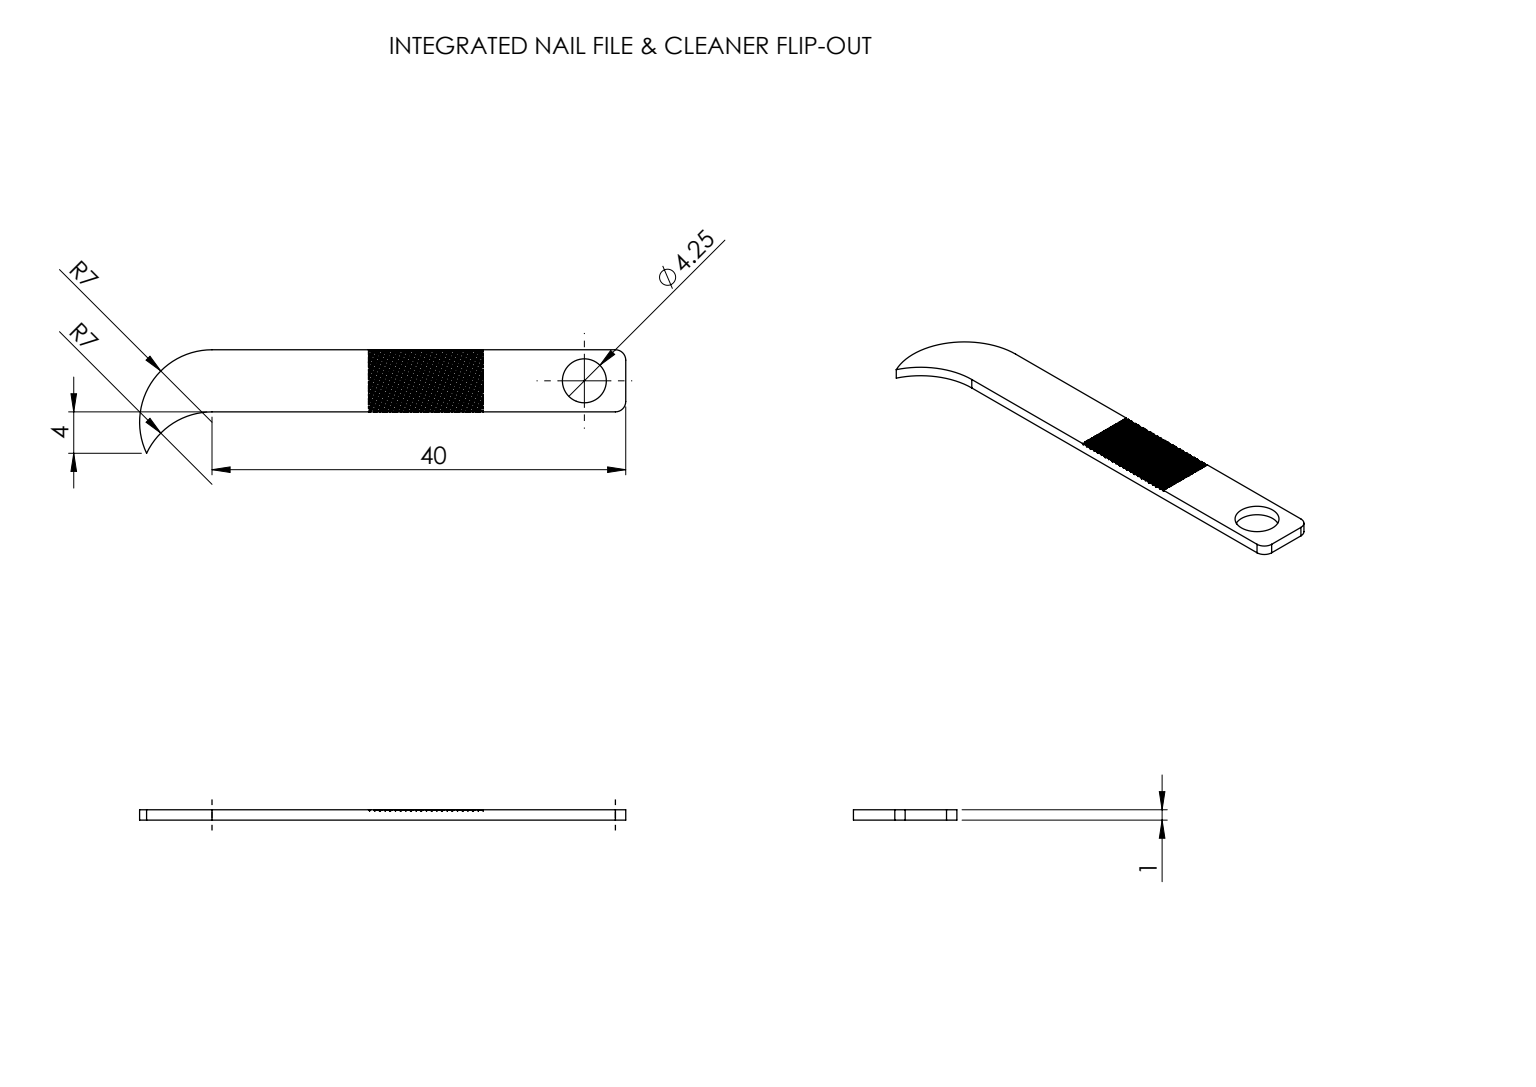
ISO-10303-21;
HEADER;
FILE_DESCRIPTION (('STEP AP214'),
    '1' );
FILE_NAME ('Integrated Nail File & Cleaner Flip-Out.step',
    '2026-09-30T04:43:20',
    ( '' ),
    ( '' ),
    'SwSTEP 2.0',
    'SolidWorks 2026',
    '' );
FILE_SCHEMA (( 'AUTOMOTIVE_DESIGN' ));
ENDSEC;

DATA;
#1=LINE ( 'NONE', #25573, #52192 ) ;
#2=VERTEX_POINT ( 'NONE', #10749 ) ;
#5=EDGE_CURVE ( 'NONE', #33225, #52332, #37701, .T. ) ;
#6=ORIENTED_EDGE ( 'NONE', *, *, #640, .F. ) ;
#7=FACE_OUTER_BOUND ( 'NONE', #50203, .T. ) ;
#8=ORIENTED_EDGE ( 'NONE', *, *, #49782, .T. ) ;
#9=DIRECTION ( 'NONE',  ( 0.7660212471507180654, -0.6427876096865404731, 0.005961354470445141482 ) ) ;
#10=EDGE_CURVE ( 'NONE', #34917, #49361, #53883, .T. ) ;
#11=ORIENTED_EDGE ( 'NONE', *, *, #22264, .F. ) ;
#12=ORIENTED_EDGE ( 'NONE', *, *, #56053, .T. ) ;
#13=ORIENTED_EDGE ( 'NONE', *, *, #9607, .F. ) ;
#14=DIRECTION ( 'NONE',  ( -0.6427681459581293666, -0.7660444431189770143, -0.005002170337467561935 ) ) ;
#15=CARTESIAN_POINT ( 'NONE',  ( -14.94838282604900748, -0.1191753592594197858, 2.588085963191248506 ) ) ;
#16=FACE_OUTER_BOUND ( 'NONE', #22473, .T. ) ;
#17=CARTESIAN_POINT ( 'NONE',  ( -15.43471928309396013, -0.1191753592594189115, 4.430961529461709070 ) ) ;
#19=ORIENTED_EDGE ( 'NONE', *, *, #1841, .F. ) ;
#20=ORIENTED_EDGE ( 'NONE', *, *, #40291, .F. ) ;
#21=CARTESIAN_POINT ( 'NONE',  ( -27.06630483948590893, -0.1191753592594197858, 7.295098399573937797 ) ) ;
#22=EDGE_LOOP ( 'NONE', ( #47630, #41472, #34640 ) ) ;
#23=PLANE ( 'NONE',  #10320 ) ;
#24=ORIENTED_EDGE ( 'NONE', *, *, #10341, .T. ) ;
#25=LINE ( 'NONE', #55156, #19677 ) ;
#26=FACE_OUTER_BOUND ( 'NONE', #52687, .T. ) ;
#28=EDGE_LOOP ( 'NONE', ( #23520, #5098, #48877, #45921 ) ) ;
#29=DIRECTION ( 'NONE',  ( -0.005961354470445682716, -0.6427876096865404731, 0.7660212471507180654 ) ) ;
#30=EDGE_CURVE ( 'NONE', #53080, #21477, #45939, .T. ) ;
#31=VERTEX_POINT ( 'NONE', #49893 ) ;
#32=AXIS2_PLACEMENT_3D ( 'NONE', #18822, #46039, #24446 ) ;
#33=CARTESIAN_POINT ( 'NONE',  ( -8.975993561185934055, -0.1191753592594197858, 10.41700724906143982 ) ) ;
#34=EDGE_LOOP ( 'NONE', ( #54000, #22369, #27701, #44259 ) ) ;
#35=CARTESIAN_POINT ( 'NONE',  ( -12.70458494993575194, -0.1191753592594197858, 11.86531876794841978 ) ) ;
#36=FACE_OUTER_BOUND ( 'NONE', #31619, .T. ) ;
#37=CARTESIAN_POINT ( 'NONE',  ( -13.73672976910459909, 0.000000000000000000, 12.22661844811216270 ) ) ;
#38=ORIENTED_EDGE ( 'NONE', *, *, #21938, .F. ) ;
#39=CARTESIAN_POINT ( 'NONE',  ( -16.82003048110239973, -0.1191753592594181482, 3.315097473835892039 ) ) ;
#40=CARTESIAN_POINT ( 'NONE',  ( -17.38829393498713571, 0.000000000000000000, 3.777097248297537124 ) ) ;
#41=DIRECTION ( 'NONE',  ( 0.007781995580012663651, -3.146120232559066537E-19, -0.9999697198139514409 ) ) ;
#42=CARTESIAN_POINT ( 'NONE',  ( -4.289188282875421088, -6.206962462949310755, 4.884439966179827231 ) ) ;
#43=CARTESIAN_POINT ( 'NONE',  ( -6.343177736738851102, -8.196582280829671774, 5.682279223835847937 ) ) ;
#44=LINE ( 'NONE', #33333, #46041 ) ;
#45=EDGE_CURVE ( 'NONE', #30649, #39352, #46465, .T. ) ;
#46=CARTESIAN_POINT ( 'NONE',  ( -17.46532115785441519, 0.000000000000000000, 13.67492996699914265 ) ) ;
#47=ORIENTED_EDGE ( 'NONE', *, *, #3666, .T. ) ;
#48=CARTESIAN_POINT ( 'NONE',  ( -10.21144203228149117, 0.000000000000000000, 2.894278973455366444 ) ) ;
#49=FACE_OUTER_BOUND ( 'NONE', #34512, .T. ) ;
#50=DIRECTION ( 'NONE',  ( -0.5449076811759708816, 0.6444004775717707689, 0.5364919789714475140 ) ) ;
#51=ORIENTED_EDGE ( 'NONE', *, *, #37599, .T. ) ;
#52=CARTESIAN_POINT ( 'NONE',  ( -19.46232870854519703, -3.756034771668159689, 10.40605410012864773 ) ) ;
#53=CARTESIAN_POINT ( 'NONE',  ( -14.22677752833734566, -0.3560938001956537868, 2.792505858709713795 ) ) ;
#54=ORIENTED_EDGE ( 'NONE', *, *, #55093, .T. ) ;
#55=DIRECTION ( 'NONE',  ( -0.005002170337468016433, -0.7660444431189770143, 0.6427681459581293666 ) ) ;
#56=AXIS2_PLACEMENT_3D ( 'NONE', #16443, #12198, #42577 ) ;
#57=EDGE_CURVE ( 'NONE', #19141, #38385, #32336, .T. ) ;
#58=LINE ( 'NONE', #52599, #10348 ) ;
#59=DIRECTION ( 'NONE',  ( 0.7660212471507180654, -0.6427876096865404731, 0.005961354470445141482 ) ) ;
#60=ADVANCED_FACE ( 'NONE', ( #15818 ), #6753, .F. ) ;
#62=ORIENTED_EDGE ( 'NONE', *, *, #8095, .T. ) ;
#64=PLANE ( 'NONE',  #40295 ) ;
#65=CARTESIAN_POINT ( 'NONE',  ( 2.072287782118878319, 0.000000000000000000, -2.950529333540147015 ) ) ;
#66=CARTESIAN_POINT ( 'NONE',  ( -10.20856797877621069, 0.000000000000000000, 2.524969270197602089 ) ) ;
#67=LINE ( 'NONE', #34732, #24784 ) ;
#68=EDGE_CURVE ( 'NONE', #2840, #34483, #50479, .T. ) ;
#69=LINE ( 'NONE', #17405, #45540 ) ;
#70=VECTOR ( 'NONE', #21292, 999.9999999999998863 ) ;
#71=FACE_OUTER_BOUND ( 'NONE', #956, .T. ) ;
#72=ORIENTED_EDGE ( 'NONE', *, *, #35043, .F. ) ;
#73=DIRECTION ( 'NONE',  ( -0.6427681459581293666, -0.7660444431189770143, -0.005002170337467561935 ) ) ;
#74=VECTOR ( 'NONE', #36543, 999.9999999999998863 ) ;
#75=ADVANCED_FACE ( 'NONE', ( #45360 ), #6472, .F. ) ;
#76=PLANE ( 'NONE',  #14275 ) ;
#77=EDGE_LOOP ( 'NONE', ( #29388, #6905, #15789, #43672 ) ) ;
#78=LINE ( 'NONE', #17411, #16572 ) ;
#79=LINE ( 'NONE', #52063, #49503 ) ;
#80=DIRECTION ( 'NONE',  ( 0.005002170337468016433, -0.7660444431189770143, -0.6427681459581293666 ) ) ;
#81=ORIENTED_EDGE ( 'NONE', *, *, #39049, .F. ) ;
#82=FACE_OUTER_BOUND ( 'NONE', #1972, .T. ) ;
#83=VERTEX_POINT ( 'NONE', #15002 ) ;
#84=ORIENTED_EDGE ( 'NONE', *, *, #47098, .T. ) ;
#85=ORIENTED_EDGE ( 'NONE', *, *, #23256, .T. ) ;
#86=ORIENTED_EDGE ( 'NONE', *, *, #47911, .T. ) ;
#87=DIRECTION ( 'NONE',  ( 0.005002170337468016433, -0.7660444431189770143, -0.6427681459581293666 ) ) ;
#88=ORIENTED_EDGE ( 'NONE', *, *, #42803, .T. ) ;
#90=DIRECTION ( 'NONE',  ( -0.5364919789714478471, 0.6444004775717705469, -0.5449076811759709926 ) ) ;
#91=AXIS2_PLACEMENT_3D ( 'NONE', #49933, #23822, #53928 ) ;
#92=VECTOR ( 'NONE', #28630, 1000.000000000000227 ) ;
#93=VERTEX_POINT ( 'NONE', #7584 ) ;
#94=CARTESIAN_POINT ( 'NONE',  ( -17.93139508144814442, 0.000000000000000000, 13.85596890686001537 ) ) ;
#95=ORIENTED_EDGE ( 'NONE', *, *, #27439, .T. ) ;
#96=CARTESIAN_POINT ( 'NONE',  ( -15.04104892662381054, -1.327505506330656670, 2.681420940547515563 ) ) ;
#97=EDGE_CURVE ( 'NONE', #51394, #16631, #45637, .T. ) ;
#98=VERTEX_POINT ( 'NONE', #19810 ) ;
#99=DIRECTION ( 'NONE',  ( -0.5449076811759708816, 0.6444004775717707689, 0.5364919789714475140 ) ) ;
#100=DIRECTION ( 'NONE',  ( 0.5449076811759707706, 0.6444004775717708799, -0.5364919789714476250 ) ) ;
#101=EDGE_CURVE ( 'NONE', #33893, #38385, #37132, .T. ) ;
#102=DIRECTION ( 'NONE',  ( 0.6427681459581294776, -0.7660444431189769032, 0.005002170337467562802 ) ) ;
#103=PLANE ( 'NONE',  #32324 ) ;
#104=DIRECTION ( 'NONE',  ( 0.9999697198139515519, 0.000000000000000000, 0.007781995580013368816 ) ) ;
#105=ORIENTED_EDGE ( 'NONE', *, *, #27186, .T. ) ;
#107=EDGE_CURVE ( 'NONE', #29873, #51521, #8427, .T. ) ;
#108=ADVANCED_FACE ( 'NONE', ( #21512 ), #30012, .F. ) ;
#109=ORIENTED_EDGE ( 'NONE', *, *, #25096, .F. ) ;
#110=DIRECTION ( 'NONE',  ( 0.005961354470445682716, -0.6427876096865404731, -0.7660212471507180654 ) ) ;
#111=PLANE ( 'NONE',  #41200 ) ;
#112=AXIS2_PLACEMENT_3D ( 'NONE', #46198, #6762, #45366 ) ;
#113=DIRECTION ( 'NONE',  ( 0.007781995580012663651, -3.146120232559066537E-19, -0.9999697198139514409 ) ) ;
#114=DIRECTION ( 'NONE',  ( -0.7660212471507179544, -0.6427876096865405842, -0.005961354470445141482 ) ) ;
#115=CARTESIAN_POINT ( 'NONE',  ( -12.13851405436063047, 0.000000000000000000, 11.68505802764555135 ) ) ;
#116=CARTESIAN_POINT ( 'NONE',  ( -18.13769215924349965, 0.000000000000000000, 6.356589746681873265 ) ) ;
#117=ORIENTED_EDGE ( 'NONE', *, *, #25709, .T. ) ;
#118=LINE ( 'NONE', #12391, #16607 ) ;
#119=CARTESIAN_POINT ( 'NONE',  ( -17.52554100038571860, -1.489407457353157049, 5.933818405385602013 ) ) ;
#120=ORIENTED_EDGE ( 'NONE', *, *, #23665, .T. ) ;
#121=DIRECTION ( 'NONE',  ( 0.5449076811759707706, 0.6444004775717708799, -0.5364919789714476250 ) ) ;
#122=LINE ( 'NONE', #21472, #18778 ) ;
#123=ADVANCED_FACE ( 'NONE', ( #38236 ), #25209, .F. ) ;
#124=DIRECTION ( 'NONE',  ( -0.7660212471507179544, -0.6427876096865405842, -0.005961354470445141482 ) ) ;
#125=FACE_OUTER_BOUND ( 'NONE', #27340, .T. ) ;
#126=EDGE_CURVE ( 'NONE', #16128, #35650, #30301, .T. ) ;
#127=LINE ( 'NONE', #17465, #18341 ) ;
#129=EDGE_LOOP ( 'NONE', ( #42984, #52877, #43620, #27077 ) ) ;
#130=EDGE_CURVE ( 'NONE', #30420, #39913, #56138, .T. ) ;
#131=DIRECTION ( 'NONE',  ( 0.007781995580012663651, 0.000000000000000000, -0.9999697198139515519 ) ) ;
#133=DIRECTION ( 'NONE',  ( -0.5449076811759708816, 0.6444004775717707689, 0.5364919789714475140 ) ) ;
#134=AXIS2_PLACEMENT_3D ( 'NONE', #24885, #20335, #55533 ) ;
#135=EDGE_CURVE ( 'NONE', #41809, #20314, #43076, .T. ) ;
#136=AXIS2_PLACEMENT_3D ( 'NONE', #8040, #24490, #3201 ) ;
#137=DIRECTION ( 'NONE',  ( 0.9999697198139515519, 0.000000000000000000, 0.007781995580013368816 ) ) ;
#138=DIRECTION ( 'NONE',  ( 0.007781995580012663651, 0.000000000000000000, -0.9999697198139515519 ) ) ;
#139=CARTESIAN_POINT ( 'NONE',  ( -18.03530320978490664, 0.7721120973665048792, 3.662821561289850703 ) ) ;
#140=DIRECTION ( 'NONE',  ( 0.5364919789714477361, 0.6444004775717706579, 0.5449076811759711036 ) ) ;
#141=EDGE_CURVE ( 'NONE', #45048, #20126, #4465, .T. ) ;
#142=EDGE_LOOP ( 'NONE', ( #43408, #23853, #54595 ) ) ;
#143=DIRECTION ( 'NONE',  ( 0.5449076811759707706, 0.6444004775717708799, -0.5364919789714476250 ) ) ;
#144=CARTESIAN_POINT ( 'NONE',  ( -12.60458797795435615, 0.000000000000000000, 11.86609696750642229 ) ) ;
#146=ORIENTED_EDGE ( 'NONE', *, *, #35409, .F. ) ;
#147=LINE ( 'NONE', #43889, #14715 ) ;
#148=ORIENTED_EDGE ( 'NONE', *, *, #30639, .T. ) ;
#149=DIRECTION ( 'NONE',  ( 0.007781995580012663651, 0.000000000000000000, -0.9999697198139515519 ) ) ;
#150=DIRECTION ( 'NONE',  ( 0.005961354470445682716, -0.6427876096865404731, -0.7660212471507180654 ) ) ;
#151=ORIENTED_EDGE ( 'NONE', *, *, #26951, .F. ) ;
#152=AXIS2_PLACEMENT_3D ( 'NONE', #22680, #53358, #9066 ) ;
#153=ORIENTED_EDGE ( 'NONE', *, *, #46826, .T. ) ;
#154=VECTOR ( 'NONE', #54316, 999.9999999999998863 ) ;
#155=ORIENTED_EDGE ( 'NONE', *, *, #18719, .T. ) ;
#156=VERTEX_POINT ( 'NONE', #55864 ) ;
#157=ORIENTED_EDGE ( 'NONE', *, *, #3395, .T. ) ;
#158=EDGE_LOOP ( 'NONE', ( #12558, #55338, #5576, #52336 ) ) ;
#159=LINE ( 'NONE', #30004, #37792 ) ;
#160=DIRECTION ( 'NONE',  ( -0.5364919789714478471, 0.6444004775717705469, -0.5449076811759709926 ) ) ;
#161=LINE ( 'NONE', #43615, #10427 ) ;
#162=ORIENTED_EDGE ( 'NONE', *, *, #35168, .T. ) ;
#163=DIRECTION ( 'NONE',  ( 0.9999697198139515519, 0.000000000000000000, 0.007781995580013368816 ) ) ;
#164=ORIENTED_EDGE ( 'NONE', *, *, #30145, .F. ) ;
#165=VERTEX_POINT ( 'NONE', #25754 ) ;
#166=CARTESIAN_POINT ( 'NONE',  ( -28.92982233430281980, 0.000000000000000000, 7.919257187036034651 ) ) ;
#167=DIRECTION ( 'NONE',  ( 0.000000000000000000, -0.000000000000000000, -1.000000000000000000 ) ) ;
#168=PLANE ( 'NONE',  #1458 ) ;
#169=ORIENTED_EDGE ( 'NONE', *, *, #7771, .F. ) ;
#170=LINE ( 'NONE', #34552, #2862 ) ;
#171=VERTEX_POINT ( 'NONE', #17226 ) ;
#172=EDGE_CURVE ( 'NONE', #2345, #30417, #47903, .T. ) ;
#173=EDGE_CURVE ( 'NONE', #12870, #165, #47619, .T. ) ;
#174=VECTOR ( 'NONE', #52609, 999.9999999999998863 ) ;
#175=AXIS2_PLACEMENT_3D ( 'NONE', #29245, #50566, #11082 ) ;
#176=DIRECTION ( 'NONE',  ( -0.6246952433987893460, -0.7422098413412802076, 0.2426528472758542054 ) ) ;
#177=FACE_OUTER_BOUND ( 'NONE', #19384, .T. ) ;
#178=ADVANCED_FACE ( 'NONE', ( #38828 ), #34544, .F. ) ;
#179=PLANE ( 'NONE',  #54119 ) ;
#180=VECTOR ( 'NONE', #20646, 999.9999999999998863 ) ;
#181=VECTOR ( 'NONE', #8523, 999.9999999999998863 ) ;
#182=CARTESIAN_POINT ( 'NONE',  ( -13.92566315350489958, 0.000000000000000000, 2.496041976053526401 ) ) ;
#183=DIRECTION ( 'NONE',  ( 0.9999697198139515519, 0.000000000000000000, 0.007781995580013368816 ) ) ;
#184=PLANE ( 'NONE',  #4946 ) ;
#185=DIRECTION ( 'NONE',  ( 0.9999697198139515519, 0.000000000000000000, 0.007781995580013368816 ) ) ;
#187=VERTEX_POINT ( 'NONE', #9005 ) ;
#188=LINE ( 'NONE', #21229, #46462 ) ;
#189=LINE ( 'NONE', #16995, #9319 ) ;
#190=FACE_OUTER_BOUND ( 'NONE', #52164, .T. ) ;
#191=CARTESIAN_POINT ( 'NONE',  ( -10.67549210721878694, 8.288742281967422798, 0.9283501000179719131 ) ) ;
#194=DIRECTION ( 'NONE',  ( 0.000000000000000000, -0.000000000000000000, -1.000000000000000000 ) ) ;
#195=ADVANCED_FACE ( 'NONE', ( #42236 ), #20662, .F. ) ;
#196=DIRECTION ( 'NONE',  ( 0.005961354470445682716, -0.6427876096865404731, -0.7660212471507180654 ) ) ;
#197=DIRECTION ( 'NONE',  ( 0.5449076811759707706, 0.6444004775717708799, -0.5364919789714476250 ) ) ;
#199=ORIENTED_EDGE ( 'NONE', *, *, #4188, .F. ) ;
#200=ADVANCED_FACE ( 'NONE', ( #33997 ), #16371, .F. ) ;
#201=FACE_OUTER_BOUND ( 'NONE', #9129, .T. ) ;
#202=FACE_OUTER_BOUND ( 'NONE', #53678, .T. ) ;
#203=DIRECTION ( 'NONE',  ( 0.6427681459581294776, -0.7660444431189769032, 0.005002170337467562802 ) ) ;
#204=EDGE_CURVE ( 'NONE', #54577, #15326, #19532, .T. ) ;
#205=DIRECTION ( 'NONE',  ( 0.9999697198139515519, 0.000000000000000000, 0.007781995580013368816 ) ) ;
#206=CARTESIAN_POINT ( 'NONE',  ( -13.48976679171663484, 0.000000000000000000, 6.192754920399180740 ) ) ;
#207=VECTOR ( 'NONE', #19976, 1000.000000000000227 ) ;
#208=EDGE_CURVE ( 'NONE', #16268, #38932, #12121, .T. ) ;
#209=CARTESIAN_POINT ( 'NONE',  ( -15.52531589500150666, 0.000000000000000000, 3.222257248149021258 ) ) ;
#211=CARTESIAN_POINT ( 'NONE',  ( -19.32961685222932147, 0.000000000000000000, 14.39908572644263351 ) ) ;
#212=CARTESIAN_POINT ( 'NONE',  ( -17.36187534420177769, 4.333955019861509328, 10.73802165171122347 ) ) ;
#213=EDGE_CURVE ( 'NONE', #291, #19762, #47053, .T. ) ;
#214=AXIS2_PLACEMENT_3D ( 'NONE', #5223, #35051, #73 ) ;
#215=EDGE_LOOP ( 'NONE', ( #36869, #50678, #13094, #16447 ) ) ;
#216=DIRECTION ( 'NONE',  ( 0.5364919789714477361, 0.6444004775717706579, 0.5449076811759711036 ) ) ;
#217=EDGE_CURVE ( 'NONE', #7467, #3951, #3878, .T. ) ;
#218=VECTOR ( 'NONE', #12479, 1000.000000000000227 ) ;
#219=AXIS2_PLACEMENT_3D ( 'NONE', #34025, #46802, #8180 ) ;
#220=EDGE_LOOP ( 'NONE', ( #56199, #45802, #49366, #38955 ) ) ;
#221=ADVANCED_FACE ( 'NONE', ( #13537 ), #1011, .F. ) ;
#222=VECTOR ( 'NONE', #40260, 1000.000000000000227 ) ;
#223=VERTEX_POINT ( 'NONE', #1301 ) ;
#224=EDGE_LOOP ( 'NONE', ( #49282, #54509, #50774, #34578 ) ) ;
#225=AXIS2_PLACEMENT_3D ( 'NONE', #48781, #44235, #9876 ) ;
#226=ORIENTED_EDGE ( 'NONE', *, *, #56206, .F. ) ;
#227=ORIENTED_EDGE ( 'NONE', *, *, #29291, .F. ) ;
#228=CARTESIAN_POINT ( 'NONE',  ( -14.01701317841955508, 0.000000000000000000, 2.326005055450897085 ) ) ;
#229=DIRECTION ( 'NONE',  ( -0.005961354470445682716, -0.6427876096865404731, 0.7660212471507180654 ) ) ;
#230=ORIENTED_EDGE ( 'NONE', *, *, #6847, .F. ) ;
#231=ORIENTED_EDGE ( 'NONE', *, *, #14544, .F. ) ;
#232=VECTOR ( 'NONE', #3897, 1000.000000000000227 ) ;
#233=AXIS2_PLACEMENT_3D ( 'NONE', #39851, #932, #52902 ) ;
#234=LINE ( 'NONE', #25830, #10239 ) ;
#235=VERTEX_POINT ( 'NONE', #4730 ) ;
#236=CARTESIAN_POINT ( 'NONE',  ( -18.67619601524082285, 0.000000000000000000, 3.936400510096834893 ) ) ;
#238=ORIENTED_EDGE ( 'NONE', *, *, #26646, .F. ) ;
#239=FACE_OUTER_BOUND ( 'NONE', #22439, .T. ) ;
#240=AXIS2_PLACEMENT_3D ( 'NONE', #41868, #37631, #6419 ) ;
#241=EDGE_CURVE ( 'NONE', #29572, #36873, #1603, .T. ) ;
#242=ORIENTED_EDGE ( 'NONE', *, *, #47787, .F. ) ;
#243=DIRECTION ( 'NONE',  ( 0.000000000000000000, -1.000000000000000000, 0.000000000000000000 ) ) ;
#244=VECTOR ( 'NONE', #39775, 1000.000000000000114 ) ;
#245=EDGE_CURVE ( 'NONE', #18842, #26839, #48755, .T. ) ;
#246=EDGE_CURVE ( 'NONE', #931, #21351, #36247, .T. ) ;
#247=CARTESIAN_POINT ( 'NONE',  ( -13.46034487804917390, 5.305366725996514710, 1.741117822157838724 ) ) ;
#248=EDGE_LOOP ( 'NONE', ( #22673, #25406, #16303, #10944 ) ) ;
#249=PLANE ( 'NONE',  #50315 ) ;
#250=CARTESIAN_POINT ( 'NONE',  ( -14.17032429916292813, 0.000000000000000000, 8.234125069766777827 ) ) ;
#251=CARTESIAN_POINT ( 'NONE',  ( -11.20636620717317378, 0.000000000000000000, 11.32298014792380414 ) ) ;
#252=VECTOR ( 'NONE', #13641, 999.9999999999998863 ) ;
#254=CARTESIAN_POINT ( 'NONE',  ( -23.33849165029409889, 0.000000000000000000, 5.946783852668351855 ) ) ;
#255=ORIENTED_EDGE ( 'NONE', *, *, #35065, .T. ) ;
#256=VECTOR ( 'NONE', #15844, 1000.000000000000227 ) ;
#257=AXIS2_PLACEMENT_3D ( 'NONE', #26686, #13372, #44005 ) ;
#258=DIRECTION ( 'NONE',  ( -0.6427681459581293666, -0.7660444431189770143, -0.005002170337467561935 ) ) ;
#259=LINE ( 'NONE', #22700, #51384 ) ;
#260=DIRECTION ( 'NONE',  ( -0.9999697198139514409, -0.000000000000000000, -0.007781995580013368816 ) ) ;
#261=DIRECTION ( 'NONE',  ( -0.6427681459581293666, -0.7660444431189770143, -0.005002170337467561935 ) ) ;
#262=PLANE ( 'NONE',  #7783 ) ;
#263=CARTESIAN_POINT ( 'NONE',  ( -18.19747506107908563, 0.000000000000000000, 14.03856424583689311 ) ) ;
#264=DIRECTION ( 'NONE',  ( -0.7660212471507179544, -0.6427876096865405842, -0.005961354470445141482 ) ) ;
#265=AXIS2_PLACEMENT_3D ( 'NONE', #36413, #10611, #26789 ) ;
#266=DIRECTION ( 'NONE',  ( 0.000000000000000000, -0.000000000000000000, -1.000000000000000000 ) ) ;
#267=VECTOR ( 'NONE', #8315, 999.9999999999998863 ) ;
#268=CARTESIAN_POINT ( 'NONE',  ( -23.33771345073609638, -0.1191753592594197858, 5.846786880686956955 ) ) ;
#269=ORIENTED_EDGE ( 'NONE', *, *, #16189, .T. ) ;
#270=DIRECTION ( 'NONE',  ( -0.005002170337468016433, -0.7660444431189770143, 0.6427681459581293666 ) ) ;
#271=LINE ( 'NONE', #1112, #10920 ) ;
#272=CARTESIAN_POINT ( 'NONE',  ( 2.072287782118878319, 0.000000000000000000, -2.950529333540147015 ) ) ;
#273=CARTESIAN_POINT ( 'NONE',  ( -11.87243407472968926, 0.000000000000000000, 11.50246268866867361 ) ) ;
#274=AXIS2_PLACEMENT_3D ( 'NONE', #26963, #39157, #26121 ) ;
#275=AXIS2_PLACEMENT_3D ( 'NONE', #49131, #52299, #27016 ) ;
#276=EDGE_CURVE ( 'NONE', #2654, #52427, #22050, .T. ) ;
#277=FACE_OUTER_BOUND ( 'NONE', #5267, .T. ) ;
#278=CARTESIAN_POINT ( 'NONE',  ( -16.79925329029790149, 0.000000000000000000, 13.49544742625427496 ) ) ;
#279=ORIENTED_EDGE ( 'NONE', *, *, #9058, .T. ) ;
#281=EDGE_CURVE ( 'NONE', #14069, #52686, #39928, .T. ) ;
#282=DIRECTION ( 'NONE',  ( 0.005002170337468016433, -0.7660444431189770143, -0.6427681459581293666 ) ) ;
#283=CARTESIAN_POINT ( 'NONE',  ( -17.73140113748535285, 0.000000000000000000, 13.85752530597602039 ) ) ;
#284=ORIENTED_EDGE ( 'NONE', *, *, #29998, .F. ) ;
#285=VECTOR ( 'NONE', #53236, 1000.000000000000227 ) ;
#286=FACE_OUTER_BOUND ( 'NONE', #8165, .T. ) ;
#287=EDGE_LOOP ( 'NONE', ( #31043, #13115, #52818, #45322 ) ) ;
#288=CARTESIAN_POINT ( 'NONE',  ( -19.79569077582305070, 0.000000000000000000, 14.58012466630350445 ) ) ;
#289=EDGE_CURVE ( 'NONE', #36837, #44524, #470, .T. ) ;
#290=VECTOR ( 'NONE', #6881, 999.9999999999998863 ) ;
#291=VERTEX_POINT ( 'NONE', #9262 ) ;
#292=CARTESIAN_POINT ( 'NONE',  ( -18.44716714978218164, 2.876837460659007473, 8.768207690109344199 ) ) ;
#293=ORIENTED_EDGE ( 'NONE', *, *, #18760, .T. ) ;
#294=VERTEX_POINT ( 'NONE', #53546 ) ;
#295=ORIENTED_EDGE ( 'NONE', *, *, #8160, .T. ) ;
#296=CARTESIAN_POINT ( 'NONE',  ( -15.86710544311044302, 0.000000000000000000, 13.13336954653252953 ) ) ;
#297=VECTOR ( 'NONE', #13524, 1000.000000000000000 ) ;
#298=FACE_OUTER_BOUND ( 'NONE', #53215, .T. ) ;
#300=EDGE_CURVE ( 'NONE', #33548, #11209, #18927, .T. ) ;
#301=AXIS2_PLACEMENT_3D ( 'NONE', #8298, #21377, #55722 ) ;
#302=VECTOR ( 'NONE', #4764, 999.9999999999998863 ) ;
#303=DIRECTION ( 'NONE',  ( 0.007781995580012663651, 0.000000000000000000, -0.9999697198139515519 ) ) ;
#304=EDGE_LOOP ( 'NONE', ( #25150, #34611, #28054, #8360, #39695 ) ) ;
#305=ORIENTED_EDGE ( 'NONE', *, *, #38261, .F. ) ;
#306=EDGE_CURVE ( 'NONE', #53467, #42919, #52440, .T. ) ;
#307=VECTOR ( 'NONE', #12261, 1000.000000000000114 ) ;
#308=VERTEX_POINT ( 'NONE', #35146 ) ;
#309=VECTOR ( 'NONE', #14747, 999.9999999999998863 ) ;
#311=DIRECTION ( 'NONE',  ( 0.9999697198139515519, 0.000000000000000000, 0.007781995580013368816 ) ) ;
#312=ORIENTED_EDGE ( 'NONE', *, *, #31310, .T. ) ;
#313=DIRECTION ( 'NONE',  ( 0.000000000000000000, -0.000000000000000000, -1.000000000000000000 ) ) ;
#314=EDGE_CURVE ( 'NONE', #9163, #26799, #27158, .T. ) ;
#315=ORIENTED_EDGE ( 'NONE', *, *, #40972, .T. ) ;
#316=PLANE ( 'NONE',  #44171 ) ;
#317=LINE ( 'NONE', #31273, #54806 ) ;
#318=ORIENTED_EDGE ( 'NONE', *, *, #12951, .T. ) ;
#319=EDGE_CURVE ( 'NONE', #50963, #26160, #44464, .T. ) ;
#320=CARTESIAN_POINT ( 'NONE',  ( -27.99767448711536133, 0.000000000000000000, 7.557179307314289218 ) ) ;
#321=ORIENTED_EDGE ( 'NONE', *, *, #1045, .T. ) ;
#322=EDGE_CURVE ( 'NONE', #38023, #19674, #26588, .T. ) ;
#323=LINE ( 'NONE', #12572, #26385 ) ;
#324=VECTOR ( 'NONE', #8090, 1000.000000000000227 ) ;
#325=ORIENTED_EDGE ( 'NONE', *, *, #12524, .F. ) ;
#326=CARTESIAN_POINT ( 'NONE',  ( -20.54049170961573267, 0.000000000000000000, 4.660556269540326646 ) ) ;
#327=CARTESIAN_POINT ( 'NONE',  ( -17.33634854152196780, -0.1191753592594171213, 9.952400094065581015 ) ) ;
#328=DIRECTION ( 'NONE',  ( 0.6427681459581294776, -0.7660444431189769032, 0.005002170337467562802 ) ) ;
#329=VERTEX_POINT ( 'NONE', #5025 ) ;
#330=VECTOR ( 'NONE', #29769, 999.9999999999998863 ) ;
#331=EDGE_CURVE ( 'NONE', #20000, #39753, #13803, .T. ) ;
#332=LINE ( 'NONE', #21661, #54656 ) ;
#333=CARTESIAN_POINT ( 'NONE',  ( -17.75117697256323268, -2.298917212465658277, 7.350006499361532164 ) ) ;
#334=CARTESIAN_POINT ( 'NONE',  ( -17.36532418587302473, -0.1191753592594177458, 13.67570816655714516 ) ) ;
#335=VECTOR ( 'NONE', #1032, 999.9999999999998863 ) ;
#336=LINE ( 'NONE', #47792, #17706 ) ;
#337=LINE ( 'NONE', #39552, #37612 ) ;
#338=DIRECTION ( 'NONE',  ( 0.9999697198139515519, 0.000000000000000000, 0.007781995580013368816 ) ) ;
#340=DIRECTION ( 'NONE',  ( -0.7660212471507179544, -0.6427876096865405842, -0.005961354470445141482 ) ) ;
#341=ORIENTED_EDGE ( 'NONE', *, *, #38336, .T. ) ;
#342=CARTESIAN_POINT ( 'NONE',  ( 2.072287782118878319, 0.000000000000000000, -2.950529333540147015 ) ) ;
#343=LINE ( 'NONE', #21391, #3196 ) ;
#344=DIRECTION ( 'NONE',  ( 0.007781995580012662783, 0.000000000000000000, -0.9999697198139514409 ) ) ;
#345=VERTEX_POINT ( 'NONE', #31128 ) ;
#346=VECTOR ( 'NONE', #15392, 999.9999999999998863 ) ;
#347=DIRECTION ( 'NONE',  ( 0.7660212471507180654, -0.6427876096865404731, 0.005961354470445141482 ) ) ;
#348=FACE_OUTER_BOUND ( 'NONE', #54993, .T. ) ;
#349=VERTEX_POINT ( 'NONE', #31706 ) ;
#350=VECTOR ( 'NONE', #2759, 999.9999999999998863 ) ;
#352=DIRECTION ( 'NONE',  ( 0.5449076811759707706, 0.6444004775717708799, -0.5364919789714476250 ) ) ;
#353=DIRECTION ( 'NONE',  ( 0.7660212471507180654, -0.6427876096865404731, 0.005961354470445141482 ) ) ;
#355=ORIENTED_EDGE ( 'NONE', *, *, #29279, .T. ) ;
#356=VECTOR ( 'NONE', #10520, 1000.000000000000114 ) ;
#357=VECTOR ( 'NONE', #13768, 1000.000000000000000 ) ;
#358=ORIENTED_EDGE ( 'NONE', *, *, #4456, .T. ) ;
#359=CARTESIAN_POINT ( 'NONE',  ( -19.33878870862964305, -1.975113310420658852, 7.435271445270302593 ) ) ;
#360=DIRECTION ( 'NONE',  ( 0.007781995580012662783, 0.000000000000000000, -0.9999697198139514409 ) ) ;
#361=DIRECTION ( 'NONE',  ( -0.9999697198139514409, -0.000000000000000000, -0.007781995580013368816 ) ) ;
#362=PLANE ( 'NONE',  #37468 ) ;
#363=DIRECTION ( 'NONE',  ( 0.5449076811759707706, 0.6444004775717708799, -0.5364919789714476250 ) ) ;
#364=FACE_OUTER_BOUND ( 'NONE', #14108, .T. ) ;
#365=EDGE_CURVE ( 'NONE', #15522, #6083, #49011, .T. ) ;
#367=LINE ( 'NONE', #4924, #1109 ) ;
#368=VECTOR ( 'NONE', #37920, 1000.000000000000227 ) ;
#370=VERTEX_POINT ( 'NONE', #48452 ) ;
#371=AXIS2_PLACEMENT_3D ( 'NONE', #6600, #33303, #28757 ) ;
#372=DIRECTION ( 'NONE',  ( 0.005961354470445682716, -0.6427876096865404731, -0.7660212471507180654 ) ) ;
#374=AXIS2_PLACEMENT_3D ( 'NONE', #30248, #4416, #8373 ) ;
#375=LINE ( 'NONE', #930, #8550 ) ;
#376=EDGE_CURVE ( 'NONE', #36173, #27809, #10111, .T. ) ;
#377=ORIENTED_EDGE ( 'NONE', *, *, #20121, .F. ) ;
#378=PLANE ( 'NONE',  #3086 ) ;
#379=VECTOR ( 'NONE', #26653, 1000.000000000000114 ) ;
#380=ORIENTED_EDGE ( 'NONE', *, *, #23171, .F. ) ;
#381=EDGE_CURVE ( 'NONE', #34243, #38141, #26893, .T. ) ;
#382=ADVANCED_FACE ( 'NONE', ( #5312 ), #20295, .F. ) ;
#383=ORIENTED_EDGE ( 'NONE', *, *, #43761, .F. ) ;
#384=EDGE_LOOP ( 'NONE', ( #49839, #18862, #38770, #29467 ) ) ;
#385=ORIENTED_EDGE ( 'NONE', *, *, #20357, .F. ) ;
#386=VECTOR ( 'NONE', #38602, 999.9999999999998863 ) ;
#387=PLANE ( 'NONE',  #36628 ) ;
#388=ORIENTED_EDGE ( 'NONE', *, *, #50925, .F. ) ;
#389=CARTESIAN_POINT ( 'NONE',  ( -18.35912213213254773, 0.000000000000000000, 9.109517029665196830 ) ) ;
#390=VECTOR ( 'NONE', #55175, 999.9999999999998863 ) ;
#391=ORIENTED_EDGE ( 'NONE', *, *, #38213, .F. ) ;
#392=LINE ( 'NONE', #30530, #43118 ) ;
#393=EDGE_CURVE ( 'NONE', #50596, #19103, #2684, .T. ) ;
#394=VERTEX_POINT ( 'NONE', #27729 ) ;
#395=DIRECTION ( 'NONE',  ( 0.8531650599175527594, 0.4028455766673922356, -0.3313982828793700652 ) ) ;
#397=EDGE_CURVE ( 'NONE', #27291, #53062, #24006, .T. ) ;
#398=VECTOR ( 'NONE', #12673, 999.9999999999998863 ) ;
#399=VECTOR ( 'NONE', #24658, 1000.000000000000227 ) ;
#400=LINE ( 'NONE', #29953, #50150 ) ;
#401=LINE ( 'NONE', #38179, #16866 ) ;
#402=DIRECTION ( 'NONE',  ( -0.5449076811759708816, 0.6444004775717707689, 0.5364919789714475140 ) ) ;
#403=CARTESIAN_POINT ( 'NONE',  ( -26.13337879274045505, 0.000000000000000000, 6.833023547870798353 ) ) ;
#404=DIRECTION ( 'NONE',  ( 0.5449076811759707706, 0.6444004775717708799, -0.5364919789714476250 ) ) ;
#405=ORIENTED_EDGE ( 'NONE', *, *, #31844, .T. ) ;
#406=EDGE_CURVE ( 'NONE', #17338, #35631, #37331, .T. ) ;
#407=ORIENTED_EDGE ( 'NONE', *, *, #12412, .F. ) ;
#408=PLANE ( 'NONE',  #43098 ) ;
#409=LINE ( 'NONE', #47855, #23972 ) ;
#410=FACE_OUTER_BOUND ( 'NONE', #52245, .T. ) ;
#411=VECTOR ( 'NONE', #55065, 1000.000000000000227 ) ;
#412=ADVANCED_FACE ( 'NONE', ( #32269 ), #15751, .F. ) ;
#413=CARTESIAN_POINT ( 'NONE',  ( -11.79828090536769203, 0.000000000000000000, 1.973939673224830660 ) ) ;
#414=AXIS2_PLACEMENT_3D ( 'NONE', #46926, #25913, #21902 ) ;
#415=DIRECTION ( 'NONE',  ( 0.007781995580012662783, 0.000000000000000000, -0.9999697198139514409 ) ) ;
#416=DIRECTION ( 'NONE',  ( 0.005002170337468016433, -0.7660444431189770143, -0.6427681459581293666 ) ) ;
#417=ORIENTED_EDGE ( 'NONE', *, *, #24919, .T. ) ;
#419=DIRECTION ( 'NONE',  ( 0.007781995580012663651, -3.146120232559066537E-19, -0.9999697198139514409 ) ) ;
#420=AXIS2_PLACEMENT_3D ( 'NONE', #54266, #23873, #24706 ) ;
#421=ORIENTED_EDGE ( 'NONE', *, *, #9837, .T. ) ;
#422=DIRECTION ( 'NONE',  ( -0.7660212471507179544, -0.6427876096865405842, -0.005961354470445141482 ) ) ;
#423=CARTESIAN_POINT ( 'NONE',  ( -27.99845268667336384, -0.1191753592594197858, 7.657176279295684118 ) ) ;
#424=VECTOR ( 'NONE', #53367, 1000.000000000000227 ) ;
#425=LINE ( 'NONE', #973, #5079 ) ;
#426=FACE_OUTER_BOUND ( 'NONE', #14338, .T. ) ;
#427=CARTESIAN_POINT ( 'NONE',  ( -14.15727168602579766, 0.000000000000000000, 6.556892312772929721 ) ) ;
#428=VERTEX_POINT ( 'NONE', #28541 ) ;
#429=VECTOR ( 'NONE', #53252, 999.9999999999998863 ) ;
#430=ORIENTED_EDGE ( 'NONE', *, *, #18527, .F. ) ;
#431=AXIS2_PLACEMENT_3D ( 'NONE', #56006, #3733, #42926 ) ;
#432=CARTESIAN_POINT ( 'NONE',  ( -11.26448342554532012, -0.1191753592594185784, 5.940743548404852525 ) ) ;
#434=LINE ( 'NONE', #30827, #44226 ) ;
#435=AXIS2_PLACEMENT_3D ( 'NONE', #40606, #36325, #43706 ) ;
#436=CARTESIAN_POINT ( 'NONE',  ( -13.73672976910459909, 0.000000000000000000, 12.22661844811216270 ) ) ;
#437=DIRECTION ( 'NONE',  ( 0.6427681459581294776, -0.7660444431189769032, 0.005002170337467562802 ) ) ;
#438=EDGE_CURVE ( 'NONE', #41253, #2345, #2131, .T. ) ;
#439=DIRECTION ( 'NONE',  ( -0.5449076811759708816, 0.6444004775717707689, 0.5364919789714475140 ) ) ;
#440=CARTESIAN_POINT ( 'NONE',  ( -27.06552663992790997, 0.000000000000000000, 7.195101427592543786 ) ) ;
#441=VERTEX_POINT ( 'NONE', #46137 ) ;
#442=VECTOR ( 'NONE', #33608, 999.9999999999998863 ) ;
#443=FACE_OUTER_BOUND ( 'NONE', #30904, .T. ) ;
#444=VECTOR ( 'NONE', #34245, 1000.000000000000000 ) ;
#445=LINE ( 'NONE', #48427, #46891 ) ;
#447=EDGE_CURVE ( 'NONE', #485, #27823, #40779, .T. ) ;
#448=ORIENTED_EDGE ( 'NONE', *, *, #34618, .F. ) ;
#449=CARTESIAN_POINT ( 'NONE',  ( -16.04172443374966761, 4.495856970884011261, 2.769640905047572321 ) ) ;
#450=EDGE_LOOP ( 'NONE', ( #19965, #9347, #24938, #27730 ) ) ;
#451=DIRECTION ( 'NONE',  ( 0.9321478471874541372, 0.000000000000000000, -0.3620778797217453771 ) ) ;
#452=ADVANCED_FACE ( 'NONE', ( #1852 ), #50104, .F. ) ;
#453=ADVANCED_FACE ( 'NONE', ( #7244 ), #2428, .F. ) ;
#454=LINE ( 'NONE', #35131, #43843 ) ;
#456=ORIENTED_EDGE ( 'NONE', *, *, #13239, .F. ) ;
#457=ORIENTED_EDGE ( 'NONE', *, *, #32580, .T. ) ;
#458=EDGE_CURVE ( 'NONE', #51710, #23249, #53825, .T. ) ;
#459=VECTOR ( 'NONE', #16090, 1000.000000000000114 ) ;
#461=ORIENTED_EDGE ( 'NONE', *, *, #35316, .F. ) ;
#462=ORIENTED_EDGE ( 'NONE', *, *, #15003, .T. ) ;
#463=AXIS2_PLACEMENT_3D ( 'NONE', #24547, #54121, #23720 ) ;
#464=ORIENTED_EDGE ( 'NONE', *, *, #30689, .T. ) ;
#465=DIRECTION ( 'NONE',  ( -0.005002170337468016433, -0.7660444431189770143, 0.6427681459581293666 ) ) ;
#466=CARTESIAN_POINT ( 'NONE',  ( 2.072287782118878319, 0.000000000000000000, -2.950529333540147015 ) ) ;
#467=DIRECTION ( 'NONE',  ( 0.007781995580012663651, -3.146120232559066537E-19, -0.9999697198139514409 ) ) ;
#468=AXIS2_PLACEMENT_3D ( 'NONE', #39473, #17904, #31219 ) ;
#469=EDGE_LOOP ( 'NONE', ( #53568, #47753, #23192, #24265 ) ) ;
#470=LINE ( 'NONE', #52994, #35822 ) ;
#471=EDGE_CURVE ( 'NONE', #12574, #40953, #33382, .T. ) ;
#472=ORIENTED_EDGE ( 'NONE', *, *, #19438, .F. ) ;
#473=AXIS2_PLACEMENT_3D ( 'NONE', #21788, #43922, #34860 ) ;
#474=EDGE_LOOP ( 'NONE', ( #13344, #7979, #54982, #50764 ) ) ;
#475=EDGE_CURVE ( 'NONE', #5277, #30292, #6413, .T. ) ;
#476=AXIS2_PLACEMENT_3D ( 'NONE', #44666, #26511, #49210 ) ;
#477=AXIS2_PLACEMENT_3D ( 'NONE', #5497, #53744, #35905 ) ;
#478=CARTESIAN_POINT ( 'NONE',  ( -16.79925329029790149, 0.000000000000000000, 13.49544742625427496 ) ) ;
#479=DIRECTION ( 'NONE',  ( -0.6427681459581293666, -0.7660444431189770143, -0.005002170337467561935 ) ) ;
#480=EDGE_CURVE ( 'NONE', #29959, #40913, #28257, .T. ) ;
#481=AXIS2_PLACEMENT_3D ( 'NONE', #37816, #3148, #21324 ) ;
#482=CARTESIAN_POINT ( 'NONE',  ( -17.46532115785441519, 0.000000000000000000, 13.67492996699914265 ) ) ;
#483=ORIENTED_EDGE ( 'NONE', *, *, #47027, .F. ) ;
#485=VERTEX_POINT ( 'NONE', #6690 ) ;
#486=VECTOR ( 'NONE', #22922, 1000.000000000000000 ) ;
#487=ADVANCED_FACE ( 'NONE', ( #41340 ), #54375, .F. ) ;
#488=VECTOR ( 'NONE', #16446, 1000.000000000000227 ) ;
#489=CARTESIAN_POINT ( 'NONE',  ( -9.274408763410345813, 2.384096728371167817, 3.117008339208958034 ) ) ;
#490=FACE_OUTER_BOUND ( 'NONE', #41737, .T. ) ;
#491=AXIS2_PLACEMENT_3D ( 'NONE', #51141, #37826, #24737 ) ;
#493=AXIS2_PLACEMENT_3D ( 'NONE', #21084, #8312, #42665 ) ;
#494=DIRECTION ( 'NONE',  ( 0.007781995580012663651, -3.146120232559066537E-19, -0.9999697198139514409 ) ) ;
#497=LINE ( 'NONE', #34563, #49322 ) ;
#498=CARTESIAN_POINT ( 'NONE',  ( -16.43317633868556626, -0.1191753592594197858, 13.31363028683540151 ) ) ;
#499=ORIENTED_EDGE ( 'NONE', *, *, #29532, .F. ) ;
#500=CARTESIAN_POINT ( 'NONE',  ( -16.81190032086591302, 0.000000000000000000, 3.212244750653343583 ) ) ;
#501=LINE ( 'NONE', #50440, #2942 ) ;
#502=CARTESIAN_POINT ( 'NONE',  ( -8.129252104341238905, 0.000000000000000000, 6.065145671608219935 ) ) ;
#503=DIRECTION ( 'NONE',  ( -0.7660212471507179544, -0.6427876096865405842, -0.005961354470445141482 ) ) ;
#504=DIRECTION ( 'NONE',  ( 0.000000000000000000, -0.000000000000000000, -1.000000000000000000 ) ) ;
#505=LINE ( 'NONE', #40549, #49453 ) ;
#506=LINE ( 'NONE', #14144, #19589 ) ;
#507=AXIS2_PLACEMENT_3D ( 'NONE', #4307, #52278, #48266 ) ;
#508=LINE ( 'NONE', #12467, #14837 ) ;
#509=VECTOR ( 'NONE', #35497, 999.9999999999998863 ) ;
#510=ORIENTED_EDGE ( 'NONE', *, *, #7779, .T. ) ;
#511=DIRECTION ( 'NONE',  ( 0.005002170337468016433, -0.7660444431189770143, -0.6427681459581293666 ) ) ;
#512=DIRECTION ( 'NONE',  ( -0.7660212471507179544, -0.6427876096865405842, -0.005961354470445141482 ) ) ;
#513=CARTESIAN_POINT ( 'NONE',  ( -11.87243407472968926, 0.000000000000000000, 11.50246268866867361 ) ) ;
#514=AXIS2_PLACEMENT_3D ( 'NONE', #20814, #20245, #54594 ) ;
#515=DIRECTION ( 'NONE',  ( 0.6427681459581294776, -0.7660444431189769032, 0.005002170337467562802 ) ) ;
#516=AXIS2_PLACEMENT_3D ( 'NONE', #41205, #19635, #11091 ) ;
#517=DIRECTION ( 'NONE',  ( 0.5449076811759707706, 0.6444004775717708799, -0.5364919789714476250 ) ) ;
#519=DIRECTION ( 'NONE',  ( 0.007781995580012662783, 0.000000000000000000, -0.9999697198139514409 ) ) ;
#520=DIRECTION ( 'NONE',  ( -0.5449076811759708816, 0.6444004775717707689, 0.5364919789714475140 ) ) ;
#521=AXIS2_PLACEMENT_3D ( 'NONE', #2355, #53746, #14865 ) ;
#522=EDGE_CURVE ( 'NONE', #20635, #3861, #4114, .T. ) ;
#523=FACE_OUTER_BOUND ( 'NONE', #1524, .T. ) ;
#524=VECTOR ( 'NONE', #3188, 999.9999999999998863 ) ;
#525=DIRECTION ( 'NONE',  ( 0.007781995580012663651, 0.000000000000000000, -0.9999697198139515519 ) ) ;
#526=EDGE_CURVE ( 'NONE', #25674, #51083, #56082, .T. ) ;
#527=VECTOR ( 'NONE', #10360, 1000.000000000000227 ) ;
#528=EDGE_CURVE ( 'NONE', #1446, #21707, #38460, .T. ) ;
#529=EDGE_CURVE ( 'NONE', #49849, #20973, #21442, .T. ) ;
#530=VERTEX_POINT ( 'NONE', #7826 ) ;
#532=VECTOR ( 'NONE', #47092, 1000.000000000000227 ) ;
#535=ORIENTED_EDGE ( 'NONE', *, *, #54295, .T. ) ;
#536=VECTOR ( 'NONE', #8972, 999.9999999999998863 ) ;
#537=ORIENTED_EDGE ( 'NONE', *, *, #7657, .T. ) ;
#538=ORIENTED_EDGE ( 'NONE', *, *, #30952, .T. ) ;
#539=ORIENTED_EDGE ( 'NONE', *, *, #36020, .F. ) ;
#540=DIRECTION ( 'NONE',  ( 0.000000000000000000, -1.000000000000000000, 0.000000000000000000 ) ) ;
#541=CARTESIAN_POINT ( 'NONE',  ( -29.86352658060627618, 0.000000000000000000, 8.481329010720569883 ) ) ;
#542=ORIENTED_EDGE ( 'NONE', *, *, #52767, .T. ) ;
#543=ORIENTED_EDGE ( 'NONE', *, *, #26233, .T. ) ;
#544=EDGE_CURVE ( 'NONE', #8877, #51526, #29948, .T. ) ;
#545=VECTOR ( 'NONE', #143, 1000.000000000000114 ) ;
#546=DIRECTION ( 'NONE',  ( 0.007781995580012663651, 0.000000000000000000, -0.9999697198139515519 ) ) ;
#547=VERTEX_POINT ( 'NONE', #50943 ) ;
#548=EDGE_CURVE ( 'NONE', #41034, #45002, #12631, .T. ) ;
#549=PLANE ( 'NONE',  #48198 ) ;
#550=CARTESIAN_POINT ( 'NONE',  ( -18.76354595665420177, -0.1191753592594177458, 14.21882498613976331 ) ) ;
#551=ORIENTED_EDGE ( 'NONE', *, *, #39784, .T. ) ;
#552=VECTOR ( 'NONE', #28211, 1000.000000000000227 ) ;
#553=CARTESIAN_POINT ( 'NONE',  ( 2.072287782118878319, 0.000000000000000000, -2.950529333540147015 ) ) ;
#554=EDGE_LOOP ( 'NONE', ( #27214, #4765, #35761, #21660 ) ) ;
#555=EDGE_CURVE ( 'NONE', #23263, #55993, #51792, .T. ) ;
#556=DIRECTION ( 'NONE',  ( 0.007781995580012662783, 0.000000000000000000, -0.9999697198139514409 ) ) ;
#557=VECTOR ( 'NONE', #29488, 999.9999999999998863 ) ;
#558=EDGE_CURVE ( 'NONE', #9839, #31046, #34234, .T. ) ;
#559=CARTESIAN_POINT ( 'NONE',  ( -16.72498074857254124, 0.000000000000000000, 3.951585318476526165 ) ) ;
#560=CARTESIAN_POINT ( 'NONE',  ( -12.14776819164751309, 3.686347215771509145, 7.649850626033056322 ) ) ;
#561=AXIS2_PLACEMENT_3D ( 'NONE', #36902, #10769, #32613 ) ;
#562=VECTOR ( 'NONE', #9493, 1000.000000000000000 ) ;
#564=DIRECTION ( 'NONE',  ( -0.005961354470445682716, -0.6427876096865404731, 0.7660212471507180654 ) ) ;
#565=LINE ( 'NONE', #9928, #26557 ) ;
#566=FACE_OUTER_BOUND ( 'NONE', #49151, .T. ) ;
#567=ORIENTED_EDGE ( 'NONE', *, *, #4643, .T. ) ;
#568=CARTESIAN_POINT ( 'NONE',  ( -24.26908309836554878, 0.000000000000000000, 6.108867788427308376 ) ) ;
#569=ORIENTED_EDGE ( 'NONE', *, *, #49303, .F. ) ;
#570=VECTOR ( 'NONE', #19577, 1000.000000000000227 ) ;
#572=CARTESIAN_POINT ( 'NONE',  ( -14.31835180280831032, 0.7721120973665051013, 3.710222702829293784 ) ) ;
#573=LINE ( 'NONE', #48546, #32385 ) ;
#574=CARTESIAN_POINT ( 'NONE',  ( -14.56888064431065821, -0.1191753592594197858, 12.58947452739191064 ) ) ;
#575=CARTESIAN_POINT ( 'NONE',  ( -18.67775241435682432, 0.000000000000000000, 4.136394454059623804 ) ) ;
#576=DIRECTION ( 'NONE',  ( -0.7660212471507179544, -0.6427876096865405842, -0.005961354470445141482 ) ) ;
#577=DIRECTION ( 'NONE',  ( -0.005961354470445682716, -0.6427876096865404731, 0.7660212471507180654 ) ) ;
#578=FACE_OUTER_BOUND ( 'NONE', #34988, .T. ) ;
#579=AXIS2_PLACEMENT_3D ( 'NONE', #39286, #43295, #22800 ) ;
#580=VECTOR ( 'NONE', #27612, 1000.000000000000227 ) ;
#581=DIRECTION ( 'NONE',  ( -0.6427681459581293666, -0.7660444431189770143, -0.005002170337467561935 ) ) ;
#583=DIRECTION ( 'NONE',  ( 0.007781995580012662783, 0.000000000000000000, -0.9999697198139514409 ) ) ;
#584=ORIENTED_EDGE ( 'NONE', *, *, #25515, .T. ) ;
#585=CARTESIAN_POINT ( 'NONE',  ( -29.86352658060627618, 0.000000000000000000, 8.481329010720569883 ) ) ;
#586=DIRECTION ( 'NONE',  ( 0.005961354470445682716, -0.6427876096865404731, -0.7660212471507180654 ) ) ;
#587=DIRECTION ( 'NONE',  ( 0.5364919789714477361, 0.6444004775717706579, 0.5449076811759711036 ) ) ;
#588=FACE_OUTER_BOUND ( 'NONE', #19042, .T. ) ;
#589=DIRECTION ( 'NONE',  ( 0.7660212471507180654, -0.6427876096865404731, 0.005961354470445141482 ) ) ;
#590=CARTESIAN_POINT ( 'NONE',  ( -16.06709938707323460, 0.000000000000000000, 13.13181314741652628 ) ) ;
#591=VECTOR ( 'NONE', #18457, 1000.000000000000227 ) ;
#592=EDGE_LOOP ( 'NONE', ( #35703, #16663, #21212, #3946 ) ) ;
#593=VERTEX_POINT ( 'NONE', #47249 ) ;
#594=DIRECTION ( 'NONE',  ( 0.005002170337468016433, -0.7660444431189770143, -0.6427681459581293666 ) ) ;
#595=CARTESIAN_POINT ( 'NONE',  ( -30.79411802867772607, 0.000000000000000000, 8.643412946479525516 ) ) ;
#596=AXIS2_PLACEMENT_3D ( 'NONE', #22993, #40312, #41442 ) ;
#597=ADVANCED_FACE ( 'NONE', ( #12900 ), #30231, .F. ) ;
#598=ORIENTED_EDGE ( 'NONE', *, *, #54063, .F. ) ;
#599=LINE ( 'NONE', #43470, #29524 ) ;
#600=AXIS2_PLACEMENT_3D ( 'NONE', #53044, #795, #17864 ) ;
#601=ORIENTED_EDGE ( 'NONE', *, *, #47560, .F. ) ;
#602=DIRECTION ( 'NONE',  ( 0.5364919789714477361, 0.6444004775717706579, 0.5449076811759711036 ) ) ;
#603=ADVANCED_FACE ( 'NONE', ( #16312 ), #46704, .F. ) ;
#604=ADVANCED_FACE ( 'NONE', ( #8660 ), #46992, .F. ) ;
#605=VECTOR ( 'NONE', #30042, 1000.000000000000227 ) ;
#606=VERTEX_POINT ( 'NONE', #33927 ) ;
#608=VERTEX_POINT ( 'NONE', #43310 ) ;
#609=CARTESIAN_POINT ( 'NONE',  ( -19.53004645065075096, 0.000000000000000000, 6.145748067415055971 ) ) ;
#610=PLANE ( 'NONE',  #25062 ) ;
#611=DIRECTION ( 'NONE',  ( -0.6246952433987894571, 0.7422098413412802076, 0.2426528472758539834 ) ) ;
#612=VECTOR ( 'NONE', #28011, 1000.000000000000227 ) ;
#613=LINE ( 'NONE', #17941, #43776 ) ;
#615=ORIENTED_EDGE ( 'NONE', *, *, #49932, .F. ) ;
#617=VECTOR ( 'NONE', #49691, 1000.000000000000000 ) ;
#618=CARTESIAN_POINT ( 'NONE',  ( -24.26986129792355129, -0.1191753592594197858, 6.208864760408702388 ) ) ;
#619=EDGE_LOOP ( 'NONE', ( #16851, #28850, #45454, #750 ) ) ;
#620=DIRECTION ( 'NONE',  ( -0.6427681459581293666, -0.7660444431189770143, -0.005002170337467561935 ) ) ;
#621=VERTEX_POINT ( 'NONE', #21132 ) ;
#622=DIRECTION ( 'NONE',  ( 0.007781995580012663651, -3.146120232559066537E-19, -0.9999697198139514409 ) ) ;
#623=LINE ( 'NONE', #13414, #8577 ) ;
#624=ORIENTED_EDGE ( 'NONE', *, *, #35606, .T. ) ;
#625=LINE ( 'NONE', #17951, #37691 ) ;
#626=ORIENTED_EDGE ( 'NONE', *, *, #33083, .F. ) ;
#627=EDGE_CURVE ( 'NONE', #9201, #34530, #21715, .T. ) ;
#628=VECTOR ( 'NONE', #26135, 1000.000000000000000 ) ;
#629=DIRECTION ( 'NONE',  ( 0.7660212471507180654, -0.6427876096865404731, 0.005961354470445141482 ) ) ;
#630=ORIENTED_EDGE ( 'NONE', *, *, #51305, .F. ) ;
#631=ADVANCED_FACE ( 'NONE', ( #8097 ), #25681, .F. ) ;
#632=PLANE ( 'NONE',  #51220 ) ;
#633=DIRECTION ( 'NONE',  ( 0.7660212471507180654, -0.6427876096865404731, 0.005961354470445141482 ) ) ;
#634=PLANE ( 'NONE',  #54566 ) ;
#635=EDGE_CURVE ( 'NONE', #12509, #54234, #44135, .T. ) ;
#636=VERTEX_POINT ( 'NONE', #26809 ) ;
#637=FACE_OUTER_BOUND ( 'NONE', #19734, .T. ) ;
#638=CARTESIAN_POINT ( 'NONE',  ( -12.13851405436063047, 0.000000000000000000, 11.68505802764555135 ) ) ;
#639=VECTOR ( 'NONE', #8987, 1000.000000000000227 ) ;
#640=EDGE_CURVE ( 'NONE', #7467, #15470, #13194, .T. ) ;
#642=PLANE ( 'NONE',  #54018 ) ;
#643=FACE_OUTER_BOUND ( 'NONE', #43485, .T. ) ;
#644=CARTESIAN_POINT ( 'NONE',  ( -6.856675100204708606, -8.693987235299761807, 5.881739038249853557 ) ) ;
#645=VECTOR ( 'NONE', #14355, 999.9999999999998863 ) ;
#647=ORIENTED_EDGE ( 'NONE', *, *, #17303, .F. ) ;
#648=LINE ( 'NONE', #35292, #46115 ) ;
#649=LINE ( 'NONE', #10277, #15006 ) ;
#650=DIRECTION ( 'NONE',  ( 0.5449076811759707706, 0.6444004775717708799, -0.5364919789714476250 ) ) ;
#651=ORIENTED_EDGE ( 'NONE', *, *, #50347, .T. ) ;
#652=DIRECTION ( 'NONE',  ( 0.000000000000000000, -0.000000000000000000, -1.000000000000000000 ) ) ;
#654=EDGE_LOOP ( 'NONE', ( #18887, #14699, #6276, #17282 ) ) ;
#655=DIRECTION ( 'NONE',  ( 0.6427681459581294776, -0.7660444431189769032, 0.005002170337467562802 ) ) ;
#656=AXIS2_PLACEMENT_3D ( 'NONE', #49372, #27815, #45127 ) ;
#657=CARTESIAN_POINT ( 'NONE',  ( -32.65841372305263235, 0.000000000000000000, 9.367568705923016381 ) ) ;
#658=LINE ( 'NONE', #8914, #45018 ) ;
#659=FACE_OUTER_BOUND ( 'NONE', #24133, .T. ) ;
#660=EDGE_LOOP ( 'NONE', ( #9631, #12538, #45330, #12184 ) ) ;
#661=VERTEX_POINT ( 'NONE', #44397 ) ;
#662=PLANE ( 'NONE',  #17637 ) ;
#663=CARTESIAN_POINT ( 'NONE',  ( -13.07066190154808361, 0.000000000000000000, 12.04713590736729678 ) ) ;
#664=DIRECTION ( 'NONE',  ( -0.6427681459581293666, -0.7660444431189770143, -0.005002170337467561935 ) ) ;
#665=ADVANCED_FACE ( 'NONE', ( #14026 ), #9200, .F. ) ;
#666=CARTESIAN_POINT ( 'NONE',  ( -17.73140113748535285, 0.000000000000000000, 13.85752530597602039 ) ) ;
#667=EDGE_CURVE ( 'NONE', #48589, #43836, #26245, .T. ) ;
#668=CARTESIAN_POINT ( 'NONE',  ( -14.15179153153711944, -3.594132820645663084, 2.263685890564126613 ) ) ;
#669=DIRECTION ( 'NONE',  ( -0.5364919789714478471, 0.6444004775717705469, -0.5449076811759709926 ) ) ;
#670=ORIENTED_EDGE ( 'NONE', *, *, #55307, .F. ) ;
#671=LINE ( 'NONE', #17991, #33788 ) ;
#672=EDGE_CURVE ( 'NONE', #23998, #48095, #5247, .T. ) ;
#673=DIRECTION ( 'NONE',  ( 0.007781995580012663651, 0.000000000000000000, -0.9999697198139515519 ) ) ;
#676=LINE ( 'NONE', #5229, #15931 ) ;
#677=DIRECTION ( 'NONE',  ( 0.9999697198139515519, 0.000000000000000000, 0.007781995580013368816 ) ) ;
#678=VERTEX_POINT ( 'NONE', #1225 ) ;
#679=CARTESIAN_POINT ( 'NONE',  ( -14.93495759592298988, 0.000000000000000000, 12.77129166681078409 ) ) ;
#680=ORIENTED_EDGE ( 'NONE', *, *, #9478, .T. ) ;
#681=EDGE_CURVE ( 'NONE', #23840, #12179, #22555, .T. ) ;
#683=AXIS2_PLACEMENT_3D ( 'NONE', #13512, #43590, #4698 ) ;
#684=ORIENTED_EDGE ( 'NONE', *, *, #35245, .F. ) ;
#686=ORIENTED_EDGE ( 'NONE', *, *, #20248, .T. ) ;
#687=DIRECTION ( 'NONE',  ( 0.5364919789714477361, 0.6444004775717706579, 0.5449076811759711036 ) ) ;
#690=VECTOR ( 'NONE', #32497, 999.9999999999998863 ) ;
#691=ORIENTED_EDGE ( 'NONE', *, *, #53911, .F. ) ;
#693=VERTEX_POINT ( 'NONE', #18268 ) ;
#694=CARTESIAN_POINT ( 'NONE',  ( -30.79489622823572859, -0.1191753592594197858, 8.743409918460921304 ) ) ;
#695=VERTEX_POINT ( 'NONE', #5499 ) ;
#696=CARTESIAN_POINT ( 'NONE',  ( -11.33208760941060333, 0.000000000000000000, 1.777561641030050543 ) ) ;
#698=DIRECTION ( 'NONE',  ( 0.5449076811759707706, 0.6444004775717708799, -0.5364919789714476250 ) ) ;
#699=DIRECTION ( 'NONE',  ( 0.5364919789714477361, 0.6444004775717706579, 0.5449076811759711036 ) ) ;
#700=FACE_OUTER_BOUND ( 'NONE', #10945, .T. ) ;
#701=ORIENTED_EDGE ( 'NONE', *, *, #46881, .T. ) ;
#702=ORIENTED_EDGE ( 'NONE', *, *, #51890, .F. ) ;
#703=DIRECTION ( 'NONE',  ( 0.5449076811759707706, 0.6444004775717708799, -0.5364919789714476250 ) ) ;
#704=EDGE_CURVE ( 'NONE', #51394, #48900, #35074, .T. ) ;
#705=PLANE ( 'NONE',  #42988 ) ;
#706=CARTESIAN_POINT ( 'NONE',  ( -17.92576495860976493, -3.594132820645661308, 9.543491873778670254 ) ) ;
#707=LINE ( 'NONE', #5517, #23983 ) ;
#708=LINE ( 'NONE', #56098, #4999 ) ;
#710=ORIENTED_EDGE ( 'NONE', *, *, #19298, .F. ) ;
#711=CARTESIAN_POINT ( 'NONE',  ( -11.16526465312192506, 0.000000000000000000, 6.041518719944250826 ) ) ;
#712=CARTESIAN_POINT ( 'NONE',  ( -18.61514292449499663, 0.000000000000000000, 7.999528407239896666 ) ) ;
#713=VERTEX_POINT ( 'NONE', #30793 ) ;
#714=EDGE_CURVE ( 'NONE', #18910, #36080, #39864, .T. ) ;
#715=LINE ( 'NONE', #35102, #2539 ) ;
#716=DIRECTION ( 'NONE',  ( -0.5364919789714478471, 0.6444004775717705469, -0.5449076811759709926 ) ) ;
#718=EDGE_CURVE ( 'NONE', #14438, #53765, #392, .T. ) ;
#719=EDGE_CURVE ( 'NONE', #45990, #23916, #47841, .T. ) ;
#720=CARTESIAN_POINT ( 'NONE',  ( -28.93137873341882127, 0.000000000000000000, 8.119251130998824451 ) ) ;
#721=CARTESIAN_POINT ( 'NONE',  ( -11.19767518203325807, -2.298917212465660054, 1.157530937302438057 ) ) ;
#722=VERTEX_POINT ( 'NONE', #35907 ) ;
#723=ORIENTED_EDGE ( 'NONE', *, *, #7385, .F. ) ;
#724=LINE ( 'NONE', #22590, #4018 ) ;
#725=PLANE ( 'NONE',  #5945 ) ;
#726=CARTESIAN_POINT ( 'NONE',  ( -8.409922665610809034, 0.000000000000000000, 10.23674650875856962 ) ) ;
#728=VECTOR ( 'NONE', #25296, 999.9999999999998863 ) ;
#729=CARTESIAN_POINT ( 'NONE',  ( -13.20656186341736316, 0.000000000000000000, 3.809640454209623606 ) ) ;
#730=EDGE_CURVE ( 'NONE', #36112, #44493, #22276, .T. ) ;
#731=LINE ( 'NONE', #17782, #17679 ) ;
#733=DIRECTION ( 'NONE',  ( -0.7660212471507179544, -0.6427876096865405842, -0.005961354470445141482 ) ) ;
#734=EDGE_CURVE ( 'NONE', #931, #20189, #34762, .T. ) ;
#735=LINE ( 'NONE', #27135, #14181 ) ;
#736=CARTESIAN_POINT ( 'NONE',  ( -10.47421230394850866, 0.000000000000000000, 10.95934586908605723 ) ) ;
#737=EDGE_LOOP ( 'NONE', ( #27448, #47886, #41645, #33349 ) ) ;
#738=FACE_OUTER_BOUND ( 'NONE', #7670, .T. ) ;
#739=EDGE_LOOP ( 'NONE', ( #34761, #3095, #2567, #15272 ) ) ;
#740=LINE ( 'NONE', #40192, #35004 ) ;
#741=CARTESIAN_POINT ( 'NONE',  ( -13.11188176427955021, -5.051250379848162275, 10.06499431649357135 ) ) ;
#742=ADVANCED_FACE ( 'NONE', ( #43558 ), #48679, .F. ) ;
#743=EDGE_LOOP ( 'NONE', ( #16734, #26904, #34478, #37376 ) ) ;
#744=CARTESIAN_POINT ( 'NONE',  ( -19.53447690327204000, 0.000000000000000000, 6.715051714635608349 ) ) ;
#745=ORIENTED_EDGE ( 'NONE', *, *, #46697, .F. ) ;
#747=EDGE_LOOP ( 'NONE', ( #1784, #12752, #14548, #47746 ) ) ;
#748=EDGE_LOOP ( 'NONE', ( #4796, #32251, #45492, #46225 ) ) ;
#749=CARTESIAN_POINT ( 'NONE',  ( -22.40556560354864146, -0.1191753592594197858, 5.484709000965211523 ) ) ;
#750=ORIENTED_EDGE ( 'NONE', *, *, #21517, .T. ) ;
#751=ORIENTED_EDGE ( 'NONE', *, *, #19934, .F. ) ;
#752=DIRECTION ( 'NONE',  ( -0.9999697198139514409, -0.000000000000000000, -0.007781995580013368816 ) ) ;
#753=CARTESIAN_POINT ( 'NONE',  ( -15.06223539727642446, 0.000000000000000000, 3.425867103879820519 ) ) ;
#754=EDGE_LOOP ( 'NONE', ( #38885, #6213, #1229, #11222 ) ) ;
#755=EDGE_LOOP ( 'NONE', ( #56123, #8490, #39156, #20788 ) ) ;
#757=ORIENTED_EDGE ( 'NONE', *, *, #46611, .F. ) ;
#758=ORIENTED_EDGE ( 'NONE', *, *, #26540, .F. ) ;
#759=DIRECTION ( 'NONE',  ( 0.5449076811759707706, 0.6444004775717708799, -0.5364919789714476250 ) ) ;
#760=CARTESIAN_POINT ( 'NONE',  ( -19.69569380384165669, -0.1191753592594177458, 14.58090286586150697 ) ) ;
#762=ORIENTED_EDGE ( 'NONE', *, *, #37791, .F. ) ;
#763=FACE_OUTER_BOUND ( 'NONE', #43535, .T. ) ;
#764=EDGE_LOOP ( 'NONE', ( #4573, #19800, #42115, #4177 ) ) ;
#765=CIRCLE ( 'NONE', #52451, 6.999999999999988454 ) ;
#766=EDGE_CURVE ( 'NONE', #40769, #6080, #17627, .T. ) ;
#767=DIRECTION ( 'NONE',  ( 0.7660212471507180654, -0.6427876096865404731, 0.005961354470445141482 ) ) ;
#768=CARTESIAN_POINT ( 'NONE',  ( -17.73140113748535285, 0.000000000000000000, 13.85752530597602039 ) ) ;
#769=CARTESIAN_POINT ( 'NONE',  ( -18.33768610320628767, 0.000000000000000000, 6.355033347565870017 ) ) ;
#770=CARTESIAN_POINT ( 'NONE',  ( -18.13038765311693368, 0.000000000000000000, 5.417976396203555645 ) ) ;
#772=DIRECTION ( 'NONE',  ( 0.6427681459581294776, -0.7660444431189769032, 0.005002170337467562802 ) ) ;
#773=LINE ( 'NONE', #5051, #27725 ) ;
#774=ORIENTED_EDGE ( 'NONE', *, *, #17283, .T. ) ;
#775=LINE ( 'NONE', #14417, #8425 ) ;
#776=ADVANCED_FACE ( 'NONE', ( #4006 ), #51696, .F. ) ;
#777=CARTESIAN_POINT ( 'NONE',  ( -15.78376999578702211, 1.419719901456505617, 2.767587519033712695 ) ) ;
#778=DIRECTION ( 'NONE',  ( -0.9999697198139514409, -0.000000000000000000, -0.007781995580013368816 ) ) ;
#779=DIRECTION ( 'NONE',  ( -0.5449076811759708816, 0.6444004775717707689, 0.5364919789714475140 ) ) ;
#781=FACE_OUTER_BOUND ( 'NONE', #23886, .T. ) ;
#782=EDGE_CURVE ( 'NONE', #48488, #51983, #46900, .T. ) ;
#783=CARTESIAN_POINT ( 'NONE',  ( -20.26176469941677993, 0.000000000000000000, 14.76116360616437895 ) ) ;
#784=DIRECTION ( 'NONE',  ( 0.5449076811759707706, 0.6444004775717708799, -0.5364919789714476250 ) ) ;
#785=EDGE_LOOP ( 'NONE', ( #49145, #47097, #14506, #35154 ) ) ;
#786=LINE ( 'NONE', #27189, #22992 ) ;
#787=DIRECTION ( 'NONE',  ( 0.6427681459581294776, -0.7660444431189769032, 0.005002170337467562802 ) ) ;
#788=CARTESIAN_POINT ( 'NONE',  ( -20.21451535923326048, 0.000000000000000000, 5.601763288707669375 ) ) ;
#789=CARTESIAN_POINT ( 'NONE',  ( -25.20123094555300369, 0.000000000000000000, 6.470945668149052032 ) ) ;
#790=ADVANCED_FACE ( 'NONE', ( #42897 ), #30124, .F. ) ;
#791=DIRECTION ( 'NONE',  ( 0.5364919789714477361, 0.6444004775717706579, 0.5449076811759711036 ) ) ;
#792=CARTESIAN_POINT ( 'NONE',  ( -17.36532418587302473, -0.1191753592594177458, 13.67570816655714516 ) ) ;
#793=LINE ( 'NONE', #34887, #12928 ) ;
#794=ADVANCED_FACE ( 'NONE', ( #30422 ), #47438, .F. ) ;
#795=DIRECTION ( 'NONE',  ( 0.005961354470445682716, -0.6427876096865404731, -0.7660212471507180654 ) ) ;
#796=DIRECTION ( 'NONE',  ( 0.000000000000000000, -0.000000000000000000, -1.000000000000000000 ) ) ;
#797=EDGE_CURVE ( 'NONE', #8862, #33893, #21029, .T. ) ;
#798=AXIS2_PLACEMENT_3D ( 'NONE', #26207, #47495, #43510 ) ;
#799=ORIENTED_EDGE ( 'NONE', *, *, #34159, .F. ) ;
#800=EDGE_LOOP ( 'NONE', ( #34379, #40262, #53179, #16521 ) ) ;
#801=EDGE_LOOP ( 'NONE', ( #50622, #1176, #31607, #10321 ) ) ;
#802=ORIENTED_EDGE ( 'NONE', *, *, #22600, .F. ) ;
#803=EDGE_LOOP ( 'NONE', ( #41732, #40202, #30983, #54274 ) ) ;
#804=CARTESIAN_POINT ( 'NONE',  ( -20.92640044469605698, -1.651309408375657428, 7.520536391179072133 ) ) ;
#805=DIRECTION ( 'NONE',  ( 0.005002170337468016433, -0.7660444431189770143, -0.6427681459581293666 ) ) ;
#806=ORIENTED_EDGE ( 'NONE', *, *, #27941, .T. ) ;
#807=ORIENTED_EDGE ( 'NONE', *, *, #43920, .T. ) ;
#808=CARTESIAN_POINT ( 'NONE',  ( -14.87373766733476543, 0.000000000000000000, 4.904662316026882074 ) ) ;
#809=ORIENTED_EDGE ( 'NONE', *, *, #21309, .T. ) ;
#810=DIRECTION ( 'NONE',  ( 0.007781995580012662783, 0.000000000000000000, -0.9999697198139514409 ) ) ;
#811=CARTESIAN_POINT ( 'NONE',  ( -13.97686547933248313, 0.9340140483890051470, 2.081221001769270718 ) ) ;
#812=EDGE_LOOP ( 'NONE', ( #7481, #934, #10633, #30423 ) ) ;
#813=PLANE ( 'NONE',  #17394 ) ;
#814=ADVANCED_FACE ( 'NONE', ( #34965 ), #21621, .F. ) ;
#815=ORIENTED_EDGE ( 'NONE', *, *, #55028, .T. ) ;
#816=LINE ( 'NONE', #31202, #6482 ) ;
#817=EDGE_CURVE ( 'NONE', #29054, #35683, #8551, .T. ) ;
#819=CARTESIAN_POINT ( 'NONE',  ( -16.43317633868556626, -0.1191753592594197858, 13.31363028683540151 ) ) ;
#820=DIRECTION ( 'NONE',  ( 0.9999697198139515519, 0.000000000000000000, 0.007781995580013368816 ) ) ;
#821=ORIENTED_EDGE ( 'NONE', *, *, #1158, .F. ) ;
#822=CARTESIAN_POINT ( 'NONE',  ( 2.072287782118878319, 0.000000000000000000, -2.950529333540147015 ) ) ;
#823=LINE ( 'NONE', #4809, #12037 ) ;
#824=DIRECTION ( 'NONE',  ( -0.9999697198139514409, -0.000000000000000000, -0.007781995580013368816 ) ) ;
#825=EDGE_CURVE ( 'NONE', #18340, #40757, #55982, .T. ) ;
#826=ORIENTED_EDGE ( 'NONE', *, *, #31707, .T. ) ;
#827=CARTESIAN_POINT ( 'NONE',  ( -15.03495456790438389, -0.1191753592594197858, 12.77051346725278158 ) ) ;
#828=ORIENTED_EDGE ( 'NONE', *, *, #6980, .T. ) ;
#829=ADVANCED_FACE ( 'NONE', ( #7709 ), #51441, .F. ) ;
#830=ADVANCED_FACE ( 'NONE', ( #43211 ), #17330, .F. ) ;
#831=EDGE_CURVE ( 'NONE', #12964, #15779, #47153, .T. ) ;
#832=AXIS2_PLACEMENT_3D ( 'NONE', #32437, #46287, #42036 ) ;
#833=LINE ( 'NONE', #9080, #34650 ) ;
#834=CARTESIAN_POINT ( 'NONE',  ( -22.40478740399063895, 0.000000000000000000, 5.384712028983816623 ) ) ;
#835=CARTESIAN_POINT ( 'NONE',  ( -17.91524326081876950, 4.981562823951510843, 12.01580327878066790 ) ) ;
#836=CARTESIAN_POINT ( 'NONE',  ( -19.52010663574562344, 0.000000000000000000, 4.868503198346786576 ) ) ;
#837=LINE ( 'NONE', #17906, #4175 ) ;
#838=DIRECTION ( 'NONE',  ( -0.6246952433987894571, 0.7422098413412802076, 0.2426528472758539834 ) ) ;
#839=CARTESIAN_POINT ( 'NONE',  ( -15.10378980073966204, 0.000000000000000000, 8.765518708783501367 ) ) ;
#840=CARTESIAN_POINT ( 'NONE',  ( -19.58700580672034519, -2.298917212465660054, 4.416231854798146728 ) ) ;
#842=FACE_OUTER_BOUND ( 'NONE', #30586, .T. ) ;
#843=ORIENTED_EDGE ( 'NONE', *, *, #24261, .T. ) ;
#844=LINE ( 'NONE', #18163, #21196 ) ;
#845=DIRECTION ( 'NONE',  ( 0.7660212471507180654, -0.6427876096865404731, 0.005961354470445141482 ) ) ;
#846=DIRECTION ( 'NONE',  ( 0.7660212471507180654, -0.6427876096865404731, 0.005961354470445141482 ) ) ;
#847=CARTESIAN_POINT ( 'NONE',  ( -15.87975247367846166, 0.000000000000000000, 2.850166870931599927 ) ) ;
#848=FACE_OUTER_BOUND ( 'NONE', #36100, .T. ) ;
#849=EDGE_CURVE ( 'NONE', #38597, #41331, #1, .T. ) ;
#850=DIRECTION ( 'NONE',  ( 0.9999697198139515519, 0.000000000000000000, 0.007781995580013368816 ) ) ;
#851=EDGE_CURVE ( 'NONE', #6183, #53549, #4564, .T. ) ;
#852=DIRECTION ( 'NONE',  ( -0.9999697198139514409, -0.000000000000000000, -0.007781995580013368816 ) ) ;
#853=ORIENTED_EDGE ( 'NONE', *, *, #11175, .F. ) ;
#854=ADVANCED_FACE ( 'NONE', ( #3448 ), #20765, .F. ) ;
#855=ORIENTED_EDGE ( 'NONE', *, *, #28585, .T. ) ;
#856=ADVANCED_FACE ( 'NONE', ( #33820 ), #23304, .F. ) ;
#857=DIRECTION ( 'NONE',  ( 0.9999697198139515519, 0.000000000000000000, 0.007781995580013368816 ) ) ;
#858=DIRECTION ( 'NONE',  ( -0.005002170337468016433, -0.7660444431189770143, 0.6427681459581293666 ) ) ;
#859=ADVANCED_FACE ( 'NONE', ( #52543 ), #1124, .F. ) ;
#860=ORIENTED_EDGE ( 'NONE', *, *, #9914, .T. ) ;
#861=DIRECTION ( 'NONE',  ( 0.5364919789714477361, 0.6444004775717706579, 0.5449076811759711036 ) ) ;
#862=ORIENTED_EDGE ( 'NONE', *, *, #20952, .F. ) ;
#863=CARTESIAN_POINT ( 'NONE',  ( -9.772671616987951282, 0.000000000000000000, 6.221682214543255540 ) ) ;
#864=EDGE_CURVE ( 'NONE', #18999, #53740, #1426, .T. ) ;
#865=ORIENTED_EDGE ( 'NONE', *, *, #18651, .T. ) ;
#866=VERTEX_POINT ( 'NONE', #18458 ) ;
#867=ORIENTED_EDGE ( 'NONE', *, *, #30697, .F. ) ;
#868=CARTESIAN_POINT ( 'NONE',  ( -13.53673582514181106, 0.000000000000000000, 12.22817484722816772 ) ) ;
#869=DIRECTION ( 'NONE',  ( 0.007781995580012662783, 0.000000000000000000, -0.9999697198139514409 ) ) ;
#870=CARTESIAN_POINT ( 'NONE',  ( -25.20123094555300369, 0.000000000000000000, 6.470945668149052032 ) ) ;
#871=ORIENTED_EDGE ( 'NONE', *, *, #22259, .F. ) ;
#872=CARTESIAN_POINT ( 'NONE',  ( -15.86710544311044302, 0.000000000000000000, 13.13336954653252953 ) ) ;
#873=VERTEX_POINT ( 'NONE', #14235 ) ;
#874=ORIENTED_EDGE ( 'NONE', *, *, #20758, .T. ) ;
#875=CARTESIAN_POINT ( 'NONE',  ( -14.13140520447825388, 0.000000000000000000, 3.233104983453049641 ) ) ;
#876=ORIENTED_EDGE ( 'NONE', *, *, #34204, .F. ) ;
#877=DIRECTION ( 'NONE',  ( -0.005961354470445682716, -0.6427876096865404731, 0.7660212471507180654 ) ) ;
#878=ORIENTED_EDGE ( 'NONE', *, *, #14782, .T. ) ;
#879=CARTESIAN_POINT ( 'NONE',  ( 2.072287782118878319, 0.000000000000000000, -2.950529333540147015 ) ) ;
#880=DIRECTION ( 'NONE',  ( 0.007781995580012663651, 0.000000000000000000, -0.9999697198139515519 ) ) ;
#881=ORIENTED_EDGE ( 'NONE', *, *, #130, .F. ) ;
#882=DIRECTION ( 'NONE',  ( 0.000000000000000000, -1.000000000000000000, 0.000000000000000000 ) ) ;
#883=VERTEX_POINT ( 'NONE', #40037 ) ;
#884=LINE ( 'NONE', #45187, #36368 ) ;
#885=ORIENTED_EDGE ( 'NONE', *, *, #21590, .F. ) ;
#886=CARTESIAN_POINT ( 'NONE',  ( -18.39746900504187010, 0.000000000000000000, 14.03700784672088808 ) ) ;
#887=CARTESIAN_POINT ( 'NONE',  ( -13.16225250642930078, -4.079838673713163111, 1.863818768663334069 ) ) ;
#888=DIRECTION ( 'NONE',  ( -0.5449076811759708816, 0.6444004775717707689, 0.5364919789714475140 ) ) ;
#889=ORIENTED_EDGE ( 'NONE', *, *, #10422, .T. ) ;
#890=EDGE_CURVE ( 'NONE', #5503, #38452, #22724, .T. ) ;
#891=EDGE_CURVE ( 'NONE', #14388, #9720, #9381, .T. ) ;
#892=LINE ( 'NONE', #47788, #42868 ) ;
#893=LINE ( 'NONE', #48893, #11053 ) ;
#894=DIRECTION ( 'NONE',  ( 0.9999697198139515519, 0.000000000000000000, 0.007781995580013368816 ) ) ;
#895=CARTESIAN_POINT ( 'NONE',  ( -17.55224900710100044, -2.653845599528779520, 12.45560879478165184 ) ) ;
#896=ADVANCED_FACE ( 'NONE', ( #27003 ), #35798, .F. ) ;
#897=FACE_OUTER_BOUND ( 'NONE', #29201, .T. ) ;
#898=CARTESIAN_POINT ( 'NONE',  ( -14.19192946519435417, 1.743523803501506375, 2.138931558044772085 ) ) ;
#899=AXIS2_PLACEMENT_3D ( 'NONE', #35422, #22386, #47649 ) ;
#900=ORIENTED_EDGE ( 'NONE', *, *, #52309, .T. ) ;
#901=LINE ( 'NONE', #53997, #50661 ) ;
#902=CARTESIAN_POINT ( 'NONE',  ( -16.52924358339377164, 5.629170628041515023, 2.922851259777623500 ) ) ;
#903=CARTESIAN_POINT ( 'NONE',  ( -13.14027533394136071, -0.1191753592594181482, 8.142138120879399921 ) ) ;
#904=VERTEX_POINT ( 'NONE', #40625 ) ;
#905=DIRECTION ( 'NONE',  ( -0.6427681459581293666, -0.7660444431189770143, -0.005002170337467561935 ) ) ;
#906=DIRECTION ( 'NONE',  ( -0.7660212471507179544, -0.6427876096865405842, -0.005961354470445141482 ) ) ;
#907=ORIENTED_EDGE ( 'NONE', *, *, #38915, .F. ) ;
#908=PLANE ( 'NONE',  #55197 ) ;
#909=CARTESIAN_POINT ( 'NONE',  ( -17.73140113748535285, 0.000000000000000000, 13.85752530597602039 ) ) ;
#910=DIRECTION ( 'NONE',  ( -0.5364919789714478471, 0.6444004775717705469, -0.5449076811759709926 ) ) ;
#911=EDGE_CURVE ( 'NONE', #21477, #24227, #26703, .T. ) ;
#912=CARTESIAN_POINT ( 'NONE',  ( -16.95658928109344288, 0.000000000000000000, 8.012435655195931261 ) ) ;
#913=ORIENTED_EDGE ( 'NONE', *, *, #52568, .F. ) ;
#915=CARTESIAN_POINT ( 'NONE',  ( -18.32044178217458708, 0.000000000000000000, 4.139175128019283001 ) ) ;
#916=DIRECTION ( 'NONE',  ( 0.007781995580012662783, 0.000000000000000000, -0.9999697198139514409 ) ) ;
#917=CARTESIAN_POINT ( 'NONE',  ( -21.47419595591918906, 0.000000000000000000, 5.222628093224860102 ) ) ;
#918=DIRECTION ( 'NONE',  ( 0.5364919789714477361, 0.6444004775717706579, 0.5449076811759711036 ) ) ;
#920=CARTESIAN_POINT ( 'NONE',  ( -12.08304223278296874, 0.000000000000000000, 4.557048083377176262 ) ) ;
#921=ORIENTED_EDGE ( 'NONE', *, *, #19041, .F. ) ;
#922=CARTESIAN_POINT ( 'NONE',  ( -19.59569683186026268, 0.000000000000000000, 14.58168106541950948 ) ) ;
#923=EDGE_CURVE ( 'NONE', #2679, #53048, #44027, .T. ) ;
#924=FACE_OUTER_BOUND ( 'NONE', #49835, .T. ) ;
#925=ORIENTED_EDGE ( 'NONE', *, *, #9121, .F. ) ;
#926=ADVANCED_FACE ( 'NONE', ( #44865 ), #23006, .F. ) ;
#928=DIRECTION ( 'NONE',  ( -0.3620778797217457101, 0.000000000000000000, -0.9321478471874540261 ) ) ;
#929=EDGE_CURVE ( 'NONE', #51848, #27227, #40328, .T. ) ;
#930=CARTESIAN_POINT ( 'NONE',  ( -16.83345271725875136, -4.565544526780663581, 3.274341045371267800 ) ) ;
#931=VERTEX_POINT ( 'NONE', #9101 ) ;
#932=DIRECTION ( 'NONE',  ( 0.7660212471507180654, -0.6427876096865404731, 0.005961354470445141482 ) ) ;
#934=ORIENTED_EDGE ( 'NONE', *, *, #4863, .T. ) ;
#935=VECTOR ( 'NONE', #8845, 1000.000000000000000 ) ;
#936=EDGE_LOOP ( 'NONE', ( #37602, #6068, #49001, #22421 ) ) ;
#937=ORIENTED_EDGE ( 'NONE', *, *, #53272, .F. ) ;
#938=ORIENTED_EDGE ( 'NONE', *, *, #25465, .T. ) ;
#939=CARTESIAN_POINT ( 'NONE',  ( -12.33850799832341849, 0.000000000000000000, 11.68350162852954632 ) ) ;
#940=VERTEX_POINT ( 'NONE', #22167 ) ;
#941=PLANE ( 'NONE',  #37648 ) ;
#942=LINE ( 'NONE', #19105, #39482 ) ;
#943=ORIENTED_EDGE ( 'NONE', *, *, #31942, .T. ) ;
#944=CARTESIAN_POINT ( 'NONE',  ( -10.27421835998572064, 0.000000000000000000, 10.96090226820206048 ) ) ;
#946=DIRECTION ( 'NONE',  ( 0.5449076811759707706, 0.6444004775717708799, -0.5364919789714476250 ) ) ;
#947=VERTEX_POINT ( 'NONE', #48859 ) ;
#948=PLANE ( 'NONE',  #54545 ) ;
#949=CARTESIAN_POINT ( 'NONE',  ( -14.02258558381341658, -2.298917212465657833, 5.901694980474549546 ) ) ;
#950=CARTESIAN_POINT ( 'NONE',  ( -26.13337879274045505, 0.000000000000000000, 6.833023547870798353 ) ) ;
#952=CARTESIAN_POINT ( 'NONE',  ( -11.60822677631003152, 0.000000000000000000, 3.252740941409099751 ) ) ;
#953=DIRECTION ( 'NONE',  ( -0.7660212471507179544, -0.6427876096865405842, -0.005961354470445141482 ) ) ;
#954=EDGE_LOOP ( 'NONE', ( #10869, #39100, #31754, #41856 ) ) ;
#955=ADVANCED_FACE ( 'NONE', ( #36093 ), #49115, .F. ) ;
#956=EDGE_LOOP ( 'NONE', ( #1313, #15938, #4938, #5565 ) ) ;
#957=CARTESIAN_POINT ( 'NONE',  ( -2.730566055856384011, -5.007877867457373178, -2.157728989155597077 ) ) ;
#959=EDGE_CURVE ( 'NONE', #15160, #32655, #19024, .T. ) ;
#960=EDGE_CURVE ( 'NONE', #29871, #32511, #43730, .T. ) ;
#961=LINE ( 'NONE', #48109, #12461 ) ;
#962=CARTESIAN_POINT ( 'NONE',  ( -15.43942292826481477, 4.333955019861512881, 2.540852065959424255 ) ) ;
#964=DIRECTION ( 'NONE',  ( 0.6427681459581294776, -0.7660444431189769032, 0.005002170337467562802 ) ) ;
#965=DIRECTION ( 'NONE',  ( -0.9999697198139514409, -0.000000000000000000, -0.007781995580013368816 ) ) ;
#966=ORIENTED_EDGE ( 'NONE', *, *, #16669, .T. ) ;
#967=PLANE ( 'NONE',  #37478 ) ;
#969=EDGE_LOOP ( 'NONE', ( #47151, #36627, #20030, #10583 ) ) ;
#971=LINE ( 'NONE', #18595, #52330 ) ;
#972=VECTOR ( 'NONE', #8034, 1000.000000000000000 ) ;
#973=CARTESIAN_POINT ( 'NONE',  ( -11.30636317915456779, -0.1191753592594197858, 11.32220194836580340 ) ) ;
#975=VECTOR ( 'NONE', #31233, 1000.000000000000227 ) ;
#977=ORIENTED_EDGE ( 'NONE', *, *, #21951, .F. ) ;
#978=ORIENTED_EDGE ( 'NONE', *, *, #32584, .T. ) ;
#979=PLANE ( 'NONE',  #20299 ) ;
#980=DIRECTION ( 'NONE',  ( 0.000000000000000000, -0.000000000000000000, -1.000000000000000000 ) ) ;
#981=DIRECTION ( 'NONE',  ( 0.007781995580012663651, -3.146120232559066537E-19, -0.9999697198139514409 ) ) ;
#982=DIRECTION ( 'NONE',  ( -0.005961354470445682716, -0.6427876096865404731, 0.7660212471507180654 ) ) ;
#983=DIRECTION ( 'NONE',  ( 0.007781995580012663651, -3.146120232559066537E-19, -0.9999697198139514409 ) ) ;
#984=ORIENTED_EDGE ( 'NONE', *, *, #52966, .F. ) ;
#986=LINE ( 'NONE', #1824, #42914 ) ;
#987=CARTESIAN_POINT ( 'NONE',  ( -7.416723841188632704, 7.236484701362529748, 6.099280988583309693 ) ) ;
#988=FACE_OUTER_BOUND ( 'NONE', #30286, .T. ) ;
#990=LINE ( 'NONE', #27405, #40172 ) ;
#991=ORIENTED_EDGE ( 'NONE', *, *, #20362, .F. ) ;
#992=CARTESIAN_POINT ( 'NONE',  ( -9.542064456761055524, 0.000000000000000000, 10.59726798936431180 ) ) ;
#993=DIRECTION ( 'NONE',  ( 0.000000000000000000, -1.000000000000000000, 0.000000000000000000 ) ) ;
#995=VECTOR ( 'NONE', #13081, 999.9999999999998863 ) ;
#996=VECTOR ( 'NONE', #24156, 1000.000000000000000 ) ;
#997=LINE ( 'NONE', #53534, #29938 ) ;
#998=EDGE_CURVE ( 'NONE', #8255, #46454, #9688, .T. ) ;
#999=ORIENTED_EDGE ( 'NONE', *, *, #22365, .T. ) ;
#1000=ORIENTED_EDGE ( 'NONE', *, *, #40100, .F. ) ;
#1001=ORIENTED_EDGE ( 'NONE', *, *, #101, .T. ) ;
#1002=CARTESIAN_POINT ( 'NONE',  ( -16.53317331066696383, 0.000000000000000000, 13.31285208727739899 ) ) ;
#1003=VERTEX_POINT ( 'NONE', #37450 ) ;
#1004=VERTEX_POINT ( 'NONE', #19594 ) ;
#1005=CARTESIAN_POINT ( 'NONE',  ( -13.70700505671111991, 0.000000000000000000, 8.407056740829760955 ) ) ;
#1006=CARTESIAN_POINT ( 'NONE',  ( -11.74258550959773473, -2.946525016555661125, 1.348530534211536569 ) ) ;
#1007=EDGE_LOOP ( 'NONE', ( #32540, #50590, #12185 ) ) ;
#1010=ORIENTED_EDGE ( 'NONE', *, *, #51804, .T. ) ;
#1011=PLANE ( 'NONE',  #21343 ) ;
#1012=ORIENTED_EDGE ( 'NONE', *, *, #34768, .T. ) ;
#1013=EDGE_CURVE ( 'NONE', #52907, #40102, #40881, .T. ) ;
#1014=ORIENTED_EDGE ( 'NONE', *, *, #44687, .F. ) ;
#1015=EDGE_CURVE ( 'NONE', #6174, #4939, #19857, .T. ) ;
#1016=AXIS2_PLACEMENT_3D ( 'NONE', #11002, #28060, #6476 ) ;
#1017=CARTESIAN_POINT ( 'NONE',  ( -14.01545677930355183, 0.000000000000000000, 2.126011111488108174 ) ) ;
#1018=DIRECTION ( 'NONE',  ( 0.007781995580012662783, 0.000000000000000000, -0.9999697198139514409 ) ) ;
#1019=DIRECTION ( 'NONE',  ( 0.9999697198139515519, 0.000000000000000000, 0.007781995580013368816 ) ) ;
#1020=DIRECTION ( 'NONE',  ( 0.5449076811759707706, 0.6444004775717708799, -0.5364919789714476250 ) ) ;
#1021=ADVANCED_FACE ( 'NONE', ( #54225 ), #6262, .F. ) ;
#1022=EDGE_LOOP ( 'NONE', ( #31924, #11783, #54419, #4672 ) ) ;
#1023=DIRECTION ( 'NONE',  ( -0.7660212471507179544, -0.6427876096865405842, -0.005961354470445141482 ) ) ;
#1025=EDGE_CURVE ( 'NONE', #25299, #40139, #41984, .T. ) ;
#1026=CARTESIAN_POINT ( 'NONE',  ( -24.26908309836554878, 0.000000000000000000, 6.108867788427308376 ) ) ;
#1027=ADVANCED_FACE ( 'NONE', ( #28102 ), #46241, .F. ) ;
#1028=CARTESIAN_POINT ( 'NONE',  ( -21.47263955680318404, 0.000000000000000000, 5.022634149262071190 ) ) ;
#1029=CARTESIAN_POINT ( 'NONE',  ( -27.99923088623136636, 0.000000000000000000, 7.757173251277078130 ) ) ;
#1030=CARTESIAN_POINT ( 'NONE',  ( -16.99924723426068951, 0.000000000000000000, 13.49389102713827171 ) ) ;
#1032=DIRECTION ( 'NONE',  ( 0.9999697198139515519, 0.000000000000000000, 0.007781995580013368816 ) ) ;
#1033=DIRECTION ( 'NONE',  ( 0.8531650599175529814, -0.4028455766673920135, -0.3313982828793697877 ) ) ;
#1034=ORIENTED_EDGE ( 'NONE', *, *, #29741, .T. ) ;
#1035=DIRECTION ( 'NONE',  ( -0.7660212471507179544, -0.6427876096865405842, -0.005961354470445141482 ) ) ;
#1036=EDGE_CURVE ( 'NONE', #40968, #15460, #7347, .T. ) ;
#1037=VECTOR ( 'NONE', #30828, 1000.000000000000227 ) ;
#1038=VECTOR ( 'NONE', #2284, 1000.000000000000227 ) ;
#1040=PLANE ( 'NONE',  #55004 ) ;
#1041=PLANE ( 'NONE',  #6322 ) ;
#1043=PLANE ( 'NONE',  #11381 ) ;
#1044=PLANE ( 'NONE',  #25022 ) ;
#1045=EDGE_CURVE ( 'NONE', #53756, #29871, #2790, .T. ) ;
#1046=DIRECTION ( 'NONE',  ( 0.007781995580012663651, 0.000000000000000000, -0.9999697198139515519 ) ) ;
#1047=VECTOR ( 'NONE', #21180, 1000.000000000000114 ) ;
#1048=ORIENTED_EDGE ( 'NONE', *, *, #6882, .T. ) ;
#1049=CARTESIAN_POINT ( 'NONE',  ( 2.072287782118878319, 0.000000000000000000, -2.950529333540147015 ) ) ;
#1051=DIRECTION ( 'NONE',  ( 0.9999697198139515519, 0.000000000000000000, 0.007781995580013368816 ) ) ;
#1052=CARTESIAN_POINT ( 'NONE',  ( -15.45392365408441826, 1.581621852479004664, 2.634298478400116661 ) ) ;
#1053=LINE ( 'NONE', #49050, #32156 ) ;
#1054=DIRECTION ( 'NONE',  ( -0.6427681459581293666, -0.7660444431189770143, -0.005002170337467561935 ) ) ;
#1055=DIRECTION ( 'NONE',  ( 0.9999697198139515519, 0.000000000000000000, 0.007781995580013368816 ) ) ;
#1056=AXIS2_PLACEMENT_3D ( 'NONE', #46333, #7749, #45795 ) ;
#1057=CARTESIAN_POINT ( 'NONE',  ( -10.42448858938141321, 0.000000000000000000, 4.569955331333209969 ) ) ;
#1058=LINE ( 'NONE', #4508, #34692 ) ;
#1059=ORIENTED_EDGE ( 'NONE', *, *, #9491, .T. ) ;
#1060=EDGE_CURVE ( 'NONE', #52765, #2187, #54478, .T. ) ;
#1061=ORIENTED_EDGE ( 'NONE', *, *, #28759, .T. ) ;
#1062=ORIENTED_EDGE ( 'NONE', *, *, #16103, .T. ) ;
#1063=ORIENTED_EDGE ( 'NONE', *, *, #52829, .T. ) ;
#1064=ORIENTED_EDGE ( 'NONE', *, *, #44421, .T. ) ;
#1066=CARTESIAN_POINT ( 'NONE',  ( -22.40556560354864146, -0.1191753592594197858, 5.484709000965211523 ) ) ;
#1067=EDGE_CURVE ( 'NONE', #38273, #21098, #53942, .T. ) ;
#1068=AXIS2_PLACEMENT_3D ( 'NONE', #38433, #16875, #51514 ) ;
#1069=VECTOR ( 'NONE', #18804, 999.9999999999998863 ) ;
#1070=ORIENTED_EDGE ( 'NONE', *, *, #44192, .T. ) ;
#1071=ORIENTED_EDGE ( 'NONE', *, *, #14890, .T. ) ;
#1072=EDGE_CURVE ( 'NONE', #30915, #18980, #14765, .T. ) ;
#1073=VECTOR ( 'NONE', #39471, 1000.000000000000227 ) ;
#1075=ORIENTED_EDGE ( 'NONE', *, *, #36477, .T. ) ;
#1076=PLANE ( 'NONE',  #9214 ) ;
#1077=DIRECTION ( 'NONE',  ( 0.007781995580012663651, -3.146120232559066537E-19, -0.9999697198139514409 ) ) ;
#1078=ORIENTED_EDGE ( 'NONE', *, *, #56058, .F. ) ;
#1079=FACE_OUTER_BOUND ( 'NONE', #48733, .T. ) ;
#1080=VERTEX_POINT ( 'NONE', #32094 ) ;
#1081=CARTESIAN_POINT ( 'NONE',  ( -18.66354898467281132, 0.000000000000000000, 14.21960318569776582 ) ) ;
#1082=ADVANCED_FACE ( 'NONE', ( #28673 ), #23565, .F. ) ;
#1084=DIRECTION ( 'NONE',  ( -0.9999697198139514409, -0.000000000000000000, -0.007781995580013368816 ) ) ;
#1085=EDGE_CURVE ( 'NONE', #36106, #20635, #41457, .T. ) ;
#1086=CARTESIAN_POINT ( 'NONE',  ( -10.66613911421745264, 0.000000000000000000, 1.613418192619087588 ) ) ;
#1087=PLANE ( 'NONE',  #45093 ) ;
#1088=ORIENTED_EDGE ( 'NONE', *, *, #55992, .F. ) ;
#1089=CARTESIAN_POINT ( 'NONE',  ( -14.65381140700083229, -1.975113310420658852, 2.510342657734869753 ) ) ;
#1090=CARTESIAN_POINT ( 'NONE',  ( -19.45503627000849889, -1.000000000000000000, 7.556996783084074742 ) ) ;
#1091=CARTESIAN_POINT ( 'NONE',  ( -27.06708303904391144, 0.000000000000000000, 7.395095371555332697 ) ) ;
#1092=EDGE_LOOP ( 'NONE', ( #33982, #22318, #12217, #35445 ) ) ;
#1093=LINE ( 'NONE', #23536, #39186 ) ;
#1094=ORIENTED_EDGE ( 'NONE', *, *, #34768, .F. ) ;
#1095=EDGE_CURVE ( 'NONE', #28751, #18842, #32389, .T. ) ;
#1096=LINE ( 'NONE', #39754, #2894 ) ;
#1097=CARTESIAN_POINT ( 'NONE',  ( -19.60990026154428278, 0.000000000000000000, 4.498472333781370125 ) ) ;
#1098=PLANE ( 'NONE',  #40317 ) ;
#1099=DIRECTION ( 'NONE',  ( 0.6427681459581294776, -0.7660444431189769032, 0.005002170337467562802 ) ) ;
#1100=AXIS2_PLACEMENT_3D ( 'NONE', #1492, #4626, #4911 ) ;
#1101=DIRECTION ( 'NONE',  ( -0.005002170337468016433, -0.7660444431189770143, 0.6427681459581293666 ) ) ;
#1102=FACE_OUTER_BOUND ( 'NONE', #19728, .T. ) ;
#1103=CARTESIAN_POINT ( 'NONE',  ( -9.847580306979804021, -0.1191753592594190225, 2.997113657646766516 ) ) ;
#1104=EDGE_CURVE ( 'NONE', #32862, #27005, #10793, .T. ) ;
#1105=PLANE ( 'NONE',  #11081 ) ;
#1106=SURFACE_STYLE_FILL_AREA ( #18752 ) ;
#1108=ORIENTED_EDGE ( 'NONE', *, *, #24121, .F. ) ;
#1109=VECTOR ( 'NONE', #22249, 1000.000000000000227 ) ;
#1110=CARTESIAN_POINT ( 'NONE',  ( -17.18961764541363024, 0.000000000000000000, 3.947969406708516704 ) ) ;
#1111=PLANE ( 'NONE',  #28547 ) ;
#1112=CARTESIAN_POINT ( 'NONE',  ( -19.97424332634331989, -1.651309408375658760, 4.587310137610792538 ) ) ;
#1113=CARTESIAN_POINT ( 'NONE',  ( -22.40556560354864146, -0.1191753592594197858, 5.484709000965211523 ) ) ;
#1114=VECTOR ( 'NONE', #14489, 1000.000000000000227 ) ;
#1115=VECTOR ( 'NONE', #5387, 999.9999999999998863 ) ;
#1116=LINE ( 'NONE', #25872, #47246 ) ;
#1117=PLANE ( 'NONE',  #16062 ) ;
#1118=DIRECTION ( 'NONE',  ( 0.6427681459581294776, -0.7660444431189769032, 0.005002170337467562802 ) ) ;
#1119=VERTEX_POINT ( 'NONE', #15325 ) ;
#1120=VECTOR ( 'NONE', #5356, 999.9999999999998863 ) ;
#1121=VECTOR ( 'NONE', #32886, 1000.000000000000227 ) ;
#1122=ORIENTED_EDGE ( 'NONE', *, *, #48950, .T. ) ;
#1124=PLANE ( 'NONE',  #9605 ) ;
#1125=EDGE_LOOP ( 'NONE', ( #11524, #5118, #3400, #21702 ) ) ;
#1126=PLANE ( 'NONE',  #50338 ) ;
#1127=ADVANCED_FACE ( 'NONE', ( #41701 ), #45409, .F. ) ;
#1128=VERTEX_POINT ( 'NONE', #11045 ) ;
#1129=LINE ( 'NONE', #31252, #252 ) ;
#1130=EDGE_LOOP ( 'NONE', ( #36116, #1815, #51661, #8244 ) ) ;
#1131=VERTEX_POINT ( 'NONE', #28370 ) ;
#1132=EDGE_CURVE ( 'NONE', #3861, #40733, #6809, .T. ) ;
#1133=ORIENTED_EDGE ( 'NONE', *, *, #12182, .F. ) ;
#1134=EDGE_CURVE ( 'NONE', #21716, #44513, #51470, .T. ) ;
#1135=LINE ( 'NONE', #22480, #12068 ) ;
#1136=DIRECTION ( 'NONE',  ( 0.7660212471507180654, -0.6427876096865404731, 0.005961354470445141482 ) ) ;
#1137=PLANE ( 'NONE',  #47499 ) ;
#1138=ADVANCED_FACE ( 'NONE', ( #33850 ), #50875, .F. ) ;
#1139=ADVANCED_FACE ( 'NONE', ( #33566 ), #7742, .F. ) ;
#1140=EDGE_CURVE ( 'NONE', #29285, #27679, #8026, .T. ) ;
#1141=DIRECTION ( 'NONE',  ( -0.7660212471507179544, -0.6427876096865405842, -0.005961354470445141482 ) ) ;
#1142=ORIENTED_EDGE ( 'NONE', *, *, #25881, .F. ) ;
#1144=VECTOR ( 'NONE', #22161, 999.9999999999998863 ) ;
#1145=CARTESIAN_POINT ( 'NONE',  ( -17.80222495869421451, -1.813211359398156919, 6.572709218920322449 ) ) ;
#1146=ORIENTED_EDGE ( 'NONE', *, *, #41593, .F. ) ;
#1147=VECTOR ( 'NONE', #55689, 1000.000000000000114 ) ;
#1148=CARTESIAN_POINT ( 'NONE',  ( -17.74404816805336793, 0.000000000000000000, 3.574322630375089460 ) ) ;
#1149=EDGE_LOOP ( 'NONE', ( #52643, #9477, #12356, #26488 ) ) ;
#1150=DIRECTION ( 'NONE',  ( 0.9999697198139515519, 0.000000000000000000, 0.007781995580013368816 ) ) ;
#1151=FACE_OUTER_BOUND ( 'NONE', #44393, .T. ) ;
#1152=VECTOR ( 'NONE', #35541, 1000.000000000000227 ) ;
#1153=AXIS2_PLACEMENT_3D ( 'NONE', #22380, #1035, #40542 ) ;
#1154=VERTEX_POINT ( 'NONE', #25339 ) ;
#1155=CARTESIAN_POINT ( 'NONE',  ( -14.93495759592298988, 0.000000000000000000, 12.77129166681078409 ) ) ;
#1156=EDGE_CURVE ( 'NONE', #29456, #32397, #8288, .T. ) ;
#1157=ORIENTED_EDGE ( 'NONE', *, *, #53864, .F. ) ;
#1158=EDGE_CURVE ( 'NONE', #34260, #18621, #47181, .T. ) ;
#1159=VECTOR ( 'NONE', #7810, 1000.000000000000114 ) ;
#1160=DIRECTION ( 'NONE',  ( 0.5364919789714477361, 0.6444004775717706579, 0.5449076811759711036 ) ) ;
#1161=AXIS2_PLACEMENT_3D ( 'NONE', #8248, #51124, #25562 ) ;
#1162=ORIENTED_EDGE ( 'NONE', *, *, #48359, .F. ) ;
#1163=PLANE ( 'NONE',  #31379 ) ;
#1164=DIRECTION ( 'NONE',  ( 0.9999697198139515519, 0.000000000000000000, 0.007781995580013368816 ) ) ;
#1165=EDGE_CURVE ( 'NONE', #13096, #1131, #46626, .T. ) ;
#1166=DIRECTION ( 'NONE',  ( 0.007781995580012662783, 0.000000000000000000, -0.9999697198139514409 ) ) ;
#1167=VERTEX_POINT ( 'NONE', #38105 ) ;
#1168=ADVANCED_FACE ( 'NONE', ( #51169 ), #12282, .F. ) ;
#1169=CARTESIAN_POINT ( 'NONE',  ( -14.67804947269237203, -1.975113310420657520, 5.624882046661574542 ) ) ;
#1170=DIRECTION ( 'NONE',  ( 0.000000000000000000, -0.000000000000000000, -1.000000000000000000 ) ) ;
#1171=AXIS2_PLACEMENT_3D ( 'NONE', #24094, #11305, #41422 ) ;
#1172=FACE_OUTER_BOUND ( 'NONE', #56171, .T. ) ;
#1173=VECTOR ( 'NONE', #47615, 1000.000000000000227 ) ;
#1174=DIRECTION ( 'NONE',  ( -0.6427681459581293666, -0.7660444431189770143, -0.005002170337467561935 ) ) ;
#1175=CARTESIAN_POINT ( 'NONE',  ( -9.394439624159845792, -0.1191753592594179401, 4.477968382445831175 ) ) ;
#1176=ORIENTED_EDGE ( 'NONE', *, *, #5629, .F. ) ;
#1177=DIRECTION ( 'NONE',  ( 0.007781995580012662783, 0.000000000000000000, -0.9999697198139514409 ) ) ;
#1178=FACE_OUTER_BOUND ( 'NONE', #8509, .T. ) ;
#1179=CARTESIAN_POINT ( 'NONE',  ( -18.67619601524082285, 0.000000000000000000, 3.936400510096834893 ) ) ;
#1181=PLANE ( 'NONE',  #2092 ) ;
#1182=FACE_OUTER_BOUND ( 'NONE', #21499, .T. ) ;
#1183=ORIENTED_EDGE ( 'NONE', *, *, #22124, .F. ) ;
#1184=AXIS2_PLACEMENT_3D ( 'NONE', #26250, #51542, #51252 ) ;
#1185=DIRECTION ( 'NONE',  ( -0.7660212471507179544, -0.6427876096865405842, -0.005961354470445141482 ) ) ;
#1186=CARTESIAN_POINT ( 'NONE',  ( -15.60102546347950536, 0.000000000000000000, 12.95077420755565356 ) ) ;
#1187=AXIS2_PLACEMENT_3D ( 'NONE', #30707, #43214, #21625 ) ;
#1188=LINE ( 'NONE', #18521, #5171 ) ;
#1189=DIRECTION ( 'NONE',  ( 0.5364919789714477361, 0.6444004775717706579, 0.5449076811759711036 ) ) ;
#1190=EDGE_LOOP ( 'NONE', ( #52515, #25889, #24218, #32180 ) ) ;
#1192=DIRECTION ( 'NONE',  ( -0.6427681459581293666, -0.7660444431189770143, -0.005002170337467561935 ) ) ;
#1193=PLANE ( 'NONE',  #17787 ) ;
#1194=VECTOR ( 'NONE', #24398, 1000.000000000000227 ) ;
#1195=CARTESIAN_POINT ( 'NONE',  ( -13.58191980274018462, -0.1191753592594188005, 5.184044583049274735 ) ) ;
#1197=FACE_OUTER_BOUND ( 'NONE', #37198, .T. ) ;
#1198=AXIS2_PLACEMENT_3D ( 'NONE', #51681, #25861, #30690 ) ;
#1199=CARTESIAN_POINT ( 'NONE',  ( -14.94760462649100496, 0.000000000000000000, 2.488088991209854051 ) ) ;
#1200=CARTESIAN_POINT ( 'NONE',  ( -20.26688789326949092, -0.6003329984493698257, 5.466933331983609534 ) ) ;
#1201=VERTEX_POINT ( 'NONE', #43241 ) ;
#1202=CARTESIAN_POINT ( 'NONE',  ( -15.03495456790438389, -0.1191753592594197858, 12.77051346725278158 ) ) ;
#1203=VECTOR ( 'NONE', #49764, 1000.000000000000227 ) ;
#1204=DIRECTION ( 'NONE',  ( 0.005961354470445682716, -0.6427876096865404731, -0.7660212471507180654 ) ) ;
#1205=AXIS2_PLACEMENT_3D ( 'NONE', #21549, #51628, #34880 ) ;
#1206=ORIENTED_EDGE ( 'NONE', *, *, #7060, .F. ) ;
#1207=DIRECTION ( 'NONE',  ( -0.7660212471507179544, -0.6427876096865405842, -0.005961354470445141482 ) ) ;
#1208=FACE_OUTER_BOUND ( 'NONE', #45868, .T. ) ;
#1209=DIRECTION ( 'NONE',  ( 0.6427681459581294776, -0.7660444431189769032, 0.005002170337467562802 ) ) ;
#1210=EDGE_CURVE ( 'NONE', #11984, #43814, #42642, .T. ) ;
#1211=ADVANCED_FACE ( 'NONE', ( #21362 ), #55420, .F. ) ;
#1212=ORIENTED_EDGE ( 'NONE', *, *, #28692, .F. ) ;
#1213=CARTESIAN_POINT ( 'NONE',  ( -10.42580624377069398, 0.000000000000000000, 4.739271090628184524 ) ) ;
#1214=ORIENTED_EDGE ( 'NONE', *, *, #17604, .T. ) ;
#1215=ADVANCED_FACE ( 'NONE', ( #55710 ), #42932, .F. ) ;
#1216=ORIENTED_EDGE ( 'NONE', *, *, #54700, .F. ) ;
#1217=ORIENTED_EDGE ( 'NONE', *, *, #5235, .F. ) ;
#1219=DIRECTION ( 'NONE',  ( 0.000000000000000000, -1.000000000000000000, 0.000000000000000000 ) ) ;
#1220=VERTEX_POINT ( 'NONE', #4337 ) ;
#1221=VECTOR ( 'NONE', #37144, 1000.000000000000114 ) ;
#1222=CARTESIAN_POINT ( 'NONE',  ( -20.26176469941677993, 0.000000000000000000, 14.76116360616437895 ) ) ;
#1223=LINE ( 'NONE', #56140, #49492 ) ;
#1224=VERTEX_POINT ( 'NONE', #34158 ) ;
#1225=CARTESIAN_POINT ( 'NONE',  ( -11.15796014699535910, 0.000000000000000000, 5.102905369465933205 ) ) ;
#1227=CARTESIAN_POINT ( 'NONE',  ( -31.72782227498118601, 0.000000000000000000, 9.205484770164058972 ) ) ;
#1228=VECTOR ( 'NONE', #3408, 999.9999999999998863 ) ;
#1229=ORIENTED_EDGE ( 'NONE', *, *, #9897, .F. ) ;
#1230=EDGE_CURVE ( 'NONE', #31801, #20518, #12566, .T. ) ;
#1231=CARTESIAN_POINT ( 'NONE',  ( -17.93139508144814442, 0.000000000000000000, 13.85596890686001537 ) ) ;
#1232=PLANE ( 'NONE',  #41080 ) ;
#1233=DIRECTION ( 'NONE',  ( 0.6427681459581294776, -0.7660444431189769032, 0.005002170337467562802 ) ) ;
#1235=EDGE_CURVE ( 'NONE', #37629, #10857, #21649, .T. ) ;
#1236=FACE_OUTER_BOUND ( 'NONE', #19862, .T. ) ;
#1237=AXIS2_PLACEMENT_3D ( 'NONE', #54105, #41025, #45852 ) ;
#1238=LINE ( 'NONE', #10643, #55534 ) ;
#1239=ORIENTED_EDGE ( 'NONE', *, *, #43794, .T. ) ;
#1240=VECTOR ( 'NONE', #9345, 1000.000000000000000 ) ;
#1241=EDGE_CURVE ( 'NONE', #8596, #49849, #12831, .T. ) ;
#1242=EDGE_LOOP ( 'NONE', ( #33007, #29909, #54777, #5167 ) ) ;
#1243=CARTESIAN_POINT ( 'NONE',  ( -17.75217832828985820, -0.1191753592594190225, 3.677175353557638360 ) ) ;
#1244=CARTESIAN_POINT ( 'NONE',  ( -13.27065584551087163, 0.000000000000000000, 12.04557950825129176 ) ) ;
#1245=ADVANCED_FACE ( 'NONE', ( #26 ), #17357, .F. ) ;
#1246=DIRECTION ( 'NONE',  ( 0.005002170337468016433, -0.7660444431189770143, -0.6427681459581293666 ) ) ;
#1247=AXIS2_PLACEMENT_3D ( 'NONE', #53931, #1951, #32382 ) ;
#1248=VECTOR ( 'NONE', #31091, 999.9999999999998863 ) ;
#1249=CARTESIAN_POINT ( 'NONE',  ( -24.26908309836554878, 0.000000000000000000, 6.108867788427308376 ) ) ;
#1250=EDGE_LOOP ( 'NONE', ( #46634, #5454, #20723, #15875 ) ) ;
#1251=CARTESIAN_POINT ( 'NONE',  ( -11.20636620717317378, 0.000000000000000000, 11.32298014792380414 ) ) ;
#1252=CARTESIAN_POINT ( 'NONE',  ( -14.49107522188537800, -0.1191753592594191197, 2.591644836708906663 ) ) ;
#1253=ORIENTED_EDGE ( 'NONE', *, *, #34974, .T. ) ;
#1255=CARTESIAN_POINT ( 'NONE',  ( -8.975993561185934055, -0.1191753592594197858, 10.41700724906143982 ) ) ;
#1256=VERTEX_POINT ( 'NONE', #4590 ) ;
#1257=DIRECTION ( 'NONE',  ( 0.9999697198139515519, 0.000000000000000000, 0.007781995580013368816 ) ) ;
#1258=CARTESIAN_POINT ( 'NONE',  ( -19.60990026154428278, 0.000000000000000000, 4.498472333781370125 ) ) ;
#1259=PLANE ( 'NONE',  #49497 ) ;
#1260=DIRECTION ( 'NONE',  ( -0.6427681459581293666, -0.7660444431189770143, -0.005002170337467561935 ) ) ;
#1261=CARTESIAN_POINT ( 'NONE',  ( -9.867698681516781534, -0.1191753592594181482, 5.582281580451115666 ) ) ;
#1262=EDGE_LOOP ( 'NONE', ( #22416, #28896, #47549, #43417 ) ) ;
#1263=VECTOR ( 'NONE', #44655, 1000.000000000000227 ) ;
#1264=ORIENTED_EDGE ( 'NONE', *, *, #30729, .T. ) ;
#1265=CARTESIAN_POINT ( 'NONE',  ( -15.13495153988577968, 0.000000000000000000, 12.76973526769478084 ) ) ;
#1266=FACE_OUTER_BOUND ( 'NONE', #11393, .T. ) ;
#1267=LINE ( 'NONE', #22855, #52369 ) ;
#1268=AXIS2_PLACEMENT_3D ( 'NONE', #28854, #37644, #54973 ) ;
#1269=DIRECTION ( 'NONE',  ( 0.7660212471507180654, -0.6427876096865404731, 0.005961354470445141482 ) ) ;
#1270=CARTESIAN_POINT ( 'NONE',  ( -16.79925329029790149, 0.000000000000000000, 13.49544742625427496 ) ) ;
#1271=VECTOR ( 'NONE', #54648, 999.9999999999998863 ) ;
#1272=ORIENTED_EDGE ( 'NONE', *, *, #50044, .F. ) ;
#1273=FACE_OUTER_BOUND ( 'NONE', #23658, .T. ) ;
#1274=CARTESIAN_POINT ( 'NONE',  ( -14.59739752808399693, -5.698858183938163791, 11.70485382328475765 ) ) ;
#1275=DIRECTION ( 'NONE',  ( 0.9999697198139515519, 0.000000000000000000, 0.007781995580013368816 ) ) ;
#1276=CARTESIAN_POINT ( 'NONE',  ( -18.48268442577178661, -3.756034771668162797, 3.940786248539256853 ) ) ;
#1277=ORIENTED_EDGE ( 'NONE', *, *, #6006, .F. ) ;
#1278=AXIS2_PLACEMENT_3D ( 'NONE', #55144, #50605, #11698 ) ;
#1279=DIRECTION ( 'NONE',  ( 0.6427681459581294776, -0.7660444431189769032, 0.005002170337467562802 ) ) ;
#1280=EDGE_LOOP ( 'NONE', ( #46976, #26824, #5714, #7174 ) ) ;
#1281=DIRECTION ( 'NONE',  ( 0.007781995580012662783, 0.000000000000000000, -0.9999697198139514409 ) ) ;
#1282=FACE_OUTER_BOUND ( 'NONE', #16307, .T. ) ;
#1283=VECTOR ( 'NONE', #40595, 999.9999999999998863 ) ;
#1284=ADVANCED_FACE ( 'NONE', ( #1151 ), #13661, .F. ) ;
#1285=ORIENTED_EDGE ( 'NONE', *, *, #18893, .T. ) ;
#1286=CARTESIAN_POINT ( 'NONE',  ( -10.21431608578677519, 0.000000000000000000, 3.263588676713128578 ) ) ;
#1287=VERTEX_POINT ( 'NONE', #44333 ) ;
#1288=EDGE_CURVE ( 'NONE', #9606, #17353, #317, .T. ) ;
#1289=EDGE_CURVE ( 'NONE', #42137, #2279, #22746, .T. ) ;
#1290=VECTOR ( 'NONE', #5907, 1000.000000000000114 ) ;
#1291=EDGE_LOOP ( 'NONE', ( #10494, #29693, #27691, #54552 ) ) ;
#1292=VERTEX_POINT ( 'NONE', #35527 ) ;
#1293=CARTESIAN_POINT ( 'NONE',  ( -18.02080248396530848, 3.524445264749011208, 3.569375148849157853 ) ) ;
#1294=VECTOR ( 'NONE', #21814, 1000.000000000000227 ) ;
#1295=ORIENTED_EDGE ( 'NONE', *, *, #24887, .F. ) ;
#1296=ORIENTED_EDGE ( 'NONE', *, *, #16534, .F. ) ;
#1297=CARTESIAN_POINT ( 'NONE',  ( -5.829680373272994487, -7.699177326359582629, 5.482819409421843204 ) ) ;
#1298=LINE ( 'NONE', #9849, #30364 ) ;
#1299=ORIENTED_EDGE ( 'NONE', *, *, #8340, .T. ) ;
#1300=VERTEX_POINT ( 'NONE', #31572 ) ;
#1301=CARTESIAN_POINT ( 'NONE',  ( -15.36136699221811064, 0.000000000000000000, 7.855524030320988338 ) ) ;
#1302=ORIENTED_EDGE ( 'NONE', *, *, #43624, .T. ) ;
#1303=ORIENTED_EDGE ( 'NONE', *, *, #54137, .T. ) ;
#1304=AXIS2_PLACEMENT_3D ( 'NONE', #45579, #12056, #50690 ) ;
#1305=DIRECTION ( 'NONE',  ( -0.5364919789714478471, 0.6444004775717705469, -0.5449076811759709926 ) ) ;
#1306=VECTOR ( 'NONE', #56012, 1000.000000000000227 ) ;
#1308=CARTESIAN_POINT ( 'NONE',  ( -16.77606153933838229, -5.051250379848164052, 3.236551803192220245 ) ) ;
#1309=DIRECTION ( 'NONE',  ( -0.5449076811759708816, 0.6444004775717707689, 0.5364919789714475140 ) ) ;
#1310=ORIENTED_EDGE ( 'NONE', *, *, #55422, .T. ) ;
#1311=LINE ( 'NONE', #54384, #47388 ) ;
#1312=AXIS2_PLACEMENT_3D ( 'NONE', #4287, #55657, #30394 ) ;
#1313=ORIENTED_EDGE ( 'NONE', *, *, #45290, .F. ) ;
#1314=PLANE ( 'NONE',  #36669 ) ;
#1315=ADVANCED_FACE ( 'NONE', ( #14515 ), #5437, .F. ) ;
#1316=DIRECTION ( 'NONE',  ( 0.9999697198139515519, 0.000000000000000000, 0.007781995580013368816 ) ) ;
#1317=VECTOR ( 'NONE', #25702, 999.9999999999998863 ) ;
#1318=CARTESIAN_POINT ( 'NONE',  ( -12.00514593104556305, -3.756034771668160577, 7.509431062354686937 ) ) ;
#1319=LINE ( 'NONE', #30867, #45881 ) ;
#1320=EDGE_CURVE ( 'NONE', #15806, #5087, #40357, .T. ) ;
#1322=AXIS2_PLACEMENT_3D ( 'NONE', #44807, #9906, #32032 ) ;
#1323=CARTESIAN_POINT ( 'NONE',  ( -15.03495456790438389, -0.1191753592594197858, 12.77051346725278158 ) ) ;
#1324=ORIENTED_EDGE ( 'NONE', *, *, #35734, .T. ) ;
#1325=CARTESIAN_POINT ( 'NONE',  ( -13.86208312349174854, 1.905425754524006532, 2.005642517411173831 ) ) ;
#1326=EDGE_CURVE ( 'NONE', #22884, #34361, #1455, .T. ) ;
#1327=VERTEX_POINT ( 'NONE', #6014 ) ;
#1328=AXIS2_PLACEMENT_3D ( 'NONE', #55885, #8446, #34562 ) ;
#1329=FACE_OUTER_BOUND ( 'NONE', #32283, .T. ) ;
#1331=PLANE ( 'NONE',  #55336 ) ;
#1332=ADVANCED_FACE ( 'NONE', ( #52836 ), #48293, .F. ) ;
#1333=PLANE ( 'NONE',  #14999 ) ;
#1334=CARTESIAN_POINT ( 'NONE',  ( -25.20278734466900517, 0.000000000000000000, 6.670939612111840944 ) ) ;
#1335=VECTOR ( 'NONE', #36218, 1000.000000000000114 ) ;
#1337=VECTOR ( 'NONE', #51375, 999.9999999999998863 ) ;
#1338=ORIENTED_EDGE ( 'NONE', *, *, #28103, .T. ) ;
#1339=CARTESIAN_POINT ( 'NONE',  ( -2.056461029976381472, 6.659969651376628441, 4.017172877417169552 ) ) ;
#1340=LINE ( 'NONE', #54159, #41235 ) ;
#1341=CARTESIAN_POINT ( 'NONE',  ( -18.67775241435682432, 0.000000000000000000, 4.136394454059623804 ) ) ;
#1342=DIRECTION ( 'NONE',  ( 0.005002170337468016433, -0.7660444431189770143, -0.6427681459581293666 ) ) ;
#1343=DIRECTION ( 'NONE',  ( 0.007781995580012663651, 0.000000000000000000, -0.9999697198139515519 ) ) ;
#1344=CARTESIAN_POINT ( 'NONE',  ( -21.88142947281899708, -3.917936722690662066, 5.255808726792642105 ) ) ;
#1345=EDGE_CURVE ( 'NONE', #55101, #40102, #9409, .T. ) ;
#1346=DIRECTION ( 'NONE',  ( 0.005961354470445682716, -0.6427876096865404731, -0.7660212471507180654 ) ) ;
#1347=VECTOR ( 'NONE', #7334, 1000.000000000000227 ) ;
#1348=DIRECTION ( 'NONE',  ( -0.005961354470445682716, -0.6427876096865404731, 0.7660212471507180654 ) ) ;
#1349=VECTOR ( 'NONE', #22887, 1000.000000000000227 ) ;
#1350=CARTESIAN_POINT ( 'NONE',  ( -14.60466426183518607, 0.000000000000000000, 4.337418181458335020 ) ) ;
#1351=ADVANCED_FACE ( 'NONE', ( #9975 ), #36114, .F. ) ;
#1353=VERTEX_POINT ( 'NONE', #53417 ) ;
#1354=ADVANCED_FACE ( 'NONE', ( #9716 ), #13947, .F. ) ;
#1355=VECTOR ( 'NONE', #9417, 1000.000000000000114 ) ;
#1356=EDGE_CURVE ( 'NONE', #43988, #8731, #22491, .T. ) ;
#1357=ADVANCED_FACE ( 'NONE', ( #52312 ), #31828, .F. ) ;
#1358=VERTEX_POINT ( 'NONE', #48600 ) ;
#1359=EDGE_LOOP ( 'NONE', ( #10415, #15887, #48999, #40635 ) ) ;
#1360=VECTOR ( 'NONE', #27646, 1000.000000000000000 ) ;
#1361=VECTOR ( 'NONE', #49736, 999.9999999999998863 ) ;
#1362=ORIENTED_EDGE ( 'NONE', *, *, #53870, .F. ) ;
#1363=AXIS2_PLACEMENT_3D ( 'NONE', #48257, #22158, #39494 ) ;
#1365=PLANE ( 'NONE',  #48657 ) ;
#1366=CARTESIAN_POINT ( 'NONE',  ( -14.60622066095118576, 0.000000000000000000, 4.537412125421123932 ) ) ;
#1367=VECTOR ( 'NONE', #37803, 1000.000000000000227 ) ;
#1368=ORIENTED_EDGE ( 'NONE', *, *, #8155, .F. ) ;
#1369=VERTEX_POINT ( 'NONE', #34996 ) ;
#1371=EDGE_CURVE ( 'NONE', #27421, #2828, #623, .T. ) ;
#1372=VECTOR ( 'NONE', #49413, 1000.000000000000227 ) ;
#1373=VECTOR ( 'NONE', #51812, 999.9999999999998863 ) ;
#1374=CARTESIAN_POINT ( 'NONE',  ( -9.033451952363439119, 0.000000000000000000, 4.950112769895002707 ) ) ;
#1375=CARTESIAN_POINT ( 'NONE',  ( -18.31855849401743086, 0.000000000000000000, 3.897176644277617896 ) ) ;
#1376=DIRECTION ( 'NONE',  ( 0.005961354470445682716, -0.6427876096865404731, -0.7660212471507180654 ) ) ;
#1377=ORIENTED_EDGE ( 'NONE', *, *, #26173, .T. ) ;
#1378=LINE ( 'NONE', #4800, #8362 ) ;
#1380=DIRECTION ( 'NONE',  ( 0.7660212471507180654, -0.6427876096865404731, 0.005961354470445141482 ) ) ;
#1381=DIRECTION ( 'NONE',  ( 0.9321478471874540261, 0.000000000000000000, -0.3620778797217456546 ) ) ;
#1382=AXIS2_PLACEMENT_3D ( 'NONE', #22527, #31018, #9452 ) ;
#1383=CARTESIAN_POINT ( 'NONE',  ( -12.33850799832341849, 0.000000000000000000, 11.68350162852954632 ) ) ;
#1384=LINE ( 'NONE', #9925, #1544 ) ;
#1385=LINE ( 'NONE', #14460, #45774 ) ;
#1386=DIRECTION ( 'NONE',  ( 0.9999697198139515519, 0.000000000000000000, 0.007781995580013368816 ) ) ;
#1387=CARTESIAN_POINT ( 'NONE',  ( -13.07066190154808361, 0.000000000000000000, 12.04713590736729678 ) ) ;
#1388=VECTOR ( 'NONE', #53123, 999.9999999999998863 ) ;
#1389=ORIENTED_EDGE ( 'NONE', *, *, #17850, .T. ) ;
#1390=DIRECTION ( 'NONE',  ( 0.9999697198139515519, 0.000000000000000000, 0.007781995580013368816 ) ) ;
#1391=ORIENTED_EDGE ( 'NONE', *, *, #47578, .T. ) ;
#1392=VECTOR ( 'NONE', #54145, 999.9999999999998863 ) ;
#1393=PLANE ( 'NONE',  #27403 ) ;
#1394=LINE ( 'NONE', #31785, #45045 ) ;
#1395=LINE ( 'NONE', #27519, #14987 ) ;
#1396=DIRECTION ( 'NONE',  ( -0.005002170337468016433, -0.7660444431189770143, 0.6427681459581293666 ) ) ;
#1397=ADVANCED_FACE ( 'NONE', ( #10249 ), #27572, .F. ) ;
#1398=VECTOR ( 'NONE', #29174, 999.9999999999998863 ) ;
#1399=CARTESIAN_POINT ( 'NONE',  ( -17.46532115785441519, 0.000000000000000000, 13.67492996699914265 ) ) ;
#1400=PLANE ( 'NONE',  #3189 ) ;
#1401=FACE_OUTER_BOUND ( 'NONE', #53127, .T. ) ;
#1402=CARTESIAN_POINT ( 'NONE',  ( -14.20280369269832832, 0.000000000000000000, 12.40765738797303719 ) ) ;
#1403=AXIS2_PLACEMENT_3D ( 'NONE', #38051, #46555, #50813 ) ;
#1404=AXIS2_PLACEMENT_3D ( 'NONE', #55284, #38238, #29759 ) ;
#1406=DIRECTION ( 'NONE',  ( 0.007781995580012662783, 0.000000000000000000, -0.9999697198139514409 ) ) ;
#1407=ORIENTED_EDGE ( 'NONE', *, *, #43869, .T. ) ;
#1408=CARTESIAN_POINT ( 'NONE',  ( -14.46888367232926420, 0.000000000000000000, 12.59025272694991315 ) ) ;
#1410=CARTESIAN_POINT ( 'NONE',  ( 2.072287782118878319, 0.000000000000000000, -2.950529333540147015 ) ) ;
#1411=DIRECTION ( 'NONE',  ( -0.9999697198139514409, -0.000000000000000000, -0.007781995580013368816 ) ) ;
#1412=VECTOR ( 'NONE', #29489, 999.9999999999998863 ) ;
#1414=VECTOR ( 'NONE', #33309, 1000.000000000000227 ) ;
#1415=CARTESIAN_POINT ( 'NONE',  ( -16.44346267919223692, 1.095915999411505526, 3.034165600300908316 ) ) ;
#1416=AXIS2_PLACEMENT_3D ( 'NONE', #28813, #46114, #2932 ) ;
#1417=EDGE_CURVE ( 'NONE', #18340, #51526, #19618, .T. ) ;
#1418=PLANE ( 'NONE',  #2434 ) ;
#1419=ADVANCED_FACE ( 'NONE', ( #45430 ), #46018, .F. ) ;
#1420=DIRECTION ( 'NONE',  ( -0.005961354470445682716, -0.6427876096865404731, 0.7660212471507180654 ) ) ;
#1421=VERTEX_POINT ( 'NONE', #36366 ) ;
#1422=VECTOR ( 'NONE', #47528, 999.9999999999998863 ) ;
#1423=AXIS2_PLACEMENT_3D ( 'NONE', #1553, #32215, #31919 ) ;
#1424=ORIENTED_EDGE ( 'NONE', *, *, #42445, .T. ) ;
#1425=DIRECTION ( 'NONE',  ( -0.3620778797217455991, 0.000000000000000000, -0.9321478471874540261 ) ) ;
#1426=LINE ( 'NONE', #22468, #34979 ) ;
#1427=EDGE_CURVE ( 'NONE', #54304, #8877, #15346, .T. ) ;
#1428=VERTEX_POINT ( 'NONE', #53969 ) ;
#1429=EDGE_CURVE ( 'NONE', #4025, #83, #14793, .T. ) ;
#1430=CARTESIAN_POINT ( 'NONE',  ( -16.06709938707323460, 0.000000000000000000, 13.13181314741652628 ) ) ;
#1431=EDGE_LOOP ( 'NONE', ( #16342, #44010, #36700, #33808 ) ) ;
#1432=DIRECTION ( 'NONE',  ( 0.005961354470445682716, -0.6427876096865404731, -0.7660212471507180654 ) ) ;
#1433=ADVANCED_FACE ( 'NONE', ( #11069 ), #23584, .F. ) ;
#1434=VECTOR ( 'NONE', #38934, 1000.000000000000227 ) ;
#1435=VERTEX_POINT ( 'NONE', #54250 ) ;
#1436=ORIENTED_EDGE ( 'NONE', *, *, #48216, .T. ) ;
#1437=VERTEX_POINT ( 'NONE', #50556 ) ;
#1438=AXIS2_PLACEMENT_3D ( 'NONE', #9953, #1699, #27259 ) ;
#1439=PLANE ( 'NONE',  #39281 ) ;
#1440=LINE ( 'NONE', #54237, #2392 ) ;
#1441=AXIS2_PLACEMENT_3D ( 'NONE', #56035, #34438, #47497 ) ;
#1442=CARTESIAN_POINT ( 'NONE',  ( -15.53393805551735518, 0.000000000000000000, 4.330186357922316986 ) ) ;
#1443=EDGE_CURVE ( 'NONE', #5744, #52834, #50257, .T. ) ;
#1444=DIRECTION ( 'NONE',  ( 0.005002170337468016433, -0.7660444431189770143, -0.6427681459581293666 ) ) ;
#1445=ORIENTED_EDGE ( 'NONE', *, *, #245, .T. ) ;
#1446=VERTEX_POINT ( 'NONE', #24416 ) ;
#1447=EDGE_CURVE ( 'NONE', #35209, #22415, #6545, .T. ) ;
#1448=VECTOR ( 'NONE', #51351, 1000.000000000000227 ) ;
#1449=VECTOR ( 'NONE', #30800, 999.9999999999998863 ) ;
#1451=VERTEX_POINT ( 'NONE', #20143 ) ;
#1452=CARTESIAN_POINT ( 'NONE',  ( -18.66354898467281132, 0.000000000000000000, 14.21960318569776582 ) ) ;
#1453=ORIENTED_EDGE ( 'NONE', *, *, #9204, .F. ) ;
#1454=CARTESIAN_POINT ( 'NONE',  ( -10.27421835998572064, 0.000000000000000000, 10.96090226820206048 ) ) ;
#1455=LINE ( 'NONE', #26729, #38520 ) ;
#1457=ORIENTED_EDGE ( 'NONE', *, *, #49593, .F. ) ;
#1458=AXIS2_PLACEMENT_3D ( 'NONE', #12983, #17516, #34849 ) ;
#1460=EDGE_LOOP ( 'NONE', ( #55447, #31584, #11570, #21958 ) ) ;
#1461=VECTOR ( 'NONE', #27925, 1000.000000000000227 ) ;
#1462=CARTESIAN_POINT ( 'NONE',  ( -19.45503627000849889, 0.000000000000000000, 7.556996783084074742 ) ) ;
#1463=VECTOR ( 'NONE', #33129, 1000.000000000000000 ) ;
#1464=EDGE_LOOP ( 'NONE', ( #52364, #1521, #20842, #38091 ) ) ;
#1465=LINE ( 'NONE', #326, #4980 ) ;
#1466=DIRECTION ( 'NONE',  ( 0.5449076811759707706, 0.6444004775717708799, -0.5364919789714476250 ) ) ;
#1467=CARTESIAN_POINT ( 'NONE',  ( -12.60458797795435615, 0.000000000000000000, 11.86609696750642229 ) ) ;
#1468=EDGE_LOOP ( 'NONE', ( #876, #46291, #23991, #39804 ) ) ;
#1469=CARTESIAN_POINT ( 'NONE',  ( -17.62242848232430248, -0.5179957512181546653, 3.709944023437250937 ) ) ;
#1470=CARTESIAN_POINT ( 'NONE',  ( -17.68167742291825917, 0.000000000000000000, 7.468134768223175790 ) ) ;
#1471=EDGE_CURVE ( 'NONE', #33376, #28974, #15086, .T. ) ;
#1472=CARTESIAN_POINT ( 'NONE',  ( -11.40636015113596180, 0.000000000000000000, 11.32142374880780089 ) ) ;
#1473=DIRECTION ( 'NONE',  ( -0.7660212471507179544, -0.6427876096865405842, -0.005961354470445141482 ) ) ;
#1474=DIRECTION ( 'NONE',  ( 0.7660212471507180654, -0.6427876096865404731, 0.005961354470445141482 ) ) ;
#1475=VECTOR ( 'NONE', #48134, 1000.000000000000227 ) ;
#1476=DIRECTION ( 'NONE',  ( 0.005002170337468016433, -0.7660444431189770143, -0.6427681459581293666 ) ) ;
#1477=VERTEX_POINT ( 'NONE', #37476 ) ;
#1478=DIRECTION ( 'NONE',  ( 0.7660212471507180654, -0.6427876096865404731, 0.005961354470445141482 ) ) ;
#1479=DIRECTION ( 'NONE',  ( 0.005002170337468016433, -0.7660444431189770143, -0.6427681459581293666 ) ) ;
#1481=ORIENTED_EDGE ( 'NONE', *, *, #25153, .F. ) ;
#1482=CARTESIAN_POINT ( 'NONE',  ( -13.53673582514181106, 0.000000000000000000, 12.22817484722816772 ) ) ;
#1483=DIRECTION ( 'NONE',  ( 0.9999697198139515519, 0.000000000000000000, 0.007781995580013368816 ) ) ;
#1484=VECTOR ( 'NONE', #18223, 999.9999999999998863 ) ;
#1485=ORIENTED_EDGE ( 'NONE', *, *, #19321, .F. ) ;
#1486=EDGE_CURVE ( 'NONE', #3168, #13096, #49718, .T. ) ;
#1487=EDGE_CURVE ( 'NONE', #51971, #54306, #32119, .T. ) ;
#1488=VECTOR ( 'NONE', #8921, 1000.000000000000227 ) ;
#1489=LINE ( 'NONE', #5748, #12278 ) ;
#1490=CARTESIAN_POINT ( 'NONE',  ( -12.28303617674575676, 0.000000000000000000, 4.555491684261172125 ) ) ;
#1491=EDGE_CURVE ( 'NONE', #22884, #49289, #1983, .T. ) ;
#1492=CARTESIAN_POINT ( 'NONE',  ( 2.072287782118878319, 0.000000000000000000, -2.950529333540147015 ) ) ;
#1493=ORIENTED_EDGE ( 'NONE', *, *, #46265, .F. ) ;
#1494=VECTOR ( 'NONE', #9598, 1000.000000000000227 ) ;
#1495=VERTEX_POINT ( 'NONE', #32662 ) ;
#1496=FACE_OUTER_BOUND ( 'NONE', #15908, .T. ) ;
#1497=DIRECTION ( 'NONE',  ( 0.6427681459581294776, -0.7660444431189769032, 0.005002170337467562802 ) ) ;
#1499=DIRECTION ( 'NONE',  ( 0.007781995580012663651, 0.000000000000000000, -0.9999697198139515519 ) ) ;
#1500=AXIS2_PLACEMENT_3D ( 'NONE', #43014, #38774, #50692 ) ;
#1501=DIRECTION ( 'NONE',  ( 0.007781995580012663651, -3.146120232559066537E-19, -0.9999697198139514409 ) ) ;
#1502=ORIENTED_EDGE ( 'NONE', *, *, #53584, .F. ) ;
#1503=EDGE_CURVE ( 'NONE', #30960, #29943, #6837, .T. ) ;
#1504=LINE ( 'NONE', #1200, #53029 ) ;
#1505=ORIENTED_EDGE ( 'NONE', *, *, #3606, .T. ) ;
#1506=DIRECTION ( 'NONE',  ( 0.000000000000000000, 1.000000000000000000, 0.000000000000000000 ) ) ;
#1507=AXIS2_PLACEMENT_3D ( 'NONE', #20130, #46845, #16175 ) ;
#1508=ADVANCED_FACE ( 'NONE', ( #2560 ), #19881, .F. ) ;
#1510=CARTESIAN_POINT ( 'NONE',  ( -20.03477888584858846, 2.553033558614007603, 8.853472636018112851 ) ) ;
#1511=ORIENTED_EDGE ( 'NONE', *, *, #27999, .T. ) ;
#1512=EDGE_CURVE ( 'NONE', #29979, #50929, #15906, .T. ) ;
#1513=FACE_OUTER_BOUND ( 'NONE', #55549, .T. ) ;
#1514=DIRECTION ( 'NONE',  ( 0.6427681459581294776, -0.7660444431189769032, 0.005002170337467562802 ) ) ;
#1515=LINE ( 'NONE', #26231, #7564 ) ;
#1516=EDGE_LOOP ( 'NONE', ( #28306, #44050, #3769, #25827 ) ) ;
#1517=EDGE_CURVE ( 'NONE', #28225, #21479, #11655, .T. ) ;
#1518=DIRECTION ( 'NONE',  ( -0.6427681459581293666, -0.7660444431189770143, -0.005002170337467561935 ) ) ;
#1519=ORIENTED_EDGE ( 'NONE', *, *, #39376, .F. ) ;
#1520=VECTOR ( 'NONE', #41202, 1000.000000000000227 ) ;
#1521=ORIENTED_EDGE ( 'NONE', *, *, #45656, .F. ) ;
#1522=ORIENTED_EDGE ( 'NONE', *, *, #10895, .F. ) ;
#1523=CARTESIAN_POINT ( 'NONE',  ( -13.43725194175183901, 0.2864062442990034651, 2.570847542666338192 ) ) ;
#1524=EDGE_LOOP ( 'NONE', ( #27416, #46123, #51377, #53382 ) ) ;
#1525=CARTESIAN_POINT ( 'NONE',  ( -19.84496024468298003, -5.375054281893166142, 4.418285240812005910 ) ) ;
#1526=ORIENTED_EDGE ( 'NONE', *, *, #11212, .T. ) ;
#1527=DIRECTION ( 'NONE',  ( 0.007781995580012663651, -3.146120232559066537E-19, -0.9999697198139514409 ) ) ;
#1528=CARTESIAN_POINT ( 'NONE',  ( -21.47341775636118655, -0.1191753592594197858, 5.122631121243466090 ) ) ;
#1530=AXIS2_PLACEMENT_3D ( 'NONE', #51224, #50923, #33906 ) ;
#1531=CARTESIAN_POINT ( 'NONE',  ( -9.777102069609235002, 0.000000000000000000, 6.790985861763807030 ) ) ;
#1532=ORIENTED_EDGE ( 'NONE', *, *, #1719, .F. ) ;
#1534=LINE ( 'NONE', #39869, #13793 ) ;
#1535=FACE_OUTER_BOUND ( 'NONE', #7711, .T. ) ;
#1536=CARTESIAN_POINT ( 'NONE',  ( -22.40634380310664397, 0.000000000000000000, 5.584705972946605534 ) ) ;
#1537=FACE_OUTER_BOUND ( 'NONE', #25561, .T. ) ;
#1538=CARTESIAN_POINT ( 'NONE',  ( -17.74560456716937296, 0.000000000000000000, 3.774316574337878372 ) ) ;
#1539=PLANE ( 'NONE',  #18308 ) ;
#1541=ORIENTED_EDGE ( 'NONE', *, *, #2850, .F. ) ;
#1542=ADVANCED_FACE ( 'NONE', ( #25538 ), #55356, .F. ) ;
#1543=ORIENTED_EDGE ( 'NONE', *, *, #7873, .F. ) ;
#1544=VECTOR ( 'NONE', #27226, 1000.000000000000114 ) ;
#1545=LINE ( 'NONE', #15176, #16486 ) ;
#1546=CARTESIAN_POINT ( 'NONE',  ( -6.389729114256917697, 6.241674792422348794, 5.700361359755299340 ) ) ;
#1547=EDGE_CURVE ( 'NONE', #35486, #53425, #42856, .T. ) ;
#1548=CARTESIAN_POINT ( 'NONE',  ( -20.31146284415708791, 2.876837460659007473, 9.492363449552833288 ) ) ;
#1549=VECTOR ( 'NONE', #27844, 999.9999999999998863 ) ;
#1550=CARTESIAN_POINT ( 'NONE',  ( -19.85946097050258174, -2.622721114510660367, 4.511731653252694763 ) ) ;
#1553=CARTESIAN_POINT ( 'NONE',  ( -15.88130887279446490, 0.000000000000000000, 3.050160814894388839 ) ) ;
#1555=ORIENTED_EDGE ( 'NONE', *, *, #5021, .T. ) ;
#1556=LINE ( 'NONE', #14052, #54697 ) ;
#1557=DIRECTION ( 'NONE',  ( -0.5364919789714478471, 0.6444004775717705469, -0.5449076811759709926 ) ) ;
#1558=VERTEX_POINT ( 'NONE', #16745 ) ;
#1559=EDGE_CURVE ( 'NONE', #32592, #16959, #50811, .T. ) ;
#1560=ADVANCED_FACE ( 'NONE', ( #7372 ), #3960, .F. ) ;
#1561=EDGE_CURVE ( 'NONE', #35486, #15388, #38900, .T. ) ;
#1563=CARTESIAN_POINT ( 'NONE',  ( -12.15271748404464880, 0.000000000000000000, 1.601849296007406664 ) ) ;
#1564=CARTESIAN_POINT ( 'NONE',  ( -26.13337879274045505, 0.000000000000000000, 6.833023547870798353 ) ) ;
#1565=ADVANCED_FACE ( 'NONE', ( #21285 ), #16449, .F. ) ;
#1566=PLANE ( 'NONE',  #2395 ) ;
#1567=DIRECTION ( 'NONE',  ( -0.9999697198139514409, -0.000000000000000000, -0.007781995580013368816 ) ) ;
#1568=EDGE_LOOP ( 'NONE', ( #10952, #49342, #29271, #51314 ) ) ;
#1570=DIRECTION ( 'NONE',  ( 0.6427681459581294776, -0.7660444431189769032, 0.005002170337467562802 ) ) ;
#1571=DIRECTION ( 'NONE',  ( 0.000000000000000000, -0.000000000000000000, -1.000000000000000000 ) ) ;
#1572=DIRECTION ( 'NONE',  ( 0.6427681459581294776, -0.7660444431189769032, 0.005002170337467562802 ) ) ;
#1573=CARTESIAN_POINT ( 'NONE',  ( -26.13493519185646008, 0.000000000000000000, 7.033017491833586377 ) ) ;
#1575=VERTEX_POINT ( 'NONE', #34083 ) ;
#1576=CARTESIAN_POINT ( 'NONE',  ( -15.70074161002902180, -1.003701604285657911, 2.947999021814709852 ) ) ;
#1577=CARTESIAN_POINT ( 'NONE',  ( -29.86197018149027116, 0.000000000000000000, 8.281335066757780083 ) ) ;
#1578=EDGE_CURVE ( 'NONE', #13246, #30223, #12504, .T. ) ;
#1579=DIRECTION ( 'NONE',  ( 0.5364919789714477361, 0.6444004775717706579, 0.5449076811759711036 ) ) ;
#1580=VECTOR ( 'NONE', #33352, 1000.000000000000000 ) ;
#1581=DIRECTION ( 'NONE',  ( -0.9999697198139514409, -0.000000000000000000, -0.007781995580013368816 ) ) ;
#1582=ORIENTED_EDGE ( 'NONE', *, *, #44254, .F. ) ;
#1583=EDGE_CURVE ( 'NONE', #28250, #41541, #34356, .T. ) ;
#1584=CARTESIAN_POINT ( 'NONE',  ( -24.26908309836554878, 0.000000000000000000, 6.108867788427308376 ) ) ;
#1585=EDGE_LOOP ( 'NONE', ( #23253, #50007, #8190, #13525 ) ) ;
#1586=LINE ( 'NONE', #52975, #43142 ) ;
#1587=LINE ( 'NONE', #18914, #3012 ) ;
#1588=VERTEX_POINT ( 'NONE', #29546 ) ;
#1589=ADVANCED_FACE ( 'NONE', ( #55100 ), #12204, .F. ) ;
#1590=VECTOR ( 'NONE', #12067, 1000.000000000000227 ) ;
#1591=CARTESIAN_POINT ( 'NONE',  ( -21.64383464956858560, 4.981562823951511731, 13.46411479766764785 ) ) ;
#1592=ORIENTED_EDGE ( 'NONE', *, *, #6327, .F. ) ;
#1593=EDGE_CURVE ( 'NONE', #30130, #34473, #3113, .T. ) ;
#1594=ORIENTED_EDGE ( 'NONE', *, *, #32462, .T. ) ;
#1595=ORIENTED_EDGE ( 'NONE', *, *, #40065, .F. ) ;
#1596=DIRECTION ( 'NONE',  ( 0.005002170337468016433, -0.7660444431189770143, -0.6427681459581293666 ) ) ;
#1597=ORIENTED_EDGE ( 'NONE', *, *, #51155, .F. ) ;
#1598=EDGE_LOOP ( 'NONE', ( #12539, #23880, #1828, #12173 ) ) ;
#1600=FACE_OUTER_BOUND ( 'NONE', #30295, .T. ) ;
#1601=ORIENTED_EDGE ( 'NONE', *, *, #54889, .T. ) ;
#1602=EDGE_LOOP ( 'NONE', ( #43725, #53528, #14096, #9125 ) ) ;
#1603=LINE ( 'NONE', #18643, #29493 ) ;
#1604=VERTEX_POINT ( 'NONE', #46550 ) ;
#1605=ORIENTED_EDGE ( 'NONE', *, *, #16748, .T. ) ;
#1606=CARTESIAN_POINT ( 'NONE',  ( 2.072287782118878319, 0.000000000000000000, -2.950529333540147015 ) ) ;
#1607=CARTESIAN_POINT ( 'NONE',  ( -17.65868499487599763, 0.000000000000000000, 4.513657142161060065 ) ) ;
#1608=CARTESIAN_POINT ( 'NONE',  ( 2.072287782118878319, 0.000000000000000000, -2.950529333540147015 ) ) ;
#1609=DIRECTION ( 'NONE',  ( 0.005961354470445682716, -0.6427876096865404731, -0.7660212471507180654 ) ) ;
#1610=EDGE_LOOP ( 'NONE', ( #22629, #50899, #33846, #1644 ) ) ;
#1611=CARTESIAN_POINT ( 'NONE',  ( -20.04277098628171672, 4.819660872929012463, 4.313452222389104307 ) ) ;
#1612=ORIENTED_EDGE ( 'NONE', *, *, #40578, .F. ) ;
#1613=DIRECTION ( 'NONE',  ( 0.5364919789714477361, 0.6444004775717706579, 0.5449076811759711036 ) ) ;
#1614=FACE_OUTER_BOUND ( 'NONE', #10339, .T. ) ;
#1615=VECTOR ( 'NONE', #55757, 999.9999999999998863 ) ;
#1616=CARTESIAN_POINT ( 'NONE',  ( -19.60912206198628027, -0.1191753592594197858, 4.398475361799976113 ) ) ;
#1617=DIRECTION ( 'NONE',  ( -0.005961354470445682716, -0.6427876096865404731, 0.7660212471507180654 ) ) ;
#1618=CARTESIAN_POINT ( 'NONE',  ( -13.09143909235258363, -0.1191753592594181482, 1.866785954948907866 ) ) ;
#1619=LINE ( 'NONE', #17833, #9611 ) ;
#1620=EDGE_LOOP ( 'NONE', ( #6107, #50680, #51894, #38119 ) ) ;
#1621=CARTESIAN_POINT ( 'NONE',  ( -10.47421230394850866, 0.000000000000000000, 10.95934586908605723 ) ) ;
#1622=EDGE_LOOP ( 'NONE', ( #44451, #53456, #18787, #13593 ) ) ;
#1623=EDGE_CURVE ( 'NONE', #29206, #2049, #17289, .T. ) ;
#1624=EDGE_CURVE ( 'NONE', #10121, #53596, #17042, .T. ) ;
#1625=VECTOR ( 'NONE', #36384, 1000.000000000000227 ) ;
#1626=DIRECTION ( 'NONE',  ( -0.5449076811759708816, 0.6444004775717707689, 0.5364919789714475140 ) ) ;
#1627=CARTESIAN_POINT ( 'NONE',  ( -12.19950532623806083, -0.1191753592594194527, 6.672131131384362313 ) ) ;
#1628=DIRECTION ( 'NONE',  ( 0.007781995580012663651, -3.146120232559066537E-19, -0.9999697198139514409 ) ) ;
#1629=DIRECTION ( 'NONE',  ( 0.5364919789714477361, 0.6444004775717706579, 0.5449076811759711036 ) ) ;
#1630=EDGE_CURVE ( 'NONE', #15384, #51326, #24995, .T. ) ;
#1631=FACE_OUTER_BOUND ( 'NONE', #54256, .T. ) ;
#1633=EDGE_LOOP ( 'NONE', ( #50284, #3568, #21928 ) ) ;
#1635=CARTESIAN_POINT ( 'NONE',  ( -9.601946002769009780, -9.248839861434568377, 0.5113483352705097129 ) ) ;
#1637=LINE ( 'NONE', #36281, #49116 ) ;
#1638=DIRECTION ( 'NONE',  ( 0.9999697198139515519, 0.000000000000000000, 0.007781995580013368816 ) ) ;
#1639=FACE_OUTER_BOUND ( 'NONE', #12689, .T. ) ;
#1640=LINE ( 'NONE', #18969, #39650 ) ;
#1641=CARTESIAN_POINT ( 'NONE',  ( -20.54204810873173415, 0.000000000000000000, 4.860550213503115558 ) ) ;
#1642=ORIENTED_EDGE ( 'NONE', *, *, #33678, .F. ) ;
#1643=EDGE_CURVE ( 'NONE', #21963, #1847, #29822, .T. ) ;
#1644=ORIENTED_EDGE ( 'NONE', *, *, #32334, .T. ) ;
#1645=VERTEX_POINT ( 'NONE', #42583 ) ;
#1646=ORIENTED_EDGE ( 'NONE', *, *, #2853, .T. ) ;
#1647=EDGE_CURVE ( 'NONE', #9132, #31598, #12762, .T. ) ;
#1648=ORIENTED_EDGE ( 'NONE', *, *, #21805, .T. ) ;
#1649=CARTESIAN_POINT ( 'NONE',  ( -16.53317331066696383, 0.000000000000000000, 13.31285208727739899 ) ) ;
#1650=FACE_OUTER_BOUND ( 'NONE', #10084, .T. ) ;
#1651=VECTOR ( 'NONE', #21471, 999.9999999999998863 ) ;
#1652=ORIENTED_EDGE ( 'NONE', *, *, #31807, .T. ) ;
#1653=ORIENTED_EDGE ( 'NONE', *, *, #47917, .F. ) ;
#1654=EDGE_CURVE ( 'NONE', #18340, #41698, #56203, .T. ) ;
#1655=ORIENTED_EDGE ( 'NONE', *, *, #42198, .T. ) ;
#1657=LINE ( 'NONE', #15534, #41867 ) ;
#1658=CARTESIAN_POINT ( 'NONE',  ( -19.60990026154428278, 0.000000000000000000, 4.498472333781370125 ) ) ;
#1659=ORIENTED_EDGE ( 'NONE', *, *, #8572, .F. ) ;
#1660=CARTESIAN_POINT ( 'NONE',  ( -14.01701317841955508, 0.000000000000000000, 2.326005055450897085 ) ) ;
#1661=VERTEX_POINT ( 'NONE', #52502 ) ;
#1662=CARTESIAN_POINT ( 'NONE',  ( -16.81190032086591302, 0.000000000000000000, 3.212244750653343583 ) ) ;
#1663=FACE_OUTER_BOUND ( 'NONE', #52430, .T. ) ;
#1664=LINE ( 'NONE', #819, #18243 ) ;
#1665=CARTESIAN_POINT ( 'NONE',  ( -21.47263955680318404, 0.000000000000000000, 5.022634149262071190 ) ) ;
#1666=CARTESIAN_POINT ( 'NONE',  ( -18.15206242676991266, 0.000000000000000000, 8.203138262970696815 ) ) ;
#1667=CARTESIAN_POINT ( 'NONE',  ( -12.15193928448664629, -0.1191753592594197858, 1.501852324026012209 ) ) ;
#1669=FACE_OUTER_BOUND ( 'NONE', #21654, .T. ) ;
#1670=ORIENTED_EDGE ( 'NONE', *, *, #52960, .T. ) ;
#1671=CARTESIAN_POINT ( 'NONE',  ( -13.11440885239381693, -0.1191753592594183703, 4.818350791559519841 ) ) ;
#1672=ADVANCED_FACE ( 'NONE', ( #1079 ), #17888, .F. ) ;
#1673=ORIENTED_EDGE ( 'NONE', *, *, #54482, .F. ) ;
#1674=EDGE_CURVE ( 'NONE', #6876, #28453, #39741, .T. ) ;
#1675=CARTESIAN_POINT ( 'NONE',  ( -13.31607370880347929, -3.108426967578159061, 6.955805194728735152 ) ) ;
#1676=DIRECTION ( 'NONE',  ( -0.5364919789714478471, 0.6444004775717705469, -0.5449076811759709926 ) ) ;
#1677=FACE_OUTER_BOUND ( 'NONE', #42898, .T. ) ;
#1678=DIRECTION ( 'NONE',  ( 0.007781995580012663651, 0.000000000000000000, -0.9999697198139515519 ) ) ;
#1679=CARTESIAN_POINT ( 'NONE',  ( -13.48270103031678957, 0.000000000000000000, 5.284819754588673923 ) ) ;
#1680=CARTESIAN_POINT ( 'NONE',  ( -23.33693525117809386, 0.000000000000000000, 5.746789908705562944 ) ) ;
#1681=ADVANCED_FACE ( 'NONE', ( #18414 ), #9333, .F. ) ;
#1682=EDGE_CURVE ( 'NONE', #1080, #35417, #22122, .T. ) ;
#1683=DIRECTION ( 'NONE',  ( 0.7660212471507180654, -0.6427876096865404731, 0.005961354470445141482 ) ) ;
#1684=DIRECTION ( 'NONE',  ( 0.7660212471507180654, -0.6427876096865404731, 0.005961354470445141482 ) ) ;
#1685=FACE_OUTER_BOUND ( 'NONE', #47461, .T. ) ;
#1686=ORIENTED_EDGE ( 'NONE', *, *, #18158, .F. ) ;
#1687=LINE ( 'NONE', #31535, #13941 ) ;
#1688=DIRECTION ( 'NONE',  ( -0.005002170337468016433, -0.7660444431189770143, 0.6427681459581293666 ) ) ;
#1690=FACE_OUTER_BOUND ( 'NONE', #55480, .T. ) ;
#1692=DIRECTION ( 'NONE',  ( 0.007781995580012662783, 0.000000000000000000, -0.9999697198139514409 ) ) ;
#1693=LINE ( 'NONE', #31541, #10608 ) ;
#1694=CARTESIAN_POINT ( 'NONE',  ( -28.93137873341882127, 0.000000000000000000, 8.119251130998824451 ) ) ;
#1695=ADVANCED_FACE ( 'NONE', ( #9918 ), #31506, .F. ) ;
#1696=ORIENTED_EDGE ( 'NONE', *, *, #17502, .T. ) ;
#1697=ORIENTED_EDGE ( 'NONE', *, *, #15275, .T. ) ;
#1698=FACE_OUTER_BOUND ( 'NONE', #9318, .T. ) ;
#1699=DIRECTION ( 'NONE',  ( -0.005961354470445682716, -0.6427876096865404731, 0.7660212471507180654 ) ) ;
#1700=ORIENTED_EDGE ( 'NONE', *, *, #48020, .F. ) ;
#1701=CARTESIAN_POINT ( 'NONE',  ( -19.60990026154428278, 0.000000000000000000, 4.498472333781370125 ) ) ;
#1702=VERTEX_POINT ( 'NONE', #44276 ) ;
#1704=ORIENTED_EDGE ( 'NONE', *, *, #38915, .T. ) ;
#1705=ORIENTED_EDGE ( 'NONE', *, *, #38327, .F. ) ;
#1706=ORIENTED_EDGE ( 'NONE', *, *, #33420, .F. ) ;
#1707=DIRECTION ( 'NONE',  ( 0.9999697198139515519, 0.000000000000000000, 0.007781995580013368816 ) ) ;
#1708=LINE ( 'NONE', #19605, #26848 ) ;
#1709=DIRECTION ( 'NONE',  ( 0.6427681459581294776, -0.7660444431189769032, 0.005002170337467562802 ) ) ;
#1710=EDGE_LOOP ( 'NONE', ( #9317, #630, #4247, #49002 ) ) ;
#1711=EDGE_CURVE ( 'NONE', #14416, #38344, #35207, .T. ) ;
#1712=ORIENTED_EDGE ( 'NONE', *, *, #14966, .F. ) ;
#1713=DIRECTION ( 'NONE',  ( -0.5364919789714478471, 0.6444004775717705469, -0.5449076811759709926 ) ) ;
#1714=EDGE_LOOP ( 'NONE', ( #14645, #47327, #53878, #47076 ) ) ;
#1715=FACE_OUTER_BOUND ( 'NONE', #7240, .T. ) ;
#1716=VERTEX_POINT ( 'NONE', #35753 ) ;
#1717=PLANE ( 'NONE',  #40309 ) ;
#1718=DIRECTION ( 'NONE',  ( 0.7660212471507180654, -0.6427876096865404731, 0.005961354470445141482 ) ) ;
#1719=EDGE_CURVE ( 'NONE', #2367, #13439, #22962, .T. ) ;
#1720=EDGE_LOOP ( 'NONE', ( #41677, #45771, #5248, #31726 ) ) ;
#1721=DIRECTION ( 'NONE',  ( 0.5449076811759707706, 0.6444004775717708799, -0.5364919789714476250 ) ) ;
#1722=ORIENTED_EDGE ( 'NONE', *, *, #3150, .T. ) ;
#1723=EDGE_CURVE ( 'NONE', #25204, #23927, #44525, .T. ) ;
#1724=ADVANCED_FACE ( 'NONE', ( #4528 ), #39456, .F. ) ;
#1725=CARTESIAN_POINT ( 'NONE',  ( -26.13415699229845757, -0.1191753592594197858, 6.933020519852192365 ) ) ;
#1726=ORIENTED_EDGE ( 'NONE', *, *, #18025, .T. ) ;
#1727=FACE_OUTER_BOUND ( 'NONE', #754, .T. ) ;
#1728=DIRECTION ( 'NONE',  ( -0.2426528472758542054, 0.7422098413412800966, -0.6246952433987894571 ) ) ;
#1729=DIRECTION ( 'NONE',  ( 0.7660212471507180654, -0.6427876096865404731, 0.005961354470445141482 ) ) ;
#1730=ADVANCED_FACE ( 'NONE', ( #34922 ), #22430, .F. ) ;
#1731=ORIENTED_EDGE ( 'NONE', *, *, #49822, .F. ) ;
#1732=EDGE_CURVE ( 'NONE', #55625, #45339, #1378, .T. ) ;
#1733=DIRECTION ( 'NONE',  ( -0.8531650599175529814, -0.4028455766673920135, 0.3313982828793697877 ) ) ;
#1734=LINE ( 'NONE', #6296, #1520 ) ;
#1735=CARTESIAN_POINT ( 'NONE',  ( -14.55352977697969585, -0.1941918491731554897, 2.528210585817464384 ) ) ;
#1737=PLANE ( 'NONE',  #40329 ) ;
#1738=ADVANCED_FACE ( 'NONE', ( #13345 ), #813, .F. ) ;
#1739=CARTESIAN_POINT ( 'NONE',  ( -12.09166439329881726, 0.000000000000000000, 5.664977193150467549 ) ) ;
#1740=CARTESIAN_POINT ( 'NONE',  ( 3.004435629306332345, 0.000000000000000000, -3.312607213261892003 ) ) ;
#1742=ORIENTED_EDGE ( 'NONE', *, *, #52628, .F. ) ;
#1744=PLANE ( 'NONE',  #25922 ) ;
#1746=EDGE_LOOP ( 'NONE', ( #15239, #15077, #53540, #43309 ) ) ;
#1747=DIRECTION ( 'NONE',  ( -0.5364919789714478471, 0.6444004775717705469, -0.5449076811759709926 ) ) ;
#1748=CARTESIAN_POINT ( 'NONE',  ( -14.03218643205485883, -0.1191753592594197164, 3.333880154992445277 ) ) ;
#1750=ADVANCED_FACE ( 'NONE', ( #47698 ), #36054, .F. ) ;
#1751=DIRECTION ( 'NONE',  ( -0.2426528472758542054, 0.7422098413412800966, -0.6246952433987894571 ) ) ;
#1752=CARTESIAN_POINT ( 'NONE',  ( -15.86710544311044302, 0.000000000000000000, 13.13336954653252953 ) ) ;
#1753=CARTESIAN_POINT ( 'NONE',  ( -27.99923088623136636, 0.000000000000000000, 7.757173251277078130 ) ) ;
#1754=ADVANCED_FACE ( 'NONE', ( #239 ), #30667, .F. ) ;
#1755=ORIENTED_EDGE ( 'NONE', *, *, #44018, .T. ) ;
#1756=ORIENTED_EDGE ( 'NONE', *, *, #38402, .T. ) ;
#1757=CARTESIAN_POINT ( 'NONE',  ( -17.69161723782338669, 0.000000000000000000, 8.745379637291446073 ) ) ;
#1758=CARTESIAN_POINT ( 'NONE',  ( -28.93060053386082231, -0.1191753592594197858, 8.019254159017428663 ) ) ;
#1759=DIRECTION ( 'NONE',  ( 0.007781995580012663651, -3.146120232559066537E-19, -0.9999697198139514409 ) ) ;
#1761=ORIENTED_EDGE ( 'NONE', *, *, #21176, .F. ) ;
#1762=CARTESIAN_POINT ( 'NONE',  ( -19.60834386242827776, 0.000000000000000000, 4.298478389818581213 ) ) ;
#1763=EDGE_LOOP ( 'NONE', ( #33530, #9431, #3298, #1481 ) ) ;
#1764=CARTESIAN_POINT ( 'NONE',  ( -18.68917496928920485, -0.1134144341941974582, 4.041136669461655728 ) ) ;
#1766=ORIENTED_EDGE ( 'NONE', *, *, #22536, .T. ) ;
#1767=CARTESIAN_POINT ( 'NONE',  ( -7.241878385602738888, 3.035725714417215393, 8.349636240898133721 ) ) ;
#1768=CARTESIAN_POINT ( 'NONE',  ( -12.13851405436063047, 0.000000000000000000, 11.68505802764555135 ) ) ;
#1769=FACE_OUTER_BOUND ( 'NONE', #8875, .T. ) ;
#1770=ORIENTED_EDGE ( 'NONE', *, *, #31393, .T. ) ;
#1771=FACE_OUTER_BOUND ( 'NONE', #10275, .T. ) ;
#1772=EDGE_CURVE ( 'NONE', #19751, #25320, #26659, .T. ) ;
#1773=ORIENTED_EDGE ( 'NONE', *, *, #35731, .T. ) ;
#1774=ORIENTED_EDGE ( 'NONE', *, *, #48004, .F. ) ;
#1775=ORIENTED_EDGE ( 'NONE', *, *, #40793, .T. ) ;
#1776=CARTESIAN_POINT ( 'NONE',  ( -16.81345671998191449, 0.000000000000000000, 3.412238694616132495 ) ) ;
#1777=ORIENTED_EDGE ( 'NONE', *, *, #37045, .T. ) ;
#1778=LINE ( 'NONE', #1525, #29366 ) ;
#1779=ORIENTED_EDGE ( 'NONE', *, *, #52572, .F. ) ;
#1780=DIRECTION ( 'NONE',  ( -0.9999697198139514409, -0.000000000000000000, -0.007781995580013368816 ) ) ;
#1781=LINE ( 'NONE', #1528, #50375 ) ;
#1782=EDGE_LOOP ( 'NONE', ( #5617, #52032, #32023, #12756 ) ) ;
#1783=PLANE ( 'NONE',  #41250 ) ;
#1784=ORIENTED_EDGE ( 'NONE', *, *, #40845, .F. ) ;
#1785=EDGE_CURVE ( 'NONE', #28760, #24516, #10176, .T. ) ;
#1786=LINE ( 'NONE', #35607, #52772 ) ;
#1787=DIRECTION ( 'NONE',  ( 0.000000000000000000, -1.000000000000000000, 0.000000000000000000 ) ) ;
#1788=CARTESIAN_POINT ( 'NONE',  ( -9.110551994824897193, 0.000000000000000000, 3.538847790438064411 ) ) ;
#1789=LINE ( 'NONE', #5797, #9397 ) ;
#1790=PLANE ( 'NONE',  #53200 ) ;
#1791=LINE ( 'NONE', #32730, #8345 ) ;
#1792=DIRECTION ( 'NONE',  ( -0.7660212471507179544, -0.6427876096865405842, -0.005961354470445141482 ) ) ;
#1793=ORIENTED_EDGE ( 'NONE', *, *, #49135, .F. ) ;
#1794=EDGE_LOOP ( 'NONE', ( #7989, #15707, #6396, #6214 ) ) ;
#1796=CARTESIAN_POINT ( 'NONE',  ( -19.06409189942038651, 0.000000000000000000, 5.980048219888089989 ) ) ;
#1797=CARTESIAN_POINT ( 'NONE',  ( 2.072287782118878319, 0.000000000000000000, -2.950529333540147015 ) ) ;
#1798=EDGE_CURVE ( 'NONE', #10838, #20767, #53890, .T. ) ;
#1799=PLANE ( 'NONE',  #29697 ) ;
#1800=FACE_OUTER_BOUND ( 'NONE', #16212, .T. ) ;
#1801=ORIENTED_EDGE ( 'NONE', *, *, #21933, .F. ) ;
#1802=DIRECTION ( 'NONE',  ( 0.005961354470445682716, -0.6427876096865404731, -0.7660212471507180654 ) ) ;
#1803=DIRECTION ( 'NONE',  ( 0.9999697198139515519, 0.000000000000000000, 0.007781995580013368816 ) ) ;
#1804=EDGE_LOOP ( 'NONE', ( #46986, #41214, #8796, #21069 ) ) ;
#1805=CARTESIAN_POINT ( 'NONE',  ( -17.36532418587302473, -0.1191753592594177458, 13.67570816655714516 ) ) ;
#1806=FACE_OUTER_BOUND ( 'NONE', #12422, .T. ) ;
#1807=ORIENTED_EDGE ( 'NONE', *, *, #39907, .F. ) ;
#1808=EDGE_CURVE ( 'NONE', #9203, #5331, #5940, .T. ) ;
#1810=DIRECTION ( 'NONE',  ( -0.5364919789714478471, 0.6444004775717705469, -0.5449076811759709926 ) ) ;
#1811=CARTESIAN_POINT ( 'NONE',  ( -15.57130075108602618, 0.000000000000000000, 9.131212500273253596 ) ) ;
#1812=LINE ( 'NONE', #22848, #12386 ) ;
#1813=CARTESIAN_POINT ( 'NONE',  ( -15.87975247367846166, 0.000000000000000000, 2.850166870931599927 ) ) ;
#1814=EDGE_CURVE ( 'NONE', #40640, #13341, #41412, .T. ) ;
#1815=ORIENTED_EDGE ( 'NONE', *, *, #7028, .T. ) ;
#1816=ORIENTED_EDGE ( 'NONE', *, *, #27941, .F. ) ;
#1817=LINE ( 'NONE', #45282, #36653 ) ;
#1818=FACE_OUTER_BOUND ( 'NONE', #11541, .T. ) ;
#1819=CARTESIAN_POINT ( 'NONE',  ( -13.93672754567525018, -2.784623065533161856, 2.205975334288626133 ) ) ;
#1820=DIRECTION ( 'NONE',  ( 0.000000000000000000, -0.000000000000000000, -1.000000000000000000 ) ) ;
#1821=DIRECTION ( 'NONE',  ( 0.6246952433987893460, 0.7422098413412802076, -0.2426528472758539279 ) ) ;
#1822=ORIENTED_EDGE ( 'NONE', *, *, #18531, .F. ) ;
#1823=CARTESIAN_POINT ( 'NONE',  ( -19.22961988024793101, -0.1191753592594177458, 14.39986392600063603 ) ) ;
#1824=CARTESIAN_POINT ( 'NONE',  ( -11.20636620717317378, 0.000000000000000000, 11.32298014792380414 ) ) ;
#1825=AXIS2_PLACEMENT_3D ( 'NONE', #11547, #16336, #50711 ) ;
#1826=CARTESIAN_POINT ( 'NONE',  ( -14.59316804781405352, 0.000000000000000000, 2.860179368427277602 ) ) ;
#1828=ORIENTED_EDGE ( 'NONE', *, *, #26813, .T. ) ;
#1829=FACE_OUTER_BOUND ( 'NONE', #1763, .T. ) ;
#1830=ORIENTED_EDGE ( 'NONE', *, *, #42815, .T. ) ;
#1831=PLANE ( 'NONE',  #19535 ) ;
#1832=ADVANCED_FACE ( 'NONE', ( #49075 ), #7056, .F. ) ;
#1833=DIRECTION ( 'NONE',  ( -0.3620778797217457101, 0.000000000000000000, -0.9321478471874540261 ) ) ;
#1834=ORIENTED_EDGE ( 'NONE', *, *, #7038, .F. ) ;
#1835=CARTESIAN_POINT ( 'NONE',  ( -11.87243407472968926, 0.000000000000000000, 11.50246268866867361 ) ) ;
#1836=ADVANCED_FACE ( 'NONE', ( #32600 ), #19820, .F. ) ;
#1837=EDGE_LOOP ( 'NONE', ( #12268, #29340, #18634, #34154 ) ) ;
#1838=EDGE_LOOP ( 'NONE', ( #6597, #46127, #54432, #23639 ) ) ;
#1839=ORIENTED_EDGE ( 'NONE', *, *, #23407, .T. ) ;
#1841=EDGE_CURVE ( 'NONE', #39352, #17429, #23262, .T. ) ;
#1842=ORIENTED_EDGE ( 'NONE', *, *, #12734, .T. ) ;
#1843=EDGE_CURVE ( 'NONE', #48446, #42740, #49362, .T. ) ;
#1844=ORIENTED_EDGE ( 'NONE', *, *, #33961, .T. ) ;
#1845=PLANE ( 'NONE',  #52857 ) ;
#1846=CARTESIAN_POINT ( 'NONE',  ( -7.296103114018933411, -3.208161209119383628, 8.210037920513791221 ) ) ;
#1847=VERTEX_POINT ( 'NONE', #6765 ) ;
#1848=ADVANCED_FACE ( 'NONE', ( #23525 ), #54723, .F. ) ;
#1849=EDGE_CURVE ( 'NONE', #50804, #17276, #37402, .T. ) ;
#1850=EDGE_CURVE ( 'NONE', #29513, #38157, #10481, .T. ) ;
#1851=ORIENTED_EDGE ( 'NONE', *, *, #8213, .F. ) ;
#1852=FACE_OUTER_BOUND ( 'NONE', #55211, .T. ) ;
#1853=VERTEX_POINT ( 'NONE', #6223 ) ;
#1854=VERTEX_POINT ( 'NONE', #49659 ) ;
#1855=DIRECTION ( 'NONE',  ( 0.5364919789714477361, 0.6444004775717706579, 0.5449076811759711036 ) ) ;
#1856=LINE ( 'NONE', #14400, #15807 ) ;
#1858=CARTESIAN_POINT ( 'NONE',  ( -16.76102578975193680, 0.000000000000000000, 8.583295701532488664 ) ) ;
#1859=ORIENTED_EDGE ( 'NONE', *, *, #27376, .T. ) ;
#1860=DIRECTION ( 'NONE',  ( 0.9999697198139515519, 0.000000000000000000, 0.007781995580013368816 ) ) ;
#1861=ORIENTED_EDGE ( 'NONE', *, *, #23294, .F. ) ;
#1862=AXIS2_PLACEMENT_3D ( 'NONE', #32665, #37204, #36662 ) ;
#1863=EDGE_CURVE ( 'NONE', #7513, #21986, #2499, .T. ) ;
#1864=LINE ( 'NONE', #31143, #6672 ) ;
#1865=AXIS2_PLACEMENT_3D ( 'NONE', #9153, #13691, #35858 ) ;
#1866=EDGE_CURVE ( 'NONE', #42382, #46574, #32870, .T. ) ;
#1867=DIRECTION ( 'NONE',  ( 0.000000000000000000, -0.000000000000000000, -1.000000000000000000 ) ) ;
#1868=CARTESIAN_POINT ( 'NONE',  ( -14.95858617223174569, -0.1191753592594189115, 2.957338628198661556 ) ) ;
#1869=PLANE ( 'NONE',  #6895 ) ;
#1870=EDGE_CURVE ( 'NONE', #47896, #25894, #45645, .T. ) ;
#1871=LINE ( 'NONE', #18668, #29375 ) ;
#1872=FACE_OUTER_BOUND ( 'NONE', #39528, .T. ) ;
#1873=ORIENTED_EDGE ( 'NONE', *, *, #3756, .F. ) ;
#1874=CARTESIAN_POINT ( 'NONE',  ( -11.34645787693701635, 0.000000000000000000, 3.624110157318871206 ) ) ;
#1876=EDGE_CURVE ( 'NONE', #26373, #28453, #50184, .T. ) ;
#1877=CARTESIAN_POINT ( 'NONE',  ( -19.15468851132792949, -0.1191753592594168992, 4.771343938575395072 ) ) ;
#1878=LINE ( 'NONE', #28028, #3322 ) ;
#1879=DIRECTION ( 'NONE',  ( 0.9999697198139515519, 0.000000000000000000, 0.007781995580013368816 ) ) ;
#1880=CARTESIAN_POINT ( 'NONE',  ( -11.21901323774118708, 0.000000000000000000, 1.039777472322872098 ) ) ;
#1881=DIRECTION ( 'NONE',  ( 0.5364919789714477361, 0.6444004775717706579, 0.5449076811759711036 ) ) ;
#1882=LINE ( 'NONE', #53030, #51097 ) ;
#1883=ORIENTED_EDGE ( 'NONE', *, *, #48403, .T. ) ;
#1884=CARTESIAN_POINT ( 'NONE',  ( -10.37421533196711465, -0.1191753592594197858, 10.96012406864405975 ) ) ;
#1885=CARTESIAN_POINT ( 'NONE',  ( -21.10695443357304768, -5.213152330870665097, 4.913652161167348709 ) ) ;
#1886=LINE ( 'NONE', #45092, #74 ) ;
#1887=VECTOR ( 'NONE', #32657, 999.9999999999998863 ) ;
#1888=DIRECTION ( 'NONE',  ( -0.5449076811759708816, 0.6444004775717707689, 0.5364919789714475140 ) ) ;
#1889=DIRECTION ( 'NONE',  ( -0.5449076811759708816, 0.6444004775717707689, 0.5364919789714475140 ) ) ;
#1890=CARTESIAN_POINT ( 'NONE',  ( -18.86354292863559579, 0.000000000000000000, 14.21804678658176080 ) ) ;
#1891=PLANE ( 'NONE',  #16563 ) ;
#1892=DIRECTION ( 'NONE',  ( -0.005961354470445682716, -0.6427876096865404731, 0.7660212471507180654 ) ) ;
#1893=DIRECTION ( 'NONE',  ( -0.5364919789714478471, 0.6444004775717705469, -0.5449076811759709926 ) ) ;
#1895=EDGE_LOOP ( 'NONE', ( #2877, #24204, #52473, #51482 ) ) ;
#1896=VECTOR ( 'NONE', #13418, 1000.000000000000227 ) ;
#1897=VECTOR ( 'NONE', #27769, 1000.000000000000000 ) ;
#1898=ORIENTED_EDGE ( 'NONE', *, *, #3465, .T. ) ;
#1899=EDGE_LOOP ( 'NONE', ( #54836, #24136, #39930, #22886 ) ) ;
#1900=EDGE_LOOP ( 'NONE', ( #22867, #22739, #46322, #54821 ) ) ;
#1901=VERTEX_POINT ( 'NONE', #2205 ) ;
#1902=FACE_OUTER_BOUND ( 'NONE', #4725, .T. ) ;
#1903=LINE ( 'NONE', #36571, #15791 ) ;
#1905=EDGE_CURVE ( 'NONE', #33489, #34665, #55035, .T. ) ;
#1907=EDGE_LOOP ( 'NONE', ( #23537, #20296, #38827, #53020 ) ) ;
#1908=ORIENTED_EDGE ( 'NONE', *, *, #1427, .F. ) ;
#1909=VERTEX_POINT ( 'NONE', #51604 ) ;
#1910=ADVANCED_FACE ( 'NONE', ( #42247 ), #16380, .F. ) ;
#1911=LINE ( 'NONE', #18409, #14781 ) ;
#1912=CARTESIAN_POINT ( 'NONE',  ( -10.67607892912258194, 0.000000000000000000, 2.890663061687355651 ) ) ;
#1913=LINE ( 'NONE', #19247, #34098 ) ;
#1914=VERTEX_POINT ( 'NONE', #28905 ) ;
#1915=DIRECTION ( 'NONE',  ( -0.6427681459581293666, -0.7660444431189770143, -0.005002170337467561935 ) ) ;
#1916=ORIENTED_EDGE ( 'NONE', *, *, #43531, .T. ) ;
#1917=VECTOR ( 'NONE', #13379, 1000.000000000000000 ) ;
#1918=VECTOR ( 'NONE', #52240, 1000.000000000000227 ) ;
#1919=DIRECTION ( 'NONE',  ( -0.6427681459581293666, -0.7660444431189770143, -0.005002170337467561935 ) ) ;
#1920=LINE ( 'NONE', #14725, #40237 ) ;
#1921=DIRECTION ( 'NONE',  ( 0.9999697198139515519, 0.000000000000000000, 0.007781995580013368816 ) ) ;
#1922=DIRECTION ( 'NONE',  ( 0.005002170337468016433, -0.7660444431189770143, -0.6427681459581293666 ) ) ;
#1924=CARTESIAN_POINT ( 'NONE',  ( -18.34343421021684861, 0.000000000000000000, 7.093652754081396949 ) ) ;
#1925=FACE_OUTER_BOUND ( 'NONE', #48388, .T. ) ;
#1926=LINE ( 'NONE', #7067, #350 ) ;
#1927=EDGE_CURVE ( 'NONE', #43311, #9641, #11589, .T. ) ;
#1928=CARTESIAN_POINT ( 'NONE',  ( -9.470713295052064495, 9.226104519242889879, 6.897120246239332175 ) ) ;
#1929=ORIENTED_EDGE ( 'NONE', *, *, #37571, .T. ) ;
#1930=CARTESIAN_POINT ( 'NONE',  ( 2.072287782118878319, 0.000000000000000000, -2.950529333540147015 ) ) ;
#1931=ORIENTED_EDGE ( 'NONE', *, *, #36461, .F. ) ;
#1932=EDGE_CURVE ( 'NONE', #7363, #44540, #47328, .T. ) ;
#1933=CARTESIAN_POINT ( 'NONE',  ( -20.48605083020362017, 4.172053068839010059, 11.68584882396997493 ) ) ;
#1934=DIRECTION ( 'NONE',  ( 0.5449076811759707706, 0.6444004775717708799, -0.5364919789714476250 ) ) ;
#1935=LINE ( 'NONE', #12075, #34937 ) ;
#1936=CARTESIAN_POINT ( 'NONE',  ( -9.319383251525813705, -0.1191753592594193140, 3.001224209265955345 ) ) ;
#1937=FACE_OUTER_BOUND ( 'NONE', #6335, .T. ) ;
#1938=DIRECTION ( 'NONE',  ( -0.6427681459581293666, -0.7660444431189770143, -0.005002170337467561935 ) ) ;
#1939=CARTESIAN_POINT ( 'NONE',  ( -17.93139508144814442, 0.000000000000000000, 13.85596890686001537 ) ) ;
#1940=VECTOR ( 'NONE', #11066, 1000.000000000000227 ) ;
#1941=CARTESIAN_POINT ( 'NONE',  ( -16.79925329029790149, 0.000000000000000000, 13.49544742625427496 ) ) ;
#1944=ORIENTED_EDGE ( 'NONE', *, *, #33891, .T. ) ;
#1945=CARTESIAN_POINT ( 'NONE',  ( -13.63673279712320507, -0.1191753592594197858, 12.22739664767016521 ) ) ;
#1946=LINE ( 'NONE', #36615, #45762 ) ;
#1947=DIRECTION ( 'NONE',  ( 0.005002170337468016433, -0.7660444431189770143, -0.6427681459581293666 ) ) ;
#1948=EDGE_CURVE ( 'NONE', #13435, #15529, #41937, .T. ) ;
#1949=DIRECTION ( 'NONE',  ( 0.007781995580012663651, -3.146120232559066537E-19, -0.9999697198139514409 ) ) ;
#1950=LINE ( 'NONE', #10784, #4659 ) ;
#1951=DIRECTION ( 'NONE',  ( -0.7660212471507179544, -0.6427876096865405842, -0.005961354470445141482 ) ) ;
#1952=CARTESIAN_POINT ( 'NONE',  ( -12.45966937092331861, -2.137015261443157677, 1.652897857657781522 ) ) ;
#1953=DIRECTION ( 'NONE',  ( 0.005961354470445682716, -0.6427876096865404731, -0.7660212471507180654 ) ) ;
#1954=EDGE_LOOP ( 'NONE', ( #7900, #50069, #40658, #38237 ) ) ;
#1955=ORIENTED_EDGE ( 'NONE', *, *, #2128, .F. ) ;
#1956=LINE ( 'NONE', #27849, #51338 ) ;
#1957=CARTESIAN_POINT ( 'NONE',  ( -19.79569077582305070, 0.000000000000000000, 14.58012466630350445 ) ) ;
#1958=AXIS2_PLACEMENT_3D ( 'NONE', #2173, #18379, #49628 ) ;
#1959=VECTOR ( 'NONE', #888, 1000.000000000000227 ) ;
#1960=ORIENTED_EDGE ( 'NONE', *, *, #23851, .F. ) ;
#1961=CARTESIAN_POINT ( 'NONE',  ( -25.20278734466900517, 0.000000000000000000, 6.670939612111840944 ) ) ;
#1962=ORIENTED_EDGE ( 'NONE', *, *, #49369, .T. ) ;
#1963=LINE ( 'NONE', #10230, #31121 ) ;
#1964=EDGE_LOOP ( 'NONE', ( #32203, #28848, #1655, #21035 ) ) ;
#1966=VECTOR ( 'NONE', #50986, 1000.000000000000114 ) ;
#1967=ORIENTED_EDGE ( 'NONE', *, *, #41514, .F. ) ;
#1968=CARTESIAN_POINT ( 'NONE',  ( -15.93812677074078721, -0.1191753592594209099, 9.409283274482961090 ) ) ;
#1969=LINE ( 'NONE', #2268, #2342 ) ;
#1970=FACE_OUTER_BOUND ( 'NONE', #7950, .T. ) ;
#1971=ADVANCED_FACE ( 'NONE', ( #24924 ), #8438, .F. ) ;
#1972=EDGE_LOOP ( 'NONE', ( #41603, #54047, #31424, #43067 ) ) ;
#1973=AXIS2_PLACEMENT_3D ( 'NONE', #13811, #48164, #17233 ) ;
#1974=ORIENTED_EDGE ( 'NONE', *, *, #10264, .T. ) ;
#1975=ADVANCED_FACE ( 'NONE', ( #34010 ), #25763, .F. ) ;
#1976=ADVANCED_FACE ( 'NONE', ( #3348 ), #37712, .F. ) ;
#1977=VECTOR ( 'NONE', #25078, 1000.000000000000227 ) ;
#1978=LINE ( 'NONE', #14787, #34533 ) ;
#1980=CARTESIAN_POINT ( 'NONE',  ( -27.06708303904391144, 0.000000000000000000, 7.395095371555332697 ) ) ;
#1981=ORIENTED_EDGE ( 'NONE', *, *, #46750, .F. ) ;
#1982=DIRECTION ( 'NONE',  ( -0.5449076811759708816, 0.6444004775717707689, 0.5364919789714475140 ) ) ;
#1983=LINE ( 'NONE', #54796, #14941 ) ;
#1984=ORIENTED_EDGE ( 'NONE', *, *, #34145, .F. ) ;
#1985=LINE ( 'NONE', #22493, #38584 ) ;
#1986=DIRECTION ( 'NONE',  ( 0.7660212471507180654, -0.6427876096865404731, 0.005961354470445141482 ) ) ;
#1987=VERTEX_POINT ( 'NONE', #46789 ) ;
#1989=LINE ( 'NONE', #6291, #26660 ) ;
#1990=VECTOR ( 'NONE', #53920, 999.9999999999998863 ) ;
#1991=CARTESIAN_POINT ( 'NONE',  ( -13.63673279712320507, -0.1191753592594197858, 12.22739664767016521 ) ) ;
#1992=ORIENTED_EDGE ( 'NONE', *, *, #45850, .T. ) ;
#1993=AXIS2_PLACEMENT_3D ( 'NONE', #42978, #47518, #29671 ) ;
#1994=VECTOR ( 'NONE', #1166, 1000.000000000000227 ) ;
#1995=DIRECTION ( 'NONE',  ( 0.000000000000000000, -1.000000000000000000, 0.000000000000000000 ) ) ;
#1996=PLANE ( 'NONE',  #5144 ) ;
#1997=CARTESIAN_POINT ( 'NONE',  ( -17.64587796725810165, 3.409179049219567048, 12.21456663636006468 ) ) ;
#1998=LINE ( 'NONE', #38063, #24999 ) ;
#1999=ADVANCED_FACE ( 'NONE', ( #38837 ), #42782, .F. ) ;
#2000=LINE ( 'NONE', #22509, #23109 ) ;
#2001=DIRECTION ( 'NONE',  ( -0.5364919789714478471, 0.6444004775717705469, -0.5449076811759709926 ) ) ;
#2002=AXIS2_PLACEMENT_3D ( 'NONE', #16355, #46758, #25447 ) ;
#2004=VECTOR ( 'NONE', #49455, 1000.000000000000227 ) ;
#2005=ORIENTED_EDGE ( 'NONE', *, *, #22159, .T. ) ;
#2006=CARTESIAN_POINT ( 'NONE',  ( -16.17100751540999681, 0.7721120973665049902, 2.938665801846358505 ) ) ;
#2007=EDGE_CURVE ( 'NONE', #47104, #36655, #15828, .T. ) ;
#2008=FACE_OUTER_BOUND ( 'NONE', #4329, .T. ) ;
#2010=VERTEX_POINT ( 'NONE', #20372 ) ;
#2011=LINE ( 'NONE', #19346, #23865 ) ;
#2012=CARTESIAN_POINT ( 'NONE',  ( 2.072287782118878319, 0.000000000000000000, -2.950529333540147015 ) ) ;
#2013=EDGE_CURVE ( 'NONE', #9641, #50706, #51334, .T. ) ;
#2014=DIRECTION ( 'NONE',  ( -0.9999697198139514409, -0.000000000000000000, -0.007781995580013368816 ) ) ;
#2015=VECTOR ( 'NONE', #2440, 999.9999999999998863 ) ;
#2016=LINE ( 'NONE', #49175, #30593 ) ;
#2017=CARTESIAN_POINT ( 'NONE',  ( 2.072287782118878319, 0.000000000000000000, -2.950529333540147015 ) ) ;
#2019=ORIENTED_EDGE ( 'NONE', *, *, #43484, .F. ) ;
#2020=CARTESIAN_POINT ( 'NONE',  ( -11.72912032238640556, -0.1191753592594190225, 5.937127636636843953 ) ) ;
#2021=CARTESIAN_POINT ( 'NONE',  ( -14.93495759592298988, 0.000000000000000000, 12.77129166681078409 ) ) ;
#2022=ORIENTED_EDGE ( 'NONE', *, *, #51670, .F. ) ;
#2024=AXIS2_PLACEMENT_3D ( 'NONE', #25241, #11614, #24379 ) ;
#2025=ORIENTED_EDGE ( 'NONE', *, *, #30562, .T. ) ;
#2026=DIRECTION ( 'NONE',  ( 0.000000000000000000, 1.000000000000000000, 0.000000000000000000 ) ) ;
#2027=EDGE_CURVE ( 'NONE', #28956, #29054, #50749, .T. ) ;
#2028=VERTEX_POINT ( 'NONE', #46476 ) ;
#2029=EDGE_LOOP ( 'NONE', ( #22916, #37565, #35525, #17878 ) ) ;
#2030=CARTESIAN_POINT ( 'NONE',  ( -20.54049170961573267, 0.000000000000000000, 4.660556269540326646 ) ) ;
#2031=CIRCLE ( 'NONE', #34679, 6.999999999999988454 ) ;
#2032=EDGE_CURVE ( 'NONE', #36770, #46531, #37987, .T. ) ;
#2033=CARTESIAN_POINT ( 'NONE',  ( -20.19095613468760320, 0.000000000000000000, 5.662415103335279198 ) ) ;
#2034=CARTESIAN_POINT ( 'NONE',  ( -25.20123094555300369, 0.000000000000000000, 6.470945668149052032 ) ) ;
#2035=ORIENTED_EDGE ( 'NONE', *, *, #5359, .T. ) ;
#2036=VECTOR ( 'NONE', #18693, 1000.000000000000227 ) ;
#2037=VECTOR ( 'NONE', #47569, 1000.000000000000227 ) ;
#2038=LINE ( 'NONE', #2872, #4928 ) ;
#2039=EDGE_CURVE ( 'NONE', #37913, #17469, #33705, .T. ) ;
#2040=ORIENTED_EDGE ( 'NONE', *, *, #5282, .T. ) ;
#2041=ADVANCED_FACE ( 'NONE', ( #7905 ), #29765, .F. ) ;
#2042=VERTEX_POINT ( 'NONE', #25476 ) ;
#2043=AXIS2_PLACEMENT_3D ( 'NONE', #54026, #36162, #6074 ) ;
#2044=ORIENTED_EDGE ( 'NONE', *, *, #13964, .F. ) ;
#2045=LINE ( 'NONE', #45489, #38592 ) ;
#2046=VECTOR ( 'NONE', #9933, 1000.000000000000227 ) ;
#2047=ORIENTED_EDGE ( 'NONE', *, *, #7137, .F. ) ;
#2048=CARTESIAN_POINT ( 'NONE',  ( -24.27063949748155380, 0.000000000000000000, 6.308861732390097288 ) ) ;
#2049=VERTEX_POINT ( 'NONE', #47061 ) ;
#2050=LINE ( 'NONE', #10328, #54862 ) ;
#2051=DIRECTION ( 'NONE',  ( -0.005961354470445682716, -0.6427876096865404731, 0.7660212471507180654 ) ) ;
#2052=EDGE_CURVE ( 'NONE', #44744, #47896, #52708, .T. ) ;
#2053=ORIENTED_EDGE ( 'NONE', *, *, #52670, .F. ) ;
#2054=DIRECTION ( 'NONE',  ( -0.7660212471507179544, -0.6427876096865405842, -0.005961354470445141482 ) ) ;
#2055=VECTOR ( 'NONE', #51107, 1000.000000000000227 ) ;
#2056=ORIENTED_EDGE ( 'NONE', *, *, #49126, .T. ) ;
#2057=VECTOR ( 'NONE', #31968, 1000.000000000000227 ) ;
#2058=ADVANCED_FACE ( 'NONE', ( #763 ), #22630, .F. ) ;
#2059=DIRECTION ( 'NONE',  ( -0.7660212471507179544, -0.6427876096865405842, -0.005961354470445141482 ) ) ;
#2060=LINE ( 'NONE', #19393, #53805 ) ;
#2061=DIRECTION ( 'NONE',  ( 0.005961354470445682716, -0.6427876096865404731, -0.7660212471507180654 ) ) ;
#2062=PLANE ( 'NONE',  #51096 ) ;
#2063=DIRECTION ( 'NONE',  ( 0.007781995580012662783, 0.000000000000000000, -0.9999697198139514409 ) ) ;
#2064=LINE ( 'NONE', #40722, #15582 ) ;
#2065=EDGE_LOOP ( 'NONE', ( #43818, #17178, #9439, #28162 ) ) ;
#2066=AXIS2_PLACEMENT_3D ( 'NONE', #5631, #49655, #13868 ) ;
#2069=LINE ( 'NONE', #29330, #9466 ) ;
#2070=VECTOR ( 'NONE', #39496, 1000.000000000000227 ) ;
#2071=CARTESIAN_POINT ( 'NONE',  ( -13.17065887352947762, -0.1191753592594197858, 12.04635770780929427 ) ) ;
#2072=LINE ( 'NONE', #33035, #26965 ) ;
#2073=DIRECTION ( 'NONE',  ( -0.005961354470445682716, -0.6427876096865404731, 0.7660212471507180654 ) ) ;
#2074=ORIENTED_EDGE ( 'NONE', *, *, #27339, .T. ) ;
#2075=FACE_OUTER_BOUND ( 'NONE', #2430, .T. ) ;
#2076=PLANE ( 'NONE',  #26868 ) ;
#2077=ORIENTED_EDGE ( 'NONE', *, *, #16674, .T. ) ;
#2079=DIRECTION ( 'NONE',  ( 0.007781995580012663651, -3.146120232559066537E-19, -0.9999697198139514409 ) ) ;
#2080=DIRECTION ( 'NONE',  ( 0.000000000000000000, -0.000000000000000000, -1.000000000000000000 ) ) ;
#2081=EDGE_LOOP ( 'NONE', ( #41452, #25307, #16223, #11978 ) ) ;
#2082=AXIS2_PLACEMENT_3D ( 'NONE', #20184, #45027, #27133 ) ;
#2083=VECTOR ( 'NONE', #15039, 1000.000000000000227 ) ;
#2084=CARTESIAN_POINT ( 'NONE',  ( -13.52026565332740482, -1.165603555308156736, 3.846616072963900290 ) ) ;
#2085=LINE ( 'NONE', #48971, #39656 ) ;
#2086=EDGE_CURVE ( 'NONE', #51694, #9097, #27167, .T. ) ;
#2087=CARTESIAN_POINT ( 'NONE',  ( -18.67775241435682432, 0.000000000000000000, 4.136394454059623804 ) ) ;
#2088=FACE_OUTER_BOUND ( 'NONE', #24345, .T. ) ;
#2089=DIRECTION ( 'NONE',  ( 0.007781995580012662783, 0.000000000000000000, -0.9999697198139514409 ) ) ;
#2090=ORIENTED_EDGE ( 'NONE', *, *, #30344, .F. ) ;
#2091=VECTOR ( 'NONE', #34344, 1000.000000000000000 ) ;
#2092=AXIS2_PLACEMENT_3D ( 'NONE', #14288, #27307, #5459 ) ;
#2093=ORIENTED_EDGE ( 'NONE', *, *, #49879, .T. ) ;
#2094=FACE_OUTER_BOUND ( 'NONE', #7215, .T. ) ;
#2095=PLANE ( 'NONE',  #55793 ) ;
#2096=LINE ( 'NONE', #1819, #46032 ) ;
#2097=ADVANCED_FACE ( 'NONE', ( #39937 ), #56149, .F. ) ;
#2098=LINE ( 'NONE', #5833, #41850 ) ;
#2099=DIRECTION ( 'NONE',  ( -0.005961354470445682716, -0.6427876096865404731, 0.7660212471507180654 ) ) ;
#2100=EDGE_LOOP ( 'NONE', ( #22012, #1505, #24804, #48534 ) ) ;
#2101=EDGE_CURVE ( 'NONE', #3819, #47757, #26066, .T. ) ;
#2102=DIRECTION ( 'NONE',  ( 0.000000000000000000, -0.000000000000000000, -1.000000000000000000 ) ) ;
#2103=AXIS2_PLACEMENT_3D ( 'NONE', #41336, #54640, #24002 ) ;
#2104=EDGE_CURVE ( 'NONE', #31339, #2694, #170, .T. ) ;
#2105=DIRECTION ( 'NONE',  ( -0.005002170337468016433, -0.7660444431189770143, 0.6427681459581293666 ) ) ;
#2106=DIRECTION ( 'NONE',  ( 0.9999697198139515519, 0.000000000000000000, 0.007781995580013368816 ) ) ;
#2107=EDGE_LOOP ( 'NONE', ( #47687, #15501, #17139, #35280 ) ) ;
#2108=DIRECTION ( 'NONE',  ( 0.7660212471507180654, -0.6427876096865404731, 0.005961354470445141482 ) ) ;
#2109=EDGE_LOOP ( 'NONE', ( #6, #16158, #21082, #50793 ) ) ;
#2110=DIRECTION ( 'NONE',  ( 0.7660212471507180654, -0.6427876096865404731, 0.005961354470445141482 ) ) ;
#2111=VECTOR ( 'NONE', #48952, 1000.000000000000000 ) ;
#2112=DIRECTION ( 'NONE',  ( -0.6427681459581293666, -0.7660444431189770143, -0.005002170337467561935 ) ) ;
#2113=ORIENTED_EDGE ( 'NONE', *, *, #38991, .T. ) ;
#2114=PLANE ( 'NONE',  #54024 ) ;
#2115=EDGE_CURVE ( 'NONE', #42375, #18224, #18351, .T. ) ;
#2116=VECTOR ( 'NONE', #43468, 999.9999999999998863 ) ;
#2117=EDGE_LOOP ( 'NONE', ( #22976, #10330, #5618, #19865 ) ) ;
#2118=ADVANCED_FACE ( 'NONE', ( #9273 ), #43914, .F. ) ;
#2119=ORIENTED_EDGE ( 'NONE', *, *, #8292, .T. ) ;
#2120=EDGE_LOOP ( 'NONE', ( #29756, #40103, #54588, #22343 ) ) ;
#2122=ORIENTED_EDGE ( 'NONE', *, *, #28360, .F. ) ;
#2123=ORIENTED_EDGE ( 'NONE', *, *, #25714, .T. ) ;
#2124=VECTOR ( 'NONE', #55210, 999.9999999999998863 ) ;
#2125=LINE ( 'NONE', #18923, #2057 ) ;
#2126=VERTEX_POINT ( 'NONE', #53007 ) ;
#2127=VECTOR ( 'NONE', #54884, 1000.000000000000114 ) ;
#2128=EDGE_CURVE ( 'NONE', #29102, #17107, #31140, .T. ) ;
#2129=VECTOR ( 'NONE', #43312, 1000.000000000000227 ) ;
#2130=ORIENTED_EDGE ( 'NONE', *, *, #10800, .T. ) ;
#2131=LINE ( 'NONE', #19175, #54850 ) ;
#2132=VERTEX_POINT ( 'NONE', #9013 ) ;
#2133=ORIENTED_EDGE ( 'NONE', *, *, #18160, .T. ) ;
#2134=ORIENTED_EDGE ( 'NONE', *, *, #35473, .T. ) ;
#2135=EDGE_CURVE ( 'NONE', #54647, #50938, #44472, .T. ) ;
#2136=AXIS2_PLACEMENT_3D ( 'NONE', #23823, #10785, #54760 ) ;
#2137=VECTOR ( 'NONE', #13624, 1000.000000000000227 ) ;
#2138=DIRECTION ( 'NONE',  ( 0.5449076811759707706, 0.6444004775717708799, -0.5364919789714476250 ) ) ;
#2139=PLANE ( 'NONE',  #29403 ) ;
#2140=LINE ( 'NONE', #53003, #45922 ) ;
#2141=CARTESIAN_POINT ( 'NONE',  ( -24.26908309836554878, 0.000000000000000000, 6.108867788427308376 ) ) ;
#2143=DIRECTION ( 'NONE',  ( 0.007781995580012663651, 0.000000000000000000, -0.9999697198139515519 ) ) ;
#2144=ORIENTED_EDGE ( 'NONE', *, *, #3036, .F. ) ;
#2145=EDGE_LOOP ( 'NONE', ( #7055, #3714, #30518, #47275 ) ) ;
#2146=DIRECTION ( 'NONE',  ( 0.6427681459581294776, -0.7660444431189769032, 0.005002170337467562802 ) ) ;
#2147=PLANE ( 'NONE',  #40587 ) ;
#2148=LINE ( 'NONE', #19485, #38495 ) ;
#2149=VECTOR ( 'NONE', #50327, 999.9999999999998863 ) ;
#2150=LINE ( 'NONE', #6437, #21219 ) ;
#2151=DIRECTION ( 'NONE',  ( -0.3620778797217455991, 0.000000000000000000, -0.9321478471874540261 ) ) ;
#2152=ORIENTED_EDGE ( 'NONE', *, *, #43562, .F. ) ;
#2153=DIRECTION ( 'NONE',  ( -0.005961354470445682716, -0.6427876096865404731, 0.7660212471507180654 ) ) ;
#2154=AXIS2_PLACEMENT_3D ( 'NONE', #49605, #44224, #2146 ) ;
#2155=EDGE_LOOP ( 'NONE', ( #4127, #53544, #41314, #16182 ) ) ;
#2156=DIRECTION ( 'NONE',  ( 0.9999697198139515519, 0.000000000000000000, 0.007781995580013368816 ) ) ;
#2157=LINE ( 'NONE', #10435, #45918 ) ;
#2158=DIRECTION ( 'NONE',  ( 0.7660212471507180654, -0.6427876096865404731, 0.005961354470445141482 ) ) ;
#2159=ADVANCED_FACE ( 'NONE', ( #4738 ), #47629, .F. ) ;
#2160=VECTOR ( 'NONE', #24632, 999.9999999999998863 ) ;
#2161=CARTESIAN_POINT ( 'NONE',  ( -16.99924723426068951, 0.000000000000000000, 13.49389102713827171 ) ) ;
#2162=CARTESIAN_POINT ( 'NONE',  ( -12.27285761711391032, 0.000000000000000000, 3.247568630525088818 ) ) ;
#2163=EDGE_CURVE ( 'NONE', #40212, #12044, #48461, .T. ) ;
#2164=ORIENTED_EDGE ( 'NONE', *, *, #19730, .T. ) ;
#2165=AXIS2_PLACEMENT_3D ( 'NONE', #34407, #30138, #47456 ) ;
#2166=CARTESIAN_POINT ( 'NONE',  ( -19.16420072258311436, -0.6798977022406551551, 5.241786070853162727 ) ) ;
#2167=CARTESIAN_POINT ( 'NONE',  ( -13.73672976910459909, 0.000000000000000000, 12.22661844811216270 ) ) ;
#2168=DIRECTION ( 'NONE',  ( -0.5449076811759708816, 0.6444004775717707689, 0.5364919789714475140 ) ) ;
#2170=ADVANCED_FACE ( 'NONE', ( #13282 ), #9863, .F. ) ;
#2171=EDGE_CURVE ( 'NONE', #33602, #55501, #5321, .T. ) ;
#2172=VECTOR ( 'NONE', #7976, 1000.000000000000114 ) ;
#2173=CARTESIAN_POINT ( 'NONE',  ( -22.40478740399063895, 0.000000000000000000, 5.384712028983816623 ) ) ;
#2174=PLANE ( 'NONE',  #43896 ) ;
#2175=CARTESIAN_POINT ( 'NONE',  ( -18.67697421479882181, -0.1191753592594197858, 4.036397482078229793 ) ) ;
#2176=LINE ( 'NONE', #15263, #34685 ) ;
#2177=ADVANCED_FACE ( 'NONE', ( #47913 ), #22059, .F. ) ;
#2178=VECTOR ( 'NONE', #1638, 999.9999999999998863 ) ;
#2179=VECTOR ( 'NONE', #10973, 999.9999999999998863 ) ;
#2180=DIRECTION ( 'NONE',  ( -0.9321478471874540261, 0.000000000000000000, 0.3620778797217457656 ) ) ;
#2181=DIRECTION ( 'NONE',  ( 0.5449076811759707706, 0.6444004775717708799, -0.5364919789714476250 ) ) ;
#2182=EDGE_LOOP ( 'NONE', ( #18550, #14027, #27487, #4916, #1801 ) ) ;
#2183=EDGE_CURVE ( 'NONE', #11699, #42663, #13547, .T. ) ;
#2184=EDGE_CURVE ( 'NONE', #38162, #8156, #45882, .T. ) ;
#2185=AXIS2_PLACEMENT_3D ( 'NONE', #45061, #6168, #53305 ) ;
#2187=VERTEX_POINT ( 'NONE', #15481 ) ;
#2188=ORIENTED_EDGE ( 'NONE', *, *, #4643, .F. ) ;
#2189=EDGE_CURVE ( 'NONE', #44901, #31339, #6173, .T. ) ;
#2190=ORIENTED_EDGE ( 'NONE', *, *, #32674, .T. ) ;
#2191=LINE ( 'NONE', #31758, #34148 ) ;
#2192=DIRECTION ( 'NONE',  ( -0.6427681459581293666, -0.7660444431189770143, -0.005002170337467561935 ) ) ;
#2194=EDGE_CURVE ( 'NONE', #33225, #40269, #49301, .T. ) ;
#2195=ORIENTED_EDGE ( 'NONE', *, *, #43381, .T. ) ;
#2196=DIRECTION ( 'NONE',  ( 0.5364919789714477361, 0.6444004775717706579, 0.5449076811759711036 ) ) ;
#2197=ORIENTED_EDGE ( 'NONE', *, *, #42916, .F. ) ;
#2199=AXIS2_PLACEMENT_3D ( 'NONE', #5585, #30619, #14130 ) ;
#2201=VECTOR ( 'NONE', #17876, 1000.000000000000227 ) ;
#2202=DIRECTION ( 'NONE',  ( 0.9999697198139515519, 0.000000000000000000, 0.007781995580013368816 ) ) ;
#2203=CARTESIAN_POINT ( 'NONE',  ( -19.25103323024604052, 0.000000000000000000, 4.301259063778239522 ) ) ;
#2204=ORIENTED_EDGE ( 'NONE', *, *, #17300, .T. ) ;
#2205=CARTESIAN_POINT ( 'NONE',  ( -13.00213746683328964, 0.000000000000000000, 3.241893206105073144 ) ) ;
#2206=VECTOR ( 'NONE', #38846, 999.9999999999998863 ) ;
#2207=DIRECTION ( 'NONE',  ( 0.5449076811759707706, 0.6444004775717708799, -0.5364919789714476250 ) ) ;
#2208=FACE_OUTER_BOUND ( 'NONE', #20967, .T. ) ;
#2209=VECTOR ( 'NONE', #45024, 1000.000000000000114 ) ;
#2210=DIRECTION ( 'NONE',  ( -0.5449076811759708816, 0.6444004775717707689, 0.5364919789714475140 ) ) ;
#2211=PLANE ( 'NONE',  #3368 ) ;
#2212=AXIS2_PLACEMENT_3D ( 'NONE', #3387, #41454, #36924 ) ;
#2214=DIRECTION ( 'NONE',  ( -0.7660212471507179544, -0.6427876096865405842, -0.005961354470445141482 ) ) ;
#2215=CARTESIAN_POINT ( 'NONE',  ( -0.9971735401232131313, -6.078073896745635807, 3.605709642803621939 ) ) ;
#2216=CARTESIAN_POINT ( 'NONE',  ( -16.32763152475235913, 5.305366725996512045, 11.93053833287189747 ) ) ;
#2218=CARTESIAN_POINT ( 'NONE',  ( -10.37421533196711465, -0.1191753592594197858, 10.96012406864405975 ) ) ;
#2219=ORIENTED_EDGE ( 'NONE', *, *, #45835, .F. ) ;
#2220=ADVANCED_FACE ( 'NONE', ( #14946 ), #5877, .F. ) ;
#2221=LINE ( 'NONE', #19563, #29258 ) ;
#2222=FACE_OUTER_BOUND ( 'NONE', #39220, .T. ) ;
#2223=FACE_OUTER_BOUND ( 'NONE', #4457, .T. ) ;
#2224=DIRECTION ( 'NONE',  ( -0.5449076811759708816, 0.6444004775717707689, 0.5364919789714475140 ) ) ;
#2225=ADVANCED_FACE ( 'NONE', ( #41351 ), #11231, .F. ) ;
#2226=CARTESIAN_POINT ( 'NONE',  ( -8.061453912371437269, -7.756624998024296502, -0.08703110797150630240 ) ) ;
#2227=CARTESIAN_POINT ( 'NONE',  ( -19.60990026154428278, 0.000000000000000000, 4.498472333781370125 ) ) ;
#2228=VECTOR ( 'NONE', #20101, 999.9999999999998863 ) ;
#2229=DIRECTION ( 'NONE',  ( 0.9999697198139515519, 0.000000000000000000, 0.007781995580013368816 ) ) ;
#2231=VECTOR ( 'NONE', #47775, 1000.000000000000114 ) ;
#2232=DIRECTION ( 'NONE',  ( 0.005961354470445682716, -0.6427876096865404731, -0.7660212471507180654 ) ) ;
#2233=DIRECTION ( 'NONE',  ( 0.000000000000000000, -1.000000000000000000, 0.000000000000000000 ) ) ;
#2234=DIRECTION ( 'NONE',  ( -0.5449076811759708816, 0.6444004775717707689, 0.5364919789714475140 ) ) ;
#2236=VECTOR ( 'NONE', #48621, 999.9999999999998863 ) ;
#2237=EDGE_CURVE ( 'NONE', #29513, #1224, #14661, .T. ) ;
#2238=DIRECTION ( 'NONE',  ( 0.9999697198139515519, 0.000000000000000000, 0.007781995580013368816 ) ) ;
#2239=EDGE_CURVE ( 'NONE', #19378, #19054, #36516, .T. ) ;
#2240=EDGE_CURVE ( 'NONE', #3565, #2953, #31981, .T. ) ;
#2241=DIRECTION ( 'NONE',  ( 0.9999697198139515519, 0.000000000000000000, 0.007781995580013368816 ) ) ;
#2243=DIRECTION ( 'NONE',  ( 0.007781995580012663651, 0.000000000000000000, -0.9999697198139515519 ) ) ;
#2244=EDGE_CURVE ( 'NONE', #32088, #34543, #40225, .T. ) ;
#2245=FACE_OUTER_BOUND ( 'NONE', #33427, .T. ) ;
#2246=DIRECTION ( 'NONE',  ( 0.005002170337468016433, -0.7660444431189770143, -0.6427681459581293666 ) ) ;
#2247=ORIENTED_EDGE ( 'NONE', *, *, #39992, .T. ) ;
#2248=FACE_OUTER_BOUND ( 'NONE', #43148, .T. ) ;
#2249=VECTOR ( 'NONE', #33727, 1000.000000000000227 ) ;
#2250=VECTOR ( 'NONE', #24711, 999.9999999999998863 ) ;
#2251=ORIENTED_EDGE ( 'NONE', *, *, #8873, .T. ) ;
#2252=PLANE ( 'NONE',  #47739 ) ;
#2254=DIRECTION ( 'NONE',  ( 0.6427681459581294776, -0.7660444431189769032, 0.005002170337467562802 ) ) ;
#2255=AXIS2_PLACEMENT_3D ( 'NONE', #15107, #33523, #11926 ) ;
#2256=ORIENTED_EDGE ( 'NONE', *, *, #53680, .F. ) ;
#2257=CARTESIAN_POINT ( 'NONE',  ( -12.92993527630429185, 1.905425754524006532, 1.643564637689428620 ) ) ;
#2258=ORIENTED_EDGE ( 'NONE', *, *, #4489, .T. ) ;
#2260=EDGE_CURVE ( 'NONE', #16010, #10235, #23730, .T. ) ;
#2261=VECTOR ( 'NONE', #14306, 1000.000000000000114 ) ;
#2262=VERTEX_POINT ( 'NONE', #19763 ) ;
#2263=VECTOR ( 'NONE', #21465, 1000.000000000000227 ) ;
#2264=ORIENTED_EDGE ( 'NONE', *, *, #8457, .F. ) ;
#2265=ORIENTED_EDGE ( 'NONE', *, *, #22264, .T. ) ;
#2266=EDGE_CURVE ( 'NONE', #42909, #30703, #14404, .T. ) ;
#2267=DIRECTION ( 'NONE',  ( -0.005002170337468016433, -0.7660444431189770143, 0.6427681459581293666 ) ) ;
#2268=CARTESIAN_POINT ( 'NONE',  ( -10.15248364251277913, -0.02656858173836865178, 0.8564570764427139604 ) ) ;
#2269=FACE_OUTER_BOUND ( 'NONE', #13609, .T. ) ;
#2270=EDGE_CURVE ( 'NONE', #25263, #29020, #1311, .T. ) ;
#2271=ORIENTED_EDGE ( 'NONE', *, *, #27435, .T. ) ;
#2272=ORIENTED_EDGE ( 'NONE', *, *, #5337, .F. ) ;
#2273=ADVANCED_FACE ( 'NONE', ( #19186 ), #53834, .F. ) ;
#2274=VECTOR ( 'NONE', #50073, 1000.000000000000227 ) ;
#2275=LINE ( 'NONE', #45710, #1887 ) ;
#2276=VECTOR ( 'NONE', #2196, 999.9999999999998863 ) ;
#2277=ORIENTED_EDGE ( 'NONE', *, *, #28600, .T. ) ;
#2278=FACE_OUTER_BOUND ( 'NONE', #17971, .T. ) ;
#2279=VERTEX_POINT ( 'NONE', #45320 ) ;
#2282=DIRECTION ( 'NONE',  ( -0.5449076811759708816, 0.6444004775717707689, 0.5364919789714475140 ) ) ;
#2283=ORIENTED_EDGE ( 'NONE', *, *, #11508, .F. ) ;
#2284=DIRECTION ( 'NONE',  ( -0.5449076811759708816, 0.6444004775717707689, 0.5364919789714475140 ) ) ;
#2285=VECTOR ( 'NONE', #16986, 1000.000000000000227 ) ;
#2286=PLANE ( 'NONE',  #5528 ) ;
#2287=VECTOR ( 'NONE', #6286, 1000.000000000000227 ) ;
#2288=VECTOR ( 'NONE', #24226, 999.9999999999998863 ) ;
#2289=VERTEX_POINT ( 'NONE', #41052 ) ;
#2290=FACE_OUTER_BOUND ( 'NONE', #31705, .T. ) ;
#2291=DIRECTION ( 'NONE',  ( -0.8531650599175529814, -0.4028455766673920135, 0.3313982828793697877 ) ) ;
#2292=CARTESIAN_POINT ( 'NONE',  ( -29.86197018149027116, 0.000000000000000000, 8.281335066757780083 ) ) ;
#2293=EDGE_LOOP ( 'NONE', ( #35221, #36493, #16059, #46308 ) ) ;
#2294=VECTOR ( 'NONE', #54153, 999.9999999999998863 ) ;
#2295=VECTOR ( 'NONE', #34920, 999.9999999999998863 ) ;
#2297=CARTESIAN_POINT ( 'NONE',  ( -12.60458797795435615, 0.000000000000000000, 11.86609696750642229 ) ) ;
#2298=CARTESIAN_POINT ( 'NONE',  ( -21.04994044461160740, -3.432230869623158487, 10.49131904603741816 ) ) ;
#2299=CARTESIAN_POINT ( 'NONE',  ( 2.072287782118878319, 0.000000000000000000, -2.950529333540147015 ) ) ;
#2300=CARTESIAN_POINT ( 'NONE',  ( -12.71165780605550211, -2.946525016555658905, 6.455320848100502218 ) ) ;
#2301=DIRECTION ( 'NONE',  ( 0.9999697198139515519, 0.000000000000000000, 0.007781995580013368816 ) ) ;
#2302=VECTOR ( 'NONE', #13178, 999.9999999999998863 ) ;
#2303=VECTOR ( 'NONE', #26760, 1000.000000000000114 ) ;
#2305=VERTEX_POINT ( 'NONE', #18936 ) ;
#2306=DIRECTION ( 'NONE',  ( 0.007781995580012663651, -3.146120232559066537E-19, -0.9999697198139514409 ) ) ;
#2307=DIRECTION ( 'NONE',  ( 0.000000000000000000, -0.000000000000000000, -1.000000000000000000 ) ) ;
#2309=VERTEX_POINT ( 'NONE', #40531 ) ;
#2310=CARTESIAN_POINT ( 'NONE',  ( 2.072287782118878319, 0.000000000000000000, -2.950529333540147015 ) ) ;
#2311=PLANE ( 'NONE',  #19096 ) ;
#2312=EDGE_CURVE ( 'NONE', #32666, #3230, #31717, .T. ) ;
#2313=DIRECTION ( 'NONE',  ( 0.007781995580012663651, -3.146120232559066537E-19, -0.9999697198139514409 ) ) ;
#2314=EDGE_CURVE ( 'NONE', #9006, #32397, #19475, .T. ) ;
#2316=CARTESIAN_POINT ( 'NONE',  ( -14.01623497886155256, -0.1191753592594197858, 2.226008083469502630 ) ) ;
#2317=LINE ( 'NONE', #27614, #44686 ) ;
#2318=VECTOR ( 'NONE', #9380, 999.9999999999998863 ) ;
#2319=ORIENTED_EDGE ( 'NONE', *, *, #30602, .T. ) ;
#2320=VERTEX_POINT ( 'NONE', #32550 ) ;
#2321=VECTOR ( 'NONE', #48092, 1000.000000000000114 ) ;
#2322=CARTESIAN_POINT ( 'NONE',  ( -24.26908309836554878, 0.000000000000000000, 6.108867788427308376 ) ) ;
#2323=VECTOR ( 'NONE', #41289, 999.9999999999998863 ) ;
#2324=CARTESIAN_POINT ( 'NONE',  ( -18.24265903867745919, -0.1191753592594168992, 6.994433981658000121 ) ) ;
#2325=ORIENTED_EDGE ( 'NONE', *, *, #1723, .T. ) ;
#2326=CARTESIAN_POINT ( 'NONE',  ( -28.93060053386082231, -0.1191753592594197858, 8.019254159017428663 ) ) ;
#2327=VECTOR ( 'NONE', #19336, 1000.000000000000114 ) ;
#2328=VERTEX_POINT ( 'NONE', #10951 ) ;
#2329=DIRECTION ( 'NONE',  ( 0.007781995580012663651, -3.146120232559066537E-19, -0.9999697198139514409 ) ) ;
#2330=VECTOR ( 'NONE', #30164, 999.9999999999998863 ) ;
#2331=ORIENTED_EDGE ( 'NONE', *, *, #41111, .F. ) ;
#2332=ORIENTED_EDGE ( 'NONE', *, *, #33090, .F. ) ;
#2333=CARTESIAN_POINT ( 'NONE',  ( -10.77972815416725894, -0.1191753592594185784, 3.359191537368509728 ) ) ;
#2334=LINE ( 'NONE', #44955, #15973 ) ;
#2335=CARTESIAN_POINT ( 'NONE',  ( -14.94838282604900748, -0.1191753592594197858, 2.588085963191248506 ) ) ;
#2336=VECTOR ( 'NONE', #43038, 999.9999999999998863 ) ;
#2337=EDGE_LOOP ( 'NONE', ( #55218, #651, #33952, #27378 ) ) ;
#2338=VECTOR ( 'NONE', #44819, 999.9999999999998863 ) ;
#2339=DIRECTION ( 'NONE',  ( 0.007781995580012663651, -3.146120232559066537E-19, -0.9999697198139514409 ) ) ;
#2340=ORIENTED_EDGE ( 'NONE', *, *, #7096, .F. ) ;
#2341=ADVANCED_FACE ( 'NONE', ( #41611 ), #7836, .F. ) ;
#2342=VECTOR ( 'NONE', #53666, 1000.000000000000114 ) ;
#2343=EDGE_LOOP ( 'NONE', ( #38952, #30792, #45064, #46395 ) ) ;
#2344=VECTOR ( 'NONE', #45609, 1000.000000000000000 ) ;
#2345=VERTEX_POINT ( 'NONE', #12060 ) ;
#2346=DIRECTION ( 'NONE',  ( 0.5449076811759707706, 0.6444004775717708799, -0.5364919789714476250 ) ) ;
#2347=ADVANCED_FACE ( 'NONE', ( #50693 ), #2693, .F. ) ;
#2348=ORIENTED_EDGE ( 'NONE', *, *, #44025, .T. ) ;
#2349=PLANE ( 'NONE',  #13952 ) ;
#2350=ORIENTED_EDGE ( 'NONE', *, *, #40253, .F. ) ;
#2351=LINE ( 'NONE', #45241, #7733 ) ;
#2352=DIRECTION ( 'NONE',  ( -0.5364919789714478471, 0.6444004775717705469, -0.5449076811759709926 ) ) ;
#2353=ORIENTED_EDGE ( 'NONE', *, *, #52080, .T. ) ;
#2354=ADVANCED_FACE ( 'NONE', ( #33638 ), #11782, .F. ) ;
#2355=CARTESIAN_POINT ( 'NONE',  ( -15.60102546347950536, 0.000000000000000000, 12.95077420755565356 ) ) ;
#2356=EDGE_LOOP ( 'NONE', ( #53429, #41604, #29760, #51916 ) ) ;
#2357=VECTOR ( 'NONE', #19289, 1000.000000000000227 ) ;
#2358=LINE ( 'NONE', #15412, #4721 ) ;
#2359=CARTESIAN_POINT ( 'NONE',  ( -20.54049170961573267, 0.000000000000000000, 4.660556269540326646 ) ) ;
#2360=DIRECTION ( 'NONE',  ( -0.6427681459581293666, -0.7660444431189770143, -0.005002170337467561935 ) ) ;
#2361=FACE_OUTER_BOUND ( 'NONE', #24008, .T. ) ;
#2362=DIRECTION ( 'NONE',  ( -0.7660212471507179544, -0.6427876096865405842, -0.005961354470445141482 ) ) ;
#2363=LINE ( 'NONE', #17826, #17373 ) ;
#2364=CARTESIAN_POINT ( 'NONE',  ( -19.25546368286732601, 0.000000000000000000, 4.870562710998793676 ) ) ;
#2365=AXIS2_PLACEMENT_3D ( 'NONE', #3828, #16925, #51554 ) ;
#2366=ORIENTED_EDGE ( 'NONE', *, *, #16292, .T. ) ;
#2367=VERTEX_POINT ( 'NONE', #47001 ) ;
#2368=DIRECTION ( 'NONE',  ( 0.6427681459581294776, -0.7660444431189769032, 0.005002170337467562802 ) ) ;
#2370=VECTOR ( 'NONE', #45386, 999.9999999999998863 ) ;
#2371=DIRECTION ( 'NONE',  ( -0.5364919789714478471, 0.6444004775717705469, -0.5449076811759709926 ) ) ;
#2372=CARTESIAN_POINT ( 'NONE',  ( -17.93139508144814442, 0.000000000000000000, 13.85596890686001537 ) ) ;
#2373=VECTOR ( 'NONE', #13068, 999.9999999999998863 ) ;
#2374=VECTOR ( 'NONE', #13671, 1000.000000000000000 ) ;
#2375=DIRECTION ( 'NONE',  ( 0.005002170337468016433, -0.7660444431189770143, -0.6427681459581293666 ) ) ;
#2376=VERTEX_POINT ( 'NONE', #16604 ) ;
#2377=CARTESIAN_POINT ( 'NONE',  ( -19.06773268699349799, 2.553033558614008047, 4.007031512929001948 ) ) ;
#2378=DIRECTION ( 'NONE',  ( -0.7660212471507179544, -0.6427876096865405842, -0.005961354470445141482 ) ) ;
#2379=ORIENTED_EDGE ( 'NONE', *, *, #46707, .F. ) ;
#2380=DIRECTION ( 'NONE',  ( -0.9999697198139514409, -0.000000000000000000, -0.007781995580013368816 ) ) ;
#2381=EDGE_CURVE ( 'NONE', #33688, #5490, #37341, .T. ) ;
#2382=CARTESIAN_POINT ( 'NONE',  ( -13.27065584551087163, 0.000000000000000000, 12.04557950825129176 ) ) ;
#2383=EDGE_LOOP ( 'NONE', ( #27741, #52301, #35795, #41586, #3485 ) ) ;
#2384=VECTOR ( 'NONE', #45879, 999.9999999999998863 ) ;
#2385=EDGE_CURVE ( 'NONE', #30192, #45499, #7253, .T. ) ;
#2387=DIRECTION ( 'NONE',  ( 0.7660212471507180654, -0.6427876096865404731, 0.005961354470445141482 ) ) ;
#2388=AXIS2_PLACEMENT_3D ( 'NONE', #29323, #46637, #20534 ) ;
#2389=LINE ( 'NONE', #19717, #5975 ) ;
#2390=ADVANCED_FACE ( 'NONE', ( #16910 ), #55498, .F. ) ;
#2391=CARTESIAN_POINT ( 'NONE',  ( -24.27063949748155380, 0.000000000000000000, 6.308861732390097288 ) ) ;
#2392=VECTOR ( 'NONE', #40341, 1000.000000000000227 ) ;
#2394=VERTEX_POINT ( 'NONE', #24854 ) ;
#2395=AXIS2_PLACEMENT_3D ( 'NONE', #36209, #18892, #27385 ) ;
#2396=EDGE_LOOP ( 'NONE', ( #12277, #6153, #16177, #40514 ) ) ;
#2398=LINE ( 'NONE', #36215, #42166 ) ;
#2399=DIRECTION ( 'NONE',  ( -0.5364919789714478471, 0.6444004775717705469, -0.5449076811759709926 ) ) ;
#2400=DIRECTION ( 'NONE',  ( -0.5449076811759708816, 0.6444004775717707689, 0.5364919789714475140 ) ) ;
#2402=LINE ( 'NONE', #48983, #20377 ) ;
#2403=VERTEX_POINT ( 'NONE', #20304 ) ;
#2404=CARTESIAN_POINT ( 'NONE',  ( -13.27065584551087163, 0.000000000000000000, 12.04557950825129176 ) ) ;
#2405=VECTOR ( 'NONE', #46121, 999.9999999999998863 ) ;
#2406=EDGE_CURVE ( 'NONE', #54118, #12005, #54654, .T. ) ;
#2407=CARTESIAN_POINT ( 'NONE',  ( -20.54126990917373519, -0.1191753592594197858, 4.760553241521720658 ) ) ;
#2408=LINE ( 'NONE', #14914, #53228 ) ;
#2409=ORIENTED_EDGE ( 'NONE', *, *, #10214, .T. ) ;
#2413=AXIS2_PLACEMENT_3D ( 'NONE', #3140, #55121, #12229 ) ;
#2414=FACE_OUTER_BOUND ( 'NONE', #44645, .T. ) ;
#2415=ORIENTED_EDGE ( 'NONE', *, *, #54672, .T. ) ;
#2416=FACE_OUTER_BOUND ( 'NONE', #22042, .T. ) ;
#2417=VECTOR ( 'NONE', #51836, 999.9999999999998863 ) ;
#2418=ORIENTED_EDGE ( 'NONE', *, *, #48924, .F. ) ;
#2419=ORIENTED_EDGE ( 'NONE', *, *, #18520, .F. ) ;
#2420=AXIS2_PLACEMENT_3D ( 'NONE', #19201, #40546, #40240 ) ;
#2421=ORIENTED_EDGE ( 'NONE', *, *, #14087, .F. ) ;
#2422=ORIENTED_EDGE ( 'NONE', *, *, #14638, .T. ) ;
#2423=EDGE_LOOP ( 'NONE', ( #14543, #51405, #35060, #33867 ) ) ;
#2424=DIRECTION ( 'NONE',  ( 0.7660212471507180654, -0.6427876096865404731, 0.005961354470445141482 ) ) ;
#2425=ORIENTED_EDGE ( 'NONE', *, *, #48924, .T. ) ;
#2426=VECTOR ( 'NONE', #40847, 999.9999999999998863 ) ;
#2428=PLANE ( 'NONE',  #14148 ) ;
#2429=EDGE_CURVE ( 'NONE', #40913, #40301, #8105, .T. ) ;
#2430=EDGE_LOOP ( 'NONE', ( #10941, #48817, #52631, #54645 ) ) ;
#2431=ORIENTED_EDGE ( 'NONE', *, *, #15801, .T. ) ;
#2433=ORIENTED_EDGE ( 'NONE', *, *, #21854, .F. ) ;
#2434=AXIS2_PLACEMENT_3D ( 'NONE', #10521, #45154, #6256 ) ;
#2435=LINE ( 'NONE', #11227, #7557 ) ;
#2436=DIRECTION ( 'NONE',  ( -0.005961354470445682716, -0.6427876096865404731, 0.7660212471507180654 ) ) ;
#2437=DIRECTION ( 'NONE',  ( -0.7660212471507179544, -0.6427876096865405842, -0.005961354470445141482 ) ) ;
#2438=LINE ( 'NONE', #2141, #14166 ) ;
#2439=ORIENTED_EDGE ( 'NONE', *, *, #30729, .F. ) ;
#2440=DIRECTION ( 'NONE',  ( 0.5364919789714477361, 0.6444004775717706579, 0.5449076811759711036 ) ) ;
#2441=ORIENTED_EDGE ( 'NONE', *, *, #25891, .F. ) ;
#2442=EDGE_CURVE ( 'NONE', #8484, #36489, #3818, .T. ) ;
#2443=ORIENTED_EDGE ( 'NONE', *, *, #20343, .T. ) ;
#2444=DIRECTION ( 'NONE',  ( -0.5364919789714478471, 0.6444004775717705469, -0.5449076811759709926 ) ) ;
#2445=DIRECTION ( 'NONE',  ( 0.000000000000000000, -0.000000000000000000, -1.000000000000000000 ) ) ;
#2447=EDGE_CURVE ( 'NONE', #83, #1327, #16319, .T. ) ;
#2448=EDGE_CURVE ( 'NONE', #52648, #17442, #47259, .T. ) ;
#2449=VECTOR ( 'NONE', #17949, 1000.000000000000000 ) ;
#2451=DIRECTION ( 'NONE',  ( -0.5449076811759708816, 0.6444004775717707689, 0.5364919789714475140 ) ) ;
#2453=DIRECTION ( 'NONE',  ( -0.9999697198139514409, -0.000000000000000000, -0.007781995580013368816 ) ) ;
#2454=ORIENTED_EDGE ( 'NONE', *, *, #7570, .T. ) ;
#2455=PLANE ( 'NONE',  #34686 ) ;
#2456=EDGE_CURVE ( 'NONE', #13435, #22728, #39034, .T. ) ;
#2457=EDGE_LOOP ( 'NONE', ( #12102, #15454, #25794, #32455 ) ) ;
#2459=DIRECTION ( 'NONE',  ( 0.9999697198139515519, 0.000000000000000000, 0.007781995580013368816 ) ) ;
#2460=ADVANCED_FACE ( 'NONE', ( #12911 ), #31064, .F. ) ;
#2461=VECTOR ( 'NONE', #30511, 1000.000000000000000 ) ;
#2463=LINE ( 'NONE', #24321, #2294 ) ;
#2464=EDGE_CURVE ( 'NONE', #22669, #33221, #48103, .T. ) ;
#2465=FACE_OUTER_BOUND ( 'NONE', #50742, .T. ) ;
#2466=VECTOR ( 'NONE', #3509, 999.9999999999998863 ) ;
#2467=ORIENTED_EDGE ( 'NONE', *, *, #54466, .T. ) ;
#2468=DIRECTION ( 'NONE',  ( 0.007781995580012663651, 0.000000000000000000, -0.9999697198139515519 ) ) ;
#2469=DIRECTION ( 'NONE',  ( -0.7660212471507179544, -0.6427876096865405842, -0.005961354470445141482 ) ) ;
#2470=LINE ( 'NONE', #15794, #3398 ) ;
#2471=ADVANCED_FACE ( 'NONE', ( #21724 ), #8671, .F. ) ;
#2472=AXIS2_PLACEMENT_3D ( 'NONE', #20023, #24025, #10712 ) ;
#2473=DIRECTION ( 'NONE',  ( -0.005002170337468016433, -0.7660444431189770143, 0.6427681459581293666 ) ) ;
#2474=PLANE ( 'NONE',  #3105 ) ;
#2475=DIRECTION ( 'NONE',  ( 0.000000000000000000, 1.000000000000000000, 0.000000000000000000 ) ) ;
#2476=PLANE ( 'NONE',  #53730 ) ;
#2477=EDGE_CURVE ( 'NONE', #27257, #5134, #34774, .T. ) ;
#2478=DIRECTION ( 'NONE',  ( -0.3620778797217457656, 0.000000000000000000, -0.9321478471874540261 ) ) ;
#2479=CARTESIAN_POINT ( 'NONE',  ( -25.20278734466900517, 0.000000000000000000, 6.670939612111840944 ) ) ;
#2480=ORIENTED_EDGE ( 'NONE', *, *, #19962, .F. ) ;
#2481=ORIENTED_EDGE ( 'NONE', *, *, #31753, .F. ) ;
#2482=ORIENTED_EDGE ( 'NONE', *, *, #34192, .T. ) ;
#2483=ORIENTED_EDGE ( 'NONE', *, *, #36120, .T. ) ;
#2484=ORIENTED_EDGE ( 'NONE', *, *, #53692, .T. ) ;
#2486=DIRECTION ( 'NONE',  ( 0.005002170337468016433, -0.7660444431189770143, -0.6427681459581293666 ) ) ;
#2487=LINE ( 'NONE', #19805, #38349 ) ;
#2488=CARTESIAN_POINT ( 'NONE',  ( -15.43759333659924415, -0.1191753592594194527, 4.800271232719476089 ) ) ;
#2489=ORIENTED_EDGE ( 'NONE', *, *, #45101, .T. ) ;
#2490=DIRECTION ( 'NONE',  ( -0.5364919789714478471, 0.6444004775717705469, -0.5449076811759709926 ) ) ;
#2491=EDGE_CURVE ( 'NONE', #9864, #44261, #18280, .T. ) ;
#2492=ORIENTED_EDGE ( 'NONE', *, *, #46593, .F. ) ;
#2493=VERTEX_POINT ( 'NONE', #21985 ) ;
#2494=VECTOR ( 'NONE', #36470, 999.9999999999998863 ) ;
#2496=DIRECTION ( 'NONE',  ( 0.6246952433987893460, 0.7422098413412802076, -0.2426528472758539279 ) ) ;
#2497=FACE_OUTER_BOUND ( 'NONE', #3491, .T. ) ;
#2498=ORIENTED_EDGE ( 'NONE', *, *, #32208, .T. ) ;
#2499=LINE ( 'NONE', #49903, #12904 ) ;
#2500=EDGE_CURVE ( 'NONE', #23765, #44810, #25999, .T. ) ;
#2501=VECTOR ( 'NONE', #29255, 1000.000000000000227 ) ;
#2502=DIRECTION ( 'NONE',  ( 0.9999697198139515519, 0.000000000000000000, 0.007781995580013368816 ) ) ;
#2503=PLANE ( 'NONE',  #16677 ) ;
#2504=EDGE_CURVE ( 'NONE', #18224, #23248, #5257, .T. ) ;
#2505=LINE ( 'NONE', #40846, #24484 ) ;
#2506=DIRECTION ( 'NONE',  ( -0.5449076811759708816, 0.6444004775717707689, 0.5364919789714475140 ) ) ;
#2507=LINE ( 'NONE', #10185, #14989 ) ;
#2508=DIRECTION ( 'NONE',  ( -0.5449076811759708816, 0.6444004775717707689, 0.5364919789714475140 ) ) ;
#2509=CARTESIAN_POINT ( 'NONE',  ( -9.110551994824897193, -1.000000000000000000, 3.538847790438064411 ) ) ;
#2510=CARTESIAN_POINT ( 'NONE',  ( -13.73537992771392702, 3.362543313726507499, 7.735115571941824086 ) ) ;
#2511=ORIENTED_EDGE ( 'NONE', *, *, #44312, .T. ) ;
#2513=ORIENTED_EDGE ( 'NONE', *, *, #16957, .T. ) ;
#2514=DIRECTION ( 'NONE',  ( 0.9999697198139515519, 0.000000000000000000, 0.007781995580013368816 ) ) ;
#2515=CARTESIAN_POINT ( 'NONE',  ( -11.69321732157139948, -0.1191753592594181482, 1.323669135366288829 ) ) ;
#2516=EDGE_CURVE ( 'NONE', #55726, #52569, #22564, .T. ) ;
#2517=LINE ( 'NONE', #37157, #45875 ) ;
#2518=PLANE ( 'NONE',  #19609 ) ;
#2519=CARTESIAN_POINT ( 'NONE',  ( -11.40636015113596180, 0.000000000000000000, 11.32142374880780089 ) ) ;
#2520=EDGE_CURVE ( 'NONE', #35585, #1901, #9497, .T. ) ;
#2521=LINE ( 'NONE', #41960, #31031 ) ;
#2522=ORIENTED_EDGE ( 'NONE', *, *, #37873, .F. ) ;
#2523=CARTESIAN_POINT ( 'NONE',  ( -20.54204810873173415, 0.000000000000000000, 4.860550213503115558 ) ) ;
#2524=FACE_OUTER_BOUND ( 'NONE', #13127, .T. ) ;
#2525=DIRECTION ( 'NONE',  ( 0.9999697198139515519, 0.000000000000000000, 0.007781995580013368816 ) ) ;
#2526=DIRECTION ( 'NONE',  ( 0.000000000000000000, -0.000000000000000000, -1.000000000000000000 ) ) ;
#2527=CARTESIAN_POINT ( 'NONE',  ( -24.26986129792355129, -0.1191753592594197858, 6.208864760408702388 ) ) ;
#2528=ADVANCED_FACE ( 'NONE', ( #25691 ), #26821, .F. ) ;
#2529=LINE ( 'NONE', #44857, #52683 ) ;
#2530=LINE ( 'NONE', #36622, #11225 ) ;
#2531=DIRECTION ( 'NONE',  ( 0.005002170337468016433, -0.7660444431189770143, -0.6427681459581293666 ) ) ;
#2532=LINE ( 'NONE', #45682, #29280 ) ;
#2533=ORIENTED_EDGE ( 'NONE', *, *, #522, .F. ) ;
#2534=EDGE_CURVE ( 'NONE', #41874, #50265, #39621, .T. ) ;
#2535=CARTESIAN_POINT ( 'NONE',  ( -10.28764359011176488, -0.1191753592594198830, 0.7776965645825208995 ) ) ;
#2536=EDGE_LOOP ( 'NONE', ( #8985, #21040, #11183, #53662 ) ) ;
#2537=CARTESIAN_POINT ( 'NONE',  ( -17.83139810946674686, -0.1191753592594197858, 13.85674710641801788 ) ) ;
#2538=DIRECTION ( 'NONE',  ( 0.9999697198139515519, 0.000000000000000000, 0.007781995580013368816 ) ) ;
#2539=VECTOR ( 'NONE', #9517, 1000.000000000000114 ) ;
#2540=ORIENTED_EDGE ( 'NONE', *, *, #55280, .F. ) ;
#2542=CARTESIAN_POINT ( 'NONE',  ( -12.73617685956571322, 0.000000000000000000, 3.074636959462103469 ) ) ;
#2543=ORIENTED_EDGE ( 'NONE', *, *, #53364, .T. ) ;
#2544=ORIENTED_EDGE ( 'NONE', *, *, #39856, .T. ) ;
#2545=VERTEX_POINT ( 'NONE', #34489 ) ;
#2546=DIRECTION ( 'NONE',  ( -0.9999697198139514409, -0.000000000000000000, -0.007781995580013368816 ) ) ;
#2547=LINE ( 'NONE', #32402, #38641 ) ;
#2548=DIRECTION ( 'NONE',  ( 0.000000000000000000, -1.000000000000000000, 0.000000000000000000 ) ) ;
#2549=ADVANCED_FACE ( 'NONE', ( #700 ), #35613, .F. ) ;
#2550=ORIENTED_EDGE ( 'NONE', *, *, #45445, .F. ) ;
#2551=EDGE_CURVE ( 'NONE', #49537, #2028, #30541, .T. ) ;
#2552=VERTEX_POINT ( 'NONE', #30242 ) ;
#2554=LINE ( 'NONE', #19876, #6454 ) ;
#2555=ORIENTED_EDGE ( 'NONE', *, *, #37718, .T. ) ;
#2556=EDGE_CURVE ( 'NONE', #8862, #55978, #35341, .T. ) ;
#2557=PLANE ( 'NONE',  #26432 ) ;
#2558=ORIENTED_EDGE ( 'NONE', *, *, #16904, .T. ) ;
#2559=LINE ( 'NONE', #49717, #10363 ) ;
#2560=FACE_OUTER_BOUND ( 'NONE', #8428, .T. ) ;
#2561=EDGE_CURVE ( 'NONE', #37629, #44931, #8954, .T. ) ;
#2562=ADVANCED_FACE ( 'NONE', ( #13485 ), #21454, .F. ) ;
#2563=EDGE_CURVE ( 'NONE', #52991, #17775, #32202, .T. ) ;
#2564=ORIENTED_EDGE ( 'NONE', *, *, #36836, .F. ) ;
#2565=CARTESIAN_POINT ( 'NONE',  ( -11.40636015113596180, 0.000000000000000000, 11.32142374880780089 ) ) ;
#2566=PLANE ( 'NONE',  #24559 ) ;
#2567=ORIENTED_EDGE ( 'NONE', *, *, #25164, .T. ) ;
#2569=LINE ( 'NONE', #23593, #40251 ) ;
#2570=CARTESIAN_POINT ( 'NONE',  ( -13.96236475351288497, 3.686347215771509589, 1.987774589328580532 ) ) ;
#2571=ORIENTED_EDGE ( 'NONE', *, *, #2504, .T. ) ;
#2572=VECTOR ( 'NONE', #43518, 1000.000000000000000 ) ;
#2574=CARTESIAN_POINT ( 'NONE',  ( -19.88163492745564298, 4.010151117816508126, 11.18536447734173933 ) ) ;
#2576=ADVANCED_FACE ( 'NONE', ( #10049 ), #49526, .F. ) ;
#2577=DIRECTION ( 'NONE',  ( -0.9999697198139514409, -0.000000000000000000, -0.007781995580013368816 ) ) ;
#2578=CARTESIAN_POINT ( 'NONE',  ( -17.83139810946674686, -0.1191753592594197858, 13.85674710641801788 ) ) ;
#2579=DIRECTION ( 'NONE',  ( 0.6427681459581294776, -0.7660444431189769032, 0.005002170337467562802 ) ) ;
#2580=EDGE_CURVE ( 'NONE', #35585, #12064, #10884, .T. ) ;
#2581=FACE_OUTER_BOUND ( 'NONE', #35716, .T. ) ;
#2582=ORIENTED_EDGE ( 'NONE', *, *, #6427, .T. ) ;
#2583=CARTESIAN_POINT ( 'NONE',  ( -17.74560456716937296, 0.000000000000000000, 3.774316574337878372 ) ) ;
#2584=LINE ( 'NONE', #37810, #48571 ) ;
#2585=ADVANCED_FACE ( 'NONE', ( #49792 ), #23123, .F. ) ;
#2588=CARTESIAN_POINT ( 'NONE',  ( -16.53317331066696383, 0.000000000000000000, 13.31285208727739899 ) ) ;
#2590=CARTESIAN_POINT ( 'NONE',  ( -12.67969208061091813, 1.581621852479006440, 4.402255037361733514 ) ) ;
#2591=EDGE_CURVE ( 'NONE', #7363, #17655, #15417, .T. ) ;
#2592=CARTESIAN_POINT ( 'NONE',  ( 2.072287782118878319, 0.000000000000000000, -2.950529333540147015 ) ) ;
#2593=CARTESIAN_POINT ( 'NONE',  ( -23.33693525117809386, 0.000000000000000000, 5.746789908705562944 ) ) ;
#2594=EDGE_CURVE ( 'NONE', #20663, #18937, #19696, .T. ) ;
#2595=LINE ( 'NONE', #1753, #23849 ) ;
#2596=ORIENTED_EDGE ( 'NONE', *, *, #22720, .T. ) ;
#2597=ORIENTED_EDGE ( 'NONE', *, *, #9887, .T. ) ;
#2598=DIRECTION ( 'NONE',  ( 0.007781995580012663651, -3.146120232559066537E-19, -0.9999697198139514409 ) ) ;
#2599=CARTESIAN_POINT ( 'NONE',  ( -16.75240362923608473, 0.000000000000000000, 7.475366591759194712 ) ) ;
#2600=VERTEX_POINT ( 'NONE', #2364 ) ;
#2601=CARTESIAN_POINT ( 'NONE',  ( -15.53262040112807441, 0.000000000000000000, 4.160870598627338879 ) ) ;
#2603=DIRECTION ( 'NONE',  ( 0.005002170337468016433, -0.7660444431189770143, -0.6427681459581293666 ) ) ;
#2605=ORIENTED_EDGE ( 'NONE', *, *, #26683, .T. ) ;
#2606=CARTESIAN_POINT ( 'NONE',  ( -11.65596995895249854, -1.165603555308155626, 3.122460313520408093 ) ) ;
#2607=PLANE ( 'NONE',  #50430 ) ;
#2608=DIRECTION ( 'NONE',  ( 0.5364919789714477361, 0.6444004775717706579, 0.5449076811759711036 ) ) ;
#2609=ORIENTED_EDGE ( 'NONE', *, *, #31310, .F. ) ;
#2610=AXIS2_PLACEMENT_3D ( 'NONE', #34638, #13373, #3697 ) ;
#2611=DIRECTION ( 'NONE',  ( 0.007781995580012662783, 0.000000000000000000, -0.9999697198139514409 ) ) ;
#2612=ORIENTED_EDGE ( 'NONE', *, *, #21713, .T. ) ;
#2613=ORIENTED_EDGE ( 'NONE', *, *, #24050, .F. ) ;
#2614=ORIENTED_EDGE ( 'NONE', *, *, #25582, .F. ) ;
#2615=DIRECTION ( 'NONE',  ( 0.005002170337468016433, -0.7660444431189770143, -0.6427681459581293666 ) ) ;
#2616=EDGE_LOOP ( 'NONE', ( #31636, #8403, #13235, #6325 ) ) ;
#2617=DIRECTION ( 'NONE',  ( 0.6427681459581294776, -0.7660444431189769032, 0.005002170337467562802 ) ) ;
#2619=DIRECTION ( 'NONE',  ( -0.7660212471507179544, -0.6427876096865405842, -0.005961354470445141482 ) ) ;
#2620=CARTESIAN_POINT ( 'NONE',  ( -14.01701317841955508, 0.000000000000000000, 2.326005055450897085 ) ) ;
#2621=EDGE_CURVE ( 'NONE', #25423, #34828, #1238, .T. ) ;
#2622=EDGE_CURVE ( 'NONE', #10480, #16665, #45252, .T. ) ;
#2623=ORIENTED_EDGE ( 'NONE', *, *, #45, .F. ) ;
#2624=DIRECTION ( 'NONE',  ( -0.005002170337468016433, -0.7660444431189770143, 0.6427681459581293666 ) ) ;
#2625=ORIENTED_EDGE ( 'NONE', *, *, #41798, .T. ) ;
#2626=EDGE_CURVE ( 'NONE', #4790, #18918, #44406, .T. ) ;
#2627=LINE ( 'NONE', #24485, #51846 ) ;
#2629=CARTESIAN_POINT ( 'NONE',  ( -27.06630483948590893, -0.1191753592594197858, 7.295098399573937797 ) ) ;
#2630=DIRECTION ( 'NONE',  ( 0.005961354470445682716, -0.6427876096865404731, -0.7660212471507180654 ) ) ;
#2631=CARTESIAN_POINT ( 'NONE',  ( -11.87243407472968926, 0.000000000000000000, 11.50246268866867361 ) ) ;
#2632=VERTEX_POINT ( 'NONE', #31908 ) ;
#2633=VERTEX_POINT ( 'NONE', #40723 ) ;
#2634=DIRECTION ( 'NONE',  ( -0.9999697198139514409, -0.000000000000000000, -0.007781995580013368816 ) ) ;
#2635=DIRECTION ( 'NONE',  ( 0.007781995580012663651, -3.146120232559066537E-19, -0.9999697198139514409 ) ) ;
#2636=CARTESIAN_POINT ( 'NONE',  ( -15.50102849149811135, -0.1191753592594197858, 12.95155240711365430 ) ) ;
#2638=EDGE_CURVE ( 'NONE', #33054, #36712, #49224, .T. ) ;
#2639=PLANE ( 'NONE',  #52159 ) ;
#2640=ORIENTED_EDGE ( 'NONE', *, *, #14569, .F. ) ;
#2641=CARTESIAN_POINT ( 'NONE',  ( -9.075990533167328067, 0.000000000000000000, 10.41622904950343909 ) ) ;
#2642=DIRECTION ( 'NONE',  ( 0.000000000000000000, -1.000000000000000000, 0.000000000000000000 ) ) ;
#2643=ORIENTED_EDGE ( 'NONE', *, *, #5906, .T. ) ;
#2644=CARTESIAN_POINT ( 'NONE',  ( -16.95084117408287483, 0.000000000000000000, 7.273816248680401664 ) ) ;
#2645=DIRECTION ( 'NONE',  ( 0.7660212471507180654, -0.6427876096865404731, 0.005961354470445141482 ) ) ;
#2646=ORIENTED_EDGE ( 'NONE', *, *, #34681, .T. ) ;
#2647=CARTESIAN_POINT ( 'NONE',  ( -11.80690306588353877, 0.000000000000000000, 3.081868782998124168 ) ) ;
#2648=CARTESIAN_POINT ( 'NONE',  ( -8.409922665610809034, 0.000000000000000000, 10.23674650875856962 ) ) ;
#2649=ADVANCED_FACE ( 'NONE', ( #44679 ), #10338, .F. ) ;
#2650=CARTESIAN_POINT ( 'NONE',  ( -15.87975247367846166, 0.000000000000000000, 2.850166870931599927 ) ) ;
#2651=EDGE_CURVE ( 'NONE', #48176, #17974, #6105, .T. ) ;
#2652=LINE ( 'NONE', #50370, #9671 ) ;
#2653=LINE ( 'NONE', #41571, #207 ) ;
#2654=VERTEX_POINT ( 'NONE', #56210 ) ;
#2655=ADVANCED_FACE ( 'NONE', ( #28480 ), #25286, .F. ) ;
#2656=EDGE_LOOP ( 'NONE', ( #28530, #2219, #10536, #11574 ) ) ;
#2657=FACE_OUTER_BOUND ( 'NONE', #21406, .T. ) ;
#2658=LINE ( 'NONE', #8068, #39459 ) ;
#2659=LINE ( 'NONE', #7218, #55894 ) ;
#2660=ADVANCED_FACE ( 'NONE', ( #8824 ), #55954, .F. ) ;
#2661=FACE_OUTER_BOUND ( 'NONE', #13265, .T. ) ;
#2662=LINE ( 'NONE', #37053, #38291 ) ;
#2663=ADVANCED_FACE ( 'NONE', ( #11154 ), #16458, .F. ) ;
#2664=PLANE ( 'NONE',  #47596 ) ;
#2665=ORIENTED_EDGE ( 'NONE', *, *, #16428, .T. ) ;
#2666=DIRECTION ( 'NONE',  ( -0.7660212471507179544, -0.6427876096865405842, -0.005961354470445141482 ) ) ;
#2667=LINE ( 'NONE', #33066, #23300 ) ;
#2668=LINE ( 'NONE', #46682, #49617 ) ;
#2669=ORIENTED_EDGE ( 'NONE', *, *, #33178, .T. ) ;
#2670=CARTESIAN_POINT ( 'NONE',  ( 2.072287782118878319, 0.000000000000000000, -2.950529333540147015 ) ) ;
#2671=DIRECTION ( 'NONE',  ( 0.005002170337468016433, -0.7660444431189770143, -0.6427681459581293666 ) ) ;
#2672=FACE_OUTER_BOUND ( 'NONE', #36158, .T. ) ;
#2673=VERTEX_POINT ( 'NONE', #17048 ) ;
#2674=LINE ( 'NONE', #28246, #4137 ) ;
#2675=EDGE_LOOP ( 'NONE', ( #22676, #55865, #37196, #47851 ) ) ;
#2676=ORIENTED_EDGE ( 'NONE', *, *, #13463, .F. ) ;
#2678=ORIENTED_EDGE ( 'NONE', *, *, #50651, .T. ) ;
#2679=VERTEX_POINT ( 'NONE', #34363 ) ;
#2680=CARTESIAN_POINT ( 'NONE',  ( -12.66989033008971077, -0.1191753592594181482, 7.407134626131880673 ) ) ;
#2681=ORIENTED_EDGE ( 'NONE', *, *, #18929, .T. ) ;
#2682=EDGE_CURVE ( 'NONE', #19674, #30623, #30386, .T. ) ;
#2684=LINE ( 'NONE', #10404, #50307 ) ;
#2685=ORIENTED_EDGE ( 'NONE', *, *, #33239, .F. ) ;
#2687=EDGE_CURVE ( 'NONE', #41949, #53748, #25005, .T. ) ;
#2688=ADVANCED_FACE ( 'NONE', ( #29555 ), #33786, .F. ) ;
#2689=LINE ( 'NONE', #24012, #47534 ) ;
#2690=DIRECTION ( 'NONE',  ( -0.5449076811759708816, 0.6444004775717707689, 0.5364919789714475140 ) ) ;
#2692=DIRECTION ( 'NONE',  ( 0.5449076811759707706, 0.6444004775717708799, -0.5364919789714476250 ) ) ;
#2693=PLANE ( 'NONE',  #22921 ) ;
#2694=VERTEX_POINT ( 'NONE', #3683 ) ;
#2695=VERTEX_POINT ( 'NONE', #25547 ) ;
#2696=DIRECTION ( 'NONE',  ( 0.9999697198139515519, 0.000000000000000000, 0.007781995580013368816 ) ) ;
#2697=CARTESIAN_POINT ( 'NONE',  ( -16.33317936670417225, 0.000000000000000000, 13.31440848639340224 ) ) ;
#2698=EDGE_CURVE ( 'NONE', #38787, #27265, #51667, .T. ) ;
#2699=FACE_OUTER_BOUND ( 'NONE', #6781, .T. ) ;
#2700=DIRECTION ( 'NONE',  ( -0.005961354470445682716, -0.6427876096865404731, 0.7660212471507180654 ) ) ;
#2701=DIRECTION ( 'NONE',  ( 0.9321478471874541372, 0.000000000000000000, -0.3620778797217453771 ) ) ;
#2702=DIRECTION ( 'NONE',  ( 0.7660212471507180654, -0.6427876096865404731, 0.005961354470445141482 ) ) ;
#2703=ORIENTED_EDGE ( 'NONE', *, *, #46106, .T. ) ;
#2704=LINE ( 'NONE', #54669, #7488 ) ;
#2705=ORIENTED_EDGE ( 'NONE', *, *, #17146, .F. ) ;
#2706=DIRECTION ( 'NONE',  ( 0.005961354470445682716, -0.6427876096865404731, -0.7660212471507180654 ) ) ;
#2707=DIRECTION ( 'NONE',  ( 0.7660212471507180654, -0.6427876096865404731, 0.005961354470445141482 ) ) ;
#2708=CARTESIAN_POINT ( 'NONE',  ( -12.09672020551653127, 4.172053068839010059, 8.427147906474264261 ) ) ;
#2709=CARTESIAN_POINT ( 'NONE',  ( -21.47419595591918906, 0.000000000000000000, 5.222628093224860102 ) ) ;
#2710=EDGE_CURVE ( 'NONE', #34537, #54647, #20738, .T. ) ;
#2711=LINE ( 'NONE', #55250, #33218 ) ;
#2712=VECTOR ( 'NONE', #41371, 999.9999999999998863 ) ;
#2714=CARTESIAN_POINT ( 'NONE',  ( -21.43680077527565686, -5.051250379848164052, 5.046941201800946963 ) ) ;
#2715=DIRECTION ( 'NONE',  ( 0.7660212471507180654, -0.6427876096865404731, 0.005961354470445141482 ) ) ;
#2716=DIRECTION ( 'NONE',  ( -0.9321478471874540261, 0.000000000000000000, 0.3620778797217457656 ) ) ;
#2717=CARTESIAN_POINT ( 'NONE',  ( -13.27065584551087163, 0.000000000000000000, 12.04557950825129176 ) ) ;
#2718=EDGE_CURVE ( 'NONE', #16343, #8547, #13061, .T. ) ;
#2719=DIRECTION ( 'NONE',  ( -0.9999697198139514409, -0.000000000000000000, -0.007781995580013368816 ) ) ;
#2720=PLANE ( 'NONE',  #51756 ) ;
#2721=LINE ( 'NONE', #21181, #31080 ) ;
#2723=CARTESIAN_POINT ( 'NONE',  ( -11.39548592363199120, 1.743523803501506375, 1.052697918879536676 ) ) ;
#2724=ORIENTED_EDGE ( 'NONE', *, *, #36479, .F. ) ;
#2725=ADVANCED_FACE ( 'NONE', ( #46869 ), #3423, .F. ) ;
#2726=VERTEX_POINT ( 'NONE', #250 ) ;
#2727=EDGE_CURVE ( 'NONE', #44057, #38668, #38322, .T. ) ;
#2728=EDGE_CURVE ( 'NONE', #10018, #30955, #55651, .T. ) ;
#2729=ORIENTED_EDGE ( 'NONE', *, *, #52591, .F. ) ;
#2730=EDGE_LOOP ( 'NONE', ( #27336, #48814, #5995 ) ) ;
#2731=EDGE_LOOP ( 'NONE', ( #39469, #448, #52549, #15398 ) ) ;
#2732=ORIENTED_EDGE ( 'NONE', *, *, #27498, .T. ) ;
#2733=DIRECTION ( 'NONE',  ( 0.007781995580012663651, 0.000000000000000000, -0.9999697198139515519 ) ) ;
#2734=LINE ( 'NONE', #15525, #45608 ) ;
#2735=EDGE_CURVE ( 'NONE', #52431, #43283, #16754, .T. ) ;
#2736=PLANE ( 'NONE',  #48471 ) ;
#2737=ORIENTED_EDGE ( 'NONE', *, *, #55575, .T. ) ;
#2738=EDGE_CURVE ( 'NONE', #55501, #41332, #51938, .T. ) ;
#2739=CARTESIAN_POINT ( 'NONE',  ( -15.96710241509184058, -0.1191753592594218814, 13.13259134697452879 ) ) ;
#2740=ORIENTED_EDGE ( 'NONE', *, *, #5946, .F. ) ;
#2741=LINE ( 'NONE', #54716, #19523 ) ;
#2742=ORIENTED_EDGE ( 'NONE', *, *, #8559, .T. ) ;
#2743=EDGE_CURVE ( 'NONE', #11370, #17587, #12511, .T. ) ;
#2744=VECTOR ( 'NONE', #28996, 999.9999999999998863 ) ;
#2746=CARTESIAN_POINT ( 'NONE',  ( -10.71015603238914515, -1.165603555308157846, 1.004320582572386655 ) ) ;
#2747=DIRECTION ( 'NONE',  ( 0.9999697198139515519, 0.000000000000000000, 0.007781995580013368816 ) ) ;
#2748=ORIENTED_EDGE ( 'NONE', *, *, #41111, .T. ) ;
#2749=DIRECTION ( 'NONE',  ( -0.5449076811759708816, 0.6444004775717707689, 0.5364919789714475140 ) ) ;
#2750=ORIENTED_EDGE ( 'NONE', *, *, #1486, .F. ) ;
#2751=EDGE_CURVE ( 'NONE', #25140, #49888, #47129, .T. ) ;
#2752=LINE ( 'NONE', #54726, #20044 ) ;
#2753=LINE ( 'NONE', #3620, #4887 ) ;
#2754=EDGE_CURVE ( 'NONE', #38944, #15364, #30676, .T. ) ;
#2755=LINE ( 'NONE', #32875, #40834 ) ;
#2756=DIRECTION ( 'NONE',  ( -0.7660212471507179544, -0.6427876096865405842, -0.005961354470445141482 ) ) ;
#2757=DIRECTION ( 'NONE',  ( 0.7660212471507180654, -0.6427876096865404731, 0.005961354470445141482 ) ) ;
#2758=DIRECTION ( 'NONE',  ( -0.5449076811759708816, 0.6444004775717707689, 0.5364919789714475140 ) ) ;
#2759=DIRECTION ( 'NONE',  ( 0.9999697198139515519, 0.000000000000000000, 0.007781995580013368816 ) ) ;
#2760=CARTESIAN_POINT ( 'NONE',  ( -10.74029228357944987, 0.000000000000000000, 11.14194120806293320 ) ) ;
#2761=CARTESIAN_POINT ( 'NONE',  ( -17.68012102380225414, 0.000000000000000000, 7.268140824260386879 ) ) ;
#2762=EDGE_LOOP ( 'NONE', ( #56046, #24354, #14204, #40634 ) ) ;
#2765=VECTOR ( 'NONE', #55631, 1000.000000000000227 ) ;
#2767=DIRECTION ( 'NONE',  ( 0.9999697198139515519, 0.000000000000000000, 0.007781995580013368816 ) ) ;
#2768=DIRECTION ( 'NONE',  ( 0.005002170337468016433, -0.7660444431189770143, -0.6427681459581293666 ) ) ;
#2769=LINE ( 'NONE', #36906, #22342 ) ;
#2770=FACE_OUTER_BOUND ( 'NONE', #9873, .T. ) ;
#2771=LINE ( 'NONE', #16147, #55511 ) ;
#2773=ORIENTED_EDGE ( 'NONE', *, *, #22297, .F. ) ;
#2774=LINE ( 'NONE', #51050, #21993 ) ;
#2775=DIRECTION ( 'NONE',  ( -0.6246952433987893460, -0.7422098413412802076, 0.2426528472758542054 ) ) ;
#2776=CARTESIAN_POINT ( 'NONE',  ( -11.16658230751120584, 0.000000000000000000, 6.210834479239226269 ) ) ;
#2777=DIRECTION ( 'NONE',  ( 0.005002170337468016433, -0.7660444431189770143, -0.6427681459581293666 ) ) ;
#2778=DIRECTION ( 'NONE',  ( 0.6246952433987894571, -0.7422098413412800966, -0.2426528472758541777 ) ) ;
#2779=VECTOR ( 'NONE', #30383, 1000.000000000000114 ) ;
#2780=CARTESIAN_POINT ( 'NONE',  ( -11.24522430293745501, 0.4483081953215036219, 1.985098250129335495 ) ) ;
#2781=ADVANCED_FACE ( 'NONE', ( #40004 ), #9656, .F. ) ;
#2782=DIRECTION ( 'NONE',  ( 0.6427681459581294776, -0.7660444431189769032, 0.005002170337467562802 ) ) ;
#2783=LINE ( 'NONE', #20408, #617 ) ;
#2784=DIRECTION ( 'NONE',  ( -0.2426528472758541499, 0.7422098413412800966, -0.6246952433987894571 ) ) ;
#2786=VECTOR ( 'NONE', #9300, 1000.000000000000227 ) ;
#2787=DIRECTION ( 'NONE',  ( 0.007781995580012663651, 0.000000000000000000, -0.9999697198139515519 ) ) ;
#2788=DIRECTION ( 'NONE',  ( 0.5449076811759707706, 0.6444004775717708799, -0.5364919789714476250 ) ) ;
#2789=VERTEX_POINT ( 'NONE', #26670 ) ;
#2790=LINE ( 'NONE', #15878, #12215 ) ;
#2791=CARTESIAN_POINT ( 'NONE',  ( -9.745487481051126721, 0.000000000000000000, 2.728579125928399574 ) ) ;
#2792=EDGE_CURVE ( 'NONE', #32241, #56100, #565, .T. ) ;
#2793=ORIENTED_EDGE ( 'NONE', *, *, #11703, .F. ) ;
#2794=ORIENTED_EDGE ( 'NONE', *, *, #32132, .T. ) ;
#2795=CARTESIAN_POINT ( 'NONE',  ( -15.60102546347950536, 0.000000000000000000, 12.95077420755565356 ) ) ;
#2796=ADVANCED_FACE ( 'NONE', ( #35468 ), #26380, .F. ) ;
#2797=ORIENTED_EDGE ( 'NONE', *, *, #4762, .F. ) ;
#2798=ORIENTED_EDGE ( 'NONE', *, *, #40347, .T. ) ;
#2799=VERTEX_POINT ( 'NONE', #39464 ) ;
#2801=PLANE ( 'NONE',  #50166 ) ;
#2802=FACE_OUTER_BOUND ( 'NONE', #39333, .T. ) ;
#2804=DIRECTION ( 'NONE',  ( -0.005961354470445682716, -0.6427876096865404731, 0.7660212471507180654 ) ) ;
#2805=AXIS2_PLACEMENT_3D ( 'NONE', #4769, #22095, #9613 ) ;
#2806=AXIS2_PLACEMENT_3D ( 'NONE', #29236, #24997, #28705 ) ;
#2807=ADVANCED_FACE ( 'NONE', ( #5114 ), #27229, .T. ) ;
#2808=ORIENTED_EDGE ( 'NONE', *, *, #17190, .T. ) ;
#2809=ORIENTED_EDGE ( 'NONE', *, *, #18861, .T. ) ;
#2810=EDGE_CURVE ( 'NONE', #28463, #18921, #43990, .T. ) ;
#2811=DIRECTION ( 'NONE',  ( 0.000000000000000000, -0.000000000000000000, -1.000000000000000000 ) ) ;
#2813=ORIENTED_EDGE ( 'NONE', *, *, #381, .F. ) ;
#2814=DIRECTION ( 'NONE',  ( -0.005002170337468016433, -0.7660444431189770143, 0.6427681459581293666 ) ) ;
#2815=VERTEX_POINT ( 'NONE', #18732 ) ;
#2816=PLANE ( 'NONE',  #41191 ) ;
#2817=DIRECTION ( 'NONE',  ( 0.007781995580012662783, 0.000000000000000000, -0.9999697198139514409 ) ) ;
#2818=EDGE_CURVE ( 'NONE', #40788, #43960, #13883, .T. ) ;
#2819=ORIENTED_EDGE ( 'NONE', *, *, #33090, .T. ) ;
#2821=VECTOR ( 'NONE', #46547, 1000.000000000000000 ) ;
#2822=EDGE_CURVE ( 'NONE', #42246, #17041, #52778, .T. ) ;
#2823=PLANE ( 'NONE',  #30010 ) ;
#2824=ORIENTED_EDGE ( 'NONE', *, *, #16381, .F. ) ;
#2825=PLANE ( 'NONE',  #20406 ) ;
#2826=CARTESIAN_POINT ( 'NONE',  ( -14.32396506529822666, -2.137015261443159009, 2.377053617101271499 ) ) ;
#2827=LINE ( 'NONE', #46871, #26501 ) ;
#2828=VERTEX_POINT ( 'NONE', #39749 ) ;
#2830=CARTESIAN_POINT ( 'NONE',  ( -15.08522782531868245, 0.000000000000000000, 6.380344729941936244 ) ) ;
#2831=LINE ( 'NONE', #37493, #29453 ) ;
#2832=DIRECTION ( 'NONE',  ( -0.005961354470445682716, -0.6427876096865404731, 0.7660212471507180654 ) ) ;
#2833=CARTESIAN_POINT ( 'NONE',  ( -13.02512989487554940, 0.000000000000000000, 6.196370832167189313 ) ) ;
#2834=DIRECTION ( 'NONE',  ( 0.2426528472758541499, 0.7422098413412800966, 0.6246952433987894571 ) ) ;
#2835=DIRECTION ( 'NONE',  ( 0.5364919789714477361, 0.6444004775717706579, 0.5449076811759711036 ) ) ;
#2836=ORIENTED_EDGE ( 'NONE', *, *, #20286, .T. ) ;
#2837=CARTESIAN_POINT ( 'NONE',  ( -25.20200914511100265, -0.1191753592594197858, 6.570942640130446932 ) ) ;
#2838=DIRECTION ( 'NONE',  ( 0.005002170337468016433, -0.7660444431189770143, -0.6427681459581293666 ) ) ;
#2839=FACE_OUTER_BOUND ( 'NONE', #25705, .T. ) ;
#2840=VERTEX_POINT ( 'NONE', #5384 ) ;
#2841=FACE_OUTER_BOUND ( 'NONE', #18482, .T. ) ;
#2842=LINE ( 'NONE', #29264, #19987 ) ;
#2843=VECTOR ( 'NONE', #20640, 1000.000000000000227 ) ;
#2844=AXIS2_PLACEMENT_3D ( 'NONE', #47481, #8595, #4349 ) ;
#2845=CARTESIAN_POINT ( 'NONE',  ( -18.29747203306047609, -0.1191753592594177458, 14.03778604627889059 ) ) ;
#2846=EDGE_CURVE ( 'NONE', #12718, #33290, #53368, .T. ) ;
#2847=CARTESIAN_POINT ( 'NONE',  ( -12.06711556614055425, 0.000000000000000000, 2.510505623125562913 ) ) ;
#2849=ORIENTED_EDGE ( 'NONE', *, *, #8680, .T. ) ;
#2850=EDGE_CURVE ( 'NONE', #42368, #7355, #52513, .T. ) ;
#2851=AXIS2_PLACEMENT_3D ( 'NONE', #4890, #39549, #12848 ) ;
#2852=ORIENTED_EDGE ( 'NONE', *, *, #36181, .T. ) ;
#2853=EDGE_CURVE ( 'NONE', #41757, #16888, #43694, .T. ) ;
#2854=CARTESIAN_POINT ( 'NONE',  ( -14.20280369269832832, 0.000000000000000000, 12.40765738797303719 ) ) ;
#2856=EDGE_CURVE ( 'NONE', #44514, #12005, #22441, .T. ) ;
#2857=EDGE_CURVE ( 'NONE', #33148, #14703, #823, .T. ) ;
#2858=DIRECTION ( 'NONE',  ( 0.5364919789714477361, 0.6444004775717706579, 0.5449076811759711036 ) ) ;
#2859=CARTESIAN_POINT ( 'NONE',  ( -18.62663913851612563, 0.000000000000000000, 9.476767220270952308 ) ) ;
#2860=EDGE_LOOP ( 'NONE', ( #1705, #6529, #37523, #49504 ) ) ;
#2861=CARTESIAN_POINT ( 'NONE',  ( -13.02093818698098637, 0.000000000000000000, 5.657745369614448627 ) ) ;
#2862=VECTOR ( 'NONE', #12985, 1000.000000000000227 ) ;
#2863=EDGE_LOOP ( 'NONE', ( #42435, #41654, #17547, #53947 ) ) ;
#2864=CARTESIAN_POINT ( 'NONE',  ( 1.086233639165236964, 0.000000000000000000, 2.796443541562362078 ) ) ;
#2865=AXIS2_PLACEMENT_3D ( 'NONE', #17953, #29888, #34422 ) ;
#2866=VERTEX_POINT ( 'NONE', #30924 ) ;
#2867=VERTEX_POINT ( 'NONE', #48827 ) ;
#2868=DIRECTION ( 'NONE',  ( -0.5449076811759708816, 0.6444004775717707689, 0.5364919789714475140 ) ) ;
#2869=DIRECTION ( 'NONE',  ( -0.7660212471507179544, -0.6427876096865405842, -0.005961354470445141482 ) ) ;
#2870=FACE_OUTER_BOUND ( 'NONE', #43731, .T. ) ;
#2871=ORIENTED_EDGE ( 'NONE', *, *, #8357, .T. ) ;
#2872=CARTESIAN_POINT ( 'NONE',  ( -18.09544690614880835, -4.403642575758163424, 3.769707965726611487 ) ) ;
#2873=EDGE_CURVE ( 'NONE', #5037, #51473, #23271, .T. ) ;
#2874=ORIENTED_EDGE ( 'NONE', *, *, #30411, .T. ) ;
#2875=ADVANCED_FACE ( 'NONE', ( #47974 ), #48233, .F. ) ;
#2877=ORIENTED_EDGE ( 'NONE', *, *, #44526, .F. ) ;
#2879=CARTESIAN_POINT ( 'NONE',  ( -17.88741947389161524, 0.000000000000000000, 8.205197775622702139 ) ) ;
#2880=EDGE_CURVE ( 'NONE', #24728, #43341, #28914, .T. ) ;
#2881=ORIENTED_EDGE ( 'NONE', *, *, #27054, .F. ) ;
#2882=FACE_OUTER_BOUND ( 'NONE', #23254, .T. ) ;
#2883=ORIENTED_EDGE ( 'NONE', *, *, #24520, .T. ) ;
#2884=CARTESIAN_POINT ( 'NONE',  ( -11.69463168032301326, -0.1191753592594202577, 1.505411197543670365 ) ) ;
#2885=CARTESIAN_POINT ( 'NONE',  ( -15.87975247367846166, 0.000000000000000000, 2.850166870931599927 ) ) ;
#2886=VECTOR ( 'NONE', #39581, 1000.000000000000114 ) ;
#2887=EDGE_CURVE ( 'NONE', #43329, #54540, #28637, .T. ) ;
#2888=VECTOR ( 'NONE', #13063, 999.9999999999998863 ) ;
#2889=ORIENTED_EDGE ( 'NONE', *, *, #52752, .T. ) ;
#2890=PLANE ( 'NONE',  #39525 ) ;
#2891=ORIENTED_EDGE ( 'NONE', *, *, #15645, .F. ) ;
#2892=CARTESIAN_POINT ( 'NONE',  ( -11.87243407472968926, 0.000000000000000000, 11.50246268866867361 ) ) ;
#2893=LINE ( 'NONE', #46080, #9382 ) ;
#2894=VECTOR ( 'NONE', #48238, 1000.000000000000227 ) ;
#2895=DIRECTION ( 'NONE',  ( 0.7660212471507180654, -0.6427876096865404731, 0.005961354470445141482 ) ) ;
#2896=LINE ( 'NONE', #11986, #27515 ) ;
#2897=CARTESIAN_POINT ( 'NONE',  ( -28.92982233430281980, 0.000000000000000000, 7.919257187036034651 ) ) ;
#2898=CARTESIAN_POINT ( 'NONE',  ( -20.43633616049215718, 0.000000000000000000, 5.030698901913927656 ) ) ;
#2899=ORIENTED_EDGE ( 'NONE', *, *, #21688, .T. ) ;
#2900=ORIENTED_EDGE ( 'NONE', *, *, #32772, .F. ) ;
#2902=LINE ( 'NONE', #16003, #44808 ) ;
#2903=VECTOR ( 'NONE', #33445, 999.9999999999998863 ) ;
#2905=DIRECTION ( 'NONE',  ( 0.005961354470445682716, -0.6427876096865404731, -0.7660212471507180654 ) ) ;
#2906=FACE_OUTER_BOUND ( 'NONE', #32702, .T. ) ;
#2907=PLANE ( 'NONE',  #7691 ) ;
#2908=ORIENTED_EDGE ( 'NONE', *, *, #24683, .F. ) ;
#2909=PLANE ( 'NONE',  #55826 ) ;
#2910=FACE_OUTER_BOUND ( 'NONE', #55312, .T. ) ;
#2912=DIRECTION ( 'NONE',  ( 0.9999697198139515519, 0.000000000000000000, 0.007781995580013368816 ) ) ;
#2913=PLANE ( 'NONE',  #14153 ) ;
#2914=ORIENTED_EDGE ( 'NONE', *, *, #43481, .T. ) ;
#2915=DIRECTION ( 'NONE',  ( -0.6427681459581293666, -0.7660444431189770143, -0.005002170337467561935 ) ) ;
#2916=DIRECTION ( 'NONE',  ( 0.007781995580012662783, 0.000000000000000000, -0.9999697198139514409 ) ) ;
#2917=FACE_OUTER_BOUND ( 'NONE', #18796, .T. ) ;
#2918=AXIS2_PLACEMENT_3D ( 'NONE', #41002, #46366, #32228 ) ;
#2919=PLANE ( 'NONE',  #19624 ) ;
#2920=CARTESIAN_POINT ( 'NONE',  ( -19.59569683186026268, 0.000000000000000000, 14.58168106541950948 ) ) ;
#2921=EDGE_LOOP ( 'NONE', ( #19656, #11735, #44024, #28947 ) ) ;
#2922=EDGE_CURVE ( 'NONE', #20518, #8803, #19258, .T. ) ;
#2923=EDGE_LOOP ( 'NONE', ( #52614, #13442, #55232, #24009 ) ) ;
#2924=LINE ( 'NONE', #28228, #44797 ) ;
#2925=DIRECTION ( 'NONE',  ( 0.007781995580012662783, 0.000000000000000000, -0.9999697198139514409 ) ) ;
#2926=VECTOR ( 'NONE', #5765, 1000.000000000000000 ) ;
#2927=CARTESIAN_POINT ( 'NONE',  ( -11.80822072027282132, 0.000000000000000000, 3.251184542293097390 ) ) ;
#2928=EDGE_CURVE ( 'NONE', #4850, #1558, #10491, .T. ) ;
#2929=ADVANCED_FACE ( 'NONE', ( #37411 ), #36312, .F. ) ;
#2930=ADVANCED_FACE ( 'NONE', ( #1925 ), #54732, .F. ) ;
#2931=VECTOR ( 'NONE', #10735, 1000.000000000000227 ) ;
#2932=DIRECTION ( 'NONE',  ( 0.005002170337468016433, -0.7660444431189770143, -0.6427681459581293666 ) ) ;
#2933=VECTOR ( 'NONE', #18950, 1000.000000000000227 ) ;
#2934=CARTESIAN_POINT ( 'NONE',  ( -23.33693525117809386, 0.000000000000000000, 5.746789908705562944 ) ) ;
#2935=DIRECTION ( 'NONE',  ( -0.005961354470445682716, -0.6427876096865404731, 0.7660212471507180654 ) ) ;
#2936=ORIENTED_EDGE ( 'NONE', *, *, #46529, .T. ) ;
#2937=EDGE_CURVE ( 'NONE', #32587, #49888, #53902, .T. ) ;
#2938=DIRECTION ( 'NONE',  ( 0.9999697198139515519, 0.000000000000000000, 0.007781995580013368816 ) ) ;
#2939=PLANE ( 'NONE',  #34163 ) ;
#2940=VECTOR ( 'NONE', #5078, 1000.000000000000227 ) ;
#2941=DIRECTION ( 'NONE',  ( 0.007781995580012662783, 0.000000000000000000, -0.9999697198139514409 ) ) ;
#2942=VECTOR ( 'NONE', #45333, 999.9999999999998863 ) ;
#2943=VERTEX_POINT ( 'NONE', #36590 ) ;
#2945=PLANE ( 'NONE',  #8701 ) ;
#2946=DIRECTION ( 'NONE',  ( 0.7660212471507180654, -0.6427876096865404731, 0.005961354470445141482 ) ) ;
#2947=ORIENTED_EDGE ( 'NONE', *, *, #28986, .T. ) ;
#2948=LINE ( 'NONE', #28831, #5967 ) ;
#2949=AXIS2_PLACEMENT_3D ( 'NONE', #19117, #1792, #27952 ) ;
#2950=ORIENTED_EDGE ( 'NONE', *, *, #25639, .T. ) ;
#2951=AXIS2_PLACEMENT_3D ( 'NONE', #679, #52619, #23096 ) ;
#2952=ADVANCED_FACE ( 'NONE', ( #28070 ), #53623, .F. ) ;
#2953=VERTEX_POINT ( 'NONE', #41673 ) ;
#2954=ORIENTED_EDGE ( 'NONE', *, *, #25341, .T. ) ;
#2955=ORIENTED_EDGE ( 'NONE', *, *, #45559, .F. ) ;
#2956=EDGE_CURVE ( 'NONE', #40825, #9112, #32054, .T. ) ;
#2957=ORIENTED_EDGE ( 'NONE', *, *, #28999, .F. ) ;
#2958=DIRECTION ( 'NONE',  ( -0.9999697198139514409, -0.000000000000000000, -0.007781995580013368816 ) ) ;
#2959=EDGE_LOOP ( 'NONE', ( #42217, #35903, #17895, #34758 ) ) ;
#2960=VECTOR ( 'NONE', #50948, 1000.000000000000000 ) ;
#2961=EDGE_CURVE ( 'NONE', #19083, #21088, #50196, .T. ) ;
#2962=ORIENTED_EDGE ( 'NONE', *, *, #16469, .F. ) ;
#2965=VECTOR ( 'NONE', #31800, 999.9999999999998863 ) ;
#2966=ORIENTED_EDGE ( 'NONE', *, *, #35287, .T. ) ;
#2967=ADVANCED_FACE ( 'NONE', ( #33182 ), #50501, .F. ) ;
#2968=DIRECTION ( 'NONE',  ( 0.007781995580012663651, -3.146120232559066537E-19, -0.9999697198139514409 ) ) ;
#2969=CARTESIAN_POINT ( 'NONE',  ( -18.86354292863559579, 0.000000000000000000, 14.21804678658176080 ) ) ;
#2970=LINE ( 'NONE', #50419, #13270 ) ;
#2971=CARTESIAN_POINT ( 'NONE',  ( -12.65552006256329776, -0.1191753592594181482, 5.560586109843058011 ) ) ;
#2972=VECTOR ( 'NONE', #20123, 999.9999999999998863 ) ;
#2973=CARTESIAN_POINT ( 'NONE',  ( -17.73140113748535285, 0.000000000000000000, 13.85752530597602039 ) ) ;
#2974=ORIENTED_EDGE ( 'NONE', *, *, #54492, .T. ) ;
#2975=AXIS2_PLACEMENT_3D ( 'NONE', #51575, #8402, #13516 ) ;
#2976=VECTOR ( 'NONE', #2912, 999.9999999999998863 ) ;
#2977=ORIENTED_EDGE ( 'NONE', *, *, #26956, .F. ) ;
#2978=CARTESIAN_POINT ( 'NONE',  ( -12.76491739461853925, 0.000000000000000000, 6.767733992039747015 ) ) ;
#2979=DIRECTION ( 'NONE',  ( 0.000000000000000000, -1.000000000000000000, 0.000000000000000000 ) ) ;
#2980=DIRECTION ( 'NONE',  ( 0.005961354470445682716, -0.6427876096865404731, -0.7660212471507180654 ) ) ;
#2981=AXIS2_PLACEMENT_3D ( 'NONE', #1584, #27709, #18911 ) ;
#2982=VECTOR ( 'NONE', #50286, 1000.000000000000227 ) ;
#2983=CARTESIAN_POINT ( 'NONE',  ( -16.33317936670417225, 0.000000000000000000, 13.31440848639340224 ) ) ;
#2984=DIRECTION ( 'NONE',  ( 0.007781995580012662783, 0.000000000000000000, -0.9999697198139514409 ) ) ;
#2985=LINE ( 'NONE', #20027, #25899 ) ;
#2986=ORIENTED_EDGE ( 'NONE', *, *, #28270, .F. ) ;
#2987=CARTESIAN_POINT ( 'NONE',  ( -17.73140113748535285, 0.000000000000000000, 13.85752530597602039 ) ) ;
#2988=ORIENTED_EDGE ( 'NONE', *, *, #29125, .F. ) ;
#2989=CARTESIAN_POINT ( 'NONE',  ( -10.00813838035478298, 0.000000000000000000, 10.77830692922518452 ) ) ;
#2990=CARTESIAN_POINT ( 'NONE',  ( -9.442067484779661513, -0.1191753592594197858, 10.59804618892231254 ) ) ;
#2991=CARTESIAN_POINT ( 'NONE',  ( -18.19747506107908563, 0.000000000000000000, 14.03856424583689311 ) ) ;
#2992=CARTESIAN_POINT ( 'NONE',  ( -16.03843301287463419, 0.000000000000000000, 9.448245625342075016 ) ) ;
#2993=VECTOR ( 'NONE', #22135, 1000.000000000000227 ) ;
#2994=CARTESIAN_POINT ( 'NONE',  ( -15.13495153988577968, 0.000000000000000000, 12.76973526769478084 ) ) ;
#2995=VECTOR ( 'NONE', #14646, 999.9999999999998863 ) ;
#2996=CARTESIAN_POINT ( 'NONE',  ( -20.17205406794205302, 1.095915999411505526, 4.482477119187890935 ) ) ;
#2997=EDGE_LOOP ( 'NONE', ( #8233, #40338, #18781, #7169 ) ) ;
#2998=ORIENTED_EDGE ( 'NONE', *, *, #49170, .T. ) ;
#2999=LINE ( 'NONE', #20331, #9449 ) ;
#3000=DIRECTION ( 'NONE',  ( -0.8531650599175529814, -0.4028455766673920135, 0.3313982828793697877 ) ) ;
#3001=PLANE ( 'NONE',  #24276 ) ;
#3002=VECTOR ( 'NONE', #42716, 1000.000000000000114 ) ;
#3003=ADVANCED_FACE ( 'NONE', ( #45654 ), #7315, .F. ) ;
#3004=PLANE ( 'NONE',  #134 ) ;
#3006=AXIS2_PLACEMENT_3D ( 'NONE', #31023, #4920, #47517 ) ;
#3007=EDGE_CURVE ( 'NONE', #29949, #485, #45375, .T. ) ;
#3008=PLANE ( 'NONE',  #46303 ) ;
#3009=ADVANCED_FACE ( 'NONE', ( #54446 ), #23796, .F. ) ;
#3010=DIRECTION ( 'NONE',  ( 0.5364919789714477361, 0.6444004775717706579, 0.5449076811759711036 ) ) ;
#3011=CARTESIAN_POINT ( 'NONE',  ( -19.95974260052372529, -4.403642575758163424, 4.493863725170102796 ) ) ;
#3012=VECTOR ( 'NONE', #48995, 1000.000000000000227 ) ;
#3013=CARTESIAN_POINT ( 'NONE',  ( -17.40439531852770827, -1.726076655135827531, 12.83624927358758150 ) ) ;
#3015=VECTOR ( 'NONE', #7754, 1000.000000000000227 ) ;
#3016=VECTOR ( 'NONE', #30105, 999.9999999999998863 ) ;
#3017=ORIENTED_EDGE ( 'NONE', *, *, #22656, .F. ) ;
#3018=VECTOR ( 'NONE', #21344, 1000.000000000000000 ) ;
#3019=EDGE_LOOP ( 'NONE', ( #37350, #37916, #12693, #18271 ) ) ;
#3020=VERTEX_POINT ( 'NONE', #32606 ) ;
#3021=AXIS2_PLACEMENT_3D ( 'NONE', #14685, #49329, #511 ) ;
#3022=VERTEX_POINT ( 'NONE', #36894 ) ;
#3023=ORIENTED_EDGE ( 'NONE', *, *, #25164, .F. ) ;
#3024=CARTESIAN_POINT ( 'NONE',  ( -12.57198921205559650, 0.000000000000000000, 7.677225556966255304 ) ) ;
#3025=CARTESIAN_POINT ( 'NONE',  ( -12.70458494993575194, -0.1191753592594197858, 11.86531876794841978 ) ) ;
#3026=CARTESIAN_POINT ( 'NONE',  ( -9.308034720146865837, 0.000000000000000000, 6.225298126311265889 ) ) ;
#3027=ORIENTED_EDGE ( 'NONE', *, *, #20319, .T. ) ;
#3028=ORIENTED_EDGE ( 'NONE', *, *, #21970, .T. ) ;
#3030=PLANE ( 'NONE',  #30447 ) ;
#3031=ORIENTED_EDGE ( 'NONE', *, *, #36729, .T. ) ;
#3032=EDGE_CURVE ( 'NONE', #9919, #40769, #54197, .T. ) ;
#3034=AXIS2_PLACEMENT_3D ( 'NONE', #9972, #36111, #27280 ) ;
#3036=EDGE_CURVE ( 'NONE', #46187, #16497, #51341, .T. ) ;
#3037=LINE ( 'NONE', #46473, #16500 ) ;
#3038=CARTESIAN_POINT ( 'NONE',  ( -12.66937793510369836, -0.1117717739993998177, 8.139590219543800131 ) ) ;
#3039=EDGE_CURVE ( 'NONE', #547, #45990, #8174, .T. ) ;
#3040=EDGE_LOOP ( 'NONE', ( #25753, #41866, #19410, #8096 ) ) ;
#3041=CARTESIAN_POINT ( 'NONE',  ( -17.24885704207722270, -1.165603555308156736, 5.294927591850882465 ) ) ;
#3042=VECTOR ( 'NONE', #26070, 999.9999999999998863 ) ;
#3043=EDGE_LOOP ( 'NONE', ( #5014, #21818, #42478, #22197 ) ) ;
#3044=CARTESIAN_POINT ( 'NONE',  ( -17.38673753587113424, 0.000000000000000000, 3.577103304334748213 ) ) ;
#3045=ADVANCED_FACE ( 'NONE', ( #29175 ), #55578, .F. ) ;
#3046=CARTESIAN_POINT ( 'NONE',  ( -16.89925026227929195, -0.1191753592594197858, 13.49466922669627422 ) ) ;
#3047=VECTOR ( 'NONE', #25229, 1000.000000000000227 ) ;
#3048=CARTESIAN_POINT ( 'NONE',  ( -12.83283603900386538, 0.1245042932765033361, 2.070363196038105702 ) ) ;
#3049=CARTESIAN_POINT ( 'NONE',  ( -11.87243407472968926, 0.000000000000000000, 11.50246268866867361 ) ) ;
#3051=LINE ( 'NONE', #46487, #53022 ) ;
#3053=AXIS2_PLACEMENT_3D ( 'NONE', #49954, #2548, #49129 ) ;
#3054=DIRECTION ( 'NONE',  ( 0.9999697198139515519, 0.000000000000000000, 0.007781995580013368816 ) ) ;
#3055=ORIENTED_EDGE ( 'NONE', *, *, #35926, .F. ) ;
#3056=FACE_OUTER_BOUND ( 'NONE', #42855, .T. ) ;
#3058=AXIS2_PLACEMENT_3D ( 'NONE', #13884, #18146, #35469 ) ;
#3059=LINE ( 'NONE', #10499, #1121 ) ;
#3060=CARTESIAN_POINT ( 'NONE',  ( -22.40634380310664397, 0.000000000000000000, 5.584705972946605534 ) ) ;
#3061=LINE ( 'NONE', #20941, #16905 ) ;
#3062=LINE ( 'NONE', #3634, #51225 ) ;
#3063=DIRECTION ( 'NONE',  ( 0.007781995580012663651, -3.146120232559066537E-19, -0.9999697198139514409 ) ) ;
#3064=AXIS2_PLACEMENT_3D ( 'NONE', #35299, #43277, #22232 ) ;
#3065=DIRECTION ( 'NONE',  ( -0.5364919789714478471, 0.6444004775717705469, -0.5449076811759709926 ) ) ;
#3066=VECTOR ( 'NONE', #50377, 1000.000000000000227 ) ;
#3068=EDGE_LOOP ( 'NONE', ( #47046, #46184, #18788, #22466 ) ) ;
#3069=FACE_OUTER_BOUND ( 'NONE', #44691, .T. ) ;
#3070=DIRECTION ( 'NONE',  ( 0.5449076811759707706, 0.6444004775717708799, -0.5364919789714476250 ) ) ;
#3071=DIRECTION ( 'NONE',  ( 0.007781995580012662783, 0.000000000000000000, -0.9999697198139514409 ) ) ;
#3072=EDGE_CURVE ( 'NONE', #14373, #36044, #12141, .T. ) ;
#3073=LINE ( 'NONE', #55599, #38188 ) ;
#3074=DIRECTION ( 'NONE',  ( 0.000000000000000000, -1.000000000000000000, 0.000000000000000000 ) ) ;
#3075=DIRECTION ( 'NONE',  ( -0.5449076811759708816, 0.6444004775717707689, 0.5364919789714475140 ) ) ;
#3076=FACE_OUTER_BOUND ( 'NONE', #6412, .T. ) ;
#3077=CARTESIAN_POINT ( 'NONE',  ( -27.99767448711536133, 0.000000000000000000, 7.557179307314289218 ) ) ;
#3078=EDGE_CURVE ( 'NONE', #55515, #38688, #12994, .T. ) ;
#3079=DIRECTION ( 'NONE',  ( 0.5364919789714477361, 0.6444004775717706579, 0.5449076811759711036 ) ) ;
#3080=ADVANCED_FACE ( 'NONE', ( #17240 ), #56156, .F. ) ;
#3081=EDGE_LOOP ( 'NONE', ( #39139, #29071, #8654, #36254 ) ) ;
#3082=VECTOR ( 'NONE', #11779, 1000.000000000000114 ) ;
#3083=CARTESIAN_POINT ( 'NONE',  ( -17.26532721389163072, 0.000000000000000000, 13.67648636611514590 ) ) ;
#3084=PLANE ( 'NONE',  #20541 ) ;
#3085=VERTEX_POINT ( 'NONE', #42791 ) ;
#3086=AXIS2_PLACEMENT_3D ( 'NONE', #4649, #12620, #3798 ) ;
#3087=CARTESIAN_POINT ( 'NONE',  ( -14.00280974873554030, 0.000000000000000000, 12.40921378708904044 ) ) ;
#3088=DIRECTION ( 'NONE',  ( 0.5449076811759707706, 0.6444004775717708799, -0.5364919789714476250 ) ) ;
#3089=VECTOR ( 'NONE', #48108, 1000.000000000000114 ) ;
#3090=EDGE_LOOP ( 'NONE', ( #5536, #2164, #53372, #44752, #49270 ) ) ;
#3091=VECTOR ( 'NONE', #39681, 1000.000000000000000 ) ;
#3092=ORIENTED_EDGE ( 'NONE', *, *, #22942, .F. ) ;
#3093=DIRECTION ( 'NONE',  ( 0.5364919789714477361, 0.6444004775717706579, 0.5449076811759711036 ) ) ;
#3094=ADVANCED_FACE ( 'NONE', ( #37722 ), #33715, .F. ) ;
#3095=ORIENTED_EDGE ( 'NONE', *, *, #13668, .T. ) ;
#3096=ORIENTED_EDGE ( 'NONE', *, *, #20339, .T. ) ;
#3097=ORIENTED_EDGE ( 'NONE', *, *, #53075, .T. ) ;
#3098=DIRECTION ( 'NONE',  ( 0.000000000000000000, -1.000000000000000000, 0.000000000000000000 ) ) ;
#3099=VECTOR ( 'NONE', #43967, 999.9999999999998863 ) ;
#3100=LINE ( 'NONE', #29810, #46864 ) ;
#3101=DIRECTION ( 'NONE',  ( 0.9999697198139515519, 0.000000000000000000, 0.007781995580013368816 ) ) ;
#3102=VECTOR ( 'NONE', #38409, 1000.000000000000227 ) ;
#3103=ORIENTED_EDGE ( 'NONE', *, *, #38974, .T. ) ;
#3104=ORIENTED_EDGE ( 'NONE', *, *, #20854, .F. ) ;
#3105=AXIS2_PLACEMENT_3D ( 'NONE', #32314, #36282, #32013 ) ;
#3106=AXIS2_PLACEMENT_3D ( 'NONE', #19590, #15577, #54222 ) ;
#3107=LINE ( 'NONE', #16180, #1228 ) ;
#3108=DIRECTION ( 'NONE',  ( -0.9999697198139514409, -0.000000000000000000, -0.007781995580013368816 ) ) ;
#3109=ORIENTED_EDGE ( 'NONE', *, *, #43723, .F. ) ;
#3110=LINE ( 'NONE', #15343, #18247 ) ;
#3111=ORIENTED_EDGE ( 'NONE', *, *, #14473, .F. ) ;
#3112=LINE ( 'NONE', #20991, #23085 ) ;
#3113=LINE ( 'NONE', #29234, #50267 ) ;
#3114=ORIENTED_EDGE ( 'NONE', *, *, #51577, .T. ) ;
#3116=EDGE_CURVE ( 'NONE', #39305, #54919, #7913, .T. ) ;
#3117=VECTOR ( 'NONE', #13013, 1000.000000000000000 ) ;
#3118=LINE ( 'NONE', #55103, #11872 ) ;
#3119=ORIENTED_EDGE ( 'NONE', *, *, #2464, .F. ) ;
#3120=CARTESIAN_POINT ( 'NONE',  ( -20.26176469941677993, 0.000000000000000000, 14.76116360616437895 ) ) ;
#3121=CARTESIAN_POINT ( 'NONE',  ( -15.98897725045028650, -1.327505506330656893, 5.071256179035622758 ) ) ;
#3122=VECTOR ( 'NONE', #46264, 1000.000000000000227 ) ;
#3123=DIRECTION ( 'NONE',  ( -0.5364919789714478471, 0.6444004775717705469, -0.5449076811759709926 ) ) ;
#3124=ORIENTED_EDGE ( 'NONE', *, *, #25835, .F. ) ;
#3125=VECTOR ( 'NONE', #18742, 999.9999999999998863 ) ;
#3126=ADVANCED_FACE ( 'NONE', ( #38845 ), #12712, .F. ) ;
#3127=FACE_OUTER_BOUND ( 'NONE', #39854, .T. ) ;
#3128=CARTESIAN_POINT ( 'NONE',  ( -28.92982233430281980, 0.000000000000000000, 7.919257187036034651 ) ) ;
#3129=CARTESIAN_POINT ( 'NONE',  ( -15.13495153988577968, 0.000000000000000000, 12.76973526769478084 ) ) ;
#3130=DIRECTION ( 'NONE',  ( 0.7660212471507180654, -0.6427876096865404731, 0.005961354470445141482 ) ) ;
#3131=EDGE_CURVE ( 'NONE', #28798, #27319, #46486, .T. ) ;
#3132=CARTESIAN_POINT ( 'NONE',  ( -20.54049170961573267, 0.000000000000000000, 4.660556269540326646 ) ) ;
#3133=CARTESIAN_POINT ( 'NONE',  ( -15.87975247367846166, 0.000000000000000000, 2.850166870931599927 ) ) ;
#3134=EDGE_CURVE ( 'NONE', #24424, #39217, #55884, .T. ) ;
#3136=VECTOR ( 'NONE', #37095, 1000.000000000000227 ) ;
#3137=ORIENTED_EDGE ( 'NONE', *, *, #32947, .F. ) ;
#3138=DIRECTION ( 'NONE',  ( 0.007781995580012663651, 0.000000000000000000, -0.9999697198139515519 ) ) ;
#3139=DIRECTION ( 'NONE',  ( -0.7660212471507179544, -0.6427876096865405842, -0.005961354470445141482 ) ) ;
#3140=CARTESIAN_POINT ( 'NONE',  ( -17.93139508144814442, 0.000000000000000000, 13.85596890686001537 ) ) ;
#3141=EDGE_LOOP ( 'NONE', ( #28178, #47376, #2053, #11930 ) ) ;
#3142=VECTOR ( 'NONE', #44207, 1000.000000000000000 ) ;
#3143=DIRECTION ( 'NONE',  ( 0.9999697198139515519, 0.000000000000000000, 0.007781995580013368816 ) ) ;
#3144=EDGE_CURVE ( 'NONE', #5924, #13188, #16987, .T. ) ;
#3145=LINE ( 'NONE', #50840, #34510 ) ;
#3146=AXIS2_PLACEMENT_3D ( 'NONE', #45199, #6300, #44919 ) ;
#3148=DIRECTION ( 'NONE',  ( -0.7660212471507179544, -0.6427876096865405842, -0.005961354470445141482 ) ) ;
#3149=DIRECTION ( 'NONE',  ( -0.005961354470445682716, -0.6427876096865404731, 0.7660212471507180654 ) ) ;
#3150=EDGE_CURVE ( 'NONE', #5616, #32386, #20381, .T. ) ;
#3151=PLANE ( 'NONE',  #12051 ) ;
#3152=ORIENTED_EDGE ( 'NONE', *, *, #56206, .T. ) ;
#3153=VECTOR ( 'NONE', #27066, 1000.000000000000000 ) ;
#3154=VECTOR ( 'NONE', #26834, 1000.000000000000000 ) ;
#3155=ORIENTED_EDGE ( 'NONE', *, *, #46332, .F. ) ;
#3157=DIRECTION ( 'NONE',  ( -0.005961354470445682716, -0.6427876096865404731, 0.7660212471507180654 ) ) ;
#3159=EDGE_CURVE ( 'NONE', #52910, #43897, #16135, .T. ) ;
#3160=EDGE_LOOP ( 'NONE', ( #36097, #10100, #38673, #5435 ) ) ;
#3161=CARTESIAN_POINT ( 'NONE',  ( -15.96710241509184058, -0.1191753592594218814, 13.13259134697452879 ) ) ;
#3162=ORIENTED_EDGE ( 'NONE', *, *, #44223, .F. ) ;
#3163=FACE_OUTER_BOUND ( 'NONE', #1568, .T. ) ;
#3164=AXIS2_PLACEMENT_3D ( 'NONE', #43944, #53034, #34881 ) ;
#3166=VERTEX_POINT ( 'NONE', #55296 ) ;
#3167=VERTEX_POINT ( 'NONE', #770 ) ;
#3168=VERTEX_POINT ( 'NONE', #43384 ) ;
#3169=VECTOR ( 'NONE', #18339, 999.9999999999998863 ) ;
#3170=DIRECTION ( 'NONE',  ( 0.007781995580012663651, 0.000000000000000000, -0.9999697198139515519 ) ) ;
#3171=DIRECTION ( 'NONE',  ( 0.007781995580012663651, -3.146120232559066537E-19, -0.9999697198139514409 ) ) ;
#3172=VECTOR ( 'NONE', #33044, 1000.000000000000227 ) ;
#3173=DIRECTION ( 'NONE',  ( 0.007781995580012663651, -3.146120232559066537E-19, -0.9999697198139514409 ) ) ;
#3174=LINE ( 'NONE', #49769, #14771 ) ;
#3175=VECTOR ( 'NONE', #55438, 999.9999999999998863 ) ;
#3176=ORIENTED_EDGE ( 'NONE', *, *, #1230, .T. ) ;
#3177=EDGE_LOOP ( 'NONE', ( #23035, #7420, #52955, #11886, #36290 ) ) ;
#3178=VERTEX_POINT ( 'NONE', #9591 ) ;
#3179=VECTOR ( 'NONE', #19684, 999.9999999999998863 ) ;
#3180=CARTESIAN_POINT ( 'NONE',  ( -20.54049170961573267, 0.000000000000000000, 4.660556269540326646 ) ) ;
#3181=VECTOR ( 'NONE', #26205, 1000.000000000000227 ) ;
#3182=FACE_OUTER_BOUND ( 'NONE', #22117, .T. ) ;
#3183=ORIENTED_EDGE ( 'NONE', *, *, #52450, .T. ) ;
#3184=VECTOR ( 'NONE', #23070, 1000.000000000000000 ) ;
#3185=CARTESIAN_POINT ( 'NONE',  ( -19.60834386242827776, 0.000000000000000000, 4.298478389818581213 ) ) ;
#3186=VERTEX_POINT ( 'NONE', #36008 ) ;
#3187=CARTESIAN_POINT ( 'NONE',  ( -19.27689971179358253, 0.000000000000000000, 7.625046393098118713 ) ) ;
#3188=DIRECTION ( 'NONE',  ( 0.9999697198139515519, 0.000000000000000000, 0.007781995580013368816 ) ) ;
#3189=AXIS2_PLACEMENT_3D ( 'NONE', #52789, #31223, #31529 ) ;
#3190=EDGE_LOOP ( 'NONE', ( #23473, #4661, #4874, #25203 ) ) ;
#3191=DIRECTION ( 'NONE',  ( 0.7660212471507180654, -0.6427876096865404731, 0.005961354470445141482 ) ) ;
#3192=EDGE_CURVE ( 'NONE', #54019, #5570, #53317, .T. ) ;
#3193=VERTEX_POINT ( 'NONE', #31457 ) ;
#3194=VECTOR ( 'NONE', #41765, 999.9999999999998863 ) ;
#3195=FACE_OUTER_BOUND ( 'NONE', #20613, .T. ) ;
#3196=VECTOR ( 'NONE', #12858, 1000.000000000000227 ) ;
#3197=FACE_OUTER_BOUND ( 'NONE', #32327, .T. ) ;
#3198=CARTESIAN_POINT ( 'NONE',  ( -11.80402901237825652, 0.000000000000000000, 2.712559079740358481 ) ) ;
#3199=CARTESIAN_POINT ( 'NONE',  ( -15.13495153988577968, 0.000000000000000000, 12.76973526769478084 ) ) ;
#3200=FACE_OUTER_BOUND ( 'NONE', #36237, .T. ) ;
#3201=DIRECTION ( 'NONE',  ( -0.6427681459581293666, -0.7660444431189770143, -0.005002170337467561935 ) ) ;
#3202=VERTEX_POINT ( 'NONE', #48771 ) ;
#3203=EDGE_CURVE ( 'NONE', #52569, #44385, #40231, .T. ) ;
#3204=EDGE_CURVE ( 'NONE', #39994, #11098, #1319, .T. ) ;
#3205=ORIENTED_EDGE ( 'NONE', *, *, #34669, .T. ) ;
#3206=PLANE ( 'NONE',  #8309 ) ;
#3207=CARTESIAN_POINT ( 'NONE',  ( -12.32763377081944789, 1.743523803501506375, 1.414775798601282331 ) ) ;
#3208=LINE ( 'NONE', #15695, #30442 ) ;
#3209=DIRECTION ( 'NONE',  ( 0.9999697198139515519, 0.000000000000000000, 0.007781995580013368816 ) ) ;
#3210=LINE ( 'NONE', #46947, #14326 ) ;
#3211=ADVANCED_FACE ( 'NONE', ( #49026 ), #9870, .F. ) ;
#3212=VECTOR ( 'NONE', #48720, 1000.000000000000227 ) ;
#3213=FACE_OUTER_BOUND ( 'NONE', #44582, .T. ) ;
#3214=ORIENTED_EDGE ( 'NONE', *, *, #24753, .T. ) ;
#3215=AXIS2_PLACEMENT_3D ( 'NONE', #595, #13635, #39779 ) ;
#3216=DIRECTION ( 'NONE',  ( 0.007781995580012663651, -3.146120232559066537E-19, -0.9999697198139514409 ) ) ;
#3217=CARTESIAN_POINT ( 'NONE',  ( 2.072287782118878319, 0.000000000000000000, -2.950529333540147015 ) ) ;
#3218=EDGE_LOOP ( 'NONE', ( #44652, #1493, #28736, #47844 ) ) ;
#3219=CARTESIAN_POINT ( 'NONE',  ( -21.92051860787708506, 5.305366725996512045, 14.10300561120236829 ) ) ;
#3220=VECTOR ( 'NONE', #52177, 1000.000000000000227 ) ;
#3221=EDGE_LOOP ( 'NONE', ( #24910, #12552, #9508, #26640 ) ) ;
#3222=PLANE ( 'NONE',  #31625 ) ;
#3223=CARTESIAN_POINT ( 'NONE',  ( -24.26908309836554878, 0.000000000000000000, 6.108867788427308376 ) ) ;
#3225=VECTOR ( 'NONE', #30101, 999.9999999999998863 ) ;
#3226=CARTESIAN_POINT ( 'NONE',  ( -19.59569683186026268, 0.000000000000000000, 14.58168106541950948 ) ) ;
#3227=LINE ( 'NONE', #37042, #11485 ) ;
#3228=EDGE_CURVE ( 'NONE', #33629, #48984, #22375, .T. ) ;
#3230=VERTEX_POINT ( 'NONE', #52714 ) ;
#3231=VECTOR ( 'NONE', #27577, 1000.000000000000227 ) ;
#3232=VECTOR ( 'NONE', #6092, 999.9999999999998863 ) ;
#3233=ORIENTED_EDGE ( 'NONE', *, *, #22010, .F. ) ;
#3235=FACE_OUTER_BOUND ( 'NONE', #53824, .T. ) ;
#3236=FACE_OUTER_BOUND ( 'NONE', #25218, .T. ) ;
#3237=AXIS2_PLACEMENT_3D ( 'NONE', #27969, #23963, #15190 ) ;
#3238=CARTESIAN_POINT ( 'NONE',  ( -17.74404816805336793, 0.000000000000000000, 3.574322630375089460 ) ) ;
#3239=ADVANCED_FACE ( 'NONE', ( #31723 ), #44479, .F. ) ;
#3240=AXIS2_PLACEMENT_3D ( 'NONE', #51092, #25274, #47395 ) ;
#3241=DIRECTION ( 'NONE',  ( 0.000000000000000000, -1.000000000000000000, 0.000000000000000000 ) ) ;
#3242=CARTESIAN_POINT ( 'NONE',  ( -24.27063949748155380, 0.000000000000000000, 6.308861732390097288 ) ) ;
#3243=VECTOR ( 'NONE', #8785, 1000.000000000000227 ) ;
#3244=ORIENTED_EDGE ( 'NONE', *, *, #54262, .F. ) ;
#3245=LINE ( 'NONE', #33904, #42826 ) ;
#3246=AXIS2_PLACEMENT_3D ( 'NONE', #12349, #21117, #50672 ) ;
#3247=CARTESIAN_POINT ( 'NONE',  ( -12.15193928448664629, -0.1191753592594197858, 1.501852324026012209 ) ) ;
#3248=VECTOR ( 'NONE', #32969, 999.9999999999998863 ) ;
#3249=LINE ( 'NONE', #55470, #45951 ) ;
#3250=EDGE_LOOP ( 'NONE', ( #6976, #32229, #2742, #44453 ) ) ;
#3251=PLANE ( 'NONE',  #10255 ) ;
#3252=LINE ( 'NONE', #42695, #44967 ) ;
#3254=VERTEX_POINT ( 'NONE', #9020 ) ;
#3255=DIRECTION ( 'NONE',  ( 0.007781995580012663651, 0.000000000000000000, -0.9999697198139515519 ) ) ;
#3256=ORIENTED_EDGE ( 'NONE', *, *, #41988, .F. ) ;
#3257=AXIS2_PLACEMENT_3D ( 'NONE', #65, #56049, #26482 ) ;
#3258=ORIENTED_EDGE ( 'NONE', *, *, #48896, .F. ) ;
#3259=ORIENTED_EDGE ( 'NONE', *, *, #22885, .F. ) ;
#3260=EDGE_LOOP ( 'NONE', ( #43362, #36796, #10568, #21821 ) ) ;
#3261=DIRECTION ( 'NONE',  ( 0.5449076811759707706, 0.6444004775717708799, -0.5364919789714476250 ) ) ;
#3262=AXIS2_PLACEMENT_3D ( 'NONE', #3217, #29053, #8313 ) ;
#3263=ORIENTED_EDGE ( 'NONE', *, *, #15711, .F. ) ;
#3264=EDGE_CURVE ( 'NONE', #42364, #52074, #22911, .T. ) ;
#3265=ORIENTED_EDGE ( 'NONE', *, *, #16683, .T. ) ;
#3266=CARTESIAN_POINT ( 'NONE',  ( -15.87975247367846166, 0.000000000000000000, 2.850166870931599927 ) ) ;
#3267=ORIENTED_EDGE ( 'NONE', *, *, #47021, .F. ) ;
#3268=VECTOR ( 'NONE', #33871, 1000.000000000000227 ) ;
#3269=EDGE_CURVE ( 'NONE', #6150, #1131, #31147, .T. ) ;
#3270=ORIENTED_EDGE ( 'NONE', *, *, #27910, .T. ) ;
#3271=VECTOR ( 'NONE', #11860, 1000.000000000000227 ) ;
#3272=VECTOR ( 'NONE', #12374, 1000.000000000000227 ) ;
#3273=DIRECTION ( 'NONE',  ( 0.000000000000000000, -0.000000000000000000, -1.000000000000000000 ) ) ;
#3274=LINE ( 'NONE', #41869, #26685 ) ;
#3277=CARTESIAN_POINT ( 'NONE',  ( -12.66060981992452028, -3.432230869623160263, 7.232618128541711933 ) ) ;
#3279=ORIENTED_EDGE ( 'NONE', *, *, #10440, .F. ) ;
#3280=EDGE_CURVE ( 'NONE', #20837, #35428, #4748, .T. ) ;
#3281=VECTOR ( 'NONE', #53110, 999.9999999999998863 ) ;
#3282=EDGE_CURVE ( 'NONE', #55101, #50478, #35161, .T. ) ;
#3283=EDGE_CURVE ( 'NONE', #23095, #33080, #52458, .T. ) ;
#3284=ORIENTED_EDGE ( 'NONE', *, *, #29779, .T. ) ;
#3285=AXIS2_PLACEMENT_3D ( 'NONE', #54437, #15535, #25215 ) ;
#3286=CARTESIAN_POINT ( 'NONE',  ( -24.27063949748155380, 0.000000000000000000, 6.308861732390097288 ) ) ;
#3287=CARTESIAN_POINT ( 'NONE',  ( -10.89774764673834895, 0.000000000000000000, 5.674268529338492684 ) ) ;
#3288=EDGE_CURVE ( 'NONE', #51394, #40825, #9283, .T. ) ;
#3289=VECTOR ( 'NONE', #3171, 1000.000000000000227 ) ;
#3290=CARTESIAN_POINT ( 'NONE',  ( 2.072287782118878319, 0.000000000000000000, -2.950529333540147015 ) ) ;
#3291=VECTOR ( 'NONE', #16278, 999.9999999999998863 ) ;
#3292=DIRECTION ( 'NONE',  ( 0.005961354470445682716, -0.6427876096865404731, -0.7660212471507180654 ) ) ;
#3293=CARTESIAN_POINT ( 'NONE',  ( -12.71762380888595700, -5.213152330870666873, 1.654951243671639372 ) ) ;
#3294=DIRECTION ( 'NONE',  ( 0.005002170337468016433, -0.7660444431189770143, -0.6427681459581293666 ) ) ;
#3296=DIRECTION ( 'NONE',  ( 0.7660212471507180654, -0.6427876096865404731, 0.005961354470445141482 ) ) ;
#3297=FACE_OUTER_BOUND ( 'NONE', #42415, .T. ) ;
#3298=ORIENTED_EDGE ( 'NONE', *, *, #15621, .T. ) ;
#3299=DIRECTION ( 'NONE',  ( 0.000000000000000000, -0.000000000000000000, -1.000000000000000000 ) ) ;
#3300=DIRECTION ( 'NONE',  ( -0.6427681459581293666, -0.7660444431189770143, -0.005002170337467561935 ) ) ;
#3301=DIRECTION ( 'NONE',  ( 0.2426528472758542054, 0.7422098413412800966, 0.6246952433987894571 ) ) ;
#3302=EDGE_CURVE ( 'NONE', #33305, #52665, #43923, .T. ) ;
#3303=DIRECTION ( 'NONE',  ( -0.005961354470445682716, -0.6427876096865404731, 0.7660212471507180654 ) ) ;
#3304=CARTESIAN_POINT ( 'NONE',  ( -27.06630483948590893, -0.1191753592594197858, 7.295098399573937797 ) ) ;
#3305=AXIS2_PLACEMENT_3D ( 'NONE', #10676, #41318, #14371 ) ;
#3306=EDGE_CURVE ( 'NONE', #36173, #14307, #35413, .T. ) ;
#3307=ORIENTED_EDGE ( 'NONE', *, *, #34691, .F. ) ;
#3308=VERTEX_POINT ( 'NONE', #32811 ) ;
#3309=EDGE_CURVE ( 'NONE', #4402, #17065, #10425, .T. ) ;
#3310=LINE ( 'NONE', #56111, #16705 ) ;
#3311=CARTESIAN_POINT ( 'NONE',  ( -19.03013902487656495, 0.2864062442990046309, 4.743314820996812564 ) ) ;
#3312=LINE ( 'NONE', #37109, #33320 ) ;
#3313=VECTOR ( 'NONE', #5201, 999.9999999999998863 ) ;
#3314=EDGE_CURVE ( 'NONE', #18318, #35555, #54665, .T. ) ;
#3315=DIRECTION ( 'NONE',  ( 0.005961354470445682716, -0.6427876096865404731, -0.7660212471507180654 ) ) ;
#3316=VECTOR ( 'NONE', #3388, 1000.000000000000227 ) ;
#3317=DIRECTION ( 'NONE',  ( 0.005002170337468016433, -0.7660444431189770143, -0.6427681459581293666 ) ) ;
#3319=LINE ( 'NONE', #20643, #46461 ) ;
#3320=EDGE_CURVE ( 'NONE', #3819, #39923, #41619, .T. ) ;
#3321=CARTESIAN_POINT ( 'NONE',  ( -10.44173291041310847, 0.000000000000000000, 6.785813550879795208 ) ) ;
#3322=VECTOR ( 'NONE', #6718, 1000.000000000000227 ) ;
#3324=CARTESIAN_POINT ( 'NONE',  ( -21.47341775636118655, -0.1191753592594197858, 5.122631121243466090 ) ) ;
#3325=ORIENTED_EDGE ( 'NONE', *, *, #9204, .T. ) ;
#3326=CARTESIAN_POINT ( 'NONE',  ( -14.17742873937475423, 4.495856970884013037, 2.045485145604081012 ) ) ;
#3327=ORIENTED_EDGE ( 'NONE', *, *, #36979, .T. ) ;
#3328=VECTOR ( 'NONE', #20303, 1000.000000000000000 ) ;
#3329=VECTOR ( 'NONE', #39144, 1000.000000000000000 ) ;
#3330=ORIENTED_EDGE ( 'NONE', *, *, #8084, .F. ) ;
#3331=VECTOR ( 'NONE', #37226, 1000.000000000000227 ) ;
#3332=EDGE_LOOP ( 'NONE', ( #33829, #36635, #20089, #6403 ) ) ;
#3333=ORIENTED_EDGE ( 'NONE', *, *, #7758, .T. ) ;
#3334=ORIENTED_EDGE ( 'NONE', *, *, #28833, .T. ) ;
#3335=PLANE ( 'NONE',  #53205 ) ;
#3336=LINE ( 'NONE', #46458, #12081 ) ;
#3338=ORIENTED_EDGE ( 'NONE', *, *, #31775, .T. ) ;
#3339=CARTESIAN_POINT ( 'NONE',  ( 2.072287782118878319, 0.000000000000000000, -2.950529333540147015 ) ) ;
#3340=VERTEX_POINT ( 'NONE', #14666 ) ;
#3341=DIRECTION ( 'NONE',  ( 0.000000000000000000, -0.000000000000000000, -1.000000000000000000 ) ) ;
#3342=ORIENTED_EDGE ( 'NONE', *, *, #41815, .F. ) ;
#3343=VECTOR ( 'NONE', #17600, 999.9999999999998863 ) ;
#3345=DIRECTION ( 'NONE',  ( 0.005002170337468016433, -0.7660444431189770143, -0.6427681459581293666 ) ) ;
#3347=ORIENTED_EDGE ( 'NONE', *, *, #48896, .T. ) ;
#3348=FACE_OUTER_BOUND ( 'NONE', #55072, .T. ) ;
#3350=ORIENTED_EDGE ( 'NONE', *, *, #1814, .F. ) ;
#3351=ADVANCED_FACE ( 'NONE', ( #40798 ), #1869, .F. ) ;
#3352=ADVANCED_FACE ( 'NONE', ( #10958 ), #31991, .F. ) ;
#3354=CARTESIAN_POINT ( 'NONE',  ( -17.99722147484924051, 0.000000000000000000, 3.772358433381585385 ) ) ;
#3355=VECTOR ( 'NONE', #10923, 999.9999999999998863 ) ;
#3356=DIRECTION ( 'NONE',  ( 0.7660212471507180654, -0.6427876096865404731, 0.005961354470445141482 ) ) ;
#3357=EDGE_CURVE ( 'NONE', #50871, #10700, #50130, .T. ) ;
#3358=LINE ( 'NONE', #24627, #10647 ) ;
#3359=VECTOR ( 'NONE', #47213, 1000.000000000000227 ) ;
#3360=CARTESIAN_POINT ( 'NONE',  ( -16.33317936670417225, 0.000000000000000000, 13.31440848639340224 ) ) ;
#3362=CARTESIAN_POINT ( 'NONE',  ( -14.03793453906542688, -0.1191753592594188005, 4.072499561507972210 ) ) ;
#3364=PLANE ( 'NONE',  #24748 ) ;
#3366=CARTESIAN_POINT ( 'NONE',  ( -13.73672976910459909, 0.000000000000000000, 12.22661844811216270 ) ) ;
#3367=ORIENTED_EDGE ( 'NONE', *, *, #9914, .F. ) ;
#3368=AXIS2_PLACEMENT_3D ( 'NONE', #36891, #41125, #54730 ) ;
#3369=DIRECTION ( 'NONE',  ( 0.000000000000000000, -1.000000000000000000, 0.000000000000000000 ) ) ;
#3370=CARTESIAN_POINT ( 'NONE',  ( -17.88454542038633122, 0.000000000000000000, 7.835888072364936008 ) ) ;
#3371=CARTESIAN_POINT ( 'NONE',  ( -19.59569683186026268, 0.000000000000000000, 14.58168106541950948 ) ) ;
#3372=FACE_OUTER_BOUND ( 'NONE', #26240, .T. ) ;
#3373=LINE ( 'NONE', #17542, #6853 ) ;
#3374=AXIS2_PLACEMENT_3D ( 'NONE', #20265, #51217, #6961 ) ;
#3376=ORIENTED_EDGE ( 'NONE', *, *, #44258, .T. ) ;
#3377=FACE_OUTER_BOUND ( 'NONE', #36993, .T. ) ;
#3378=CARTESIAN_POINT ( 'NONE',  ( -9.075990533167328067, 0.000000000000000000, 10.41622904950343909 ) ) ;
#3379=CARTESIAN_POINT ( 'NONE',  ( -15.52687229411750813, 0.000000000000000000, 3.422251192111810170 ) ) ;
#3380=CARTESIAN_POINT ( 'NONE',  ( -13.09628788616446116, -0.1134144341942139589, 1.868669391131170698 ) ) ;
#3381=CARTESIAN_POINT ( 'NONE',  ( -14.01545677930355183, 0.000000000000000000, 2.126011111488108174 ) ) ;
#3382=DIRECTION ( 'NONE',  ( 0.007781995580012663651, -3.146120232559066537E-19, -0.9999697198139514409 ) ) ;
#3383=ADVANCED_FACE ( 'NONE', ( #23480 ), #11239, .F. ) ;
#3384=LINE ( 'NONE', #34586, #54928 ) ;
#3385=DIRECTION ( 'NONE',  ( 0.000000000000000000, 1.000000000000000000, 0.000000000000000000 ) ) ;
#3386=ORIENTED_EDGE ( 'NONE', *, *, #19417, .F. ) ;
#3387=CARTESIAN_POINT ( 'NONE',  ( -10.47421230394850866, 0.000000000000000000, 10.95934586908605723 ) ) ;
#3388=DIRECTION ( 'NONE',  ( 0.007781995580012662783, 0.000000000000000000, -0.9999697198139514409 ) ) ;
#3389=ORIENTED_EDGE ( 'NONE', *, *, #27915, .F. ) ;
#3390=ADVANCED_FACE ( 'NONE', ( #28565 ), #44769, .F. ) ;
#3391=ORIENTED_EDGE ( 'NONE', *, *, #39249, .F. ) ;
#3392=LINE ( 'NONE', #37451, #42835 ) ;
#3393=EDGE_CURVE ( 'NONE', #3819, #12179, #10126, .T. ) ;
#3394=ORIENTED_EDGE ( 'NONE', *, *, #2477, .T. ) ;
#3395=EDGE_CURVE ( 'NONE', #44587, #48743, #24028, .T. ) ;
#3396=ORIENTED_EDGE ( 'NONE', *, *, #41729, .F. ) ;
#3397=DIRECTION ( 'NONE',  ( -0.5364919789714478471, 0.6444004775717705469, -0.5449076811759709926 ) ) ;
#3398=VECTOR ( 'NONE', #2716, 1000.000000000000000 ) ;
#3399=VERTEX_POINT ( 'NONE', #23210 ) ;
#3400=ORIENTED_EDGE ( 'NONE', *, *, #34127, .T. ) ;
#3401=ORIENTED_EDGE ( 'NONE', *, *, #40228, .F. ) ;
#3402=CARTESIAN_POINT ( 'NONE',  ( -25.20200914511100265, -0.1191753592594197858, 6.570942640130446932 ) ) ;
#3403=CARTESIAN_POINT ( 'NONE',  ( -28.92982233430281980, 0.000000000000000000, 7.919257187036034651 ) ) ;
#3404=DIRECTION ( 'NONE',  ( -0.005002170337468016433, -0.7660444431189770143, 0.6427681459581293666 ) ) ;
#3405=AXIS2_PLACEMENT_3D ( 'NONE', #26830, #13493, #44156 ) ;
#3406=ORIENTED_EDGE ( 'NONE', *, *, #8580, .F. ) ;
#3407=ORIENTED_EDGE ( 'NONE', *, *, #44777, .T. ) ;
#3408=DIRECTION ( 'NONE',  ( 0.9999697198139515519, 0.000000000000000000, 0.007781995580013368816 ) ) ;
#3409=DIRECTION ( 'NONE',  ( 0.5449076811759707706, 0.6444004775717708799, -0.5364919789714476250 ) ) ;
#3410=ORIENTED_EDGE ( 'NONE', *, *, #39397, .T. ) ;
#3411=CARTESIAN_POINT ( 'NONE',  ( -13.59629007026659941, -0.1191753592594190225, 7.030593099338098284 ) ) ;
#3412=ORIENTED_EDGE ( 'NONE', *, *, #28944, .F. ) ;
#3413=CARTESIAN_POINT ( 'NONE',  ( -21.55226037509761738, -4.565544526780660917, 12.54639795354807141 ) ) ;
#3414=CARTESIAN_POINT ( 'NONE',  ( -19.69569380384165669, -0.1191753592594177458, 14.58090286586150697 ) ) ;
#3415=EDGE_CURVE ( 'NONE', #17026, #4038, #28277, .T. ) ;
#3416=EDGE_LOOP ( 'NONE', ( #23314, #10175, #32909, #13734 ) ) ;
#3417=DIRECTION ( 'NONE',  ( -0.005002170337468016433, -0.7660444431189770143, 0.6427681459581293666 ) ) ;
#3418=EDGE_CURVE ( 'NONE', #29528, #18631, #15243, .T. ) ;
#3419=ADVANCED_FACE ( 'NONE', ( #45892 ), #7007, .F. ) ;
#3420=DIRECTION ( 'NONE',  ( 0.5449076811759707706, 0.6444004775717708799, -0.5364919789714476250 ) ) ;
#3421=ORIENTED_EDGE ( 'NONE', *, *, #10902, .T. ) ;
#3422=DIRECTION ( 'NONE',  ( 0.005961354470445682716, -0.6427876096865404731, -0.7660212471507180654 ) ) ;
#3423=PLANE ( 'NONE',  #39244 ) ;
#3424=CARTESIAN_POINT ( 'NONE',  ( -15.16984770538739014, 4.495856970884011261, 10.15227235917422455 ) ) ;
#3425=DIRECTION ( 'NONE',  ( 0.005002170337468016433, -0.7660444431189770143, -0.6427681459581293666 ) ) ;
#3427=CARTESIAN_POINT ( 'NONE',  ( -13.11936205432852987, -1.813211359398158029, 1.919475938924976255 ) ) ;
#3428=CARTESIAN_POINT ( 'NONE',  ( -13.02800394838083342, 0.000000000000000000, 6.565680535424952780 ) ) ;
#3429=CARTESIAN_POINT ( 'NONE',  ( -13.39181721811076997, -2.137015261443160341, 2.014975737379525178 ) ) ;
#3430=LINE ( 'NONE', #8834, #40458 ) ;
#3431=DIRECTION ( 'NONE',  ( 0.005961354470445682716, -0.6427876096865404731, -0.7660212471507180654 ) ) ;
#3432=CARTESIAN_POINT ( 'NONE',  ( -19.59569683186026268, 0.000000000000000000, 14.58168106541950948 ) ) ;
#3433=EDGE_CURVE ( 'NONE', #83, #29572, #24309, .T. ) ;
#3435=ORIENTED_EDGE ( 'NONE', *, *, #26539, .T. ) ;
#3436=FACE_OUTER_BOUND ( 'NONE', #35039, .T. ) ;
#3437=CARTESIAN_POINT ( 'NONE',  ( -16.33317936670417225, 0.000000000000000000, 13.31440848639340224 ) ) ;
#3438=ORIENTED_EDGE ( 'NONE', *, *, #9188, .T. ) ;
#3439=DIRECTION ( 'NONE',  ( 0.005961354470445682716, -0.6427876096865404731, -0.7660212471507180654 ) ) ;
#3440=CARTESIAN_POINT ( 'NONE',  ( -15.93097076849315386, -0.1191753592594191752, 8.489752353529109286 ) ) ;
#3441=VECTOR ( 'NONE', #40082, 999.9999999999998863 ) ;
#3442=DIRECTION ( 'NONE',  ( -0.5364919789714478471, 0.6444004775717705469, -0.5449076811759709926 ) ) ;
#3444=CARTESIAN_POINT ( 'NONE',  ( -24.27063949748155380, 0.000000000000000000, 6.308861732390097288 ) ) ;
#3445=ORIENTED_EDGE ( 'NONE', *, *, #11205, .T. ) ;
#3446=ORIENTED_EDGE ( 'NONE', *, *, #29401, .F. ) ;
#3447=LINE ( 'NONE', #2322, #16849 ) ;
#3448=FACE_OUTER_BOUND ( 'NONE', #11114, .T. ) ;
#3451=ORIENTED_EDGE ( 'NONE', *, *, #8832, .F. ) ;
#3453=EDGE_CURVE ( 'NONE', #55170, #5309, #45325, .T. ) ;
#3454=ORIENTED_EDGE ( 'NONE', *, *, #18798, .F. ) ;
#3455=CARTESIAN_POINT ( 'NONE',  ( 2.072287782118878319, 0.000000000000000000, -2.950529333540147015 ) ) ;
#3456=VERTEX_POINT ( 'NONE', #41062 ) ;
#3457=EDGE_LOOP ( 'NONE', ( #36767, #49794, #55702, #37261 ) ) ;
#3458=ORIENTED_EDGE ( 'NONE', *, *, #42269, .T. ) ;
#3459=LINE ( 'NONE', #2606, #40218 ) ;
#3460=CARTESIAN_POINT ( 'NONE',  ( -26.13337879274045505, 0.000000000000000000, 6.833023547870798353 ) ) ;
#3461=CARTESIAN_POINT ( 'NONE',  ( -10.37219204796779337, -9.994947293139700761, 0.8105380568915174777 ) ) ;
#3462=EDGE_CURVE ( 'NONE', #41178, #1421, #2148, .T. ) ;
#3463=LINE ( 'NONE', #20779, #50227 ) ;
#3465=EDGE_CURVE ( 'NONE', #40362, #49112, #54143, .T. ) ;
#3466=ADVANCED_FACE ( 'NONE', ( #50434 ), #16617, .F. ) ;
#3467=ORIENTED_EDGE ( 'NONE', *, *, #56052, .F. ) ;
#3468=VERTEX_POINT ( 'NONE', #20619 ) ;
#3469=FACE_OUTER_BOUND ( 'NONE', #45038, .T. ) ;
#3470=CARTESIAN_POINT ( 'NONE',  ( -16.86599266918588924, -0.1191753592594177180, 9.221139936508615520 ) ) ;
#3471=ORIENTED_EDGE ( 'NONE', *, *, #15401, .F. ) ;
#3472=LINE ( 'NONE', #38102, #42939 ) ;
#3474=ORIENTED_EDGE ( 'NONE', *, *, #47318, .T. ) ;
#3475=DIRECTION ( 'NONE',  ( 0.000000000000000000, -1.000000000000000000, 0.000000000000000000 ) ) ;
#3476=DIRECTION ( 'NONE',  ( 0.005961354470445682716, -0.6427876096865404731, -0.7660212471507180654 ) ) ;
#3477=VECTOR ( 'NONE', #12224, 999.9999999999998863 ) ;
#3478=VERTEX_POINT ( 'NONE', #43025 ) ;
#3479=EDGE_CURVE ( 'NONE', #27552, #55206, #25166, .T. ) ;
#3480=CARTESIAN_POINT ( 'NONE',  ( -21.47263955680318404, 0.000000000000000000, 5.022634149262071190 ) ) ;
#3481=VERTEX_POINT ( 'NONE', #24566 ) ;
#3482=EDGE_CURVE ( 'NONE', #29459, #34227, #11538, .T. ) ;
#3483=LINE ( 'NONE', #20795, #5612 ) ;
#3484=DIRECTION ( 'NONE',  ( -0.9999697198139514409, -0.000000000000000000, -0.007781995580013368816 ) ) ;
#3485=ORIENTED_EDGE ( 'NONE', *, *, #50766, .F. ) ;
#3486=DIRECTION ( 'NONE',  ( -0.005002170337468016433, -0.7660444431189770143, 0.6427681459581293666 ) ) ;
#3487=CARTESIAN_POINT ( 'NONE',  ( -14.97295643975815871, -0.1191753592594183703, 4.803887144487482885 ) ) ;
#3488=DIRECTION ( 'NONE',  ( -0.5364919789714478471, 0.6444004775717705469, -0.5449076811759709926 ) ) ;
#3489=ADVANCED_FACE ( 'NONE', ( #24861 ), #16326, .F. ) ;
#3490=DIRECTION ( 'NONE',  ( 0.000000000000000000, -0.000000000000000000, -1.000000000000000000 ) ) ;
#3491=EDGE_LOOP ( 'NONE', ( #24539, #39559, #35140, #18071 ) ) ;
#3492=EDGE_CURVE ( 'NONE', #29905, #3617, #47010, .T. ) ;
#3493=EDGE_LOOP ( 'NONE', ( #13375, #23166, #30243, #39850 ) ) ;
#3494=DIRECTION ( 'NONE',  ( 0.000000000000000000, -0.000000000000000000, -1.000000000000000000 ) ) ;
#3495=CARTESIAN_POINT ( 'NONE',  ( -9.943925025897915049, 0.000000000000000000, 2.527028782849607857 ) ) ;
#3496=LINE ( 'NONE', #30172, #4132 ) ;
#3497=LINE ( 'NONE', #11729, #50288 ) ;
#3498=CARTESIAN_POINT ( 'NONE',  ( -13.07066190154808361, 0.000000000000000000, 12.04713590736729678 ) ) ;
#3499=EDGE_CURVE ( 'NONE', #25139, #32467, #20869, .T. ) ;
#3500=CARTESIAN_POINT ( 'NONE',  ( -14.00280974873554030, 0.000000000000000000, 12.40921378708904044 ) ) ;
#3501=ORIENTED_EDGE ( 'NONE', *, *, #44751, .T. ) ;
#3504=CARTESIAN_POINT ( 'NONE',  ( -19.15040009907104235, -0.1191753592594162470, 4.220292173140257397 ) ) ;
#3505=VERTEX_POINT ( 'NONE', #56097 ) ;
#3506=CARTESIAN_POINT ( 'NONE',  ( -16.06709938707323460, 0.000000000000000000, 13.13181314741652628 ) ) ;
#3507=ORIENTED_EDGE ( 'NONE', *, *, #25874, .F. ) ;
#3509=DIRECTION ( 'NONE',  ( 0.9999697198139515519, 0.000000000000000000, 0.007781995580013368816 ) ) ;
#3510=CARTESIAN_POINT ( 'NONE',  ( -30.79411802867772607, 0.000000000000000000, 8.643412946479525516 ) ) ;
#3511=DIRECTION ( 'NONE',  ( -0.005002170337468016433, -0.7660444431189770143, 0.6427681459581293666 ) ) ;
#3514=ORIENTED_EDGE ( 'NONE', *, *, #26059, .F. ) ;
#3516=CARTESIAN_POINT ( 'NONE',  ( -13.27065584551087163, 0.000000000000000000, 12.04557950825129176 ) ) ;
#3517=DIRECTION ( 'NONE',  ( 0.005961354470445682716, -0.6427876096865404731, -0.7660212471507180654 ) ) ;
#3518=CARTESIAN_POINT ( 'NONE',  ( 2.072287782118878319, 0.000000000000000000, -2.950529333540147015 ) ) ;
#3519=VECTOR ( 'NONE', #51754, 1000.000000000000114 ) ;
#3520=PLANE ( 'NONE',  #16519 ) ;
#3521=DIRECTION ( 'NONE',  ( 0.000000000000000000, -0.000000000000000000, -1.000000000000000000 ) ) ;
#3522=ADVANCED_FACE ( 'NONE', ( #42728 ), #33650, .F. ) ;
#3523=ORIENTED_EDGE ( 'NONE', *, *, #7285, .T. ) ;
#3524=CARTESIAN_POINT ( 'NONE',  ( -16.49770049126292193, 0.000000000000000000, 8.754670973479470319 ) ) ;
#3525=DIRECTION ( 'NONE',  ( 0.5449076811759707706, 0.6444004775717708799, -0.5364919789714476250 ) ) ;
#3526=LINE ( 'NONE', #54622, #44137 ) ;
#3527=ORIENTED_EDGE ( 'NONE', *, *, #8696, .F. ) ;
#3530=DIRECTION ( 'NONE',  ( 0.7660212471507180654, -0.6427876096865404731, 0.005961354470445141482 ) ) ;
#3531=VERTEX_POINT ( 'NONE', #38480 ) ;
#3532=CARTESIAN_POINT ( 'NONE',  ( -19.53866861116660303, 0.000000000000000000, 7.253677177188349035 ) ) ;
#3533=ORIENTED_EDGE ( 'NONE', *, *, #246, .T. ) ;
#3534=ADVANCED_FACE ( 'NONE', ( #33395 ), #29712, .F. ) ;
#3536=ORIENTED_EDGE ( 'NONE', *, *, #11158, .F. ) ;
#3537=ORIENTED_EDGE ( 'NONE', *, *, #25672, .T. ) ;
#3538=LINE ( 'NONE', #42159, #49263 ) ;
#3539=ORIENTED_EDGE ( 'NONE', *, *, #51811, .F. ) ;
#3541=EDGE_LOOP ( 'NONE', ( #15578, #43860, #22731, #39612 ) ) ;
#3543=ADVANCED_FACE ( 'NONE', ( #47269 ), #37931, .F. ) ;
#3544=ORIENTED_EDGE ( 'NONE', *, *, #20901, .F. ) ;
#3545=ORIENTED_EDGE ( 'NONE', *, *, #18337, .T. ) ;
#3546=EDGE_CURVE ( 'NONE', #32426, #10918, #7846, .T. ) ;
#3547=CARTESIAN_POINT ( 'NONE',  ( -10.42736264288669723, 0.000000000000000000, 4.939265034590974324 ) ) ;
#3548=CARTESIAN_POINT ( 'NONE',  ( -20.97744843082703881, -1.165603555308156736, 6.743239110737863307 ) ) ;
#3549=LINE ( 'NONE', #37921, #33249 ) ;
#3550=FACE_OUTER_BOUND ( 'NONE', #51387, .T. ) ;
#3552=EDGE_LOOP ( 'NONE', ( #12740, #41321, #55076, #31005 ) ) ;
#3553=EDGE_CURVE ( 'NONE', #18849, #17489, #33945, .T. ) ;
#3554=VECTOR ( 'NONE', #6570, 1000.000000000000000 ) ;
#3555=ORIENTED_EDGE ( 'NONE', *, *, #245, .F. ) ;
#3556=DIRECTION ( 'NONE',  ( 0.9999697198139515519, 0.000000000000000000, 0.007781995580013368816 ) ) ;
#3557=DIRECTION ( 'NONE',  ( 0.005961354470445682716, -0.6427876096865404731, -0.7660212471507180654 ) ) ;
#3560=DIRECTION ( 'NONE',  ( 0.7660212471507180654, -0.6427876096865404731, 0.005961354470445141482 ) ) ;
#3561=EDGE_CURVE ( 'NONE', #29456, #7607, #8376, .T. ) ;
#3562=DIRECTION ( 'NONE',  ( 0.005002170337468016433, -0.7660444431189770143, -0.6427681459581293666 ) ) ;
#3563=LINE ( 'NONE', #3293, #12241 ) ;
#3564=CARTESIAN_POINT ( 'NONE',  ( -23.33849165029409889, 0.000000000000000000, 5.946783852668351855 ) ) ;
#3565=VERTEX_POINT ( 'NONE', #54978 ) ;
#3566=CARTESIAN_POINT ( 'NONE',  ( -14.54935328597183819, -0.1191753592594172878, 8.869836490052643185 ) ) ;
#3567=CARTESIAN_POINT ( 'NONE',  ( -16.06146926423485866, -3.594132820645661308, 8.819336114335181165 ) ) ;
#3568=ORIENTED_EDGE ( 'NONE', *, *, #40271, .T. ) ;
#3569=LINE ( 'NONE', #7855, #27979 ) ;
#3570=CARTESIAN_POINT ( 'NONE',  ( -14.61196876796175204, 0.000000000000000000, 5.276031531936651753 ) ) ;
#3571=FACE_OUTER_BOUND ( 'NONE', #44321, .T. ) ;
#3572=CARTESIAN_POINT ( 'NONE',  ( -18.76354595665420177, -0.1191753592594177458, 14.21882498613976331 ) ) ;
#3573=PLANE ( 'NONE',  #9628 ) ;
#3574=EDGE_LOOP ( 'NONE', ( #36640, #40801, #23513 ) ) ;
#3575=EDGE_LOOP ( 'NONE', ( #25272, #45240, #10854, #12770 ) ) ;
#3576=LINE ( 'NONE', #26027, #8516 ) ;
#3577=DIRECTION ( 'NONE',  ( 0.000000000000000000, -0.000000000000000000, -1.000000000000000000 ) ) ;
#3579=EDGE_CURVE ( 'NONE', #11430, #10812, #50701, .T. ) ;
#3580=CARTESIAN_POINT ( 'NONE',  ( -13.93957187223785077, 1.419719901456504285, 4.625926450176987892 ) ) ;
#3581=DIRECTION ( 'NONE',  ( 0.007781995580012663651, 0.000000000000000000, -0.9999697198139515519 ) ) ;
#3582=EDGE_CURVE ( 'NONE', #54123, #13455, #39041, .T. ) ;
#3583=CARTESIAN_POINT ( 'NONE',  ( -19.60990026154428278, 0.000000000000000000, 4.498472333781370125 ) ) ;
#3584=DIRECTION ( 'NONE',  ( -0.6427681459581293666, -0.7660444431189770143, -0.005002170337467561935 ) ) ;
#3585=CARTESIAN_POINT ( 'NONE',  ( -10.28842178966973897, 0.000000000000000000, 0.8776935365639153552 ) ) ;
#3587=EDGE_CURVE ( 'NONE', #21782, #10029, #14046, .T. ) ;
#3588=ADVANCED_FACE ( 'NONE', ( #30809 ), #52100, .F. ) ;
#3589=LINE ( 'NONE', #33682, #180 ) ;
#3591=DIRECTION ( 'NONE',  ( 0.9321478471874540261, 0.000000000000000000, -0.3620778797217457101 ) ) ;
#3592=EDGE_CURVE ( 'NONE', #44810, #31885, #47564, .T. ) ;
#3593=EDGE_CURVE ( 'NONE', #47105, #49493, #707, .T. ) ;
#3594=ADVANCED_FACE ( 'NONE', ( #35350 ), #4968, .F. ) ;
#3595=ORIENTED_EDGE ( 'NONE', *, *, #3264, .F. ) ;
#3598=ORIENTED_EDGE ( 'NONE', *, *, #11027, .T. ) ;
#3599=ORIENTED_EDGE ( 'NONE', *, *, #8048, .F. ) ;
#3600=ORIENTED_EDGE ( 'NONE', *, *, #52374, .F. ) ;
#3601=CARTESIAN_POINT ( 'NONE',  ( -27.06552663992790997, 0.000000000000000000, 7.195101427592543786 ) ) ;
#3602=PLANE ( 'NONE',  #41073 ) ;
#3604=ORIENTED_EDGE ( 'NONE', *, *, #45738, .T. ) ;
#3605=DIRECTION ( 'NONE',  ( 0.6427681459581294776, -0.7660444431189769032, 0.005002170337467562802 ) ) ;
#3606=EDGE_CURVE ( 'NONE', #21318, #55411, #52647, .T. ) ;
#3607=ORIENTED_EDGE ( 'NONE', *, *, #29372, .F. ) ;
#3608=DIRECTION ( 'NONE',  ( 0.9999697198139515519, 0.000000000000000000, 0.007781995580013368816 ) ) ;
#3609=ORIENTED_EDGE ( 'NONE', *, *, #22281, .T. ) ;
#3610=EDGE_CURVE ( 'NONE', #21327, #34381, #34498, .T. ) ;
#3611=DIRECTION ( 'NONE',  ( 0.7660212471507180654, -0.6427876096865404731, 0.005961354470445141482 ) ) ;
#3612=ADVANCED_FACE ( 'NONE', ( #13753 ), #17449, .F. ) ;
#3613=CARTESIAN_POINT ( 'NONE',  ( -13.68113857516357967, 0.000000000000000000, 5.083269411509881763 ) ) ;
#3614=FACE_OUTER_BOUND ( 'NONE', #12624, .T. ) ;
#3615=VERTEX_POINT ( 'NONE', #22571 ) ;
#3616=CARTESIAN_POINT ( 'NONE',  ( -3.335658863730355694, -6.482724466489810489, -1.922690393539094433 ) ) ;
#3617=VERTEX_POINT ( 'NONE', #34786 ) ;
#3618=EDGE_CURVE ( 'NONE', #8639, #20837, #4678, .T. ) ;
#3619=DIRECTION ( 'NONE',  ( 0.007781995580012663651, -3.146120232559066537E-19, -0.9999697198139514409 ) ) ;
#3620=CARTESIAN_POINT ( 'NONE',  ( -16.15650678959040221, 3.524445264749011208, 2.845219389405668320 ) ) ;
#3621=VECTOR ( 'NONE', #5850, 1000.000000000000000 ) ;
#3623=CARTESIAN_POINT ( 'NONE',  ( -16.49638283687364293, 0.000000000000000000, 8.585355214184495765 ) ) ;
#3624=CARTESIAN_POINT ( 'NONE',  ( -19.32961685222932147, 0.000000000000000000, 14.39908572644263351 ) ) ;
#3626=FACE_OUTER_BOUND ( 'NONE', #3696, .T. ) ;
#3628=VERTEX_POINT ( 'NONE', #31071 ) ;
#3630=EDGE_LOOP ( 'NONE', ( #44556, #45588, #23509, #56008 ) ) ;
#3631=CARTESIAN_POINT ( 'NONE',  ( -11.15478472993248715, -0.03228989815065527735, 1.213188107564080020 ) ) ;
#3632=LINE ( 'NONE', #16698, #16948 ) ;
#3633=LINE ( 'NONE', #7326, #10551 ) ;
#3634=CARTESIAN_POINT ( 'NONE',  ( -21.26187472307101345, 2.391131607591508335, 4.864476313006088404 ) ) ;
#3635=CARTESIAN_POINT ( 'NONE',  ( -11.52190826124595091, 0.7721120973665037690, 2.623989063664057042 ) ) ;
#3636=LINE ( 'NONE', #42547, #9270 ) ;
#3638=ORIENTED_EDGE ( 'NONE', *, *, #20025, .T. ) ;
#3639=DIRECTION ( 'NONE',  ( 0.000000000000000000, -0.000000000000000000, -1.000000000000000000 ) ) ;
#3640=PLANE ( 'NONE',  #53043 ) ;
#3641=DIRECTION ( 'NONE',  ( 0.5364919789714477361, 0.6444004775717706579, 0.5449076811759711036 ) ) ;
#3642=CARTESIAN_POINT ( 'NONE',  ( -13.17065887352947762, -0.1191753592594197858, 12.04635770780929427 ) ) ;
#3643=CARTESIAN_POINT ( 'NONE',  ( -14.89316374707889423, 4.172053068839010059, 9.513381545639502335 ) ) ;
#3644=DIRECTION ( 'NONE',  ( 0.007781995580012662783, 0.000000000000000000, -0.9999697198139514409 ) ) ;
#3645=CARTESIAN_POINT ( 'NONE',  ( -17.42122617793452477, 0.000000000000000000, 8.008819743427922688 ) ) ;
#3646=ORIENTED_EDGE ( 'NONE', *, *, #15003, .F. ) ;
#3647=CARTESIAN_POINT ( 'NONE',  ( -16.93647090655645826, 0.000000000000000000, 5.427267732391580779 ) ) ;
#3648=CARTESIAN_POINT ( 'NONE',  ( -14.34960227313585790, 3.038739411681509850, 2.158852872141225898 ) ) ;
#3649=VERTEX_POINT ( 'NONE', #413 ) ;
#3650=VERTEX_POINT ( 'NONE', #51810 ) ;
#3651=CARTESIAN_POINT ( 'NONE',  ( -12.20525343324862355, -0.1191753592594177180, 7.410750537899888357 ) ) ;
#3652=EDGE_CURVE ( 'NONE', #22884, #21327, #9507, .T. ) ;
#3653=EDGE_CURVE ( 'NONE', #40408, #13812, #12920, .T. ) ;
#3654=VERTEX_POINT ( 'NONE', #8684 ) ;
#3655=FACE_OUTER_BOUND ( 'NONE', #46060, .T. ) ;
#3656=EDGE_CURVE ( 'NONE', #39352, #20003, #13215, .T. ) ;
#3657=VECTOR ( 'NONE', #6871, 1000.000000000000227 ) ;
#3659=EDGE_LOOP ( 'NONE', ( #42625, #8808, #26182, #49251 ) ) ;
#3660=VERTEX_POINT ( 'NONE', #44159 ) ;
#3661=FACE_OUTER_BOUND ( 'NONE', #42039, .T. ) ;
#3663=CARTESIAN_POINT ( 'NONE',  ( -20.34698012014669999, -3.756034771668160577, 4.664942007982749494 ) ) ;
#3664=ORIENTED_EDGE ( 'NONE', *, *, #36806, .T. ) ;
#3665=VERTEX_POINT ( 'NONE', #35623 ) ;
#3666=EDGE_CURVE ( 'NONE', #49206, #6270, #35094, .T. ) ;
#3667=FACE_OUTER_BOUND ( 'NONE', #8087, .T. ) ;
#3668=CARTESIAN_POINT ( 'NONE',  ( -13.27065584551087163, 0.000000000000000000, 12.04557950825129176 ) ) ;
#3669=ORIENTED_EDGE ( 'NONE', *, *, #23512, .F. ) ;
#3670=EDGE_CURVE ( 'NONE', #15326, #187, #52940, .T. ) ;
#3671=FACE_OUTER_BOUND ( 'NONE', #40330, .T. ) ;
#3672=CARTESIAN_POINT ( 'NONE',  ( -24.26986129792355129, -0.1191753592594197858, 6.208864760408702388 ) ) ;
#3673=VERTEX_POINT ( 'NONE', #31380 ) ;
#3674=FACE_OUTER_BOUND ( 'NONE', #5919, .T. ) ;
#3676=ORIENTED_EDGE ( 'NONE', *, *, #53272, .T. ) ;
#3677=EDGE_CURVE ( 'NONE', #52348, #36108, #48701, .T. ) ;
#3678=CARTESIAN_POINT ( 'NONE',  ( -22.40478740399063895, 0.000000000000000000, 5.384712028983816623 ) ) ;
#3679=EDGE_CURVE ( 'NONE', #27005, #10812, #36748, .T. ) ;
#3680=LINE ( 'NONE', #7972, #35439 ) ;
#3681=VERTEX_POINT ( 'NONE', #18880 ) ;
#3682=DIRECTION ( 'NONE',  ( -0.9999697198139514409, -0.000000000000000000, -0.007781995580013368816 ) ) ;
#3683=CARTESIAN_POINT ( 'NONE',  ( -11.81552522639938907, 0.000000000000000000, 4.189797892771416343 ) ) ;
#3684=DIRECTION ( 'NONE',  ( 0.007781995580012663651, 0.000000000000000000, -0.9999697198139515519 ) ) ;
#3685=FACE_OUTER_BOUND ( 'NONE', #34439, .T. ) ;
#3686=EDGE_LOOP ( 'NONE', ( #27087, #1582, #10444, #55744, #6293 ) ) ;
#3687=VECTOR ( 'NONE', #38903, 999.9999999999998863 ) ;
#3688=CARTESIAN_POINT ( 'NONE',  ( -17.29990502820820453, -0.6798977022406551551, 4.517630311409670973 ) ) ;
#3689=FACE_OUTER_BOUND ( 'NONE', #39722, .T. ) ;
#3690=FACE_OUTER_BOUND ( 'NONE', #36286, .T. ) ;
#3691=DIRECTION ( 'NONE',  ( -0.5364919789714478471, 0.6444004775717705469, -0.5449076811759709926 ) ) ;
#3692=FACE_OUTER_BOUND ( 'NONE', #23485, .T. ) ;
#3693=CARTESIAN_POINT ( 'NONE',  ( -13.47484560386877028, 2.553033558614008047, 1.834564234598528465 ) ) ;
#3694=VECTOR ( 'NONE', #30113, 1000.000000000000227 ) ;
#3695=DIRECTION ( 'NONE',  ( 0.007781995580012662783, 0.000000000000000000, -0.9999697198139514409 ) ) ;
#3696=EDGE_LOOP ( 'NONE', ( #50013, #22668, #7321, #9847 ) ) ;
#3697=DIRECTION ( 'NONE',  ( 1.000000000000000000, 0.000000000000000000, 0.000000000000000000 ) ) ;
#3699=VERTEX_POINT ( 'NONE', #6935 ) ;
#3700=CARTESIAN_POINT ( 'NONE',  ( -18.68332481975068760, -2.298917212465658277, 7.712084379083277597 ) ) ;
#3701=CARTESIAN_POINT ( 'NONE',  ( -18.12332189171708663, 0.000000000000000000, 4.510041230393051492 ) ) ;
#3702=DIRECTION ( 'NONE',  ( -0.005002170337468016433, -0.7660444431189770143, 0.6427681459581293666 ) ) ;
#3703=LINE ( 'NONE', #34647, #41439 ) ;
#3704=CARTESIAN_POINT ( 'NONE',  ( -12.62864409447993808, 2.067327705546504912, 5.179552317802938788 ) ) ;
#3705=ORIENTED_EDGE ( 'NONE', *, *, #45656, .T. ) ;
#3706=VERTEX_POINT ( 'NONE', #45261 ) ;
#3707=FACE_OUTER_BOUND ( 'NONE', #4565, .T. ) ;
#3708=CARTESIAN_POINT ( 'NONE',  ( -26.13493519185646008, 0.000000000000000000, 7.033017491833586377 ) ) ;
#3710=CARTESIAN_POINT ( 'NONE',  ( -8.831699957570222637, -8.502732429729430663, 0.2121586136495015040 ) ) ;
#3711=EDGE_CURVE ( 'NONE', #40367, #11131, #54069, .T. ) ;
#3712=VECTOR ( 'NONE', #23295, 999.9999999999998863 ) ;
#3713=VECTOR ( 'NONE', #30723, 999.9999999999998863 ) ;
#3714=ORIENTED_EDGE ( 'NONE', *, *, #35463, .T. ) ;
#3715=LINE ( 'NONE', #55396, #3194 ) ;
#3716=ORIENTED_EDGE ( 'NONE', *, *, #25034, .F. ) ;
#3717=LINE ( 'NONE', #24460, #6642 ) ;
#3720=ORIENTED_EDGE ( 'NONE', *, *, #36641, .T. ) ;
#3721=ORIENTED_EDGE ( 'NONE', *, *, #24479, .F. ) ;
#3722=ORIENTED_EDGE ( 'NONE', *, *, #16123, .F. ) ;
#3723=CARTESIAN_POINT ( 'NONE',  ( -10.24493344548221430, 0.000000000000000000, 7.197853645293383451 ) ) ;
#3724=CARTESIAN_POINT ( 'NONE',  ( -19.19976828709737049, -2.946525016555661125, 4.245153571985499141 ) ) ;
#3725=DIRECTION ( 'NONE',  ( 0.6246952433987894571, -0.7422098413412800966, -0.2426528472758541777 ) ) ;
#3726=AXIS2_PLACEMENT_3D ( 'NONE', #10183, #26665, #18992 ) ;
#3728=VERTEX_POINT ( 'NONE', #24247 ) ;
#3729=VECTOR ( 'NONE', #31537, 1000.000000000000227 ) ;
#3730=ORIENTED_EDGE ( 'NONE', *, *, #17146, .T. ) ;
#3731=ORIENTED_EDGE ( 'NONE', *, *, #14251, .T. ) ;
#3732=CARTESIAN_POINT ( 'NONE',  ( 2.072287782118878319, 0.000000000000000000, -2.950529333540147015 ) ) ;
#3733=DIRECTION ( 'NONE',  ( 0.7660212471507180654, -0.6427876096865404731, 0.005961354470445141482 ) ) ;
#3734=ORIENTED_EDGE ( 'NONE', *, *, #14449, .F. ) ;
#3735=CARTESIAN_POINT ( 'NONE',  ( -13.96458224818957561, 0.000000000000000000, 7.497062062367251478 ) ) ;
#3736=ORIENTED_EDGE ( 'NONE', *, *, #39966, .T. ) ;
#3737=LINE ( 'NONE', #7438, #12438 ) ;
#3738=DIRECTION ( 'NONE',  ( 0.007781995580012662783, 0.000000000000000000, -0.9999697198139514409 ) ) ;
#3740=LINE ( 'NONE', #47777, #35884 ) ;
#3741=ORIENTED_EDGE ( 'NONE', *, *, #39483, .F. ) ;
#3742=EDGE_CURVE ( 'NONE', #21263, #55546, #15180, .T. ) ;
#3743=LINE ( 'NONE', #25921, #14695 ) ;
#3744=LINE ( 'NONE', #29889, #55585 ) ;
#3745=ORIENTED_EDGE ( 'NONE', *, *, #55058, .T. ) ;
#3746=ADVANCED_FACE ( 'NONE', ( #14598 ), #14345, .F. ) ;
#3747=DIRECTION ( 'NONE',  ( 0.6427681459581294776, -0.7660444431189769032, 0.005002170337467562802 ) ) ;
#3748=CARTESIAN_POINT ( 'NONE',  ( -17.73140113748535285, 0.000000000000000000, 13.85752530597602039 ) ) ;
#3750=DIRECTION ( 'NONE',  ( 0.9999697198139515519, 0.000000000000000000, 0.007781995580013368816 ) ) ;
#3751=ADVANCED_FACE ( 'NONE', ( #19126 ), #49232, .F. ) ;
#3753=AXIS2_PLACEMENT_3D ( 'NONE', #49561, #26856, #1820 ) ;
#3754=VECTOR ( 'NONE', #35210, 1000.000000000000114 ) ;
#3756=EDGE_CURVE ( 'NONE', #7643, #16969, #49536, .T. ) ;
#3757=FACE_OUTER_BOUND ( 'NONE', #26067, .T. ) ;
#3758=CARTESIAN_POINT ( 'NONE',  ( -9.751071550147864642, -0.1191753592594205075, 1.889868501687798741 ) ) ;
#3759=DIRECTION ( 'NONE',  ( 0.005002170337468016433, -0.7660444431189770143, -0.6427681459581293666 ) ) ;
#3760=DIRECTION ( 'NONE',  ( -0.9999697198139514409, -0.000000000000000000, -0.007781995580013368816 ) ) ;
#3761=DIRECTION ( 'NONE',  ( 0.007781995580012663651, 0.000000000000000000, -0.9999697198139515519 ) ) ;
#3762=VECTOR ( 'NONE', #52967, 999.9999999999998863 ) ;
#3763=ORIENTED_EDGE ( 'NONE', *, *, #25850, .T. ) ;
#3764=CARTESIAN_POINT ( 'NONE',  ( 2.072287782118878319, 0.000000000000000000, -2.950529333540147015 ) ) ;
#3765=DIRECTION ( 'NONE',  ( 0.000000000000000000, -1.000000000000000000, 0.000000000000000000 ) ) ;
#3766=CARTESIAN_POINT ( 'NONE',  ( -16.13086958175276919, -2.622721114510659479, 3.063420134365714809 ) ) ;
#3767=VERTEX_POINT ( 'NONE', #45519 ) ;
#3768=FACE_OUTER_BOUND ( 'NONE', #49837, .T. ) ;
#3769=ORIENTED_EDGE ( 'NONE', *, *, #11557, .T. ) ;
#3770=DIRECTION ( 'NONE',  ( -0.7660212471507179544, -0.6427876096865405842, -0.005961354470445141482 ) ) ;
#3771=CARTESIAN_POINT ( 'NONE',  ( -8.875996589204540044, 0.000000000000000000, 10.41778544861944233 ) ) ;
#3772=ADVANCED_FACE ( 'NONE', ( #10350 ), #23413, .F. ) ;
#3773=CARTESIAN_POINT ( 'NONE',  ( -17.73140113748535285, 0.000000000000000000, 13.85752530597602039 ) ) ;
#3774=VECTOR ( 'NONE', #31503, 1000.000000000000227 ) ;
#3776=ORIENTED_EDGE ( 'NONE', *, *, #20339, .F. ) ;
#3777=ORIENTED_EDGE ( 'NONE', *, *, #24800, .T. ) ;
#3780=DIRECTION ( 'NONE',  ( -0.5449076811759708816, 0.6444004775717707689, 0.5364919789714475140 ) ) ;
#3781=ADVANCED_FACE ( 'NONE', ( #1800 ), #19409, .F. ) ;
#3782=CARTESIAN_POINT ( 'NONE',  ( -21.66636548695712250, -3.108426967578159950, 5.198098170517139849 ) ) ;
#3783=FACE_OUTER_BOUND ( 'NONE', #50688, .T. ) ;
#3784=EDGE_CURVE ( 'NONE', #40645, #45163, #45001, .T. ) ;
#3785=DIRECTION ( 'NONE',  ( -0.2426528472758541499, 0.7422098413412800966, -0.6246952433987894571 ) ) ;
#3786=ORIENTED_EDGE ( 'NONE', *, *, #16463, .F. ) ;
#3787=LINE ( 'NONE', #29072, #21101 ) ;
#3788=EDGE_CURVE ( 'NONE', #42922, #32724, #35930, .T. ) ;
#3789=LINE ( 'NONE', #21111, #45069 ) ;
#3790=CARTESIAN_POINT ( 'NONE',  ( -17.76560056444620272, -4.565544526780662693, 3.636418925093014121 ) ) ;
#3791=VERTEX_POINT ( 'NONE', #27959 ) ;
#3792=LINE ( 'NONE', #8079, #24755 ) ;
#3793=CARTESIAN_POINT ( 'NONE',  ( -16.73072885558310929, 0.000000000000000000, 4.690204724992056207 ) ) ;
#3794=CARTESIAN_POINT ( 'NONE',  ( -12.24460538506144580, -1.327505506330657781, 1.595187301382279488 ) ) ;
#3795=ORIENTED_EDGE ( 'NONE', *, *, #30079, .F. ) ;
#3796=VECTOR ( 'NONE', #18535, 1000.000000000000114 ) ;
#3797=VECTOR ( 'NONE', #43253, 999.9999999999998863 ) ;
#3798=DIRECTION ( 'NONE',  ( -0.6427681459581293666, -0.7660444431189770143, -0.005002170337467561935 ) ) ;
#3799=VERTEX_POINT ( 'NONE', #53764 ) ;
#3800=EDGE_CURVE ( 'NONE', #40584, #33081, #23952, .T. ) ;
#3801=EDGE_LOOP ( 'NONE', ( #49292, #19039, #48026, #9314, #35593 ) ) ;
#3802=ORIENTED_EDGE ( 'NONE', *, *, #47332, .F. ) ;
#3803=VECTOR ( 'NONE', #6295, 1000.000000000000114 ) ;
#3804=VERTEX_POINT ( 'NONE', #50053 ) ;
#3805=FACE_OUTER_BOUND ( 'NONE', #21835, .T. ) ;
#3806=ORIENTED_EDGE ( 'NONE', *, *, #31549, .F. ) ;
#3807=CARTESIAN_POINT ( 'NONE',  ( -16.84012618763835434, -0.1191753592594188005, 5.897352607188737217 ) ) ;
#3808=ORIENTED_EDGE ( 'NONE', *, *, #48998, .T. ) ;
#3809=CARTESIAN_POINT ( 'NONE',  ( -11.42723989371472548, -0.3560938001956568399, 1.308687906018629166 ) ) ;
#3810=ORIENTED_EDGE ( 'NONE', *, *, #21752, .F. ) ;
#3811=VECTOR ( 'NONE', #16978, 1000.000000000000114 ) ;
#3812=ORIENTED_EDGE ( 'NONE', *, *, #56007, .T. ) ;
#3813=VECTOR ( 'NONE', #23785, 1000.000000000000227 ) ;
#3814=DIRECTION ( 'NONE',  ( -0.7660212471507179544, -0.6427876096865405842, -0.005961354470445141482 ) ) ;
#3815=DIRECTION ( 'NONE',  ( 0.5449076811759707706, 0.6444004775717708799, -0.5364919789714476250 ) ) ;
#3816=PLANE ( 'NONE',  #33117 ) ;
#3817=FACE_OUTER_BOUND ( 'NONE', #29021, .T. ) ;
#3818=LINE ( 'NONE', #15762, #5686 ) ;
#3819=VERTEX_POINT ( 'NONE', #11165 ) ;
#3820=ORIENTED_EDGE ( 'NONE', *, *, #22266, .F. ) ;
#3821=CARTESIAN_POINT ( 'NONE',  ( 2.072287782118878319, 0.000000000000000000, -2.950529333540147015 ) ) ;
#3822=EDGE_CURVE ( 'NONE', #34361, #51066, #10057, .T. ) ;
#3824=VECTOR ( 'NONE', #41146, 1000.000000000000227 ) ;
#3825=LINE ( 'NONE', #21153, #16093 ) ;
#3826=DIRECTION ( 'NONE',  ( 0.5449076811759707706, 0.6444004775717708799, -0.5364919789714476250 ) ) ;
#3827=DIRECTION ( 'NONE',  ( 0.007781995580012662783, 0.000000000000000000, -0.9999697198139514409 ) ) ;
#3828=CARTESIAN_POINT ( 'NONE',  ( -23.33849165029409889, 0.000000000000000000, 5.946783852668351855 ) ) ;
#3829=ORIENTED_EDGE ( 'NONE', *, *, #37551, .T. ) ;
#3830=VECTOR ( 'NONE', #21801, 1000.000000000000227 ) ;
#3831=CARTESIAN_POINT ( 'NONE',  ( -17.39404204199770376, 0.000000000000000000, 4.515716654813066278 ) ) ;
#3832=CARTESIAN_POINT ( 'NONE',  ( -19.99336569310255740, 0.000000000000000000, 5.972816396352070178 ) ) ;
#3833=ORIENTED_EDGE ( 'NONE', *, *, #50571, .F. ) ;
#3834=ADVANCED_FACE ( 'NONE', ( #44690 ), #25361, .F. ) ;
#3835=VECTOR ( 'NONE', #31745, 1000.000000000000227 ) ;
#3836=VECTOR ( 'NONE', #19329, 1000.000000000000227 ) ;
#3837=DIRECTION ( 'NONE',  ( 0.007781995580012662783, 0.000000000000000000, -0.9999697198139514409 ) ) ;
#3838=DIRECTION ( 'NONE',  ( 0.7660212471507180654, -0.6427876096865404731, 0.005961354470445141482 ) ) ;
#3840=EDGE_CURVE ( 'NONE', #17107, #4086, #7466, .T. ) ;
#3841=EDGE_CURVE ( 'NONE', #12750, #47914, #19964, .T. ) ;
#3842=LINE ( 'NONE', #50143, #8744 ) ;
#3843=ORIENTED_EDGE ( 'NONE', *, *, #35667, .T. ) ;
#3844=VECTOR ( 'NONE', #525, 999.9999999999998863 ) ;
#3845=VECTOR ( 'NONE', #40239, 999.9999999999998863 ) ;
#3846=ORIENTED_EDGE ( 'NONE', *, *, #10440, .T. ) ;
#3847=PLANE ( 'NONE',  #23951 ) ;
#3849=CARTESIAN_POINT ( 'NONE',  ( -10.37421533196711465, -0.1191753592594197858, 10.96012406864405975 ) ) ;
#3850=EDGE_CURVE ( 'NONE', #25320, #21782, #7768, .T. ) ;
#3852=EDGE_CURVE ( 'NONE', #42332, #5412, #42662, .T. ) ;
#3854=CARTESIAN_POINT ( 'NONE',  ( -18.39746900504187010, 0.000000000000000000, 14.03700784672088808 ) ) ;
#3855=CARTESIAN_POINT ( 'NONE',  ( 2.072287782118878319, 0.000000000000000000, -2.950529333540147015 ) ) ;
#3856=CARTESIAN_POINT ( 'NONE',  ( -19.12962290826653700, 0.000000000000000000, 14.40064212555863854 ) ) ;
#3857=ADVANCED_FACE ( 'NONE', ( #54587 ), #25098, .F. ) ;
#3859=PLANE ( 'NONE',  #26922 ) ;
#3860=FACE_OUTER_BOUND ( 'NONE', #50099, .T. ) ;
#3861=VERTEX_POINT ( 'NONE', #29050 ) ;
#3862=CARTESIAN_POINT ( 'NONE',  ( -12.66414222307914450, -0.1191753592594190225, 6.668515219616352852 ) ) ;
#3863=EDGE_CURVE ( 'NONE', #19811, #13531, #16544, .T. ) ;
#3864=ORIENTED_EDGE ( 'NONE', *, *, #48035, .F. ) ;
#3865=ORIENTED_EDGE ( 'NONE', *, *, #3822, .T. ) ;
#3866=ADVANCED_FACE ( 'NONE', ( #21081 ), #33875, .F. ) ;
#3867=ORIENTED_EDGE ( 'NONE', *, *, #714, .T. ) ;
#3868=EDGE_LOOP ( 'NONE', ( #33554, #45631, #19997 ) ) ;
#3869=ORIENTED_EDGE ( 'NONE', *, *, #29298, .F. ) ;
#3870=ORIENTED_EDGE ( 'NONE', *, *, #6691, .T. ) ;
#3871=VECTOR ( 'NONE', #24820, 1000.000000000000227 ) ;
#3872=CARTESIAN_POINT ( 'NONE',  ( -21.30476517517178436, 4.657758921906512306, 4.808819142744448882 ) ) ;
#3873=CARTESIAN_POINT ( 'NONE',  ( -12.60458797795435615, 0.000000000000000000, 11.86609696750642229 ) ) ;
#3874=LINE ( 'NONE', #46460, #20330 ) ;
#3875=AXIS2_PLACEMENT_3D ( 'NONE', #52206, #47944, #52481 ) ;
#3876=VECTOR ( 'NONE', #15494, 999.9999999999998863 ) ;
#3877=ORIENTED_EDGE ( 'NONE', *, *, #48509, .T. ) ;
#3878=LINE ( 'NONE', #21203, #53963 ) ;
#3879=ORIENTED_EDGE ( 'NONE', *, *, #41297, .F. ) ;
#3880=CARTESIAN_POINT ( 'NONE',  ( -19.22617103857668397, 4.333955019861509328, 11.46217741115471433 ) ) ;
#3881=ORIENTED_EDGE ( 'NONE', *, *, #17818, .F. ) ;
#3882=AXIS2_PLACEMENT_3D ( 'NONE', #2030, #49190, #10309 ) ;
#3883=VECTOR ( 'NONE', #18095, 1000.000000000000000 ) ;
#3884=PLANE ( 'NONE',  #30184 ) ;
#3885=LINE ( 'NONE', #34007, #47308 ) ;
#3886=DIRECTION ( 'NONE',  ( 0.005002170337468016433, -0.7660444431189770143, -0.6427681459581293666 ) ) ;
#3888=DIRECTION ( 'NONE',  ( 0.000000000000000000, -1.000000000000000000, 0.000000000000000000 ) ) ;
#3890=DIRECTION ( 'NONE',  ( 0.9999697198139515519, 0.000000000000000000, 0.007781995580013368816 ) ) ;
#3891=VECTOR ( 'NONE', #14337, 999.9999999999998863 ) ;
#3892=ADVANCED_FACE ( 'NONE', ( #54897 ), #2907, .F. ) ;
#3893=PLANE ( 'NONE',  #17572 ) ;
#3894=AXIS2_PLACEMENT_3D ( 'NONE', #12116, #46189, #29149 ) ;
#3895=DIRECTION ( 'NONE',  ( -0.7660212471507179544, -0.6427876096865405842, -0.005961354470445141482 ) ) ;
#3896=PLANE ( 'NONE',  #9569 ) ;
#3897=DIRECTION ( 'NONE',  ( 0.007781995580012662783, 0.000000000000000000, -0.9999697198139514409 ) ) ;
#3898=LINE ( 'NONE', #30031, #10387 ) ;
#3899=LINE ( 'NONE', #50760, #12137 ) ;
#3900=DIRECTION ( 'NONE',  ( 0.9999697198139515519, 0.000000000000000000, 0.007781995580013368816 ) ) ;
#3901=ORIENTED_EDGE ( 'NONE', *, *, #25657, .F. ) ;
#3902=CARTESIAN_POINT ( 'NONE',  ( -19.99468334749183995, 0.000000000000000000, 6.142132155647047398 ) ) ;
#3903=ORIENTED_EDGE ( 'NONE', *, *, #49899, .T. ) ;
#3904=ADVANCED_FACE ( 'NONE', ( #50898 ), #29646, .F. ) ;
#3905=VECTOR ( 'NONE', #43838, 999.9999999999998863 ) ;
#3906=EDGE_CURVE ( 'NONE', #17592, #39633, #51197, .T. ) ;
#3907=ADVANCED_FACE ( 'NONE', ( #3213 ), #55736, .F. ) ;
#3908=DIRECTION ( 'NONE',  ( 0.5449076811759707706, 0.6444004775717708799, -0.5364919789714476250 ) ) ;
#3909=DIRECTION ( 'NONE',  ( 0.9999697198139515519, 0.000000000000000000, 0.007781995580013368816 ) ) ;
#3910=CARTESIAN_POINT ( 'NONE',  ( -17.93139508144814442, 0.000000000000000000, 13.85596890686001537 ) ) ;
#3911=AXIS2_PLACEMENT_3D ( 'NONE', #9096, #31240, #1118 ) ;
#3912=DIRECTION ( 'NONE',  ( -0.5449076811759708816, 0.6444004775717707689, 0.5364919789714475140 ) ) ;
#3913=CARTESIAN_POINT ( 'NONE',  ( -12.56911515855031425, 0.000000000000000000, 7.307915853708490950 ) ) ;
#3914=EDGE_CURVE ( 'NONE', #49603, #49579, #33334, .T. ) ;
#3915=FACE_OUTER_BOUND ( 'NONE', #2107, .T. ) ;
#3917=VERTEX_POINT ( 'NONE', #20809 ) ;
#3918=AXIS2_PLACEMENT_3D ( 'NONE', #48578, #47754, #43219 ) ;
#3919=DIRECTION ( 'NONE',  ( -0.005002170337468016433, -0.7660444431189770143, 0.6427681459581293666 ) ) ;
#3920=FACE_OUTER_BOUND ( 'NONE', #45311, .T. ) ;
#3921=DIRECTION ( 'NONE',  ( 0.9999697198139515519, 0.000000000000000000, 0.007781995580013368816 ) ) ;
#3922=AXIS2_PLACEMENT_3D ( 'NONE', #49264, #35961, #5544 ) ;
#3923=VECTOR ( 'NONE', #34377, 1000.000000000000000 ) ;
#3925=EDGE_CURVE ( 'NONE', #428, #13272, #25627, .T. ) ;
#3926=DIRECTION ( 'NONE',  ( 0.9999697198139515519, 0.000000000000000000, 0.007781995580013368816 ) ) ;
#3927=DIRECTION ( 'NONE',  ( -0.005961354470445682716, -0.6427876096865404731, 0.7660212471507180654 ) ) ;
#3928=CARTESIAN_POINT ( 'NONE',  ( 2.072287782118878319, 0.000000000000000000, -2.950529333540147015 ) ) ;
#3929=VERTEX_POINT ( 'NONE', #46949 ) ;
#3930=ADVANCED_FACE ( 'NONE', ( #8050 ), #2639, .F. ) ;
#3931=VECTOR ( 'NONE', #41468, 1000.000000000000000 ) ;
#3932=DIRECTION ( 'NONE',  ( 0.9999697198139515519, 0.000000000000000000, 0.007781995580013368816 ) ) ;
#3933=VECTOR ( 'NONE', #48905, 999.9999999999998863 ) ;
#3934=CARTESIAN_POINT ( 'NONE',  ( -23.33849165029409889, 0.000000000000000000, 5.946783852668351855 ) ) ;
#3935=ORIENTED_EDGE ( 'NONE', *, *, #53244, .T. ) ;
#3936=ADVANCED_FACE ( 'NONE', ( #29336 ), #46092, .F. ) ;
#3937=ORIENTED_EDGE ( 'NONE', *, *, #27808, .F. ) ;
#3938=DIRECTION ( 'NONE',  ( 0.007781995580012663651, 0.000000000000000000, -0.9999697198139515519 ) ) ;
#3939=ADVANCED_FACE ( 'NONE', ( #25937 ), #30478, .F. ) ;
#3940=ORIENTED_EDGE ( 'NONE', *, *, #55010, .T. ) ;
#3941=ORIENTED_EDGE ( 'NONE', *, *, #53311, .T. ) ;
#3942=ORIENTED_EDGE ( 'NONE', *, *, #40428, .T. ) ;
#3943=ORIENTED_EDGE ( 'NONE', *, *, #51392, .F. ) ;
#3944=VECTOR ( 'NONE', #49207, 1000.000000000000114 ) ;
#3945=CARTESIAN_POINT ( 'NONE',  ( -19.60834386242827776, 0.000000000000000000, 4.298478389818581213 ) ) ;
#3946=ORIENTED_EDGE ( 'NONE', *, *, #3320, .F. ) ;
#3947=DIRECTION ( 'NONE',  ( -0.5364919789714478471, 0.6444004775717705469, -0.5449076811759709926 ) ) ;
#3948=CARTESIAN_POINT ( 'NONE',  ( -13.91947430141211584, 1.419719901456504507, 2.043431759590222718 ) ) ;
#3949=VECTOR ( 'NONE', #11593, 999.9999999999998863 ) ;
#3950=ORIENTED_EDGE ( 'NONE', *, *, #15506, .F. ) ;
#3951=VERTEX_POINT ( 'NONE', #13145 ) ;
#3953=DIRECTION ( 'NONE',  ( 0.000000000000000000, -0.000000000000000000, -1.000000000000000000 ) ) ;
#3954=CARTESIAN_POINT ( 'NONE',  ( -13.89383709357448282, -0.5179957512181557755, 2.261632504550268763 ) ) ;
#3955=ORIENTED_EDGE ( 'NONE', *, *, #20590, .T. ) ;
#3956=VECTOR ( 'NONE', #41846, 1000.000000000000227 ) ;
#3957=CARTESIAN_POINT ( 'NONE',  ( -20.28683642378279117, 0.1245042932765029059, 4.558055603545987822 ) ) ;
#3958=DIRECTION ( 'NONE',  ( 0.007781995580012663651, -3.146120232559066537E-19, -0.9999697198139514409 ) ) ;
#3959=ORIENTED_EDGE ( 'NONE', *, *, #34204, .T. ) ;
#3960=PLANE ( 'NONE',  #10410 ) ;
#3961=EDGE_CURVE ( 'NONE', #25102, #1588, #52860, .T. ) ;
#3962=VECTOR ( 'NONE', #698, 1000.000000000000114 ) ;
#3963=VERTEX_POINT ( 'NONE', #17681 ) ;
#3964=FACE_OUTER_BOUND ( 'NONE', #56057, .T. ) ;
#3965=EDGE_CURVE ( 'NONE', #23095, #41647, #43264, .T. ) ;
#3966=AXIS2_PLACEMENT_3D ( 'NONE', #39829, #9158, #22521 ) ;
#3967=PLANE ( 'NONE',  #6430 ) ;
#3968=VECTOR ( 'NONE', #55064, 999.9999999999998863 ) ;
#3969=ORIENTED_EDGE ( 'NONE', *, *, #41662, .F. ) ;
#3970=LINE ( 'NONE', #11917, #30396 ) ;
#3971=DIRECTION ( 'NONE',  ( -0.3313982828793700652, 0.4028455766673916250, -0.8531650599175529814 ) ) ;
#3972=LINE ( 'NONE', #55363, #17586 ) ;
#3973=DIRECTION ( 'NONE',  ( 0.5449076811759707706, 0.6444004775717708799, -0.5364919789714476250 ) ) ;
#3974=ORIENTED_EDGE ( 'NONE', *, *, #35887, .F. ) ;
#3975=EDGE_CURVE ( 'NONE', #37937, #52731, #21387, .T. ) ;
#3977=EDGE_CURVE ( 'NONE', #41994, #11772, #52331, .T. ) ;
#3978=PLANE ( 'NONE',  #54572 ) ;
#3979=CARTESIAN_POINT ( 'NONE',  ( -14.66887761629205222, 0.000000000000000000, 12.58869632783390990 ) ) ;
#3980=PLANE ( 'NONE',  #1312 ) ;
#3982=EDGE_CURVE ( 'NONE', #21963, #34820, #42952, .T. ) ;
#3983=CARTESIAN_POINT ( 'NONE',  ( -18.32501161783028110, -2.460819163488160655, 3.920864934442803040 ) ) ;
#3984=DIRECTION ( 'NONE',  ( -0.7660212471507179544, -0.6427876096865405842, -0.005961354470445141482 ) ) ;
#3985=LINE ( 'NONE', #18159, #3016 ) ;
#3986=LINE ( 'NONE', #4294, #41302 ) ;
#3988=VERTEX_POINT ( 'NONE', #30750 ) ;
#3989=CARTESIAN_POINT ( 'NONE',  ( 2.072287782118878319, 0.000000000000000000, -2.950529333540147015 ) ) ;
#3990=ORIENTED_EDGE ( 'NONE', *, *, #45835, .T. ) ;
#3991=PLANE ( 'NONE',  #46517 ) ;
#3992=MANIFOLD_SOLID_BREP ( 'Boss-Extrude3', #22238 ) ;
#3993=CARTESIAN_POINT ( 'NONE',  ( -27.06552663992790997, 0.000000000000000000, 7.195101427592543786 ) ) ;
#3994=AXIS2_PLACEMENT_3D ( 'NONE', #9213, #16917, #4964 ) ;
#3995=DIRECTION ( 'NONE',  ( 0.5449076811759707706, 0.6444004775717708799, -0.5364919789714476250 ) ) ;
#3996=AXIS2_PLACEMENT_3D ( 'NONE', #7317, #29177, #55298 ) ;
#3997=CARTESIAN_POINT ( 'NONE',  ( 1.086233639165236964, 0.000000000000000000, 2.796443541562362078 ) ) ;
#3998=EDGE_CURVE ( 'NONE', #13117, #49510, #35549, .T. ) ;
#3999=CARTESIAN_POINT ( 'NONE',  ( -13.60152578229115505, -0.1117717739994002479, 8.501668099265545564 ) ) ;
#4000=ORIENTED_EDGE ( 'NONE', *, *, #19227, .F. ) ;
#4001=ADVANCED_FACE ( 'NONE', ( #30175 ), #21667, .F. ) ;
#4002=ORIENTED_EDGE ( 'NONE', *, *, #5169, .T. ) ;
#4003=EDGE_CURVE ( 'NONE', #56039, #14373, #8606, .T. ) ;
#4004=LINE ( 'NONE', #42615, #50400 ) ;
#4005=VECTOR ( 'NONE', #5772, 1000.000000000000227 ) ;
#4006=FACE_OUTER_BOUND ( 'NONE', #15641, .T. ) ;
#4007=ORIENTED_EDGE ( 'NONE', *, *, #29411, .F. ) ;
#4008=VECTOR ( 'NONE', #1466, 1000.000000000000114 ) ;
#4009=FACE_OUTER_BOUND ( 'NONE', #1359, .T. ) ;
#4010=ADVANCED_FACE ( 'NONE', ( #13683 ), #30996, .F. ) ;
#4012=CARTESIAN_POINT ( 'NONE',  ( -21.47263955680318404, 0.000000000000000000, 5.022634149262071190 ) ) ;
#4014=LINE ( 'NONE', #28747, #12967 ) ;
#4015=EDGE_CURVE ( 'NONE', #21230, #9004, #40085, .T. ) ;
#4016=VECTOR ( 'NONE', #791, 999.9999999999998863 ) ;
#4017=ORIENTED_EDGE ( 'NONE', *, *, #55575, .F. ) ;
#4018=VECTOR ( 'NONE', #18303, 999.9999999999998863 ) ;
#4019=ORIENTED_EDGE ( 'NONE', *, *, #10225, .F. ) ;
#4020=ORIENTED_EDGE ( 'NONE', *, *, #21577, .T. ) ;
#4021=FACE_OUTER_BOUND ( 'NONE', #50685, .T. ) ;
#4022=CARTESIAN_POINT ( 'NONE',  ( -13.73672976910459909, 0.000000000000000000, 12.22661844811216270 ) ) ;
#4023=LINE ( 'NONE', #3461, #48429 ) ;
#4024=CARTESIAN_POINT ( 'NONE',  ( -10.47421230394850866, 0.000000000000000000, 10.95934586908605723 ) ) ;
#4025=VERTEX_POINT ( 'NONE', #28144 ) ;
#4026=ORIENTED_EDGE ( 'NONE', *, *, #35168, .F. ) ;
#4029=LINE ( 'NONE', #7433, #1414 ) ;
#4030=DIRECTION ( 'NONE',  ( 0.007781995580012663651, 0.000000000000000000, -0.9999697198139515519 ) ) ;
#4031=VECTOR ( 'NONE', #30379, 1000.000000000000227 ) ;
#4032=VERTEX_POINT ( 'NONE', #36676 ) ;
#4033=DIRECTION ( 'NONE',  ( -0.5364919789714478471, 0.6444004775717705469, -0.5449076811759709926 ) ) ;
#4034=ORIENTED_EDGE ( 'NONE', *, *, #44223, .T. ) ;
#4035=VECTOR ( 'NONE', #38334, 1000.000000000000114 ) ;
#4036=FACE_OUTER_BOUND ( 'NONE', #24428, .T. ) ;
#4037=CARTESIAN_POINT ( 'NONE',  ( -28.92982233430281980, 0.000000000000000000, 7.919257187036034651 ) ) ;
#4038=VERTEX_POINT ( 'NONE', #1740 ) ;
#4039=CARTESIAN_POINT ( 'NONE',  ( -22.43336023615409047, -5.051250379848161387, 13.68577311371102567 ) ) ;
#4040=EDGE_LOOP ( 'NONE', ( #4527, #28209, #32537, #50784 ) ) ;
#4041=DIRECTION ( 'NONE',  ( 0.007781995580012662783, 0.000000000000000000, -0.9999697198139514409 ) ) ;
#4042=DIRECTION ( 'NONE',  ( 0.9999697198139515519, 0.000000000000000000, 0.007781995580013368816 ) ) ;
#4043=VECTOR ( 'NONE', #44228, 999.9999999999998863 ) ;
#4045=LINE ( 'NONE', #17111, #19571 ) ;
#4046=LINE ( 'NONE', #38397, #47457 ) ;
#4047=AXIS2_PLACEMENT_3D ( 'NONE', #46006, #50545, #12189 ) ;
#4048=CARTESIAN_POINT ( 'NONE',  ( -10.68625748875443016, 0.000000000000000000, 4.198586115423438514 ) ) ;
#4050=VECTOR ( 'NONE', #33033, 1000.000000000000000 ) ;
#4052=LINE ( 'NONE', #9141, #17382 ) ;
#4054=LINE ( 'NONE', #38406, #52203 ) ;
#4055=EDGE_CURVE ( 'NONE', #10808, #55191, #46883, .T. ) ;
#4056=ADVANCED_FACE ( 'NONE', ( #15626 ), #41746, .F. ) ;
#4057=CARTESIAN_POINT ( 'NONE',  ( -27.99767448711536133, 0.000000000000000000, 7.557179307314289218 ) ) ;
#4058=LINE ( 'NONE', #50897, #16130 ) ;
#4060=VECTOR ( 'NONE', #29509, 1000.000000000000114 ) ;
#4061=DIRECTION ( 'NONE',  ( -0.5449076811759708816, 0.6444004775717707689, 0.5364919789714475140 ) ) ;
#4062=EDGE_LOOP ( 'NONE', ( #33383, #6408, #9272, #13183 ) ) ;
#4063=CARTESIAN_POINT ( 'NONE',  ( -18.13194405223293515, 0.000000000000000000, 5.617970340166344556 ) ) ;
#4064=DIRECTION ( 'NONE',  ( 0.005961354470445682716, -0.6427876096865404731, -0.7660212471507180654 ) ) ;
#4065=DIRECTION ( 'NONE',  ( 0.000000000000000000, 1.000000000000000000, 0.000000000000000000 ) ) ;
#4067=CARTESIAN_POINT ( 'NONE',  ( -19.24265873919813430, -5.213152330870665097, 4.189496401723858732 ) ) ;
#4068=DIRECTION ( 'NONE',  ( 0.000000000000000000, -0.000000000000000000, -1.000000000000000000 ) ) ;
#4069=ORIENTED_EDGE ( 'NONE', *, *, #13133, .T. ) ;
#4071=LINE ( 'NONE', #42671, #8621 ) ;
#4072=CARTESIAN_POINT ( 'NONE',  ( -14.10280672071693431, -0.1191753592594197858, 12.40843558753103792 ) ) ;
#4074=VECTOR ( 'NONE', #54463, 1000.000000000000227 ) ;
#4075=ORIENTED_EDGE ( 'NONE', *, *, #12242, .F. ) ;
#4076=ORIENTED_EDGE ( 'NONE', *, *, #34202, .T. ) ;
#4077=VECTOR ( 'NONE', #35395, 999.9999999999998863 ) ;
#4079=PLANE ( 'NONE',  #3257 ) ;
#4080=PLANE ( 'NONE',  #26106 ) ;
#4081=AXIS2_PLACEMENT_3D ( 'NONE', #10660, #27114, #39888 ) ;
#4082=DIRECTION ( 'NONE',  ( 0.007781995580012663651, -3.146120232559066537E-19, -0.9999697198139514409 ) ) ;
#4083=LINE ( 'NONE', #12337, #35540 ) ;
#4084=DIRECTION ( 'NONE',  ( 0.005002170337468016433, -0.7660444431189770143, -0.6427681459581293666 ) ) ;
#4085=AXIS2_PLACEMENT_3D ( 'NONE', #18495, #5443, #48038 ) ;
#4086=VERTEX_POINT ( 'NONE', #29571 ) ;
#4088=EDGE_CURVE ( 'NONE', #13096, #45339, #33802, .T. ) ;
#4089=CARTESIAN_POINT ( 'NONE',  ( -18.67775241435682432, 0.000000000000000000, 4.136394454059623804 ) ) ;
#4090=AXIS2_PLACEMENT_3D ( 'NONE', #29696, #46990, #34477 ) ;
#4093=EDGE_CURVE ( 'NONE', #47084, #291, #11929, .T. ) ;
#4094=VECTOR ( 'NONE', #46295, 1000.000000000000114 ) ;
#4095=AXIS2_PLACEMENT_3D ( 'NONE', #52990, #49007, #6159 ) ;
#4096=CARTESIAN_POINT ( 'NONE',  ( -26.13493519185646008, 0.000000000000000000, 7.033017491833586377 ) ) ;
#4097=CARTESIAN_POINT ( 'NONE',  ( -11.36945030497927789, 0.000000000000000000, 6.578587783380987375 ) ) ;
#4098=ADVANCED_FACE ( 'NONE', ( #11392 ), #7988, .F. ) ;
#4099=CARTESIAN_POINT ( 'NONE',  ( -9.542064456761055524, 0.000000000000000000, 10.59726798936431180 ) ) ;
#4100=VECTOR ( 'NONE', #30103, 999.9999999999998863 ) ;
#4101=ORIENTED_EDGE ( 'NONE', *, *, #5244, .T. ) ;
#4102=LINE ( 'NONE', #12352, #20311 ) ;
#4103=EDGE_CURVE ( 'NONE', #20460, #40803, #46285, .T. ) ;
#4104=VERTEX_POINT ( 'NONE', #55374 ) ;
#4105=VECTOR ( 'NONE', #44639, 1000.000000000000227 ) ;
#4106=EDGE_LOOP ( 'NONE', ( #43685, #39669, #51110, #44680 ) ) ;
#4107=VECTOR ( 'NONE', #26526, 1000.000000000000000 ) ;
#4108=EDGE_LOOP ( 'NONE', ( #16444, #19843, #55183, #6160, #885 ) ) ;
#4109=ORIENTED_EDGE ( 'NONE', *, *, #10021, .T. ) ;
#4110=FACE_OUTER_BOUND ( 'NONE', #46545, .T. ) ;
#4111=ORIENTED_EDGE ( 'NONE', *, *, #51080, .T. ) ;
#4112=LINE ( 'NONE', #29384, #17712 ) ;
#4113=ORIENTED_EDGE ( 'NONE', *, *, #51878, .T. ) ;
#4114=LINE ( 'NONE', #12366, #29539 ) ;
#4115=EDGE_LOOP ( 'NONE', ( #8416, #31665, #54866, #30897 ) ) ;
#4116=FACE_OUTER_BOUND ( 'NONE', #51961, .T. ) ;
#4117=ORIENTED_EDGE ( 'NONE', *, *, #16794, .T. ) ;
#4118=AXIS2_PLACEMENT_3D ( 'NONE', #38499, #12403, #55830 ) ;
#4119=CARTESIAN_POINT ( 'NONE',  ( -10.90193935463291375, 0.000000000000000000, 6.212893991891234258 ) ) ;
#4120=VECTOR ( 'NONE', #42359, 999.9999999999998863 ) ;
#4121=LINE ( 'NONE', #29954, #29598 ) ;
#4122=DIRECTION ( 'NONE',  ( 0.005961354470445682716, -0.6427876096865404731, -0.7660212471507180654 ) ) ;
#4124=EDGE_CURVE ( 'NONE', #34978, #31046, #7392, .T. ) ;
#4125=CARTESIAN_POINT ( 'NONE',  ( -12.33850799832341849, 0.000000000000000000, 11.68350162852954632 ) ) ;
#4126=VECTOR ( 'NONE', #54667, 1000.000000000000227 ) ;
#4127=ORIENTED_EDGE ( 'NONE', *, *, #24960, .F. ) ;
#4128=ADVANCED_FACE ( 'NONE', ( #19900 ), #20474, .F. ) ;
#4129=ORIENTED_EDGE ( 'NONE', *, *, #51950, .F. ) ;
#4131=CARTESIAN_POINT ( 'NONE',  ( -17.79814051637334416, -0.1191753592594177180, 9.583217816230360953 ) ) ;
#4132=VECTOR ( 'NONE', #16845, 1000.000000000000227 ) ;
#4133=EDGE_CURVE ( 'NONE', #15482, #24338, #46572, .T. ) ;
#4134=EDGE_CURVE ( 'NONE', #25745, #47834, #55116, .T. ) ;
#4135=LINE ( 'NONE', #12918, #25188 ) ;
#4136=VECTOR ( 'NONE', #16248, 1000.000000000000000 ) ;
#4137=VECTOR ( 'NONE', #33076, 1000.000000000000114 ) ;
#4138=DIRECTION ( 'NONE',  ( -0.005961354470445682716, -0.6427876096865404731, 0.7660212471507180654 ) ) ;
#4139=CARTESIAN_POINT ( 'NONE',  ( -24.27063949748155380, 0.000000000000000000, 6.308861732390097288 ) ) ;
#4140=LINE ( 'NONE', #42474, #28645 ) ;
#4141=ORIENTED_EDGE ( 'NONE', *, *, #1948, .F. ) ;
#4142=PLANE ( 'NONE',  #39276 ) ;
#4143=LINE ( 'NONE', #30814, #42173 ) ;
#4144=ORIENTED_EDGE ( 'NONE', *, *, #12828, .T. ) ;
#4145=VECTOR ( 'NONE', #34317, 1000.000000000000114 ) ;
#4146=LINE ( 'NONE', #51819, #39771 ) ;
#4147=CARTESIAN_POINT ( 'NONE',  ( -14.69394934065806346, 0.1245042932765029059, 2.385588325215514782 ) ) ;
#4148=VECTOR ( 'NONE', #45780, 1000.000000000000227 ) ;
#4150=DIRECTION ( 'NONE',  ( 0.5449076811759707706, 0.6444004775717708799, -0.5364919789714476250 ) ) ;
#4152=AXIS2_PLACEMENT_3D ( 'NONE', #25449, #3591, #55543 ) ;
#4153=ORIENTED_EDGE ( 'NONE', *, *, #41885, .T. ) ;
#4154=VECTOR ( 'NONE', #7203, 1000.000000000000227 ) ;
#4155=ORIENTED_EDGE ( 'NONE', *, *, #51174, .T. ) ;
#4156=DIRECTION ( 'NONE',  ( -0.3620778797217457656, 0.000000000000000000, -0.9321478471874539151 ) ) ;
#4157=LINE ( 'NONE', #34516, #27716 ) ;
#4158=CARTESIAN_POINT ( 'NONE',  ( -17.87149280724919720, 0.000000000000000000, 6.158655315371090566 ) ) ;
#4159=DIRECTION ( 'NONE',  ( -0.6427681459581293666, -0.7660444431189770143, -0.005002170337467561935 ) ) ;
#4160=FACE_OUTER_BOUND ( 'NONE', #9057, .T. ) ;
#4161=CARTESIAN_POINT ( 'NONE',  ( -12.27153996272462955, 0.000000000000000000, 3.078252871230112486 ) ) ;
#4162=CARTESIAN_POINT ( 'NONE',  ( -12.23851102634202448, -0.1191753592594197858, 11.68427982808754884 ) ) ;
#4163=ORIENTED_EDGE ( 'NONE', *, *, #10390, .T. ) ;
#4165=DIRECTION ( 'NONE',  ( 0.005002170337468016433, -0.7660444431189770143, -0.6427681459581293666 ) ) ;
#4166=DIRECTION ( 'NONE',  ( 0.5364919789714477361, 0.6444004775717706579, 0.5449076811759711036 ) ) ;
#4168=ORIENTED_EDGE ( 'NONE', *, *, #10986, .F. ) ;
#4169=DIRECTION ( 'NONE',  ( 0.000000000000000000, -1.000000000000000000, 0.000000000000000000 ) ) ;
#4170=EDGE_LOOP ( 'NONE', ( #12133, #46183, #26468, #26256 ) ) ;
#4171=CARTESIAN_POINT ( 'NONE',  ( -7.081010562957787080, 4.806907600676791681, -0.4678686008800659324 ) ) ;
#4172=VECTOR ( 'NONE', #31383, 1000.000000000000227 ) ;
#4173=ORIENTED_EDGE ( 'NONE', *, *, #24544, .T. ) ;
#4174=ADVANCED_FACE ( 'NONE', ( #2581 ), #37807, .F. ) ;
#4175=VECTOR ( 'NONE', #52788, 999.9999999999998863 ) ;
#4176=ORIENTED_EDGE ( 'NONE', *, *, #15511, .T. ) ;
#4177=ORIENTED_EDGE ( 'NONE', *, *, #2682, .F. ) ;
#4178=VECTOR ( 'NONE', #21601, 999.9999999999998863 ) ;
#4179=ORIENTED_EDGE ( 'NONE', *, *, #24442, .F. ) ;
#4180=VECTOR ( 'NONE', #35081, 1000.000000000000227 ) ;
#4181=EDGE_LOOP ( 'NONE', ( #52548, #34976, #4615, #32027 ) ) ;
#4182=VERTEX_POINT ( 'NONE', #55967 ) ;
#4183=CARTESIAN_POINT ( 'NONE',  ( 3.882677180727608146, 0.000000000000000000, 1.710209902397122894 ) ) ;
#4184=AXIS2_PLACEMENT_3D ( 'NONE', #34248, #3292, #51552 ) ;
#4185=CARTESIAN_POINT ( 'NONE',  ( -14.62765668987744228, 0.000000000000000000, 7.291895807520449857 ) ) ;
#4186=FACE_OUTER_BOUND ( 'NONE', #40053, .T. ) ;
#4187=VECTOR ( 'NONE', #12397, 1000.000000000000227 ) ;
#4188=EDGE_CURVE ( 'NONE', #37711, #28907, #51425, .T. ) ;
#4189=AXIS2_PLACEMENT_3D ( 'NONE', #32343, #24085, #16125 ) ;
#4190=EDGE_LOOP ( 'NONE', ( #16548, #22768, #40044, #24905 ) ) ;
#4192=ORIENTED_EDGE ( 'NONE', *, *, #17150, .F. ) ;
#4193=DIRECTION ( 'NONE',  ( -0.6427681459581293666, -0.7660444431189770143, -0.005002170337467561935 ) ) ;
#4194=EDGE_CURVE ( 'NONE', #27982, #52283, #47730, .T. ) ;
#4196=EDGE_CURVE ( 'NONE', #30483, #51416, #8839, .T. ) ;
#4197=VECTOR ( 'NONE', #31560, 1000.000000000000227 ) ;
#4198=AXIS2_PLACEMENT_3D ( 'NONE', #18957, #12083, #21169 ) ;
#4199=LINE ( 'NONE', #34005, #19306 ) ;
#4200=CARTESIAN_POINT ( 'NONE',  ( -12.23851102634202448, -0.1191753592594197858, 11.68427982808754884 ) ) ;
#4201=DIRECTION ( 'NONE',  ( -0.005002170337468016433, -0.7660444431189770143, 0.6427681459581293666 ) ) ;
#4202=EDGE_CURVE ( 'NONE', #8687, #29343, #13073, .T. ) ;
#4203=ORIENTED_EDGE ( 'NONE', *, *, #14094, .F. ) ;
#4204=CARTESIAN_POINT ( 'NONE',  ( -18.39746900504187010, 0.000000000000000000, 14.03700784672088808 ) ) ;
#4205=ORIENTED_EDGE ( 'NONE', *, *, #53531, .T. ) ;
#4206=LINE ( 'NONE', #12447, #34604 ) ;
#4207=EDGE_CURVE ( 'NONE', #35585, #45114, #34378, .T. ) ;
#4208=DIRECTION ( 'NONE',  ( 0.005961354470445682716, -0.6427876096865404731, -0.7660212471507180654 ) ) ;
#4209=EDGE_CURVE ( 'NONE', #13117, #16694, #51682, .T. ) ;
#4210=VECTOR ( 'NONE', #1275, 999.9999999999998863 ) ;
#4211=LINE ( 'NONE', #16984, #21498 ) ;
#4212=DIRECTION ( 'NONE',  ( 0.005002170337468016433, -0.7660444431189770143, -0.6427681459581293666 ) ) ;
#4213=CARTESIAN_POINT ( 'NONE',  ( 2.072287782118878319, 0.000000000000000000, -2.950529333540147015 ) ) ;
#4214=DIRECTION ( 'NONE',  ( -0.9999697198139514409, -0.000000000000000000, -0.007781995580013368816 ) ) ;
#4215=CARTESIAN_POINT ( 'NONE',  ( -19.27115160478301803, 0.000000000000000000, 6.886426986582589116 ) ) ;
#4216=DIRECTION ( 'NONE',  ( 0.000000000000000000, -1.000000000000000000, 0.000000000000000000 ) ) ;
#4218=FACE_OUTER_BOUND ( 'NONE', #10818, .T. ) ;
#4220=VECTOR ( 'NONE', #583, 1000.000000000000227 ) ;
#4221=EDGE_CURVE ( 'NONE', #16268, #24035, #38920, .T. ) ;
#4223=DIRECTION ( 'NONE',  ( 0.7660212471507180654, -0.6427876096865404731, 0.005961354470445141482 ) ) ;
#4224=AXIS2_PLACEMENT_3D ( 'NONE', #3934, #11881, #35189 ) ;
#4225=CARTESIAN_POINT ( 'NONE',  ( 2.072287782118878319, 0.000000000000000000, -2.950529333540147015 ) ) ;
#4226=CARTESIAN_POINT ( 'NONE',  ( -10.00813838035478298, 0.000000000000000000, 10.77830692922518452 ) ) ;
#4227=DIRECTION ( 'NONE',  ( -0.5449076811759708816, 0.6444004775717707689, 0.5364919789714475140 ) ) ;
#4228=CARTESIAN_POINT ( 'NONE',  ( -6.007464458508009919, -5.767005180143939036, -0.8848703656275269669 ) ) ;
#4229=ADVANCED_FACE ( 'NONE', ( #30106 ), #47422, .F. ) ;
#4230=VECTOR ( 'NONE', #42195, 1000.000000000000227 ) ;
#4231=FACE_OUTER_BOUND ( 'NONE', #13736, .T. ) ;
#4232=ORIENTED_EDGE ( 'NONE', *, *, #27277, .T. ) ;
#4234=LINE ( 'NONE', #25243, #40348 ) ;
#4235=PLANE ( 'NONE',  #11878 ) ;
#4236=VECTOR ( 'NONE', #2238, 999.9999999999998863 ) ;
#4237=VECTOR ( 'NONE', #26254, 1000.000000000000000 ) ;
#4240=LINE ( 'NONE', #46825, #15051 ) ;
#4241=PLANE ( 'NONE',  #3875 ) ;
#4242=ORIENTED_EDGE ( 'NONE', *, *, #45670, .T. ) ;
#4243=VECTOR ( 'NONE', #24341, 1000.000000000000227 ) ;
#4244=AXIS2_PLACEMENT_3D ( 'NONE', #3773, #42968, #17395 ) ;
#4245=CARTESIAN_POINT ( 'NONE',  ( -11.62547109734172501, 0.000000000000000000, 5.468599160955688987 ) ) ;
#4247=ORIENTED_EDGE ( 'NONE', *, *, #33800, .T. ) ;
#4248=ORIENTED_EDGE ( 'NONE', *, *, #8217, .F. ) ;
#4249=CARTESIAN_POINT ( 'NONE',  ( -19.22961988024793101, -0.1191753592594177458, 14.39986392600063603 ) ) ;
#4250=ORIENTED_EDGE ( 'NONE', *, *, #53798, .F. ) ;
#4251=EDGE_CURVE ( 'NONE', #38604, #17725, #8243, .T. ) ;
#4252=AXIS2_PLACEMENT_3D ( 'NONE', #32134, #53987, #23599 ) ;
#4253=VERTEX_POINT ( 'NONE', #43195 ) ;
#4254=ORIENTED_EDGE ( 'NONE', *, *, #35222, .T. ) ;
#4255=ORIENTED_EDGE ( 'NONE', *, *, #23423, .F. ) ;
#4256=LINE ( 'NONE', #3402, #9402 ) ;
#4258=CARTESIAN_POINT ( 'NONE',  ( -17.41850097848045920, 3.362543313726510164, 3.340586309761012451 ) ) ;
#4259=FACE_OUTER_BOUND ( 'NONE', #15402, .T. ) ;
#4260=VECTOR ( 'NONE', #42754, 1000.000000000000227 ) ;
#4261=EDGE_LOOP ( 'NONE', ( #25981, #22306, #30077, #5804 ) ) ;
#4262=ORIENTED_EDGE ( 'NONE', *, *, #26618, .T. ) ;
#4263=EDGE_CURVE ( 'NONE', #44057, #46834, #3986, .T. ) ;
#4264=VECTOR ( 'NONE', #7782, 1000.000000000000227 ) ;
#4265=CARTESIAN_POINT ( 'NONE',  ( -19.60990026154428278, 0.000000000000000000, 4.498472333781370125 ) ) ;
#4266=ORIENTED_EDGE ( 'NONE', *, *, #54011, .F. ) ;
#4267=PLANE ( 'NONE',  #15519 ) ;
#4268=PLANE ( 'NONE',  #3240 ) ;
#4269=VERTEX_POINT ( 'NONE', #33439 ) ;
#4270=DIRECTION ( 'NONE',  ( 0.6427681459581294776, -0.7660444431189769032, 0.005002170337467562802 ) ) ;
#4271=ORIENTED_EDGE ( 'NONE', *, *, #6842, .F. ) ;
#4272=VECTOR ( 'NONE', #820, 999.9999999999998863 ) ;
#4273=DIRECTION ( 'NONE',  ( 0.000000000000000000, -0.000000000000000000, -1.000000000000000000 ) ) ;
#4275=EDGE_CURVE ( 'NONE', #8639, #947, #46467, .T. ) ;
#4276=CARTESIAN_POINT ( 'NONE',  ( -16.17376003385353300, -4.889348428825664783, 3.007762964104071735 ) ) ;
#4277=VECTOR ( 'NONE', #36690, 999.9999999999998863 ) ;
#4278=EDGE_LOOP ( 'NONE', ( #3722, #27860, #49278, #43043 ) ) ;
#4279=LINE ( 'NONE', #51937, #10421 ) ;
#4280=DIRECTION ( 'NONE',  ( -0.005002170337468016433, -0.7660444431189770143, 0.6427681459581293666 ) ) ;
#4281=CARTESIAN_POINT ( 'NONE',  ( -17.69604769044466863, 0.000000000000000000, 9.314683284511998451 ) ) ;
#4282=LINE ( 'NONE', #52516, #43719 ) ;
#4284=EDGE_CURVE ( 'NONE', #6902, #6537, #34290, .T. ) ;
#4285=CARTESIAN_POINT ( 'NONE',  ( 2.072287782118878319, 0.000000000000000000, -2.950529333540147015 ) ) ;
#4286=DIRECTION ( 'NONE',  ( -0.7660212471507179544, -0.6427876096865405842, -0.005961354470445141482 ) ) ;
#4287=CARTESIAN_POINT ( 'NONE',  ( -29.86197018149027116, 0.000000000000000000, 8.281335066757780083 ) ) ;
#4288=DIRECTION ( 'NONE',  ( 0.000000000000000000, -1.000000000000000000, 0.000000000000000000 ) ) ;
#4289=LINE ( 'NONE', #17308, #27773 ) ;
#4290=CARTESIAN_POINT ( 'NONE',  ( -15.38203175034444747, 4.819660872929013351, 2.503062823780374924 ) ) ;
#4291=PLANE ( 'NONE',  #47915 ) ;
#4292=EDGE_CURVE ( 'NONE', #35264, #24902, #50743, .T. ) ;
#4293=CARTESIAN_POINT ( 'NONE',  ( -16.50057454476819885, 0.000000000000000000, 9.123980676737234674 ) ) ;
#4294=CARTESIAN_POINT ( 'NONE',  ( -9.808144436391993182, 0.000000000000000000, 10.77986332834118777 ) ) ;
#4295=EDGE_LOOP ( 'NONE', ( #23358, #5510, #1944, #12764 ) ) ;
#4296=CARTESIAN_POINT ( 'NONE',  ( -18.29747203306047609, -0.1191753592594177458, 14.03778604627889059 ) ) ;
#4297=ORIENTED_EDGE ( 'NONE', *, *, #7814, .F. ) ;
#4298=FACE_OUTER_BOUND ( 'NONE', #19361, .T. ) ;
#4299=LINE ( 'NONE', #14225, #3729 ) ;
#4301=FACE_OUTER_BOUND ( 'NONE', #19185, .T. ) ;
#4302=PLANE ( 'NONE',  #36910 ) ;
#4303=CARTESIAN_POINT ( 'NONE',  ( -25.20278734466900517, 0.000000000000000000, 6.670939612111840944 ) ) ;
#4304=ORIENTED_EDGE ( 'NONE', *, *, #17856, .T. ) ;
#4305=VECTOR ( 'NONE', #12404, 1000.000000000000227 ) ;
#4306=ORIENTED_EDGE ( 'NONE', *, *, #29314, .T. ) ;
#4307=CARTESIAN_POINT ( 'NONE',  ( -17.73140113748535285, 0.000000000000000000, 13.85752530597602039 ) ) ;
#4308=DIRECTION ( 'NONE',  ( -0.6427681459581293666, -0.7660444431189770143, -0.005002170337467561935 ) ) ;
#4309=VERTEX_POINT ( 'NONE', #7899 ) ;
#4310=ADVANCED_FACE ( 'NONE', ( #25211 ), #7049, .F. ) ;
#4311=PLANE ( 'NONE',  #25684 ) ;
#4312=VECTOR ( 'NONE', #39628, 1000.000000000000114 ) ;
#4313=EDGE_LOOP ( 'NONE', ( #49019, #12159, #54261, #55365, #15419 ) ) ;
#4314=PLANE ( 'NONE',  #11347 ) ;
#4315=ADVANCED_FACE ( 'NONE', ( #45941 ), #16373, .F. ) ;
#4316=ORIENTED_EDGE ( 'NONE', *, *, #45969, .F. ) ;
#4317=DIRECTION ( 'NONE',  ( -0.9999697198139514409, -0.000000000000000000, -0.007781995580013368816 ) ) ;
#4318=ORIENTED_EDGE ( 'NONE', *, *, #4451, .T. ) ;
#4319=ORIENTED_EDGE ( 'NONE', *, *, #529, .T. ) ;
#4320=ORIENTED_EDGE ( 'NONE', *, *, #31957, .F. ) ;
#4321=ADVANCED_FACE ( 'NONE', ( #29155 ), #47055, .F. ) ;
#4322=CARTESIAN_POINT ( 'NONE',  ( -15.07660566480283748, 0.000000000000000000, 5.272415620168643180 ) ) ;
#4323=DIRECTION ( 'NONE',  ( 0.005002170337468016433, -0.7660444431189770143, -0.6427681459581293666 ) ) ;
#4324=CARTESIAN_POINT ( 'NONE',  ( -12.13851405436063047, 0.000000000000000000, 11.68505802764555135 ) ) ;
#4325=EDGE_CURVE ( 'NONE', #43270, #32747, #21206, .T. ) ;
#4326=EDGE_CURVE ( 'NONE', #33148, #46628, #33699, .T. ) ;
#4327=EDGE_CURVE ( 'NONE', #21477, #9006, #28899, .T. ) ;
#4328=CARTESIAN_POINT ( 'NONE',  ( 2.072287782118878319, 0.000000000000000000, -2.950529333540147015 ) ) ;
#4329=EDGE_LOOP ( 'NONE', ( #27371, #12486, #40200, #8277 ) ) ;
#4330=ORIENTED_EDGE ( 'NONE', *, *, #42708, .T. ) ;
#4331=ORIENTED_EDGE ( 'NONE', *, *, #13855, .T. ) ;
#4332=PLANE ( 'NONE',  #46684 ) ;
#4333=ORIENTED_EDGE ( 'NONE', *, *, #12165, .T. ) ;
#4334=PLANE ( 'NONE',  #11198 ) ;
#4335=EDGE_LOOP ( 'NONE', ( #43770, #37186, #35086, #8647 ) ) ;
#4336=DIRECTION ( 'NONE',  ( -0.005961354470445682716, -0.6427876096865404731, 0.7660212471507180654 ) ) ;
#4337=CARTESIAN_POINT ( 'NONE',  ( -11.36370219796871339, 0.000000000000000000, 5.839968376865459554 ) ) ;
#4338=ORIENTED_EDGE ( 'NONE', *, *, #6358, .T. ) ;
#4339=PLANE ( 'NONE',  #51266 ) ;
#4340=ADVANCED_FACE ( 'NONE', ( #7297 ), #25467, .F. ) ;
#4341=ORIENTED_EDGE ( 'NONE', *, *, #47393, .T. ) ;
#4342=EDGE_CURVE ( 'NONE', #18162, #17751, #2741, .T. ) ;
#4343=VECTOR ( 'NONE', #9043, 1000.000000000000114 ) ;
#4344=CARTESIAN_POINT ( 'NONE',  ( -11.40636015113596180, 0.000000000000000000, 11.32142374880780089 ) ) ;
#4346=FACE_OUTER_BOUND ( 'NONE', #23649, .T. ) ;
#4347=FACE_OUTER_BOUND ( 'NONE', #48451, .T. ) ;
#4348=EDGE_CURVE ( 'NONE', #42292, #36024, #33165, .T. ) ;
#4349=DIRECTION ( 'NONE',  ( -0.005002170337468016433, -0.7660444431189770143, 0.6427681459581293666 ) ) ;
#4350=ORIENTED_EDGE ( 'NONE', *, *, #40743, .T. ) ;
#4351=LINE ( 'NONE', #25929, #40163 ) ;
#4352=ADVANCED_FACE ( 'NONE', ( #41928 ), #3030, .F. ) ;
#4353=VECTOR ( 'NONE', #8603, 1000.000000000000114 ) ;
#4355=PLANE ( 'NONE',  #54810 ) ;
#4356=DIRECTION ( 'NONE',  ( 0.5449076811759707706, 0.6444004775717708799, -0.5364919789714476250 ) ) ;
#4357=LINE ( 'NONE', #21665, #19492 ) ;
#4358=ADVANCED_FACE ( 'NONE', ( #22553 ), #48676, .F. ) ;
#4359=CARTESIAN_POINT ( 'NONE',  ( -15.82732154344847864, 0.000000000000000000, 8.021223877847955208 ) ) ;
#4361=CARTESIAN_POINT ( 'NONE',  ( -10.70350180978612542, 0.000000000000000000, 6.414444334970025530 ) ) ;
#4362=PLANE ( 'NONE',  #42202 ) ;
#4363=DIRECTION ( 'NONE',  ( 0.007781995580012663651, 0.000000000000000000, -0.9999697198139515519 ) ) ;
#4364=ORIENTED_EDGE ( 'NONE', *, *, #34202, .F. ) ;
#4365=CARTESIAN_POINT ( 'NONE',  ( -15.45771171113622167, -0.1191753592594177180, 7.385439155523823906 ) ) ;
#4366=CARTESIAN_POINT ( 'NONE',  ( -17.73140113748535285, 0.000000000000000000, 13.85752530597602039 ) ) ;
#4367=ORIENTED_EDGE ( 'NONE', *, *, #16453, .F. ) ;
#4369=DIRECTION ( 'NONE',  ( -0.6427681459581293666, -0.7660444431189770143, -0.005002170337467561935 ) ) ;
#4370=CARTESIAN_POINT ( 'NONE',  ( -14.93495759592298988, 0.000000000000000000, 12.77129166681078409 ) ) ;
#4372=ORIENTED_EDGE ( 'NONE', *, *, #55975, .T. ) ;
#4373=ORIENTED_EDGE ( 'NONE', *, *, #548, .F. ) ;
#4374=LINE ( 'NONE', #9755, #42106 ) ;
#4375=CARTESIAN_POINT ( 'NONE',  ( -10.19707176475507815, 0.000000000000000000, 1.047730457166543783 ) ) ;
#4376=CARTESIAN_POINT ( 'NONE',  ( -13.27065584551087163, 0.000000000000000000, 12.04557950825129176 ) ) ;
#4377=DIRECTION ( 'NONE',  ( 0.6427681459581294776, -0.7660444431189769032, 0.005002170337467562802 ) ) ;
#4378=DIRECTION ( 'NONE',  ( 0.5364919789714477361, 0.6444004775717706579, 0.5449076811759711036 ) ) ;
#4379=PLANE ( 'NONE',  #43056 ) ;
#4380=ORIENTED_EDGE ( 'NONE', *, *, #5523, .T. ) ;
#4381=DIRECTION ( 'NONE',  ( -0.6427681459581293666, -0.7660444431189770143, -0.005002170337467561935 ) ) ;
#4383=EDGE_LOOP ( 'NONE', ( #29653, #51259, #50694, #43168 ) ) ;
#4384=LINE ( 'NONE', #26494, #14761 ) ;
#4385=DIRECTION ( 'NONE',  ( -0.7660212471507179544, -0.6427876096865405842, -0.005961354470445141482 ) ) ;
#4386=CARTESIAN_POINT ( 'NONE',  ( -13.63673279712320507, -0.1191753592594197858, 12.22739664767016521 ) ) ;
#4387=EDGE_CURVE ( 'NONE', #36809, #37046, #1781, .T. ) ;
#4388=EDGE_CURVE ( 'NONE', #36400, #44385, #942, .T. ) ;
#4389=EDGE_LOOP ( 'NONE', ( #6909, #4179, #56103, #38966 ) ) ;
#4390=AXIS2_PLACEMENT_3D ( 'NONE', #31082, #40741, #22845 ) ;
#4391=CYLINDRICAL_SURFACE ( 'NONE', #27582, 2.125000000000000000 ) ;
#4392=ORIENTED_EDGE ( 'NONE', *, *, #44249, .T. ) ;
#4393=EDGE_CURVE ( 'NONE', #1220, #41647, #35599, .T. ) ;
#4394=ORIENTED_EDGE ( 'NONE', *, *, #28199, .T. ) ;
#4395=EDGE_LOOP ( 'NONE', ( #35165, #27222, #49716, #38811 ) ) ;
#4396=EDGE_LOOP ( 'NONE', ( #3514, #52501, #14243, #7609 ) ) ;
#4397=FACE_OUTER_BOUND ( 'NONE', #3040, .T. ) ;
#4398=ORIENTED_EDGE ( 'NONE', *, *, #1711, .T. ) ;
#4400=ORIENTED_EDGE ( 'NONE', *, *, #23595, .F. ) ;
#4401=CARTESIAN_POINT ( 'NONE',  ( -29.86274838104827367, -0.1191753592594197858, 8.381332038739175871 ) ) ;
#4402=VERTEX_POINT ( 'NONE', #44395 ) ;
#4403=DIRECTION ( 'NONE',  ( 0.7660212471507180654, -0.6427876096865404731, 0.005961354470445141482 ) ) ;
#4405=ADVANCED_FACE ( 'NONE', ( #36429 ), #18857, .F. ) ;
#4406=CARTESIAN_POINT ( 'NONE',  ( -4.592488342126416434, 4.500757451777032792, 5.002252009306281444 ) ) ;
#4408=CARTESIAN_POINT ( 'NONE',  ( -14.94916102560700821, 0.000000000000000000, 2.688082935172642962 ) ) ;
#4409=FACE_OUTER_BOUND ( 'NONE', #32469, .T. ) ;
#4410=PLANE ( 'NONE',  #29607 ) ;
#4411=DIRECTION ( 'NONE',  ( 0.7660212471507180654, -0.6427876096865404731, 0.005961354470445141482 ) ) ;
#4412=ORIENTED_EDGE ( 'NONE', *, *, #47711, .T. ) ;
#4413=ADVANCED_FACE ( 'NONE', ( #53480 ), #53225, .F. ) ;
#4414=ORIENTED_EDGE ( 'NONE', *, *, #32772, .T. ) ;
#4415=CARTESIAN_POINT ( 'NONE',  ( -13.49994535134848661, 0.000000000000000000, 7.500677974135260939 ) ) ;
#4416=DIRECTION ( 'NONE',  ( 0.7660212471507180654, -0.6427876096865404731, 0.005961354470445141482 ) ) ;
#4417=ADVANCED_FACE ( 'NONE', ( #14580 ), #34546, .F. ) ;
#4418=LINE ( 'NONE', #47009, #16994 ) ;
#4419=CARTESIAN_POINT ( 'NONE',  ( -11.40636015113596180, 0.000000000000000000, 11.32142374880780089 ) ) ;
#4420=ADVANCED_FACE ( 'NONE', ( #22813 ), #40132, .F. ) ;
#4421=CARTESIAN_POINT ( 'NONE',  ( -1.086233639165236964, 0.000000000000000000, -2.796443541562362078 ) ) ;
#4422=FACE_OUTER_BOUND ( 'NONE', #25383, .T. ) ;
#4423=ORIENTED_EDGE ( 'NONE', *, *, #319, .F. ) ;
#4424=CARTESIAN_POINT ( 'NONE',  ( -19.21524870871409618, -0.1941918491731548790, 4.464488790411954788 ) ) ;
#4425=EDGE_CURVE ( 'NONE', #48142, #48104, #31638, .T. ) ;
#4426=LINE ( 'NONE', #51557, #26778 ) ;
#4427=ORIENTED_EDGE ( 'NONE', *, *, #10218, .T. ) ;
#4428=VECTOR ( 'NONE', #18508, 1000.000000000000227 ) ;
#4429=CARTESIAN_POINT ( 'NONE',  ( -16.02156738040070394, 0.000000000000000000, 7.281048072216421474 ) ) ;
#4430=CARTESIAN_POINT ( 'NONE',  ( -13.47252247068494135, 0.000000000000000000, 3.976896700852591948 ) ) ;
#4431=ADVANCED_FACE ( 'NONE', ( #27347 ), #26806, .F. ) ;
#4432=PLANE ( 'NONE',  #34097 ) ;
#4433=CARTESIAN_POINT ( 'NONE',  ( -27.99767448711536133, 0.000000000000000000, 7.557179307314289218 ) ) ;
#4434=CARTESIAN_POINT ( 'NONE',  ( -21.47263955680318404, 0.000000000000000000, 5.022634149262071190 ) ) ;
#4435=ORIENTED_EDGE ( 'NONE', *, *, #37563, .F. ) ;
#4436=ORIENTED_EDGE ( 'NONE', *, *, #42302, .F. ) ;
#4437=DIRECTION ( 'NONE',  ( 0.000000000000000000, -1.000000000000000000, 0.000000000000000000 ) ) ;
#4438=DIRECTION ( 'NONE',  ( 0.005002170337468016433, -0.7660444431189770143, -0.6427681459581293666 ) ) ;
#4439=PLANE ( 'NONE',  #19732 ) ;
#4440=LINE ( 'NONE', #22322, #25525 ) ;
#4441=LINE ( 'NONE', #43881, #55690 ) ;
#4442=DIRECTION ( 'NONE',  ( -0.5449076811759708816, 0.6444004775717707689, 0.5364919789714475140 ) ) ;
#4443=DIRECTION ( 'NONE',  ( 0.7660212471507180654, -0.6427876096865404731, 0.005961354470445141482 ) ) ;
#4444=ORIENTED_EDGE ( 'NONE', *, *, #29952, .T. ) ;
#4445=DIRECTION ( 'NONE',  ( 0.9999697198139515519, 0.000000000000000000, 0.007781995580013368816 ) ) ;
#4446=CARTESIAN_POINT ( 'NONE',  ( 2.072287782118878319, 0.000000000000000000, -2.950529333540147015 ) ) ;
#4447=ORIENTED_EDGE ( 'NONE', *, *, #27977, .T. ) ;
#4448=DIRECTION ( 'NONE',  ( -0.005961354470445682716, -0.6427876096865404731, 0.7660212471507180654 ) ) ;
#4449=VERTEX_POINT ( 'NONE', #10326 ) ;
#4450=FACE_OUTER_BOUND ( 'NONE', #17507, .T. ) ;
#4451=EDGE_CURVE ( 'NONE', #24292, #14805, #51860, .T. ) ;
#4452=ORIENTED_EDGE ( 'NONE', *, *, #23447, .F. ) ;
#4453=ORIENTED_EDGE ( 'NONE', *, *, #38327, .T. ) ;
#4456=EDGE_CURVE ( 'NONE', #45853, #47084, #13729, .T. ) ;
#4457=EDGE_LOOP ( 'NONE', ( #9913, #22248, #14318, #18600 ) ) ;
#4458=EDGE_LOOP ( 'NONE', ( #4807, #41929, #53330, #20915 ) ) ;
#4459=ORIENTED_EDGE ( 'NONE', *, *, #37806, .T. ) ;
#4460=ORIENTED_EDGE ( 'NONE', *, *, #9376, .F. ) ;
#4461=DIRECTION ( 'NONE',  ( 0.007781995580012663651, 0.000000000000000000, -0.9999697198139515519 ) ) ;
#4462=PLANE ( 'NONE',  #27492 ) ;
#4463=FACE_OUTER_BOUND ( 'NONE', #9263, .T. ) ;
#4464=EDGE_LOOP ( 'NONE', ( #14186, #33756, #40060, #26649 ) ) ;
#4465=LINE ( 'NONE', #30601, #33098 ) ;
#4466=VERTEX_POINT ( 'NONE', #38830 ) ;
#4467=ORIENTED_EDGE ( 'NONE', *, *, #6960, .T. ) ;
#4468=EDGE_CURVE ( 'NONE', #52808, #46492, #1223, .T. ) ;
#4469=CARTESIAN_POINT ( 'NONE',  ( -21.47341775636118655, -0.1191753592594197858, 5.122631121243466090 ) ) ;
#4470=PLANE ( 'NONE',  #18701 ) ;
#4471=ORIENTED_EDGE ( 'NONE', *, *, #8942, .T. ) ;
#4472=DIRECTION ( 'NONE',  ( 0.005002170337468016433, -0.7660444431189770143, -0.6427681459581293666 ) ) ;
#4473=ORIENTED_EDGE ( 'NONE', *, *, #7377, .T. ) ;
#4474=DIRECTION ( 'NONE',  ( 0.007781995580012663651, -3.146120232559066537E-19, -0.9999697198139514409 ) ) ;
#4475=CARTESIAN_POINT ( 'NONE',  ( -24.26908309836554878, 0.000000000000000000, 6.108867788427308376 ) ) ;
#4477=CARTESIAN_POINT ( 'NONE',  ( -15.60102546347950536, 0.000000000000000000, 12.95077420755565356 ) ) ;
#4478=PLANE ( 'NONE',  #473 ) ;
#4479=CARTESIAN_POINT ( 'NONE',  ( -27.99845268667336384, -0.1191753592594197858, 7.657176279295684118 ) ) ;
#4480=EDGE_CURVE ( 'NONE', #24312, #13470, #41539, .T. ) ;
#4481=CARTESIAN_POINT ( 'NONE',  ( -19.24620501330758060, -0.1191753592594167188, 8.094620364256195799 ) ) ;
#4482=DIRECTION ( 'NONE',  ( -0.9999697198139514409, -0.000000000000000000, -0.007781995580013368816 ) ) ;
#4486=CARTESIAN_POINT ( 'NONE',  ( -11.37519841198984416, 0.000000000000000000, 7.317207189896516972 ) ) ;
#4488=FACE_OUTER_BOUND ( 'NONE', #32078, .T. ) ;
#4489=EDGE_CURVE ( 'NONE', #25204, #52744, #41793, .T. ) ;
#4491=CARTESIAN_POINT ( 'NONE',  ( -13.01231602646514141, 0.000000000000000000, 4.549816259841156452 ) ) ;
#4492=DIRECTION ( 'NONE',  ( 0.5364919789714477361, 0.6444004775717706579, 0.5449076811759711036 ) ) ;
#4493=CARTESIAN_POINT ( 'NONE',  ( -16.29064078590028330, 0.000000000000000000, 7.848292206784967640 ) ) ;
#4497=DIRECTION ( 'NONE',  ( 0.007781995580012663651, -3.146120232559066537E-19, -0.9999697198139514409 ) ) ;
#4498=CARTESIAN_POINT ( 'NONE',  ( -16.81190032086591302, 0.000000000000000000, 3.212244750653343583 ) ) ;
#4500=LINE ( 'NONE', #39716, #29131 ) ;
#4501=LINE ( 'NONE', #17008, #4865 ) ;
#4502=CARTESIAN_POINT ( 'NONE',  ( -13.73672976910459909, 0.000000000000000000, 12.22661844811216270 ) ) ;
#4503=ADVANCED_FACE ( 'NONE', ( #46326 ), #24477, .F. ) ;
#4504=DIRECTION ( 'NONE',  ( 0.9999697198139515519, 0.000000000000000000, 0.007781995580013368816 ) ) ;
#4505=CARTESIAN_POINT ( 'NONE',  ( 2.072287782118878319, 0.000000000000000000, -2.950529333540147015 ) ) ;
#4507=VERTEX_POINT ( 'NONE', #32476 ) ;
#4508=CARTESIAN_POINT ( 'NONE',  ( -13.33515596948987714, 1.257817950434005461, 4.125442103548757622 ) ) ;
#4509=ADVANCED_FACE ( 'NONE', ( #45788 ), #37263, .F. ) ;
#4510=ORIENTED_EDGE ( 'NONE', *, *, #12597, .F. ) ;
#4512=EDGE_CURVE ( 'NONE', #10554, #46790, #50618, .T. ) ;
#4513=ORIENTED_EDGE ( 'NONE', *, *, #1785, .F. ) ;
#4514=ORIENTED_EDGE ( 'NONE', *, *, #2638, .T. ) ;
#4515=ORIENTED_EDGE ( 'NONE', *, *, #24498, .T. ) ;
#4516=ORIENTED_EDGE ( 'NONE', *, *, #46167, .F. ) ;
#4517=FACE_OUTER_BOUND ( 'NONE', #37004, .T. ) ;
#4518=CARTESIAN_POINT ( 'NONE',  ( -16.81345671998191449, 0.000000000000000000, 3.412238694616132495 ) ) ;
#4519=EDGE_CURVE ( 'NONE', #8314, #46588, #37548, .T. ) ;
#4520=EDGE_CURVE ( 'NONE', #5827, #38038, #10873, .T. ) ;
#4521=ORIENTED_EDGE ( 'NONE', *, *, #53652, .F. ) ;
#4522=EDGE_CURVE ( 'NONE', #53284, #31756, #7439, .T. ) ;
#4523=DIRECTION ( 'NONE',  ( -0.6427681459581293666, -0.7660444431189770143, -0.005002170337467561935 ) ) ;
#4524=EDGE_LOOP ( 'NONE', ( #35276, #1445, #55737, #37988 ) ) ;
#4525=DIRECTION ( 'NONE',  ( 0.000000000000000000, -0.000000000000000000, -1.000000000000000000 ) ) ;
#4526=DIRECTION ( 'NONE',  ( -0.9999697198139514409, -0.000000000000000000, -0.007781995580013368816 ) ) ;
#4527=ORIENTED_EDGE ( 'NONE', *, *, #22969, .F. ) ;
#4528=FACE_OUTER_BOUND ( 'NONE', #15448, .T. ) ;
#4530=DIRECTION ( 'NONE',  ( -0.6427681459581293666, -0.7660444431189770143, -0.005002170337467561935 ) ) ;
#4531=DIRECTION ( 'NONE',  ( 0.007781995580012662783, 0.000000000000000000, -0.9999697198139514409 ) ) ;
#4532=EDGE_LOOP ( 'NONE', ( #16575, #23388, #20917, #37832 ) ) ;
#4533=DIRECTION ( 'NONE',  ( 0.007781995580012663651, -3.146120232559066537E-19, -0.9999697198139514409 ) ) ;
#4534=CARTESIAN_POINT ( 'NONE',  ( -27.06708303904391144, 0.000000000000000000, 7.395095371555332697 ) ) ;
#4535=DIRECTION ( 'NONE',  ( -0.9321478471874540261, 0.000000000000000000, 0.3620778797217457656 ) ) ;
#4536=EDGE_LOOP ( 'NONE', ( #47272, #38177, #28158, #5649 ) ) ;
#4539=LINE ( 'NONE', #47413, #52807 ) ;
#4540=DIRECTION ( 'NONE',  ( -0.005961354470445682716, -0.6427876096865404731, 0.7660212471507180654 ) ) ;
#4541=CARTESIAN_POINT ( 'NONE',  ( -27.99767448711536133, 0.000000000000000000, 7.557179307314289218 ) ) ;
#4542=PLANE ( 'NONE',  #12371 ) ;
#4544=LINE ( 'NONE', #29839, #39521 ) ;
#4545=DIRECTION ( 'NONE',  ( 0.8531650599175527594, 0.4028455766673922356, -0.3313982828793700652 ) ) ;
#4546=PLANE ( 'NONE',  #25258 ) ;
#4547=CARTESIAN_POINT ( 'NONE',  ( -13.25978161800689747, 1.743523803501506375, 1.776853678323026431 ) ) ;
#4548=CARTESIAN_POINT ( 'NONE',  ( -10.74029228357944987, 0.000000000000000000, 11.14194120806293320 ) ) ;
#4549=DIRECTION ( 'NONE',  ( 0.9999697198139515519, 0.000000000000000000, 0.007781995580013368816 ) ) ;
#4550=EDGE_LOOP ( 'NONE', ( #55627, #25518, #33804, #3183 ) ) ;
#4551=CARTESIAN_POINT ( 'NONE',  ( -20.54204810873173415, 0.000000000000000000, 4.860550213503115558 ) ) ;
#4552=FACE_OUTER_BOUND ( 'NONE', #4108, .T. ) ;
#4553=DIRECTION ( 'NONE',  ( -0.005002170337468016433, -0.7660444431189770143, 0.6427681459581293666 ) ) ;
#4554=ADVANCED_FACE ( 'NONE', ( #20522 ), #32721, .F. ) ;
#4556=EDGE_CURVE ( 'NONE', #55970, #15628, #40965, .T. ) ;
#4557=DIRECTION ( 'NONE',  ( 0.005002170337468016433, -0.7660444431189770143, -0.6427681459581293666 ) ) ;
#4558=ADVANCED_FACE ( 'NONE', ( #28768 ), #41260, .F. ) ;
#4559=DIRECTION ( 'NONE',  ( -0.5364919789714478471, 0.6444004775717705469, -0.5449076811759709926 ) ) ;
#4560=ORIENTED_EDGE ( 'NONE', *, *, #55040, .F. ) ;
#4561=VECTOR ( 'NONE', #52467, 999.9999999999998863 ) ;
#4562=ORIENTED_EDGE ( 'NONE', *, *, #21166, .F. ) ;
#4563=LINE ( 'NONE', #39195, #29535 ) ;
#4564=LINE ( 'NONE', #25040, #4120 ) ;
#4565=EDGE_LOOP ( 'NONE', ( #19931, #23706, #10728, #20773 ) ) ;
#4566=CARTESIAN_POINT ( 'NONE',  ( -10.27421835998572064, 0.000000000000000000, 10.96090226820206048 ) ) ;
#4567=ORIENTED_EDGE ( 'NONE', *, *, #37915, .F. ) ;
#4568=EDGE_CURVE ( 'NONE', #40584, #5725, #19387, .T. ) ;
#4569=DIRECTION ( 'NONE',  ( 0.007781995580012662783, 0.000000000000000000, -0.9999697198139514409 ) ) ;
#4570=VERTEX_POINT ( 'NONE', #50028 ) ;
#4571=CARTESIAN_POINT ( 'NONE',  ( -12.97282572840506276, 4.172053068839010947, 1.587907467427786878 ) ) ;
#4572=EDGE_CURVE ( 'NONE', #45990, #32478, #33012, .T. ) ;
#4573=ORIENTED_EDGE ( 'NONE', *, *, #4877, .T. ) ;
#4574=ORIENTED_EDGE ( 'NONE', *, *, #9358, .F. ) ;
#4575=VERTEX_POINT ( 'NONE', #11140 ) ;
#4576=CARTESIAN_POINT ( 'NONE',  ( -17.26532721389163072, 0.000000000000000000, 13.67648636611514590 ) ) ;
#4577=DIRECTION ( 'NONE',  ( 0.000000000000000000, -1.000000000000000000, 0.000000000000000000 ) ) ;
#4578=FACE_OUTER_BOUND ( 'NONE', #47962, .T. ) ;
#4579=EDGE_CURVE ( 'NONE', #35206, #4870, #46073, .T. ) ;
#4580=DIRECTION ( 'NONE',  ( 0.6427681459581294776, -0.7660444431189769032, 0.005002170337467562802 ) ) ;
#4581=ORIENTED_EDGE ( 'NONE', *, *, #27597, .T. ) ;
#4582=ORIENTED_EDGE ( 'NONE', *, *, #53363, .T. ) ;
#4583=ADVANCED_FACE ( 'NONE', ( #37614 ), #28529, .F. ) ;
#4584=ORIENTED_EDGE ( 'NONE', *, *, #9060, .T. ) ;
#4585=DIRECTION ( 'NONE',  ( -0.6427681459581293666, -0.7660444431189770143, -0.005002170337467561935 ) ) ;
#4586=VERTEX_POINT ( 'NONE', #42152 ) ;
#4587=LINE ( 'NONE', #16515, #28420 ) ;
#4588=ORIENTED_EDGE ( 'NONE', *, *, #12266, .F. ) ;
#4589=DIRECTION ( 'NONE',  ( 0.6427681459581294776, -0.7660444431189769032, 0.005002170337467562802 ) ) ;
#4590=CARTESIAN_POINT ( 'NONE',  ( -10.80559463571480450, -0.1191753592594190225, 6.682978866688390696 ) ) ;
#4591=VERTEX_POINT ( 'NONE', #32784 ) ;
#4592=CARTESIAN_POINT ( 'NONE',  ( -13.20787951780664393, 0.000000000000000000, 3.978956213504597272 ) ) ;
#4593=VERTEX_POINT ( 'NONE', #50093 ) ;
#4594=VECTOR ( 'NONE', #31004, 999.9999999999998863 ) ;
#4596=VERTEX_POINT ( 'NONE', #54940 ) ;
#4597=CARTESIAN_POINT ( 'NONE',  ( 2.072287782118878319, 0.000000000000000000, -2.950529333540147015 ) ) ;
#4598=CARTESIAN_POINT ( 'NONE',  ( -11.36813265058999889, 0.000000000000000000, 6.409272024086013708 ) ) ;
#4599=DIRECTION ( 'NONE',  ( -0.005002170337468016433, -0.7660444431189770143, 0.6427681459581293666 ) ) ;
#4600=EDGE_LOOP ( 'NONE', ( #20810, #41303, #5689, #28557 ) ) ;
#4601=DIRECTION ( 'NONE',  ( 0.5449076811759707706, 0.6444004775717708799, -0.5364919789714476250 ) ) ;
#4602=DIRECTION ( 'NONE',  ( 0.000000000000000000, -1.000000000000000000, 0.000000000000000000 ) ) ;
#4603=CARTESIAN_POINT ( 'NONE',  ( -10.36412444188097837, -0.03739765774599676518, 0.8457230899663811252 ) ) ;
#4604=EDGE_CURVE ( 'NONE', #40212, #48365, #46128, .T. ) ;
#4605=LINE ( 'NONE', #48047, #35925 ) ;
#4606=CARTESIAN_POINT ( 'NONE',  ( 2.072287782118878319, 0.000000000000000000, -2.950529333540147015 ) ) ;
#4607=DIRECTION ( 'NONE',  ( 0.007781995580012662783, 0.000000000000000000, -0.9999697198139514409 ) ) ;
#4608=EDGE_CURVE ( 'NONE', #49012, #1661, #2674, .T. ) ;
#4609=FILL_AREA_STYLE ('',( #48050 ) ) ;
#4610=EDGE_LOOP ( 'NONE', ( #6702, #32543, #4812, #11437 ) ) ;
#4611=CARTESIAN_POINT ( 'NONE',  ( -9.342070512798265725, 0.000000000000000000, 10.59882438848031505 ) ) ;
#4612=ADVANCED_FACE ( 'NONE', ( #45854 ), #11204, .F. ) ;
#4613=CARTESIAN_POINT ( 'NONE',  ( -21.47419595591918906, 0.000000000000000000, 5.222628093224860102 ) ) ;
#4614=CARTESIAN_POINT ( 'NONE',  ( -10.68913154225971418, 0.000000000000000000, 4.567895818681203757 ) ) ;
#4615=ORIENTED_EDGE ( 'NONE', *, *, #44256, .T. ) ;
#4616=DIRECTION ( 'NONE',  ( 0.007781995580012663651, -3.146120232559066537E-19, -0.9999697198139514409 ) ) ;
#4618=EDGE_LOOP ( 'NONE', ( #48224, #4467, #25533, #11808, #50889 ) ) ;
#4619=EDGE_CURVE ( 'NONE', #27886, #21134, #6977, .T. ) ;
#4620=EDGE_CURVE ( 'NONE', #34091, #12500, #2948, .T. ) ;
#4621=ADVANCED_FACE ( 'NONE', ( #2416 ), #7504, .F. ) ;
#4622=CARTESIAN_POINT ( 'NONE',  ( -16.47183400971537282, 0.000000000000000000, 5.430883644159590240 ) ) ;
#4623=VECTOR ( 'NONE', #33418, 1000.000000000000227 ) ;
#4624=DIRECTION ( 'NONE',  ( 0.000000000000000000, -0.000000000000000000, -1.000000000000000000 ) ) ;
#4625=FACE_OUTER_BOUND ( 'NONE', #36330, .T. ) ;
#4626=DIRECTION ( 'NONE',  ( 0.000000000000000000, -1.000000000000000000, 0.000000000000000000 ) ) ;
#4627=ORIENTED_EDGE ( 'NONE', *, *, #19660, .T. ) ;
#4631=DIRECTION ( 'NONE',  ( 0.5364919789714477361, 0.6444004775717706579, 0.5449076811759711036 ) ) ;
#4632=CARTESIAN_POINT ( 'NONE',  ( -16.53317331066696383, 0.000000000000000000, 13.31285208727739899 ) ) ;
#4633=LINE ( 'NONE', #17704, #42784 ) ;
#4634=VECTOR ( 'NONE', #27506, 1000.000000000000000 ) ;
#4635=EDGE_CURVE ( 'NONE', #3505, #30167, #37904, .T. ) ;
#4636=PLANE ( 'NONE',  #36693 ) ;
#4637=ORIENTED_EDGE ( 'NONE', *, *, #26651, .T. ) ;
#4639=AXIS2_PLACEMENT_3D ( 'NONE', #44559, #49396, #36333 ) ;
#4640=ADVANCED_FACE ( 'NONE', ( #6676 ), #2114, .F. ) ;
#4641=CARTESIAN_POINT ( 'NONE',  ( -18.66354898467281132, 0.000000000000000000, 14.21960318569776582 ) ) ;
#4642=ORIENTED_EDGE ( 'NONE', *, *, #21273, .F. ) ;
#4643=EDGE_CURVE ( 'NONE', #47620, #19207, #7234, .T. ) ;
#4644=CARTESIAN_POINT ( 'NONE',  ( -22.71004419446258993, -5.375054281893161701, 14.32466392724574256 ) ) ;
#4645=DIRECTION ( 'NONE',  ( 0.9999697198139515519, 0.000000000000000000, 0.007781995580013368816 ) ) ;
#4646=CARTESIAN_POINT ( 'NONE',  ( -16.87027461792824212, -0.1191753592594190225, 9.771361154204708299 ) ) ;
#4647=ORIENTED_EDGE ( 'NONE', *, *, #10087, .F. ) ;
#4648=EDGE_CURVE ( 'NONE', #3650, #47902, #19742, .T. ) ;
#4649=CARTESIAN_POINT ( 'NONE',  ( -15.86710544311044302, 0.000000000000000000, 13.13336954653252953 ) ) ;
#4650=EDGE_LOOP ( 'NONE', ( #27067, #1842, #2188, #36358 ) ) ;
#4652=EDGE_LOOP ( 'NONE', ( #16229, #4076, #49345, #27637 ) ) ;
#4654=VERTEX_POINT ( 'NONE', #54364 ) ;
#4655=DIRECTION ( 'NONE',  ( 0.005002170337468016433, -0.7660444431189770143, -0.6427681459581293666 ) ) ;
#4657=ORIENTED_EDGE ( 'NONE', *, *, #54244, .F. ) ;
#4658=LINE ( 'NONE', #43829, #31280 ) ;
#4659=VECTOR ( 'NONE', #15050, 999.9999999999998863 ) ;
#4660=AXIS2_PLACEMENT_3D ( 'NONE', #21217, #55571, #56151 ) ;
#4661=ORIENTED_EDGE ( 'NONE', *, *, #29292, .F. ) ;
#4662=CARTESIAN_POINT ( 'NONE',  ( -16.01042127810387683, -4.079838673713161334, 9.596633394776388215 ) ) ;
#4663=ORIENTED_EDGE ( 'NONE', *, *, #53798, .T. ) ;
#4664=CARTESIAN_POINT ( 'NONE',  ( -10.94028622754223967, 0.000000000000000000, 11.14038480894692995 ) ) ;
#4665=ORIENTED_EDGE ( 'NONE', *, *, #6546, .T. ) ;
#4666=PLANE ( 'NONE',  #18415 ) ;
#4667=CARTESIAN_POINT ( 'NONE',  ( -18.67697421479882181, -0.1191753592594197858, 4.036397482078229793 ) ) ;
#4668=LINE ( 'NONE', #38773, #52162 ) ;
#4669=LINE ( 'NONE', #35612, #16915 ) ;
#4670=DIRECTION ( 'NONE',  ( -0.005961354470445682716, -0.6427876096865404731, 0.7660212471507180654 ) ) ;
#4671=ORIENTED_EDGE ( 'NONE', *, *, #17504, .T. ) ;
#4672=ORIENTED_EDGE ( 'NONE', *, *, #31453, .F. ) ;
#4673=LINE ( 'NONE', #51549, #55780 ) ;
#4674=PLANE ( 'NONE',  #374 ) ;
#4675=EDGE_CURVE ( 'NONE', #15181, #18631, #20584, .T. ) ;
#4676=AXIS2_PLACEMENT_3D ( 'NONE', #36363, #18483, #52833 ) ;
#4677=PLANE ( 'NONE',  #37867 ) ;
#4678=LINE ( 'NONE', #40154, #55719 ) ;
#4679=LINE ( 'NONE', #17451, #39450 ) ;
#4680=CARTESIAN_POINT ( 'NONE',  ( -15.03495456790438389, -0.1191753592594197858, 12.77051346725278158 ) ) ;
#4681=ORIENTED_EDGE ( 'NONE', *, *, #19211, .F. ) ;
#4682=DIRECTION ( 'NONE',  ( 0.9999697198139515519, 0.000000000000000000, 0.007781995580013368816 ) ) ;
#4683=CARTESIAN_POINT ( 'NONE',  ( -10.86613305818024244, 0.000000000000000000, 1.611861793503084783 ) ) ;
#4684=EDGE_LOOP ( 'NONE', ( #28834, #20802, #50716, #30370 ) ) ;
#4685=EDGE_CURVE ( 'NONE', #29674, #19075, #29083, .T. ) ;
#4686=ADVANCED_FACE ( 'NONE', ( #55212 ), #20283, .F. ) ;
#4687=EDGE_CURVE ( 'NONE', #41210, #44810, #23704, .T. ) ;
#4688=PLANE ( 'NONE',  #54263 ) ;
#4689=CARTESIAN_POINT ( 'NONE',  ( -18.81513686845778111, 0.000000000000000000, 7.997972008123892529 ) ) ;
#4690=DIRECTION ( 'NONE',  ( -0.6427681459581293666, -0.7660444431189770143, -0.005002170337467561935 ) ) ;
#4691=EDGE_CURVE ( 'NONE', #51537, #46161, #15215, .T. ) ;
#4692=DIRECTION ( 'NONE',  ( -0.6427681459581293666, -0.7660444431189770143, -0.005002170337467561935 ) ) ;
#4693=DIRECTION ( 'NONE',  ( 0.000000000000000000, -0.000000000000000000, -1.000000000000000000 ) ) ;
#4695=ORIENTED_EDGE ( 'NONE', *, *, #8334, .T. ) ;
#4696=DIRECTION ( 'NONE',  ( 0.9999697198139515519, 0.000000000000000000, 0.007781995580013368816 ) ) ;
#4697=CARTESIAN_POINT ( 'NONE',  ( -26.13493519185646008, 0.000000000000000000, 7.033017491833586377 ) ) ;
#4698=DIRECTION ( 'NONE',  ( 0.005002170337468016433, -0.7660444431189770143, -0.6427681459581293666 ) ) ;
#4699=VECTOR ( 'NONE', #6389, 1000.000000000000000 ) ;
#4700=VECTOR ( 'NONE', #6355, 1000.000000000000114 ) ;
#4702=DIRECTION ( 'NONE',  ( -0.7660212471507179544, -0.6427876096865405842, -0.005961354470445141482 ) ) ;
#4703=PLANE ( 'NONE',  #4709 ) ;
#4704=LINE ( 'NONE', #440, #23859 ) ;
#4705=ORIENTED_EDGE ( 'NONE', *, *, #25445, .F. ) ;
#4706=EDGE_CURVE ( 'NONE', #32268, #14910, #51236, .T. ) ;
#4707=DIRECTION ( 'NONE',  ( 0.6246952433987893460, 0.7422098413412802076, -0.2426528472758539279 ) ) ;
#4709=AXIS2_PLACEMENT_3D ( 'NONE', #22024, #17783, #26559 ) ;
#4710=ADVANCED_FACE ( 'NONE', ( #82 ), #13467, .F. ) ;
#4711=EDGE_LOOP ( 'NONE', ( #20363, #4716, #10512, #3937 ) ) ;
#4712=LINE ( 'NONE', #449, #11980 ) ;
#4713=ORIENTED_EDGE ( 'NONE', *, *, #21220, .T. ) ;
#4714=DIRECTION ( 'NONE',  ( -0.7660212471507179544, -0.6427876096865405842, -0.005961354470445141482 ) ) ;
#4715=FACE_OUTER_BOUND ( 'NONE', #54681, .T. ) ;
#4716=ORIENTED_EDGE ( 'NONE', *, *, #35208, .F. ) ;
#4717=EDGE_CURVE ( 'NONE', #30652, #9548, #38448, .T. ) ;
#4718=AXIS2_PLACEMENT_3D ( 'NONE', #553, #17585, #30913 ) ;
#4719=ORIENTED_EDGE ( 'NONE', *, *, #20424, .T. ) ;
#4720=ADVANCED_FACE ( 'NONE', ( #55776 ), #4391, .F. ) ;
#4721=VECTOR ( 'NONE', #41544, 1000.000000000000227 ) ;
#4722=ORIENTED_EDGE ( 'NONE', *, *, #1156, .T. ) ;
#4723=VERTEX_POINT ( 'NONE', #42991 ) ;
#4724=EDGE_LOOP ( 'NONE', ( #46716, #23607, #27045, #41861 ) ) ;
#4725=EDGE_LOOP ( 'NONE', ( #21949, #25511, #26549, #4961 ) ) ;
#4726=CARTESIAN_POINT ( 'NONE',  ( -11.16945636101648809, 0.000000000000000000, 6.580144182496990624 ) ) ;
#4727=LINE ( 'NONE', #25751, #19299 ) ;
#4728=CARTESIAN_POINT ( 'NONE',  ( -16.99924723426068951, 0.000000000000000000, 13.49389102713827171 ) ) ;
#4729=ORIENTED_EDGE ( 'NONE', *, *, #45073, .F. ) ;
#4730=CARTESIAN_POINT ( 'NONE',  ( -17.39116798849241974, 0.000000000000000000, 4.146406951555302811 ) ) ;
#4731=VERTEX_POINT ( 'NONE', #34748 ) ;
#4732=EDGE_LOOP ( 'NONE', ( #36213, #20385, #16789, #18805 ) ) ;
#4733=CARTESIAN_POINT ( 'NONE',  ( -16.98309541363131814, 4.981562823951510843, 11.65372539905892069 ) ) ;
#4734=FACE_OUTER_BOUND ( 'NONE', #19166, .T. ) ;
#4736=AXIS2_PLACEMENT_3D ( 'NONE', #39028, #4403, #17739 ) ;
#4737=ORIENTED_EDGE ( 'NONE', *, *, #55921, .F. ) ;
#4738=FACE_OUTER_BOUND ( 'NONE', #20647, .T. ) ;
#4739=VERTEX_POINT ( 'NONE', #8646 ) ;
#4740=VECTOR ( 'NONE', #4378, 999.9999999999998863 ) ;
#4741=VECTOR ( 'NONE', #54260, 1000.000000000000227 ) ;
#4742=DIRECTION ( 'NONE',  ( 0.005002170337468016433, -0.7660444431189770143, -0.6427681459581293666 ) ) ;
#4743=DIRECTION ( 'NONE',  ( 0.9999697198139515519, 0.000000000000000000, 0.007781995580013368816 ) ) ;
#4744=CARTESIAN_POINT ( 'NONE',  ( -14.94760462649100496, 0.000000000000000000, 2.488088991209854051 ) ) ;
#4745=AXIS2_PLACEMENT_3D ( 'NONE', #29991, #26040, #16950 ) ;
#4746=VECTOR ( 'NONE', #52021, 1000.000000000000227 ) ;
#4747=DIRECTION ( 'NONE',  ( 0.9999697198139515519, 0.000000000000000000, 0.007781995580013368816 ) ) ;
#4748=LINE ( 'NONE', #52174, #24116 ) ;
#4749=DIRECTION ( 'NONE',  ( -0.005961354470445682716, -0.6427876096865404731, 0.7660212471507180654 ) ) ;
#4750=DIRECTION ( 'NONE',  ( 0.000000000000000000, -1.000000000000000000, 0.000000000000000000 ) ) ;
#4752=ORIENTED_EDGE ( 'NONE', *, *, #55010, .F. ) ;
#4753=CARTESIAN_POINT ( 'NONE',  ( -11.09208034454450775, 1.905425754524005200, 4.316990091452962197 ) ) ;
#4754=ADVANCED_FACE ( 'NONE', ( #16889 ), #8346, .F. ) ;
#4755=CARTESIAN_POINT ( 'NONE',  ( -30.79411802867772607, 0.000000000000000000, 8.643412946479525516 ) ) ;
#4756=CARTESIAN_POINT ( 'NONE',  ( -14.01701317841955508, 0.000000000000000000, 2.326005055450897085 ) ) ;
#4757=LINE ( 'NONE', #38565, #22675 ) ;
#4758=VECTOR ( 'NONE', #32489, 1000.000000000000227 ) ;
#4760=FACE_OUTER_BOUND ( 'NONE', #19363, .T. ) ;
#4761=EDGE_CURVE ( 'NONE', #6528, #16795, #51529, .T. ) ;
#4762=EDGE_CURVE ( 'NONE', #17219, #12564, #4102, .T. ) ;
#4763=CARTESIAN_POINT ( 'NONE',  ( -21.47419595591918906, 0.000000000000000000, 5.222628093224860102 ) ) ;
#4764=DIRECTION ( 'NONE',  ( 0.9999697198139515519, 0.000000000000000000, 0.007781995580013368816 ) ) ;
#4765=ORIENTED_EDGE ( 'NONE', *, *, #13222, .F. ) ;
#4766=PLANE ( 'NONE',  #34785 ) ;
#4767=FACE_OUTER_BOUND ( 'NONE', #9387, .T. ) ;
#4768=DIRECTION ( 'NONE',  ( -0.7660212471507179544, -0.6427876096865405842, -0.005961354470445141482 ) ) ;
#4769=CARTESIAN_POINT ( 'NONE',  ( -12.13851405436063047, 0.000000000000000000, 11.68505802764555135 ) ) ;
#4770=CARTESIAN_POINT ( 'NONE',  ( -17.77262100021681945, -5.051250379848161387, 11.87538371510229673 ) ) ;
#4771=VECTOR ( 'NONE', #1406, 1000.000000000000227 ) ;
#4772=CARTESIAN_POINT ( 'NONE',  ( -1.086233639165236964, 0.000000000000000000, -2.796443541562362078 ) ) ;
#4773=DIRECTION ( 'NONE',  ( 0.007781995580012663651, -3.146120232559066537E-19, -0.9999697198139514409 ) ) ;
#4774=LINE ( 'NONE', #39429, #11461 ) ;
#4775=AXIS2_PLACEMENT_3D ( 'NONE', #34481, #35334, #18270 ) ;
#4776=CARTESIAN_POINT ( 'NONE',  ( -16.79925329029790149, 0.000000000000000000, 13.49544742625427496 ) ) ;
#4777=VECTOR ( 'NONE', #3079, 999.9999999999998863 ) ;
#4778=AXIS2_PLACEMENT_3D ( 'NONE', #11542, #24866, #50705 ) ;
#4779=EDGE_LOOP ( 'NONE', ( #37352, #48207, #16588, #21709 ) ) ;
#4780=ADVANCED_FACE ( 'NONE', ( #25976 ), #378, .F. ) ;
#4781=VECTOR ( 'NONE', #14007, 999.9999999999998863 ) ;
#4782=EDGE_LOOP ( 'NONE', ( #24536, #15010, #279, #31129 ) ) ;
#4783=EDGE_LOOP ( 'NONE', ( #24569, #29689, #34119, #52291 ) ) ;
#4784=VECTOR ( 'NONE', #45135, 1000.000000000000227 ) ;
#4785=ORIENTED_EDGE ( 'NONE', *, *, #44025, .F. ) ;
#4786=EDGE_CURVE ( 'NONE', #48904, #36106, #7815, .T. ) ;
#4787=ORIENTED_EDGE ( 'NONE', *, *, #11387, .T. ) ;
#4788=PLANE ( 'NONE',  #52303 ) ;
#4789=DIRECTION ( 'NONE',  ( -0.9999697198139514409, -0.000000000000000000, -0.007781995580013368816 ) ) ;
#4790=VERTEX_POINT ( 'NONE', #3532 ) ;
#4792=EDGE_CURVE ( 'NONE', #25448, #49293, #43544, .T. ) ;
#4793=AXIS2_PLACEMENT_3D ( 'NONE', #46562, #7676, #4280 ) ;
#4794=AXIS2_PLACEMENT_3D ( 'NONE', #51459, #17346, #4580 ) ;
#4795=PLANE ( 'NONE',  #49356 ) ;
#4796=ORIENTED_EDGE ( 'NONE', *, *, #48274, .F. ) ;
#4797=FACE_OUTER_BOUND ( 'NONE', #4115, .T. ) ;
#4798=CARTESIAN_POINT ( 'NONE',  ( -9.290790399115168796, 0.000000000000000000, 4.009439906764677097 ) ) ;
#4799=ORIENTED_EDGE ( 'NONE', *, *, #39261, .F. ) ;
#4800=CARTESIAN_POINT ( 'NONE',  ( -18.66354898467281132, 0.000000000000000000, 14.21960318569776582 ) ) ;
#4801=VECTOR ( 'NONE', #759, 1000.000000000000114 ) ;
#4802=ORIENTED_EDGE ( 'NONE', *, *, #26406, .F. ) ;
#4803=CARTESIAN_POINT ( 'NONE',  ( -5.619483069058131441, 5.495567360717212857, 5.401171638134291797 ) ) ;
#4804=VECTOR ( 'NONE', #26216, 1000.000000000000227 ) ;
#4805=PLANE ( 'NONE',  #55405 ) ;
#4806=CARTESIAN_POINT ( 'NONE',  ( -15.88130887279446490, 0.000000000000000000, 3.050160814894388839 ) ) ;
#4807=ORIENTED_EDGE ( 'NONE', *, *, #35426, .F. ) ;
#4808=DIRECTION ( 'NONE',  ( 0.005961354470445682716, -0.6427876096865404731, -0.7660212471507180654 ) ) ;
#4809=CARTESIAN_POINT ( 'NONE',  ( -19.08354877797473037, -4.403642575758160760, 11.32175784747634673 ) ) ;
#4810=DIRECTION ( 'NONE',  ( -0.7660212471507179544, -0.6427876096865405842, -0.005961354470445141482 ) ) ;
#4811=VECTOR ( 'NONE', #9109, 1000.000000000000114 ) ;
#4812=ORIENTED_EDGE ( 'NONE', *, *, #35245, .T. ) ;
#4813=DIRECTION ( 'NONE',  ( 0.007781995580012663651, 0.000000000000000000, -0.9999697198139515519 ) ) ;
#4814=ADVANCED_FACE ( 'NONE', ( #47533 ), #42698, .F. ) ;
#4815=ORIENTED_EDGE ( 'NONE', *, *, #5590, .F. ) ;
#4816=VECTOR ( 'NONE', #45377, 1000.000000000000227 ) ;
#4817=AXIS2_PLACEMENT_3D ( 'NONE', #6504, #40310, #6244 ) ;
#4818=LINE ( 'NONE', #36319, #30121 ) ;
#4819=DIRECTION ( 'NONE',  ( 0.005961354470445682716, -0.6427876096865404731, -0.7660212471507180654 ) ) ;
#4820=CARTESIAN_POINT ( 'NONE',  ( 2.072287782118878319, 0.000000000000000000, -2.950529333540147015 ) ) ;
#4821=DIRECTION ( 'NONE',  ( 0.007781995580012662783, 0.000000000000000000, -0.9999697198139514409 ) ) ;
#4822=CARTESIAN_POINT ( 'NONE',  ( -15.50102849149811135, -0.1191753592594197858, 12.95155240711365430 ) ) ;
#4823=CARTESIAN_POINT ( 'NONE',  ( -12.53330886209764117, 0.000000000000000000, 2.706883655320341919 ) ) ;
#4824=ADVANCED_FACE ( 'NONE', ( #46982 ), #38163, .F. ) ;
#4825=CARTESIAN_POINT ( 'NONE',  ( -21.47263955680318404, 0.000000000000000000, 5.022634149262071190 ) ) ;
#4826=VECTOR ( 'NONE', #12553, 999.9999999999998863 ) ;
#4827=LINE ( 'NONE', #13621, #53775 ) ;
#4828=VECTOR ( 'NONE', #47803, 999.9999999999998863 ) ;
#4829=DIRECTION ( 'NONE',  ( 0.000000000000000000, -0.000000000000000000, -1.000000000000000000 ) ) ;
#4830=VERTEX_POINT ( 'NONE', #8083 ) ;
#4831=DIRECTION ( 'NONE',  ( 0.5449076811759707706, 0.6444004775717708799, -0.5364919789714476250 ) ) ;
#4832=CARTESIAN_POINT ( 'NONE',  ( -17.68586913081282219, 0.000000000000000000, 8.006760230775915588 ) ) ;
#4833=LINE ( 'NONE', #46959, #31389 ) ;
#4834=CARTESIAN_POINT ( 'NONE',  ( -20.08902568218405449, -0.6798977022406558213, 4.662888621968888536 ) ) ;
#4835=VECTOR ( 'NONE', #33509, 1000.000000000000227 ) ;
#4837=CARTESIAN_POINT ( 'NONE',  ( -1.086233639165236964, 0.000000000000000000, -2.796443541562362078 ) ) ;
#4838=PLANE ( 'NONE',  #35619 ) ;
#4840=ORIENTED_EDGE ( 'NONE', *, *, #46193, .F. ) ;
#4841=EDGE_LOOP ( 'NONE', ( #27717, #13397, #38909, #40421 ) ) ;
#4842=LINE ( 'NONE', #34121, #1434 ) ;
#4843=CARTESIAN_POINT ( 'NONE',  ( -26.13337879274045505, 0.000000000000000000, 6.833023547870798353 ) ) ;
#4844=ORIENTED_EDGE ( 'NONE', *, *, #52200, .T. ) ;
#4845=VECTOR ( 'NONE', #12573, 1000.000000000000227 ) ;
#4846=LINE ( 'NONE', #4566, #45649 ) ;
#4847=ORIENTED_EDGE ( 'NONE', *, *, #54362, .F. ) ;
#4848=FACE_OUTER_BOUND ( 'NONE', #48453, .T. ) ;
#4849=AXIS2_PLACEMENT_3D ( 'NONE', #55133, #24455, #11688 ) ;
#4850=VERTEX_POINT ( 'NONE', #52365 ) ;
#4851=DIRECTION ( 'NONE',  ( -0.6427681459581293666, -0.7660444431189770143, -0.005002170337467561935 ) ) ;
#4853=ORIENTED_EDGE ( 'NONE', *, *, #14983, .F. ) ;
#4854=ORIENTED_EDGE ( 'NONE', *, *, #11241, .F. ) ;
#4855=DIRECTION ( 'NONE',  ( 0.9999697198139515519, 0.000000000000000000, 0.007781995580013368816 ) ) ;
#4856=AXIS2_PLACEMENT_3D ( 'NONE', #39915, #5296, #13785 ) ;
#4857=DIRECTION ( 'NONE',  ( 0.000000000000000000, -0.000000000000000000, -1.000000000000000000 ) ) ;
#4858=LINE ( 'NONE', #26716, #13975 ) ;
#4859=VECTOR ( 'NONE', #32127, 999.9999999999998863 ) ;
#4860=AXIS2_PLACEMENT_3D ( 'NONE', #26091, #55899, #34318 ) ;
#4861=DIRECTION ( 'NONE',  ( -0.005961354470445682716, -0.6427876096865404731, 0.7660212471507180654 ) ) ;
#4862=ORIENTED_EDGE ( 'NONE', *, *, #891, .T. ) ;
#4863=EDGE_CURVE ( 'NONE', #39017, #19141, #55478, .T. ) ;
#4864=ORIENTED_EDGE ( 'NONE', *, *, #12599, .T. ) ;
#4865=VECTOR ( 'NONE', #34584, 1000.000000000000227 ) ;
#4866=VECTOR ( 'NONE', #22457, 1000.000000000000114 ) ;
#4868=ORIENTED_EDGE ( 'NONE', *, *, #12708, .F. ) ;
#4869=FACE_OUTER_BOUND ( 'NONE', #20593, .T. ) ;
#4870=VERTEX_POINT ( 'NONE', #16581 ) ;
#4871=DIRECTION ( 'NONE',  ( 0.007781995580012663651, 0.000000000000000000, -0.9999697198139515519 ) ) ;
#4872=DIRECTION ( 'NONE',  ( 0.005002170337468016433, -0.7660444431189770143, -0.6427681459581293666 ) ) ;
#4873=EDGE_CURVE ( 'NONE', #16497, #34987, #12889, .T. ) ;
#4874=ORIENTED_EDGE ( 'NONE', *, *, #10852, .T. ) ;
#4875=CARTESIAN_POINT ( 'NONE',  ( -14.94916102560700821, 0.000000000000000000, 2.688082935172642962 ) ) ;
#4876=ORIENTED_EDGE ( 'NONE', *, *, #37121, .F. ) ;
#4877=EDGE_CURVE ( 'NONE', #19674, #12574, #27079, .T. ) ;
#4878=EDGE_CURVE ( 'NONE', #33225, #39974, #9185, .T. ) ;
#4879=FACE_OUTER_BOUND ( 'NONE', #54378, .T. ) ;
#4880=VECTOR ( 'NONE', #25983, 999.9999999999998863 ) ;
#4881=ORIENTED_EDGE ( 'NONE', *, *, #28199, .F. ) ;
#4882=FACE_OUTER_BOUND ( 'NONE', #32398, .T. ) ;
#4883=LINE ( 'NONE', #35837, #18432 ) ;
#4884=LINE ( 'NONE', #9419, #3797 ) ;
#4885=EDGE_CURVE ( 'NONE', #26046, #12964, #18548, .T. ) ;
#4886=EDGE_LOOP ( 'NONE', ( #14796, #43143, #51428, #32221 ) ) ;
#4887=VECTOR ( 'NONE', #16681, 1000.000000000000000 ) ;
#4888=PLANE ( 'NONE',  #44699 ) ;
#4889=ADVANCED_FACE ( 'NONE', ( #31884 ), #5774, .F. ) ;
#4890=CARTESIAN_POINT ( 'NONE',  ( 2.072287782118878319, 0.000000000000000000, -2.950529333540147015 ) ) ;
#4891=CARTESIAN_POINT ( 'NONE',  ( -17.06507362766180691, 0.000000000000000000, 3.410280553659843505 ) ) ;
#4892=AXIS2_PLACEMENT_3D ( 'NONE', #46012, #11649, #37469 ) ;
#4893=CARTESIAN_POINT ( 'NONE',  ( -13.60491223078244616, -0.1191753592594181482, 8.138522209111389571 ) ) ;
#4894=DIRECTION ( 'NONE',  ( 0.7660212471507180654, -0.6427876096865404731, 0.005961354470445141482 ) ) ;
#4895=ADVANCED_FACE ( 'NONE', ( #48934 ), #14568, .F. ) ;
#4896=DIRECTION ( 'NONE',  ( 0.9999697198139515519, 0.000000000000000000, 0.007781995580013368816 ) ) ;
#4897=ORIENTED_EDGE ( 'NONE', *, *, #39111, .T. ) ;
#4898=DIRECTION ( 'NONE',  ( -0.7660212471507179544, -0.6427876096865405842, -0.005961354470445141482 ) ) ;
#4899=PLANE ( 'NONE',  #19536 ) ;
#4901=EDGE_LOOP ( 'NONE', ( #10034, #23064, #8167, #23110, #42832 ) ) ;
#4902=VECTOR ( 'NONE', #36997, 999.9999999999998863 ) ;
#4903=PLANE ( 'NONE',  #32028 ) ;
#4904=PLANE ( 'NONE',  #1865 ) ;
#4905=ORIENTED_EDGE ( 'NONE', *, *, #48509, .F. ) ;
#4906=VECTOR ( 'NONE', #23868, 1000.000000000000114 ) ;
#4907=EDGE_CURVE ( 'NONE', #29013, #27017, #13720, .T. ) ;
#4908=PLANE ( 'NONE',  #7132 ) ;
#4909=PLANE ( 'NONE',  #3064 ) ;
#4910=LINE ( 'NONE', #39568, #42288 ) ;
#4911=DIRECTION ( 'NONE',  ( 0.000000000000000000, -0.000000000000000000, -1.000000000000000000 ) ) ;
#4912=ADVANCED_FACE ( 'NONE', ( #36418 ), #36167, .F. ) ;
#4913=ORIENTED_EDGE ( 'NONE', *, *, #4480, .F. ) ;
#4914=VECTOR ( 'NONE', #21751, 1000.000000000000227 ) ;
#4915=AXIS2_PLACEMENT_3D ( 'NONE', #48127, #18898, #31674 ) ;
#4916=ORIENTED_EDGE ( 'NONE', *, *, #5344, .T. ) ;
#4918=DIRECTION ( 'NONE',  ( -0.7660212471507179544, -0.6427876096865405842, -0.005961354470445141482 ) ) ;
#4919=DIRECTION ( 'NONE',  ( -0.7660212471507179544, -0.6427876096865405842, -0.005961354470445141482 ) ) ;
#4920=DIRECTION ( 'NONE',  ( 0.005961354470445682716, -0.6427876096865404731, -0.7660212471507180654 ) ) ;
#4921=LINE ( 'NONE', #22244, #2886 ) ;
#4922=CARTESIAN_POINT ( 'NONE',  ( -10.66458271510145117, 0.000000000000000000, 1.413424248656298676 ) ) ;
#4923=ORIENTED_EDGE ( 'NONE', *, *, #5709, .T. ) ;
#4924=CARTESIAN_POINT ( 'NONE',  ( -12.92677208044202253, 5.143464774974012776, 10.34382034707842912 ) ) ;
#4925=VECTOR ( 'NONE', #52090, 999.9999999999998863 ) ;
#4926=LINE ( 'NONE', #12614, #26954 ) ;
#4928=VECTOR ( 'NONE', #41244, 999.9999999999998863 ) ;
#4929=DIRECTION ( 'NONE',  ( -0.005002170337468016433, -0.7660444431189770143, 0.6427681459581293666 ) ) ;
#4930=LINE ( 'NONE', #14008, #21371 ) ;
#4931=VECTOR ( 'NONE', #34246, 999.9999999999998863 ) ;
#4932=DIRECTION ( 'NONE',  ( -0.7660212471507179544, -0.6427876096865405842, -0.005961354470445141482 ) ) ;
#4933=ORIENTED_EDGE ( 'NONE', *, *, #33996, .T. ) ;
#4934=CARTESIAN_POINT ( 'NONE',  ( -32.65919192261063841, -0.1191753592594197858, 9.467565677904410393 ) ) ;
#4935=EDGE_CURVE ( 'NONE', #27147, #19740, #22803, .T. ) ;
#4936=ORIENTED_EDGE ( 'NONE', *, *, #15714, .T. ) ;
#4937=ORIENTED_EDGE ( 'NONE', *, *, #11703, .T. ) ;
#4938=ORIENTED_EDGE ( 'NONE', *, *, #33034, .T. ) ;
#4939=VERTEX_POINT ( 'NONE', #1213 ) ;
#4940=VECTOR ( 'NONE', #55020, 1000.000000000000227 ) ;
#4941=DIRECTION ( 'NONE',  ( 0.005002170337468016433, -0.7660444431189770143, -0.6427681459581293666 ) ) ;
#4943=ADVANCED_FACE ( 'NONE', ( #1771 ), #40423, .F. ) ;
#4944=CARTESIAN_POINT ( 'NONE',  ( -20.15831888576414244, 4.333955019861509328, 11.82425529087645977 ) ) ;
#4946=AXIS2_PLACEMENT_3D ( 'NONE', #39401, #31458, #18090 ) ;
#4947=ORIENTED_EDGE ( 'NONE', *, *, #3587, .T. ) ;
#4948=CARTESIAN_POINT ( 'NONE',  ( -13.05847201118137768, 0.9340140483890039258, 3.486551290014034965 ) ) ;
#4949=ORIENTED_EDGE ( 'NONE', *, *, #47919, .T. ) ;
#4950=FACE_OUTER_BOUND ( 'NONE', #48058, .T. ) ;
#4951=ORIENTED_EDGE ( 'NONE', *, *, #38855, .T. ) ;
#4952=EDGE_CURVE ( 'NONE', #6678, #15287, #53214, .T. ) ;
#4953=AXIS2_PLACEMENT_3D ( 'NONE', #13454, #30506, #35310 ) ;
#4954=VECTOR ( 'NONE', #38998, 1000.000000000000114 ) ;
#4955=DIRECTION ( 'NONE',  ( -0.7660212471507179544, -0.6427876096865405842, -0.005961354470445141482 ) ) ;
#4956=CARTESIAN_POINT ( 'NONE',  ( -19.72010057970841146, 0.000000000000000000, 4.866946799230784215 ) ) ;
#4957=PLANE ( 'NONE',  #27692 ) ;
#4958=CARTESIAN_POINT ( 'NONE',  ( -9.493658396583240844, 0.000000000000000000, 4.377193210906439980 ) ) ;
#4959=CARTESIAN_POINT ( 'NONE',  ( -10.94028622754223967, 0.000000000000000000, 11.14038480894692995 ) ) ;
#4960=ORIENTED_EDGE ( 'NONE', *, *, #9307, .F. ) ;
#4961=ORIENTED_EDGE ( 'NONE', *, *, #51856, .F. ) ;
#4962=EDGE_CURVE ( 'NONE', #1446, #37525, #53732, .T. ) ;
#4963=CARTESIAN_POINT ( 'NONE',  ( -12.33850799832341849, 0.000000000000000000, 11.68350162852954632 ) ) ;
#4964=DIRECTION ( 'NONE',  ( 0.6427681459581294776, -0.7660444431189769032, 0.005002170337467562802 ) ) ;
#4965=ADVANCED_FACE ( 'NONE', ( #31626 ), #31037, .F. ) ;
#4966=FACE_OUTER_BOUND ( 'NONE', #30441, .T. ) ;
#4967=VECTOR ( 'NONE', #52196, 999.9999999999998863 ) ;
#4968=PLANE ( 'NONE',  #51177 ) ;
#4969=VECTOR ( 'NONE', #16187, 1000.000000000000000 ) ;
#4970=DIRECTION ( 'NONE',  ( 0.007781995580012663651, 0.000000000000000000, -0.9999697198139515519 ) ) ;
#4971=LINE ( 'NONE', #48704, #15071 ) ;
#4972=ORIENTED_EDGE ( 'NONE', *, *, #44268, .T. ) ;
#4974=CARTESIAN_POINT ( 'NONE',  ( -16.53317331066696383, 0.000000000000000000, 13.31285208727739899 ) ) ;
#4975=VECTOR ( 'NONE', #14528, 1000.000000000000227 ) ;
#4976=ORIENTED_EDGE ( 'NONE', *, *, #6151, .T. ) ;
#4977=EDGE_CURVE ( 'NONE', #8089, #36178, #9469, .T. ) ;
#4978=CARTESIAN_POINT ( 'NONE',  ( -13.63673279712320507, -0.1191753592594197858, 12.22739664767016521 ) ) ;
#4979=DIRECTION ( 'NONE',  ( 0.5449076811759707706, 0.6444004775717708799, -0.5364919789714476250 ) ) ;
#4980=VECTOR ( 'NONE', #22755, 999.9999999999998863 ) ;
#4981=LINE ( 'NONE', #48712, #23240 ) ;
#4982=FACE_OUTER_BOUND ( 'NONE', #24546, .T. ) ;
#4983=DIRECTION ( 'NONE',  ( -0.005961354470445682716, -0.6427876096865404731, 0.7660212471507180654 ) ) ;
#4984=ORIENTED_EDGE ( 'NONE', *, *, #12178, .F. ) ;
#4985=VECTOR ( 'NONE', #10632, 1000.000000000000114 ) ;
#4986=VECTOR ( 'NONE', #48627, 1000.000000000000227 ) ;
#4987=EDGE_LOOP ( 'NONE', ( #430, #2685, #2467, #17533 ) ) ;
#4988=AXIS2_PLACEMENT_3D ( 'NONE', #30147, #42077, #17352 ) ;
#4989=LINE ( 'NONE', #39646, #1248 ) ;
#4990=LINE ( 'NONE', #35366, #52188 ) ;
#4991=DIRECTION ( 'NONE',  ( 0.000000000000000000, -0.000000000000000000, -1.000000000000000000 ) ) ;
#4992=AXIS2_PLACEMENT_3D ( 'NONE', #49734, #24178, #45733 ) ;
#4993=DIRECTION ( 'NONE',  ( 0.5449076811759707706, 0.6444004775717708799, -0.5364919789714476250 ) ) ;
#4994=CARTESIAN_POINT ( 'NONE',  ( -12.75054712709212623, 0.000000000000000000, 4.921185475750926130 ) ) ;
#4995=LINE ( 'NONE', #22325, #3762 ) ;
#4996=CARTESIAN_POINT ( 'NONE',  ( -13.27065584551087163, 0.000000000000000000, 12.04557950825129176 ) ) ;
#4997=VECTOR ( 'NONE', #23690, 1000.000000000000000 ) ;
#4998=DIRECTION ( 'NONE',  ( -0.7660212471507179544, -0.6427876096865405842, -0.005961354470445141482 ) ) ;
#4999=VECTOR ( 'NONE', #34499, 1000.000000000000000 ) ;
#5000=FACE_OUTER_BOUND ( 'NONE', #32329, .T. ) ;
#5002=ORIENTED_EDGE ( 'NONE', *, *, #5251, .T. ) ;
#5003=CARTESIAN_POINT ( 'NONE',  ( -15.87975247367846166, 0.000000000000000000, 2.850166870931599927 ) ) ;
#5004=ORIENTED_EDGE ( 'NONE', *, *, #10381, .T. ) ;
#5005=PLANE ( 'NONE',  #20472 ) ;
#5006=ADVANCED_FACE ( 'NONE', ( #35588 ), #5232, .F. ) ;
#5007=CARTESIAN_POINT ( 'NONE',  ( -19.60834386242827776, 0.000000000000000000, 4.298478389818581213 ) ) ;
#5008=ORIENTED_EDGE ( 'NONE', *, *, #53310, .F. ) ;
#5009=ADVANCED_FACE ( 'NONE', ( #14013 ), #31341, .F. ) ;
#5010=VERTEX_POINT ( 'NONE', #15394 ) ;
#5011=VECTOR ( 'NONE', #37889, 1000.000000000000227 ) ;
#5012=ORIENTED_EDGE ( 'NONE', *, *, #46994, .T. ) ;
#5013=VERTEX_POINT ( 'NONE', #23635 ) ;
#5014=ORIENTED_EDGE ( 'NONE', *, *, #38271, .F. ) ;
#5015=VECTOR ( 'NONE', #27422, 999.9999999999998863 ) ;
#5016=EDGE_CURVE ( 'NONE', #2953, #18999, #19375, .T. ) ;
#5018=LINE ( 'NONE', #22351, #37457 ) ;
#5019=CARTESIAN_POINT ( 'NONE',  ( -14.85437466704310516, -5.536956232915666298, 2.474606801569680492 ) ) ;
#5020=VECTOR ( 'NONE', #52256, 1000.000000000000000 ) ;
#5021=EDGE_CURVE ( 'NONE', #7467, #10997, #46315, .T. ) ;
#5022=EDGE_CURVE ( 'NONE', #33373, #44514, #45484, .T. ) ;
#5023=EDGE_CURVE ( 'NONE', #547, #23151, #3174, .T. ) ;
#5024=ORIENTED_EDGE ( 'NONE', *, *, #29108, .T. ) ;
#5025=CARTESIAN_POINT ( 'NONE',  ( -13.14168322917842069, -0.1191753592594198830, 8.323049635317726569 ) ) ;
#5026=VERTEX_POINT ( 'NONE', #36711 ) ;
#5027=AXIS2_PLACEMENT_3D ( 'NONE', #34431, #12303, #51740 ) ;
#5028=EDGE_LOOP ( 'NONE', ( #49887, #43223, #54034, #13700 ) ) ;
#5029=AXIS2_PLACEMENT_3D ( 'NONE', #48032, #22199, #8587 ) ;
#5030=AXIS2_PLACEMENT_3D ( 'NONE', #14325, #36177, #40438 ) ;
#5031=DIRECTION ( 'NONE',  ( -0.9999697198139514409, -0.000000000000000000, -0.007781995580013368816 ) ) ;
#5032=DIRECTION ( 'NONE',  ( 0.007781995580012662783, 0.000000000000000000, -0.9999697198139514409 ) ) ;
#5033=VECTOR ( 'NONE', #30539, 1000.000000000000227 ) ;
#5035=ORIENTED_EDGE ( 'NONE', *, *, #19421, .T. ) ;
#5036=CARTESIAN_POINT ( 'NONE',  ( -9.110551994824897193, -1.000000000000000000, 3.538847790438064411 ) ) ;
#5037=VERTEX_POINT ( 'NONE', #32177 ) ;
#5039=VECTOR ( 'NONE', #3958, 1000.000000000000227 ) ;
#5040=ADVANCED_FACE ( 'NONE', ( #24467 ), #54554, .F. ) ;
#5041=DIRECTION ( 'NONE',  ( -0.6427681459581293666, -0.7660444431189770143, -0.005002170337467561935 ) ) ;
#5042=VECTOR ( 'NONE', #29861, 1000.000000000000227 ) ;
#5043=ADVANCED_FACE ( 'NONE', ( #36999 ), #20509, .F. ) ;
#5044=PLANE ( 'NONE',  #55089 ) ;
#5046=DIRECTION ( 'NONE',  ( -0.5449076811759708816, 0.6444004775717707689, 0.5364919789714475140 ) ) ;
#5047=CARTESIAN_POINT ( 'NONE',  ( -18.39746900504187010, 0.000000000000000000, 14.03700784672088808 ) ) ;
#5048=DIRECTION ( 'NONE',  ( 0.9999697198139515519, 0.000000000000000000, 0.007781995580013368816 ) ) ;
#5050=CARTESIAN_POINT ( 'NONE',  ( -21.47419595591918906, 0.000000000000000000, 5.222628093224860102 ) ) ;
#5051=CARTESIAN_POINT ( 'NONE',  ( -14.01623497886155256, -0.1191753592594197858, 2.226008083469502630 ) ) ;
#5052=VERTEX_POINT ( 'NONE', #11432 ) ;
#5053=LINE ( 'NONE', #14670, #13852 ) ;
#5054=ADVANCED_FACE ( 'NONE', ( #7428 ), #42069, .F. ) ;
#5055=LINE ( 'NONE', #5594, #3845 ) ;
#5056=LINE ( 'NONE', #30627, #23269 ) ;
#5057=DIRECTION ( 'NONE',  ( 0.7660212471507180654, -0.6427876096865404731, 0.005961354470445141482 ) ) ;
#5059=DIRECTION ( 'NONE',  ( -0.005002170337468016433, -0.7660444431189770143, 0.6427681459581293666 ) ) ;
#5060=EDGE_CURVE ( 'NONE', #873, #34138, #46061, .T. ) ;
#5061=DIRECTION ( 'NONE',  ( 0.9999697198139515519, 0.000000000000000000, 0.007781995580013368816 ) ) ;
#5062=AXIS2_PLACEMENT_3D ( 'NONE', #33287, #29004, #17328 ) ;
#5063=DIRECTION ( 'NONE',  ( -0.9999697198139514409, -0.000000000000000000, -0.007781995580013368816 ) ) ;
#5064=VECTOR ( 'NONE', #12049, 999.9999999999998863 ) ;
#5065=ORIENTED_EDGE ( 'NONE', *, *, #26541, .T. ) ;
#5066=CARTESIAN_POINT ( 'NONE',  ( -14.04080859257070912, -0.1191753592594186895, 4.441809264765737453 ) ) ;
#5067=FACE_OUTER_BOUND ( 'NONE', #9366, .T. ) ;
#5068=LINE ( 'NONE', #51897, #35441 ) ;
#5069=VECTOR ( 'NONE', #55446, 1000.000000000000114 ) ;
#5070=LINE ( 'NONE', #13315, #53614 ) ;
#5071=AXIS2_PLACEMENT_3D ( 'NONE', #37494, #32431, #49459 ) ;
#5072=LINE ( 'NONE', #48493, #50248 ) ;
#5073=LINE ( 'NONE', #23974, #30461 ) ;
#5074=CARTESIAN_POINT ( 'NONE',  ( -17.74404816805336793, 0.000000000000000000, 3.574322630375089460 ) ) ;
#5075=AXIS2_PLACEMENT_3D ( 'NONE', #26732, #21904, #34689 ) ;
#5076=CARTESIAN_POINT ( 'NONE',  ( -14.60179020832990204, 0.000000000000000000, 3.968108478200570666 ) ) ;
#5077=VECTOR ( 'NONE', #49831, 999.9999999999998863 ) ;
#5078=DIRECTION ( 'NONE',  ( -0.9999697198139514409, -0.000000000000000000, -0.007781995580013368816 ) ) ;
#5079=VECTOR ( 'NONE', #35946, 1000.000000000000227 ) ;
#5080=ORIENTED_EDGE ( 'NONE', *, *, #14001, .F. ) ;
#5081=VECTOR ( 'NONE', #41348, 1000.000000000000227 ) ;
#5082=AXIS2_PLACEMENT_3D ( 'NONE', #20958, #21249, #30056 ) ;
#5083=VECTOR ( 'NONE', #39661, 1000.000000000000227 ) ;
#5084=VERTEX_POINT ( 'NONE', #20202 ) ;
#5087=VERTEX_POINT ( 'NONE', #23917 ) ;
#5089=DIRECTION ( 'NONE',  ( -0.5364919789714478471, 0.6444004775717705469, -0.5449076811759709926 ) ) ;
#5090=DIRECTION ( 'NONE',  ( 0.000000000000000000, 1.000000000000000000, 0.000000000000000000 ) ) ;
#5091=EDGE_CURVE ( 'NONE', #50886, #29241, #54300, .T. ) ;
#5092=EDGE_CURVE ( 'NONE', #40865, #15204, #2038, .T. ) ;
#5093=ORIENTED_EDGE ( 'NONE', *, *, #2810, .T. ) ;
#5095=ADVANCED_FACE ( 'NONE', ( #50019 ), #11701, .F. ) ;
#5096=AXIS2_PLACEMENT_3D ( 'NONE', #6807, #29739, #46755 ) ;
#5097=DIRECTION ( 'NONE',  ( 0.7660212471507180654, -0.6427876096865404731, 0.005961354470445141482 ) ) ;
#5098=ORIENTED_EDGE ( 'NONE', *, *, #35815, .T. ) ;
#5099=DIRECTION ( 'NONE',  ( -0.7660212471507179544, -0.6427876096865405842, -0.005961354470445141482 ) ) ;
#5100=DIRECTION ( 'NONE',  ( 0.9999697198139515519, 0.000000000000000000, 0.007781995580013368816 ) ) ;
#5101=ORIENTED_EDGE ( 'NONE', *, *, #22730, .F. ) ;
#5102=AXIS2_PLACEMENT_3D ( 'NONE', #16328, #7848, #55509 ) ;
#5103=CARTESIAN_POINT ( 'NONE',  ( -11.67244013076689946, 0.000000000000000000, 11.50401908778467863 ) ) ;
#5104=EDGE_LOOP ( 'NONE', ( #29800, #7473, #29320, #10867 ) ) ;
#5105=LINE ( 'NONE', #39743, #25526 ) ;
#5106=VECTOR ( 'NONE', #41436, 1000.000000000000000 ) ;
#5107=LINE ( 'NONE', #38112, #30270 ) ;
#5108=CARTESIAN_POINT ( 'NONE',  ( -17.20267025855076426, 0.000000000000000000, 5.625202163702363478 ) ) ;
#5109=LINE ( 'NONE', #35465, #53247 ) ;
#5110=VECTOR ( 'NONE', #30685, 999.9999999999998863 ) ;
#5111=AXIS2_PLACEMENT_3D ( 'NONE', #52015, #12575, #8297 ) ;
#5112=ORIENTED_EDGE ( 'NONE', *, *, #49843, .T. ) ;
#5113=CARTESIAN_POINT ( 'NONE',  ( -11.87243407472968926, 0.000000000000000000, 11.50246268866867361 ) ) ;
#5114=FACE_OUTER_BOUND ( 'NONE', #8974, .T. ) ;
#5116=ORIENTED_EDGE ( 'NONE', *, *, #40879, .F. ) ;
#5117=CARTESIAN_POINT ( 'NONE',  ( -15.34412267118641715, 0.000000000000000000, 5.639665810774401322 ) ) ;
#5118=ORIENTED_EDGE ( 'NONE', *, *, #42816, .F. ) ;
#5119=AXIS2_PLACEMENT_3D ( 'NONE', #11619, #15569, #45980 ) ;
#5120=AXIS2_PLACEMENT_3D ( 'NONE', #42653, #22131, #42397 ) ;
#5121=LINE ( 'NONE', #572, #2046 ) ;
#5122=PLANE ( 'NONE',  #41407 ) ;
#5123=CARTESIAN_POINT ( 'NONE',  ( -14.01623497886155256, -0.1191753592594197858, 2.226008083469502630 ) ) ;
#5124=CARTESIAN_POINT ( 'NONE',  ( -15.08367142620268098, 0.000000000000000000, 6.180350785979147332 ) ) ;
#5125=CARTESIAN_POINT ( 'NONE',  ( -11.83564360093636658, 0.000000000000000000, 6.774965815575766825 ) ) ;
#5126=ADVANCED_FACE ( 'NONE', ( #6334 ), #27928, .F. ) ;
#5127=DIRECTION ( 'NONE',  ( 0.005961354470445682716, -0.6427876096865404731, -0.7660212471507180654 ) ) ;
#5129=VECTOR ( 'NONE', #24464, 999.9999999999998863 ) ;
#5130=VECTOR ( 'NONE', #9816, 1000.000000000000227 ) ;
#5131=LINE ( 'NONE', #43709, #51056 ) ;
#5132=EDGE_CURVE ( 'NONE', #39753, #44131, #45233, .T. ) ;
#5133=CARTESIAN_POINT ( 'NONE',  ( -14.20280369269832832, 0.000000000000000000, 12.40765738797303719 ) ) ;
#5134=VERTEX_POINT ( 'NONE', #6901 ) ;
#5135=DIRECTION ( 'NONE',  ( 0.007781995580012663651, 0.000000000000000000, -0.9999697198139515519 ) ) ;
#5136=LINE ( 'NONE', #39766, #33285 ) ;
#5137=FACE_OUTER_BOUND ( 'NONE', #19379, .T. ) ;
#5138=ADVANCED_FACE ( 'NONE', ( #42917 ), #43229, .F. ) ;
#5140=ADVANCED_FACE ( 'NONE', ( #8868 ), #42631, .F. ) ;
#5141=CARTESIAN_POINT ( 'NONE',  ( -11.77243710274829525, -0.1191753592594197858, 11.50324088822667612 ) ) ;
#5142=PLANE ( 'NONE',  #34197 ) ;
#5143=LINE ( 'NONE', #43724, #1144 ) ;
#5144=AXIS2_PLACEMENT_3D ( 'NONE', #24175, #45447, #53691 ) ;
#5145=EDGE_LOOP ( 'NONE', ( #14642, #22516, #34299, #53745 ) ) ;
#5146=ORIENTED_EDGE ( 'NONE', *, *, #20846, .T. ) ;
#5147=DIRECTION ( 'NONE',  ( 0.5449076811759707706, 0.6444004775717708799, -0.5364919789714476250 ) ) ;
#5149=CARTESIAN_POINT ( 'NONE',  ( -12.60458797795435615, 0.000000000000000000, 11.86609696750642229 ) ) ;
#5150=VECTOR ( 'NONE', #18510, 1000.000000000000227 ) ;
#5151=EDGE_LOOP ( 'NONE', ( #53537, #52965, #38342, #36972 ) ) ;
#5152=LINE ( 'NONE', #48007, #10475 ) ;
#5153=VECTOR ( 'NONE', #32017, 999.9999999999998863 ) ;
#5154=ORIENTED_EDGE ( 'NONE', *, *, #47091, .T. ) ;
#5156=VECTOR ( 'NONE', #47930, 999.9999999999998863 ) ;
#5157=ORIENTED_EDGE ( 'NONE', *, *, #45855, .T. ) ;
#5158=VERTEX_POINT ( 'NONE', #51994 ) ;
#5159=ORIENTED_EDGE ( 'NONE', *, *, #20970, .T. ) ;
#5160=CARTESIAN_POINT ( 'NONE',  ( -8.940786546353891140, -0.1117717739994061044, 6.691278700656821066 ) ) ;
#5161=DIRECTION ( 'NONE',  ( 0.6246952433987894571, -0.7422098413412800966, -0.2426528472758541777 ) ) ;
#5162=DIRECTION ( 'NONE',  ( 0.6427681459581294776, -0.7660444431189769032, 0.005002170337467562802 ) ) ;
#5163=ADVANCED_FACE ( 'NONE', ( #43480 ), #12265, .F. ) ;
#5164=AXIS2_PLACEMENT_3D ( 'NONE', #46484, #20378, #37720 ) ;
#5165=CARTESIAN_POINT ( 'NONE',  ( -32.65841372305263235, 0.000000000000000000, 9.367568705923016381 ) ) ;
#5166=ORIENTED_EDGE ( 'NONE', *, *, #34783, .F. ) ;
#5167=ORIENTED_EDGE ( 'NONE', *, *, #34885, .F. ) ;
#5168=EDGE_CURVE ( 'NONE', #55683, #51210, #21637, .T. ) ;
#5169=EDGE_CURVE ( 'NONE', #39497, #29979, #21044, .T. ) ;
#5170=VECTOR ( 'NONE', #16436, 1000.000000000000227 ) ;
#5171=VECTOR ( 'NONE', #35864, 1000.000000000000227 ) ;
#5172=LINE ( 'NONE', #13409, #8261 ) ;
#5173=EDGE_LOOP ( 'NONE', ( #45810, #49233, #40598, #47149 ) ) ;
#5174=DIRECTION ( 'NONE',  ( -0.6427681459581293666, -0.7660444431189770143, -0.005002170337467561935 ) ) ;
#5175=ORIENTED_EDGE ( 'NONE', *, *, #23296, .F. ) ;
#5176=LINE ( 'NONE', #30727, #26944 ) ;
#5177=DIRECTION ( 'NONE',  ( 0.000000000000000000, -0.000000000000000000, -1.000000000000000000 ) ) ;
#5178=EDGE_LOOP ( 'NONE', ( #35111, #37001, #4562, #13465 ) ) ;
#5179=FACE_OUTER_BOUND ( 'NONE', #52698, .T. ) ;
#5180=EDGE_LOOP ( 'NONE', ( #26217, #26167, #30151, #24634 ) ) ;
#5181=AXIS2_PLACEMENT_3D ( 'NONE', #40356, #22490, #13119 ) ;
#5182=EDGE_CURVE ( 'NONE', #29996, #49857, #51709, .T. ) ;
#5183=CARTESIAN_POINT ( 'NONE',  ( -17.74560456716937296, 0.000000000000000000, 3.774316574337878372 ) ) ;
#5184=ORIENTED_EDGE ( 'NONE', *, *, #45461, .F. ) ;
#5185=DIRECTION ( 'NONE',  ( 0.6427681459581294776, -0.7660444431189769032, 0.005002170337467562802 ) ) ;
#5186=CARTESIAN_POINT ( 'NONE',  ( -15.55693048355961672, 0.000000000000000000, 7.284663983984430935 ) ) ;
#5187=DIRECTION ( 'NONE',  ( 0.005961354470445682716, -0.6427876096865404731, -0.7660212471507180654 ) ) ;
#5189=CARTESIAN_POINT ( 'NONE',  ( -13.72166355981337738, -1.975113310420658852, 2.148264778013123877 ) ) ;
#5190=LINE ( 'NONE', #22505, #13819 ) ;
#5191=AXIS2_PLACEMENT_3D ( 'NONE', #25128, #42434, #37310 ) ;
#5192=LINE ( 'NONE', #1735, #2236 ) ;
#5194=PLANE ( 'NONE',  #31289 ) ;
#5195=CARTESIAN_POINT ( 'NONE',  ( -24.26908309836554878, 0.000000000000000000, 6.108867788427308376 ) ) ;
#5196=VECTOR ( 'NONE', #716, 1000.000000000000000 ) ;
#5197=DIRECTION ( 'NONE',  ( 0.6427681459581294776, -0.7660444431189769032, 0.005002170337467562802 ) ) ;
#5198=EDGE_LOOP ( 'NONE', ( #37033, #31982, #40882, #49241 ) ) ;
#5199=DIRECTION ( 'NONE',  ( 0.7660212471507180654, -0.6427876096865404731, 0.005961354470445141482 ) ) ;
#5200=DIRECTION ( 'NONE',  ( -0.5449076811759708816, 0.6444004775717707689, 0.5364919789714475140 ) ) ;
#5201=DIRECTION ( 'NONE',  ( 0.9999697198139515519, 0.000000000000000000, 0.007781995580013368816 ) ) ;
#5202=EDGE_LOOP ( 'NONE', ( #2056, #40033, #32232, #42776, #31641 ) ) ;
#5203=FACE_OUTER_BOUND ( 'NONE', #55401, .T. ) ;
#5204=CARTESIAN_POINT ( 'NONE',  ( -23.33693525117809386, 0.000000000000000000, 5.746789908705562944 ) ) ;
#5205=ORIENTED_EDGE ( 'NONE', *, *, #9048, .F. ) ;
#5206=DIRECTION ( 'NONE',  ( -0.5364919789714478471, 0.6444004775717705469, -0.5449076811759709926 ) ) ;
#5207=VECTOR ( 'NONE', #11790, 999.9999999999998863 ) ;
#5208=EDGE_CURVE ( 'NONE', #10857, #25116, #29870, .T. ) ;
#5209=PLANE ( 'NONE',  #3966 ) ;
#5210=DIRECTION ( 'NONE',  ( 0.6427681459581294776, -0.7660444431189769032, 0.005002170337467562802 ) ) ;
#5211=DIRECTION ( 'NONE',  ( 0.007781995580012663651, 0.000000000000000000, -0.9999697198139515519 ) ) ;
#5212=ORIENTED_EDGE ( 'NONE', *, *, #42571, .T. ) ;
#5213=ORIENTED_EDGE ( 'NONE', *, *, #54497, .T. ) ;
#5214=CARTESIAN_POINT ( 'NONE',  ( -14.00280974873554030, 0.000000000000000000, 12.40921378708904044 ) ) ;
#5215=DIRECTION ( 'NONE',  ( 0.005002170337468016433, -0.7660444431189770143, -0.6427681459581293666 ) ) ;
#5217=ADVANCED_FACE ( 'NONE', ( #55145 ), #16507, .F. ) ;
#5218=LINE ( 'NONE', #48068, #53810 ) ;
#5219=DIRECTION ( 'NONE',  ( -0.5449076811759708816, 0.6444004775717707689, 0.5364919789714475140 ) ) ;
#5220=PLANE ( 'NONE',  #4953 ) ;
#5221=ORIENTED_EDGE ( 'NONE', *, *, #11737, .F. ) ;
#5222=ADVANCED_FACE ( 'NONE', ( #38377 ), #8015, .F. ) ;
#5223=CARTESIAN_POINT ( 'NONE',  ( -11.67244013076689946, 0.000000000000000000, 11.50401908778467863 ) ) ;
#5224=EDGE_CURVE ( 'NONE', #3767, #7042, #11960, .T. ) ;
#5226=EDGE_LOOP ( 'NONE', ( #52178, #26962, #6543, #15584 ) ) ;
#5227=PLANE ( 'NONE',  #265 ) ;
#5228=EDGE_CURVE ( 'NONE', #30507, #31662, #25901, .T. ) ;
#5229=CARTESIAN_POINT ( 'NONE',  ( -14.93495759592298988, 0.000000000000000000, 12.77129166681078409 ) ) ;
#5230=DIRECTION ( 'NONE',  ( 0.007781995580012663651, 0.000000000000000000, -0.9999697198139515519 ) ) ;
#5231=ORIENTED_EDGE ( 'NONE', *, *, #20545, .T. ) ;
#5232=PLANE ( 'NONE',  #233 ) ;
#5234=ORIENTED_EDGE ( 'NONE', *, *, #27983, .T. ) ;
#5235=EDGE_CURVE ( 'NONE', #33148, #13801, #42373, .T. ) ;
#5236=ORIENTED_EDGE ( 'NONE', *, *, #18610, .T. ) ;
#5237=VECTOR ( 'NONE', #26029, 999.9999999999998863 ) ;
#5238=ORIENTED_EDGE ( 'NONE', *, *, #730, .F. ) ;
#5239=ORIENTED_EDGE ( 'NONE', *, *, #32639, .T. ) ;
#5240=FACE_OUTER_BOUND ( 'NONE', #8591, .T. ) ;
#5241=EDGE_LOOP ( 'NONE', ( #47600, #15520, #23028, #38428 ) ) ;
#5243=DIRECTION ( 'NONE',  ( 0.007781995580012663651, -3.146120232559066537E-19, -0.9999697198139514409 ) ) ;
#5244=EDGE_CURVE ( 'NONE', #38808, #44862, #47168, .T. ) ;
#5245=AXIS2_PLACEMENT_3D ( 'NONE', #32677, #32965, #24179 ) ;
#5246=ORIENTED_EDGE ( 'NONE', *, *, #5360, .T. ) ;
#5247=LINE ( 'NONE', #39304, #54899 ) ;
#5248=ORIENTED_EDGE ( 'NONE', *, *, #44490, .T. ) ;
#5249=PLANE ( 'NONE',  #35628 ) ;
#5250=ORIENTED_EDGE ( 'NONE', *, *, #21287, .F. ) ;
#5251=EDGE_CURVE ( 'NONE', #33592, #45853, #3463, .T. ) ;
#5252=LINE ( 'NONE', #22559, #38270 ) ;
#5253=DIRECTION ( 'NONE',  ( -0.9999697198139514409, -0.000000000000000000, -0.007781995580013368816 ) ) ;
#5254=FACE_OUTER_BOUND ( 'NONE', #45192, .T. ) ;
#5255=CARTESIAN_POINT ( 'NONE',  ( -23.33849165029409889, 0.000000000000000000, 5.946783852668351855 ) ) ;
#5256=DIRECTION ( 'NONE',  ( 0.7660212471507180654, -0.6427876096865404731, 0.005961354470445141482 ) ) ;
#5257=LINE ( 'NONE', #31367, #18370 ) ;
#5258=ORIENTED_EDGE ( 'NONE', *, *, #53760, .T. ) ;
#5259=ORIENTED_EDGE ( 'NONE', *, *, #14393, .T. ) ;
#5260=CARTESIAN_POINT ( 'NONE',  ( -12.30734625917730085, 0.000000000000000000, 7.679285069618262405 ) ) ;
#5261=DIRECTION ( 'NONE',  ( 0.005961354470445682716, -0.6427876096865404731, -0.7660212471507180654 ) ) ;
#5262=CARTESIAN_POINT ( 'NONE',  ( -11.87243407472968926, 0.000000000000000000, 11.50246268866867361 ) ) ;
#5263=DIRECTION ( 'NONE',  ( 0.007781995580012662783, 0.000000000000000000, -0.9999697198139514409 ) ) ;
#5264=EDGE_LOOP ( 'NONE', ( #3833, #43863, #8611, #53821 ) ) ;
#5266=CARTESIAN_POINT ( 'NONE',  ( -28.93060053386082231, -0.1191753592594197858, 8.019254159017428663 ) ) ;
#5267=EDGE_LOOP ( 'NONE', ( #11711, #23640, #37389, #37561 ) ) ;
#5268=CARTESIAN_POINT ( 'NONE',  ( -9.442067484779661513, -0.1191753592594197858, 10.59804618892231254 ) ) ;
#5269=CARTESIAN_POINT ( 'NONE',  ( -14.63783524950929404, 0.000000000000000000, 8.599818861256533609 ) ) ;
#5270=ORIENTED_EDGE ( 'NONE', *, *, #51039, .T. ) ;
#5272=CARTESIAN_POINT ( 'NONE',  ( -17.44488905577733817, -5.213152330870661544, 12.01379018200878512 ) ) ;
#5273=ADVANCED_FACE ( 'NONE', ( #25326 ), #25590, .F. ) ;
#5274=CARTESIAN_POINT ( 'NONE',  ( -10.41431002974956321, 0.000000000000000000, 3.262032277597125773 ) ) ;
#5276=LINE ( 'NONE', #22587, #40110 ) ;
#5277=VERTEX_POINT ( 'NONE', #17 ) ;
#5278=ORIENTED_EDGE ( 'NONE', *, *, #44157, .F. ) ;
#5279=CARTESIAN_POINT ( 'NONE',  ( -10.47421230394850866, 0.000000000000000000, 10.95934586908605723 ) ) ;
#5280=CARTESIAN_POINT ( 'NONE',  ( -15.88130887279446490, 0.000000000000000000, 3.050160814894388839 ) ) ;
#5281=CARTESIAN_POINT ( 'NONE',  ( -19.32961685222932147, 0.000000000000000000, 14.39908572644263351 ) ) ;
#5282=EDGE_CURVE ( 'NONE', #34792, #24768, #39210, .T. ) ;
#5283=VECTOR ( 'NONE', #25710, 999.9999999999998863 ) ;
#5284=FACE_OUTER_BOUND ( 'NONE', #10109, .T. ) ;
#5285=DIRECTION ( 'NONE',  ( 0.5364919789714477361, 0.6444004775717706579, 0.5449076811759711036 ) ) ;
#5286=ORIENTED_EDGE ( 'NONE', *, *, #44268, .F. ) ;
#5287=LINE ( 'NONE', #40490, #9244 ) ;
#5288=LINE ( 'NONE', #43350, #12062 ) ;
#5289=EDGE_CURVE ( 'NONE', #25391, #40382, #30966, .T. ) ;
#5290=PLANE ( 'NONE',  #18715 ) ;
#5291=DIRECTION ( 'NONE',  ( -0.005961354470445682716, -0.6427876096865404731, 0.7660212471507180654 ) ) ;
#5293=FACE_OUTER_BOUND ( 'NONE', #53876, .T. ) ;
#5294=EDGE_LOOP ( 'NONE', ( #32492, #21844, #14852, #50467 ) ) ;
#5295=DIRECTION ( 'NONE',  ( 0.5449076811759707706, 0.6444004775717708799, -0.5364919789714476250 ) ) ;
#5296=DIRECTION ( 'NONE',  ( -0.005961354470445682716, -0.6427876096865404731, 0.7660212471507180654 ) ) ;
#5297=ORIENTED_EDGE ( 'NONE', *, *, #29418, .F. ) ;
#5298=LINE ( 'NONE', #22610, #52621 ) ;
#5299=EDGE_CURVE ( 'NONE', #36106, #1914, #31562, .T. ) ;
#5300=ORIENTED_EDGE ( 'NONE', *, *, #21017, .T. ) ;
#5301=ADVANCED_FACE ( 'NONE', ( #40343 ), #44586, .F. ) ;
#5302=ORIENTED_EDGE ( 'NONE', *, *, #44378, .T. ) ;
#5303=ORIENTED_EDGE ( 'NONE', *, *, #17504, .F. ) ;
#5304=CARTESIAN_POINT ( 'NONE',  ( -27.99845268667336384, -0.1191753592594197858, 7.657176279295684118 ) ) ;
#5305=VERTEX_POINT ( 'NONE', #14505 ) ;
#5306=ORIENTED_EDGE ( 'NONE', *, *, #46940, .T. ) ;
#5308=DIRECTION ( 'NONE',  ( 0.5364919789714477361, 0.6444004775717706579, 0.5449076811759711036 ) ) ;
#5309=VERTEX_POINT ( 'NONE', #10240 ) ;
#5310=ADVANCED_FACE ( 'NONE', ( #35518 ), #34984, .F. ) ;
#5311=ORIENTED_EDGE ( 'NONE', *, *, #38030, .F. ) ;
#5312=FACE_OUTER_BOUND ( 'NONE', #23302, .T. ) ;
#5313=ORIENTED_EDGE ( 'NONE', *, *, #47830, .F. ) ;
#5314=EDGE_LOOP ( 'NONE', ( #28668, #49703, #13798, #28861 ) ) ;
#5315=ADVANCED_FACE ( 'NONE', ( #9399 ), #48588, .F. ) ;
#5316=DIRECTION ( 'NONE',  ( 0.5364919789714477361, 0.6444004775717706579, 0.5449076811759711036 ) ) ;
#5317=DIRECTION ( 'NONE',  ( 0.000000000000000000, -0.000000000000000000, -1.000000000000000000 ) ) ;
#5318=FACE_OUTER_BOUND ( 'NONE', #10834, .T. ) ;
#5319=CARTESIAN_POINT ( 'NONE',  ( -21.29465867747552110, 2.391131607591507446, 9.077144048833369894 ) ) ;
#5320=ORIENTED_EDGE ( 'NONE', *, *, #13526, .F. ) ;
#5321=LINE ( 'NONE', #44221, #11950 ) ;
#5322=ORIENTED_EDGE ( 'NONE', *, *, #40791, .F. ) ;
#5323=VECTOR ( 'NONE', #24870, 999.9999999999998863 ) ;
#5324=PLANE ( 'NONE',  #38401 ) ;
#5325=DIRECTION ( 'NONE',  ( 0.000000000000000000, -1.000000000000000000, 0.000000000000000000 ) ) ;
#5326=CARTESIAN_POINT ( 'NONE',  ( -14.10280672071693431, -0.1191753592594197858, 12.40843558753103792 ) ) ;
#5327=DIRECTION ( 'NONE',  ( -0.9999697198139514409, -0.000000000000000000, -0.007781995580013368816 ) ) ;
#5328=LINE ( 'NONE', #43637, #33968 ) ;
#5329=CARTESIAN_POINT ( 'NONE',  ( -6.132980432523989833, 5.992972315187304666, 5.600631452548297418 ) ) ;
#5330=CARTESIAN_POINT ( 'NONE',  ( -13.11153479888853468, -0.1191753592594190225, 4.449041088301757263 ) ) ;
#5331=VERTEX_POINT ( 'NONE', #35816 ) ;
#5332=LINE ( 'NONE', #27757, #22004 ) ;
#5333=EDGE_CURVE ( 'NONE', #50963, #24424, #26717, .T. ) ;
#5334=DIRECTION ( 'NONE',  ( 0.9999697198139515519, 0.000000000000000000, 0.007781995580013368816 ) ) ;
#5335=PLANE ( 'NONE',  #52289 ) ;
#5336=LINE ( 'NONE', #14967, #19062 ) ;
#5337=EDGE_CURVE ( 'NONE', #21088, #41034, #613, .T. ) ;
#5339=DIRECTION ( 'NONE',  ( -0.5364919789714478471, 0.6444004775717705469, -0.5449076811759709926 ) ) ;
#5340=LINE ( 'NONE', #22084, #45891 ) ;
#5341=CARTESIAN_POINT ( 'NONE',  ( -17.54698502803930893, -4.241740624735659715, 10.45919562112636747 ) ) ;
#5342=ADVANCED_FACE ( 'NONE', ( #14249 ), #23027, .F. ) ;
#5343=VERTEX_POINT ( 'NONE', #35262 ) ;
#5344=EDGE_CURVE ( 'NONE', #20170, #13159, #52556, .T. ) ;
#5345=DIRECTION ( 'NONE',  ( -0.5364919789714478471, 0.6444004775717705469, -0.5449076811759709926 ) ) ;
#5346=DIRECTION ( 'NONE',  ( 0.000000000000000000, -1.000000000000000000, 0.000000000000000000 ) ) ;
#5347=DIRECTION ( 'NONE',  ( -0.7660212471507179544, -0.6427876096865405842, -0.005961354470445141482 ) ) ;
#5348=EDGE_CURVE ( 'NONE', #41657, #34394, #30719, .T. ) ;
#5349=EDGE_CURVE ( 'NONE', #55849, #12500, #48022, .T. ) ;
#5350=EDGE_CURVE ( 'NONE', #16795, #25477, #26429, .T. ) ;
#5352=CARTESIAN_POINT ( 'NONE',  ( -9.300968958747018789, 0.000000000000000000, 5.317362960500759961 ) ) ;
#5353=DIRECTION ( 'NONE',  ( 0.007781995580012663651, 0.000000000000000000, -0.9999697198139515519 ) ) ;
#5354=CARTESIAN_POINT ( 'NONE',  ( -16.81267852042391198, -0.1191753592594197858, 3.312241722634738039 ) ) ;
#5355=FACE_OUTER_BOUND ( 'NONE', #8662, .T. ) ;
#5356=DIRECTION ( 'NONE',  ( 0.5364919789714477361, 0.6444004775717706579, 0.5449076811759711036 ) ) ;
#5357=VECTOR ( 'NONE', #6039, 1000.000000000000227 ) ;
#5358=ORIENTED_EDGE ( 'NONE', *, *, #46368, .F. ) ;
#5359=EDGE_CURVE ( 'NONE', #22392, #11173, #52824, .T. ) ;
#5360=EDGE_CURVE ( 'NONE', #32296, #33683, #13936, .T. ) ;
#5361=ORIENTED_EDGE ( 'NONE', *, *, #31135, .F. ) ;
#5362=ORIENTED_EDGE ( 'NONE', *, *, #34330, .T. ) ;
#5363=ORIENTED_EDGE ( 'NONE', *, *, #38203, .F. ) ;
#5364=ADVANCED_FACE ( 'NONE', ( #18786 ), #31262, .F. ) ;
#5365=ORIENTED_EDGE ( 'NONE', *, *, #12607, .T. ) ;
#5366=CARTESIAN_POINT ( 'NONE',  ( -16.76234344414121580, 0.000000000000000000, 8.752611460827463219 ) ) ;
#5367=DIRECTION ( 'NONE',  ( 0.7660212471507180654, -0.6427876096865404731, 0.005961354470445141482 ) ) ;
#5368=EDGE_CURVE ( 'NONE', #50886, #40382, #18474, .T. ) ;
#5369=ORIENTED_EDGE ( 'NONE', *, *, #31371, .F. ) ;
#5370=VERTEX_POINT ( 'NONE', #7581 ) ;
#5371=FACE_OUTER_BOUND ( 'NONE', #49986, .T. ) ;
#5372=ORIENTED_EDGE ( 'NONE', *, *, #44379, .F. ) ;
#5374=CARTESIAN_POINT ( 'NONE',  ( -15.35639454250681801, -3.917936722690662954, 2.721263568740423189 ) ) ;
#5375=VERTEX_POINT ( 'NONE', #55553 ) ;
#5376=DIRECTION ( 'NONE',  ( 0.005002170337468016433, -0.7660444431189770143, -0.6427681459581293666 ) ) ;
#5377=ORIENTED_EDGE ( 'NONE', *, *, #35224, .F. ) ;
#5378=CARTESIAN_POINT ( 'NONE',  ( 2.072287782118878319, 0.000000000000000000, -2.950529333540147015 ) ) ;
#5379=DIRECTION ( 'NONE',  ( -0.3620778797217456546, 0.000000000000000000, -0.9321478471874540261 ) ) ;
#5380=CARTESIAN_POINT ( 'NONE',  ( -20.75985484760730060, 4.010151117816511679, 4.617819545835347483 ) ) ;
#5381=CARTESIAN_POINT ( 'NONE',  ( -17.74560456716937296, 0.000000000000000000, 3.774316574337878372 ) ) ;
#5383=CARTESIAN_POINT ( 'NONE',  ( -11.97215022127920392, -1.003701604285657911, 1.499687502927729010 ) ) ;
#5384=CARTESIAN_POINT ( 'NONE',  ( -9.298094905241734764, 0.000000000000000000, 4.948053257242996494 ) ) ;
#5385=DIRECTION ( 'NONE',  ( 0.7660212471507180654, -0.6427876096865404731, 0.005961354470445141482 ) ) ;
#5386=ORIENTED_EDGE ( 'NONE', *, *, #6314, .F. ) ;
#5387=DIRECTION ( 'NONE',  ( 0.5364919789714477361, 0.6444004775717706579, 0.5449076811759711036 ) ) ;
#5390=DIRECTION ( 'NONE',  ( -0.5364919789714478471, 0.6444004775717705469, -0.5449076811759709926 ) ) ;
#5391=FACE_OUTER_BOUND ( 'NONE', #5553, .T. ) ;
#5392=CARTESIAN_POINT ( 'NONE',  ( -23.33771345073609638, -0.1191753592594197858, 5.846786880686956955 ) ) ;
#5393=CARTESIAN_POINT ( 'NONE',  ( -16.33317936670417225, 0.000000000000000000, 13.31440848639340224 ) ) ;
#5394=PLANE ( 'NONE',  #55846 ) ;
#5395=DIRECTION ( 'NONE',  ( -0.005002170337468016433, -0.7660444431189770143, 0.6427681459581293666 ) ) ;
#5396=DIRECTION ( 'NONE',  ( 0.6427681459581294776, -0.7660444431189769032, 0.005002170337467562802 ) ) ;
#5397=DIRECTION ( 'NONE',  ( -0.005002170337468016433, -0.7660444431189770143, 0.6427681459581293666 ) ) ;
#5399=LINE ( 'NONE', #22708, #27806 ) ;
#5400=EDGE_LOOP ( 'NONE', ( #6954, #33903, #48942, #54106 ) ) ;
#5401=DIRECTION ( 'NONE',  ( 0.007781995580012663651, 0.000000000000000000, -0.9999697198139515519 ) ) ;
#5402=DIRECTION ( 'NONE',  ( 0.007781995580012663651, 0.000000000000000000, -0.9999697198139515519 ) ) ;
#5403=PLANE ( 'NONE',  #35410 ) ;
#5404=DIRECTION ( 'NONE',  ( -0.5364919789714478471, 0.6444004775717705469, -0.5449076811759709926 ) ) ;
#5405=EDGE_CURVE ( 'NONE', #47531, #51306, #16660, .T. ) ;
#5406=EDGE_CURVE ( 'NONE', #6150, #27710, #3336, .T. ) ;
#5407=DIRECTION ( 'NONE',  ( 0.9999697198139515519, 0.000000000000000000, 0.007781995580013368816 ) ) ;
#5408=EDGE_CURVE ( 'NONE', #18340, #54304, #11829, .T. ) ;
#5409=FACE_OUTER_BOUND ( 'NONE', #3659, .T. ) ;
#5410=DIRECTION ( 'NONE',  ( 0.6427681459581294776, -0.7660444431189769032, 0.005002170337467562802 ) ) ;
#5411=ORIENTED_EDGE ( 'NONE', *, *, #47305, .T. ) ;
#5412=VERTEX_POINT ( 'NONE', #32854 ) ;
#5414=CARTESIAN_POINT ( 'NONE',  ( -15.13495153988577968, 0.000000000000000000, 12.76973526769478084 ) ) ;
#5415=ORIENTED_EDGE ( 'NONE', *, *, #19914, .F. ) ;
#5416=DIRECTION ( 'NONE',  ( -0.005961354470445682716, -0.6427876096865404731, 0.7660212471507180654 ) ) ;
#5417=ORIENTED_EDGE ( 'NONE', *, *, #22124, .T. ) ;
#5418=DIRECTION ( 'NONE',  ( 0.3313982828793700097, 0.4028455766673916805, 0.8531650599175528704 ) ) ;
#5419=EDGE_CURVE ( 'NONE', #26758, #9638, #20656, .T. ) ;
#5420=ORIENTED_EDGE ( 'NONE', *, *, #22951, .T. ) ;
#5421=ORIENTED_EDGE ( 'NONE', *, *, #52601, .F. ) ;
#5422=ORIENTED_EDGE ( 'NONE', *, *, #3492, .T. ) ;
#5424=CARTESIAN_POINT ( 'NONE',  ( -10.74029228357944987, 0.000000000000000000, 11.14194120806293320 ) ) ;
#5425=CARTESIAN_POINT ( 'NONE',  ( -13.53673582514181106, 0.000000000000000000, 12.22817484722816772 ) ) ;
#5426=DIRECTION ( 'NONE',  ( -0.7660212471507179544, -0.6427876096865405842, -0.005961354470445141482 ) ) ;
#5427=EDGE_CURVE ( 'NONE', #33190, #36986, #24907, .T. ) ;
#5428=CARTESIAN_POINT ( 'NONE',  ( -26.13493519185646008, 0.000000000000000000, 7.033017491833586377 ) ) ;
#5429=ORIENTED_EDGE ( 'NONE', *, *, #4088, .F. ) ;
#5430=ORIENTED_EDGE ( 'NONE', *, *, #54776, .F. ) ;
#5431=ADVANCED_FACE ( 'NONE', ( #55278 ), #16112, .F. ) ;
#5433=ORIENTED_EDGE ( 'NONE', *, *, #55489, .T. ) ;
#5434=CARTESIAN_POINT ( 'NONE',  ( -18.67775241435682432, 0.000000000000000000, 4.136394454059623804 ) ) ;
#5435=ORIENTED_EDGE ( 'NONE', *, *, #29401, .T. ) ;
#5436=CARTESIAN_POINT ( 'NONE',  ( -15.20077793328688820, 0.000000000000000000, 2.686124794216351308 ) ) ;
#5437=PLANE ( 'NONE',  #20353 ) ;
#5438=ORIENTED_EDGE ( 'NONE', *, *, #53652, .T. ) ;
#5439=LINE ( 'NONE', #27286, #3231 ) ;
#5440=EDGE_LOOP ( 'NONE', ( #39725, #46621, #23708, #19308 ) ) ;
#5441=CARTESIAN_POINT ( 'NONE',  ( -17.18728735815524544, 3.038739411681508518, 8.544536277294087157 ) ) ;
#5442=ORIENTED_EDGE ( 'NONE', *, *, #18135, .F. ) ;
#5443=DIRECTION ( 'NONE',  ( -0.7660212471507179544, -0.6427876096865405842, -0.005961354470445141482 ) ) ;
#5444=CARTESIAN_POINT ( 'NONE',  ( -15.88130887279446490, 0.000000000000000000, 3.050160814894388839 ) ) ;
#5445=CARTESIAN_POINT ( 'NONE',  ( -16.79925329029790149, 0.000000000000000000, 13.49544742625427496 ) ) ;
#5446=EDGE_LOOP ( 'NONE', ( #45412, #6756, #35669, #45940 ) ) ;
#5447=LINE ( 'NONE', #40661, #3803 ) ;
#5448=LINE ( 'NONE', #23054, #31271 ) ;
#5449=CARTESIAN_POINT ( 'NONE',  ( -15.52399824061222589, 0.000000000000000000, 3.052941488854047591 ) ) ;
#5450=CARTESIAN_POINT ( 'NONE',  ( -21.47419595591918906, 0.000000000000000000, 5.222628093224860102 ) ) ;
#5451=LINE ( 'NONE', #898, #36094 ) ;
#5454=ORIENTED_EDGE ( 'NONE', *, *, #49173, .F. ) ;
#5455=LINE ( 'NONE', #27600, #9866 ) ;
#5456=DIRECTION ( 'NONE',  ( -0.5449076811759708816, 0.6444004775717707689, 0.5364919789714475140 ) ) ;
#5457=CARTESIAN_POINT ( 'NONE',  ( -9.485036236067394100, 0.000000000000000000, 3.269264101133144695 ) ) ;
#5458=ORIENTED_EDGE ( 'NONE', *, *, #44379, .T. ) ;
#5459=DIRECTION ( 'NONE',  ( 0.6427681459581294776, -0.7660444431189769032, 0.005002170337467562802 ) ) ;
#5460=CARTESIAN_POINT ( 'NONE',  ( -16.06709938707323460, 0.000000000000000000, 13.13181314741652628 ) ) ;
#5461=EDGE_LOOP ( 'NONE', ( #977, #16102, #10393, #24899 ) ) ;
#5462=ADVANCED_FACE ( 'NONE', ( #28893 ), #12430, .F. ) ;
#5463=FACE_OUTER_BOUND ( 'NONE', #27212, .T. ) ;
#5464=CARTESIAN_POINT ( 'NONE',  ( -11.12303075984975109, 1.419719901456505617, 0.9571981204249864206 ) ) ;
#5466=EDGE_CURVE ( 'NONE', #39497, #1446, #47049, .T. ) ;
#5467=CARTESIAN_POINT ( 'NONE',  ( -14.46888367232926420, 0.000000000000000000, 12.59025272694991315 ) ) ;
#5468=DIRECTION ( 'NONE',  ( 0.005961354470445682716, -0.6427876096865404731, -0.7660212471507180654 ) ) ;
#5469=ORIENTED_EDGE ( 'NONE', *, *, #8754, .F. ) ;
#5470=ORIENTED_EDGE ( 'NONE', *, *, #35942, .T. ) ;
#5471=CARTESIAN_POINT ( 'NONE',  ( -20.44450923172429668, 1.419719901456506728, 4.577976917642439858 ) ) ;
#5472=CARTESIAN_POINT ( 'NONE',  ( -20.54126990917373874, -0.1191753592594138877, 4.760553241521714440 ) ) ;
#5473=DIRECTION ( 'NONE',  ( 0.007781995580012663651, -3.146120232559066537E-19, -0.9999697198139514409 ) ) ;
#5474=DIRECTION ( 'NONE',  ( 0.005002170337468016433, -0.7660444431189770143, -0.6427681459581293666 ) ) ;
#5475=PLANE ( 'NONE',  #28315 ) ;
#5476=PLANE ( 'NONE',  #51195 ) ;
#5478=DIRECTION ( 'NONE',  ( 0.7660212471507180654, -0.6427876096865404731, 0.005961354470445141482 ) ) ;
#5479=DIRECTION ( 'NONE',  ( 0.005961354470445682716, -0.6427876096865404731, -0.7660212471507180654 ) ) ;
#5480=ORIENTED_EDGE ( 'NONE', *, *, #21309, .F. ) ;
#5481=DIRECTION ( 'NONE',  ( 0.005002170337468016433, -0.7660444431189770143, -0.6427681459581293666 ) ) ;
#5482=LINE ( 'NONE', #47826, #24081 ) ;
#5483=LINE ( 'NONE', #40118, #49284 ) ;
#5484=ORIENTED_EDGE ( 'NONE', *, *, #29952, .F. ) ;
#5485=DIRECTION ( 'NONE',  ( -0.6427681459581293666, -0.7660444431189770143, -0.005002170337467561935 ) ) ;
#5487=EDGE_CURVE ( 'NONE', #46187, #40733, #46772, .T. ) ;
#5488=AXIS2_PLACEMENT_3D ( 'NONE', #48906, #33955, #22229 ) ;
#5490=VERTEX_POINT ( 'NONE', #50476 ) ;
#5491=ADVANCED_FACE ( 'NONE', ( #55019 ), #3602, .F. ) ;
#5492=EDGE_LOOP ( 'NONE', ( #11348, #53541, #24500, #55607 ) ) ;
#5493=PLANE ( 'NONE',  #32091 ) ;
#5494=EDGE_CURVE ( 'NONE', #52808, #44596, #2487, .T. ) ;
#5495=ORIENTED_EDGE ( 'NONE', *, *, #35313, .F. ) ;
#5496=DIRECTION ( 'NONE',  ( -0.7660212471507179544, -0.6427876096865405842, -0.005961354470445141482 ) ) ;
#5497=CARTESIAN_POINT ( 'NONE',  ( -23.33849165029409889, 0.000000000000000000, 5.946783852668351855 ) ) ;
#5498=EDGE_LOOP ( 'NONE', ( #34651, #3347, #4109, #3386 ) ) ;
#5499=CARTESIAN_POINT ( 'NONE',  ( -15.73389624039720580, 0.000000000000000000, 9.329953200799501190 ) ) ;
#5500=EDGE_CURVE ( 'NONE', #21894, #4790, #2734, .T. ) ;
#5501=VERTEX_POINT ( 'NONE', #11278 ) ;
#5502=DIRECTION ( 'NONE',  ( 0.9999697198139515519, 0.000000000000000000, 0.007781995580013368816 ) ) ;
#5503=VERTEX_POINT ( 'NONE', #28610 ) ;
#5504=DIRECTION ( 'NONE',  ( 0.005961354470445682716, -0.6427876096865404731, -0.7660212471507180654 ) ) ;
#5505=PLANE ( 'NONE',  #25678 ) ;
#5506=LINE ( 'NONE', #44145, #23236 ) ;
#5507=DIRECTION ( 'NONE',  ( 0.9999697198139515519, 0.000000000000000000, 0.007781995580013368816 ) ) ;
#5508=DIRECTION ( 'NONE',  ( 0.005961354470445682716, -0.6427876096865404731, -0.7660212471507180654 ) ) ;
#5510=ORIENTED_EDGE ( 'NONE', *, *, #1356, .F. ) ;
#5511=ORIENTED_EDGE ( 'NONE', *, *, #51380, .T. ) ;
#5512=AXIS2_PLACEMENT_3D ( 'NONE', #10734, #41384, #11562 ) ;
#5513=PLANE ( 'NONE',  #20984 ) ;
#5514=LINE ( 'NONE', #40730, #34852 ) ;
#5515=EDGE_CURVE ( 'NONE', #6270, #24207, #45935, .T. ) ;
#5516=DIRECTION ( 'NONE',  ( 0.5449076811759707706, 0.6444004775717708799, -0.5364919789714476250 ) ) ;
#5517=CARTESIAN_POINT ( 'NONE',  ( -18.67619601524082285, 0.000000000000000000, 3.936400510096834893 ) ) ;
#5518=ORIENTED_EDGE ( 'NONE', *, *, #28799, .F. ) ;
#5519=DIRECTION ( 'NONE',  ( -0.6427681459581293666, -0.7660444431189770143, -0.005002170337467561935 ) ) ;
#5520=CARTESIAN_POINT ( 'NONE',  ( -15.88130887279446490, 0.000000000000000000, 3.050160814894388839 ) ) ;
#5521=ORIENTED_EDGE ( 'NONE', *, *, #30632, .T. ) ;
#5522=FACE_OUTER_BOUND ( 'NONE', #43462, .T. ) ;
#5523=EDGE_CURVE ( 'NONE', #26368, #6316, #41649, .T. ) ;
#5524=LINE ( 'NONE', #31387, #11328 ) ;
#5525=ORIENTED_EDGE ( 'NONE', *, *, #46707, .T. ) ;
#5526=DIRECTION ( 'NONE',  ( 0.007781995580012663651, -3.146120232559066537E-19, -0.9999697198139514409 ) ) ;
#5527=DIRECTION ( 'NONE',  ( 0.5449076811759707706, 0.6444004775717708799, -0.5364919789714476250 ) ) ;
#5528=AXIS2_PLACEMENT_3D ( 'NONE', #19623, #54255, #28405 ) ;
#5529=EDGE_CURVE ( 'NONE', #5490, #52907, #7291, .T. ) ;
#5530=CARTESIAN_POINT ( 'NONE',  ( -13.07066190154808361, 0.000000000000000000, 12.04713590736729678 ) ) ;
#5531=EDGE_CURVE ( 'NONE', #42246, #41830, #38523, .T. ) ;
#5532=CARTESIAN_POINT ( 'NONE',  ( 2.072287782118878319, 0.000000000000000000, -2.950529333540147015 ) ) ;
#5533=VECTOR ( 'NONE', #3641, 999.9999999999998863 ) ;
#5534=LINE ( 'NONE', #31671, #6587 ) ;
#5535=VERTEX_POINT ( 'NONE', #21769 ) ;
#5536=ORIENTED_EDGE ( 'NONE', *, *, #51283, .F. ) ;
#5537=DIRECTION ( 'NONE',  ( -0.005961354470445682716, -0.6427876096865404731, 0.7660212471507180654 ) ) ;
#5538=PLANE ( 'NONE',  #9554 ) ;
#5539=DIRECTION ( 'NONE',  ( -0.6427681459581293666, -0.7660444431189770143, -0.005002170337467561935 ) ) ;
#5540=CARTESIAN_POINT ( 'NONE',  ( -15.89935617993504913, -0.1191753592594213540, 4.427345617693702273 ) ) ;
#5541=CARTESIAN_POINT ( 'NONE',  ( -12.13851405436063047, 0.000000000000000000, 11.68505802764555135 ) ) ;
#5542=ORIENTED_EDGE ( 'NONE', *, *, #47970, .T. ) ;
#5544=DIRECTION ( 'NONE',  ( 0.005002170337468016433, -0.7660444431189770143, -0.6427681459581293666 ) ) ;
#5545=EDGE_CURVE ( 'NONE', #7363, #29459, #30847, .T. ) ;
#5546=PLANE ( 'NONE',  #23255 ) ;
#5548=EDGE_LOOP ( 'NONE', ( #13659, #55595, #11651, #54303 ) ) ;
#5549=DIRECTION ( 'NONE',  ( 0.3313982828793700097, 0.4028455766673915694, 0.8531650599175529814 ) ) ;
#5550=ORIENTED_EDGE ( 'NONE', *, *, #2270, .F. ) ;
#5551=DIRECTION ( 'NONE',  ( -0.6427681459581293666, -0.7660444431189770143, -0.005002170337467561935 ) ) ;
#5552=CARTESIAN_POINT ( 'NONE',  ( -19.60834386242827776, 0.000000000000000000, 4.298478389818581213 ) ) ;
#5553=EDGE_LOOP ( 'NONE', ( #27049, #14418, #43549, #2197 ) ) ;
#5554=AXIS2_PLACEMENT_3D ( 'NONE', #20105, #46823, #16154 ) ;
#5555=AXIS2_PLACEMENT_3D ( 'NONE', #7309, #55037, #45647 ) ;
#5556=CARTESIAN_POINT ( 'NONE',  ( -10.37421533196711465, -0.1191753592594197858, 10.96012406864405975 ) ) ;
#5557=ORIENTED_EDGE ( 'NONE', *, *, #22662, .T. ) ;
#5558=ORIENTED_EDGE ( 'NONE', *, *, #23447, .T. ) ;
#5559=ORIENTED_EDGE ( 'NONE', *, *, #27794, .T. ) ;
#5562=ORIENTED_EDGE ( 'NONE', *, *, #20447, .F. ) ;
#5563=DIRECTION ( 'NONE',  ( 0.000000000000000000, -0.000000000000000000, -1.000000000000000000 ) ) ;
#5564=DIRECTION ( 'NONE',  ( 0.5364919789714477361, 0.6444004775717706579, 0.5449076811759711036 ) ) ;
#5565=ORIENTED_EDGE ( 'NONE', *, *, #23424, .T. ) ;
#5566=ORIENTED_EDGE ( 'NONE', *, *, #46147, .T. ) ;
#5567=DIRECTION ( 'NONE',  ( -0.5449076811759708816, 0.6444004775717707689, 0.5364919789714475140 ) ) ;
#5568=ADVANCED_FACE ( 'NONE', ( #56134 ), #38825, .F. ) ;
#5570=VERTEX_POINT ( 'NONE', #4185 ) ;
#5571=VECTOR ( 'NONE', #16742, 999.9999999999998863 ) ;
#5572=DIRECTION ( 'NONE',  ( 0.7660212471507180654, -0.6427876096865404731, 0.005961354470445141482 ) ) ;
#5573=DIRECTION ( 'NONE',  ( 0.7660212471507180654, -0.6427876096865404731, 0.005961354470445141482 ) ) ;
#5574=CARTESIAN_POINT ( 'NONE',  ( -11.73486842939697006, -0.1191753592594185784, 6.675747043152371774 ) ) ;
#5575=PLANE ( 'NONE',  #23242 ) ;
#5576=ORIENTED_EDGE ( 'NONE', *, *, #36228, .F. ) ;
#5577=DIRECTION ( 'NONE',  ( -0.9999697198139514409, -0.000000000000000000, -0.007781995580013368816 ) ) ;
#5578=ORIENTED_EDGE ( 'NONE', *, *, #31690, .T. ) ;
#5579=EDGE_CURVE ( 'NONE', #12964, #18005, #51852, .T. ) ;
#5580=DIRECTION ( 'NONE',  ( 0.5364919789714477361, 0.6444004775717706579, 0.5449076811759711036 ) ) ;
#5581=EDGE_CURVE ( 'NONE', #19391, #51083, #12691, .T. ) ;
#5582=ADVANCED_FACE ( 'NONE', ( #34540 ), #4462, .F. ) ;
#5583=DIRECTION ( 'NONE',  ( -0.6427681459581293666, -0.7660444431189770143, -0.005002170337467561935 ) ) ;
#5584=DIRECTION ( 'NONE',  ( 0.007781995580012663651, 0.000000000000000000, -0.9999697198139515519 ) ) ;
#5585=CARTESIAN_POINT ( 'NONE',  ( -14.66887761629205222, 0.000000000000000000, 12.58869632783390990 ) ) ;
#5586=DIRECTION ( 'NONE',  ( 0.5364919789714477361, 0.6444004775717706579, 0.5449076811759711036 ) ) ;
#5587=LINE ( 'NONE', #36266, #48586 ) ;
#5588=ORIENTED_EDGE ( 'NONE', *, *, #53311, .F. ) ;
#5589=PLANE ( 'NONE',  #40164 ) ;
#5590=EDGE_CURVE ( 'NONE', #13391, #30427, #47314, .T. ) ;
#5592=VECTOR ( 'NONE', #35722, 1000.000000000000000 ) ;
#5593=AXIS2_PLACEMENT_3D ( 'NONE', #23122, #53755, #37021 ) ;
#5594=CARTESIAN_POINT ( 'NONE',  ( -9.110551994824897193, 0.000000000000000000, 3.538847790438064411 ) ) ;
#5595=LINE ( 'NONE', #22919, #39616 ) ;
#5596=EDGE_CURVE ( 'NONE', #30427, #10301, #18069, .T. ) ;
#5597=LINE ( 'NONE', #40548, #49871 ) ;
#5598=LINE ( 'NONE', #48481, #486 ) ;
#5599=ADVANCED_FACE ( 'NONE', ( #13533 ), #31122, .F. ) ;
#5600=CARTESIAN_POINT ( 'NONE',  ( -16.89084389517911688, -4.079838673713163111, 3.312130287550314911 ) ) ;
#5602=VECTOR ( 'NONE', #33868, 1000.000000000000227 ) ;
#5603=ORIENTED_EDGE ( 'NONE', *, *, #22061, .T. ) ;
#5605=DIRECTION ( 'NONE',  ( 0.005002170337468016433, -0.7660444431189770143, -0.6427681459581293666 ) ) ;
#5606=CARTESIAN_POINT ( 'NONE',  ( -13.08330893211609869, 0.000000000000000000, 1.763933231766363630 ) ) ;
#5607=EDGE_CURVE ( 'NONE', #17276, #904, #43902, .T. ) ;
#5609=LINE ( 'NONE', #28299, #11265 ) ;
#5610=PLANE ( 'NONE',  #26845 ) ;
#5611=DIRECTION ( 'NONE',  ( 0.7660212471507180654, -0.6427876096865404731, 0.005961354470445141482 ) ) ;
#5612=VECTOR ( 'NONE', #38111, 1000.000000000000227 ) ;
#5613=EDGE_CURVE ( 'NONE', #36877, #12432, #4727, .T. ) ;
#5614=CARTESIAN_POINT ( 'NONE',  ( -17.67592931590769112, 0.000000000000000000, 6.729515361707646193 ) ) ;
#5615=DIRECTION ( 'NONE',  ( 0.5449076811759707706, 0.6444004775717708799, -0.5364919789714476250 ) ) ;
#5616=VERTEX_POINT ( 'NONE', #34836 ) ;
#5617=ORIENTED_EDGE ( 'NONE', *, *, #28588, .T. ) ;
#5618=ORIENTED_EDGE ( 'NONE', *, *, #30492, .T. ) ;
#5619=ORIENTED_EDGE ( 'NONE', *, *, #8471, .T. ) ;
#5620=ORIENTED_EDGE ( 'NONE', *, *, #39320, .F. ) ;
#5621=CARTESIAN_POINT ( 'NONE',  ( -12.33850799832341849, 0.000000000000000000, 11.68350162852954632 ) ) ;
#5622=DIRECTION ( 'NONE',  ( -0.005961354470445682716, -0.6427876096865404731, 0.7660212471507180654 ) ) ;
#5623=AXIS2_PLACEMENT_3D ( 'NONE', #16163, #37761, #42828 ) ;
#5624=VECTOR ( 'NONE', #36125, 999.9999999999998863 ) ;
#5625=ORIENTED_EDGE ( 'NONE', *, *, #44018, .F. ) ;
#5626=EDGE_LOOP ( 'NONE', ( #12270, #18429, #24845, #18973 ) ) ;
#5627=EDGE_CURVE ( 'NONE', #31317, #43546, #12969, .T. ) ;
#5628=ORIENTED_EDGE ( 'NONE', *, *, #11680, .T. ) ;
#5629=EDGE_CURVE ( 'NONE', #33244, #48860, #30297, .T. ) ;
#5630=VECTOR ( 'NONE', #33261, 1000.000000000000227 ) ;
#5631=CARTESIAN_POINT ( 'NONE',  ( -15.40103151951671734, 0.000000000000000000, 12.95233060667165681 ) ) ;
#5632=DIRECTION ( 'NONE',  ( 0.007781995580012662783, 0.000000000000000000, -0.9999697198139514409 ) ) ;
#5633=PLANE ( 'NONE',  #41355 ) ;
#5634=ORIENTED_EDGE ( 'NONE', *, *, #26433, .T. ) ;
#5635=CARTESIAN_POINT ( 'NONE',  ( -26.13337879274045505, 0.000000000000000000, 6.833023547870798353 ) ) ;
#5636=ADVANCED_FACE ( 'NONE', ( #8734 ), #26053, .F. ) ;
#5637=EDGE_CURVE ( 'NONE', #54774, #53284, #5018, .T. ) ;
#5638=ORIENTED_EDGE ( 'NONE', *, *, #39578, .T. ) ;
#5639=LINE ( 'NONE', #36057, #43643 ) ;
#5640=VECTOR ( 'NONE', #55290, 1000.000000000000114 ) ;
#5641=CARTESIAN_POINT ( 'NONE',  ( -20.73421763976967114, -3.108426967578159950, 4.836020290795394416 ) ) ;
#5642=ADVANCED_FACE ( 'NONE', ( #42769 ), #8421, .F. ) ;
#5643=PLANE ( 'NONE',  #3726 ) ;
#5644=PLANE ( 'NONE',  #13348 ) ;
#5645=VERTEX_POINT ( 'NONE', #34285 ) ;
#5646=LINE ( 'NONE', #35467, #17661 ) ;
#5647=CARTESIAN_POINT ( 'NONE',  ( -32.65841372305263235, 0.000000000000000000, 9.367568705923016381 ) ) ;
#5648=CARTESIAN_POINT ( 'NONE',  ( -17.83139810946674686, -0.1191753592594197858, 13.85674710641801788 ) ) ;
#5649=ORIENTED_EDGE ( 'NONE', *, *, #3679, .F. ) ;
#5650=DIRECTION ( 'NONE',  ( -0.7660212471507179544, -0.6427876096865405842, -0.005961354470445141482 ) ) ;
#5651=VERTEX_POINT ( 'NONE', #51593 ) ;
#5652=DIRECTION ( 'NONE',  ( -0.5364919789714478471, 0.6444004775717705469, -0.5449076811759709926 ) ) ;
#5653=PLANE ( 'NONE',  #50415 ) ;
#5654=CARTESIAN_POINT ( 'NONE',  ( -13.27065584551087163, 0.000000000000000000, 12.04557950825129176 ) ) ;
#5655=EDGE_CURVE ( 'NONE', #27148, #20460, #49006, .T. ) ;
#5656=LINE ( 'NONE', #40858, #9653 ) ;
#5658=CARTESIAN_POINT ( 'NONE',  ( -15.40103151951671734, 0.000000000000000000, 12.95233060667165681 ) ) ;
#5659=FACE_OUTER_BOUND ( 'NONE', #3493, .T. ) ;
#5660=DIRECTION ( 'NONE',  ( -0.7660212471507179544, -0.6427876096865405842, -0.005961354470445141482 ) ) ;
#5661=EDGE_CURVE ( 'NONE', #45510, #52307, #53819, .T. ) ;
#5662=PLANE ( 'NONE',  #38420 ) ;
#5664=ADVANCED_FACE ( 'NONE', ( #32265 ), #1845, .F. ) ;
#5665=FACE_OUTER_BOUND ( 'NONE', #7153, .T. ) ;
#5666=VERTEX_POINT ( 'NONE', #48448 ) ;
#5667=AXIS2_PLACEMENT_3D ( 'NONE', #33359, #30205, #12879 ) ;
#5668=LINE ( 'NONE', #40612, #36611 ) ;
#5669=CARTESIAN_POINT ( 'NONE',  ( -10.69332325015427543, 0.000000000000000000, 5.106521281233943554 ) ) ;
#5670=CARTESIAN_POINT ( 'NONE',  ( -23.33849165029409889, 0.000000000000000000, 5.946783852668351855 ) ) ;
#5672=VECTOR ( 'NONE', #52739, 1000.000000000000227 ) ;
#5673=EDGE_CURVE ( 'NONE', #28952, #36269, #41036, .T. ) ;
#5674=VECTOR ( 'NONE', #51415, 999.9999999999998863 ) ;
#5675=LINE ( 'NONE', #54217, #33672 ) ;
#5676=DIRECTION ( 'NONE',  ( 0.005002170337468016433, -0.7660444431189770143, -0.6427681459581293666 ) ) ;
#5677=DIRECTION ( 'NONE',  ( 0.9999697198139515519, 0.000000000000000000, 0.007781995580013368816 ) ) ;
#5678=ORIENTED_EDGE ( 'NONE', *, *, #32768, .T. ) ;
#5679=VECTOR ( 'NONE', #6739, 999.9999999999998863 ) ;
#5680=VECTOR ( 'NONE', #24317, 1000.000000000000227 ) ;
#5681=ORIENTED_EDGE ( 'NONE', *, *, #46260, .T. ) ;
#5682=LINE ( 'NONE', #36629, #26861 ) ;
#5683=DIRECTION ( 'NONE',  ( 0.007781995580012662783, 0.000000000000000000, -0.9999697198139514409 ) ) ;
#5685=DIRECTION ( 'NONE',  ( -0.005961354470445682716, -0.6427876096865404731, 0.7660212471507180654 ) ) ;
#5686=VECTOR ( 'NONE', #20611, 1000.000000000000227 ) ;
#5687=ORIENTED_EDGE ( 'NONE', *, *, #3415, .F. ) ;
#5688=LINE ( 'NONE', #36932, #35674 ) ;
#5689=ORIENTED_EDGE ( 'NONE', *, *, #50119, .T. ) ;
#5690=VERTEX_POINT ( 'NONE', #49585 ) ;
#5691=ORIENTED_EDGE ( 'NONE', *, *, #6022, .T. ) ;
#5692=DIRECTION ( 'NONE',  ( 0.007781995580012663651, 0.000000000000000000, -0.9999697198139515519 ) ) ;
#5693=LINE ( 'NONE', #53136, #4197 ) ;
#5694=CARTESIAN_POINT ( 'NONE',  ( -17.74404816805336793, 0.000000000000000000, 3.574322630375089460 ) ) ;
#5697=DIRECTION ( 'NONE',  ( 0.9999697198139515519, 0.000000000000000000, 0.007781995580013368816 ) ) ;
#5698=ORIENTED_EDGE ( 'NONE', *, *, #29171, .F. ) ;
#5699=ADVANCED_FACE ( 'NONE', ( #14389 ), #31431, .F. ) ;
#5700=ORIENTED_EDGE ( 'NONE', *, *, #18864, .F. ) ;
#5701=VECTOR ( 'NONE', #28362, 1000.000000000000227 ) ;
#5702=LINE ( 'NONE', #52830, #25491 ) ;
#5703=VERTEX_POINT ( 'NONE', #44206 ) ;
#5704=VECTOR ( 'NONE', #41707, 999.9999999999998863 ) ;
#5705=DIRECTION ( 'NONE',  ( 0.005002170337468016433, -0.7660444431189770143, -0.6427681459581293666 ) ) ;
#5706=VERTEX_POINT ( 'NONE', #39924 ) ;
#5707=LINE ( 'NONE', #21901, #51424 ) ;
#5708=DIRECTION ( 'NONE',  ( -0.5364919789714478471, 0.6444004775717705469, -0.5449076811759709926 ) ) ;
#5709=EDGE_CURVE ( 'NONE', #21014, #24397, #2125, .T. ) ;
#5712=VECTOR ( 'NONE', #18052, 999.9999999999998863 ) ;
#5713=AXIS2_PLACEMENT_3D ( 'NONE', #19490, #37655, #37935 ) ;
#5714=ORIENTED_EDGE ( 'NONE', *, *, #19360, .T. ) ;
#5715=LINE ( 'NONE', #44597, #2287 ) ;
#5716=EDGE_LOOP ( 'NONE', ( #35266, #10739, #43199, #14261 ) ) ;
#5717=EDGE_CURVE ( 'NONE', #50946, #45163, #28001, .T. ) ;
#5718=VECTOR ( 'NONE', #31620, 1000.000000000000227 ) ;
#5719=CARTESIAN_POINT ( 'NONE',  ( -17.67018120889713018, 0.000000000000000000, 5.990895955192118372 ) ) ;
#5720=AXIS2_PLACEMENT_3D ( 'NONE', #34953, #8537, #21863 ) ;
#5721=EDGE_LOOP ( 'NONE', ( #34108, #16188, #51, #38760 ) ) ;
#5722=DIRECTION ( 'NONE',  ( 0.007781995580012662783, 0.000000000000000000, -0.9999697198139514409 ) ) ;
#5723=LINE ( 'NONE', #9984, #54696 ) ;
#5724=LINE ( 'NONE', #13956, #1069 ) ;
#5725=VERTEX_POINT ( 'NONE', #1005 ) ;
#5726=DIRECTION ( 'NONE',  ( 0.007781995580012662783, 0.000000000000000000, -0.9999697198139514409 ) ) ;
#5727=DIRECTION ( 'NONE',  ( 0.000000000000000000, -1.000000000000000000, 0.000000000000000000 ) ) ;
#5728=AXIS2_PLACEMENT_3D ( 'NONE', #12213, #21594, #50042 ) ;
#5729=FACE_OUTER_BOUND ( 'NONE', #46000, .T. ) ;
#5731=CARTESIAN_POINT ( 'NONE',  ( -10.41874048237084693, 0.000000000000000000, 3.831335924817679484 ) ) ;
#5733=EDGE_CURVE ( 'NONE', #27927, #31034, #19461, .T. ) ;
#5735=EDGE_LOOP ( 'NONE', ( #35507, #862, #29776, #12547 ) ) ;
#5736=DIRECTION ( 'NONE',  ( -0.6427681459581293666, -0.7660444431189770143, -0.005002170337467561935 ) ) ;
#5737=LINE ( 'NONE', #13972, #23164 ) ;
#5738=ADVANCED_FACE ( 'NONE', ( #31701 ), #6409, .F. ) ;
#5740=ORIENTED_EDGE ( 'NONE', *, *, #13032, .F. ) ;
#5741=CARTESIAN_POINT ( 'NONE',  ( -8.599902753822396662, -0.1191753592594186617, 4.853483721896219016 ) ) ;
#5742=LINE ( 'NONE', #17688, #28176 ) ;
#5744=VERTEX_POINT ( 'NONE', #54117 ) ;
#5745=AXIS2_PLACEMENT_3D ( 'NONE', #46996, #12636, #38465 ) ;
#5746=FACE_OUTER_BOUND ( 'NONE', #55715, .T. ) ;
#5747=EDGE_CURVE ( 'NONE', #12432, #53402, #27152, .T. ) ;
#5748=CARTESIAN_POINT ( 'NONE',  ( -9.750021733713985839, 1.198032013860655054, 1.892571191312284906 ) ) ;
#5749=VECTOR ( 'NONE', #47155, 999.9999999999998863 ) ;
#5750=CARTESIAN_POINT ( 'NONE',  ( -19.26408584338317098, 0.000000000000000000, 5.978491820772086740 ) ) ;
#5751=EDGE_CURVE ( 'NONE', #34091, #23582, #44742, .T. ) ;
#5752=PLANE ( 'NONE',  #1100 ) ;
#5753=VERTEX_POINT ( 'NONE', #9848 ) ;
#5754=ORIENTED_EDGE ( 'NONE', *, *, #35787, .T. ) ;
#5755=CARTESIAN_POINT ( 'NONE',  ( -20.54126990917373519, -0.1191753592594197858, 4.760553241521720658 ) ) ;
#5756=VECTOR ( 'NONE', #13716, 1000.000000000000227 ) ;
#5757=DIRECTION ( 'NONE',  ( -0.005961354470445682716, -0.6427876096865404731, 0.7660212471507180654 ) ) ;
#5759=CARTESIAN_POINT ( 'NONE',  ( -11.87243407472968926, 0.000000000000000000, 11.50246268866867361 ) ) ;
#5760=AXIS2_PLACEMENT_3D ( 'NONE', #35935, #14350, #49238 ) ;
#5761=DIRECTION ( 'NONE',  ( -0.005002170337468016433, -0.7660444431189770143, 0.6427681459581293666 ) ) ;
#5762=ORIENTED_EDGE ( 'NONE', *, *, #17362, .T. ) ;
#5763=CARTESIAN_POINT ( 'NONE',  ( -9.039200059374007168, 0.000000000000000000, 5.688732176410531416 ) ) ;
#5764=EDGE_LOOP ( 'NONE', ( #29127, #53218, #8128, #13175 ) ) ;
#5765=DIRECTION ( 'NONE',  ( -0.5364919789714478471, 0.6444004775717705469, -0.5449076811759709926 ) ) ;
#5766=VECTOR ( 'NONE', #32105, 999.9999999999998863 ) ;
#5767=DIRECTION ( 'NONE',  ( -0.5449076811759708816, 0.6444004775717707689, 0.5364919789714475140 ) ) ;
#5768=VECTOR ( 'NONE', #29789, 1000.000000000000114 ) ;
#5769=VERTEX_POINT ( 'NONE', #45309 ) ;
#5770=PLANE ( 'NONE',  #36522 ) ;
#5771=FACE_OUTER_BOUND ( 'NONE', #18979, .T. ) ;
#5772=DIRECTION ( 'NONE',  ( 0.007781995580012663651, -3.146120232559066537E-19, -0.9999697198139514409 ) ) ;
#5773=EDGE_LOOP ( 'NONE', ( #1122, #2809, #26018, #17365 ) ) ;
#5774=PLANE ( 'NONE',  #46618 ) ;
#5775=ORIENTED_EDGE ( 'NONE', *, *, #21982, .T. ) ;
#5776=ORIENTED_EDGE ( 'NONE', *, *, #33851, .F. ) ;
#5777=ORIENTED_EDGE ( 'NONE', *, *, #36764, .T. ) ;
#5778=FACE_OUTER_BOUND ( 'NONE', #16646, .T. ) ;
#5779=VECTOR ( 'NONE', #25335, 999.9999999999998863 ) ;
#5780=ORIENTED_EDGE ( 'NONE', *, *, #40899, .T. ) ;
#5782=VERTEX_POINT ( 'NONE', #22882 ) ;
#5783=VECTOR ( 'NONE', #49906, 999.9999999999998863 ) ;
#5784=DIRECTION ( 'NONE',  ( 0.007781995580012663651, -3.146120232559066537E-19, -0.9999697198139514409 ) ) ;
#5785=DIRECTION ( 'NONE',  ( -0.6427681459581293666, -0.7660444431189770143, -0.005002170337467561935 ) ) ;
#5786=ADVANCED_FACE ( 'NONE', ( #44460 ), #53542, .F. ) ;
#5787=EDGE_CURVE ( 'NONE', #16268, #48488, #6158, .T. ) ;
#5788=ORIENTED_EDGE ( 'NONE', *, *, #51919, .F. ) ;
#5789=ORIENTED_EDGE ( 'NONE', *, *, #8043, .T. ) ;
#5790=DIRECTION ( 'NONE',  ( -0.7660212471507179544, -0.6427876096865405842, -0.005961354470445141482 ) ) ;
#5791=AXIS2_PLACEMENT_3D ( 'NONE', #38307, #28694, #45709 ) ;
#5792=ORIENTED_EDGE ( 'NONE', *, *, #36954, .F. ) ;
#5793=EDGE_CURVE ( 'NONE', #44937, #28121, #3538, .T. ) ;
#5794=DIRECTION ( 'NONE',  ( 0.007781995580012663651, -3.146120232559066537E-19, -0.9999697198139514409 ) ) ;
#5795=LINE ( 'NONE', #18573, #11156 ) ;
#5796=FACE_OUTER_BOUND ( 'NONE', #1460, .T. ) ;
#5797=CARTESIAN_POINT ( 'NONE',  ( -14.94760462649100496, 0.000000000000000000, 2.488088991209854051 ) ) ;
#5798=LINE ( 'NONE', #53240, #4237 ) ;
#5799=AXIS2_PLACEMENT_3D ( 'NONE', #37189, #32928, #27864 ) ;
#5800=PLANE ( 'NONE',  #5593 ) ;
#5801=DIRECTION ( 'NONE',  ( -0.6427681459581293666, -0.7660444431189770143, -0.005002170337467561935 ) ) ;
#5802=VERTEX_POINT ( 'NONE', #11517 ) ;
#5803=VECTOR ( 'NONE', #47710, 1000.000000000000227 ) ;
#5804=ORIENTED_EDGE ( 'NONE', *, *, #9478, .F. ) ;
#5805=LINE ( 'NONE', #18283, #6530 ) ;
#5806=DIRECTION ( 'NONE',  ( 0.5449076811759707706, 0.6444004775717708799, -0.5364919789714476250 ) ) ;
#5808=AXIS2_PLACEMENT_3D ( 'NONE', #26768, #9750, #4369 ) ;
#5810=CARTESIAN_POINT ( 'NONE',  ( -14.59642022908046499, -2.460819163488160655, 2.472553415555822198 ) ) ;
#5811=ORIENTED_EDGE ( 'NONE', *, *, #54283, .T. ) ;
#5812=DIRECTION ( 'NONE',  ( 0.7660212471507180654, -0.6427876096865404731, 0.005961354470445141482 ) ) ;
#5814=ORIENTED_EDGE ( 'NONE', *, *, #30730, .F. ) ;
#5815=CARTESIAN_POINT ( 'NONE',  ( 2.072287782118878319, 0.000000000000000000, -2.950529333540147015 ) ) ;
#5817=VERTEX_POINT ( 'NONE', #11771 ) ;
#5818=DIRECTION ( 'NONE',  ( 0.005002170337468016433, -0.7660444431189770143, -0.6427681459581293666 ) ) ;
#5819=DIRECTION ( 'NONE',  ( 0.000000000000000000, 0.000000000000000000, 1.000000000000000000 ) ) ;
#5820=LINE ( 'NONE', #3226, #32284 ) ;
#5821=EDGE_CURVE ( 'NONE', #11647, #2600, #16308, .T. ) ;
#5822=CARTESIAN_POINT ( 'NONE',  ( -15.60102546347950536, 0.000000000000000000, 12.95077420755565356 ) ) ;
#5823=DIRECTION ( 'NONE',  ( 0.6427681459581294776, -0.7660444431189769032, 0.005002170337467562802 ) ) ;
#5824=EDGE_LOOP ( 'NONE', ( #8863, #29999, #13723, #22333 ) ) ;
#5825=VECTOR ( 'NONE', #44119, 999.9999999999998863 ) ;
#5826=ADVANCED_FACE ( 'NONE', ( #19749 ), #45567, .F. ) ;
#5827=VERTEX_POINT ( 'NONE', #2680 ) ;
#5828=DIRECTION ( 'NONE',  ( -0.7660212471507179544, -0.6427876096865405842, -0.005961354470445141482 ) ) ;
#5829=CARTESIAN_POINT ( 'NONE',  ( -18.66354898467281132, 0.000000000000000000, 14.21960318569776582 ) ) ;
#5830=CARTESIAN_POINT ( 'NONE',  ( -22.40634380310664397, 0.000000000000000000, 5.584705972946605534 ) ) ;
#5831=ADVANCED_FACE ( 'NONE', ( #24290 ), #55219, .F. ) ;
#5832=AXIS2_PLACEMENT_3D ( 'NONE', #10889, #32494, #20542 ) ;
#5833=CARTESIAN_POINT ( 'NONE',  ( -15.51406735044831997, -5.213152330870665097, 2.741184882836876113 ) ) ;
#5834=ADVANCED_FACE ( 'NONE', ( #54949 ), #16053, .F. ) ;
#5835=DIRECTION ( 'NONE',  ( 0.007781995580012663651, 0.000000000000000000, -0.9999697198139515519 ) ) ;
#5836=AXIS2_PLACEMENT_3D ( 'NONE', #26311, #26062, #51330 ) ;
#5837=ORIENTED_EDGE ( 'NONE', *, *, #26390, .F. ) ;
#5839=FACE_OUTER_BOUND ( 'NONE', #31708, .T. ) ;
#5840=DIRECTION ( 'NONE',  ( 0.007781995580012662783, 0.000000000000000000, -0.9999697198139514409 ) ) ;
#5841=CARTESIAN_POINT ( 'NONE',  ( -16.89925026227929195, -0.1191753592594197858, 13.49466922669627422 ) ) ;
#5842=ORIENTED_EDGE ( 'NONE', *, *, #42512, .T. ) ;
#5843=VECTOR ( 'NONE', #33761, 1000.000000000000227 ) ;
#5844=DIRECTION ( 'NONE',  ( 0.7660212471507180654, -0.6427876096865404731, 0.005961354470445141482 ) ) ;
#5845=ORIENTED_EDGE ( 'NONE', *, *, #17009, .T. ) ;
#5846=FACE_OUTER_BOUND ( 'NONE', #25240, .T. ) ;
#5847=FACE_OUTER_BOUND ( 'NONE', #24098, .T. ) ;
#5848=VECTOR ( 'NONE', #33716, 1000.000000000000227 ) ;
#5849=VERTEX_POINT ( 'NONE', #20291 ) ;
#5850=DIRECTION ( 'NONE',  ( -0.5364919789714478471, 0.6444004775717705469, -0.5449076811759709926 ) ) ;
#5851=EDGE_LOOP ( 'NONE', ( #10953, #52318, #1061, #49540 ) ) ;
#5853=ORIENTED_EDGE ( 'NONE', *, *, #39892, .F. ) ;
#5854=ORIENTED_EDGE ( 'NONE', *, *, #26539, .F. ) ;
#5855=CARTESIAN_POINT ( 'NONE',  ( -27.06708303904391144, 0.000000000000000000, 7.395095371555332697 ) ) ;
#5857=VERTEX_POINT ( 'NONE', #12043 ) ;
#5858=ORIENTED_EDGE ( 'NONE', *, *, #31690, .F. ) ;
#5859=CARTESIAN_POINT ( 'NONE',  ( -12.70458494993575194, -0.1191753592594197858, 11.86531876794841978 ) ) ;
#5860=EDGE_CURVE ( 'NONE', #2010, #8607, #33378, .T. ) ;
#5861=DIRECTION ( 'NONE',  ( 0.6427681459581294776, -0.7660444431189769032, 0.005002170337467562802 ) ) ;
#5863=EDGE_CURVE ( 'NONE', #23769, #30544, #42448, .T. ) ;
#5865=DIRECTION ( 'NONE',  ( -0.5364919789714478471, 0.6444004775717705469, -0.5449076811759709926 ) ) ;
#5866=ORIENTED_EDGE ( 'NONE', *, *, #34558, .T. ) ;
#5867=EDGE_LOOP ( 'NONE', ( #55251, #10809, #23707, #39370 ) ) ;
#5868=ADVANCED_FACE ( 'NONE', ( #7241 ), #20594, .F. ) ;
#5869=EDGE_CURVE ( 'NONE', #2187, #17736, #50939, .T. ) ;
#5870=VECTOR ( 'NONE', #14657, 1000.000000000000227 ) ;
#5871=DIRECTION ( 'NONE',  ( -0.6427681459581293666, -0.7660444431189770143, -0.005002170337467561935 ) ) ;
#5872=VECTOR ( 'NONE', #26184, 999.9999999999998863 ) ;
#5874=DIRECTION ( 'NONE',  ( -0.9999697198139514409, -0.000000000000000000, -0.007781995580013368816 ) ) ;
#5875=DIRECTION ( 'NONE',  ( 0.6427681459581294776, -0.7660444431189769032, 0.005002170337467562802 ) ) ;
#5876=ORIENTED_EDGE ( 'NONE', *, *, #31751, .F. ) ;
#5877=PLANE ( 'NONE',  #55491 ) ;
#5878=VECTOR ( 'NONE', #50572, 999.9999999999998863 ) ;
#5879=ORIENTED_EDGE ( 'NONE', *, *, #33488, .F. ) ;
#5880=DIRECTION ( 'NONE',  ( 0.007781995580012663651, 0.000000000000000000, -0.9999697198139515519 ) ) ;
#5881=EDGE_CURVE ( 'NONE', #50938, #6281, #29382, .T. ) ;
#5882=CARTESIAN_POINT ( 'NONE',  ( -25.20200914511100265, -0.1191753592594197858, 6.570942640130446932 ) ) ;
#5883=AXIS2_PLACEMENT_3D ( 'NONE', #22070, #13290, #48468 ) ;
#5885=DIRECTION ( 'NONE',  ( 0.005961354470445682716, -0.6427876096865404731, -0.7660212471507180654 ) ) ;
#5886=CARTESIAN_POINT ( 'NONE',  ( -17.74560456716937296, 0.000000000000000000, 3.774316574337878372 ) ) ;
#5887=VECTOR ( 'NONE', #47175, 1000.000000000000114 ) ;
#5888=CARTESIAN_POINT ( 'NONE',  ( -11.10260204233550496, -0.5179957512181551094, 1.844678686450966332 ) ) ;
#5889=ORIENTED_EDGE ( 'NONE', *, *, #97, .F. ) ;
#5890=CARTESIAN_POINT ( 'NONE',  ( 2.072287782118878319, 0.000000000000000000, -2.950529333540147015 ) ) ;
#5891=EDGE_LOOP ( 'NONE', ( #11041, #52070, #11588, #11052 ) ) ;
#5892=VECTOR ( 'NONE', #39817, 1000.000000000000227 ) ;
#5893=CARTESIAN_POINT ( 'NONE',  ( -21.46924666352205335, 3.686347215771509145, 11.27062942325050976 ) ) ;
#5894=DIRECTION ( 'NONE',  ( 0.5449076811759707706, 0.6444004775717708799, -0.5364919789714476250 ) ) ;
#5895=PLANE ( 'NONE',  #20882 ) ;
#5896=CARTESIAN_POINT ( 'NONE',  ( -20.10958161055168247, -0.1191753592594196887, 5.871908949099878150 ) ) ;
#5897=DIRECTION ( 'NONE',  ( 0.9321478471874540261, 0.000000000000000000, -0.3620778797217457101 ) ) ;
#5898=VECTOR ( 'NONE', #41313, 999.9999999999998863 ) ;
#5900=VECTOR ( 'NONE', #21996, 1000.000000000000000 ) ;
#5901=ORIENTED_EDGE ( 'NONE', *, *, #7231, .T. ) ;
#5902=DIRECTION ( 'NONE',  ( -0.9999697198139514409, -0.000000000000000000, -0.007781995580013368816 ) ) ;
#5903=CARTESIAN_POINT ( 'NONE',  ( -22.40478740399063895, 0.000000000000000000, 5.384712028983816623 ) ) ;
#5904=CARTESIAN_POINT ( 'NONE',  ( -19.35113876198915861, 0.000000000000000000, 7.824474703863986136 ) ) ;
#5906=EDGE_CURVE ( 'NONE', #37913, #9089, #41860, .T. ) ;
#5907=DIRECTION ( 'NONE',  ( 0.5449076811759707706, 0.6444004775717708799, -0.5364919789714476250 ) ) ;
#5908=DIRECTION ( 'NONE',  ( 0.6427681459581294776, -0.7660444431189769032, 0.005002170337467562802 ) ) ;
#5909=AXIS2_PLACEMENT_3D ( 'NONE', #8779, #13572, #5605 ) ;
#5910=FACE_OUTER_BOUND ( 'NONE', #5492, .T. ) ;
#5911=CARTESIAN_POINT ( 'NONE',  ( -14.93495759592298988, 0.000000000000000000, 12.77129166681078409 ) ) ;
#5912=VECTOR ( 'NONE', #47570, 1000.000000000000000 ) ;
#5913=EDGE_CURVE ( 'NONE', #24516, #48984, #32792, .T. ) ;
#5914=VERTEX_POINT ( 'NONE', #28253 ) ;
#5915=AXIS2_PLACEMENT_3D ( 'NONE', #22440, #9927, #30675 ) ;
#5916=EDGE_CURVE ( 'NONE', #5706, #50902, #49840, .T. ) ;
#5917=EDGE_CURVE ( 'NONE', #19489, #6417, #50100, .T. ) ;
#5919=EDGE_LOOP ( 'NONE', ( #34905, #12353, #43617, #11943 ) ) ;
#5920=AXIS2_PLACEMENT_3D ( 'NONE', #27353, #31899, #10875 ) ;
#5921=VECTOR ( 'NONE', #37574, 1000.000000000000227 ) ;
#5922=ORIENTED_EDGE ( 'NONE', *, *, #35503, .T. ) ;
#5923=VECTOR ( 'NONE', #27905, 999.9999999999998863 ) ;
#5924=VERTEX_POINT ( 'NONE', #24542 ) ;
#5925=DIRECTION ( 'NONE',  ( 0.007781995580012663651, 0.000000000000000000, -0.9999697198139515519 ) ) ;
#5929=ORIENTED_EDGE ( 'NONE', *, *, #17543, .F. ) ;
#5930=ADVANCED_FACE ( 'NONE', ( #37621 ), #38456, .F. ) ;
#5931=VERTEX_POINT ( 'NONE', #30525 ) ;
#5932=ORIENTED_EDGE ( 'NONE', *, *, #10297, .T. ) ;
#5933=ADVANCED_FACE ( 'NONE', ( #17424 ), #39022, .F. ) ;
#5934=AXIS2_PLACEMENT_3D ( 'NONE', #23567, #40883, #23834 ) ;
#5935=AXIS2_PLACEMENT_3D ( 'NONE', #24184, #3139, #33273 ) ;
#5937=LINE ( 'NONE', #30664, #3774 ) ;
#5938=CARTESIAN_POINT ( 'NONE',  ( -10.94028622754223967, 0.000000000000000000, 11.14038480894692995 ) ) ;
#5939=ORIENTED_EDGE ( 'NONE', *, *, #15241, .F. ) ;
#5940=LINE ( 'NONE', #31770, #14692 ) ;
#5941=ADVANCED_FACE ( 'NONE', ( #35069 ), #21968, .F. ) ;
#5942=ORIENTED_EDGE ( 'NONE', *, *, #26273, .T. ) ;
#5943=LINE ( 'NONE', #9336, #11007 ) ;
#5944=DIRECTION ( 'NONE',  ( -0.6427681459581293666, -0.7660444431189770143, -0.005002170337467561935 ) ) ;
#5945=AXIS2_PLACEMENT_3D ( 'NONE', #13511, #30571, #17199 ) ;
#5946=EDGE_CURVE ( 'NONE', #3951, #30703, #17732, .T. ) ;
#5947=DIRECTION ( 'NONE',  ( -0.5449076811759708816, 0.6444004775717707689, 0.5364919789714475140 ) ) ;
#5948=CARTESIAN_POINT ( 'NONE',  ( -14.01545677930355183, 0.000000000000000000, 2.126011111488108174 ) ) ;
#5950=DIRECTION ( 'NONE',  ( -0.005002170337468016433, -0.7660444431189770143, 0.6427681459581293666 ) ) ;
#5951=DIRECTION ( 'NONE',  ( -0.005961354470445682716, -0.6427876096865404731, 0.7660212471507180654 ) ) ;
#5952=VECTOR ( 'NONE', #22817, 999.9999999999998863 ) ;
#5953=EDGE_LOOP ( 'NONE', ( #19872, #47122, #30568, #3263, #13837 ) ) ;
#5954=PLANE ( 'NONE',  #9276 ) ;
#5955=ORIENTED_EDGE ( 'NONE', *, *, #41848, .T. ) ;
#5956=VECTOR ( 'NONE', #30182, 1000.000000000000114 ) ;
#5957=DIRECTION ( 'NONE',  ( 0.007781995580012662783, 0.000000000000000000, -0.9999697198139514409 ) ) ;
#5958=LINE ( 'NONE', #23278, #6982 ) ;
#5960=CARTESIAN_POINT ( 'NONE',  ( -15.33262645716528461, 0.000000000000000000, 4.162426997743341239 ) ) ;
#5961=VECTOR ( 'NONE', #29045, 1000.000000000000227 ) ;
#5962=CARTESIAN_POINT ( 'NONE',  ( -21.90706668065662654, 4.819660872929013351, 5.037607981832593396 ) ) ;
#5963=PLANE ( 'NONE',  #435 ) ;
#5965=CARTESIAN_POINT ( 'NONE',  ( 2.072287782118878319, 0.000000000000000000, -2.950529333540147015 ) ) ;
#5966=VECTOR ( 'NONE', #29884, 999.9999999999998863 ) ;
#5967=VECTOR ( 'NONE', #24284, 1000.000000000000227 ) ;
#5969=DIRECTION ( 'NONE',  ( -0.005002170337468016433, -0.7660444431189770143, 0.6427681459581293666 ) ) ;
#5970=ORIENTED_EDGE ( 'NONE', *, *, #33462, .T. ) ;
#5971=LINE ( 'NONE', #1945, #17560 ) ;
#5972=DIRECTION ( 'NONE',  ( 0.9999697198139515519, 0.000000000000000000, 0.007781995580013368816 ) ) ;
#5973=DIRECTION ( 'NONE',  ( 0.005961354470445682716, -0.6427876096865404731, -0.7660212471507180654 ) ) ;
#5974=PLANE ( 'NONE',  #15088 ) ;
#5975=VECTOR ( 'NONE', #44703, 1000.000000000000000 ) ;
#5977=LINE ( 'NONE', #40319, #25490 ) ;
#5978=VECTOR ( 'NONE', #42555, 1000.000000000000227 ) ;
#5979=EDGE_CURVE ( 'NONE', #22139, #43104, #34228, .T. ) ;
#5980=DIRECTION ( 'NONE',  ( 0.005961354470445682716, -0.6427876096865404731, -0.7660212471507180654 ) ) ;
#5981=LINE ( 'NONE', #45402, #10243 ) ;
#5982=ORIENTED_EDGE ( 'NONE', *, *, #49981, .T. ) ;
#5984=AXIS2_PLACEMENT_3D ( 'NONE', #36538, #10140, #27763 ) ;
#5985=EDGE_LOOP ( 'NONE', ( #26212, #4671, #31421, #2724 ) ) ;
#5986=DIRECTION ( 'NONE',  ( 0.5449076811759707706, 0.6444004775717708799, -0.5364919789714476250 ) ) ;
#5987=DIRECTION ( 'NONE',  ( 0.7660212471507180654, -0.6427876096865404731, 0.005961354470445141482 ) ) ;
#5988=EDGE_LOOP ( 'NONE', ( #26371, #16218, #31808, #19968 ) ) ;
#5989=DIRECTION ( 'NONE',  ( 0.007781995580012662783, 0.000000000000000000, -0.9999697198139514409 ) ) ;
#5990=ORIENTED_EDGE ( 'NONE', *, *, #12440, .F. ) ;
#5991=PLANE ( 'NONE',  #32897 ) ;
#5992=EDGE_CURVE ( 'NONE', #3929, #35510, #26241, .T. ) ;
#5993=VECTOR ( 'NONE', #13162, 999.9999999999998863 ) ;
#5994=ORIENTED_EDGE ( 'NONE', *, *, #20676, .T. ) ;
#5995=ORIENTED_EDGE ( 'NONE', *, *, #43242, .F. ) ;
#5996=EDGE_LOOP ( 'NONE', ( #36506, #54861, #40288, #50594 ) ) ;
#5997=CARTESIAN_POINT ( 'NONE',  ( 3.004435629306332345, -1.000000000000000000, -3.312607213261892003 ) ) ;
#5998=CARTESIAN_POINT ( 'NONE',  ( -16.81190032086591302, 0.000000000000000000, 3.212244750653343583 ) ) ;
#5999=AXIS2_PLACEMENT_3D ( 'NONE', #5520, #18029, #416 ) ;
#6000=DIRECTION ( 'NONE',  ( 0.7660212471507180654, -0.6427876096865404731, 0.005961354470445141482 ) ) ;
#6001=DIRECTION ( 'NONE',  ( -0.8531650599175529814, -0.4028455766673920135, 0.3313982828793697877 ) ) ;
#6002=EDGE_CURVE ( 'NONE', #5490, #12113, #13190, .T. ) ;
#6003=ORIENTED_EDGE ( 'NONE', *, *, #22469, .T. ) ;
#6004=VECTOR ( 'NONE', #16539, 1000.000000000000227 ) ;
#6005=ORIENTED_EDGE ( 'NONE', *, *, #23913, .F. ) ;
#6006=EDGE_CURVE ( 'NONE', #44182, #55542, #43553, .T. ) ;
#6007=AXIS2_PLACEMENT_3D ( 'NONE', #45138, #45667, #1396 ) ;
#6008=AXIS2_PLACEMENT_3D ( 'NONE', #49522, #2061, #28777 ) ;
#6009=PLANE ( 'NONE',  #39996 ) ;
#6010=EDGE_LOOP ( 'NONE', ( #38108, #39885, #47498, #14252, #21388 ) ) ;
#6011=DIRECTION ( 'NONE',  ( -0.005002170337468016433, -0.7660444431189770143, 0.6427681459581293666 ) ) ;
#6012=EDGE_LOOP ( 'NONE', ( #18636, #41171, #55271, #54668 ) ) ;
#6013=DIRECTION ( 'NONE',  ( 0.000000000000000000, -1.000000000000000000, 0.000000000000000000 ) ) ;
#6014=CARTESIAN_POINT ( 'NONE',  ( -10.69907135716483992, 0.000000000000000000, 5.845140687749472264 ) ) ;
#6015=AXIS2_PLACEMENT_3D ( 'NONE', #32625, #3074, #45397 ) ;
#6016=ADVANCED_FACE ( 'NONE', ( #4110 ), #21436, .F. ) ;
#6017=VERTEX_POINT ( 'NONE', #12896 ) ;
#6018=VECTOR ( 'NONE', #7054, 1000.000000000000227 ) ;
#6019=PLANE ( 'NONE',  #55808 ) ;
#6020=ORIENTED_EDGE ( 'NONE', *, *, #31135, .T. ) ;
#6021=AXIS2_PLACEMENT_3D ( 'NONE', #8866, #43478, #17641 ) ;
#6022=EDGE_CURVE ( 'NONE', #17269, #38231, #39297, .T. ) ;
#6023=DIRECTION ( 'NONE',  ( 0.000000000000000000, -1.000000000000000000, 0.000000000000000000 ) ) ;
#6024=VECTOR ( 'NONE', #4150, 1000.000000000000114 ) ;
#6025=ORIENTED_EDGE ( 'NONE', *, *, #42934, .T. ) ;
#6026=DIRECTION ( 'NONE',  ( 0.000000000000000000, -0.000000000000000000, -1.000000000000000000 ) ) ;
#6027=PLANE ( 'NONE',  #25693 ) ;
#6028=DIRECTION ( 'NONE',  ( -0.7660212471507179544, -0.6427876096865405842, -0.005961354470445141482 ) ) ;
#6029=ORIENTED_EDGE ( 'NONE', *, *, #42849, .F. ) ;
#6030=DIRECTION ( 'NONE',  ( 0.9999697198139515519, 0.000000000000000000, 0.007781995580013368816 ) ) ;
#6031=FACE_OUTER_BOUND ( 'NONE', #20733, .T. ) ;
#6032=PLANE ( 'NONE',  #35785 ) ;
#6033=DIRECTION ( 'NONE',  ( 0.007781995580012663651, 0.000000000000000000, -0.9999697198139515519 ) ) ;
#6034=DIRECTION ( 'NONE',  ( 0.6427681459581294776, -0.7660444431189769032, 0.005002170337467562802 ) ) ;
#6035=LINE ( 'NONE', #54520, #56025 ) ;
#6036=AXIS2_PLACEMENT_3D ( 'NONE', #37058, #27705, #2105 ) ;
#6038=ORIENTED_EDGE ( 'NONE', *, *, #17459, .T. ) ;
#6039=DIRECTION ( 'NONE',  ( -0.5449076811759708816, 0.6444004775717707689, 0.5364919789714475140 ) ) ;
#6040=FACE_OUTER_BOUND ( 'NONE', #12927, .T. ) ;
#6042=ORIENTED_EDGE ( 'NONE', *, *, #11758, .F. ) ;
#6043=DIRECTION ( 'NONE',  ( 0.7660212471507180654, -0.6427876096865404731, 0.005961354470445141482 ) ) ;
#6044=FACE_OUTER_BOUND ( 'NONE', #49420, .T. ) ;
#6045=VECTOR ( 'NONE', #8907, 999.9999999999998863 ) ;
#6046=ORIENTED_EDGE ( 'NONE', *, *, #26162, .F. ) ;
#6047=ADVANCED_FACE ( 'NONE', ( #3805 ), #387, .F. ) ;
#6048=VECTOR ( 'NONE', #361, 1000.000000000000227 ) ;
#6049=LINE ( 'NONE', #32151, #10464 ) ;
#6050=EDGE_CURVE ( 'NONE', #5827, #32592, #39604, .T. ) ;
#6051=CARTESIAN_POINT ( 'NONE',  ( -9.542064456761055524, 0.000000000000000000, 10.59726798936431180 ) ) ;
#6052=LINE ( 'NONE', #10845, #15649 ) ;
#6053=EDGE_LOOP ( 'NONE', ( #28188, #12542, #41951, #802 ) ) ;
#6054=VECTOR ( 'NONE', #15251, 999.9999999999998863 ) ;
#6055=EDGE_CURVE ( 'NONE', #47084, #18846, #47541, .T. ) ;
#6056=ORIENTED_EDGE ( 'NONE', *, *, #12795, .F. ) ;
#6057=ADVANCED_FACE ( 'NONE', ( #8354 ), #33921, .F. ) ;
#6058=PLANE ( 'NONE',  #47691 ) ;
#6059=LINE ( 'NONE', #44370, #53186 ) ;
#6060=EDGE_CURVE ( 'NONE', #1131, #54483, #29694, .T. ) ;
#6061=ADVANCED_FACE ( 'NONE', ( #4397 ), #21710, .F. ) ;
#6062=EDGE_CURVE ( 'NONE', #16128, #2320, #31348, .T. ) ;
#6063=LINE ( 'NONE', #53453, #29331 ) ;
#6064=AXIS2_PLACEMENT_3D ( 'NONE', #36816, #32803, #23472 ) ;
#6065=PLANE ( 'NONE',  #22856 ) ;
#6066=ORIENTED_EDGE ( 'NONE', *, *, #44117, .F. ) ;
#6067=LINE ( 'NONE', #6585, #19454 ) ;
#6068=ORIENTED_EDGE ( 'NONE', *, *, #6327, .T. ) ;
#6069=CARTESIAN_POINT ( 'NONE',  ( -13.08330893211609869, 0.000000000000000000, 1.763933231766363630 ) ) ;
#6070=VECTOR ( 'NONE', #16964, 999.9999999999998863 ) ;
#6071=AXIS2_PLACEMENT_3D ( 'NONE', #44704, #41001, #52951 ) ;
#6072=CARTESIAN_POINT ( 'NONE',  ( -20.54204810873173415, 0.000000000000000000, 4.860550213503115558 ) ) ;
#6073=ORIENTED_EDGE ( 'NONE', *, *, #10422, .F. ) ;
#6074=DIRECTION ( 'NONE',  ( -0.6427681459581293666, -0.7660444431189770143, -0.005002170337467561935 ) ) ;
#6075=LINE ( 'NONE', #32997, #45015 ) ;
#6076=CARTESIAN_POINT ( 'NONE',  ( -13.76498388619131852, 0.1245042932765033361, 2.432441075759850690 ) ) ;
#6077=ORIENTED_EDGE ( 'NONE', *, *, #37510, .T. ) ;
#6078=DIRECTION ( 'NONE',  ( 0.007781995580012663651, -3.146120232559066537E-19, -0.9999697198139514409 ) ) ;
#6079=EDGE_CURVE ( 'NONE', #18980, #34834, #23105, .T. ) ;
#6080=VERTEX_POINT ( 'NONE', #44392 ) ;
#6081=AXIS2_PLACEMENT_3D ( 'NONE', #8583, #11970, #34416 ) ;
#6082=EDGE_CURVE ( 'NONE', #33009, #27645, #1778, .T. ) ;
#6083=VERTEX_POINT ( 'NONE', #27644 ) ;
#6084=ORIENTED_EDGE ( 'NONE', *, *, #10177, .F. ) ;
#6086=EDGE_CURVE ( 'NONE', #3178, #51656, #18259, .T. ) ;
#6087=VERTEX_POINT ( 'NONE', #48366 ) ;
#6088=DIRECTION ( 'NONE',  ( 0.5364919789714477361, 0.6444004775717706579, 0.5449076811759711036 ) ) ;
#6090=EDGE_LOOP ( 'NONE', ( #37489, #8324, #27160, #40780 ) ) ;
#6092=DIRECTION ( 'NONE',  ( 0.9999697198139515519, 0.000000000000000000, 0.007781995580013368816 ) ) ;
#6093=ADVANCED_FACE ( 'NONE', ( #32186 ), #6340, .F. ) ;
#6094=ORIENTED_EDGE ( 'NONE', *, *, #34226, .F. ) ;
#6095=AXIS2_PLACEMENT_3D ( 'NONE', #52676, #43353, #13779 ) ;
#6096=DIRECTION ( 'NONE',  ( 0.9999697198139515519, 0.000000000000000000, 0.007781995580013368816 ) ) ;
#6097=VERTEX_POINT ( 'NONE', #9476 ) ;
#6099=PLANE ( 'NONE',  #55493 ) ;
#6100=CARTESIAN_POINT ( 'NONE',  ( 2.072287782118878319, 0.000000000000000000, -2.950529333540147015 ) ) ;
#6102=PLANE ( 'NONE',  #26627 ) ;
#6103=PLANE ( 'NONE',  #39580 ) ;
#6104=DIRECTION ( 'NONE',  ( 0.000000000000000000, -0.000000000000000000, -1.000000000000000000 ) ) ;
#6105=LINE ( 'NONE', #23405, #15677 ) ;
#6106=ORIENTED_EDGE ( 'NONE', *, *, #16165, .F. ) ;
#6107=ORIENTED_EDGE ( 'NONE', *, *, #52906, .T. ) ;
#6108=AXIS2_PLACEMENT_3D ( 'NONE', #20927, #3895, #25481 ) ;
#6109=CARTESIAN_POINT ( 'NONE',  ( -16.47051635532609737, 0.000000000000000000, 5.261567884864613909 ) ) ;
#6110=CARTESIAN_POINT ( 'NONE',  ( -15.28246537544034922, -2.137015261443158565, 6.125366393289809253 ) ) ;
#6111=LINE ( 'NONE', #25626, #4353 ) ;
#6113=CARTESIAN_POINT ( 'NONE',  ( -9.075990533167328067, 0.000000000000000000, 10.41622904950343909 ) ) ;
#6114=VERTEX_POINT ( 'NONE', #53220 ) ;
#6115=CARTESIAN_POINT ( 'NONE',  ( -12.70458494993575194, -0.1191753592594197858, 11.86531876794841978 ) ) ;
#6118=FACE_OUTER_BOUND ( 'NONE', #48750, .T. ) ;
#6119=CARTESIAN_POINT ( 'NONE',  ( -16.30345465431069485, 0.000000000000000000, 9.494846779111002277 ) ) ;
#6120=ORIENTED_EDGE ( 'NONE', *, *, #49303, .T. ) ;
#6122=DIRECTION ( 'NONE',  ( 0.007781995580012662783, 0.000000000000000000, -0.9999697198139514409 ) ) ;
#6123=PLANE ( 'NONE',  #3237 ) ;
#6124=DIRECTION ( 'NONE',  ( -0.005002170337468016433, -0.7660444431189770143, 0.6427681459581293666 ) ) ;
#6125=DIRECTION ( 'NONE',  ( 0.5449076811759707706, 0.6444004775717708799, -0.5364919789714476250 ) ) ;
#6126=ORIENTED_EDGE ( 'NONE', *, *, #2013, .F. ) ;
#6127=ORIENTED_EDGE ( 'NONE', *, *, #25714, .F. ) ;
#6128=DIRECTION ( 'NONE',  ( 0.000000000000000000, -1.000000000000000000, 0.000000000000000000 ) ) ;
#6129=DIRECTION ( 'NONE',  ( 0.005002170337468016433, -0.7660444431189770143, -0.6427681459581293666 ) ) ;
#6130=CARTESIAN_POINT ( 'NONE',  ( -17.74404816805336793, 0.000000000000000000, 3.574322630375089460 ) ) ;
#6131=EDGE_CURVE ( 'NONE', #31029, #33959, #9779, .T. ) ;
#6132=ADVANCED_FACE ( 'NONE', ( #10626 ), #5493, .F. ) ;
#6133=LINE ( 'NONE', #23437, #4699 ) ;
#6134=CARTESIAN_POINT ( 'NONE',  ( -19.99988053418094935, 2.553033558614008047, 4.369109392650745605 ) ) ;
#6135=ORIENTED_EDGE ( 'NONE', *, *, #8949, .T. ) ;
#6136=EDGE_CURVE ( 'NONE', #32655, #11685, #31891, .T. ) ;
#6137=DIRECTION ( 'NONE',  ( 0.000000000000000000, -0.000000000000000000, -1.000000000000000000 ) ) ;
#6138=DIRECTION ( 'NONE',  ( 0.9999697198139515519, 0.000000000000000000, 0.007781995580013368816 ) ) ;
#6139=CARTESIAN_POINT ( 'NONE',  ( -16.43317633868556626, -0.1191753592594197858, 13.31363028683540151 ) ) ;
#6140=VECTOR ( 'NONE', #33605, 999.9999999999998863 ) ;
#6141=DIRECTION ( 'NONE',  ( 0.9999697198139515519, 0.000000000000000000, 0.007781995580013368816 ) ) ;
#6142=ORIENTED_EDGE ( 'NONE', *, *, #10565, .T. ) ;
#6143=LINE ( 'NONE', #27138, #27479 ) ;
#6144=ORIENTED_EDGE ( 'NONE', *, *, #37958, .T. ) ;
#6145=FACE_OUTER_BOUND ( 'NONE', #33341, .T. ) ;
#6146=DIRECTION ( 'NONE',  ( -0.5364919789714478471, 0.6444004775717705469, -0.5449076811759709926 ) ) ;
#6147=ORIENTED_EDGE ( 'NONE', *, *, #49213, .T. ) ;
#6148=VECTOR ( 'NONE', #51551, 1000.000000000000227 ) ;
#6149=LINE ( 'NONE', #48438, #9098 ) ;
#6150=VERTEX_POINT ( 'NONE', #27086 ) ;
#6151=EDGE_CURVE ( 'NONE', #1256, #42362, #44973, .T. ) ;
#6152=VERTEX_POINT ( 'NONE', #18558 ) ;
#6153=ORIENTED_EDGE ( 'NONE', *, *, #28187, .T. ) ;
#6155=EDGE_LOOP ( 'NONE', ( #6680, #37340, #30470, #48577 ) ) ;
#6157=ORIENTED_EDGE ( 'NONE', *, *, #30261, .T. ) ;
#6158=LINE ( 'NONE', #41599, #15680 ) ;
#6159=DIRECTION ( 'NONE',  ( 0.6427681459581294776, -0.7660444431189769032, 0.005002170337467562802 ) ) ;
#6160=ORIENTED_EDGE ( 'NONE', *, *, #53723, .T. ) ;
#6161=ADVANCED_FACE ( 'NONE', ( #53741 ), #14858, .F. ) ;
#6162=VERTEX_POINT ( 'NONE', #39858 ) ;
#6163=CARTESIAN_POINT ( 'NONE',  ( -25.20123094555300369, 0.000000000000000000, 6.470945668149052032 ) ) ;
#6164=VERTEX_POINT ( 'NONE', #44127 ) ;
#6165=ORIENTED_EDGE ( 'NONE', *, *, #19215, .T. ) ;
#6166=ADVANCED_FACE ( 'NONE', ( #5240 ), #14322, .F. ) ;
#6167=PLANE ( 'NONE',  #44681 ) ;
#6168=DIRECTION ( 'NONE',  ( 0.7660212471507180654, -0.6427876096865404731, 0.005961354470445141482 ) ) ;
#6169=CARTESIAN_POINT ( 'NONE',  ( -16.00013135147444387, 0.000000000000000000, 4.526564390117095549 ) ) ;
#6170=CARTESIAN_POINT ( 'NONE',  ( -18.15050602765391119, 0.000000000000000000, 8.003144319007907015 ) ) ;
#6171=EDGE_CURVE ( 'NONE', #8281, #35209, #27344, .T. ) ;
#6172=EDGE_LOOP ( 'NONE', ( #1059, #50608, #38921, #8908 ) ) ;
#6173=LINE ( 'NONE', #53556, #48226 ) ;
#6174=VERTEX_POINT ( 'NONE', #54868 ) ;
#6175=LINE ( 'NONE', #23734, #26648 ) ;
#6176=FACE_OUTER_BOUND ( 'NONE', #25161, .T. ) ;
#6177=LINE ( 'NONE', #24785, #13211 ) ;
#6178=DIRECTION ( 'NONE',  ( -0.5449076811759708816, 0.6444004775717707689, 0.5364919789714475140 ) ) ;
#6179=PLANE ( 'NONE',  #40242 ) ;
#6180=LINE ( 'NONE', #42730, #46761 ) ;
#6181=ORIENTED_EDGE ( 'NONE', *, *, #45855, .F. ) ;
#6182=LINE ( 'NONE', #52719, #29249 ) ;
#6183=VERTEX_POINT ( 'NONE', #7436 ) ;
#6184=AXIS2_PLACEMENT_3D ( 'NONE', #13142, #17678, #35289 ) ;
#6185=CARTESIAN_POINT ( 'NONE',  ( -17.46532115785441519, 0.000000000000000000, 13.67492996699914265 ) ) ;
#6186=CARTESIAN_POINT ( 'NONE',  ( -17.93777409820730639, -3.108426967578162170, 3.749786651630157230 ) ) ;
#6187=CARTESIAN_POINT ( 'NONE',  ( -12.63827574153160072, -0.1191753592594188005, 3.344727890296471440 ) ) ;
#6188=LINE ( 'NONE', #7269, #39491 ) ;
#6189=FACE_OUTER_BOUND ( 'NONE', #5178, .T. ) ;
#6190=FACE_OUTER_BOUND ( 'NONE', #12308, .T. ) ;
#6191=ORIENTED_EDGE ( 'NONE', *, *, #48311, .T. ) ;
#6192=LINE ( 'NONE', #49873, #2179 ) ;
#6193=CARTESIAN_POINT ( 'NONE',  ( -16.43317633868556626, -0.1191753592594197858, 13.31363028683540151 ) ) ;
#6194=DIRECTION ( 'NONE',  ( 0.007781995580012663651, -3.146120232559066537E-19, -0.9999697198139514409 ) ) ;
#6195=ADVANCED_FACE ( 'NONE', ( #40960, #24763 ), #15980, .T. ) ;
#6197=CARTESIAN_POINT ( 'NONE',  ( -22.40556560354864146, -0.1191753592594197858, 5.484709000965211523 ) ) ;
#6198=ADVANCED_FACE ( 'NONE', ( #36722 ), #2349, .F. ) ;
#6199=CARTESIAN_POINT ( 'NONE',  ( 2.602374448188125350E-16, -1.000000000000000000, -2.125000000000000000 ) ) ;
#6200=EDGE_CURVE ( 'NONE', #19740, #2262, #6610, .T. ) ;
#6201=DIRECTION ( 'NONE',  ( -0.6427681459581293666, -0.7660444431189770143, -0.005002170337467561935 ) ) ;
#6202=LINE ( 'NONE', #44798, #41414 ) ;
#6203=LINE ( 'NONE', #45100, #44659 ) ;
#6204=EDGE_LOOP ( 'NONE', ( #5550, #29246, #15960 ) ) ;
#6205=ORIENTED_EDGE ( 'NONE', *, *, #43723, .T. ) ;
#6206=ORIENTED_EDGE ( 'NONE', *, *, #31930, .F. ) ;
#6207=EDGE_LOOP ( 'NONE', ( #15127, #34480, #55334, #38164 ) ) ;
#6208=EDGE_LOOP ( 'NONE', ( #14902, #5939, #43075, #20128 ) ) ;
#6209=EDGE_LOOP ( 'NONE', ( #16597, #29700, #5620, #37769 ) ) ;
#6210=LINE ( 'NONE', #27485, #9708 ) ;
#6211=LINE ( 'NONE', #23516, #47583 ) ;
#6212=VECTOR ( 'NONE', #50708, 999.9999999999998863 ) ;
#6213=ORIENTED_EDGE ( 'NONE', *, *, #30689, .F. ) ;
#6214=ORIENTED_EDGE ( 'NONE', *, *, #25445, .T. ) ;
#6215=ORIENTED_EDGE ( 'NONE', *, *, #54418, .F. ) ;
#6216=EDGE_CURVE ( 'NONE', #17655, #5535, #6910, .T. ) ;
#6218=EDGE_CURVE ( 'NONE', #27279, #33543, #41790, .T. ) ;
#6219=DIRECTION ( 'NONE',  ( 0.9999697198139515519, 0.000000000000000000, 0.007781995580013368816 ) ) ;
#6220=PLANE ( 'NONE',  #4189 ) ;
#6221=EDGE_CURVE ( 'NONE', #14352, #31046, #24474, .T. ) ;
#6222=ORIENTED_EDGE ( 'NONE', *, *, #25450, .F. ) ;
#6223=CARTESIAN_POINT ( 'NONE',  ( -17.88298902127032619, 0.000000000000000000, 7.635894128402147096 ) ) ;
#6224=ORIENTED_EDGE ( 'NONE', *, *, #37633, .F. ) ;
#6225=CARTESIAN_POINT ( 'NONE',  ( -19.35672695474844218, 0.000000000000000000, 4.300436530774871535 ) ) ;
#6226=ADVANCED_FACE ( 'NONE', ( #28765 ), #11137, .F. ) ;
#6227=DIRECTION ( 'NONE',  ( 0.6427681459581294776, -0.7660444431189769032, 0.005002170337467562802 ) ) ;
#6228=CARTESIAN_POINT ( 'NONE',  ( -18.09799117768911003, 0.2864062442990034651, 4.381236941275065355 ) ) ;
#6229=FACE_OUTER_BOUND ( 'NONE', #47798, .T. ) ;
#6230=DIRECTION ( 'NONE',  ( 0.000000000000000000, -1.000000000000000000, 0.000000000000000000 ) ) ;
#6231=DIRECTION ( 'NONE',  ( 0.007781995580012662783, 0.000000000000000000, -0.9999697198139514409 ) ) ;
#6232=DIRECTION ( 'NONE',  ( -0.005002170337468016433, -0.7660444431189770143, 0.6427681459581293666 ) ) ;
#6233=ORIENTED_EDGE ( 'NONE', *, *, #39223, .T. ) ;
#6234=DIRECTION ( 'NONE',  ( 0.6427681459581294776, -0.7660444431189769032, 0.005002170337467562802 ) ) ;
#6236=LINE ( 'NONE', #15302, #36523 ) ;
#6237=CARTESIAN_POINT ( 'NONE',  ( -17.56606728872570500, 2.391131607591507446, 7.628832529946389052 ) ) ;
#6238=LINE ( 'NONE', #23542, #36757 ) ;
#6239=LINE ( 'NONE', #11024, #37736 ) ;
#6240=DIRECTION ( 'NONE',  ( -0.005002170337468016433, -0.7660444431189770143, 0.6427681459581293666 ) ) ;
#6241=CARTESIAN_POINT ( 'NONE',  ( -16.47758211672594086, 0.000000000000000000, 6.169503050675118061 ) ) ;
#6242=LINE ( 'NONE', #33402, #30698 ) ;
#6243=ADVANCED_FACE ( 'NONE', ( #2882 ), #24222, .F. ) ;
#6244=DIRECTION ( 'NONE',  ( 0.6427681459581294776, -0.7660444431189769032, 0.005002170337467562802 ) ) ;
#6245=DIRECTION ( 'NONE',  ( -0.7660212471507179544, -0.6427876096865405842, -0.005961354470445141482 ) ) ;
#6246=ORIENTED_EDGE ( 'NONE', *, *, #28972, .T. ) ;
#6247=DIRECTION ( 'NONE',  ( 0.8531650599175529814, -0.4028455766673920135, -0.3313982828793697877 ) ) ;
#6248=CARTESIAN_POINT ( 'NONE',  ( -13.16056798344334133, -0.03739765774599676518, 1.931956729131618200 ) ) ;
#6249=EDGE_CURVE ( 'NONE', #20652, #33216, #20212, .T. ) ;
#6251=CARTESIAN_POINT ( 'NONE',  ( -18.54007560369215568, -3.270328918600661883, 3.978575490718303520 ) ) ;
#6252=AXIS2_PLACEMENT_3D ( 'NONE', #8318, #8616, #25948 ) ;
#6253=ADVANCED_FACE ( 'NONE', ( #28181 ), #19682, .F. ) ;
#6254=FACE_OUTER_BOUND ( 'NONE', #3019, .T. ) ;
#6255=CARTESIAN_POINT ( 'NONE',  ( -29.86274838104827367, -0.1191753592594197858, 8.381332038739175871 ) ) ;
#6256=DIRECTION ( 'NONE',  ( 0.005002170337468016433, -0.7660444431189770143, -0.6427681459581293666 ) ) ;
#6257=ADVANCED_FACE ( 'NONE', ( #20519 ), #37847, .F. ) ;
#6258=DIRECTION ( 'NONE',  ( 0.9999697198139515519, 0.000000000000000000, 0.007781995580013368816 ) ) ;
#6259=ORIENTED_EDGE ( 'NONE', *, *, #7028, .F. ) ;
#6260=ORIENTED_EDGE ( 'NONE', *, *, #19519, .T. ) ;
#6261=CARTESIAN_POINT ( 'NONE',  ( -24.26908309836554878, 0.000000000000000000, 6.108867788427308376 ) ) ;
#6262=PLANE ( 'NONE',  #18680 ) ;
#6264=EDGE_CURVE ( 'NONE', #45853, #24338, #37005, .T. ) ;
#6265=EDGE_LOOP ( 'NONE', ( #43088, #269, #33748, #35392 ) ) ;
#6266=PLANE ( 'NONE',  #5934 ) ;
#6267=VERTEX_POINT ( 'NONE', #33562 ) ;
#6269=ADVANCED_FACE ( 'NONE', ( #46622 ), #41256, .F. ) ;
#6270=VERTEX_POINT ( 'NONE', #19939 ) ;
#6271=ORIENTED_EDGE ( 'NONE', *, *, #47171, .F. ) ;
#6272=VERTEX_POINT ( 'NONE', #32718 ) ;
#6273=FACE_OUTER_BOUND ( 'NONE', #26902, .T. ) ;
#6274=PLANE ( 'NONE',  #54083 ) ;
#6275=CARTESIAN_POINT ( 'NONE',  ( -9.542064456761055524, 0.000000000000000000, 10.59726798936431180 ) ) ;
#6276=ORIENTED_EDGE ( 'NONE', *, *, #24919, .F. ) ;
#6277=ORIENTED_EDGE ( 'NONE', *, *, #6839, .F. ) ;
#6278=LINE ( 'NONE', #49137, #49956 ) ;
#6279=EDGE_LOOP ( 'NONE', ( #40336, #44542, #12761, #8799 ) ) ;
#6280=DIRECTION ( 'NONE',  ( -0.6427681459581293666, -0.7660444431189770143, -0.005002170337467561935 ) ) ;
#6281=VERTEX_POINT ( 'NONE', #37260 ) ;
#6282=CARTESIAN_POINT ( 'NONE',  ( 2.072287782118878319, 0.000000000000000000, -2.950529333540147015 ) ) ;
#6285=EDGE_LOOP ( 'NONE', ( #32260, #18290, #26734, #5035 ) ) ;
#6286=DIRECTION ( 'NONE',  ( -0.9999697198139514409, -0.000000000000000000, -0.007781995580013368816 ) ) ;
#6287=ADVANCED_FACE ( 'NONE', ( #54561 ), #15671, .F. ) ;
#6288=DIRECTION ( 'NONE',  ( -0.005961354470445682716, -0.6427876096865404731, 0.7660212471507180654 ) ) ;
#6289=EDGE_LOOP ( 'NONE', ( #12183, #55459, #41428, #35829, #17218 ) ) ;
#6290=CARTESIAN_POINT ( 'NONE',  ( -11.22056963685719211, 0.000000000000000000, 1.239771416285661010 ) ) ;
#6291=CARTESIAN_POINT ( 'NONE',  ( -9.518333015441259093, -1.607988201085719160, 2.489039940304945020 ) ) ;
#6292=DIRECTION ( 'NONE',  ( 0.007781995580012663651, -3.146120232559066537E-19, -0.9999697198139514409 ) ) ;
#6293=ORIENTED_EDGE ( 'NONE', *, *, #22198, .F. ) ;
#6294=EDGE_CURVE ( 'NONE', #11120, #19445, #16820, .T. ) ;
#6295=DIRECTION ( 'NONE',  ( 0.5449076811759707706, 0.6444004775717708799, -0.5364919789714476250 ) ) ;
#6296=CARTESIAN_POINT ( 'NONE',  ( -10.94028622754223967, 0.000000000000000000, 11.14038480894692995 ) ) ;
#6297=CARTESIAN_POINT ( 'NONE',  ( -16.36974118378670084, -0.1191753592594190225, 5.162349112441218857 ) ) ;
#6298=DIRECTION ( 'NONE',  ( 0.000000000000000000, -1.000000000000000000, 0.000000000000000000 ) ) ;
#6299=EDGE_CURVE ( 'NONE', #2679, #18318, #30451, .T. ) ;
#6300=DIRECTION ( 'NONE',  ( 0.7660212471507180654, -0.6427876096865404731, 0.005961354470445141482 ) ) ;
#6301=CARTESIAN_POINT ( 'NONE',  ( -27.06630483948590893, -0.1191753592594197858, 7.295098399573937797 ) ) ;
#6302=ADVANCED_FACE ( 'NONE', ( #25069 ), #23, .F. ) ;
#6304=ORIENTED_EDGE ( 'NONE', *, *, #3965, .F. ) ;
#6305=LINE ( 'NONE', #18220, #54299 ) ;
#6306=CARTESIAN_POINT ( 'NONE',  ( -12.73042875255514872, 0.000000000000000000, 2.336017552946574760 ) ) ;
#6308=ORIENTED_EDGE ( 'NONE', *, *, #54239, .F. ) ;
#6309=DIRECTION ( 'NONE',  ( 0.007781995580012662783, 0.000000000000000000, -0.9999697198139514409 ) ) ;
#6310=DIRECTION ( 'NONE',  ( 0.9999697198139515519, 0.000000000000000000, 0.007781995580013368816 ) ) ;
#6311=ADVANCED_FACE ( 'NONE', ( #47467 ), #29878, .F. ) ;
#6312=CARTESIAN_POINT ( 'NONE',  ( -15.12407731238180730, 1.743523803501506375, 2.501009437766517518 ) ) ;
#6313=LINE ( 'NONE', #36147, #22404 ) ;
#6314=EDGE_CURVE ( 'NONE', #51395, #17188, #47772, .T. ) ;
#6315=DIRECTION ( 'NONE',  ( 0.5449076811759707706, 0.6444004775717708799, -0.5364919789714476250 ) ) ;
#6316=VERTEX_POINT ( 'NONE', #51467 ) ;
#6317=ORIENTED_EDGE ( 'NONE', *, *, #53780, .T. ) ;
#6318=DIRECTION ( 'NONE',  ( 0.005961354470445682716, -0.6427876096865404731, -0.7660212471507180654 ) ) ;
#6319=FACE_OUTER_BOUND ( 'NONE', #1900, .T. ) ;
#6320=PLANE ( 'NONE',  #10285 ) ;
#6322=AXIS2_PLACEMENT_3D ( 'NONE', #35709, #48783, #9878 ) ;
#6323=EDGE_LOOP ( 'NONE', ( #49344, #38488, #17950, #23446 ) ) ;
#6324=CARTESIAN_POINT ( 'NONE',  ( -10.74029228357944987, 0.000000000000000000, 11.14194120806293320 ) ) ;
#6325=ORIENTED_EDGE ( 'NONE', *, *, #10800, .F. ) ;
#6326=CARTESIAN_POINT ( 'NONE',  ( -19.32961685222932147, 0.000000000000000000, 14.39908572644263351 ) ) ;
#6327=EDGE_CURVE ( 'NONE', #20518, #40648, #3472, .T. ) ;
#6328=ORIENTED_EDGE ( 'NONE', *, *, #15330, .F. ) ;
#6329=ORIENTED_EDGE ( 'NONE', *, *, #40063, .F. ) ;
#6330=LINE ( 'NONE', #31880, #32025 ) ;
#6331=CARTESIAN_POINT ( 'NONE',  ( -16.86311861568060877, -0.1191753592594181482, 8.851830233250854718 ) ) ;
#6332=LINE ( 'NONE', #19373, #9436 ) ;
#6333=VERTEX_POINT ( 'NONE', #3735 ) ;
#6334=FACE_OUTER_BOUND ( 'NONE', #17083, .T. ) ;
#6335=EDGE_LOOP ( 'NONE', ( #55920, #17801, #29057, #35026 ) ) ;
#6336=EDGE_LOOP ( 'NONE', ( #20328, #37787, #17576, #54888 ) ) ;
#6337=ORIENTED_EDGE ( 'NONE', *, *, #25353, .F. ) ;
#6338=FACE_OUTER_BOUND ( 'NONE', #41596, .T. ) ;
#6339=ORIENTED_EDGE ( 'NONE', *, *, #51028, .F. ) ;
#6340=PLANE ( 'NONE',  #32967 ) ;
#6341=ORIENTED_EDGE ( 'NONE', *, *, #46449, .F. ) ;
#6343=CARTESIAN_POINT ( 'NONE',  ( -15.60102546347950536, 0.000000000000000000, 12.95077420755565356 ) ) ;
#6344=DIRECTION ( 'NONE',  ( -0.005961354470445682716, -0.6427876096865404731, 0.7660212471507180654 ) ) ;
#6345=EDGE_LOOP ( 'NONE', ( #4392, #36710, #4453, #39835 ) ) ;
#6346=PLANE ( 'NONE',  #52208 ) ;
#6347=ADVANCED_FACE ( 'NONE', ( #51717 ), #34993, .F. ) ;
#6349=LINE ( 'NONE', #22821, #20096 ) ;
#6350=ADVANCED_FACE ( 'NONE', ( #25910 ), #17354, .F. ) ;
#6351=LINE ( 'NONE', #15413, #17535 ) ;
#6352=DIRECTION ( 'NONE',  ( 0.005002170337468016433, -0.7660444431189770143, -0.6427681459581293666 ) ) ;
#6353=CARTESIAN_POINT ( 'NONE',  ( -15.13495153988577968, 0.000000000000000000, 12.76973526769478084 ) ) ;
#6354=LINE ( 'NONE', #45506, #15092 ) ;
#6355=DIRECTION ( 'NONE',  ( -0.2426528472758542054, 0.7422098413412800966, -0.6246952433987894571 ) ) ;
#6356=DIRECTION ( 'NONE',  ( 0.000000000000000000, -1.000000000000000000, 0.000000000000000000 ) ) ;
#6357=VERTEX_POINT ( 'NONE', #17654 ) ;
#6358=EDGE_CURVE ( 'NONE', #37343, #49895, #4587, .T. ) ;
#6359=ADVANCED_FACE ( 'NONE', ( #34414 ), #4334, .F. ) ;
#6360=EDGE_CURVE ( 'NONE', #36106, #46689, #13411, .T. ) ;
#6361=ORIENTED_EDGE ( 'NONE', *, *, #4124, .F. ) ;
#6362=DIRECTION ( 'NONE',  ( 0.7660212471507180654, -0.6427876096865404731, 0.005961354470445141482 ) ) ;
#6363=DIRECTION ( 'NONE',  ( -0.5449076811759708816, 0.6444004775717707689, 0.5364919789714475140 ) ) ;
#6364=DIRECTION ( 'NONE',  ( 0.007781995580012663651, -3.146120232559066537E-19, -0.9999697198139514409 ) ) ;
#6365=CARTESIAN_POINT ( 'NONE',  ( -13.08408713167409942, -0.1191753592594197858, 1.863930203747758085 ) ) ;
#6366=EDGE_CURVE ( 'NONE', #1256, #20039, #30725, .T. ) ;
#6368=ORIENTED_EDGE ( 'NONE', *, *, #29237, .F. ) ;
#6369=PLANE ( 'NONE',  #13144 ) ;
#6370=LINE ( 'NONE', #11470, #53182 ) ;
#6371=ORIENTED_EDGE ( 'NONE', *, *, #6602, .T. ) ;
#6372=CARTESIAN_POINT ( 'NONE',  ( -19.60990026154428278, 0.000000000000000000, 4.498472333781370125 ) ) ;
#6373=DIRECTION ( 'NONE',  ( 0.000000000000000000, -1.000000000000000000, 0.000000000000000000 ) ) ;
#6374=ORIENTED_EDGE ( 'NONE', *, *, #38605, .F. ) ;
#6375=CARTESIAN_POINT ( 'NONE',  ( -13.01806413347570590, 0.000000000000000000, 5.288435666356683384 ) ) ;
#6377=EDGE_CURVE ( 'NONE', #42918, #19378, #21054, .T. ) ;
#6378=DIRECTION ( 'NONE',  ( 0.5364919789714477361, 0.6444004775717706579, 0.5449076811759711036 ) ) ;
#6379=DIRECTION ( 'NONE',  ( -0.005002170337468016433, -0.7660444431189770143, 0.6427681459581293666 ) ) ;
#6380=EDGE_CURVE ( 'NONE', #7777, #31631, #38386, .T. ) ;
#6381=CARTESIAN_POINT ( 'NONE',  ( -17.87724091425976169, 0.000000000000000000, 6.897274721886618387 ) ) ;
#6382=ORIENTED_EDGE ( 'NONE', *, *, #26319, .T. ) ;
#6383=ORIENTED_EDGE ( 'NONE', *, *, #30907, .F. ) ;
#6384=EDGE_CURVE ( 'NONE', #42368, #33896, #14256, .T. ) ;
#6385=LINE ( 'NONE', #11187, #49339 ) ;
#6386=LINE ( 'NONE', #44712, #18630 ) ;
#6387=CARTESIAN_POINT ( 'NONE',  ( -18.75345506656806549, -0.03739765774599677212, 4.104424007462089463 ) ) ;
#6388=ADVANCED_FACE ( 'NONE', ( #31568 ), #32116, .F. ) ;
#6389=DIRECTION ( 'NONE',  ( -0.5364919789714478471, 0.6444004775717705469, -0.5449076811759709926 ) ) ;
#6391=ORIENTED_EDGE ( 'NONE', *, *, #47063, .T. ) ;
#6393=VECTOR ( 'NONE', #27410, 1000.000000000000000 ) ;
#6394=CARTESIAN_POINT ( 'NONE',  ( -18.67697421479882181, -0.1191753592594197858, 4.036397482078229793 ) ) ;
#6395=CARTESIAN_POINT ( 'NONE',  ( -30.79489622823572859, -0.1191753592594197858, 8.743409918460921304 ) ) ;
#6396=ORIENTED_EDGE ( 'NONE', *, *, #19581, .T. ) ;
#6397=CARTESIAN_POINT ( 'NONE',  ( -30.79411802867772607, 0.000000000000000000, 8.643412946479525516 ) ) ;
#6398=VERTEX_POINT ( 'NONE', #40644 ) ;
#6399=FACE_OUTER_BOUND ( 'NONE', #34899, .T. ) ;
#6400=CARTESIAN_POINT ( 'NONE',  ( -17.73140113748535285, 0.000000000000000000, 13.85752530597602039 ) ) ;
#6401=EDGE_LOOP ( 'NONE', ( #21398, #41983, #37501, #37466 ) ) ;
#6402=DIRECTION ( 'NONE',  ( 0.5449076811759707706, 0.6444004775717708799, -0.5364919789714476250 ) ) ;
#6403=ORIENTED_EDGE ( 'NONE', *, *, #3975, .F. ) ;
#6404=ORIENTED_EDGE ( 'NONE', *, *, #27785, .T. ) ;
#6405=ORIENTED_EDGE ( 'NONE', *, *, #9455, .F. ) ;
#6406=PLANE ( 'NONE',  #50210 ) ;
#6407=VERTEX_POINT ( 'NONE', #9124 ) ;
#6408=ORIENTED_EDGE ( 'NONE', *, *, #11879, .T. ) ;
#6409=PLANE ( 'NONE',  #28377 ) ;
#6410=ORIENTED_EDGE ( 'NONE', *, *, #19360, .F. ) ;
#6411=ADVANCED_FACE ( 'NONE', ( #48290 ), #44892, .F. ) ;
#6412=EDGE_LOOP ( 'NONE', ( #11903, #53625, #19750, #6084 ) ) ;
#6413=LINE ( 'NONE', #10942, #44938 ) ;
#6414=ORIENTED_EDGE ( 'NONE', *, *, #4962, .F. ) ;
#6415=EDGE_CURVE ( 'NONE', #39023, #3706, #18193, .T. ) ;
#6416=ORIENTED_EDGE ( 'NONE', *, *, #22324, .F. ) ;
#6417=VERTEX_POINT ( 'NONE', #44330 ) ;
#6418=ADVANCED_FACE ( 'NONE', ( #4869 ), #53147, .F. ) ;
#6419=DIRECTION ( 'NONE',  ( -0.6427681459581293666, -0.7660444431189770143, -0.005002170337467561935 ) ) ;
#6420=DIRECTION ( 'NONE',  ( 0.9999697198139515519, 0.000000000000000000, 0.007781995580013368816 ) ) ;
#6421=CARTESIAN_POINT ( 'NONE',  ( -18.67697421479882181, -0.1191753592594197858, 4.036397482078229793 ) ) ;
#6422=LINE ( 'NONE', #46144, #54031 ) ;
#6423=ORIENTED_EDGE ( 'NONE', *, *, #22159, .F. ) ;
#6424=CARTESIAN_POINT ( 'NONE',  ( -15.70177159435079695, 2.391131607591507446, 6.904676770502899075 ) ) ;
#6425=ORIENTED_EDGE ( 'NONE', *, *, #12828, .F. ) ;
#6426=EDGE_CURVE ( 'NONE', #11310, #21341, #22743, .T. ) ;
#6427=EDGE_CURVE ( 'NONE', #47379, #40739, #26725, .T. ) ;
#6428=ADVANCED_FACE ( 'NONE', ( #44051 ), #35524, .F. ) ;
#6429=EDGE_LOOP ( 'NONE', ( #34279, #7161, #47602, #36465 ) ) ;
#6430=AXIS2_PLACEMENT_3D ( 'NONE', #38621, #55359, #12210 ) ;
#6431=LINE ( 'NONE', #14950, #51126 ) ;
#6433=ADVANCED_FACE ( 'NONE', ( #53413 ), #14512, .F. ) ;
#6434=VECTOR ( 'NONE', #53706, 1000.000000000000000 ) ;
#6436=CARTESIAN_POINT ( 'NONE',  ( -12.86480176444844581, -1.489407457353158160, 4.123429006776876626 ) ) ;
#6437=CARTESIAN_POINT ( 'NONE',  ( -18.38240279575065017, -1.975113310420658852, 3.958654176621851484 ) ) ;
#6438=LINE ( 'NONE', #19194, #11367 ) ;
#6439=ORIENTED_EDGE ( 'NONE', *, *, #16301, .F. ) ;
#6440=DIRECTION ( 'NONE',  ( 0.007781995580012663651, 0.000000000000000000, -0.9999697198139515519 ) ) ;
#6441=ORIENTED_EDGE ( 'NONE', *, *, #39309, .T. ) ;
#6442=DIRECTION ( 'NONE',  ( -0.7660212471507179544, -0.6427876096865405842, -0.005961354470445141482 ) ) ;
#6443=PLANE ( 'NONE',  #2420 ) ;
#6444=DIRECTION ( 'NONE',  ( -0.6427681459581293666, -0.7660444431189770143, -0.005002170337467561935 ) ) ;
#6445=CARTESIAN_POINT ( 'NONE',  ( -9.872934393541347831, -0.1117717739994080611, 7.053356580378568275 ) ) ;
#6446=ADVANCED_FACE ( 'NONE', ( #40059 ), #22191, .F. ) ;
#6447=DIRECTION ( 'NONE',  ( 0.007781995580012663651, 0.000000000000000000, -0.9999697198139515519 ) ) ;
#6448=VERTEX_POINT ( 'NONE', #43753 ) ;
#6449=ADVANCED_FACE ( 'NONE', ( #1715 ), #53674, .F. ) ;
#6450=CARTESIAN_POINT ( 'NONE',  ( -17.26532721389163072, 0.000000000000000000, 13.67648636611514590 ) ) ;
#6452=DIRECTION ( 'NONE',  ( 0.005002170337468016433, -0.7660444431189770143, -0.6427681459581293666 ) ) ;
#6453=EDGE_CURVE ( 'NONE', #20837, #22139, #52562, .T. ) ;
#6454=VECTOR ( 'NONE', #36654, 1000.000000000000227 ) ;
#6455=DIRECTION ( 'NONE',  ( 0.007781995580012662783, 0.000000000000000000, -0.9999697198139514409 ) ) ;
#6456=DIRECTION ( 'NONE',  ( 0.7660212471507180654, -0.6427876096865404731, 0.005961354470445141482 ) ) ;
#6457=PLANE ( 'NONE',  #36356 ) ;
#6458=PLANE ( 'NONE',  #33791 ) ;
#6459=EDGE_CURVE ( 'NONE', #21349, #48276, #30974, .T. ) ;
#6460=CARTESIAN_POINT ( 'NONE',  ( -31.72626587586518099, 0.000000000000000000, 9.005490826201270949 ) ) ;
#6461=CARTESIAN_POINT ( 'NONE',  ( -13.73672976910459909, 0.000000000000000000, 12.22661844811216270 ) ) ;
#6462=EDGE_LOOP ( 'NONE', ( #50734, #31075, #54859, #38899 ) ) ;
#6463=VECTOR ( 'NONE', #15837, 1000.000000000000227 ) ;
#6464=VECTOR ( 'NONE', #24382, 1000.000000000000227 ) ;
#6465=ORIENTED_EDGE ( 'NONE', *, *, #44254, .T. ) ;
#6466=ORIENTED_EDGE ( 'NONE', *, *, #17915, .T. ) ;
#6467=ORIENTED_EDGE ( 'NONE', *, *, #4691, .F. ) ;
#6468=ORIENTED_EDGE ( 'NONE', *, *, #41551, .F. ) ;
#6469=CARTESIAN_POINT ( 'NONE',  ( -21.47263955680318404, 0.000000000000000000, 5.022634149262071190 ) ) ;
#6470=DIRECTION ( 'NONE',  ( -0.005961354470445682716, -0.6427876096865404731, 0.7660212471507180654 ) ) ;
#6471=ORIENTED_EDGE ( 'NONE', *, *, #18532, .T. ) ;
#6472=PLANE ( 'NONE',  #14985 ) ;
#6473=ORIENTED_EDGE ( 'NONE', *, *, #3282, .T. ) ;
#6474=ORIENTED_EDGE ( 'NONE', *, *, #30663, .T. ) ;
#6476=DIRECTION ( 'NONE',  ( 0.000000000000000000, -0.000000000000000000, -1.000000000000000000 ) ) ;
#6477=CARTESIAN_POINT ( 'NONE',  ( -16.06709938707323460, 0.000000000000000000, 13.13181314741652628 ) ) ;
#6478=ORIENTED_EDGE ( 'NONE', *, *, #31397, .F. ) ;
#6479=DIRECTION ( 'NONE',  ( 0.005002170337468016433, -0.7660444431189770143, -0.6427681459581293666 ) ) ;
#6480=ADVANCED_FACE ( 'NONE', ( #13944 ), #31269, .F. ) ;
#6481=AXIS2_PLACEMENT_3D ( 'NONE', #40618, #36621, #40871 ) ;
#6482=VECTOR ( 'NONE', #23264, 1000.000000000000227 ) ;
#6483=CARTESIAN_POINT ( 'NONE',  ( -10.77398004715669444, -0.1191753592594188005, 2.620572130852981907 ) ) ;
#6484=DIRECTION ( 'NONE',  ( -0.005002170337468016433, -0.7660444431189770143, 0.6427681459581293666 ) ) ;
#6485=ADVANCED_FACE ( 'NONE', ( #27023 ), #19878, .F. ) ;
#6486=ADVANCED_FACE ( 'NONE', ( #24413 ), #2557, .F. ) ;
#6487=CARTESIAN_POINT ( 'NONE',  ( -15.86710544311044302, 0.000000000000000000, 13.13336954653252953 ) ) ;
#6488=FACE_OUTER_BOUND ( 'NONE', #14892, .T. ) ;
#6489=CARTESIAN_POINT ( 'NONE',  ( -20.45041684859848630, 0.000000000000000000, 4.994449012483184625 ) ) ;
#6490=CARTESIAN_POINT ( 'NONE',  ( -27.06630483948590893, -0.1191753592594197858, 7.295098399573937797 ) ) ;
#6491=CARTESIAN_POINT ( 'NONE',  ( -16.51810710137574034, -1.975113310420659740, 3.234498417178360175 ) ) ;
#6492=CARTESIAN_POINT ( 'NONE',  ( -17.26532721389163072, 0.000000000000000000, 13.67648636611514590 ) ) ;
#6493=ORIENTED_EDGE ( 'NONE', *, *, #31750, .F. ) ;
#6495=EDGE_LOOP ( 'NONE', ( #2350, #3330, #22851, #20538 ) ) ;
#6496=CARTESIAN_POINT ( 'NONE',  ( -17.82366898634780128, -4.565544526780660028, 11.09808643466108613 ) ) ;
#6497=DIRECTION ( 'NONE',  ( 0.6427681459581294776, -0.7660444431189769032, 0.005002170337467562802 ) ) ;
#6498=CARTESIAN_POINT ( 'NONE',  ( -14.94916102560700821, 0.000000000000000000, 2.688082935172642962 ) ) ;
#6499=DIRECTION ( 'NONE',  ( -0.005961354470445682716, -0.6427876096865404731, 0.7660212471507180654 ) ) ;
#6500=DIRECTION ( 'NONE',  ( 0.5449076811759707706, 0.6444004775717708799, -0.5364919789714476250 ) ) ;
#6501=CARTESIAN_POINT ( 'NONE',  ( -13.65970254623731783, 0.000000000000000000, 2.328785729410555394 ) ) ;
#6502=CARTESIAN_POINT ( 'NONE',  ( -1.148821818165424169, 4.447699752827971587, 3.664614983992416697 ) ) ;
#6503=VECTOR ( 'NONE', #18411, 1000.000000000000227 ) ;
#6504=CARTESIAN_POINT ( 'NONE',  ( -16.06709938707323460, 0.000000000000000000, 13.13181314741652628 ) ) ;
#6506=LINE ( 'NONE', #19574, #3968 ) ;
#6507=DIRECTION ( 'NONE',  ( -0.005002170337468016433, -0.7660444431189770143, 0.6427681459581293666 ) ) ;
#6508=PLANE ( 'NONE',  #20022 ) ;
#6509=PLANE ( 'NONE',  #6015 ) ;
#6510=LINE ( 'NONE', #41447, #3712 ) ;
#6511=LINE ( 'NONE', #28940, #24848 ) ;
#6512=ADVANCED_FACE ( 'NONE', ( #6833 ), #33245, .F. ) ;
#6513=CARTESIAN_POINT ( 'NONE',  ( -27.99845268667336384, -0.1191753592594197858, 7.657176279295684118 ) ) ;
#6514=CARTESIAN_POINT ( 'NONE',  ( -14.63655816273770149, 0.6102101463440035012, 2.347799083036467671 ) ) ;
#6515=ORIENTED_EDGE ( 'NONE', *, *, #21979, .F. ) ;
#6516=CARTESIAN_POINT ( 'NONE',  ( -27.99767448711536133, 0.000000000000000000, 7.557179307314289218 ) ) ;
#6517=ORIENTED_EDGE ( 'NONE', *, *, #36388, .F. ) ;
#6518=ADVANCED_FACE ( 'NONE', ( #2278 ), #45181, .F. ) ;
#6519=PLANE ( 'NONE',  #41375 ) ;
#6520=DIRECTION ( 'NONE',  ( 0.007781995580012663651, 0.000000000000000000, -0.9999697198139515519 ) ) ;
#6521=VECTOR ( 'NONE', #29133, 1000.000000000000227 ) ;
#6522=VECTOR ( 'NONE', #12298, 1000.000000000000114 ) ;
#6523=ORIENTED_EDGE ( 'NONE', *, *, #44643, .T. ) ;
#6524=LINE ( 'NONE', #15327, #34016 ) ;
#6525=ADVANCED_FACE ( 'NONE', ( #24687 ), #55097, .F. ) ;
#6526=ORIENTED_EDGE ( 'NONE', *, *, #33647, .F. ) ;
#6527=CARTESIAN_POINT ( 'NONE',  ( -18.69867377500269257, -0.1191753592594165800, 5.882888960116697596 ) ) ;
#6528=VERTEX_POINT ( 'NONE', #32413 ) ;
#6529=ORIENTED_EDGE ( 'NONE', *, *, #11707, .F. ) ;
#6530=VECTOR ( 'NONE', #35617, 1000.000000000000227 ) ;
#6531=ORIENTED_EDGE ( 'NONE', *, *, #49562, .F. ) ;
#6532=DIRECTION ( 'NONE',  ( -0.7660212471507179544, -0.6427876096865405842, -0.005961354470445141482 ) ) ;
#6533=FACE_OUTER_BOUND ( 'NONE', #45933, .T. ) ;
#6534=LINE ( 'NONE', #37774, #36682 ) ;
#6537=VERTEX_POINT ( 'NONE', #54793 ) ;
#6538=AXIS2_PLACEMENT_3D ( 'NONE', #27355, #2059, #31359 ) ;
#6539=CARTESIAN_POINT ( 'NONE',  ( -9.432946420178224045, 1.988741823534331044, 2.708862623243400769 ) ) ;
#6540=ORIENTED_EDGE ( 'NONE', *, *, #42144, .T. ) ;
#6541=LINE ( 'NONE', #28392, #53635 ) ;
#6542=ADVANCED_FACE ( 'NONE', ( #10555 ), #54247, .F. ) ;
#6543=ORIENTED_EDGE ( 'NONE', *, *, #26124, .F. ) ;
#6544=CARTESIAN_POINT ( 'NONE',  ( -14.00280974873554030, 0.000000000000000000, 12.40921378708904044 ) ) ;
#6545=LINE ( 'NONE', #23858, #32170 ) ;
#6546=EDGE_CURVE ( 'NONE', #1661, #22227, #40898, .T. ) ;
#6547=EDGE_LOOP ( 'NONE', ( #29927, #36817, #30180, #43493 ) ) ;
#6548=LINE ( 'NONE', #23862, #1038 ) ;
#6549=EDGE_CURVE ( 'NONE', #47842, #52488, #3110, .T. ) ;
#6550=FACE_OUTER_BOUND ( 'NONE', #48558, .T. ) ;
#6551=VERTEX_POINT ( 'NONE', #50553 ) ;
#6552=DIRECTION ( 'NONE',  ( -0.9999697198139514409, -0.000000000000000000, -0.007781995580013368816 ) ) ;
#6553=LINE ( 'NONE', #24171, #2172 ) ;
#6554=VECTOR ( 'NONE', #49098, 1000.000000000000000 ) ;
#6555=CARTESIAN_POINT ( 'NONE',  ( -12.75761288849197328, 0.000000000000000000, 5.829120641561431171 ) ) ;
#6556=VERTEX_POINT ( 'NONE', #27873 ) ;
#6557=VECTOR ( 'NONE', #48069, 1000.000000000000227 ) ;
#6558=VECTOR ( 'NONE', #30927, 999.9999999999998863 ) ;
#6559=DIRECTION ( 'NONE',  ( -0.5449076811759708816, 0.6444004775717707689, 0.5364919789714475140 ) ) ;
#6560=PLANE ( 'NONE',  #7901 ) ;
#6561=DIRECTION ( 'NONE',  ( 0.7660212471507180654, -0.6427876096865404731, 0.005961354470445141482 ) ) ;
#6562=FACE_OUTER_BOUND ( 'NONE', #10972, .T. ) ;
#6563=CARTESIAN_POINT ( 'NONE',  ( -9.761175402966818737, 0.000000000000000000, 4.744443401512198122 ) ) ;
#6564=FACE_OUTER_BOUND ( 'NONE', #15870, .T. ) ;
#6565=ADVANCED_FACE ( 'NONE', ( #37782 ), #23581, .F. ) ;
#6566=VECTOR ( 'NONE', #36285, 1000.000000000000227 ) ;
#6568=VECTOR ( 'NONE', #51945, 1000.000000000000114 ) ;
#6569=EDGE_LOOP ( 'NONE', ( #36596, #12206, #15666, #14016 ) ) ;
#6570=DIRECTION ( 'NONE',  ( -0.9321478471874540261, 0.000000000000000000, 0.3620778797217457656 ) ) ;
#6571=DIRECTION ( 'NONE',  ( -0.5449076811759708816, 0.6444004775717707689, 0.5364919789714475140 ) ) ;
#6573=ORIENTED_EDGE ( 'NONE', *, *, #17979, .F. ) ;
#6574=CARTESIAN_POINT ( 'NONE',  ( -17.93139508144814442, 0.000000000000000000, 13.85596890686001537 ) ) ;
#6575=PLANE ( 'NONE',  #49023 ) ;
#6576=FACE_OUTER_BOUND ( 'NONE', #16856, .T. ) ;
#6577=VECTOR ( 'NONE', #53241, 999.9999999999998863 ) ;
#6578=DIRECTION ( 'NONE',  ( -0.005961354470445682716, -0.6427876096865404731, 0.7660212471507180654 ) ) ;
#6582=CARTESIAN_POINT ( 'NONE',  ( -11.21979143729922157, -0.1191753592594201050, 1.139774444304266554 ) ) ;
#6583=FACE_OUTER_BOUND ( 'NONE', #812, .T. ) ;
#6584=ORIENTED_EDGE ( 'NONE', *, *, #32256, .T. ) ;
#6585=CARTESIAN_POINT ( 'NONE',  ( -15.68268933366439732, -4.241740624735661491, 9.735039861682876605 ) ) ;
#6586=ADVANCED_FACE ( 'NONE', ( #28697 ), #53965, .F. ) ;
#6587=VECTOR ( 'NONE', #48975, 1000.000000000000000 ) ;
#6588=ORIENTED_EDGE ( 'NONE', *, *, #9361, .T. ) ;
#6590=ORIENTED_EDGE ( 'NONE', *, *, #12205, .T. ) ;
#6591=ORIENTED_EDGE ( 'NONE', *, *, #2266, .T. ) ;
#6592=LINE ( 'NONE', #41239, #1203 ) ;
#6593=AXIS2_PLACEMENT_3D ( 'NONE', #28236, #18906, #11496 ) ;
#6594=FACE_OUTER_BOUND ( 'NONE', #17017, .T. ) ;
#6595=DIRECTION ( 'NONE',  ( -0.005961354470445682716, -0.6427876096865404731, 0.7660212471507180654 ) ) ;
#6596=EDGE_CURVE ( 'NONE', #15779, #15522, #32938, .T. ) ;
#6597=ORIENTED_EDGE ( 'NONE', *, *, #7382, .T. ) ;
#6598=VECTOR ( 'NONE', #46178, 1000.000000000000000 ) ;
#6599=VECTOR ( 'NONE', #51274, 999.9999999999998863 ) ;
#6600=CARTESIAN_POINT ( 'NONE',  ( -23.33849165029409889, 0.000000000000000000, 5.946783852668351855 ) ) ;
#6601=EDGE_LOOP ( 'NONE', ( #3523, #5146, #20964, #15091 ) ) ;
#6602=EDGE_CURVE ( 'NONE', #17094, #43539, #7369, .T. ) ;
#6603=EDGE_CURVE ( 'NONE', #25448, #35388, #10813, .T. ) ;
#6604=VERTEX_POINT ( 'NONE', #45427 ) ;
#6605=VECTOR ( 'NONE', #29367, 999.9999999999998863 ) ;
#6607=DIRECTION ( 'NONE',  ( 0.000000000000000000, -1.000000000000000000, 0.000000000000000000 ) ) ;
#6608=AXIS2_PLACEMENT_3D ( 'NONE', #45665, #49380, #24637 ) ;
#6609=ORIENTED_EDGE ( 'NONE', *, *, #43186, .T. ) ;
#6610=LINE ( 'NONE', #33312, #44770 ) ;
#6611=EDGE_CURVE ( 'NONE', #22139, #32655, #6541, .T. ) ;
#6612=ORIENTED_EDGE ( 'NONE', *, *, #41658, .F. ) ;
#6613=DIRECTION ( 'NONE',  ( 0.007781995580012663651, 0.000000000000000000, -0.9999697198139515519 ) ) ;
#6616=EDGE_CURVE ( 'NONE', #48632, #16890, #21583, .T. ) ;
#6617=CARTESIAN_POINT ( 'NONE',  ( -19.62989625882111255, -4.565544526780664469, 4.360574684536503653 ) ) ;
#6618=AXIS2_PLACEMENT_3D ( 'NONE', #16687, #34561, #21223 ) ;
#6619=ORIENTED_EDGE ( 'NONE', *, *, #37522, .T. ) ;
#6620=VECTOR ( 'NONE', #27274, 1000.000000000000227 ) ;
#6621=EDGE_CURVE ( 'NONE', #8639, #21470, #42853, .T. ) ;
#6622=CARTESIAN_POINT ( 'NONE',  ( 2.072287782118878319, 0.000000000000000000, -2.950529333540147015 ) ) ;
#6623=CARTESIAN_POINT ( 'NONE',  ( -12.03474988952295455, -0.5179957512181563306, 2.206756566172713097 ) ) ;
#6624=FACE_OUTER_BOUND ( 'NONE', #25253, .T. ) ;
#6625=CARTESIAN_POINT ( 'NONE',  ( -13.46833076279037833, 0.000000000000000000, 3.438271238299851706 ) ) ;
#6626=CARTESIAN_POINT ( 'NONE',  ( -13.13165317342551397, -0.1191753592594194527, 7.034209011106107745 ) ) ;
#6627=EDGE_LOOP ( 'NONE', ( #43377, #33752, #55801, #27306 ) ) ;
#6628=VECTOR ( 'NONE', #4042, 999.9999999999998863 ) ;
#6629=ADVANCED_FACE ( 'NONE', ( #47117 ), #29231, .F. ) ;
#6630=EDGE_LOOP ( 'NONE', ( #35466, #54308, #7503, #30337 ) ) ;
#6631=CARTESIAN_POINT ( 'NONE',  ( -13.08486533123210194, 0.000000000000000000, 1.963927175729152541 ) ) ;
#6632=LINE ( 'NONE', #19404, #31189 ) ;
#6633=VECTOR ( 'NONE', #52347, 999.9999999999998863 ) ;
#6634=CARTESIAN_POINT ( 'NONE',  ( -10.47421230394850866, 0.000000000000000000, 10.95934586908605723 ) ) ;
#6635=DIRECTION ( 'NONE',  ( 0.6427681459581294776, -0.7660444431189769032, 0.005002170337467562802 ) ) ;
#6636=EDGE_CURVE ( 'NONE', #28378, #35444, #12200, .T. ) ;
#6637=DIRECTION ( 'NONE',  ( -0.7660212471507179544, -0.6427876096865405842, -0.005961354470445141482 ) ) ;
#6638=EDGE_LOOP ( 'NONE', ( #51500, #25516, #42248, #37505 ) ) ;
#6639=PLANE ( 'NONE',  #21373 ) ;
#6640=CARTESIAN_POINT ( 'NONE',  ( 2.072287782118878319, 0.000000000000000000, -2.950529333540147015 ) ) ;
#6641=ORIENTED_EDGE ( 'NONE', *, *, #30338, .F. ) ;
#6642=VECTOR ( 'NONE', #42365, 1000.000000000000227 ) ;
#6643=DIRECTION ( 'NONE',  ( -0.5364919789714478471, 0.6444004775717705469, -0.5449076811759709926 ) ) ;
#6644=CARTESIAN_POINT ( 'NONE',  ( -24.26908309836554878, 0.000000000000000000, 6.108867788427308376 ) ) ;
#6645=ORIENTED_EDGE ( 'NONE', *, *, #21216, .T. ) ;
#6646=AXIS2_PLACEMENT_3D ( 'NONE', #1577, #53522, #6232 ) ;
#6647=VECTOR ( 'NONE', #24252, 999.9999999999998863 ) ;
#6649=LINE ( 'NONE', #24258, #12452 ) ;
#6650=LINE ( 'NONE', #1564, #39533 ) ;
#6651=LINE ( 'NONE', #35948, #27789 ) ;
#6653=EDGE_LOOP ( 'NONE', ( #18670, #3870, #21672, #36433 ) ) ;
#6654=AXIS2_PLACEMENT_3D ( 'NONE', #296, #26425, #14 ) ;
#6655=VECTOR ( 'NONE', #23066, 1000.000000000000000 ) ;
#6657=LINE ( 'NONE', #46111, #54752 ) ;
#6658=DIRECTION ( 'NONE',  ( 0.6427681459581294776, -0.7660444431189769032, 0.005002170337467562802 ) ) ;
#6659=FACE_OUTER_BOUND ( 'NONE', #5241, .T. ) ;
#6660=CARTESIAN_POINT ( 'NONE',  ( -12.80458192191714595, 0.000000000000000000, 11.86454056839041726 ) ) ;
#6661=DIRECTION ( 'NONE',  ( 0.5364919789714477361, 0.6444004775717706579, 0.5449076811759711036 ) ) ;
#6662=LINE ( 'NONE', #23976, #5898 ) ;
#6663=EDGE_CURVE ( 'NONE', #56078, #48949, #29819, .T. ) ;
#6664=ORIENTED_EDGE ( 'NONE', *, *, #31749, .F. ) ;
#6665=DIRECTION ( 'NONE',  ( 0.007781995580012663651, -3.146120232559066537E-19, -0.9999697198139514409 ) ) ;
#6666=VECTOR ( 'NONE', #10939, 1000.000000000000227 ) ;
#6667=DIRECTION ( 'NONE',  ( 0.9999697198139515519, 0.000000000000000000, 0.007781995580013368816 ) ) ;
#6668=DIRECTION ( 'NONE',  ( 0.007781995580012663651, -3.146120232559066537E-19, -0.9999697198139514409 ) ) ;
#6669=ORIENTED_EDGE ( 'NONE', *, *, #54780, .T. ) ;
#6671=DIRECTION ( 'NONE',  ( 0.9321478471874540261, 0.000000000000000000, -0.3620778797217456546 ) ) ;
#6672=VECTOR ( 'NONE', #18942, 1000.000000000000227 ) ;
#6673=ADVANCED_FACE ( 'NONE', ( #16445 ), #42579, .F. ) ;
#6674=CARTESIAN_POINT ( 'NONE',  ( 2.072287782118878319, 0.000000000000000000, -2.950529333540147015 ) ) ;
#6676=FACE_OUTER_BOUND ( 'NONE', #53165, .T. ) ;
#6677=AXIS2_PLACEMENT_3D ( 'NONE', #15383, #42360, #28437 ) ;
#6678=VERTEX_POINT ( 'NONE', #3411 ) ;
#6679=EDGE_CURVE ( 'NONE', #8091, #24779, #8221, .T. ) ;
#6680=ORIENTED_EDGE ( 'NONE', *, *, #25450, .T. ) ;
#6681=ORIENTED_EDGE ( 'NONE', *, *, #18532, .F. ) ;
#6682=ORIENTED_EDGE ( 'NONE', *, *, #12768, .T. ) ;
#6684=VECTOR ( 'NONE', #12350, 1000.000000000000227 ) ;
#6686=ORIENTED_EDGE ( 'NONE', *, *, #10964, .F. ) ;
#6688=VECTOR ( 'NONE', #28348, 1000.000000000000227 ) ;
#6690=CARTESIAN_POINT ( 'NONE',  ( -11.27597963956645089, -0.1191753592594181482, 7.417982361435909056 ) ) ;
#6691=EDGE_CURVE ( 'NONE', #22414, #5753, #20988, .T. ) ;
#6692=ORIENTED_EDGE ( 'NONE', *, *, #8618, .F. ) ;
#6693=ORIENTED_EDGE ( 'NONE', *, *, #6980, .F. ) ;
#6694=ADVANCED_FACE ( 'NONE', ( #3671 ), #4267, .F. ) ;
#6695=ORIENTED_EDGE ( 'NONE', *, *, #47633, .T. ) ;
#6696=VECTOR ( 'NONE', #49690, 1000.000000000000227 ) ;
#6697=VECTOR ( 'NONE', #19845, 1000.000000000000000 ) ;
#6698=DIRECTION ( 'NONE',  ( -0.6427681459581293666, -0.7660444431189770143, -0.005002170337467561935 ) ) ;
#6699=CARTESIAN_POINT ( 'NONE',  ( -18.12619594522237065, 0.000000000000000000, 4.879350933650815847 ) ) ;
#6700=CARTESIAN_POINT ( 'NONE',  ( -17.93139508144814442, 0.000000000000000000, 13.85596890686001537 ) ) ;
#6701=DIRECTION ( 'NONE',  ( -0.9999697198139514409, -0.000000000000000000, -0.007781995580013368816 ) ) ;
#6702=ORIENTED_EDGE ( 'NONE', *, *, #48843, .T. ) ;
#6703=DIRECTION ( 'NONE',  ( 0.9999697198139515519, 0.000000000000000000, 0.007781995580013368816 ) ) ;
#6704=ORIENTED_EDGE ( 'NONE', *, *, #45451, .T. ) ;
#6705=EDGE_CURVE ( 'NONE', #46401, #2028, #25273, .T. ) ;
#6706=VERTEX_POINT ( 'NONE', #8810 ) ;
#6707=PLANE ( 'NONE',  #11246 ) ;
#6708=CARTESIAN_POINT ( 'NONE',  ( 2.072287782118878319, 0.000000000000000000, -2.950529333540147015 ) ) ;
#6709=CARTESIAN_POINT ( 'NONE',  ( -30.79411802867772607, 0.000000000000000000, 8.643412946479525516 ) ) ;
#6710=AXIS2_PLACEMENT_3D ( 'NONE', #2048, #11710, #16243 ) ;
#6711=DIRECTION ( 'NONE',  ( 0.007781995580012663651, 0.000000000000000000, -0.9999697198139515519 ) ) ;
#6712=DIRECTION ( 'NONE',  ( 0.9999697198139515519, 0.000000000000000000, 0.007781995580013368816 ) ) ;
#6713=ORIENTED_EDGE ( 'NONE', *, *, #14409, .T. ) ;
#6714=DIRECTION ( 'NONE',  ( -0.5449076811759708816, 0.6444004775717707689, 0.5364919789714475140 ) ) ;
#6715=VECTOR ( 'NONE', #6363, 1000.000000000000227 ) ;
#6716=ORIENTED_EDGE ( 'NONE', *, *, #41092, .T. ) ;
#6717=DIRECTION ( 'NONE',  ( -0.6427681459581293666, -0.7660444431189770143, -0.005002170337467561935 ) ) ;
#6718=DIRECTION ( 'NONE',  ( 0.007781995580012662783, 0.000000000000000000, -0.9999697198139514409 ) ) ;
#6719=DIRECTION ( 'NONE',  ( 0.9999697198139515519, 0.000000000000000000, 0.007781995580013368816 ) ) ;
#6720=VECTOR ( 'NONE', #10426, 1000.000000000000000 ) ;
#6721=LINE ( 'NONE', #1880, #19529 ) ;
#6722=DIRECTION ( 'NONE',  ( 0.007781995580012662783, 0.000000000000000000, -0.9999697198139514409 ) ) ;
#6724=VECTOR ( 'NONE', #611, 1000.000000000000114 ) ;
#6725=LINE ( 'NONE', #32308, #52001 ) ;
#6726=CARTESIAN_POINT ( 'NONE',  ( -16.99924723426068951, 0.000000000000000000, 13.49389102713827171 ) ) ;
#6727=DIRECTION ( 'NONE',  ( -0.005961354470445682716, -0.6427876096865404731, 0.7660212471507180654 ) ) ;
#6728=ADVANCED_FACE ( 'NONE', ( #33772 ), #33506, .F. ) ;
#6729=VECTOR ( 'NONE', #2291, 999.9999999999998863 ) ;
#6730=LINE ( 'NONE', #24052, #39146 ) ;
#6731=DIRECTION ( 'NONE',  ( -0.000000000000000000, -1.000000000000000000, 0.000000000000000000 ) ) ;
#6733=CARTESIAN_POINT ( 'NONE',  ( 2.072287782118878319, 0.000000000000000000, -2.950529333540147015 ) ) ;
#6734=CARTESIAN_POINT ( 'NONE',  ( -19.60912206198628027, -0.1191753592594197858, 4.398475361799976113 ) ) ;
#6735=VECTOR ( 'NONE', #44794, 1000.000000000000114 ) ;
#6736=VECTOR ( 'NONE', #38207, 1000.000000000000114 ) ;
#6737=DIRECTION ( 'NONE',  ( 0.9999697198139515519, 0.000000000000000000, 0.007781995580013368816 ) ) ;
#6738=EDGE_CURVE ( 'NONE', #32684, #37529, #34353, .T. ) ;
#6739=DIRECTION ( 'NONE',  ( 0.5364919789714477361, 0.6444004775717706579, 0.5449076811759711036 ) ) ;
#6740=EDGE_CURVE ( 'NONE', #20350, #33580, #34079, .T. ) ;
#6741=ADVANCED_FACE ( 'NONE', ( #12501 ), #56200, .F. ) ;
#6742=EDGE_CURVE ( 'NONE', #29012, #5769, #34609, .T. ) ;
#6743=EDGE_LOOP ( 'NONE', ( #32775, #41751, #48940, #49886 ) ) ;
#6744=AXIS2_PLACEMENT_3D ( 'NONE', #33247, #50555, #16186 ) ;
#6745=ORIENTED_EDGE ( 'NONE', *, *, #39992, .F. ) ;
#6746=ORIENTED_EDGE ( 'NONE', *, *, #704, .T. ) ;
#6747=ORIENTED_EDGE ( 'NONE', *, *, #31131, .F. ) ;
#6748=ORIENTED_EDGE ( 'NONE', *, *, #44899, .T. ) ;
#6749=DIRECTION ( 'NONE',  ( 0.005961354470445682716, -0.6427876096865404731, -0.7660212471507180654 ) ) ;
#6750=CARTESIAN_POINT ( 'NONE',  ( -11.40636015113596180, 0.000000000000000000, 11.32142374880780089 ) ) ;
#6751=VECTOR ( 'NONE', #41, 1000.000000000000227 ) ;
#6752=ORIENTED_EDGE ( 'NONE', *, *, #13911, .T. ) ;
#6753=PLANE ( 'NONE',  #44890 ) ;
#6754=EDGE_CURVE ( 'NONE', #6764, #51258, #30376, .T. ) ;
#6755=ORIENTED_EDGE ( 'NONE', *, *, #19158, .T. ) ;
#6756=ORIENTED_EDGE ( 'NONE', *, *, #18186, .T. ) ;
#6757=ADVANCED_FACE ( 'NONE', ( #24991 ), #22677, .F. ) ;
#6758=VECTOR ( 'NONE', #17758, 1000.000000000000227 ) ;
#6760=ADVANCED_FACE ( 'NONE', ( #4797 ), #1076, .F. ) ;
#6761=VECTOR ( 'NONE', #34069, 1000.000000000000227 ) ;
#6762=DIRECTION ( 'NONE',  ( 0.000000000000000000, -1.000000000000000000, 0.000000000000000000 ) ) ;
#6763=CARTESIAN_POINT ( 'NONE',  ( -19.60990026154428278, 0.000000000000000000, 4.498472333781370125 ) ) ;
#6764=VERTEX_POINT ( 'NONE', #22427 ) ;
#6765=CARTESIAN_POINT ( 'NONE',  ( -13.23817645197547144, 0.000000000000000000, 7.872047190045031506 ) ) ;
#6766=VECTOR ( 'NONE', #25625, 1000.000000000000000 ) ;
#6767=ADVANCED_FACE ( 'NONE', ( #40582 ), #549, .F. ) ;
#6768=LINE ( 'NONE', #11592, #37277 ) ;
#6769=LINE ( 'NONE', #55293, #37509 ) ;
#6770=EDGE_CURVE ( 'NONE', #8639, #13033, #36051, .T. ) ;
#6773=DIRECTION ( 'NONE',  ( -0.6246952433987893460, -0.7422098413412802076, 0.2426528472758542054 ) ) ;
#6774=VECTOR ( 'NONE', #54476, 1000.000000000000227 ) ;
#6775=CARTESIAN_POINT ( 'NONE',  ( -10.20150221737636542, 0.000000000000000000, 1.617034104387096383 ) ) ;
#6776=DIRECTION ( 'NONE',  ( 0.007781995580012663651, -3.146120232559066537E-19, -0.9999697198139514409 ) ) ;
#6777=DIRECTION ( 'NONE',  ( -0.7660212471507179544, -0.6427876096865405842, -0.005961354470445141482 ) ) ;
#6778=LINE ( 'NONE', #41676, #53774 ) ;
#6779=VERTEX_POINT ( 'NONE', #44522 ) ;
#6780=DIRECTION ( 'NONE',  ( 0.007781995580012662783, 0.000000000000000000, -0.9999697198139514409 ) ) ;
#6781=EDGE_LOOP ( 'NONE', ( #28456, #45534, #33698, #44036 ) ) ;
#6782=CARTESIAN_POINT ( 'NONE',  ( -26.13493519185646008, 0.000000000000000000, 7.033017491833586377 ) ) ;
#6783=CARTESIAN_POINT ( 'NONE',  ( -14.07363356994439840, -1.813211359398156919, 5.124397700033340719 ) ) ;
#6784=DIRECTION ( 'NONE',  ( 0.9999697198139515519, 0.000000000000000000, 0.007781995580013368816 ) ) ;
#6785=DIRECTION ( 'NONE',  ( -0.005002170337468016433, -0.7660444431189770143, 0.6427681459581293666 ) ) ;
#6786=LINE ( 'NONE', #54747, #10468 ) ;
#6787=VECTOR ( 'NONE', #30052, 1000.000000000000227 ) ;
#6788=DIRECTION ( 'NONE',  ( -0.5449076811759708816, 0.6444004775717707689, 0.5364919789714475140 ) ) ;
#6789=AXIS2_PLACEMENT_3D ( 'NONE', #25602, #29310, #17103 ) ;
#6790=FACE_OUTER_BOUND ( 'NONE', #45076, .T. ) ;
#6791=LINE ( 'NONE', #7333, #55648 ) ;
#6792=DIRECTION ( 'NONE',  ( -0.005002170337468016433, -0.7660444431189770143, 0.6427681459581293666 ) ) ;
#6793=DIRECTION ( 'NONE',  ( -0.9999697198139514409, -0.000000000000000000, -0.007781995580013368816 ) ) ;
#6794=VECTOR ( 'NONE', #9514, 1000.000000000000227 ) ;
#6795=CARTESIAN_POINT ( 'NONE',  ( -13.07066190154808361, 0.000000000000000000, 12.04713590736729678 ) ) ;
#6796=PLANE ( 'NONE',  #6481 ) ;
#6797=AXIS2_PLACEMENT_3D ( 'NONE', #20456, #17047, #38625 ) ;
#6798=CARTESIAN_POINT ( 'NONE',  ( -21.47263955680318404, 0.000000000000000000, 5.022634149262071190 ) ) ;
#6799=DIRECTION ( 'NONE',  ( -0.005002170337468016433, -0.7660444431189770143, 0.6427681459581293666 ) ) ;
#6800=DIRECTION ( 'NONE',  ( -0.8531650599175527594, 0.4028455766673922356, 0.3313982828793700652 ) ) ;
#6801=ORIENTED_EDGE ( 'NONE', *, *, #30139, .F. ) ;
#6802=DIRECTION ( 'NONE',  ( 0.007781995580012663651, 0.000000000000000000, -0.9999697198139515519 ) ) ;
#6803=AXIS2_PLACEMENT_3D ( 'NONE', #16999, #41958, #29187 ) ;
#6804=VECTOR ( 'NONE', #41499, 999.9999999999998863 ) ;
#6805=ORIENTED_EDGE ( 'NONE', *, *, #12410, .F. ) ;
#6807=CARTESIAN_POINT ( 'NONE',  ( -33.59056157024009082, 0.000000000000000000, 9.729646585644761814 ) ) ;
#6808=VECTOR ( 'NONE', #38524, 1000.000000000000227 ) ;
#6809=LINE ( 'NONE', #24134, #33056 ) ;
#6810=VECTOR ( 'NONE', #28722, 1000.000000000000227 ) ;
#6811=EDGE_CURVE ( 'NONE', #17974, #19153, #35750, .T. ) ;
#6812=ADVANCED_FACE ( 'NONE', ( #13870 ), #31767, .F. ) ;
#6813=EDGE_LOOP ( 'NONE', ( #53295, #4976, #44860, #33084 ) ) ;
#6814=ORIENTED_EDGE ( 'NONE', *, *, #9853, .F. ) ;
#6815=FACE_OUTER_BOUND ( 'NONE', #16623, .T. ) ;
#6818=ORIENTED_EDGE ( 'NONE', *, *, #5869, .T. ) ;
#6819=AXIS2_PLACEMENT_3D ( 'NONE', #30806, #110, #8372 ) ;
#6820=EDGE_LOOP ( 'NONE', ( #7515, #41652, #28955, #40442 ) ) ;
#6821=EDGE_LOOP ( 'NONE', ( #25405, #10431, #53843, #2264 ) ) ;
#6822=DIRECTION ( 'NONE',  ( 0.005961354470445682716, -0.6427876096865404731, -0.7660212471507180654 ) ) ;
#6823=DIRECTION ( 'NONE',  ( 0.9999697198139515519, 0.000000000000000000, 0.007781995580013368816 ) ) ;
#6824=CARTESIAN_POINT ( 'NONE',  ( -27.99923088623136636, 0.000000000000000000, 7.757173251277078130 ) ) ;
#6826=VERTEX_POINT ( 'NONE', #40282 ) ;
#6827=EDGE_CURVE ( 'NONE', #51400, #40198, #14451, .T. ) ;
#6828=VECTOR ( 'NONE', #15721, 999.9999999999998863 ) ;
#6830=DIRECTION ( 'NONE',  ( 0.9999697198139515519, 0.000000000000000000, 0.007781995580013368816 ) ) ;
#6833=FACE_OUTER_BOUND ( 'NONE', #747, .T. ) ;
#6834=ORIENTED_EDGE ( 'NONE', *, *, #44318, .F. ) ;
#6835=VECTOR ( 'NONE', #8120, 1000.000000000000114 ) ;
#6836=LINE ( 'NONE', #11068, #33944 ) ;
#6837=LINE ( 'NONE', #7121, #22189 ) ;
#6838=ORIENTED_EDGE ( 'NONE', *, *, #28804, .T. ) ;
#6839=EDGE_CURVE ( 'NONE', #55994, #1128, #52763, .T. ) ;
#6841=VECTOR ( 'NONE', #33714, 1000.000000000000227 ) ;
#6842=EDGE_CURVE ( 'NONE', #42246, #28007, #5937, .T. ) ;
#6843=FACE_OUTER_BOUND ( 'NONE', #29165, .T. ) ;
#6844=VECTOR ( 'NONE', #10819, 999.9999999999998863 ) ;
#6845=VECTOR ( 'NONE', #29843, 1000.000000000000227 ) ;
#6846=ORIENTED_EDGE ( 'NONE', *, *, #7978, .T. ) ;
#6847=EDGE_CURVE ( 'NONE', #28953, #24378, #47963, .T. ) ;
#6848=CARTESIAN_POINT ( 'NONE',  ( -22.40478740399063895, 0.000000000000000000, 5.384712028983816623 ) ) ;
#6849=DIRECTION ( 'NONE',  ( 0.000000000000000000, -0.000000000000000000, -1.000000000000000000 ) ) ;
#6850=DIRECTION ( 'NONE',  ( -0.7660212471507179544, -0.6427876096865405842, -0.005961354470445141482 ) ) ;
#6851=EDGE_CURVE ( 'NONE', #37046, #34473, #35453, .T. ) ;
#6852=ORIENTED_EDGE ( 'NONE', *, *, #21676, .T. ) ;
#6853=VECTOR ( 'NONE', #25496, 1000.000000000000227 ) ;
#6854=VECTOR ( 'NONE', #4526, 1000.000000000000227 ) ;
#6855=CARTESIAN_POINT ( 'NONE',  ( 2.072287782118878319, 0.000000000000000000, -2.950529333540147015 ) ) ;
#6856=DIRECTION ( 'NONE',  ( -0.6427681459581293666, -0.7660444431189770143, -0.005002170337467561935 ) ) ;
#6858=PLANE ( 'NONE',  #9515 ) ;
#6859=CARTESIAN_POINT ( 'NONE',  ( -19.60834386242827776, 0.000000000000000000, 4.298478389818581213 ) ) ;
#6860=DIRECTION ( 'NONE',  ( 0.005002170337468016433, -0.7660444431189770143, -0.6427681459581293666 ) ) ;
#6861=CARTESIAN_POINT ( 'NONE',  ( -27.06630483948590893, -0.1191753592594197858, 7.295098399573937797 ) ) ;
#6862=AXIS2_PLACEMENT_3D ( 'NONE', #18321, #30587, #23169 ) ;
#6863=VECTOR ( 'NONE', #5456, 1000.000000000000227 ) ;
#6865=ORIENTED_EDGE ( 'NONE', *, *, #51964, .F. ) ;
#6866=CARTESIAN_POINT ( 'NONE',  ( -11.67244013076689946, 0.000000000000000000, 11.50401908778467863 ) ) ;
#6867=CARTESIAN_POINT ( 'NONE',  ( -9.879165764022332041, -0.1191753592594198830, 7.055777056291618443 ) ) ;
#6869=ORIENTED_EDGE ( 'NONE', *, *, #33116, .T. ) ;
#6870=CARTESIAN_POINT ( 'NONE',  ( -20.77435557342690231, 1.257817950434006793, 4.711265958276037225 ) ) ;
#6871=DIRECTION ( 'NONE',  ( -0.5449076811759708816, 0.6444004775717707689, 0.5364919789714475140 ) ) ;
#6872=PLANE ( 'NONE',  #47626 ) ;
#6873=DIRECTION ( 'NONE',  ( 0.007781995580012663651, -3.146120232559066537E-19, -0.9999697198139514409 ) ) ;
#6874=CARTESIAN_POINT ( 'NONE',  ( -10.42161453587613096, 0.000000000000000000, 4.200645628075444726 ) ) ;
#6876=VERTEX_POINT ( 'NONE', #1375 ) ;
#6877=ORIENTED_EDGE ( 'NONE', *, *, #23320, .F. ) ;
#6879=DIRECTION ( 'NONE',  ( 0.9999697198139515519, 0.000000000000000000, 0.007781995580013368816 ) ) ;
#6880=VECTOR ( 'NONE', #23958, 1000.000000000000227 ) ;
#6881=DIRECTION ( 'NONE',  ( 0.9999697198139515519, 0.000000000000000000, 0.007781995580013368816 ) ) ;
#6882=EDGE_CURVE ( 'NONE', #53298, #43550, #52499, .T. ) ;
#6883=EDGE_LOOP ( 'NONE', ( #46419, #26015, #45572, #20922 ) ) ;
#6884=LINE ( 'NONE', #32698, #14030 ) ;
#6885=VECTOR ( 'NONE', #43188, 999.9999999999998863 ) ;
#6886=VERTEX_POINT ( 'NONE', #30910 ) ;
#6888=ADVANCED_FACE ( 'NONE', ( #27218 ), #48220, .F. ) ;
#6889=ADVANCED_FACE ( 'NONE', ( #36579 ), #54436, .F. ) ;
#6890=VECTOR ( 'NONE', #50206, 1000.000000000000227 ) ;
#6891=VECTOR ( 'NONE', #30238, 1000.000000000000000 ) ;
#6892=ORIENTED_EDGE ( 'NONE', *, *, #52371, .F. ) ;
#6893=ORIENTED_EDGE ( 'NONE', *, *, #25514, .T. ) ;
#6894=LINE ( 'NONE', #20774, #33841 ) ;
#6895=AXIS2_PLACEMENT_3D ( 'NONE', #6709, #5885, #37347 ) ;
#6897=PLANE ( 'NONE',  #42051 ) ;
#6898=AXIS2_PLACEMENT_3D ( 'NONE', #3510, #43456, #4553 ) ;
#6899=ORIENTED_EDGE ( 'NONE', *, *, #39907, .T. ) ;
#6900=VECTOR ( 'NONE', #9011, 999.9999999999998863 ) ;
#6901=CARTESIAN_POINT ( 'NONE',  ( -13.67539046815301162, 0.000000000000000000, 4.344650004994353942 ) ) ;
#6902=VERTEX_POINT ( 'NONE', #11291 ) ;
#6903=ADVANCED_FACE ( 'NONE', ( #10753 ), #15825, .F. ) ;
#6904=AXIS2_PLACEMENT_3D ( 'NONE', #1768, #10310, #40697 ) ;
#6905=ORIENTED_EDGE ( 'NONE', *, *, #49213, .F. ) ;
#6906=AXIS2_PLACEMENT_3D ( 'NONE', #54154, #5897, #23751 ) ;
#6907=VERTEX_POINT ( 'NONE', #36301 ) ;
#6908=LINE ( 'NONE', #7175, #8695 ) ;
#6909=ORIENTED_EDGE ( 'NONE', *, *, #9002, .F. ) ;
#6910=LINE ( 'NONE', #49778, #26642 ) ;
#6911=ORIENTED_EDGE ( 'NONE', *, *, #46153, .F. ) ;
#6912=PLANE ( 'NONE',  #40365 ) ;
#6913=CARTESIAN_POINT ( 'NONE',  ( -16.91648110301675345, 4.981562823951512620, 3.093929542590271087 ) ) ;
#6914=EDGE_LOOP ( 'NONE', ( #7714, #18468, #39455, #27145 ) ) ;
#6915=CARTESIAN_POINT ( 'NONE',  ( -11.67244013076689946, 0.000000000000000000, 11.50401908778467863 ) ) ;
#6916=EDGE_LOOP ( 'NONE', ( #7862, #55693, #10027, #1048 ) ) ;
#6917=EDGE_CURVE ( 'NONE', #46950, #1369, #50488, .T. ) ;
#6918=VECTOR ( 'NONE', #5147, 1000.000000000000114 ) ;
#6919=PLANE ( 'NONE',  #37335 ) ;
#6920=CARTESIAN_POINT ( 'NONE',  ( -2.428019651919397948, -4.270454567941153634, -2.275248286963848177 ) ) ;
#6921=DIRECTION ( 'NONE',  ( 0.5449076811759707706, 0.6444004775717708799, -0.5364919789714476250 ) ) ;
#6922=CARTESIAN_POINT ( 'NONE',  ( -11.40636015113596180, 0.000000000000000000, 11.32142374880780089 ) ) ;
#6923=DIRECTION ( 'NONE',  ( 0.6427681459581294776, -0.7660444431189769032, 0.005002170337467562802 ) ) ;
#6924=CARTESIAN_POINT ( 'NONE',  ( 2.072287782118878319, 0.000000000000000000, -2.950529333540147015 ) ) ;
#6925=AXIS2_PLACEMENT_3D ( 'NONE', #55444, #25101, #42956 ) ;
#6926=ORIENTED_EDGE ( 'NONE', *, *, #37234, .F. ) ;
#6929=VECTOR ( 'NONE', #16717, 999.9999999999998863 ) ;
#6930=EDGE_CURVE ( 'NONE', #32088, #41657, #28324, .T. ) ;
#6931=CARTESIAN_POINT ( 'NONE',  ( -17.74560456716937296, 0.000000000000000000, 3.774316574337878372 ) ) ;
#6932=CARTESIAN_POINT ( 'NONE',  ( -21.06902270529800347, 1.581621852479006440, 7.660955954857441519 ) ) ;
#6933=CARTESIAN_POINT ( 'NONE',  ( -17.65081820860546813, -5.536956232915666298, 3.560840440734917234 ) ) ;
#6934=VECTOR ( 'NONE', #2459, 999.9999999999998863 ) ;
#6935=CARTESIAN_POINT ( 'NONE',  ( -16.49350878336835891, 0.000000000000000000, 8.216045510926729634 ) ) ;
#6936=ORIENTED_EDGE ( 'NONE', *, *, #22789, .T. ) ;
#6937=DIRECTION ( 'NONE',  ( 0.2426528472758542054, 0.7422098413412800966, 0.6246952433987894571 ) ) ;
#6938=DIRECTION ( 'NONE',  ( 0.6246952433987893460, 0.7422098413412802076, -0.2426528472758539279 ) ) ;
#6939=ORIENTED_EDGE ( 'NONE', *, *, #48204, .F. ) ;
#6940=CARTESIAN_POINT ( 'NONE',  ( -1.451368222102410455, 5.185123052344191130, 3.782134281800667797 ) ) ;
#6941=DIRECTION ( 'NONE',  ( -0.6427681459581293666, -0.7660444431189770143, -0.005002170337467561935 ) ) ;
#6942=ORIENTED_EDGE ( 'NONE', *, *, #33046, .F. ) ;
#6943=VECTOR ( 'NONE', #40869, 1000.000000000000000 ) ;
#6944=EDGE_CURVE ( 'NONE', #36692, #13999, #28624, .T. ) ;
#6946=CARTESIAN_POINT ( 'NONE',  ( -19.12962290826653700, 0.000000000000000000, 14.40064212555863854 ) ) ;
#6947=AXIS2_PLACEMENT_3D ( 'NONE', #15685, #2630, #50344 ) ;
#6948=DIRECTION ( 'NONE',  ( 0.5364919789714477361, 0.6444004775717706579, 0.5449076811759711036 ) ) ;
#6949=ADVANCED_FACE ( 'NONE', ( #41409 ), #14718, .F. ) ;
#6950=EDGE_CURVE ( 'NONE', #33489, #29959, #10478, .T. ) ;
#6951=DIRECTION ( 'NONE',  ( 0.005002170337468016433, -0.7660444431189770143, -0.6427681459581293666 ) ) ;
#6952=VECTOR ( 'NONE', #15524, 999.9999999999998863 ) ;
#6953=DIRECTION ( 'NONE',  ( 0.9999697198139515519, 0.000000000000000000, 0.007781995580013368816 ) ) ;
#6954=ORIENTED_EDGE ( 'NONE', *, *, #1165, .F. ) ;
#6955=AXIS2_PLACEMENT_3D ( 'NONE', #5467, #31604, #14828 ) ;
#6956=ORIENTED_EDGE ( 'NONE', *, *, #45985, .F. ) ;
#6957=CARTESIAN_POINT ( 'NONE',  ( -12.33850799832341849, 0.000000000000000000, 11.68350162852954632 ) ) ;
#6958=DIRECTION ( 'NONE',  ( -0.9999697198139514409, -0.000000000000000000, -0.007781995580013368816 ) ) ;
#6959=CARTESIAN_POINT ( 'NONE',  ( -9.110551994824897193, 0.000000000000000000, 3.538847790438064411 ) ) ;
#6960=EDGE_CURVE ( 'NONE', #41338, #51942, #27803, .T. ) ;
#6961=DIRECTION ( 'NONE',  ( 0.6427681459581294776, -0.7660444431189769032, 0.005002170337467562802 ) ) ;
#6963=EDGE_CURVE ( 'NONE', #3917, #11166, #19816, .T. ) ;
#6964=LINE ( 'NONE', #10917, #46693 ) ;
#6965=ORIENTED_EDGE ( 'NONE', *, *, #54241, .T. ) ;
#6966=CARTESIAN_POINT ( 'NONE',  ( 2.072287782118878319, 0.000000000000000000, -2.950529333540147015 ) ) ;
#6967=EDGE_CURVE ( 'NONE', #23008, #36173, #24615, .T. ) ;
#6968=VECTOR ( 'NONE', #13614, 999.9999999999998863 ) ;
#6969=CARTESIAN_POINT ( 'NONE',  ( -27.99845268667336384, -0.1191753592594197858, 7.657176279295684118 ) ) ;
#6970=FACE_OUTER_BOUND ( 'NONE', #24754, .T. ) ;
#6971=ORIENTED_EDGE ( 'NONE', *, *, #24563, .T. ) ;
#6972=DIRECTION ( 'NONE',  ( 0.000000000000000000, -0.000000000000000000, -1.000000000000000000 ) ) ;
#6973=PLANE ( 'NONE',  #18663 ) ;
#6974=LINE ( 'NONE', #46126, #20243 ) ;
#6975=EDGE_CURVE ( 'NONE', #55993, #27150, #1657, .T. ) ;
#6976=ORIENTED_EDGE ( 'NONE', *, *, #6679, .F. ) ;
#6977=LINE ( 'NONE', #46389, #54918 ) ;
#6978=AXIS2_PLACEMENT_3D ( 'NONE', #24592, #11565, #7282 ) ;
#6979=ORIENTED_EDGE ( 'NONE', *, *, #53792, .T. ) ;
#6980=EDGE_CURVE ( 'NONE', #35417, #14078, #18982, .T. ) ;
#6981=ORIENTED_EDGE ( 'NONE', *, *, #2052, .F. ) ;
#6982=VECTOR ( 'NONE', #34028, 1000.000000000000000 ) ;
#6983=ORIENTED_EDGE ( 'NONE', *, *, #51950, .T. ) ;
#6984=ORIENTED_EDGE ( 'NONE', *, *, #44079, .T. ) ;
#6985=ORIENTED_EDGE ( 'NONE', *, *, #23359, .F. ) ;
#6986=DIRECTION ( 'NONE',  ( 0.9999697198139515519, 0.000000000000000000, 0.007781995580013368816 ) ) ;
#6988=VECTOR ( 'NONE', #42252, 1000.000000000000000 ) ;
#6989=ORIENTED_EDGE ( 'NONE', *, *, #44960, .T. ) ;
#6990=CARTESIAN_POINT ( 'NONE',  ( -14.16520784441536662, 2.229229656569005957, 6.042114544152918043 ) ) ;
#6991=VERTEX_POINT ( 'NONE', #45945 ) ;
#6992=ORIENTED_EDGE ( 'NONE', *, *, #41203, .T. ) ;
#6993=VECTOR ( 'NONE', #50290, 1000.000000000000227 ) ;
#6994=CARTESIAN_POINT ( 'NONE',  ( -18.19747506107908563, 0.000000000000000000, 14.03856424583689311 ) ) ;
#6995=CARTESIAN_POINT ( 'NONE',  ( -16.03058795173162920, -0.8417996532631574214, 3.081288062448307663 ) ) ;
#6996=PLANE ( 'NONE',  #25058 ) ;
#6997=LINE ( 'NONE', #49299, #23276 ) ;
#6998=CARTESIAN_POINT ( 'NONE',  ( -24.27063949748155380, 0.000000000000000000, 6.308861732390097288 ) ) ;
#6999=ORIENTED_EDGE ( 'NONE', *, *, #54811, .F. ) ;
#7000=ORIENTED_EDGE ( 'NONE', *, *, #44997, .F. ) ;
#7001=CARTESIAN_POINT ( 'NONE',  ( -27.06708303904391144, 0.000000000000000000, 7.395095371555332697 ) ) ;
#7002=EDGE_CURVE ( 'NONE', #55978, #19207, #49656, .T. ) ;
#7003=FACE_OUTER_BOUND ( 'NONE', #2731, .T. ) ;
#7004=VECTOR ( 'NONE', #48880, 999.9999999999998863 ) ;
#7005=FACE_OUTER_BOUND ( 'NONE', #6638, .T. ) ;
#7006=EDGE_CURVE ( 'NONE', #38002, #25423, #32597, .T. ) ;
#7007=PLANE ( 'NONE',  #31386 ) ;
#7008=CARTESIAN_POINT ( 'NONE',  ( -12.74611667447084251, 0.000000000000000000, 4.351881828530372864 ) ) ;
#7009=LINE ( 'NONE', #10960, #30437 ) ;
#7010=ORIENTED_EDGE ( 'NONE', *, *, #39150, .F. ) ;
#7011=CARTESIAN_POINT ( 'NONE',  ( -13.07066190154808361, 0.000000000000000000, 12.04713590736729678 ) ) ;
#7012=VERTEX_POINT ( 'NONE', #1912 ) ;
#7013=EDGE_CURVE ( 'NONE', #7579, #27972, #24352, .T. ) ;
#7014=FACE_OUTER_BOUND ( 'NONE', #40520, .T. ) ;
#7015=PLANE ( 'NONE',  #42356 ) ;
#7016=AXIS2_PLACEMENT_3D ( 'NONE', #21113, #8636, #12880 ) ;
#7017=DIRECTION ( 'NONE',  ( -0.7660212471507179544, -0.6427876096865405842, -0.005961354470445141482 ) ) ;
#7018=CARTESIAN_POINT ( 'NONE',  ( -15.13495153988577968, 0.000000000000000000, 12.76973526769478084 ) ) ;
#7019=EDGE_CURVE ( 'NONE', #17655, #33054, #19246, .T. ) ;
#7020=CARTESIAN_POINT ( 'NONE',  ( -15.88053067323648371, -0.1191753592594190225, 2.950163842912993939 ) ) ;
#7021=CIRCLE ( 'NONE', #30582, 2.125000000000000000 ) ;
#7022=ORIENTED_EDGE ( 'NONE', *, *, #766, .F. ) ;
#7024=DIRECTION ( 'NONE',  ( 0.6427681459581294776, -0.7660444431189769032, 0.005002170337467562802 ) ) ;
#7025=DIRECTION ( 'NONE',  ( 0.005002170337468016433, -0.7660444431189770143, -0.6427681459581293666 ) ) ;
#7027=FACE_OUTER_BOUND ( 'NONE', #31184, .T. ) ;
#7028=EDGE_CURVE ( 'NONE', #873, #46046, #37398, .T. ) ;
#7029=CARTESIAN_POINT ( 'NONE',  ( 2.072287782118878319, 0.000000000000000000, -2.950529333540147015 ) ) ;
#7030=LINE ( 'NONE', #2175, #4623 ) ;
#7031=CARTESIAN_POINT ( 'NONE',  ( -10.94028622754223967, 0.000000000000000000, 11.14038480894692995 ) ) ;
#7032=ADVANCED_FACE ( 'NONE', ( #54720 ), #19538, .F. ) ;
#7033=FACE_OUTER_BOUND ( 'NONE', #18093, .T. ) ;
#7034=CARTESIAN_POINT ( 'NONE',  ( -23.33849165029409889, 0.000000000000000000, 5.946783852668351855 ) ) ;
#7035=ORIENTED_EDGE ( 'NONE', *, *, #49838, .T. ) ;
#7036=ADVANCED_FACE ( 'NONE', ( #16124 ), #55873, .F. ) ;
#7037=ORIENTED_EDGE ( 'NONE', *, *, #2880, .F. ) ;
#7038=EDGE_CURVE ( 'NONE', #20767, #39658, #47058, .T. ) ;
#7039=ORIENTED_EDGE ( 'NONE', *, *, #33930, .F. ) ;
#7040=ORIENTED_EDGE ( 'NONE', *, *, #47911, .F. ) ;
#7041=VERTEX_POINT ( 'NONE', #3613 ) ;
#7042=VERTEX_POINT ( 'NONE', #33702 ) ;
#7043=LINE ( 'NONE', #41401, #4243 ) ;
#7044=CARTESIAN_POINT ( 'NONE',  ( -20.48739968382506405, 3.686347215771509589, 4.522319747380798560 ) ) ;
#7045=PLANE ( 'NONE',  #27643 ) ;
#7046=ORIENTED_EDGE ( 'NONE', *, *, #20839, .F. ) ;
#7047=EDGE_LOOP ( 'NONE', ( #3544, #29454, #16168, #24602, #55140 ) ) ;
#7048=VERTEX_POINT ( 'NONE', #29160 ) ;
#7049=PLANE ( 'NONE',  #20454 ) ;
#7050=ORIENTED_EDGE ( 'NONE', *, *, #7885, .F. ) ;
#7051=VECTOR ( 'NONE', #50149, 1000.000000000000000 ) ;
#7053=DIRECTION ( 'NONE',  ( 0.007781995580012663651, -3.146120232559066537E-19, -0.9999697198139514409 ) ) ;
#7054=DIRECTION ( 'NONE',  ( 0.007781995580012662783, 0.000000000000000000, -0.9999697198139514409 ) ) ;
#7055=ORIENTED_EDGE ( 'NONE', *, *, #33265, .T. ) ;
#7056=PLANE ( 'NONE',  #39160 ) ;
#7057=ORIENTED_EDGE ( 'NONE', *, *, #55520, .F. ) ;
#7059=DIRECTION ( 'NONE',  ( 0.5364919789714477361, 0.6444004775717706579, 0.5449076811759711036 ) ) ;
#7060=EDGE_CURVE ( 'NONE', #25539, #30922, #56145, .T. ) ;
#7061=PLANE ( 'NONE',  #44775 ) ;
#7062=FACE_OUTER_BOUND ( 'NONE', #19501, .T. ) ;
#7063=LINE ( 'NONE', #19548, #35134 ) ;
#7064=ADVANCED_FACE ( 'NONE', ( #8163 ), #42779, .F. ) ;
#7065=DIRECTION ( 'NONE',  ( 0.9999697198139515519, 0.000000000000000000, 0.007781995580013368816 ) ) ;
#7066=DIRECTION ( 'NONE',  ( -0.7660212471507179544, -0.6427876096865405842, -0.005961354470445141482 ) ) ;
#7067=CARTESIAN_POINT ( 'NONE',  ( -31.72782227498118601, 0.000000000000000000, 9.205484770164058972 ) ) ;
#7068=EDGE_CURVE ( 'NONE', #43270, #30652, #41934, .T. ) ;
#7069=DIRECTION ( 'NONE',  ( -0.5449076811759708816, 0.6444004775717707689, 0.5364919789714475140 ) ) ;
#7070=DIRECTION ( 'NONE',  ( 0.000000000000000000, -1.000000000000000000, 0.000000000000000000 ) ) ;
#7071=EDGE_LOOP ( 'NONE', ( #24673, #2794, #53827, #55925 ) ) ;
#7072=LINE ( 'NONE', #7918, #39225 ) ;
#7073=ORIENTED_EDGE ( 'NONE', *, *, #2534, .T. ) ;
#7074=EDGE_CURVE ( 'NONE', #33995, #10709, #51601, .T. ) ;
#7075=EDGE_CURVE ( 'NONE', #50804, #12359, #46786, .T. ) ;
#7076=EDGE_CURVE ( 'NONE', #16783, #48336, #3037, .T. ) ;
#7077=CARTESIAN_POINT ( 'NONE',  ( -25.20278734466900517, 0.000000000000000000, 6.670939612111840944 ) ) ;
#7078=DIRECTION ( 'NONE',  ( -0.7660212471507179544, -0.6427876096865405842, -0.005961354470445141482 ) ) ;
#7079=FACE_OUTER_BOUND ( 'NONE', #16825, .T. ) ;
#7080=CARTESIAN_POINT ( 'NONE',  ( -27.06552663992790997, 0.000000000000000000, 7.195101427592543786 ) ) ;
#7081=FACE_OUTER_BOUND ( 'NONE', #13026, .T. ) ;
#7082=LINE ( 'NONE', #28930, #45538 ) ;
#7085=PLANE ( 'NONE',  #2024 ) ;
#7086=LINE ( 'NONE', #10778, #23910 ) ;
#7087=DIRECTION ( 'NONE',  ( 0.6427681459581294776, -0.7660444431189769032, 0.005002170337467562802 ) ) ;
#7088=CARTESIAN_POINT ( 'NONE',  ( -17.74482636761137044, -0.1191753592594197858, 3.674319602356483916 ) ) ;
#7089=DIRECTION ( 'NONE',  ( 0.9999697198139515519, 0.000000000000000000, 0.007781995580013368816 ) ) ;
#7090=LINE ( 'NONE', #3642, #11895 ) ;
#7091=EDGE_CURVE ( 'NONE', #42498, #29609, #3885, .T. ) ;
#7092=FACE_OUTER_BOUND ( 'NONE', #48936, .T. ) ;
#7093=CARTESIAN_POINT ( 'NONE',  ( -28.92982233430281980, 0.000000000000000000, 7.919257187036034651 ) ) ;
#7094=LINE ( 'NONE', #49404, #37422 ) ;
#7095=EDGE_LOOP ( 'NONE', ( #48864, #17265, #20511, #29446 ) ) ;
#7096=EDGE_CURVE ( 'NONE', #9163, #46599, #21210, .T. ) ;
#7097=DIRECTION ( 'NONE',  ( 0.9999697198139515519, 0.000000000000000000, 0.007781995580013368816 ) ) ;
#7098=VERTEX_POINT ( 'NONE', #25214 ) ;
#7099=ADVANCED_FACE ( 'NONE', ( #48377 ), #30019, .F. ) ;
#7100=DIRECTION ( 'NONE',  ( -0.005961354470445682716, -0.6427876096865404731, 0.7660212471507180654 ) ) ;
#7101=CARTESIAN_POINT ( 'NONE',  ( -19.36023273628322983, -4.727446477803162850, 11.96064866101106716 ) ) ;
#7102=EDGE_CURVE ( 'NONE', #47628, #3649, #20920, .T. ) ;
#7103=VECTOR ( 'NONE', #13761, 1000.000000000000000 ) ;
#7104=ORIENTED_EDGE ( 'NONE', *, *, #46221, .T. ) ;
#7105=ORIENTED_EDGE ( 'NONE', *, *, #21392, .T. ) ;
#7106=CARTESIAN_POINT ( 'NONE',  ( -0.8462754142284378833, 3.710276453311750267, 3.547095686184165153 ) ) ;
#7107=ORIENTED_EDGE ( 'NONE', *, *, #54546, .F. ) ;
#7108=ORIENTED_EDGE ( 'NONE', *, *, #39592, .F. ) ;
#7109=VERTEX_POINT ( 'NONE', #29762 ) ;
#7110=PLANE ( 'NONE',  #36563 ) ;
#7112=LINE ( 'NONE', #16176, #5843 ) ;
#7113=ORIENTED_EDGE ( 'NONE', *, *, #41797, .T. ) ;
#7114=ORIENTED_EDGE ( 'NONE', *, *, #26471, .F. ) ;
#7115=DIRECTION ( 'NONE',  ( 0.5364919789714477361, 0.6444004775717706579, 0.5449076811759711036 ) ) ;
#7116=CARTESIAN_POINT ( 'NONE',  ( -18.29747203306047609, -0.1191753592594177458, 14.03778604627889059 ) ) ;
#7117=EDGE_LOOP ( 'NONE', ( #40148, #21455, #42706, #34078 ) ) ;
#7118=CARTESIAN_POINT ( 'NONE',  ( -27.06552663992790997, 0.000000000000000000, 7.195101427592543786 ) ) ;
#7119=ORIENTED_EDGE ( 'NONE', *, *, #17490, .F. ) ;
#7120=DIRECTION ( 'NONE',  ( 0.007781995580012662783, 0.000000000000000000, -0.9999697198139514409 ) ) ;
#7121=CARTESIAN_POINT ( 'NONE',  ( -16.06709938707323460, 0.000000000000000000, 13.13181314741652628 ) ) ;
#7122=ORIENTED_EDGE ( 'NONE', *, *, #25788, .T. ) ;
#7123=CARTESIAN_POINT ( 'NONE',  ( -14.93495759592298988, 0.000000000000000000, 12.77129166681078409 ) ) ;
#7124=FACE_OUTER_BOUND ( 'NONE', #46118, .T. ) ;
#7125=ORIENTED_EDGE ( 'NONE', *, *, #23973, .T. ) ;
#7126=LINE ( 'NONE', #53977, #12221 ) ;
#7127=LINE ( 'NONE', #45441, #27559 ) ;
#7128=DIRECTION ( 'NONE',  ( 0.6427681459581294776, -0.7660444431189769032, 0.005002170337467562802 ) ) ;
#7130=ADVANCED_FACE ( 'NONE', ( #24921 ), #25760, .F. ) ;
#7131=ADVANCED_FACE ( 'NONE', ( #42244 ), #13737, .F. ) ;
#7132=AXIS2_PLACEMENT_3D ( 'NONE', #14292, #17690, #48908 ) ;
#7133=PLANE ( 'NONE',  #43727 ) ;
#7135=PLANE ( 'NONE',  #55708 ) ;
#7136=DIRECTION ( 'NONE',  ( -0.5449076811759708816, 0.6444004775717707689, 0.5364919789714475140 ) ) ;
#7137=EDGE_CURVE ( 'NONE', #33896, #29311, #20668, .T. ) ;
#7138=CARTESIAN_POINT ( 'NONE',  ( -9.442067484779661513, -0.1191753592594197858, 10.59804618892231254 ) ) ;
#7139=FACE_OUTER_BOUND ( 'NONE', #22201, .T. ) ;
#7141=EDGE_LOOP ( 'NONE', ( #49008, #7470, #34409, #686 ) ) ;
#7142=CARTESIAN_POINT ( 'NONE',  ( -20.54049170961573267, 0.000000000000000000, 4.660556269540326646 ) ) ;
#7143=CARTESIAN_POINT ( 'NONE',  ( -22.64140378624534833, -5.375054281893165253, 5.504518879977243095 ) ) ;
#7145=EDGE_LOOP ( 'NONE', ( #22747, #33256, #14511, #3103 ) ) ;
#7146=CARTESIAN_POINT ( 'NONE',  ( -15.87975247367846166, 0.000000000000000000, 2.850166870931599927 ) ) ;
#7147=LINE ( 'NONE', #54276, #40877 ) ;
#7148=CARTESIAN_POINT ( 'NONE',  ( -16.41782547135460391, -0.1941918491731542684, 3.252366345260954805 ) ) ;
#7149=DIRECTION ( 'NONE',  ( 0.005961354470445682716, -0.6427876096865404731, -0.7660212471507180654 ) ) ;
#7150=ADVANCED_FACE ( 'NONE', ( #9793 ), #14332, .F. ) ;
#7151=CARTESIAN_POINT ( 'NONE',  ( -13.30267207010766839, 4.010151117816511679, 1.721196508061384023 ) ) ;
#7152=ORIENTED_EDGE ( 'NONE', *, *, #2260, .T. ) ;
#7153=EDGE_LOOP ( 'NONE', ( #50530, #28836, #31836, #34535 ) ) ;
#7155=FACE_OUTER_BOUND ( 'NONE', #51508, .T. ) ;
#7156=DIRECTION ( 'NONE',  ( 0.6427681459581294776, -0.7660444431189769032, 0.005002170337467562802 ) ) ;
#7157=DIRECTION ( 'NONE',  ( -0.5449076811759708816, 0.6444004775717707689, 0.5364919789714475140 ) ) ;
#7158=ADVANCED_FACE ( 'NONE', ( #49218 ), #35912, .F. ) ;
#7159=ORIENTED_EDGE ( 'NONE', *, *, #48328, .F. ) ;
#7160=CARTESIAN_POINT ( 'NONE',  ( -14.05805291360240261, -0.1191753592594190225, 6.657667484312323580 ) ) ;
#7161=ORIENTED_EDGE ( 'NONE', *, *, #24253, .F. ) ;
#7162=DIRECTION ( 'NONE',  ( 0.5449076811759707706, 0.6444004775717708799, -0.5364919789714476250 ) ) ;
#7163=EDGE_CURVE ( 'NONE', #51867, #1451, #1786, .T. ) ;
#7164=ORIENTED_EDGE ( 'NONE', *, *, #28272, .F. ) ;
#7165=ORIENTED_EDGE ( 'NONE', *, *, #16838, .F. ) ;
#7166=CARTESIAN_POINT ( 'NONE',  ( -18.66354898467281132, 0.000000000000000000, 14.21960318569776582 ) ) ;
#7167=FACE_OUTER_BOUND ( 'NONE', #38365, .T. ) ;
#7168=DIRECTION ( 'NONE',  ( -0.9999697198139514409, -0.000000000000000000, -0.007781995580013368816 ) ) ;
#7169=ORIENTED_EDGE ( 'NONE', *, *, #29158, .F. ) ;
#7170=AXIS2_PLACEMENT_3D ( 'NONE', #2583, #45455, #23881 ) ;
#7171=CARTESIAN_POINT ( 'NONE',  ( -13.17065887352947762, -0.1191753592594197858, 12.04635770780929427 ) ) ;
#7172=ORIENTED_EDGE ( 'NONE', *, *, #23422, .F. ) ;
#7173=EDGE_LOOP ( 'NONE', ( #17696, #38260, #43587, #46463 ) ) ;
#7174=ORIENTED_EDGE ( 'NONE', *, *, #41913, .T. ) ;
#7175=CARTESIAN_POINT ( 'NONE',  ( -13.53673582514181106, 0.000000000000000000, 12.22817484722816772 ) ) ;
#7176=CARTESIAN_POINT ( 'NONE',  ( -16.33317936670417225, 0.000000000000000000, 13.31440848639340224 ) ) ;
#7178=DIRECTION ( 'NONE',  ( 0.005002170337468016433, -0.7660444431189770143, -0.6427681459581293666 ) ) ;
#7179=ORIENTED_EDGE ( 'NONE', *, *, #5487, .T. ) ;
#7180=LINE ( 'NONE', #19386, #11337 ) ;
#7181=CARTESIAN_POINT ( 'NONE',  ( -11.40636015113596180, 0.000000000000000000, 11.32142374880780089 ) ) ;
#7182=ORIENTED_EDGE ( 'NONE', *, *, #9445, .F. ) ;
#7183=FACE_OUTER_BOUND ( 'NONE', #26999, .T. ) ;
#7184=ORIENTED_EDGE ( 'NONE', *, *, #672, .F. ) ;
#7185=CARTESIAN_POINT ( 'NONE',  ( -14.93495759592298988, 0.000000000000000000, 12.77129166681078409 ) ) ;
#7186=PLANE ( 'NONE',  #19348 ) ;
#7187=PLANE ( 'NONE',  #13264 ) ;
#7188=CARTESIAN_POINT ( 'NONE',  ( -13.03950016240196597, 0.000000000000000000, 8.042919348456010198 ) ) ;
#7190=CARTESIAN_POINT ( 'NONE',  ( -15.42180871032122091, -0.1191753592594190225, 2.771980654253273002 ) ) ;
#7191=ORIENTED_EDGE ( 'NONE', *, *, #44195, .F. ) ;
#7192=ADVANCED_FACE ( 'NONE', ( #49786 ), #36437, .F. ) ;
#7193=VERTEX_POINT ( 'NONE', #44401 ) ;
#7194=PLANE ( 'NONE',  #40046 ) ;
#7195=CARTESIAN_POINT ( 'NONE',  ( -8.878251335088286567, 6.547824941322106795, 0.2302407495689529626 ) ) ;
#7196=DIRECTION ( 'NONE',  ( 0.007781995580012663651, 0.000000000000000000, -0.9999697198139515519 ) ) ;
#7197=EDGE_CURVE ( 'NONE', #27809, #20135, #26815, .T. ) ;
#7198=ADVANCED_FACE ( 'NONE', ( #14586 ), #32195, .F. ) ;
#7199=CARTESIAN_POINT ( 'NONE',  ( -15.57823159443524119, 0.6102101463440037232, 3.933894115644549050 ) ) ;
#7200=CARTESIAN_POINT ( 'NONE',  ( -30.79567442779373110, 0.000000000000000000, 8.843406890442315316 ) ) ;
#7201=CARTESIAN_POINT ( 'NONE',  ( -10.74029228357944987, 0.000000000000000000, 11.14194120806293320 ) ) ;
#7202=ORIENTED_EDGE ( 'NONE', *, *, #23360, .F. ) ;
#7203=DIRECTION ( 'NONE',  ( -0.5449076811759708816, 0.6444004775717707689, 0.5364919789714475140 ) ) ;
#7204=PLANE ( 'NONE',  #34124 ) ;
#7205=VERTEX_POINT ( 'NONE', #18863 ) ;
#7206=DIRECTION ( 'NONE',  ( 0.9999697198139515519, 0.000000000000000000, 0.007781995580013368816 ) ) ;
#7207=DIRECTION ( 'NONE',  ( 0.9999697198139515519, 0.000000000000000000, 0.007781995580013368816 ) ) ;
#7208=ORIENTED_EDGE ( 'NONE', *, *, #21365, .F. ) ;
#7209=DIRECTION ( 'NONE',  ( -0.5449076811759708816, 0.6444004775717707689, 0.5364919789714475140 ) ) ;
#7210=LINE ( 'NONE', #24799, #45955 ) ;
#7211=CARTESIAN_POINT ( 'NONE',  ( -14.06667507411825113, -0.1191753592594177180, 7.765596594085615756 ) ) ;
#7212=DIRECTION ( 'NONE',  ( 0.5364919789714477361, 0.6444004775717706579, 0.5449076811759711036 ) ) ;
#7214=ORIENTED_EDGE ( 'NONE', *, *, #24051, .T. ) ;
#7215=EDGE_LOOP ( 'NONE', ( #32331, #27930, #18466, #10040 ) ) ;
#7216=LINE ( 'NONE', #10367, #42062 ) ;
#7217=DIRECTION ( 'NONE',  ( 0.005002170337468016433, -0.7660444431189770143, -0.6427681459581293666 ) ) ;
#7218=CARTESIAN_POINT ( 'NONE',  ( -18.67775241435682432, 0.000000000000000000, 4.136394454059623804 ) ) ;
#7219=DIRECTION ( 'NONE',  ( -0.9999697198139514409, -0.000000000000000000, -0.007781995580013368816 ) ) ;
#7220=LINE ( 'NONE', #37892, #20118 ) ;
#7221=CARTESIAN_POINT ( 'NONE',  ( -18.13326170662221415, 0.000000000000000000, 5.787286099461318223 ) ) ;
#7223=CARTESIAN_POINT ( 'NONE',  ( -12.34488701508258224, -3.108426967578160838, 1.577319373299684857 ) ) ;
#7224=ADVANCED_FACE ( 'NONE', ( #53750 ), #6099, .F. ) ;
#7225=CARTESIAN_POINT ( 'NONE',  ( -9.110551994824897193, 0.000000000000000000, 3.538847790438064411 ) ) ;
#7226=DIRECTION ( 'NONE',  ( 0.5449076811759707706, 0.6444004775717708799, -0.5364919789714476250 ) ) ;
#7227=EDGE_LOOP ( 'NONE', ( #27587, #54717, #21827, #3055, #53404 ) ) ;
#7228=EDGE_CURVE ( 'NONE', #7431, #16954, #6349, .T. ) ;
#7229=CARTESIAN_POINT ( 'NONE',  ( -25.20123094555300369, 0.000000000000000000, 6.470945668149052032 ) ) ;
#7230=PLANE ( 'NONE',  #29569 ) ;
#7231=EDGE_CURVE ( 'NONE', #16077, #10405, #23651, .T. ) ;
#7232=DIRECTION ( 'NONE',  ( -0.7660212471507179544, -0.6427876096865405842, -0.005961354470445141482 ) ) ;
#7233=ORIENTED_EDGE ( 'NONE', *, *, #6131, .F. ) ;
#7234=LINE ( 'NONE', #16045, #15041 ) ;
#7235=ADVANCED_FACE ( 'NONE', ( #48951 ), #10043, .F. ) ;
#7236=ORIENTED_EDGE ( 'NONE', *, *, #42285, .T. ) ;
#7237=ORIENTED_EDGE ( 'NONE', *, *, #16116, .F. ) ;
#7238=ORIENTED_EDGE ( 'NONE', *, *, #28815, .T. ) ;
#7239=VERTEX_POINT ( 'NONE', #44673 ) ;
#7240=EDGE_LOOP ( 'NONE', ( #39555, #20125, #24406, #50361 ) ) ;
#7241=FACE_OUTER_BOUND ( 'NONE', #22292, .T. ) ;
#7242=ORIENTED_EDGE ( 'NONE', *, *, #23546, .F. ) ;
#7243=ORIENTED_EDGE ( 'NONE', *, *, #46969, .T. ) ;
#7244=FACE_OUTER_BOUND ( 'NONE', #5773, .T. ) ;
#7245=ORIENTED_EDGE ( 'NONE', *, *, #38550, .T. ) ;
#7246=EDGE_LOOP ( 'NONE', ( #44820, #21683, #16798, #12114 ) ) ;
#7247=ADVANCED_FACE ( 'NONE', ( #19392 ), #40445, .F. ) ;
#7248=FACE_OUTER_BOUND ( 'NONE', #13283, .T. ) ;
#7249=DIRECTION ( 'NONE',  ( 0.5449076811759707706, 0.6444004775717708799, -0.5364919789714476250 ) ) ;
#7250=DIRECTION ( 'NONE',  ( 0.005961354470445682716, -0.6427876096865404731, -0.7660212471507180654 ) ) ;
#7251=CARTESIAN_POINT ( 'NONE',  ( -20.60218203966579864, 2.714935509636508204, 4.597898231738893671 ) ) ;
#7252=EDGE_CURVE ( 'NONE', #22744, #36173, #5252, .T. ) ;
#7253=LINE ( 'NONE', #37923, #11993 ) ;
#7254=ORIENTED_EDGE ( 'NONE', *, *, #8648, .T. ) ;
#7255=ORIENTED_EDGE ( 'NONE', *, *, #25517, .T. ) ;
#7256=EDGE_CURVE ( 'NONE', #19170, #12005, #1534, .T. ) ;
#7258=CARTESIAN_POINT ( 'NONE',  ( -11.21901323774118708, 0.000000000000000000, 1.039777472322872098 ) ) ;
#7259=ADVANCED_FACE ( 'NONE', ( #10331 ), #948, .F. ) ;
#7260=CARTESIAN_POINT ( 'NONE',  ( -26.13337879274045505, 0.000000000000000000, 6.833023547870798353 ) ) ;
#7261=CARTESIAN_POINT ( 'NONE',  ( -15.88053067323646417, -0.1191753592594197858, 2.950163842912994383 ) ) ;
#7262=CARTESIAN_POINT ( 'NONE',  ( -12.73330280606043097, 0.000000000000000000, 2.705327256204338671 ) ) ;
#7263=EDGE_LOOP ( 'NONE', ( #41067, #5901, #18043, #10744 ) ) ;
#7264=FACE_OUTER_BOUND ( 'NONE', #43826, .T. ) ;
#7265=ORIENTED_EDGE ( 'NONE', *, *, #34974, .F. ) ;
#7266=CARTESIAN_POINT ( 'NONE',  ( -13.53673582514181106, 0.000000000000000000, 12.22817484722816772 ) ) ;
#7267=FACE_OUTER_BOUND ( 'NONE', #16725, .T. ) ;
#7268=FACE_OUTER_BOUND ( 'NONE', #54246, .T. ) ;
#7269=CARTESIAN_POINT ( 'NONE',  ( -15.13495153988577968, 0.000000000000000000, 12.76973526769478084 ) ) ;
#7270=CARTESIAN_POINT ( 'NONE',  ( -25.20123094555300369, 0.000000000000000000, 6.470945668149052032 ) ) ;
#7271=EDGE_CURVE ( 'NONE', #23572, #52995, #37016, .T. ) ;
#7272=AXIS2_PLACEMENT_3D ( 'NONE', #42196, #55247, #29417 ) ;
#7273=ORIENTED_EDGE ( 'NONE', *, *, #16541, .F. ) ;
#7275=CARTESIAN_POINT ( 'NONE',  ( -19.49786065871724006, 4.172053068839010059, 4.122452625480004684 ) ) ;
#7276=DIRECTION ( 'NONE',  ( 0.5364919789714477361, 0.6444004775717706579, 0.5449076811759711036 ) ) ;
#7277=CARTESIAN_POINT ( 'NONE',  ( -12.60458797795435615, 0.000000000000000000, 11.86609696750642229 ) ) ;
#7278=FACE_OUTER_BOUND ( 'NONE', #23375, .T. ) ;
#7279=LINE ( 'NONE', #11561, #40292 ) ;
#7280=FACE_OUTER_BOUND ( 'NONE', #43465, .T. ) ;
#7281=DIRECTION ( 'NONE',  ( -0.5449076811759708816, 0.6444004775717707689, 0.5364919789714475140 ) ) ;
#7282=DIRECTION ( 'NONE',  ( -0.005002170337468016433, -0.7660444431189770143, 0.6427681459581293666 ) ) ;
#7284=ORIENTED_EDGE ( 'NONE', *, *, #53807, .F. ) ;
#7285=EDGE_CURVE ( 'NONE', #41663, #17974, #20530, .T. ) ;
#7286=EDGE_LOOP ( 'NONE', ( #50859, #12695, #12469, #47159 ) ) ;
#7287=ORIENTED_EDGE ( 'NONE', *, *, #14689, .F. ) ;
#7288=ORIENTED_EDGE ( 'NONE', *, *, #6366, .T. ) ;
#7289=ORIENTED_EDGE ( 'NONE', *, *, #15125, .F. ) ;
#7290=CARTESIAN_POINT ( 'NONE',  ( -14.93495759592298988, 0.000000000000000000, 12.77129166681078409 ) ) ;
#7291=LINE ( 'NONE', #3025, #43821 ) ;
#7293=EDGE_CURVE ( 'NONE', #9458, #49209, #50624, .T. ) ;
#7294=ORIENTED_EDGE ( 'NONE', *, *, #29078, .F. ) ;
#7295=ORIENTED_EDGE ( 'NONE', *, *, #21527, .T. ) ;
#7296=EDGE_LOOP ( 'NONE', ( #19943, #41513, #50942, #19681, #35246 ) ) ;
#7297=FACE_OUTER_BOUND ( 'NONE', #30712, .T. ) ;
#7298=EDGE_CURVE ( 'NONE', #6114, #22808, #45501, .T. ) ;
#7299=EDGE_LOOP ( 'NONE', ( #15333, #4560, #25063, #42109 ) ) ;
#7300=EDGE_CURVE ( 'NONE', #41467, #16440, #29034, .T. ) ;
#7301=VECTOR ( 'NONE', #31307, 999.9999999999998863 ) ;
#7303=CARTESIAN_POINT ( 'NONE',  ( -13.27065584551087163, 0.000000000000000000, 12.04557950825129176 ) ) ;
#7304=FACE_OUTER_BOUND ( 'NONE', #29447, .T. ) ;
#7305=EDGE_CURVE ( 'NONE', #21379, #43081, #28189, .T. ) ;
#7306=ORIENTED_EDGE ( 'NONE', *, *, #23052, .T. ) ;
#7307=CARTESIAN_POINT ( 'NONE',  ( -11.04000237409175078, -1.003701604285657911, 1.137609623205984244 ) ) ;
#7308=EDGE_LOOP ( 'NONE', ( #48443, #31680, #39904, #36091 ) ) ;
#7309=CARTESIAN_POINT ( 'NONE',  ( -15.60102546347950536, 0.000000000000000000, 12.95077420755565356 ) ) ;
#7310=ADVANCED_FACE ( 'NONE', ( #3195 ), #54880, .F. ) ;
#7311=CARTESIAN_POINT ( 'NONE',  ( -17.14604581469821909, 3.038739411681509850, 3.245086511306461752 ) ) ;
#7312=ADVANCED_FACE ( 'NONE', ( #37858 ), #19949, .F. ) ;
#7313=LINE ( 'NONE', #11847, #6988 ) ;
#7314=PLANE ( 'NONE',  #43126 ) ;
#7315=PLANE ( 'NONE',  #9326 ) ;
#7316=DIRECTION ( 'NONE',  ( 0.007781995580012663651, -3.146120232559066537E-19, -0.9999697198139514409 ) ) ;
#7317=CARTESIAN_POINT ( 'NONE',  ( -11.67244013076689946, 0.000000000000000000, 11.50401908778467863 ) ) ;
#7318=FACE_OUTER_BOUND ( 'NONE', #42612, .T. ) ;
#7319=ORIENTED_EDGE ( 'NONE', *, *, #25183, .F. ) ;
#7320=LINE ( 'NONE', #45660, #13814 ) ;
#7321=ORIENTED_EDGE ( 'NONE', *, *, #851, .F. ) ;
#7322=EDGE_CURVE ( 'NONE', #9106, #10102, #55164, .T. ) ;
#7323=VECTOR ( 'NONE', #47770, 999.9999999999998863 ) ;
#7324=DIRECTION ( 'NONE',  ( 0.9999697198139515519, 0.000000000000000000, 0.007781995580013368816 ) ) ;
#7325=LINE ( 'NONE', #29184, #5156 ) ;
#7326=CARTESIAN_POINT ( 'NONE',  ( -14.94916102560700821, 0.000000000000000000, 2.688082935172642962 ) ) ;
#7327=LINE ( 'NONE', #2226, #12368 ) ;
#7328=DIRECTION ( 'NONE',  ( -0.005002170337468016433, -0.7660444431189770143, 0.6427681459581293666 ) ) ;
#7329=EDGE_CURVE ( 'NONE', #19098, #48276, #28775, .T. ) ;
#7330=CARTESIAN_POINT ( 'NONE',  ( -15.03495456790438389, -0.1191753592594197858, 12.77051346725278158 ) ) ;
#7331=ORIENTED_EDGE ( 'NONE', *, *, #12950, .F. ) ;
#7332=DIRECTION ( 'NONE',  ( 0.6427681459581294776, -0.7660444431189769032, 0.005002170337467562802 ) ) ;
#7333=CARTESIAN_POINT ( 'NONE',  ( -11.67244013076689946, 0.000000000000000000, 11.50401908778467863 ) ) ;
#7334=DIRECTION ( 'NONE',  ( -0.9999697198139514409, -0.000000000000000000, -0.007781995580013368816 ) ) ;
#7335=CARTESIAN_POINT ( 'NONE',  ( -13.08408713167409942, -0.1191753592594197858, 1.863930203747758085 ) ) ;
#7336=FACE_OUTER_BOUND ( 'NONE', #17214, .T. ) ;
#7337=AXIS2_PLACEMENT_3D ( 'NONE', #31579, #18206, #35533 ) ;
#7338=DIRECTION ( 'NONE',  ( 0.8531650599175529814, -0.4028455766673920135, -0.3313982828793697877 ) ) ;
#7339=DIRECTION ( 'NONE',  ( -0.9999697198139514409, -0.000000000000000000, -0.007781995580013368816 ) ) ;
#7340=LINE ( 'NONE', #54761, #49501 ) ;
#7341=FACE_OUTER_BOUND ( 'NONE', #29879, .T. ) ;
#7342=EDGE_LOOP ( 'NONE', ( #52812, #49636, #14250, #10871, #29337 ) ) ;
#7343=VECTOR ( 'NONE', #17005, 1000.000000000000227 ) ;
#7344=DIRECTION ( 'NONE',  ( -0.7660212471507179544, -0.6427876096865405842, -0.005961354470445141482 ) ) ;
#7345=DIRECTION ( 'NONE',  ( 0.7660212471507180654, -0.6427876096865404731, 0.005961354470445141482 ) ) ;
#7346=ORIENTED_EDGE ( 'NONE', *, *, #7947, .T. ) ;
#7347=LINE ( 'NONE', #1957, #25940 ) ;
#7348=DIRECTION ( 'NONE',  ( 0.5364919789714477361, 0.6444004775717706579, 0.5449076811759711036 ) ) ;
#7349=ORIENTED_EDGE ( 'NONE', *, *, #43431, .T. ) ;
#7350=EDGE_CURVE ( 'NONE', #16502, #53402, #3483, .T. ) ;
#7351=ORIENTED_EDGE ( 'NONE', *, *, #8364, .F. ) ;
#7352=CARTESIAN_POINT ( 'NONE',  ( -12.42445214995601077, 4.010151117816509903, 8.288741439567777647 ) ) ;
#7353=ORIENTED_EDGE ( 'NONE', *, *, #10690, .T. ) ;
#7354=ORIENTED_EDGE ( 'NONE', *, *, #30523, .F. ) ;
#7355=VERTEX_POINT ( 'NONE', #16251 ) ;
#7356=FACE_OUTER_BOUND ( 'NONE', #47162, .T. ) ;
#7357=CARTESIAN_POINT ( 'NONE',  ( -11.14646393297422833, 0.000000000000000000, 3.625666556434874455 ) ) ;
#7358=CARTESIAN_POINT ( 'NONE',  ( -31.72782227498118601, 0.000000000000000000, 9.205484770164058972 ) ) ;
#7359=ADVANCED_FACE ( 'NONE', ( #55425 ), #6919, .F. ) ;
#7360=EDGE_CURVE ( 'NONE', #50224, #21780, #33572, .T. ) ;
#7362=VECTOR ( 'NONE', #14456, 999.9999999999998863 ) ;
#7363=VERTEX_POINT ( 'NONE', #50879 ) ;
#7364=ORIENTED_EDGE ( 'NONE', *, *, #52558, .F. ) ;
#7365=EDGE_CURVE ( 'NONE', #54304, #17269, #46079, .T. ) ;
#7366=CARTESIAN_POINT ( 'NONE',  ( -15.44653166369588781, 4.819660872929010687, 10.79116317270894143 ) ) ;
#7367=CARTESIAN_POINT ( 'NONE',  ( -14.29221109521548883, 3.524445264749011208, 2.121063629962177011 ) ) ;
#7368=EDGE_LOOP ( 'NONE', ( #18118, #24141, #31352, #32680 ) ) ;
#7369=LINE ( 'NONE', #15083, #39132 ) ;
#7370=ORIENTED_EDGE ( 'NONE', *, *, #36836, .T. ) ;
#7371=PLANE ( 'NONE',  #30349 ) ;
#7372=FACE_OUTER_BOUND ( 'NONE', #31373, .T. ) ;
#7373=VERTEX_POINT ( 'NONE', #41266 ) ;
#7374=PLANE ( 'NONE',  #1403 ) ;
#7375=EDGE_CURVE ( 'NONE', #18842, #15384, #2358, .T. ) ;
#7376=AXIS2_PLACEMENT_3D ( 'NONE', #44273, #26369, #9330 ) ;
#7377=EDGE_CURVE ( 'NONE', #27029, #48144, #2627, .T. ) ;
#7378=CARTESIAN_POINT ( 'NONE',  ( -17.46532115785441519, 0.000000000000000000, 13.67492996699914265 ) ) ;
#7379=ORIENTED_EDGE ( 'NONE', *, *, #33779, .T. ) ;
#7380=CARTESIAN_POINT ( 'NONE',  ( -11.35951049007415037, 0.000000000000000000, 5.301342914312717980 ) ) ;
#7381=LINE ( 'NONE', #19328, #36646 ) ;
#7382=EDGE_CURVE ( 'NONE', #20189, #28225, #54570, .T. ) ;
#7383=PLANE ( 'NONE',  #175 ) ;
#7384=ORIENTED_EDGE ( 'NONE', *, *, #21204, .T. ) ;
#7385=EDGE_CURVE ( 'NONE', #2815, #47582, #41799, .T. ) ;
#7386=PLANE ( 'NONE',  #49161 ) ;
#7387=CARTESIAN_POINT ( 'NONE',  ( 2.072287782118878319, 0.000000000000000000, -2.950529333540147015 ) ) ;
#7389=FACE_OUTER_BOUND ( 'NONE', #26945, .T. ) ;
#7390=DIRECTION ( 'NONE',  ( -0.5449076811759708816, 0.6444004775717707689, 0.5364919789714475140 ) ) ;
#7391=LINE ( 'NONE', #7689, #8933 ) ;
#7392=LINE ( 'NONE', #21010, #2250 ) ;
#7393=EDGE_LOOP ( 'NONE', ( #12076, #23199, #29751, #16167 ) ) ;
#7394=CARTESIAN_POINT ( 'NONE',  ( -19.60912206198628027, -0.1191753592594197858, 4.398475361799976113 ) ) ;
#7395=CARTESIAN_POINT ( 'NONE',  ( -27.99767448711536133, 0.000000000000000000, 7.557179307314289218 ) ) ;
#7396=CARTESIAN_POINT ( 'NONE',  ( -14.56888064431065821, -0.1191753592594197858, 12.58947452739191064 ) ) ;
#7397=ORIENTED_EDGE ( 'NONE', *, *, #4387, .T. ) ;
#7398=LINE ( 'NONE', #33809, #35641 ) ;
#7399=LINE ( 'NONE', #24719, #38154 ) ;
#7400=AXIS2_PLACEMENT_3D ( 'NONE', #13513, #12672, #39649 ) ;
#7401=VECTOR ( 'NONE', #46084, 1000.000000000000227 ) ;
#7402=CARTESIAN_POINT ( 'NONE',  ( -11.13077601105853454, 0.000000000000000000, 1.609802280851077461 ) ) ;
#7403=FACE_OUTER_BOUND ( 'NONE', #5446, .T. ) ;
#7404=CARTESIAN_POINT ( 'NONE',  ( -16.75084723012008681, 0.000000000000000000, 7.275372647796405801 ) ) ;
#7405=EDGE_LOOP ( 'NONE', ( #36180, #55034, #29758, #21340 ) ) ;
#7406=VECTOR ( 'NONE', #21753, 999.9999999999998863 ) ;
#7407=ORIENTED_EDGE ( 'NONE', *, *, #8870, .T. ) ;
#7408=CARTESIAN_POINT ( 'NONE',  ( -16.92210063903004524, 0.000000000000000000, 3.580719216102757230 ) ) ;
#7409=ADVANCED_FACE ( 'NONE', ( #4879 ), #21907, .F. ) ;
#7410=DIRECTION ( 'NONE',  ( 0.000000000000000000, -0.000000000000000000, -1.000000000000000000 ) ) ;
#7411=ORIENTED_EDGE ( 'NONE', *, *, #43525, .F. ) ;
#7412=DIRECTION ( 'NONE',  ( 0.000000000000000000, -1.000000000000000000, 0.000000000000000000 ) ) ;
#7413=VECTOR ( 'NONE', #41117, 1000.000000000000114 ) ;
#7414=EDGE_CURVE ( 'NONE', #30062, #13266, #25345, .T. ) ;
#7415=ORIENTED_EDGE ( 'NONE', *, *, #35188, .F. ) ;
#7416=LINE ( 'NONE', #20770, #38372 ) ;
#7417=VECTOR ( 'NONE', #47475, 1000.000000000000227 ) ;
#7418=ORIENTED_EDGE ( 'NONE', *, *, #1814, .T. ) ;
#7419=ORIENTED_EDGE ( 'NONE', *, *, #54953, .F. ) ;
#7420=ORIENTED_EDGE ( 'NONE', *, *, #3998, .F. ) ;
#7421=ADVANCED_FACE ( 'NONE', ( #13125 ), #21372, .F. ) ;
#7422=CARTESIAN_POINT ( 'NONE',  ( -15.42322306907283114, -0.1191753592594189393, 2.953722716430651651 ) ) ;
#7423=LINE ( 'NONE', #38093, #16879 ) ;
#7424=DIRECTION ( 'NONE',  ( 0.6427681459581294776, -0.7660444431189769032, 0.005002170337467562802 ) ) ;
#7425=EDGE_CURVE ( 'NONE', #42825, #37960, #3743, .T. ) ;
#7426=EDGE_CURVE ( 'NONE', #2679, #41874, #51728, .T. ) ;
#7427=EDGE_CURVE ( 'NONE', #9180, #41679, #30464, .T. ) ;
#7428=FACE_OUTER_BOUND ( 'NONE', #49055, .T. ) ;
#7429=ORIENTED_EDGE ( 'NONE', *, *, #19999, .F. ) ;
#7430=EDGE_CURVE ( 'NONE', #40269, #6551, #323, .T. ) ;
#7431=VERTEX_POINT ( 'NONE', #9134 ) ;
#7432=ORIENTED_EDGE ( 'NONE', *, *, #24417, .F. ) ;
#7433=CARTESIAN_POINT ( 'NONE',  ( -21.01797471916702165, 2.067327705546507133, 8.438253235298647681 ) ) ;
#7434=DIRECTION ( 'NONE',  ( 0.007781995580012663651, -3.146120232559066537E-19, -0.9999697198139514409 ) ) ;
#7436=CARTESIAN_POINT ( 'NONE',  ( -11.71475005485999077, -0.1191753592594185784, 4.090579120348019515 ) ) ;
#7437=EDGE_LOOP ( 'NONE', ( #21125, #12984, #32146, #43957 ) ) ;
#7438=CARTESIAN_POINT ( 'NONE',  ( -18.17847529190681044, 4.819660872929011575, 3.589296462945613886 ) ) ;
#7439=LINE ( 'NONE', #45242, #22252 ) ;
#7440=VECTOR ( 'NONE', #46835, 999.9999999999998863 ) ;
#7441=VECTOR ( 'NONE', #49378, 1000.000000000000227 ) ;
#7442=EDGE_LOOP ( 'NONE', ( #40895, #33270, #55616, #40434 ) ) ;
#7443=DIRECTION ( 'NONE',  ( 0.000000000000000000, -1.000000000000000000, 0.000000000000000000 ) ) ;
#7445=ORIENTED_EDGE ( 'NONE', *, *, #47699, .T. ) ;
#7446=ADVANCED_FACE ( 'NONE', ( #26443 ), #47780, .F. ) ;
#7447=VECTOR ( 'NONE', #33422, 1000.000000000000227 ) ;
#7448=DIRECTION ( 'NONE',  ( -0.9999697198139514409, -0.000000000000000000, -0.007781995580013368816 ) ) ;
#7449=DIRECTION ( 'NONE',  ( 0.007781995580012663651, 0.000000000000000000, -0.9999697198139515519 ) ) ;
#7450=AXIS2_PLACEMENT_3D ( 'NONE', #13364, #34368, #12517 ) ;
#7451=DIRECTION ( 'NONE',  ( 0.7660212471507180654, -0.6427876096865404731, 0.005961354470445141482 ) ) ;
#7452=CARTESIAN_POINT ( 'NONE',  ( -20.54049170961573267, 0.000000000000000000, 4.660556269540326646 ) ) ;
#7454=CARTESIAN_POINT ( 'NONE',  ( -10.27421835998572064, 0.000000000000000000, 10.96090226820206048 ) ) ;
#7455=PLANE ( 'NONE',  #14673 ) ;
#7456=EDGE_LOOP ( 'NONE', ( #7917, #29300, #14272, #3555 ) ) ;
#7457=EDGE_CURVE ( 'NONE', #40214, #45690, #21655, .T. ) ;
#7458=ORIENTED_EDGE ( 'NONE', *, *, #40840, .F. ) ;
#7459=CARTESIAN_POINT ( 'NONE',  ( -21.47419595591918906, 0.000000000000000000, 5.222628093224860102 ) ) ;
#7460=FACE_OUTER_BOUND ( 'NONE', #5498, .T. ) ;
#7461=VECTOR ( 'NONE', #1860, 999.9999999999998863 ) ;
#7462=CARTESIAN_POINT ( 'NONE',  ( -17.22985439448759237, 0.000000000000000000, 9.118305252317219001 ) ) ;
#7463=LINE ( 'NONE', #32740, #8597 ) ;
#7464=EDGE_CURVE ( 'NONE', #41663, #20135, #8293, .T. ) ;
#7465=PLANE ( 'NONE',  #6184 ) ;
#7466=LINE ( 'NONE', #3500, #34948 ) ;
#7467=VERTEX_POINT ( 'NONE', #8589 ) ;
#7468=DIRECTION ( 'NONE',  ( 0.005961354470445682716, -0.6427876096865404731, -0.7660212471507180654 ) ) ;
#7469=PLANE ( 'NONE',  #51348 ) ;
#7470=ORIENTED_EDGE ( 'NONE', *, *, #27277, .F. ) ;
#7471=DIRECTION ( 'NONE',  ( 0.005961354470445682716, -0.6427876096865404731, -0.7660212471507180654 ) ) ;
#7472=LINE ( 'NONE', #25103, #53088 ) ;
#7473=ORIENTED_EDGE ( 'NONE', *, *, #52297, .T. ) ;
#7475=LINE ( 'NONE', #25106, #20589 ) ;
#7476=LINE ( 'NONE', #33596, #55860 ) ;
#7477=VECTOR ( 'NONE', #2089, 1000.000000000000227 ) ;
#7478=PLANE ( 'NONE',  #46830 ) ;
#7480=ORIENTED_EDGE ( 'NONE', *, *, #5733, .T. ) ;
#7481=ORIENTED_EDGE ( 'NONE', *, *, #35313, .T. ) ;
#7482=DIRECTION ( 'NONE',  ( 0.005002170337468016433, -0.7660444431189770143, -0.6427681459581293666 ) ) ;
#7483=PLANE ( 'NONE',  #46708 ) ;
#7484=AXIS2_PLACEMENT_3D ( 'NONE', #42138, #12026, #12342 ) ;
#7485=DIRECTION ( 'NONE',  ( -0.005002170337468016433, -0.7660444431189770143, 0.6427681459581293666 ) ) ;
#7486=VECTOR ( 'NONE', #4773, 1000.000000000000227 ) ;
#7487=PLANE ( 'NONE',  #1416 ) ;
#7488=VECTOR ( 'NONE', #11795, 999.9999999999998863 ) ;
#7489=CARTESIAN_POINT ( 'NONE',  ( -13.08330893211609869, 0.000000000000000000, 1.763933231766363630 ) ) ;
#7490=DIRECTION ( 'NONE',  ( 0.9999697198139515519, 0.000000000000000000, 0.007781995580013368816 ) ) ;
#7491=ORIENTED_EDGE ( 'NONE', *, *, #5821, .T. ) ;
#7492=DIRECTION ( 'NONE',  ( -0.3620778797217455991, 0.000000000000000000, -0.9321478471874540261 ) ) ;
#7493=DIRECTION ( 'NONE',  ( 0.005961354470445682716, -0.6427876096865404731, -0.7660212471507180654 ) ) ;
#7494=VECTOR ( 'NONE', #19925, 999.9999999999998863 ) ;
#7495=DIRECTION ( 'NONE',  ( -0.5364919789714478471, 0.6444004775717705469, -0.5449076811759709926 ) ) ;
#7496=AXIS2_PLACEMENT_3D ( 'NONE', #7266, #54149, #14674 ) ;
#7497=VERTEX_POINT ( 'NONE', #43496 ) ;
#7498=DIRECTION ( 'NONE',  ( 0.9999697198139515519, 0.000000000000000000, 0.007781995580013368816 ) ) ;
#7500=PLANE ( 'NONE',  #15704 ) ;
#7501=ADVANCED_FACE ( 'NONE', ( #42937 ), #52012, .F. ) ;
#7502=EDGE_CURVE ( 'NONE', #11834, #45314, #52317, .T. ) ;
#7503=ORIENTED_EDGE ( 'NONE', *, *, #2183, .T. ) ;
#7504=PLANE ( 'NONE',  #39526 ) ;
#7505=AXIS2_PLACEMENT_3D ( 'NONE', #8230, #17297, #42328 ) ;
#7506=ORIENTED_EDGE ( 'NONE', *, *, #46260, .F. ) ;
#7507=EDGE_CURVE ( 'NONE', #27679, #9163, #48036, .T. ) ;
#7508=VECTOR ( 'NONE', #37838, 999.9999999999998863 ) ;
#7509=ORIENTED_EDGE ( 'NONE', *, *, #49014, .F. ) ;
#7510=ORIENTED_EDGE ( 'NONE', *, *, #13855, .F. ) ;
#7511=ORIENTED_EDGE ( 'NONE', *, *, #34226, .T. ) ;
#7512=CARTESIAN_POINT ( 'NONE',  ( -13.08486533123210194, 0.000000000000000000, 1.963927175729152541 ) ) ;
#7513=VERTEX_POINT ( 'NONE', #12290 ) ;
#7514=VECTOR ( 'NONE', #49850, 1000.000000000000227 ) ;
#7515=ORIENTED_EDGE ( 'NONE', *, *, #42110, .T. ) ;
#7516=CARTESIAN_POINT ( 'NONE',  ( -22.40634380310664397, 0.000000000000000000, 5.584705972946605534 ) ) ;
#7517=ORIENTED_EDGE ( 'NONE', *, *, #46510, .T. ) ;
#7518=VECTOR ( 'NONE', #5677, 999.9999999999998863 ) ;
#7519=ORIENTED_EDGE ( 'NONE', *, *, #40515, .F. ) ;
#7520=CARTESIAN_POINT ( 'NONE',  ( -10.56836678998424439, 0.000000000000000000, 7.323486140140572864 ) ) ;
#7521=CARTESIAN_POINT ( 'NONE',  ( -10.94028622754223967, 0.000000000000000000, 11.14038480894692995 ) ) ;
#7522=LINE ( 'NONE', #20862, #46820 ) ;
#7523=PLANE ( 'NONE',  #50468 ) ;
#7524=VECTOR ( 'NONE', #43472, 999.9999999999998863 ) ;
#7525=DIRECTION ( 'NONE',  ( 0.9999697198139515519, 0.000000000000000000, 0.007781995580013368816 ) ) ;
#7526=ORIENTED_EDGE ( 'NONE', *, *, #11910, .F. ) ;
#7527=VECTOR ( 'NONE', #40759, 999.9999999999998863 ) ;
#7528=AXIS2_PLACEMENT_3D ( 'NONE', #34635, #17060, #47729 ) ;
#7529=EDGE_LOOP ( 'NONE', ( #31090, #10802, #55890, #6979, #10366 ) ) ;
#7530=DIRECTION ( 'NONE',  ( -0.5449076811759708816, 0.6444004775717707689, 0.5364919789714475140 ) ) ;
#7531=PLANE ( 'NONE',  #55672 ) ;
#7532=EDGE_CURVE ( 'NONE', #16077, #9942, #29626, .T. ) ;
#7533=DIRECTION ( 'NONE',  ( 0.5364919789714477361, 0.6444004775717706579, 0.5449076811759711036 ) ) ;
#7534=AXIS2_PLACEMENT_3D ( 'NONE', #42436, #16041, #46685 ) ;
#7535=VECTOR ( 'NONE', #4616, 1000.000000000000227 ) ;
#7536=DIRECTION ( 'NONE',  ( 0.007781995580012663651, 0.000000000000000000, -0.9999697198139515519 ) ) ;
#7537=EDGE_CURVE ( 'NONE', #16969, #38002, #55717, .T. ) ;
#7538=DIRECTION ( 'NONE',  ( 0.000000000000000000, 1.000000000000000000, 0.000000000000000000 ) ) ;
#7539=FACE_OUTER_BOUND ( 'NONE', #23124, .T. ) ;
#7540=EDGE_LOOP ( 'NONE', ( #53400, #33002, #3843, #377 ) ) ;
#7542=CARTESIAN_POINT ( 'NONE',  ( -15.06067899816041944, 0.000000000000000000, 3.225873159917031607 ) ) ;
#7543=EDGE_LOOP ( 'NONE', ( #50998, #44873, #55700, #45754 ) ) ;
#7544=DIRECTION ( 'NONE',  ( 0.6427681459581294776, -0.7660444431189769032, 0.005002170337467562802 ) ) ;
#7545=LINE ( 'NONE', #8124, #49580 ) ;
#7546=LINE ( 'NONE', #33127, #37183 ) ;
#7547=EDGE_CURVE ( 'NONE', #33592, #30111, #9414, .T. ) ;
#7548=VECTOR ( 'NONE', #42318, 1000.000000000000227 ) ;
#7549=CARTESIAN_POINT ( 'NONE',  ( -12.10890871433051430, 0.000000000000000000, 7.880835412697054565 ) ) ;
#7550=VECTOR ( 'NONE', #9001, 1000.000000000000227 ) ;
#7551=CARTESIAN_POINT ( 'NONE',  ( -19.51855023662962196, 0.000000000000000000, 4.668509254383998552 ) ) ;
#7552=ORIENTED_EDGE ( 'NONE', *, *, #52997, .T. ) ;
#7553=EDGE_LOOP ( 'NONE', ( #33492, #38053, #42759, #5303 ) ) ;
#7554=PLANE ( 'NONE',  #32994 ) ;
#7557=VECTOR ( 'NONE', #2968, 1000.000000000000227 ) ;
#7558=CARTESIAN_POINT ( 'NONE',  ( -18.76354595665420177, -0.1191753592594177458, 14.21882498613976331 ) ) ;
#7559=LINE ( 'NONE', #24886, #13100 ) ;
#7560=VECTOR ( 'NONE', #42053, 1000.000000000000227 ) ;
#7562=FACE_OUTER_BOUND ( 'NONE', #21457, .T. ) ;
#7564=VECTOR ( 'NONE', #31622, 1000.000000000000227 ) ;
#7565=LINE ( 'NONE', #24896, #40125 ) ;
#7566=ORIENTED_EDGE ( 'NONE', *, *, #38628, .T. ) ;
#7568=VECTOR ( 'NONE', #55167, 999.9999999999998863 ) ;
#7569=AXIS2_PLACEMENT_3D ( 'NONE', #9032, #13008, #30634 ) ;
#7570=EDGE_CURVE ( 'NONE', #47896, #33244, #18800, .T. ) ;
#7571=ORIENTED_EDGE ( 'NONE', *, *, #2961, .T. ) ;
#7572=ADVANCED_FACE ( 'NONE', ( #40652 ), #19049, .F. ) ;
#7573=ADVANCED_FACE ( 'NONE', ( #53681 ), #40070, .F. ) ;
#7574=VECTOR ( 'NONE', #36102, 1000.000000000000114 ) ;
#7575=ORIENTED_EDGE ( 'NONE', *, *, #52634, .T. ) ;
#7576=ORIENTED_EDGE ( 'NONE', *, *, #21982, .F. ) ;
#7577=VECTOR ( 'NONE', #40866, 1000.000000000000114 ) ;
#7578=EDGE_LOOP ( 'NONE', ( #7010, #33690, #55851, #53161 ) ) ;
#7579=VERTEX_POINT ( 'NONE', #5719 ) ;
#7580=CARTESIAN_POINT ( 'NONE',  ( -17.83139810946674686, -0.1191753592594197858, 13.85674710641801788 ) ) ;
#7581=CARTESIAN_POINT ( 'NONE',  ( -13.23949410636475399, 0.000000000000000000, 8.041362949340008726 ) ) ;
#7582=FACE_OUTER_BOUND ( 'NONE', #14446, .T. ) ;
#7583=ORIENTED_EDGE ( 'NONE', *, *, #6950, .T. ) ;
#7584=CARTESIAN_POINT ( 'NONE',  ( -9.040517713763286167, 0.000000000000000000, 5.858047935705506859 ) ) ;
#7585=VERTEX_POINT ( 'NONE', #10566 ) ;
#7587=ORIENTED_EDGE ( 'NONE', *, *, #37225, .T. ) ;
#7588=EDGE_CURVE ( 'NONE', #53603, #53756, #36372, .T. ) ;
#7591=CARTESIAN_POINT ( 'NONE',  ( -13.08486533123210194, 0.000000000000000000, 1.963927175729152541 ) ) ;
#7593=ORIENTED_EDGE ( 'NONE', *, *, #40873, .T. ) ;
#7594=DIRECTION ( 'NONE',  ( 0.5449076811759707706, 0.6444004775717708799, -0.5364919789714476250 ) ) ;
#7595=VECTOR ( 'NONE', #4743, 999.9999999999998863 ) ;
#7596=ORIENTED_EDGE ( 'NONE', *, *, #37646, .T. ) ;
#7597=DIRECTION ( 'NONE',  ( 0.5364919789714477361, 0.6444004775717706579, 0.5449076811759711036 ) ) ;
#7598=DIRECTION ( 'NONE',  ( -0.5364919789714478471, 0.6444004775717705469, -0.5449076811759709926 ) ) ;
#7599=VECTOR ( 'NONE', #46488, 1000.000000000000114 ) ;
#7600=DIRECTION ( 'NONE',  ( 0.5449076811759707706, 0.6444004775717708799, -0.5364919789714476250 ) ) ;
#7601=FACE_OUTER_BOUND ( 'NONE', #54326, .T. ) ;
#7603=LINE ( 'NONE', #47071, #44822 ) ;
#7605=AXIS2_PLACEMENT_3D ( 'NONE', #50017, #45229, #28171 ) ;
#7606=CARTESIAN_POINT ( 'NONE',  ( -30.79567442779373110, 0.000000000000000000, 8.843406890442315316 ) ) ;
#7607=VERTEX_POINT ( 'NONE', #39807 ) ;
#7608=LINE ( 'NONE', #46491, #52800 ) ;
#7609=ORIENTED_EDGE ( 'NONE', *, *, #3116, .T. ) ;
#7610=AXIS2_PLACEMENT_3D ( 'NONE', #20739, #21595, #8231 ) ;
#7611=DIRECTION ( 'NONE',  ( -0.7660212471507179544, -0.6427876096865405842, -0.005961354470445141482 ) ) ;
#7612=FACE_OUTER_BOUND ( 'NONE', #54522, .T. ) ;
#7613=CARTESIAN_POINT ( 'NONE',  ( -8.380637751107304467, 0.000000000000000000, 6.473697885849892586 ) ) ;
#7614=EDGE_CURVE ( 'NONE', #7363, #39093, #36121, .T. ) ;
#7615=CARTESIAN_POINT ( 'NONE',  ( -20.44938042942779433, 0.000000000000000000, 4.861271374810767654 ) ) ;
#7616=DIRECTION ( 'NONE',  ( 0.000000000000000000, -1.000000000000000000, 0.000000000000000000 ) ) ;
#7617=AXIS2_PLACEMENT_3D ( 'NONE', #51632, #26097, #20702 ) ;
#7618=CARTESIAN_POINT ( 'NONE',  ( -17.59819193477204990, 0.000000000000000000, 10.05410896024298140 ) ) ;
#7619=VECTOR ( 'NONE', #15502, 999.9999999999998863 ) ;
#7621=ORIENTED_EDGE ( 'NONE', *, *, #38261, .T. ) ;
#7622=DIRECTION ( 'NONE',  ( 0.9999697198139515519, 0.000000000000000000, 0.007781995580013368816 ) ) ;
#7623=DIRECTION ( 'NONE',  ( 0.007781995580012663651, 0.000000000000000000, -0.9999697198139515519 ) ) ;
#7624=DIRECTION ( 'NONE',  ( 0.005961354470445682716, -0.6427876096865404731, -0.7660212471507180654 ) ) ;
#7625=CARTESIAN_POINT ( 'NONE',  ( -13.66524968089654379, -5.698858183938163791, 11.34277594356301222 ) ) ;
#7626=EDGE_CURVE ( 'NONE', #51521, #3481, #884, .T. ) ;
#7627=CARTESIAN_POINT ( 'NONE',  ( -17.36532418587302473, -0.1191753592594177458, 13.67570816655714516 ) ) ;
#7628=CARTESIAN_POINT ( 'NONE',  ( -27.99767448711536133, 0.000000000000000000, 7.557179307314289218 ) ) ;
#7629=EDGE_CURVE ( 'NONE', #33817, #48888, #14799, .T. ) ;
#7630=LINE ( 'NONE', #7093, #25115 ) ;
#7631=ADVANCED_FACE ( 'NONE', ( #30982 ), #10256, .F. ) ;
#7632=LINE ( 'NONE', #25249, #50076 ) ;
#7633=ORIENTED_EDGE ( 'NONE', *, *, #39599, .F. ) ;
#7634=VECTOR ( 'NONE', #2690, 1000.000000000000227 ) ;
#7636=DIRECTION ( 'NONE',  ( -0.005961354470445682716, -0.6427876096865404731, 0.7660212471507180654 ) ) ;
#7637=VERTEX_POINT ( 'NONE', #44903 ) ;
#7638=AXIS2_PLACEMENT_3D ( 'NONE', #34408, #55698, #47764 ) ;
#7639=ORIENTED_EDGE ( 'NONE', *, *, #46679, .T. ) ;
#7640=CARTESIAN_POINT ( 'NONE',  ( -15.56136093618090044, 0.000000000000000000, 7.853967631204984201 ) ) ;
#7641=EDGE_CURVE ( 'NONE', #49508, #20663, #32123, .T. ) ;
#7642=VECTOR ( 'NONE', #20020, 1000.000000000000227 ) ;
#7643=VERTEX_POINT ( 'NONE', #35833 ) ;
#7644=ADVANCED_FACE ( 'NONE', ( #44339 ), #53159, .F. ) ;
#7645=VECTOR ( 'NONE', #38833, 999.9999999999998863 ) ;
#7646=ORIENTED_EDGE ( 'NONE', *, *, #51174, .F. ) ;
#7647=LINE ( 'NONE', #7106, #14789 ) ;
#7648=EDGE_CURVE ( 'NONE', #8596, #2376, #23590, .T. ) ;
#7649=ORIENTED_EDGE ( 'NONE', *, *, #672, .T. ) ;
#7650=ORIENTED_EDGE ( 'NONE', *, *, #33647, .T. ) ;
#7652=DIRECTION ( 'NONE',  ( -0.6427681459581293666, -0.7660444431189770143, -0.005002170337467561935 ) ) ;
#7653=AXIS2_PLACEMENT_3D ( 'NONE', #19806, #36043, #2192 ) ;
#7655=FACE_OUTER_BOUND ( 'NONE', #47512, .T. ) ;
#7656=AXIS2_PLACEMENT_3D ( 'NONE', #48173, #4749, #45259 ) ;
#7657=EDGE_CURVE ( 'NONE', #25423, #39170, #9723, .T. ) ;
#7658=ORIENTED_EDGE ( 'NONE', *, *, #36965, .F. ) ;
#7660=ADVANCED_FACE ( 'NONE', ( #44065 ), #22496, .F. ) ;
#7661=AXIS2_PLACEMENT_3D ( 'NONE', #29985, #8134, #30272 ) ;
#7662=AXIS2_PLACEMENT_3D ( 'NONE', #211, #34889, #25251 ) ;
#7663=FACE_OUTER_BOUND ( 'NONE', #11897, .T. ) ;
#7664=CARTESIAN_POINT ( 'NONE',  ( -17.69449129132867071, 0.000000000000000000, 9.114689340549208652 ) ) ;
#7665=ORIENTED_EDGE ( 'NONE', *, *, #27272, .T. ) ;
#7666=DIRECTION ( 'NONE',  ( 0.7660212471507180654, -0.6427876096865404731, 0.005961354470445141482 ) ) ;
#7667=ORIENTED_EDGE ( 'NONE', *, *, #42333, .F. ) ;
#7668=DIRECTION ( 'NONE',  ( 0.7660212471507180654, -0.6427876096865404731, 0.005961354470445141482 ) ) ;
#7669=DIRECTION ( 'NONE',  ( 0.007781995580012662783, 0.000000000000000000, -0.9999697198139514409 ) ) ;
#7670=EDGE_LOOP ( 'NONE', ( #24439, #34011, #46905, #16126 ) ) ;
#7671=CARTESIAN_POINT ( 'NONE',  ( -18.67619601524082285, 0.000000000000000000, 3.936400510096834893 ) ) ;
#7672=VECTOR ( 'NONE', #11616, 999.9999999999998863 ) ;
#7673=PLANE ( 'NONE',  #1862 ) ;
#7674=ORIENTED_EDGE ( 'NONE', *, *, #18968, .F. ) ;
#7675=CARTESIAN_POINT ( 'NONE',  ( 2.072287782118878319, 0.000000000000000000, -2.950529333540147015 ) ) ;
#7676=DIRECTION ( 'NONE',  ( 0.005961354470445682716, -0.6427876096865404731, -0.7660212471507180654 ) ) ;
#7678=AXIS2_PLACEMENT_3D ( 'NONE', #44896, #18196, #49142 ) ;
#7679=LINE ( 'NONE', #11379, #12888 ) ;
#7680=ORIENTED_EDGE ( 'NONE', *, *, #35511, .F. ) ;
#7681=AXIS2_PLACEMENT_3D ( 'NONE', #25854, #33795, #47415 ) ;
#7682=DIRECTION ( 'NONE',  ( 0.5364919789714477361, 0.6444004775717706579, 0.5449076811759711036 ) ) ;
#7683=CARTESIAN_POINT ( 'NONE',  ( 2.072287782118878319, 0.000000000000000000, -2.950529333540147015 ) ) ;
#7685=ADVANCED_FACE ( 'NONE', ( #27031 ), #48887, .F. ) ;
#7686=AXIS2_PLACEMENT_3D ( 'NONE', #49725, #45721, #28975 ) ;
#7687=DIRECTION ( 'NONE',  ( 0.007781995580012662783, 0.000000000000000000, -0.9999697198139514409 ) ) ;
#7688=DIRECTION ( 'NONE',  ( -0.005002170337468016433, -0.7660444431189770143, 0.6427681459581293666 ) ) ;
#7689=CARTESIAN_POINT ( 'NONE',  ( -14.94916102560700821, 0.000000000000000000, 2.688082935172642962 ) ) ;
#7690=CARTESIAN_POINT ( 'NONE',  ( -10.94028622754223967, 0.000000000000000000, 11.14038480894692995 ) ) ;
#7691=AXIS2_PLACEMENT_3D ( 'NONE', #33586, #38411, #33038 ) ;
#7692=ORIENTED_EDGE ( 'NONE', *, *, #43761, .T. ) ;
#7693=FACE_OUTER_BOUND ( 'NONE', #7437, .T. ) ;
#7694=DIRECTION ( 'NONE',  ( 0.6427681459581294776, -0.7660444431189769032, 0.005002170337467562802 ) ) ;
#7695=ORIENTED_EDGE ( 'NONE', *, *, #31514, .T. ) ;
#7696=VECTOR ( 'NONE', #4030, 999.9999999999998863 ) ;
#7697=FACE_OUTER_BOUND ( 'NONE', #11247, .T. ) ;
#7698=LINE ( 'NONE', #25030, #20918 ) ;
#7699=VECTOR ( 'NONE', #45450, 1000.000000000000227 ) ;
#7700=CARTESIAN_POINT ( 'NONE',  ( -26.13337879274045505, 0.000000000000000000, 6.833023547870798353 ) ) ;
#7701=FACE_OUTER_BOUND ( 'NONE', #21765, .T. ) ;
#7702=ADVANCED_FACE ( 'NONE', ( #23336 ), #2566, .F. ) ;
#7703=DIRECTION ( 'NONE',  ( 0.007781995580012663651, -3.146120232559066537E-19, -0.9999697198139514409 ) ) ;
#7704=ORIENTED_EDGE ( 'NONE', *, *, #18037, .F. ) ;
#7705=AXIS2_PLACEMENT_3D ( 'NONE', #41837, #2935, #20268 ) ;
#7706=VECTOR ( 'NONE', #37652, 999.9999999999998863 ) ;
#7707=VERTEX_POINT ( 'NONE', #15352 ) ;
#7708=CARTESIAN_POINT ( 'NONE',  ( -13.17065887352947762, -0.1191753592594197858, 12.04635770780929427 ) ) ;
#7709=FACE_OUTER_BOUND ( 'NONE', #40577, .T. ) ;
#7710=CARTESIAN_POINT ( 'NONE',  ( -18.81253076747439223, -3.594132820645663084, 4.074075289172853331 ) ) ;
#7711=EDGE_LOOP ( 'NONE', ( #22797, #30837, #889, #7566 ) ) ;
#7712=ADVANCED_FACE ( 'NONE', ( #19886 ), #7673, .F. ) ;
#7713=CARTESIAN_POINT ( 'NONE',  ( -17.74404816805336793, 0.000000000000000000, 3.574322630375089460 ) ) ;
#7714=ORIENTED_EDGE ( 'NONE', *, *, #11910, .T. ) ;
#7715=DIRECTION ( 'NONE',  ( 0.007781995580012663651, -3.146120232559066537E-19, -0.9999697198139514409 ) ) ;
#7716=EDGE_CURVE ( 'NONE', #46161, #28907, #50561, .T. ) ;
#7717=VECTOR ( 'NONE', #8978, 999.9999999999998863 ) ;
#7718=EDGE_LOOP ( 'NONE', ( #33667, #41199, #24264, #44118 ) ) ;
#7719=EDGE_LOOP ( 'NONE', ( #11119, #23968, #39269, #22805 ) ) ;
#7720=VERTEX_POINT ( 'NONE', #42324 ) ;
#7721=VECTOR ( 'NONE', #45055, 999.9999999999998863 ) ;
#7722=CARTESIAN_POINT ( 'NONE',  ( -18.11943520534269680, 3.038739411681508518, 8.906614157015832589 ) ) ;
#7723=FACE_OUTER_BOUND ( 'NONE', #44067, .T. ) ;
#7724=CARTESIAN_POINT ( 'NONE',  ( -16.06709938707323460, 0.000000000000000000, 13.13181314741652628 ) ) ;
#7725=EDGE_CURVE ( 'NONE', #26525, #35209, #11658, .T. ) ;
#7726=CARTESIAN_POINT ( 'NONE',  ( -18.96745105697236156, 0.7721120973665048792, 4.024899441011595691 ) ) ;
#7727=VECTOR ( 'NONE', #36524, 1000.000000000000000 ) ;
#7728=ORIENTED_EDGE ( 'NONE', *, *, #40811, .T. ) ;
#7730=ORIENTED_EDGE ( 'NONE', *, *, #51861, .T. ) ;
#7731=ADVANCED_FACE ( 'NONE', ( #32421 ), #2823, .F. ) ;
#7732=ORIENTED_EDGE ( 'NONE', *, *, #44454, .T. ) ;
#7733=VECTOR ( 'NONE', #23393, 1000.000000000000114 ) ;
#7734=DIRECTION ( 'NONE',  ( 0.000000000000000000, -1.000000000000000000, 0.000000000000000000 ) ) ;
#7736=CARTESIAN_POINT ( 'NONE',  ( -11.77243710274829525, -0.1191753592594197858, 11.50324088822667612 ) ) ;
#7737=EDGE_LOOP ( 'NONE', ( #38684, #20971, #32519, #32847 ) ) ;
#7738=VECTOR ( 'NONE', #40931, 1000.000000000000227 ) ;
#7739=CARTESIAN_POINT ( 'NONE',  ( 2.072287782118878319, 0.000000000000000000, -2.950529333540147015 ) ) ;
#7740=ORIENTED_EDGE ( 'NONE', *, *, #1289, .T. ) ;
#7741=CARTESIAN_POINT ( 'NONE',  ( -14.66887761629205222, 0.000000000000000000, 12.58869632783390990 ) ) ;
#7742=PLANE ( 'NONE',  #414 ) ;
#7743=AXIS2_PLACEMENT_3D ( 'NONE', #52469, #49869, #45085 ) ;
#7744=ORIENTED_EDGE ( 'NONE', *, *, #11158, .T. ) ;
#7745=VECTOR ( 'NONE', #21506, 1000.000000000000114 ) ;
#7746=DIRECTION ( 'NONE',  ( 0.000000000000000000, -1.000000000000000000, 0.000000000000000000 ) ) ;
#7747=ORIENTED_EDGE ( 'NONE', *, *, #10751, .T. ) ;
#7748=AXIS2_PLACEMENT_3D ( 'NONE', #50595, #7412, #34398 ) ;
#7749=DIRECTION ( 'NONE',  ( 0.005961354470445682716, -0.6427876096865404731, -0.7660212471507180654 ) ) ;
#7750=AXIS2_PLACEMENT_3D ( 'NONE', #20240, #50055, #46094 ) ;
#7751=LINE ( 'NONE', #21374, #48326 ) ;
#7752=ORIENTED_EDGE ( 'NONE', *, *, #40941, .F. ) ;
#7754=DIRECTION ( 'NONE',  ( -0.5449076811759708816, 0.6444004775717707689, 0.5364919789714475140 ) ) ;
#7755=LINE ( 'NONE', #51182, #45924 ) ;
#7756=CARTESIAN_POINT ( 'NONE',  ( -14.94760462649100496, 0.000000000000000000, 2.488088991209854051 ) ) ;
#7757=ORIENTED_EDGE ( 'NONE', *, *, #30304, .F. ) ;
#7758=EDGE_CURVE ( 'NONE', #47771, #2654, #29240, .T. ) ;
#7759=VERTEX_POINT ( 'NONE', #36957 ) ;
#7760=DIRECTION ( 'NONE',  ( 0.007781995580012663651, 0.000000000000000000, -0.9999697198139515519 ) ) ;
#7761=DIRECTION ( 'NONE',  ( 0.007781995580012663651, 0.000000000000000000, -0.9999697198139515519 ) ) ;
#7762=ADVANCED_FACE ( 'NONE', ( #24167 ), #15608, .T. ) ;
#7763=LINE ( 'NONE', #1616, #38578 ) ;
#7764=LINE ( 'NONE', #16265, #55727 ) ;
#7766=VECTOR ( 'NONE', #28159, 1000.000000000000227 ) ;
#7767=ADVANCED_FACE ( 'NONE', ( #6843 ), #37793, .F. ) ;
#7768=LINE ( 'NONE', #50639, #47624 ) ;
#7769=ORIENTED_EDGE ( 'NONE', *, *, #12847, .T. ) ;
#7770=AXIS2_PLACEMENT_3D ( 'NONE', #55488, #8359, #16594 ) ;
#7771=EDGE_CURVE ( 'NONE', #20993, #235, #46558, .T. ) ;
#7772=CARTESIAN_POINT ( 'NONE',  ( -12.81375377831746221, -1.975113310420657520, 4.900726287218082788 ) ) ;
#7773=CARTESIAN_POINT ( 'NONE',  ( -17.26532721389163072, 0.000000000000000000, 13.67648636611514590 ) ) ;
#7774=ORIENTED_EDGE ( 'NONE', *, *, #47717, .F. ) ;
#7775=FACE_OUTER_BOUND ( 'NONE', #46896, .T. ) ;
#7776=VECTOR ( 'NONE', #30622, 1000.000000000000114 ) ;
#7777=VERTEX_POINT ( 'NONE', #32950 ) ;
#7778=EDGE_CURVE ( 'NONE', #49949, #29930, #20147, .T. ) ;
#7779=EDGE_CURVE ( 'NONE', #10997, #2403, #53973, .T. ) ;
#7780=ADVANCED_FACE ( 'NONE', ( #28708 ), #11915, .F. ) ;
#7781=FACE_OUTER_BOUND ( 'NONE', #12588, .T. ) ;
#7782=DIRECTION ( 'NONE',  ( -0.5449076811759708816, 0.6444004775717707689, 0.5364919789714475140 ) ) ;
#7783=AXIS2_PLACEMENT_3D ( 'NONE', #21602, #25857, #51421 ) ;
#7784=CARTESIAN_POINT ( 'NONE',  ( -18.66354898467281132, 0.000000000000000000, 14.21960318569776582 ) ) ;
#7785=CARTESIAN_POINT ( 'NONE',  ( -18.60232905608458509, 0.000000000000000000, 6.352973834913863804 ) ) ;
#7787=ORIENTED_EDGE ( 'NONE', *, *, #9792, .T. ) ;
#7788=AXIS2_PLACEMENT_3D ( 'NONE', #42387, #7443, #37550 ) ;
#7789=AXIS2_PLACEMENT_3D ( 'NONE', #16302, #12036, #33371 ) ;
#7790=ORIENTED_EDGE ( 'NONE', *, *, #54811, .T. ) ;
#7791=DIRECTION ( 'NONE',  ( -0.005961354470445682716, -0.6427876096865404731, 0.7660212471507180654 ) ) ;
#7792=DIRECTION ( 'NONE',  ( -0.6427681459581293666, -0.7660444431189770143, -0.005002170337467561935 ) ) ;
#7793=PLANE ( 'NONE',  #35075 ) ;
#7795=CARTESIAN_POINT ( 'NONE',  ( -27.06552663992790997, 0.000000000000000000, 7.195101427592543786 ) ) ;
#7796=AXIS2_PLACEMENT_3D ( 'NONE', #39683, #31137, #39935 ) ;
#7797=LINE ( 'NONE', #25122, #23775 ) ;
#7798=ADVANCED_FACE ( 'NONE', ( #7124 ), #15095, .F. ) ;
#7799=LINE ( 'NONE', #38150, #38506 ) ;
#7800=VECTOR ( 'NONE', #29068, 1000.000000000000000 ) ;
#7801=ORIENTED_EDGE ( 'NONE', *, *, #38870, .T. ) ;
#7802=DIRECTION ( 'NONE',  ( 0.007781995580012662783, 0.000000000000000000, -0.9999697198139514409 ) ) ;
#7803=AXIS2_PLACEMENT_3D ( 'NONE', #28525, #15211, #36789 ) ;
#7804=EDGE_CURVE ( 'NONE', #37945, #12623, #3118, .T. ) ;
#7805=CARTESIAN_POINT ( 'NONE',  ( 2.072287782118878319, 0.000000000000000000, -2.950529333540147015 ) ) ;
#7806=VECTOR ( 'NONE', #38858, 1000.000000000000227 ) ;
#7807=PLANE ( 'NONE',  #5191 ) ;
#7808=ORIENTED_EDGE ( 'NONE', *, *, #10634, .T. ) ;
#7809=ADVANCED_FACE ( 'NONE', ( #6550 ), #2286, .F. ) ;
#7810=DIRECTION ( 'NONE',  ( 0.5449076811759707706, 0.6444004775717708799, -0.5364919789714476250 ) ) ;
#7811=PLANE ( 'NONE',  #45844 ) ;
#7812=CARTESIAN_POINT ( 'NONE',  ( -17.39979014900826471, 0.000000000000000000, 5.254336061328594987 ) ) ;
#7813=ORIENTED_EDGE ( 'NONE', *, *, #2738, .T. ) ;
#7814=EDGE_CURVE ( 'NONE', #2673, #43270, #43171, .T. ) ;
#7815=LINE ( 'NONE', #8934, #32002 ) ;
#7816=ORIENTED_EDGE ( 'NONE', *, *, #4425, .T. ) ;
#7817=VECTOR ( 'NONE', #36222, 1000.000000000000227 ) ;
#7818=ORIENTED_EDGE ( 'NONE', *, *, #8788, .T. ) ;
#7819=VERTEX_POINT ( 'NONE', #21839 ) ;
#7820=VERTEX_POINT ( 'NONE', #30090 ) ;
#7821=DIRECTION ( 'NONE',  ( 0.005961354470445682716, -0.6427876096865404731, -0.7660212471507180654 ) ) ;
#7822=VECTOR ( 'NONE', #38724, 999.9999999999998863 ) ;
#7823=ORIENTED_EDGE ( 'NONE', *, *, #35611, .T. ) ;
#7824=FACE_OUTER_BOUND ( 'NONE', #38120, .T. ) ;
#7826=CARTESIAN_POINT ( 'NONE',  ( -19.70461351680143736, -0.03744543421978414194, 6.914475087243958207 ) ) ;
#7827=ORIENTED_EDGE ( 'NONE', *, *, #17886, .F. ) ;
#7828=VECTOR ( 'NONE', #20943, 1000.000000000000227 ) ;
#7829=VERTEX_POINT ( 'NONE', #51935 ) ;
#7830=VECTOR ( 'NONE', #8833, 1000.000000000000227 ) ;
#7831=AXIS2_PLACEMENT_3D ( 'NONE', #23401, #44403, #31061 ) ;
#7833=DIRECTION ( 'NONE',  ( -0.3620778797217455991, 0.000000000000000000, -0.9321478471874540261 ) ) ;
#7834=CARTESIAN_POINT ( 'NONE',  ( -13.73672976910459909, 0.000000000000000000, 12.22661844811216270 ) ) ;
#7835=DIRECTION ( 'NONE',  ( -0.005002170337468016433, -0.7660444431189770143, 0.6427681459581293666 ) ) ;
#7836=PLANE ( 'NONE',  #45558 ) ;
#7837=ORIENTED_EDGE ( 'NONE', *, *, #18861, .F. ) ;
#7838=AXIS2_PLACEMENT_3D ( 'NONE', #54130, #53553, #14118 ) ;
#7839=ORIENTED_EDGE ( 'NONE', *, *, #35281, .T. ) ;
#7840=AXIS2_PLACEMENT_3D ( 'NONE', #28193, #10641, #45250 ) ;
#7842=CARTESIAN_POINT ( 'NONE',  ( -17.19823980592947876, 0.000000000000000000, 5.055898516481810212 ) ) ;
#7843=AXIS2_PLACEMENT_3D ( 'NONE', #4022, #2869, #37533 ) ;
#7844=LINE ( 'NONE', #33649, #1590 ) ;
#7845=VECTOR ( 'NONE', #18233, 999.9999999999998863 ) ;
#7846=LINE ( 'NONE', #17182, #55856 ) ;
#7847=PLANE ( 'NONE',  #25879 ) ;
#7848=DIRECTION ( 'NONE',  ( -0.005961354470445682716, -0.6427876096865404731, 0.7660212471507180654 ) ) ;
#7849=ORIENTED_EDGE ( 'NONE', *, *, #54878, .T. ) ;
#7850=LINE ( 'NONE', #25706, #19318 ) ;
#7851=DIRECTION ( 'NONE',  ( 0.007781995580012663651, 0.000000000000000000, -0.9999697198139515519 ) ) ;
#7852=ORIENTED_EDGE ( 'NONE', *, *, #43049, .T. ) ;
#7853=EDGE_CURVE ( 'NONE', #36877, #54764, #25283, .T. ) ;
#7854=EDGE_CURVE ( 'NONE', #29009, #13585, #42587, .T. ) ;
#7855=CARTESIAN_POINT ( 'NONE',  ( -18.67697421479882181, -0.1191753592594197858, 4.036397482078229793 ) ) ;
#7856=DIRECTION ( 'NONE',  ( -0.6427681459581293666, -0.7660444431189770143, -0.005002170337467561935 ) ) ;
#7857=CARTESIAN_POINT ( 'NONE',  ( -18.39746900504187010, 0.000000000000000000, 14.03700784672088808 ) ) ;
#7858=LINE ( 'NONE', #3572, #4187 ) ;
#7859=EDGE_CURVE ( 'NONE', #33225, #14263, #34089, .T. ) ;
#7860=DIRECTION ( 'NONE',  ( -0.9999697198139514409, -0.000000000000000000, -0.007781995580013368816 ) ) ;
#7861=VECTOR ( 'NONE', #24821, 1000.000000000000227 ) ;
#7862=ORIENTED_EDGE ( 'NONE', *, *, #43668, .F. ) ;
#7863=ORIENTED_EDGE ( 'NONE', *, *, #6975, .T. ) ;
#7864=DIRECTION ( 'NONE',  ( 0.5364919789714477361, 0.6444004775717706579, 0.5449076811759711036 ) ) ;
#7865=DIRECTION ( 'NONE',  ( 0.007781995580012663651, -3.146120232559066537E-19, -0.9999697198139514409 ) ) ;
#7866=CARTESIAN_POINT ( 'NONE',  ( -24.27063949748155380, 0.000000000000000000, 6.308861732390097288 ) ) ;
#7867=AXIS2_PLACEMENT_3D ( 'NONE', #2523, #40610, #15042 ) ;
#7868=LINE ( 'NONE', #46748, #14672 ) ;
#7869=AXIS2_PLACEMENT_3D ( 'NONE', #48199, #18115, #9309 ) ;
#7870=CARTESIAN_POINT ( 'NONE',  ( -12.35938774090218217, -0.3560938001956556742, 1.670765785740375931 ) ) ;
#7871=FACE_OUTER_BOUND ( 'NONE', #36528, .T. ) ;
#7872=FACE_OUTER_BOUND ( 'NONE', #5626, .T. ) ;
#7873=EDGE_CURVE ( 'NONE', #5052, #49012, #38319, .T. ) ;
#7874=CARTESIAN_POINT ( 'NONE',  ( -3.775690919409564028, -5.709557508479220722, 4.684980151765822498 ) ) ;
#7875=VECTOR ( 'NONE', #41069, 1000.000000000000227 ) ;
#7876=FACE_OUTER_BOUND ( 'NONE', #20902, .T. ) ;
#7877=EDGE_CURVE ( 'NONE', #42368, #35767, #43435, .T. ) ;
#7878=DIRECTION ( 'NONE',  ( 0.9999697198139515519, 0.000000000000000000, 0.007781995580013368816 ) ) ;
#7879=ORIENTED_EDGE ( 'NONE', *, *, #20523, .T. ) ;
#7880=CARTESIAN_POINT ( 'NONE',  ( -17.12040860686058608, -2.137015261443160341, 3.463287256266506908 ) ) ;
#7881=ORIENTED_EDGE ( 'NONE', *, *, #42500, .F. ) ;
#7882=EDGE_CURVE ( 'NONE', #31801, #3456, #17294, .T. ) ;
#7883=VECTOR ( 'NONE', #12710, 1000.000000000000227 ) ;
#7884=ORIENTED_EDGE ( 'NONE', *, *, #29190, .F. ) ;
#7885=EDGE_CURVE ( 'NONE', #11310, #37777, #52242, .T. ) ;
#7886=AXIS2_PLACEMENT_3D ( 'NONE', #53879, #14997, #2486 ) ;
#7887=EDGE_LOOP ( 'NONE', ( #50820, #53085, #15001, #46614 ) ) ;
#7888=VECTOR ( 'NONE', #29579, 1000.000000000000227 ) ;
#7889=VERTEX_POINT ( 'NONE', #34620 ) ;
#7890=ORIENTED_EDGE ( 'NONE', *, *, #6216, .F. ) ;
#7891=ORIENTED_EDGE ( 'NONE', *, *, #55975, .F. ) ;
#7892=CARTESIAN_POINT ( 'NONE',  ( -12.13851405436063047, 0.000000000000000000, 11.68505802764555135 ) ) ;
#7893=CARTESIAN_POINT ( 'NONE',  ( -20.41355881641904801, 1.905425754524007198, 7.937768888670418299 ) ) ;
#7894=EDGE_CURVE ( 'NONE', #52808, #30962, #47403, .T. ) ;
#7895=PLANE ( 'NONE',  #37559 ) ;
#7896=ORIENTED_EDGE ( 'NONE', *, *, #406, .F. ) ;
#7897=CARTESIAN_POINT ( 'NONE',  ( -10.00813838035478298, 0.000000000000000000, 10.77830692922518452 ) ) ;
#7898=ORIENTED_EDGE ( 'NONE', *, *, #39788, .F. ) ;
#7899=CARTESIAN_POINT ( 'NONE',  ( -13.23530239847019097, 0.000000000000000000, 7.502737486787267152 ) ) ;
#7900=ORIENTED_EDGE ( 'NONE', *, *, #27041, .F. ) ;
#7901=AXIS2_PLACEMENT_3D ( 'NONE', #41492, #41740, #23343 ) ;
#7903=DIRECTION ( 'NONE',  ( -0.9999697198139514409, -0.000000000000000000, -0.007781995580013368816 ) ) ;
#7904=VERTEX_POINT ( 'NONE', #47704 ) ;
#7905=FACE_OUTER_BOUND ( 'NONE', #22206, .T. ) ;
#7906=ORIENTED_EDGE ( 'NONE', *, *, #13612, .T. ) ;
#7907=CARTESIAN_POINT ( 'NONE',  ( -26.13493519185646008, 0.000000000000000000, 7.033017491833586377 ) ) ;
#7908=AXIS2_PLACEMENT_3D ( 'NONE', #22602, #26564, #43886 ) ;
#7909=CARTESIAN_POINT ( 'NONE',  ( -18.25349690304924266, -3.432230869623160263, 9.405085406872181863 ) ) ;
#7910=DIRECTION ( 'NONE',  ( 0.5364919789714477361, 0.6444004775717706579, 0.5449076811759711036 ) ) ;
#7911=AXIS2_PLACEMENT_3D ( 'NONE', #45275, #32507, #31668 ) ;
#7912=CARTESIAN_POINT ( 'NONE',  ( -16.27184006575258834, 0.000000000000000000, 5.432440043275593489 ) ) ;
#7913=LINE ( 'NONE', #51610, #232 ) ;
#7914=PLANE ( 'NONE',  #26704 ) ;
#7916=LINE ( 'NONE', #21534, #51304 ) ;
#7917=ORIENTED_EDGE ( 'NONE', *, *, #1095, .F. ) ;
#7918=CARTESIAN_POINT ( 'NONE',  ( -13.07066190154808361, 0.000000000000000000, 12.04713590736729678 ) ) ;
#7919=EDGE_LOOP ( 'NONE', ( #53073, #48892, #48367, #18125 ) ) ;
#7920=EDGE_CURVE ( 'NONE', #46912, #17870, #3680, .T. ) ;
#7921=VECTOR ( 'NONE', #12992, 1000.000000000000227 ) ;
#7922=DIRECTION ( 'NONE',  ( 0.6427681459581294776, -0.7660444431189769032, 0.005002170337467562802 ) ) ;
#7923=DIRECTION ( 'NONE',  ( 0.9999697198139515519, 0.000000000000000000, 0.007781995580013368816 ) ) ;
#7924=LINE ( 'NONE', #25236, #29597 ) ;
#7925=FACE_OUTER_BOUND ( 'NONE', #49773, .T. ) ;
#7926=CARTESIAN_POINT ( 'NONE',  ( 4.452747148193316740, -1.000000000000000000, 0.4159841754879232689 ) ) ;
#7927=EDGE_CURVE ( 'NONE', #14368, #23927, #17590, .T. ) ;
#7928=EDGE_CURVE ( 'NONE', #33489, #1369, #30673, .T. ) ;
#7929=DIRECTION ( 'NONE',  ( 0.000000000000000000, -0.000000000000000000, -1.000000000000000000 ) ) ;
#7930=ORIENTED_EDGE ( 'NONE', *, *, #2189, .T. ) ;
#7931=LINE ( 'NONE', #37741, #33782 ) ;
#7932=CARTESIAN_POINT ( 'NONE',  ( -13.01938178786498490, 0.000000000000000000, 5.457751425651659716 ) ) ;
#7933=CARTESIAN_POINT ( 'NONE',  ( -18.19747506107908563, 0.000000000000000000, 14.03856424583689311 ) ) ;
#7934=DIRECTION ( 'NONE',  ( 0.5364919789714477361, 0.6444004775717706579, 0.5449076811759711036 ) ) ;
#7935=CARTESIAN_POINT ( 'NONE',  ( -0.5433539342177339249, -4.971938947471305603, 3.429430696091245068 ) ) ;
#7936=PLANE ( 'NONE',  #32112 ) ;
#7937=CARTESIAN_POINT ( 'NONE',  ( -9.739739374040562225, 0.000000000000000000, 1.989959719412870864 ) ) ;
#7938=CARTESIAN_POINT ( 'NONE',  ( -19.60834386242827776, 0.000000000000000000, 4.298478389818581213 ) ) ;
#7939=EDGE_LOOP ( 'NONE', ( #50306, #3806, #51586, #10282 ) ) ;
#7940=FACE_OUTER_BOUND ( 'NONE', #4886, .T. ) ;
#7941=CARTESIAN_POINT ( 'NONE',  ( -19.48672417669920875, -0.5179957512181557755, 4.434099782880741358 ) ) ;
#7942=ORIENTED_EDGE ( 'NONE', *, *, #22890, .T. ) ;
#7943=ORIENTED_EDGE ( 'NONE', *, *, #6636, .F. ) ;
#7944=LINE ( 'NONE', #8203, #41887 ) ;
#7945=ORIENTED_EDGE ( 'NONE', *, *, #22829, .F. ) ;
#7946=CARTESIAN_POINT ( 'NONE',  ( -9.411683945191542833, -0.1191753592594181482, 6.693826601992417302 ) ) ;
#7947=EDGE_CURVE ( 'NONE', #44961, #38597, #47126, .T. ) ;
#7948=VECTOR ( 'NONE', #34517, 1000.000000000000227 ) ;
#7949=ORIENTED_EDGE ( 'NONE', *, *, #29580, .T. ) ;
#7950=EDGE_LOOP ( 'NONE', ( #7237, #39812, #42487, #19720 ) ) ;
#7951=EDGE_LOOP ( 'NONE', ( #21293, #37944, #11501, #38896 ) ) ;
#7952=EDGE_CURVE ( 'NONE', #12432, #9106, #47971, .T. ) ;
#7953=FACE_OUTER_BOUND ( 'NONE', #6336, .T. ) ;
#7954=CARTESIAN_POINT ( 'NONE',  ( -20.08254794625849371, -0.1191753592594172878, 4.582370052862001941 ) ) ;
#7955=EDGE_CURVE ( 'NONE', #17655, #9986, #26126, .T. ) ;
#7956=CARTESIAN_POINT ( 'NONE',  ( -26.13493519185646008, 0.000000000000000000, 7.033017491833586377 ) ) ;
#7957=VECTOR ( 'NONE', #35349, 999.9999999999998863 ) ;
#7958=ORIENTED_EDGE ( 'NONE', *, *, #53238, .F. ) ;
#7959=EDGE_CURVE ( 'NONE', #33216, #21642, #34360, .T. ) ;
#7960=ORIENTED_EDGE ( 'NONE', *, *, #41386, .F. ) ;
#7961=DIRECTION ( 'NONE',  ( 0.000000000000000000, -1.000000000000000000, 0.000000000000000000 ) ) ;
#7962=PLANE ( 'NONE',  #30916 ) ;
#7963=ORIENTED_EDGE ( 'NONE', *, *, #21216, .F. ) ;
#7965=FACE_OUTER_BOUND ( 'NONE', #55178, .T. ) ;
#7966=ORIENTED_EDGE ( 'NONE', *, *, #41593, .T. ) ;
#7967=DIRECTION ( 'NONE',  ( 0.5449076811759707706, 0.6444004775717708799, -0.5364919789714476250 ) ) ;
#7968=CARTESIAN_POINT ( 'NONE',  ( -17.93139508144814442, 0.000000000000000000, 13.85596890686001537 ) ) ;
#7969=EDGE_LOOP ( 'NONE', ( #31139, #28607, #27451, #22838 ) ) ;
#7970=CARTESIAN_POINT ( 'NONE',  ( -12.63184290468442228, -0.6798977022406560433, 1.766265584194925520 ) ) ;
#7971=ADVANCED_FACE ( 'NONE', ( #38052 ), #3967, .F. ) ;
#7972=CARTESIAN_POINT ( 'NONE',  ( -18.39746900504187010, 0.000000000000000000, 14.03700784672088808 ) ) ;
#7973=EDGE_LOOP ( 'NONE', ( #22109, #11223, #27791, #55619 ) ) ;
#7974=DIRECTION ( 'NONE',  ( 0.7660212471507180654, -0.6427876096865404731, 0.005961354470445141482 ) ) ;
#7975=DIRECTION ( 'NONE',  ( 0.7660212471507180654, -0.6427876096865404731, 0.005961354470445141482 ) ) ;
#7976=DIRECTION ( 'NONE',  ( 0.5449076811759707706, 0.6444004775717708799, -0.5364919789714476250 ) ) ;
#7977=CARTESIAN_POINT ( 'NONE',  ( -15.40103151951671734, 0.000000000000000000, 12.95233060667165681 ) ) ;
#7978=EDGE_CURVE ( 'NONE', #27927, #31613, #16455, .T. ) ;
#7979=ORIENTED_EDGE ( 'NONE', *, *, #50759, .F. ) ;
#7980=EDGE_CURVE ( 'NONE', #29025, #53596, #51103, .T. ) ;
#7981=PLANE ( 'NONE',  #41897 ) ;
#7982=CARTESIAN_POINT ( 'NONE',  ( -13.07066190154808361, 0.000000000000000000, 12.04713590736729678 ) ) ;
#7983=DIRECTION ( 'NONE',  ( 0.9999697198139515519, 0.000000000000000000, 0.007781995580013368816 ) ) ;
#7984=DIRECTION ( 'NONE',  ( 0.7660212471507180654, -0.6427876096865404731, 0.005961354470445141482 ) ) ;
#7985=CARTESIAN_POINT ( 'NONE',  ( -16.84300024114363126, -0.1191753592594194527, 6.266662310446504236 ) ) ;
#7986=EDGE_CURVE ( 'NONE', #53467, #40095, #39745, .T. ) ;
#7987=DIRECTION ( 'NONE',  ( -0.5364919789714478471, 0.6444004775717705469, -0.5449076811759709926 ) ) ;
#7988=PLANE ( 'NONE',  #31281 ) ;
#7989=ORIENTED_EDGE ( 'NONE', *, *, #36421, .F. ) ;
#7990=DIRECTION ( 'NONE',  ( 0.000000000000000000, -1.000000000000000000, 0.000000000000000000 ) ) ;
#7991=VERTEX_POINT ( 'NONE', #18728 ) ;
#7992=DIRECTION ( 'NONE',  ( -0.005002170337468016433, -0.7660444431189770143, 0.6427681459581293666 ) ) ;
#7993=PLANE ( 'NONE',  #48123 ) ;
#7994=VECTOR ( 'NONE', #51117, 999.9999999999998863 ) ;
#7995=PLANE ( 'NONE',  #21316 ) ;
#7996=PLANE ( 'NONE',  #27833 ) ;
#7997=DIRECTION ( 'NONE',  ( -0.005961354470445682716, -0.6427876096865404731, 0.7660212471507180654 ) ) ;
#7998=EDGE_CURVE ( 'NONE', #1435, #3706, #36309, .T. ) ;
#7999=ORIENTED_EDGE ( 'NONE', *, *, #18609, .T. ) ;
#8000=EDGE_LOOP ( 'NONE', ( #33377, #85, #13666, #22740 ) ) ;
#8001=DIRECTION ( 'NONE',  ( 0.007781995580012663651, 0.000000000000000000, -0.9999697198139515519 ) ) ;
#8002=CARTESIAN_POINT ( 'NONE',  ( -22.40556560354864146, -0.1191753592594197858, 5.484709000965211523 ) ) ;
#8003=ORIENTED_EDGE ( 'NONE', *, *, #40168, .F. ) ;
#8004=CARTESIAN_POINT ( 'NONE',  ( -16.95239757319887985, 0.000000000000000000, 7.473810192643190575 ) ) ;
#8005=VERTEX_POINT ( 'NONE', #35212 ) ;
#8006=PLANE ( 'NONE',  #43096 ) ;
#8007=ORIENTED_EDGE ( 'NONE', *, *, #20818, .F. ) ;
#8008=DIRECTION ( 'NONE',  ( 0.000000000000000000, -0.000000000000000000, -1.000000000000000000 ) ) ;
#8009=ORIENTED_EDGE ( 'NONE', *, *, #29334, .F. ) ;
#8010=ORIENTED_EDGE ( 'NONE', *, *, #22681, .T. ) ;
#8011=VERTEX_POINT ( 'NONE', #559 ) ;
#8012=LINE ( 'NONE', #16803, #3018 ) ;
#8013=PLANE ( 'NONE',  #9626 ) ;
#8014=DIRECTION ( 'NONE',  ( -0.5364919789714478471, 0.6444004775717705469, -0.5449076811759709926 ) ) ;
#8015=PLANE ( 'NONE',  #49217 ) ;
#8016=EDGE_CURVE ( 'NONE', #46316, #46703, #52774, .T. ) ;
#8017=EDGE_LOOP ( 'NONE', ( #55679, #17682, #19596, #20289 ) ) ;
#8018=EDGE_LOOP ( 'NONE', ( #21124, #51584, #49200, #6106 ) ) ;
#8019=VERTEX_POINT ( 'NONE', #13879 ) ;
#8020=DIRECTION ( 'NONE',  ( 0.7660212471507180654, -0.6427876096865404731, 0.005961354470445141482 ) ) ;
#8021=DIRECTION ( 'NONE',  ( -0.9999697198139514409, -0.000000000000000000, -0.007781995580013368816 ) ) ;
#8022=ORIENTED_EDGE ( 'NONE', *, *, #41391, .F. ) ;
#8023=DIRECTION ( 'NONE',  ( 0.007781995580012662783, 0.000000000000000000, -0.9999697198139514409 ) ) ;
#8024=VERTEX_POINT ( 'NONE', #5108 ) ;
#8025=FACE_OUTER_BOUND ( 'NONE', #46393, .T. ) ;
#8026=LINE ( 'NONE', #25072, #25809 ) ;
#8027=EDGE_CURVE ( 'NONE', #44511, #5651, #31206, .T. ) ;
#8028=AXIS2_PLACEMENT_3D ( 'NONE', #53918, #1683, #32370 ) ;
#8029=ORIENTED_EDGE ( 'NONE', *, *, #15266, .F. ) ;
#8030=FACE_OUTER_BOUND ( 'NONE', #33657, .T. ) ;
#8031=ORIENTED_EDGE ( 'NONE', *, *, #34221, .F. ) ;
#8032=EDGE_CURVE ( 'NONE', #22613, #21479, #35759, .T. ) ;
#8033=ADVANCED_FACE ( 'NONE', ( #22437 ), #5643, .F. ) ;
#8034=DIRECTION ( 'NONE',  ( -0.5364919789714478471, 0.6444004775717705469, -0.5449076811759709926 ) ) ;
#8035=DIRECTION ( 'NONE',  ( 0.9999697198139515519, 0.000000000000000000, 0.007781995580013368816 ) ) ;
#8036=ORIENTED_EDGE ( 'NONE', *, *, #41778, .F. ) ;
#8037=CARTESIAN_POINT ( 'NONE',  ( -15.13495153988577968, 0.000000000000000000, 12.76973526769478084 ) ) ;
#8038=DIRECTION ( 'NONE',  ( 0.007781995580012662783, 0.000000000000000000, -0.9999697198139514409 ) ) ;
#8039=LINE ( 'NONE', #25350, #9662 ) ;
#8040=CARTESIAN_POINT ( 'NONE',  ( -17.26532721389163072, 0.000000000000000000, 13.67648636611514590 ) ) ;
#8041=ORIENTED_EDGE ( 'NONE', *, *, #44751, .F. ) ;
#8042=ORIENTED_EDGE ( 'NONE', *, *, #45271, .F. ) ;
#8043=EDGE_CURVE ( 'NONE', #44617, #54500, #17892, .T. ) ;
#8044=FACE_OUTER_BOUND ( 'NONE', #21128, .T. ) ;
#8045=DIRECTION ( 'NONE',  ( 0.5449076811759707706, 0.6444004775717708799, -0.5364919789714476250 ) ) ;
#8046=CARTESIAN_POINT ( 'NONE',  ( -13.69550884268998914, 0.000000000000000000, 6.929817927798703536 ) ) ;
#8047=DIRECTION ( 'NONE',  ( 0.005961354470445682716, -0.6427876096865404731, -0.7660212471507180654 ) ) ;
#8048=EDGE_CURVE ( 'NONE', #45704, #20591, #14726, .T. ) ;
#8049=LINE ( 'NONE', #51490, #28829 ) ;
#8050=FACE_OUTER_BOUND ( 'NONE', #53557, .T. ) ;
#8051=ORIENTED_EDGE ( 'NONE', *, *, #1487, .F. ) ;
#8052=LINE ( 'NONE', #21083, #40700 ) ;
#8053=FACE_OUTER_BOUND ( 'NONE', #19809, .T. ) ;
#8054=DIRECTION ( 'NONE',  ( -0.6427681459581293666, -0.7660444431189770143, -0.005002170337467561935 ) ) ;
#8055=ORIENTED_EDGE ( 'NONE', *, *, #4326, .T. ) ;
#8056=DIRECTION ( 'NONE',  ( -0.005961354470445682716, -0.6427876096865404731, 0.7660212471507180654 ) ) ;
#8057=VERTEX_POINT ( 'NONE', #49371 ) ;
#8058=EDGE_CURVE ( 'NONE', #6678, #3929, #48532, .T. ) ;
#8059=CARTESIAN_POINT ( 'NONE',  ( -16.53317331066696383, 0.000000000000000000, 13.31285208727739899 ) ) ;
#8060=CARTESIAN_POINT ( 'NONE',  ( -19.61932540816901849, -0.1191753592594174127, 4.767728026807386499 ) ) ;
#8061=DIRECTION ( 'NONE',  ( 0.9999697198139515519, 0.000000000000000000, 0.007781995580013368816 ) ) ;
#8062=CARTESIAN_POINT ( 'NONE',  ( -22.62703048288702234, 4.495856970884011261, 13.04889539694818623 ) ) ;
#8064=EDGE_CURVE ( 'NONE', #29959, #29873, #1664, .T. ) ;
#8065=ORIENTED_EDGE ( 'NONE', *, *, #10157, .F. ) ;
#8066=ORIENTED_EDGE ( 'NONE', *, *, #29158, .T. ) ;
#8067=DIRECTION ( 'NONE',  ( 0.5364919789714477361, 0.6444004775717706579, 0.5449076811759711036 ) ) ;
#8068=CARTESIAN_POINT ( 'NONE',  ( -20.54049170961573267, 0.000000000000000000, 4.660556269540326646 ) ) ;
#8069=LINE ( 'NONE', #25647, #27811 ) ;
#8070=LINE ( 'NONE', #3782, #13226 ) ;
#8072=DIRECTION ( 'NONE',  ( 0.5364919789714477361, 0.6444004775717706579, 0.5449076811759711036 ) ) ;
#8074=ORIENTED_EDGE ( 'NONE', *, *, #14777, .T. ) ;
#8075=PLANE ( 'NONE',  #54609 ) ;
#8076=DIRECTION ( 'NONE',  ( 0.5364919789714477361, 0.6444004775717706579, 0.5449076811759711036 ) ) ;
#8077=CARTESIAN_POINT ( 'NONE',  ( -12.33850799832341849, 0.000000000000000000, 11.68350162852954632 ) ) ;
#8078=ORIENTED_EDGE ( 'NONE', *, *, #42633, .T. ) ;
#8079=CARTESIAN_POINT ( 'NONE',  ( -10.74029228357944987, 0.000000000000000000, 11.14194120806293320 ) ) ;
#8080=CARTESIAN_POINT ( 'NONE',  ( -16.81345671998191449, 0.000000000000000000, 3.412238694616132495 ) ) ;
#8081=FACE_OUTER_BOUND ( 'NONE', #45703, .T. ) ;
#8082=ORIENTED_EDGE ( 'NONE', *, *, #36826, .F. ) ;
#8083=CARTESIAN_POINT ( 'NONE',  ( -19.73159679372954045, 0.000000000000000000, 6.344185612261842522 ) ) ;
#8084=EDGE_CURVE ( 'NONE', #23572, #10480, #18141, .T. ) ;
#8085=ADVANCED_FACE ( 'NONE', ( #26968 ), #4805, .F. ) ;
#8086=VERTEX_POINT ( 'NONE', #44282 ) ;
#8087=EDGE_LOOP ( 'NONE', ( #44632, #22603, #3903, #12119 ) ) ;
#8088=ORIENTED_EDGE ( 'NONE', *, *, #26195, .T. ) ;
#8089=VERTEX_POINT ( 'NONE', #22130 ) ;
#8090=DIRECTION ( 'NONE',  ( 0.007781995580012663651, -3.146120232559066537E-19, -0.9999697198139514409 ) ) ;
#8091=VERTEX_POINT ( 'NONE', #1086 ) ;
#8092=EDGE_CURVE ( 'NONE', #47173, #10102, #13603, .T. ) ;
#8093=CARTESIAN_POINT ( 'NONE',  ( -12.74324262096555849, 0.000000000000000000, 3.982572125272607622 ) ) ;
#8094=EDGE_CURVE ( 'NONE', #7759, #27005, #18422, .T. ) ;
#8095=EDGE_CURVE ( 'NONE', #14361, #33224, #31515, .T. ) ;
#8096=ORIENTED_EDGE ( 'NONE', *, *, #7019, .F. ) ;
#8097=FACE_OUTER_BOUND ( 'NONE', #53344, .T. ) ;
#8098=ORIENTED_EDGE ( 'NONE', *, *, #55319, .F. ) ;
#8099=ORIENTED_EDGE ( 'NONE', *, *, #7075, .F. ) ;
#8100=EDGE_CURVE ( 'NONE', #44385, #26435, #9924, .T. ) ;
#8101=DIRECTION ( 'NONE',  ( 0.007781995580012663651, -3.146120232559066537E-19, -0.9999697198139514409 ) ) ;
#8102=LINE ( 'NONE', #25152, #36811 ) ;
#8103=CARTESIAN_POINT ( 'NONE',  ( -28.93137873341882127, 0.000000000000000000, 8.119251130998824451 ) ) ;
#8104=CARTESIAN_POINT ( 'NONE',  ( -11.45287710155235850, 1.257817950434005683, 1.090487161058584231 ) ) ;
#8105=LINE ( 'NONE', #55799, #41940 ) ;
#8106=ORIENTED_EDGE ( 'NONE', *, *, #55195, .F. ) ;
#8108=ORIENTED_EDGE ( 'NONE', *, *, #10194, .T. ) ;
#8109=EDGE_CURVE ( 'NONE', #22478, #32939, #31776, .T. ) ;
#8110=PLANE ( 'NONE',  #6819 ) ;
#8111=DIRECTION ( 'NONE',  ( 0.007781995580012662783, 0.000000000000000000, -0.9999697198139514409 ) ) ;
#8112=ADVANCED_FACE ( 'NONE', ( #54443 ), #33179, .F. ) ;
#8113=LINE ( 'NONE', #21730, #48738 ) ;
#8115=ADVANCED_FACE ( 'NONE', ( #27814 ), #49907, .F. ) ;
#8116=PLANE ( 'NONE',  #26757 ) ;
#8117=DIRECTION ( 'NONE',  ( 0.007781995580012663651, -3.146120232559066537E-19, -0.9999697198139514409 ) ) ;
#8118=ORIENTED_EDGE ( 'NONE', *, *, #54176, .F. ) ;
#8119=FACE_OUTER_BOUND ( 'NONE', #29179, .T. ) ;
#8120=DIRECTION ( 'NONE',  ( 0.5449076811759707706, 0.6444004775717708799, -0.5364919789714476250 ) ) ;
#8121=VERTEX_POINT ( 'NONE', #54729 ) ;
#8122=EDGE_CURVE ( 'NONE', #41133, #50088, #28333, .T. ) ;
#8123=CARTESIAN_POINT ( 'NONE',  ( -16.48776067635779441, 0.000000000000000000, 7.477426104411200924 ) ) ;
#8124=CARTESIAN_POINT ( 'NONE',  ( -10.84028925556084388, -0.1191753592594197858, 11.14116300850493246 ) ) ;
#8125=PLANE ( 'NONE',  #50832 ) ;
#8126=CARTESIAN_POINT ( 'NONE',  ( -15.40103151951671734, 0.000000000000000000, 12.95233060667165681 ) ) ;
#8127=DIRECTION ( 'NONE',  ( 0.7660212471507180654, -0.6427876096865404731, 0.005961354470445141482 ) ) ;
#8128=ORIENTED_EDGE ( 'NONE', *, *, #23016, .T. ) ;
#8130=CARTESIAN_POINT ( 'NONE',  ( -15.03495456790438389, -0.1191753592594197858, 12.77051346725278158 ) ) ;
#8131=DIRECTION ( 'NONE',  ( 0.005961354470445682716, -0.6427876096865404731, -0.7660212471507180654 ) ) ;
#8132=LINE ( 'NONE', #15504, #7051 ) ;
#8134=DIRECTION ( 'NONE',  ( 0.7660212471507180654, -0.6427876096865404731, 0.005961354470445141482 ) ) ;
#8136=CARTESIAN_POINT ( 'NONE',  ( -17.26532721389163072, 0.000000000000000000, 13.67648636611514590 ) ) ;
#8137=FACE_OUTER_BOUND ( 'NONE', #22260, .T. ) ;
#8139=PLANE ( 'NONE',  #37394 ) ;
#8140=VERTEX_POINT ( 'NONE', #36587 ) ;
#8141=CARTESIAN_POINT ( 'NONE',  ( -16.96165138597773137, 2.229229656569007290, 7.128348183318155229 ) ) ;
#8143=ORIENTED_EDGE ( 'NONE', *, *, #40264, .F. ) ;
#8144=EDGE_CURVE ( 'NONE', #26049, #7904, #28067, .T. ) ;
#8145=EDGE_LOOP ( 'NONE', ( #35752, #53299, #5889, #49854 ) ) ;
#8146=ORIENTED_EDGE ( 'NONE', *, *, #18738, .F. ) ;
#8147=ORIENTED_EDGE ( 'NONE', *, *, #54315, .F. ) ;
#8148=ORIENTED_EDGE ( 'NONE', *, *, #20545, .F. ) ;
#8149=EDGE_LOOP ( 'NONE', ( #5634, #22556, #33229, #28921 ) ) ;
#8150=DIRECTION ( 'NONE',  ( 0.5449076811759707706, 0.6444004775717708799, -0.5364919789714476250 ) ) ;
#8151=DIRECTION ( 'NONE',  ( 0.005002170337468016433, -0.7660444431189770143, -0.6427681459581293666 ) ) ;
#8152=DIRECTION ( 'NONE',  ( 0.005002170337468016433, -0.7660444431189770143, -0.6427681459581293666 ) ) ;
#8153=EDGE_CURVE ( 'NONE', #2187, #19558, #28634, .T. ) ;
#8154=EDGE_CURVE ( 'NONE', #23769, #12809, #54194, .T. ) ;
#8155=EDGE_CURVE ( 'NONE', #39340, #49361, #2505, .T. ) ;
#8156=VERTEX_POINT ( 'NONE', #45372 ) ;
#8157=DIRECTION ( 'NONE',  ( -0.9999697198139514409, -0.000000000000000000, -0.007781995580013368816 ) ) ;
#8158=ORIENTED_EDGE ( 'NONE', *, *, #52905, .F. ) ;
#8159=DIRECTION ( 'NONE',  ( 0.007781995580012662783, 0.000000000000000000, -0.9999697198139514409 ) ) ;
#8160=EDGE_CURVE ( 'NONE', #40567, #21134, #50193, .T. ) ;
#8161=ORIENTED_EDGE ( 'NONE', *, *, #20936, .F. ) ;
#8162=DIRECTION ( 'NONE',  ( 0.000000000000000000, -1.000000000000000000, 0.000000000000000000 ) ) ;
#8163=FACE_OUTER_BOUND ( 'NONE', #23984, .T. ) ;
#8164=CARTESIAN_POINT ( 'NONE',  ( -12.73462046044971174, 0.000000000000000000, 2.874643015499314558 ) ) ;
#8165=EDGE_LOOP ( 'NONE', ( #23731, #38820, #45759, #45818 ) ) ;
#8166=DIRECTION ( 'NONE',  ( -0.005002170337468016433, -0.7660444431189770143, 0.6427681459581293666 ) ) ;
#8167=ORIENTED_EDGE ( 'NONE', *, *, #27917, .F. ) ;
#8168=PLANE ( 'NONE',  #4660 ) ;
#8169=CARTESIAN_POINT ( 'NONE',  ( -18.13481810573821562, 0.000000000000000000, 5.987280043424108911 ) ) ;
#8170=ADVANCED_FACE ( 'NONE', ( #23793 ), #45651, .F. ) ;
#8171=VECTOR ( 'NONE', #44237, 999.9999999999998863 ) ;
#8173=CARTESIAN_POINT ( 'NONE',  ( -10.90062170024363297, 0.000000000000000000, 6.043578232596257038 ) ) ;
#8174=LINE ( 'NONE', #41945, #20218 ) ;
#8175=PLANE ( 'NONE',  #1328 ) ;
#8176=EDGE_CURVE ( 'NONE', #23263, #29692, #11301, .T. ) ;
#8177=LINE ( 'NONE', #55047, #3047 ) ;
#8179=ORIENTED_EDGE ( 'NONE', *, *, #48619, .F. ) ;
#8180=DIRECTION ( 'NONE',  ( 0.000000000000000000, -0.000000000000000000, -1.000000000000000000 ) ) ;
#8181=ORIENTED_EDGE ( 'NONE', *, *, #22370, .F. ) ;
#8182=EDGE_CURVE ( 'NONE', #28225, #33592, #2755, .T. ) ;
#8184=DIRECTION ( 'NONE',  ( 0.005002170337468016433, -0.7660444431189770143, -0.6427681459581293666 ) ) ;
#8185=CARTESIAN_POINT ( 'NONE',  ( -10.27421835998572064, 0.000000000000000000, 10.96090226820206048 ) ) ;
#8186=LINE ( 'NONE', #25495, #8637 ) ;
#8187=FACE_OUTER_BOUND ( 'NONE', #2863, .T. ) ;
#8188=ADVANCED_FACE ( 'NONE', ( #7062 ), #24360, .F. ) ;
#8189=CARTESIAN_POINT ( 'NONE',  ( -1.086233639165236964, 0.000000000000000000, -2.796443541562362078 ) ) ;
#8190=ORIENTED_EDGE ( 'NONE', *, *, #17450, .T. ) ;
#8191=CARTESIAN_POINT ( 'NONE',  ( -14.43915895993578502, 0.000000000000000000, 8.770691019667511412 ) ) ;
#8192=LINE ( 'NONE', #21550, #15853 ) ;
#8193=DIRECTION ( 'NONE',  ( -0.005961354470445682716, -0.6427876096865404731, 0.7660212471507180654 ) ) ;
#8194=DIRECTION ( 'NONE',  ( 0.007781995580012663651, -3.146120232559066537E-19, -0.9999697198139514409 ) ) ;
#8195=DIRECTION ( 'NONE',  ( -0.5449076811759708816, 0.6444004775717707689, 0.5364919789714475140 ) ) ;
#8196=LINE ( 'NONE', #43404, #42237 ) ;
#8198=ORIENTED_EDGE ( 'NONE', *, *, #27030, .F. ) ;
#8199=LINE ( 'NONE', #16716, #1337 ) ;
#8200=CARTESIAN_POINT ( 'NONE',  ( -16.81267852042391198, -0.1191753592594197858, 3.312241722634738039 ) ) ;
#8201=EDGE_LOOP ( 'NONE', ( #28961, #36035, #38286, #20791 ) ) ;
#8202=ORIENTED_EDGE ( 'NONE', *, *, #48286, .T. ) ;
#8203=CARTESIAN_POINT ( 'NONE',  ( -15.08393937872457791, -3.594132820645662196, 2.625763770285873377 ) ) ;
#8204=EDGE_LOOP ( 'NONE', ( #25923, #13500, #41157, #46833 ) ) ;
#8205=VECTOR ( 'NONE', #32973, 1000.000000000000000 ) ;
#8206=VERTEX_POINT ( 'NONE', #31959 ) ;
#8207=EDGE_LOOP ( 'NONE', ( #50054, #36499, #17631, #55686, #8855, #33481, #38964, #30023, #15521, #966, #853, #44657, #16811, #11888, #5681, #16108, #42187, #49212, #17983, #44204, #10008, #55510, #27109, #38459, #53833, #37444, #11051, #36435, #24752, #6989, #52277, #25982, #41057, #22494, #20552, #55853, #13948, #25433, #46256, #38646, #25003, #42449, #22631, #27397, #8108, #14040, #21896 ) ) ;
#8208=EDGE_LOOP ( 'NONE', ( #21419, #6416, #542, #50568 ) ) ;
#8209=LINE ( 'NONE', #42841, #47510 ) ;
#8211=CARTESIAN_POINT ( 'NONE',  ( -12.23851102634202448, -0.1191753592594197858, 11.68427982808754884 ) ) ;
#8213=EDGE_CURVE ( 'NONE', #7098, #42447, #6149, .T. ) ;
#8214=ORIENTED_EDGE ( 'NONE', *, *, #24597, .T. ) ;
#8215=ORIENTED_EDGE ( 'NONE', *, *, #15158, .T. ) ;
#8216=EDGE_CURVE ( 'NONE', #40269, #55983, #18916, .T. ) ;
#8217=EDGE_CURVE ( 'NONE', #42498, #30608, #39917, .T. ) ;
#8218=DIRECTION ( 'NONE',  ( -0.005002170337468016433, -0.7660444431189770143, 0.6427681459581293666 ) ) ;
#8219=DIRECTION ( 'NONE',  ( -0.9999697198139514409, -0.000000000000000000, -0.007781995580013368816 ) ) ;
#8220=ORIENTED_EDGE ( 'NONE', *, *, #1870, .T. ) ;
#8221=LINE ( 'NONE', #12759, #33687 ) ;
#8222=DIRECTION ( 'NONE',  ( 0.5364919789714477361, 0.6444004775717706579, 0.5449076811759711036 ) ) ;
#8224=DIRECTION ( 'NONE',  ( 0.000000000000000000, -1.000000000000000000, 0.000000000000000000 ) ) ;
#8225=EDGE_LOOP ( 'NONE', ( #6025, #6205, #40997, #54655 ) ) ;
#8226=CARTESIAN_POINT ( 'NONE',  ( -10.90636980725419924, 0.000000000000000000, 6.782197639111785747 ) ) ;
#8227=DIRECTION ( 'NONE',  ( 0.007781995580012663651, -3.146120232559066537E-19, -0.9999697198139514409 ) ) ;
#8228=ORIENTED_EDGE ( 'NONE', *, *, #18691, .T. ) ;
#8229=CARTESIAN_POINT ( 'NONE',  ( -21.45130150109525502, -2.298917212465658721, 5.140387614241637593 ) ) ;
#8230=CARTESIAN_POINT ( 'NONE',  ( 2.072287782118878319, 0.000000000000000000, -2.950529333540147015 ) ) ;
#8231=DIRECTION ( 'NONE',  ( 0.000000000000000000, -0.000000000000000000, -1.000000000000000000 ) ) ;
#8232=CARTESIAN_POINT ( 'NONE',  ( -12.67473335678518787, -2.946525016555661125, 1.710608413933282446 ) ) ;
#8233=ORIENTED_EDGE ( 'NONE', *, *, #40287, .F. ) ;
#8234=VECTOR ( 'NONE', #48610, 1000.000000000000227 ) ;
#8235=LINE ( 'NONE', #21598, #52760 ) ;
#8236=PLANE ( 'NONE',  #49606 ) ;
#8237=PLANE ( 'NONE',  #53008 ) ;
#8238=CARTESIAN_POINT ( 'NONE',  ( -20.34615672165342914, -0.4026555460309505508, 5.262860474000830457 ) ) ;
#8239=EDGE_CURVE ( 'NONE', #22811, #19098, #31113, .T. ) ;
#8240=FACE_OUTER_BOUND ( 'NONE', #37728, .T. ) ;
#8241=CARTESIAN_POINT ( 'NONE',  ( -17.78010129026580444, -1.813211359398158029, 3.729865337533703862 ) ) ;
#8242=AXIS2_PLACEMENT_3D ( 'NONE', #33472, #33736, #2777 ) ;
#8243=LINE ( 'NONE', #25863, #24068 ) ;
#8244=ORIENTED_EDGE ( 'NONE', *, *, #20286, .F. ) ;
#8245=ADVANCED_FACE ( 'NONE', ( #23454 ), #9552, .F. ) ;
#8246=FACE_OUTER_BOUND ( 'NONE', #29920, .T. ) ;
#8247=VERTEX_POINT ( 'NONE', #49576 ) ;
#8248=CARTESIAN_POINT ( 'NONE',  ( -23.33849165029409889, 0.000000000000000000, 5.946783852668351855 ) ) ;
#8249=DIRECTION ( 'NONE',  ( 0.000000000000000000, -0.000000000000000000, -1.000000000000000000 ) ) ;
#8250=EDGE_CURVE ( 'NONE', #1446, #50929, #997, .T. ) ;
#8251=CARTESIAN_POINT ( 'NONE',  ( -13.49066169485000977, -4.403642575758160760, 9.149290569145874130 ) ) ;
#8252=DIRECTION ( 'NONE',  ( -0.5449076811759708816, 0.6444004775717707689, 0.5364919789714475140 ) ) ;
#8253=DIRECTION ( 'NONE',  ( 0.6427681459581294776, -0.7660444431189769032, 0.005002170337467562802 ) ) ;
#8254=VERTEX_POINT ( 'NONE', #36490 ) ;
#8255=VERTEX_POINT ( 'NONE', #40502 ) ;
#8257=DIRECTION ( 'NONE',  ( 0.007781995580012663651, -3.146120232559066537E-19, -0.9999697198139514409 ) ) ;
#8258=EDGE_LOOP ( 'NONE', ( #30365, #32129, #5093, #11207 ) ) ;
#8259=FACE_OUTER_BOUND ( 'NONE', #46435, .T. ) ;
#8260=AXIS2_PLACEMENT_3D ( 'NONE', #273, #52537, #47996 ) ;
#8261=VECTOR ( 'NONE', #27021, 1000.000000000000000 ) ;
#8262=EDGE_LOOP ( 'NONE', ( #26177, #48371, #21766, #18816 ) ) ;
#8263=CARTESIAN_POINT ( 'NONE',  ( -14.51981575693820581, -0.1191753592594177180, 6.284741869286547100 ) ) ;
#8265=DIRECTION ( 'NONE',  ( 0.000000000000000000, -0.000000000000000000, -1.000000000000000000 ) ) ;
#8267=EDGE_LOOP ( 'NONE', ( #26895, #44707, #29685, #35578 ) ) ;
#8268=ORIENTED_EDGE ( 'NONE', *, *, #16534, .T. ) ;
#8269=LINE ( 'NONE', #52294, #34784 ) ;
#8270=EDGE_CURVE ( 'NONE', #46401, #35585, #39665, .T. ) ;
#8271=PLANE ( 'NONE',  #7843 ) ;
#8272=CARTESIAN_POINT ( 'NONE',  ( -15.32150246818737394, 0.000000000000000000, 2.733018303394165294 ) ) ;
#8273=ADVANCED_FACE ( 'NONE', ( #14380 ), #26872, .F. ) ;
#8274=VECTOR ( 'NONE', #10488, 1000.000000000000000 ) ;
#8275=DIRECTION ( 'NONE',  ( 0.5449076811759707706, 0.6444004775717708799, -0.5364919789714476250 ) ) ;
#8276=ORIENTED_EDGE ( 'NONE', *, *, #42192, .T. ) ;
#8277=ORIENTED_EDGE ( 'NONE', *, *, #46863, .F. ) ;
#8278=EDGE_CURVE ( 'NONE', #12964, #7991, #27714, .T. ) ;
#8279=ADVANCED_FACE ( 'NONE', ( #22341 ), #53809, .F. ) ;
#8280=VECTOR ( 'NONE', #45642, 1000.000000000000227 ) ;
#8281=VERTEX_POINT ( 'NONE', #1286 ) ;
#8282=DIRECTION ( 'NONE',  ( 0.7660212471507180654, -0.6427876096865404731, 0.005961354470445141482 ) ) ;
#8283=CARTESIAN_POINT ( 'NONE',  ( -12.76204334111325700, 0.000000000000000000, 6.398424288781984437 ) ) ;
#8286=VERTEX_POINT ( 'NONE', #744 ) ;
#8287=CARTESIAN_POINT ( 'NONE',  ( -13.08486533123210194, 0.000000000000000000, 1.963927175729152541 ) ) ;
#8288=LINE ( 'NONE', #42384, #9509 ) ;
#8289=VERTEX_POINT ( 'NONE', #18062 ) ;
#8290=CARTESIAN_POINT ( 'NONE',  ( -15.52211495245506256, 0.000000000000000000, 2.810943005112377158 ) ) ;
#8291=ORIENTED_EDGE ( 'NONE', *, *, #19449, .F. ) ;
#8292=EDGE_CURVE ( 'NONE', #21743, #21718, #52685, .T. ) ;
#8293=LINE ( 'NONE', #8888, #10954 ) ;
#8294=CARTESIAN_POINT ( 'NONE',  ( -18.67697421479882181, -0.1191753592594197858, 4.036397482078229793 ) ) ;
#8295=ORIENTED_EDGE ( 'NONE', *, *, #18344, .T. ) ;
#8297=DIRECTION ( 'NONE',  ( 0.005002170337468016433, -0.7660444431189770143, -0.6427681459581293666 ) ) ;
#8298=CARTESIAN_POINT ( 'NONE',  ( -14.66887761629205222, 0.000000000000000000, 12.58869632783390990 ) ) ;
#8299=CARTESIAN_POINT ( 'NONE',  ( -11.20636620717317378, 0.000000000000000000, 11.32298014792380414 ) ) ;
#8300=ORIENTED_EDGE ( 'NONE', *, *, #50078, .T. ) ;
#8301=AXIS2_PLACEMENT_3D ( 'NONE', #24329, #41902, #37110 ) ;
#8302=VECTOR ( 'NONE', #37716, 1000.000000000000227 ) ;
#8303=DIRECTION ( 'NONE',  ( -0.5364919789714478471, 0.6444004775717705469, -0.5449076811759709926 ) ) ;
#8304=CARTESIAN_POINT ( 'NONE',  ( -8.476662044498805670, -0.1191753592594181482, 5.962439019012909291 ) ) ;
#8305=CARTESIAN_POINT ( 'NONE',  ( -9.295220851736454293, 0.000000000000000000, 4.578743553985232140 ) ) ;
#8306=DIRECTION ( 'NONE',  ( 0.5449076811759707706, 0.6444004775717708799, -0.5364919789714476250 ) ) ;
#8307=LINE ( 'NONE', #21666, #27942 ) ;
#8308=DIRECTION ( 'NONE',  ( 0.005961354470445682716, -0.6427876096865404731, -0.7660212471507180654 ) ) ;
#8309=AXIS2_PLACEMENT_3D ( 'NONE', #37566, #37025, #50891 ) ;
#8310=ORIENTED_EDGE ( 'NONE', *, *, #39769, .T. ) ;
#8311=DIRECTION ( 'NONE',  ( 0.000000000000000000, -1.000000000000000000, 0.000000000000000000 ) ) ;
#8312=DIRECTION ( 'NONE',  ( 0.005961354470445682716, -0.6427876096865404731, -0.7660212471507180654 ) ) ;
#8313=DIRECTION ( 'NONE',  ( 0.000000000000000000, -0.000000000000000000, -1.000000000000000000 ) ) ;
#8314=VERTEX_POINT ( 'NONE', #18627 ) ;
#8315=DIRECTION ( 'NONE',  ( 0.5364919789714477361, 0.6444004775717706579, 0.5449076811759711036 ) ) ;
#8316=FACE_OUTER_BOUND ( 'NONE', #46071, .T. ) ;
#8317=ORIENTED_EDGE ( 'NONE', *, *, #36134, .T. ) ;
#8318=CARTESIAN_POINT ( 'NONE',  ( -9.075990533167328067, 0.000000000000000000, 10.41622904950343909 ) ) ;
#8319=LINE ( 'NONE', #12865, #23313 ) ;
#8320=EDGE_CURVE ( 'NONE', #21187, #11287, #5298, .T. ) ;
#8321=CARTESIAN_POINT ( 'NONE',  ( -23.33693525117809386, 0.000000000000000000, 5.746789908705562944 ) ) ;
#8322=VECTOR ( 'NONE', #16672, 999.9999999999998863 ) ;
#8324=ORIENTED_EDGE ( 'NONE', *, *, #38680, .T. ) ;
#8327=CARTESIAN_POINT ( 'NONE',  ( -20.77325648630311150, -3.108426967578157729, 9.852428232502697725 ) ) ;
#8328=DIRECTION ( 'NONE',  ( 0.007781995580012662783, 0.000000000000000000, -0.9999697198139514409 ) ) ;
#8329=EDGE_CURVE ( 'NONE', #23836, #3819, #14095, .T. ) ;
#8330=LINE ( 'NONE', #39839, #20233 ) ;
#8331=FACE_OUTER_BOUND ( 'NONE', #14888, .T. ) ;
#8332=LINE ( 'NONE', #50918, #54837 ) ;
#8333=EDGE_LOOP ( 'NONE', ( #38836, #3214, #53226, #34597, #48275, #21251, #1697, #31551 ) ) ;
#8334=EDGE_CURVE ( 'NONE', #29513, #12044, #9840, .T. ) ;
#8335=LINE ( 'NONE', #46680, #24699 ) ;
#8336=EDGE_CURVE ( 'NONE', #24506, #8726, #48997, .T. ) ;
#8337=DIRECTION ( 'NONE',  ( 0.5449076811759707706, 0.6444004775717708799, -0.5364919789714476250 ) ) ;
#8339=LINE ( 'NONE', #52615, #13856 ) ;
#8340=EDGE_CURVE ( 'NONE', #6097, #45628, #44452, .T. ) ;
#8341=LINE ( 'NONE', #38443, #44064 ) ;
#8342=DIRECTION ( 'NONE',  ( -0.9999697198139514409, -0.000000000000000000, -0.007781995580013368816 ) ) ;
#8343=EDGE_LOOP ( 'NONE', ( #3533, #24771, #17697, #15473 ) ) ;
#8344=VECTOR ( 'NONE', #363, 1000.000000000000114 ) ;
#8345=VECTOR ( 'NONE', #48166, 1000.000000000000114 ) ;
#8346=PLANE ( 'NONE',  #15773 ) ;
#8347=ADVANCED_FACE ( 'NONE', ( #40196 ), #17539, .F. ) ;
#8348=ORIENTED_EDGE ( 'NONE', *, *, #20952, .T. ) ;
#8349=EDGE_CURVE ( 'NONE', #15384, #6272, #51886, .T. ) ;
#8350=ORIENTED_EDGE ( 'NONE', *, *, #55858, .T. ) ;
#8351=EDGE_LOOP ( 'NONE', ( #34754, #5942, #41855, #26309 ) ) ;
#8352=VECTOR ( 'NONE', #13613, 999.9999999999998863 ) ;
#8353=EDGE_LOOP ( 'NONE', ( #9660, #15273, #2319, #4141 ) ) ;
#8354=FACE_OUTER_BOUND ( 'NONE', #28839, .T. ) ;
#8355=ORIENTED_EDGE ( 'NONE', *, *, #44825, .F. ) ;
#8356=CARTESIAN_POINT ( 'NONE',  ( -24.26908309836554878, 0.000000000000000000, 6.108867788427308376 ) ) ;
#8357=EDGE_CURVE ( 'NONE', #32587, #47105, #4757, .T. ) ;
#8358=ORIENTED_EDGE ( 'NONE', *, *, #864, .F. ) ;
#8359=DIRECTION ( 'NONE',  ( 0.7660212471507180654, -0.6427876096865404731, 0.005961354470445141482 ) ) ;
#8360=ORIENTED_EDGE ( 'NONE', *, *, #3998, .T. ) ;
#8361=LINE ( 'NONE', #26811, #43713 ) ;
#8362=VECTOR ( 'NONE', #43978, 999.9999999999998863 ) ;
#8363=ORIENTED_EDGE ( 'NONE', *, *, #44809, .F. ) ;
#8364=EDGE_CURVE ( 'NONE', #17269, #38033, #18098, .T. ) ;
#8365=LINE ( 'NONE', #33934, #51081 ) ;
#8366=DIRECTION ( 'NONE',  ( 0.007781995580012662783, 0.000000000000000000, -0.9999697198139514409 ) ) ;
#8367=DIRECTION ( 'NONE',  ( -0.005002170337468016433, -0.7660444431189770143, 0.6427681459581293666 ) ) ;
#8368=DIRECTION ( 'NONE',  ( 0.000000000000000000, -1.000000000000000000, 0.000000000000000000 ) ) ;
#8369=DIRECTION ( 'NONE',  ( 0.8531650599175529814, -0.4028455766673920135, -0.3313982828793697877 ) ) ;
#8370=ORIENTED_EDGE ( 'NONE', *, *, #18167, .F. ) ;
#8371=EDGE_LOOP ( 'NONE', ( #27481, #28256, #25584, #41917 ) ) ;
#8372=DIRECTION ( 'NONE',  ( -0.005002170337468016433, -0.7660444431189770143, 0.6427681459581293666 ) ) ;
#8373=DIRECTION ( 'NONE',  ( -0.6427681459581293666, -0.7660444431189770143, -0.005002170337467561935 ) ) ;
#8374=VECTOR ( 'NONE', #33051, 999.9999999999998863 ) ;
#8376=LINE ( 'NONE', #2983, #48597 ) ;
#8377=DIRECTION ( 'NONE',  ( 0.007781995580012663651, -3.146120232559066537E-19, -0.9999697198139514409 ) ) ;
#8378=PLANE ( 'NONE',  #50407 ) ;
#8379=ORIENTED_EDGE ( 'NONE', *, *, #53984, .F. ) ;
#8380=VECTOR ( 'NONE', #47252, 999.9999999999998863 ) ;
#8381=DIRECTION ( 'NONE',  ( 0.9999697198139515519, 0.000000000000000000, 0.007781995580013368816 ) ) ;
#8382=CARTESIAN_POINT ( 'NONE',  ( -19.60834386242827776, 0.000000000000000000, 4.298478389818581213 ) ) ;
#8383=ORIENTED_EDGE ( 'NONE', *, *, #28599, .F. ) ;
#8384=VECTOR ( 'NONE', #1055, 999.9999999999998863 ) ;
#8385=VECTOR ( 'NONE', #3123, 1000.000000000000000 ) ;
#8386=DIRECTION ( 'NONE',  ( 0.000000000000000000, -0.000000000000000000, -1.000000000000000000 ) ) ;
#8387=CARTESIAN_POINT ( 'NONE',  ( -12.80458192191714595, 0.000000000000000000, 11.86454056839041726 ) ) ;
#8388=EDGE_CURVE ( 'NONE', #11826, #25841, #34871, .T. ) ;
#8389=DIRECTION ( 'NONE',  ( 0.005002170337468016433, -0.7660444431189770143, -0.6427681459581293666 ) ) ;
#8390=LINE ( 'NONE', #43040, #6024 ) ;
#8391=VERTEX_POINT ( 'NONE', #13303 ) ;
#8392=AXIS2_PLACEMENT_3D ( 'NONE', #14436, #27475, #40566 ) ;
#8393=VECTOR ( 'NONE', #36600, 1000.000000000000227 ) ;
#8394=ORIENTED_EDGE ( 'NONE', *, *, #34056, .T. ) ;
#8395=DIRECTION ( 'NONE',  ( -0.5449076811759708816, 0.6444004775717707689, 0.5364919789714475140 ) ) ;
#8396=CARTESIAN_POINT ( 'NONE',  ( -16.06709938707323460, 0.000000000000000000, 13.13181314741652628 ) ) ;
#8397=CARTESIAN_POINT ( 'NONE',  ( -15.86710544311044302, 0.000000000000000000, 13.13336954653252953 ) ) ;
#8398=CARTESIAN_POINT ( 'NONE',  ( -12.16789073767994900, -0.1191753592594193972, 2.609724395548954412 ) ) ;
#8399=VECTOR ( 'NONE', #48691, 999.9999999999998863 ) ;
#8400=FACE_OUTER_BOUND ( 'NONE', #15587, .T. ) ;
#8401=CARTESIAN_POINT ( 'NONE',  ( -12.76336099550253600, 0.000000000000000000, 6.567740048076958104 ) ) ;
#8402=DIRECTION ( 'NONE',  ( 0.000000000000000000, -1.000000000000000000, 0.000000000000000000 ) ) ;
#8403=ORIENTED_EDGE ( 'NONE', *, *, #25804, .T. ) ;
#8404=ADVANCED_FACE ( 'NONE', ( #35172 ), #43933, .F. ) ;
#8405=CARTESIAN_POINT ( 'NONE',  ( -20.54049170961573267, 0.000000000000000000, 4.660556269540326646 ) ) ;
#8406=CARTESIAN_POINT ( 'NONE',  ( -13.27703486227003893, -3.108426967578160838, 1.939397253021431400 ) ) ;
#8407=FACE_OUTER_BOUND ( 'NONE', #52557, .T. ) ;
#8408=ORIENTED_EDGE ( 'NONE', *, *, #24307, .T. ) ;
#8409=DIRECTION ( 'NONE',  ( 0.6427681459581294776, -0.7660444431189769032, 0.005002170337467562802 ) ) ;
#8410=ORIENTED_EDGE ( 'NONE', *, *, #15159, .F. ) ;
#8411=EDGE_CURVE ( 'NONE', #47831, #2828, #21797, .T. ) ;
#8412=AXIS2_PLACEMENT_3D ( 'NONE', #22463, #35493, #13912 ) ;
#8413=EDGE_LOOP ( 'NONE', ( #39143, #33989, #4320, #48718 ) ) ;
#8414=ADVANCED_FACE ( 'NONE', ( #25785 ), #16997, .F. ) ;
#8415=ORIENTED_EDGE ( 'NONE', *, *, #3840, .F. ) ;
#8416=ORIENTED_EDGE ( 'NONE', *, *, #15624, .T. ) ;
#8417=EDGE_LOOP ( 'NONE', ( #21887, #54431, #12401, #47696 ) ) ;
#8418=VERTEX_POINT ( 'NONE', #43392 ) ;
#8419=AXIS2_PLACEMENT_3D ( 'NONE', #51071, #15585, #30588 ) ;
#8420=CARTESIAN_POINT ( 'NONE',  ( -25.20123094555300369, 0.000000000000000000, 6.470945668149052032 ) ) ;
#8421=PLANE ( 'NONE',  #53797 ) ;
#8423=AXIS2_PLACEMENT_3D ( 'NONE', #4996, #733, #22599 ) ;
#8424=EDGE_CURVE ( 'NONE', #6407, #41644, #30875, .T. ) ;
#8425=VECTOR ( 'NONE', #31152, 999.9999999999998863 ) ;
#8426=ORIENTED_EDGE ( 'NONE', *, *, #24722, .F. ) ;
#8427=LINE ( 'NONE', #13273, #49430 ) ;
#8428=EDGE_LOOP ( 'NONE', ( #40136, #19229, #6713, #29587 ) ) ;
#8430=EDGE_LOOP ( 'NONE', ( #40416, #24, #53357, #48947 ) ) ;
#8431=ADVANCED_FACE ( 'NONE', ( #4488 ), #39701, .F. ) ;
#8432=VECTOR ( 'NONE', #29682, 999.9999999999998863 ) ;
#8433=VECTOR ( 'NONE', #8844, 999.9999999999998863 ) ;
#8434=CARTESIAN_POINT ( 'NONE',  ( 2.072287782118878319, 0.000000000000000000, -2.950529333540147015 ) ) ;
#8435=DIRECTION ( 'NONE',  ( 0.9999697198139515519, 0.000000000000000000, 0.007781995580013368816 ) ) ;
#8436=DIRECTION ( 'NONE',  ( -0.005961354470445682716, -0.6427876096865404731, 0.7660212471507180654 ) ) ;
#8437=ORIENTED_EDGE ( 'NONE', *, *, #25767, .T. ) ;
#8438=PLANE ( 'NONE',  #51887 ) ;
#8439=EDGE_LOOP ( 'NONE', ( #5470, #19775, #13802, #51372 ) ) ;
#8440=DIRECTION ( 'NONE',  ( -0.5449076811759708816, 0.6444004775717707689, 0.5364919789714475140 ) ) ;
#8441=FACE_OUTER_BOUND ( 'NONE', #39149, .T. ) ;
#8442=VECTOR ( 'NONE', #18637, 999.9999999999998863 ) ;
#8443=FACE_OUTER_BOUND ( 'NONE', #34123, .T. ) ;
#8444=LINE ( 'NONE', #3049, #2285 ) ;
#8445=DIRECTION ( 'NONE',  ( 0.000000000000000000, -0.000000000000000000, -1.000000000000000000 ) ) ;
#8446=DIRECTION ( 'NONE',  ( 0.7660212471507180654, -0.6427876096865404731, 0.005961354470445141482 ) ) ;
#8447=CARTESIAN_POINT ( 'NONE',  ( -18.87699506648361947, 1.743523803501505709, 7.075206662320437268 ) ) ;
#8449=ORIENTED_EDGE ( 'NONE', *, *, #734, .F. ) ;
#8450=DIRECTION ( 'NONE',  ( 0.9999697198139515519, 0.000000000000000000, 0.007781995580013368816 ) ) ;
#8451=ORIENTED_EDGE ( 'NONE', *, *, #49248, .T. ) ;
#8452=ADVANCED_FACE ( 'NONE', ( #9291 ), #47348, .F. ) ;
#8453=VECTOR ( 'NONE', #15682, 1000.000000000000114 ) ;
#8454=DIRECTION ( 'NONE',  ( 0.9999697198139515519, 0.000000000000000000, 0.007781995580013368816 ) ) ;
#8455=CARTESIAN_POINT ( 'NONE',  ( 2.072287782118878319, 0.000000000000000000, -2.950529333540147015 ) ) ;
#8456=DIRECTION ( 'NONE',  ( 0.7660212471507180654, -0.6427876096865404731, 0.005961354470445141482 ) ) ;
#8457=EDGE_CURVE ( 'NONE', #14391, #45314, #39116, .T. ) ;
#8458=VECTOR ( 'NONE', #55685, 1000.000000000000227 ) ;
#8459=CARTESIAN_POINT ( 'NONE',  ( -19.27402565828830205, 0.000000000000000000, 7.255736689840353471 ) ) ;
#8460=DIRECTION ( 'NONE',  ( -0.5364919789714478471, 0.6444004775717705469, -0.5449076811759709926 ) ) ;
#8461=DIRECTION ( 'NONE',  ( 0.9999697198139515519, 0.000000000000000000, 0.007781995580013368816 ) ) ;
#8462=LINE ( 'NONE', #9296, #13935 ) ;
#8463=ORIENTED_EDGE ( 'NONE', *, *, #8464, .T. ) ;
#8464=EDGE_CURVE ( 'NONE', #25146, #26810, #30043, .T. ) ;
#8465=VECTOR ( 'NONE', #38160, 999.9999999999998863 ) ;
#8467=CARTESIAN_POINT ( 'NONE',  ( -12.28749583716221316, -3.594132820645663084, 1.539530131120636858 ) ) ;
#8468=CARTESIAN_POINT ( 'NONE',  ( -10.94028622754223967, 0.000000000000000000, 11.14038480894692995 ) ) ;
#8469=EDGE_CURVE ( 'NONE', #4723, #36189, #31156, .T. ) ;
#8470=ADVANCED_FACE ( 'NONE', ( #25494 ), #42801, .F. ) ;
#8471=EDGE_CURVE ( 'NONE', #7098, #19098, #55895, .T. ) ;
#8472=VECTOR ( 'NONE', #10334, 1000.000000000000227 ) ;
#8473=VECTOR ( 'NONE', #22453, 1000.000000000000114 ) ;
#8474=DIRECTION ( 'NONE',  ( 0.9999697198139515519, 0.000000000000000000, 0.007781995580013368816 ) ) ;
#8476=FACE_OUTER_BOUND ( 'NONE', #28182, .T. ) ;
#8477=LINE ( 'NONE', #48197, #7486 ) ;
#8478=ORIENTED_EDGE ( 'NONE', *, *, #18011, .F. ) ;
#8479=VECTOR ( 'NONE', #25897, 999.9999999999998863 ) ;
#8480=CARTESIAN_POINT ( 'NONE',  ( -23.33849165029409889, 0.000000000000000000, 5.946783852668351855 ) ) ;
#8481=VECTOR ( 'NONE', #18376, 999.9999999999998863 ) ;
#8482=CARTESIAN_POINT ( 'NONE',  ( -14.66887761629205222, 0.000000000000000000, 12.58869632783390990 ) ) ;
#8483=ORIENTED_EDGE ( 'NONE', *, *, #37229, .F. ) ;
#8484=VERTEX_POINT ( 'NONE', #51620 ) ;
#8485=CARTESIAN_POINT ( 'NONE',  ( -19.07271405993623503, 0.000000000000000000, 7.087977329661382164 ) ) ;
#8486=ORIENTED_EDGE ( 'NONE', *, *, #25176, .F. ) ;
#8487=EDGE_CURVE ( 'NONE', #56078, #51473, #56166, .T. ) ;
#8488=EDGE_CURVE ( 'NONE', #37937, #55170, #36273, .T. ) ;
#8489=ORIENTED_EDGE ( 'NONE', *, *, #1132, .T. ) ;
#8490=ORIENTED_EDGE ( 'NONE', *, *, #16918, .T. ) ;
#8491=ORIENTED_EDGE ( 'NONE', *, *, #49208, .T. ) ;
#8492=AXIS2_PLACEMENT_3D ( 'NONE', #35328, #52625, #40129 ) ;
#8493=ADVANCED_FACE ( 'NONE', ( #22920 ), #27455, .F. ) ;
#8494=DIRECTION ( 'NONE',  ( 0.6246952433987894571, -0.7422098413412800966, -0.2426528472758541777 ) ) ;
#8495=ORIENTED_EDGE ( 'NONE', *, *, #18531, .T. ) ;
#8497=LINE ( 'NONE', #4518, #10382 ) ;
#8498=VECTOR ( 'NONE', #44826, 999.9999999999998863 ) ;
#8499=ADVANCED_FACE ( 'NONE', ( #40241 ), #5895, .F. ) ;
#8500=EDGE_LOOP ( 'NONE', ( #55471, #4414, #41927, #18713 ) ) ;
#8501=ORIENTED_EDGE ( 'NONE', *, *, #25648, .T. ) ;
#8502=VECTOR ( 'NONE', #16442, 1000.000000000000227 ) ;
#8503=ADVANCED_FACE ( 'NONE', ( #53025 ), #36533, .F. ) ;
#8505=EDGE_LOOP ( 'NONE', ( #49915, #42704, #29212, #51509 ) ) ;
#8506=VECTOR ( 'NONE', #54551, 1000.000000000000227 ) ;
#8507=DIRECTION ( 'NONE',  ( -0.5364919789714478471, 0.6444004775717705469, -0.5449076811759709926 ) ) ;
#8508=DIRECTION ( 'NONE',  ( -0.9999697198139514409, -0.000000000000000000, -0.007781995580013368816 ) ) ;
#8509=EDGE_LOOP ( 'NONE', ( #42846, #33146, #48883, #54111 ) ) ;
#8510=CARTESIAN_POINT ( 'NONE',  ( -21.47263955680318404, 0.000000000000000000, 5.022634149262071190 ) ) ;
#8511=AXIS2_PLACEMENT_3D ( 'NONE', #1091, #52514, #31780 ) ;
#8512=ORIENTED_EDGE ( 'NONE', *, *, #39081, .F. ) ;
#8513=CARTESIAN_POINT ( 'NONE',  ( -21.47341775636118655, -0.1191753592594197858, 5.122631121243466090 ) ) ;
#8514=AXIS2_PLACEMENT_3D ( 'NONE', #38301, #22615, #16435 ) ;
#8515=DIRECTION ( 'NONE',  ( 0.5364919789714477361, 0.6444004775717706579, 0.5449076811759711036 ) ) ;
#8516=VECTOR ( 'NONE', #51290, 1000.000000000000227 ) ;
#8517=ORIENTED_EDGE ( 'NONE', *, *, #38534, .T. ) ;
#8518=DIRECTION ( 'NONE',  ( 0.9999697198139515519, 0.000000000000000000, 0.007781995580013368816 ) ) ;
#8519=DIRECTION ( 'NONE',  ( 0.9999697198139515519, 0.000000000000000000, 0.007781995580013368816 ) ) ;
#8520=CARTESIAN_POINT ( 'NONE',  ( -12.10603466082523028, 0.000000000000000000, 7.511525709439289322 ) ) ;
#8521=CARTESIAN_POINT ( 'NONE',  ( -16.89925026227929195, -0.1191753592594197858, 13.49466922669627422 ) ) ;
#8522=ORIENTED_EDGE ( 'NONE', *, *, #8870, .F. ) ;
#8523=DIRECTION ( 'NONE',  ( 0.9999697198139515519, 0.000000000000000000, 0.007781995580013368816 ) ) ;
#8524=CARTESIAN_POINT ( 'NONE',  ( -18.79527752321125789, 2.229229656569007734, 3.911531714474451249 ) ) ;
#8525=CARTESIAN_POINT ( 'NONE',  ( -15.10787738939381519, -0.8417996532631553119, 3.931881018872667166 ) ) ;
#8526=DIRECTION ( 'NONE',  ( 0.007781995580012663651, -3.146120232559066537E-19, -0.9999697198139514409 ) ) ;
#8527=DIRECTION ( 'NONE',  ( 0.9999697198139515519, 0.000000000000000000, 0.007781995580013368816 ) ) ;
#8528=CARTESIAN_POINT ( 'NONE',  ( -14.43053679941993650, 0.000000000000000000, 7.662761909894217460 ) ) ;
#8529=FACE_OUTER_BOUND ( 'NONE', #11270, .T. ) ;
#8530=LINE ( 'NONE', #39480, #8473 ) ;
#8531=CARTESIAN_POINT ( 'NONE',  ( -20.54204810873173415, 0.000000000000000000, 4.860550213503115558 ) ) ;
#8532=VECTOR ( 'NONE', #25668, 999.9999999999998863 ) ;
#8533=VERTEX_POINT ( 'NONE', #15252 ) ;
#8535=LINE ( 'NONE', #48557, #9689 ) ;
#8536=ORIENTED_EDGE ( 'NONE', *, *, #54787, .F. ) ;
#8537=DIRECTION ( 'NONE',  ( 0.005961354470445682716, -0.6427876096865404731, -0.7660212471507180654 ) ) ;
#8538=DIRECTION ( 'NONE',  ( 0.005002170337468016433, -0.7660444431189770143, -0.6427681459581293666 ) ) ;
#8539=VECTOR ( 'NONE', #13490, 1000.000000000000227 ) ;
#8540=EDGE_CURVE ( 'NONE', #52907, #46963, #5597, .T. ) ;
#8541=ADVANCED_FACE ( 'NONE', ( #36841 ), #18954, .F. ) ;
#8542=PLANE ( 'NONE',  #13730 ) ;
#8543=AXIS2_PLACEMENT_3D ( 'NONE', #33097, #50417, #6698 ) ;
#8544=ADVANCED_FACE ( 'NONE', ( #45083 ), #1331, .F. ) ;
#8545=DIRECTION ( 'NONE',  ( 0.5364919789714477361, 0.6444004775717706579, 0.5449076811759711036 ) ) ;
#8546=FACE_OUTER_BOUND ( 'NONE', #7173, .T. ) ;
#8547=VERTEX_POINT ( 'NONE', #6187 ) ;
#8548=ORIENTED_EDGE ( 'NONE', *, *, #49689, .F. ) ;
#8549=CARTESIAN_POINT ( 'NONE',  ( -9.778419723998514002, 0.000000000000000000, 6.960301621058782473 ) ) ;
#8550=VECTOR ( 'NONE', #17719, 999.9999999999998863 ) ;
#8551=LINE ( 'NONE', #29857, #25896 ) ;
#8552=ORIENTED_EDGE ( 'NONE', *, *, #20658, .T. ) ;
#8553=AXIS2_PLACEMENT_3D ( 'NONE', #47200, #26456, #3759 ) ;
#8554=DIRECTION ( 'NONE',  ( 0.005002170337468016433, -0.7660444431189770143, -0.6427681459581293666 ) ) ;
#8556=DIRECTION ( 'NONE',  ( 0.7660212471507180654, -0.6427876096865404731, 0.005961354470445141482 ) ) ;
#8557=ORIENTED_EDGE ( 'NONE', *, *, #28084, .F. ) ;
#8558=LINE ( 'NONE', #25890, #34729 ) ;
#8559=EDGE_CURVE ( 'NONE', #49125, #593, #53326, .T. ) ;
#8560=AXIS2_PLACEMENT_3D ( 'NONE', #13842, #9303, #27196 ) ;
#8561=ORIENTED_EDGE ( 'NONE', *, *, #13361, .T. ) ;
#8565=DIRECTION ( 'NONE',  ( -0.5364919789714478471, 0.6444004775717705469, -0.5449076811759709926 ) ) ;
#8566=DIRECTION ( 'NONE',  ( 0.000000000000000000, -0.000000000000000000, -1.000000000000000000 ) ) ;
#8567=LINE ( 'NONE', #25900, #26655 ) ;
#8568=EDGE_CURVE ( 'NONE', #39978, #45002, #19495, .T. ) ;
#8569=DIRECTION ( 'NONE',  ( 0.6427681459581294776, -0.7660444431189769032, 0.005002170337467562802 ) ) ;
#8570=ORIENTED_EDGE ( 'NONE', *, *, #14136, .T. ) ;
#8571=EDGE_LOOP ( 'NONE', ( #29218, #19174, #41864, #7236 ) ) ;
#8572=EDGE_CURVE ( 'NONE', #11724, #40325, #23490, .T. ) ;
#8574=ORIENTED_EDGE ( 'NONE', *, *, #38534, .F. ) ;
#8575=EDGE_CURVE ( 'NONE', #42504, #16374, #40806, .T. ) ;
#8576=DIRECTION ( 'NONE',  ( 0.005961354470445682716, -0.6427876096865404731, -0.7660212471507180654 ) ) ;
#8577=VECTOR ( 'NONE', #14259, 1000.000000000000114 ) ;
#8578=ORIENTED_EDGE ( 'NONE', *, *, #24544, .F. ) ;
#8579=DIRECTION ( 'NONE',  ( -0.005002170337468016433, -0.7660444431189770143, 0.6427681459581293666 ) ) ;
#8580=EDGE_CURVE ( 'NONE', #22414, #44511, #5336, .T. ) ;
#8581=ORIENTED_EDGE ( 'NONE', *, *, #49039, .F. ) ;
#8582=VECTOR ( 'NONE', #26679, 1000.000000000000227 ) ;
#8583=CARTESIAN_POINT ( 'NONE',  ( -16.06709938707323460, 0.000000000000000000, 13.13181314741652628 ) ) ;
#8584=CARTESIAN_POINT ( 'NONE',  ( -16.81190032086591302, 0.000000000000000000, 3.212244750653343583 ) ) ;
#8585=ORIENTED_EDGE ( 'NONE', *, *, #20410, .F. ) ;
#8586=ADVANCED_FACE ( 'NONE', ( #10724 ), #49034, .F. ) ;
#8587=DIRECTION ( 'NONE',  ( -0.005002170337468016433, -0.7660444431189770143, 0.6427681459581293666 ) ) ;
#8588=EDGE_LOOP ( 'NONE', ( #14549, #49847, #50979, #28258 ) ) ;
#8589=CARTESIAN_POINT ( 'NONE',  ( -12.66126816957386225, -0.1191753592594177180, 6.299205516358588497 ) ) ;
#8590=VECTOR ( 'NONE', #23737, 1000.000000000000114 ) ;
#8591=EDGE_LOOP ( 'NONE', ( #52626, #52815, #16821, #39420 ) ) ;
#8592=PLANE ( 'NONE',  #55852 ) ;
#8593=DIRECTION ( 'NONE',  ( -0.5364919789714478471, 0.6444004775717705469, -0.5449076811759709926 ) ) ;
#8594=AXIS2_PLACEMENT_3D ( 'NONE', #41104, #5622, #22950 ) ;
#8595=DIRECTION ( 'NONE',  ( 0.005961354470445682716, -0.6427876096865404731, -0.7660212471507180654 ) ) ;
#8596=VERTEX_POINT ( 'NONE', #39956 ) ;
#8597=VECTOR ( 'NONE', #24245, 999.9999999999998863 ) ;
#8598=CARTESIAN_POINT ( 'NONE',  ( -17.21925308359982409, -4.403642575758160760, 10.59760208803285408 ) ) ;
#8599=PLANE ( 'NONE',  #40086 ) ;
#8600=LINE ( 'NONE', #17675, #34895 ) ;
#8601=DIRECTION ( 'NONE',  ( 0.007781995580012663651, -3.146120232559066537E-19, -0.9999697198139514409 ) ) ;
#8602=FACE_OUTER_BOUND ( 'NONE', #46917, .T. ) ;
#8603=DIRECTION ( 'NONE',  ( 0.5449076811759707706, 0.6444004775717708799, -0.5364919789714476250 ) ) ;
#8604=VECTOR ( 'NONE', #138, 999.9999999999998863 ) ;
#8605=VECTOR ( 'NONE', #3827, 1000.000000000000227 ) ;
#8606=LINE ( 'NONE', #38979, #4986 ) ;
#8607=VERTEX_POINT ( 'NONE', #18369 ) ;
#8608=DIRECTION ( 'NONE',  ( 0.000000000000000000, -0.000000000000000000, -1.000000000000000000 ) ) ;
#8609=CARTESIAN_POINT ( 'NONE',  ( -18.60520310958986911, 0.000000000000000000, 6.722283538171627271 ) ) ;
#8610=LINE ( 'NONE', #25942, #45909 ) ;
#8611=ORIENTED_EDGE ( 'NONE', *, *, #40090, .T. ) ;
#8613=LINE ( 'NONE', #53, #5956 ) ;
#8614=ORIENTED_EDGE ( 'NONE', *, *, #19636, .F. ) ;
#8615=ADVANCED_FACE ( 'NONE', ( #10137 ), #1041, .F. ) ;
#8616=DIRECTION ( 'NONE',  ( -0.7660212471507179544, -0.6427876096865405842, -0.005961354470445141482 ) ) ;
#8618=EDGE_CURVE ( 'NONE', #38231, #40568, #49868, .T. ) ;
#8619=PLANE ( 'NONE',  #43233 ) ;
#8621=VECTOR ( 'NONE', #14224, 999.9999999999998863 ) ;
#8622=EDGE_LOOP ( 'NONE', ( #43415, #40654, #49427, #31594 ) ) ;
#8623=ORIENTED_EDGE ( 'NONE', *, *, #42193, .T. ) ;
#8625=LINE ( 'NONE', #33897, #43940 ) ;
#8626=CARTESIAN_POINT ( 'NONE',  ( -16.82575592011193422, -0.1191753592594187450, 4.050804090899914556 ) ) ;
#8627=CARTESIAN_POINT ( 'NONE',  ( -16.57549827929610942, -1.489407457353159048, 3.272287659357408618 ) ) ;
#8628=AXIS2_PLACEMENT_3D ( 'NONE', #35099, #16929, #21469 ) ;
#8629=CARTESIAN_POINT ( 'NONE',  ( -12.96689773671041124, -0.5179957512181551094, 2.568834445894457197 ) ) ;
#8630=DIRECTION ( 'NONE',  ( -0.9999697198139514409, -0.000000000000000000, -0.007781995580013368816 ) ) ;
#8631=CARTESIAN_POINT ( 'NONE',  ( -15.86710544311044302, 0.000000000000000000, 13.13336954653252953 ) ) ;
#8632=AXIS2_PLACEMENT_3D ( 'NONE', #42862, #51106, #16753 ) ;
#8633=ORIENTED_EDGE ( 'NONE', *, *, #17150, .T. ) ;
#8634=DIRECTION ( 'NONE',  ( 0.5364919789714477361, 0.6444004775717706579, 0.5449076811759711036 ) ) ;
#8635=EDGE_CURVE ( 'NONE', #18328, #15829, #7546, .T. ) ;
#8636=DIRECTION ( 'NONE',  ( 0.005961354470445682716, -0.6427876096865404731, -0.7660212471507180654 ) ) ;
#8637=VECTOR ( 'NONE', #55056, 1000.000000000000114 ) ;
#8638=VECTOR ( 'NONE', #27370, 999.9999999999998863 ) ;
#8639=VERTEX_POINT ( 'NONE', #11251 ) ;
#8640=VECTOR ( 'NONE', #49745, 1000.000000000000227 ) ;
#8641=FACE_OUTER_BOUND ( 'NONE', #31850, .T. ) ;
#8643=LINE ( 'NONE', #34466, #33881 ) ;
#8644=VECTOR ( 'NONE', #54816, 1000.000000000000000 ) ;
#8645=ORIENTED_EDGE ( 'NONE', *, *, #56069, .T. ) ;
#8646=CARTESIAN_POINT ( 'NONE',  ( -9.978413667961302025, 0.000000000000000000, 6.958745221942781001 ) ) ;
#8647=ORIENTED_EDGE ( 'NONE', *, *, #29814, .F. ) ;
#8648=EDGE_CURVE ( 'NONE', #5931, #43311, #37661, .T. ) ;
#8650=ORIENTED_EDGE ( 'NONE', *, *, #18083, .F. ) ;
#8651=VECTOR ( 'NONE', #56094, 1000.000000000000227 ) ;
#8652=ORIENTED_EDGE ( 'NONE', *, *, #26573, .F. ) ;
#8653=EDGE_CURVE ( 'NONE', #45048, #7373, #50442, .T. ) ;
#8654=ORIENTED_EDGE ( 'NONE', *, *, #54748, .T. ) ;
#8655=DIRECTION ( 'NONE',  ( -0.5364919789714478471, 0.6444004775717705469, -0.5449076811759709926 ) ) ;
#8657=EDGE_LOOP ( 'NONE', ( #14516, #47040, #12647, #45777 ) ) ;
#8659=ORIENTED_EDGE ( 'NONE', *, *, #46405, .F. ) ;
#8660=FACE_OUTER_BOUND ( 'NONE', #8351, .T. ) ;
#8661=ADVANCED_FACE ( 'NONE', ( #46165 ), #29121, .F. ) ;
#8662=EDGE_LOOP ( 'NONE', ( #33918, #34280, #11078, #53494 ) ) ;
#8663=CARTESIAN_POINT ( 'NONE',  ( -15.88130887279446490, 0.000000000000000000, 3.050160814894388839 ) ) ;
#8664=EDGE_LOOP ( 'NONE', ( #46053, #34172, #25975, #6755 ) ) ;
#8665=VECTOR ( 'NONE', #7865, 1000.000000000000227 ) ;
#8666=CARTESIAN_POINT ( 'NONE',  ( -23.33771345073609638, -0.1191753592594197858, 5.846786880686956955 ) ) ;
#8667=AXIS2_PLACEMENT_3D ( 'NONE', #283, #43464, #16788 ) ;
#8668=CARTESIAN_POINT ( 'NONE',  ( -19.45503627000849889, 0.000000000000000000, 7.556996783084074742 ) ) ;
#8669=CARTESIAN_POINT ( 'NONE',  ( -12.99007897266819889, -5.536956232915667186, 1.750451042126190737 ) ) ;
#8670=FACE_OUTER_BOUND ( 'NONE', #25400, .T. ) ;
#8671=PLANE ( 'NONE',  #42847 ) ;
#8672=AXIS2_PLACEMENT_3D ( 'NONE', #11540, #15775, #49862 ) ;
#8673=ORIENTED_EDGE ( 'NONE', *, *, #55119, .F. ) ;
#8675=ORIENTED_EDGE ( 'NONE', *, *, #46672, .F. ) ;
#8676=CARTESIAN_POINT ( 'NONE',  ( -7.074322581158991596, -1.816507792529950871, 8.780998638722685712 ) ) ;
#8677=LINE ( 'NONE', #43853, #29413 ) ;
#8678=AXIS2_PLACEMENT_3D ( 'NONE', #56155, #31146, #35412 ) ;
#8679=ADVANCED_FACE ( 'NONE', ( #7268 ), #50972, .F. ) ;
#8680=EDGE_CURVE ( 'NONE', #53576, #11173, #24575, .T. ) ;
#8682=VECTOR ( 'NONE', #55102, 999.9999999999998863 ) ;
#8683=VECTOR ( 'NONE', #12123, 1000.000000000000114 ) ;
#8684=CARTESIAN_POINT ( 'NONE',  ( -10.67188722122801892, 0.000000000000000000, 2.352037599134615409 ) ) ;
#8685=CARTESIAN_POINT ( 'NONE',  ( -14.40047860997783147, 0.000000000000000000, 3.800349118021597583 ) ) ;
#8686=DIRECTION ( 'NONE',  ( -0.5364919789714478471, 0.6444004775717705469, -0.5449076811759709926 ) ) ;
#8687=VERTEX_POINT ( 'NONE', #28287 ) ;
#8688=DIRECTION ( 'NONE',  ( 0.007781995580012663651, 0.000000000000000000, -0.9999697198139515519 ) ) ;
#8689=ADVANCED_FACE ( 'NONE', ( #3571 ), #20630, .F. ) ;
#8690=DIRECTION ( 'NONE',  ( 0.005002170337468016433, -0.7660444431189770143, -0.6427681459581293666 ) ) ;
#8691=ORIENTED_EDGE ( 'NONE', *, *, #41234, .T. ) ;
#8692=VECTOR ( 'NONE', #8460, 1000.000000000000000 ) ;
#8693=CARTESIAN_POINT ( 'NONE',  ( -14.20280369269832832, 0.000000000000000000, 12.40765738797303719 ) ) ;
#8694=LINE ( 'NONE', #17192, #10635 ) ;
#8695=VECTOR ( 'NONE', #28179, 999.9999999999998863 ) ;
#8696=EDGE_CURVE ( 'NONE', #23033, #2866, #20878, .T. ) ;
#8697=VECTOR ( 'NONE', #519, 1000.000000000000227 ) ;
#8698=LINE ( 'NONE', #51564, #11429 ) ;
#8699=ADVANCED_FACE ( 'NONE', ( #41892 ), #46737, .F. ) ;
#8700=FACE_OUTER_BOUND ( 'NONE', #27072, .T. ) ;
#8701=AXIS2_PLACEMENT_3D ( 'NONE', #20278, #54937, #50927 ) ;
#8702=ORIENTED_EDGE ( 'NONE', *, *, #21580, .F. ) ;
#8703=VECTOR ( 'NONE', #20811, 1000.000000000000114 ) ;
#8704=VERTEX_POINT ( 'NONE', #25175 ) ;
#8705=FACE_OUTER_BOUND ( 'NONE', #23367, .T. ) ;
#8707=DIRECTION ( 'NONE',  ( 0.5449076811759707706, 0.6444004775717708799, -0.5364919789714476250 ) ) ;
#8708=ADVANCED_FACE ( 'NONE', ( #38200 ), #42483, .F. ) ;
#8709=LINE ( 'NONE', #35116, #20978 ) ;
#8710=CARTESIAN_POINT ( 'NONE',  ( -13.07066190154808361, 0.000000000000000000, 12.04713590736729678 ) ) ;
#8712=CARTESIAN_POINT ( 'NONE',  ( -8.456006654281710055, -0.1191753592594182315, 5.223935624422267665 ) ) ;
#8713=VERTEX_POINT ( 'NONE', #2992 ) ;
#8714=VECTOR ( 'NONE', #19913, 999.9999999999998863 ) ;
#8715=EDGE_CURVE ( 'NONE', #6448, #22624, #20323, .T. ) ;
#8716=PLANE ( 'NONE',  #39554 ) ;
#8717=CARTESIAN_POINT ( 'NONE',  ( -14.61616047585631151, 0.000000000000000000, 5.814656994489392439 ) ) ;
#8718=VECTOR ( 'NONE', #44570, 1000.000000000000227 ) ;
#8719=EDGE_LOOP ( 'NONE', ( #24315, #30733, #2582, #42175 ) ) ;
#8720=DIRECTION ( 'NONE',  ( 0.005002170337468016433, -0.7660444431189770143, -0.6427681459581293666 ) ) ;
#8721=ORIENTED_EDGE ( 'NONE', *, *, #30895, .T. ) ;
#8722=LINE ( 'NONE', #3326, #27704 ) ;
#8723=VECTOR ( 'NONE', #344, 1000.000000000000227 ) ;
#8724=ORIENTED_EDGE ( 'NONE', *, *, #3203, .F. ) ;
#8725=AXIS2_PLACEMENT_3D ( 'NONE', #54815, #6298, #54267 ) ;
#8726=VERTEX_POINT ( 'NONE', #45605 ) ;
#8727=ORIENTED_EDGE ( 'NONE', *, *, #12704, .T. ) ;
#8728=AXIS2_PLACEMENT_3D ( 'NONE', #14003, #5479, #40113 ) ;
#8729=ORIENTED_EDGE ( 'NONE', *, *, #45254, .F. ) ;
#8730=VECTOR ( 'NONE', #7833, 1000.000000000000000 ) ;
#8731=VERTEX_POINT ( 'NONE', #24320 ) ;
#8732=EDGE_LOOP ( 'NONE', ( #41591, #33045, #42578, #36819 ) ) ;
#8733=DIRECTION ( 'NONE',  ( 0.007781995580012663651, 0.000000000000000000, -0.9999697198139515519 ) ) ;
#8734=FACE_OUTER_BOUND ( 'NONE', #1468, .T. ) ;
#8735=CARTESIAN_POINT ( 'NONE',  ( -18.52672451560416178, -0.1191753592594156363, 9.946879876886450589 ) ) ;
#8736=VECTOR ( 'NONE', #31084, 1000.000000000000000 ) ;
#8737=VECTOR ( 'NONE', #2692, 1000.000000000000114 ) ;
#8738=EDGE_LOOP ( 'NONE', ( #43371, #13469, #16977, #50736 ) ) ;
#8739=DIRECTION ( 'NONE',  ( -0.005002170337468016433, -0.7660444431189770143, 0.6427681459581293666 ) ) ;
#8740=EDGE_CURVE ( 'NONE', #54423, #55875, #41627, .T. ) ;
#8741=ORIENTED_EDGE ( 'NONE', *, *, #19180, .T. ) ;
#8742=ORIENTED_EDGE ( 'NONE', *, *, #22753, .T. ) ;
#8743=VECTOR ( 'NONE', #10805, 1000.000000000000227 ) ;
#8744=VECTOR ( 'NONE', #41895, 1000.000000000000227 ) ;
#8745=PLANE ( 'NONE',  #5836 ) ;
#8746=LINE ( 'NONE', #30020, #49547 ) ;
#8747=ORIENTED_EDGE ( 'NONE', *, *, #29596, .F. ) ;
#8749=ORIENTED_EDGE ( 'NONE', *, *, #28103, .F. ) ;
#8750=ADVANCED_FACE ( 'NONE', ( #54989 ), #37357, .F. ) ;
#8751=CARTESIAN_POINT ( 'NONE',  ( -19.12962290826653700, 0.000000000000000000, 14.40064212555863854 ) ) ;
#8752=DIRECTION ( 'NONE',  ( 0.005961354470445682716, -0.6427876096865404731, -0.7660212471507180654 ) ) ;
#8753=EDGE_CURVE ( 'NONE', #55515, #23328, #53181, .T. ) ;
#8754=EDGE_CURVE ( 'NONE', #48148, #53080, #52338, .T. ) ;
#8755=AXIS2_PLACEMENT_3D ( 'NONE', #43885, #4998, #51835 ) ;
#8756=DIRECTION ( 'NONE',  ( -0.9321478471874540261, 0.000000000000000000, 0.3620778797217457656 ) ) ;
#8757=CARTESIAN_POINT ( 'NONE',  ( -15.86710544311044302, 0.000000000000000000, 13.13336954653252953 ) ) ;
#8759=CARTESIAN_POINT ( 'NONE',  ( -17.29614092396359126, -0.1191753592594168992, 4.785807585647434692 ) ) ;
#8760=DIRECTION ( 'NONE',  ( -0.5364919789714478471, 0.6444004775717705469, -0.5449076811759709926 ) ) ;
#8762=EDGE_LOOP ( 'NONE', ( #38245, #27201, #20780, #43137 ) ) ;
#8763=LINE ( 'NONE', #30624, #27437 ) ;
#8764=VECTOR ( 'NONE', #17064, 999.9999999999998863 ) ;
#8765=LINE ( 'NONE', #42541, #51015 ) ;
#8766=CARTESIAN_POINT ( 'NONE',  ( -23.33771345073609638, -0.1191753592594197858, 5.846786880686956955 ) ) ;
#8767=EDGE_CURVE ( 'NONE', #43300, #9606, #22518, .T. ) ;
#8768=VECTOR ( 'NONE', #18240, 999.9999999999998863 ) ;
#8769=CARTESIAN_POINT ( 'NONE',  ( -27.06552663992790997, 0.000000000000000000, 7.195101427592543786 ) ) ;
#8770=CARTESIAN_POINT ( 'NONE',  ( -13.47827057769550585, 0.000000000000000000, 4.715516107368122434 ) ) ;
#8771=PLANE ( 'NONE',  #34956 ) ;
#8772=ADVANCED_FACE ( 'NONE', ( #26764 ), #48057, .F. ) ;
#8773=DIRECTION ( 'NONE',  ( 0.000000000000000000, -1.000000000000000000, 0.000000000000000000 ) ) ;
#8774=VECTOR ( 'NONE', #29722, 999.9999999999998863 ) ;
#8775=PLANE ( 'NONE',  #4860 ) ;
#8776=PRODUCT_CONTEXT ( 'NONE', #26081, 'mechanical' ) ;
#8777=ORIENTED_EDGE ( 'NONE', *, *, #47036, .F. ) ;
#8778=CARTESIAN_POINT ( 'NONE',  ( -20.04530058363958389, -1.165603555308155626, 6.381161231016116986 ) ) ;
#8779=CARTESIAN_POINT ( 'NONE',  ( -18.67775241435682432, 0.000000000000000000, 4.136394454059623804 ) ) ;
#8780=LINE ( 'NONE', #30053, #42689 ) ;
#8781=ADVANCED_FACE ( 'NONE', ( #1182 ), #27051, .F. ) ;
#8782=AXIS2_PLACEMENT_3D ( 'NONE', #48955, #43566, #26521 ) ;
#8783=PLANE ( 'NONE',  #18229 ) ;
#8784=LINE ( 'NONE', #21248, #24891 ) ;
#8785=DIRECTION ( 'NONE',  ( 0.007781995580012663651, -3.146120232559066537E-19, -0.9999697198139514409 ) ) ;
#8787=VECTOR ( 'NONE', #9322, 1000.000000000000227 ) ;
#8788=EDGE_CURVE ( 'NONE', #37046, #54767, #13441, .T. ) ;
#8789=AXIS2_PLACEMENT_3D ( 'NONE', #9226, #35360, #4692 ) ;
#8790=CARTESIAN_POINT ( 'NONE',  ( -22.40634380310664397, 0.000000000000000000, 5.584705972946605534 ) ) ;
#8791=CARTESIAN_POINT ( 'NONE',  ( -10.74029228357944987, 0.000000000000000000, 11.14194120806293320 ) ) ;
#8792=ORIENTED_EDGE ( 'NONE', *, *, #13650, .T. ) ;
#8793=DIRECTION ( 'NONE',  ( -0.5449076811759708816, 0.6444004775717707689, 0.5364919789714475140 ) ) ;
#8794=ORIENTED_EDGE ( 'NONE', *, *, #38562, .T. ) ;
#8795=VECTOR ( 'NONE', #48834, 1000.000000000000227 ) ;
#8796=ORIENTED_EDGE ( 'NONE', *, *, #12125, .T. ) ;
#8799=ORIENTED_EDGE ( 'NONE', *, *, #24102, .T. ) ;
#8800=DIRECTION ( 'NONE',  ( 0.5364919789714477361, 0.6444004775717706579, 0.5449076811759711036 ) ) ;
#8801=DIRECTION ( 'NONE',  ( 0.000000000000000000, -1.000000000000000000, 0.000000000000000000 ) ) ;
#8802=AXIS2_PLACEMENT_3D ( 'NONE', #33977, #37956, #51299 ) ;
#8803=VERTEX_POINT ( 'NONE', #39825 ) ;
#8804=EDGE_CURVE ( 'NONE', #3505, #30407, #25429, .T. ) ;
#8805=AXIS2_PLACEMENT_3D ( 'NONE', #9944, #845, #47505 ) ;
#8806=ADVANCED_FACE ( 'NONE', ( #348 ), #4904, .F. ) ;
#8807=CARTESIAN_POINT ( 'NONE',  ( -15.86710544311044302, 0.000000000000000000, 13.13336954653252953 ) ) ;
#8808=ORIENTED_EDGE ( 'NONE', *, *, #36036, .F. ) ;
#8810=CARTESIAN_POINT ( 'NONE',  ( -16.75527768274136875, 0.000000000000000000, 7.844676295016960843 ) ) ;
#8812=ORIENTED_EDGE ( 'NONE', *, *, #28786, .F. ) ;
#8813=CARTESIAN_POINT ( 'NONE',  ( -10.74029228357944987, 0.000000000000000000, 11.14194120806293320 ) ) ;
#8814=EDGE_CURVE ( 'NONE', #41178, #13383, #10001, .T. ) ;
#8815=ADVANCED_FACE ( 'NONE', ( #29723 ), #26467, .F. ) ;
#8816=EDGE_CURVE ( 'NONE', #49529, #19075, #47020, .T. ) ;
#8817=ORIENTED_EDGE ( 'NONE', *, *, #2561, .T. ) ;
#8820=CARTESIAN_POINT ( 'NONE',  ( -28.93060053386082231, -0.1191753592594197858, 8.019254159017428663 ) ) ;
#8822=ORIENTED_EDGE ( 'NONE', *, *, #2857, .F. ) ;
#8823=LINE ( 'NONE', #21841, #11331 ) ;
#8824=FACE_OUTER_BOUND ( 'NONE', #8225, .T. ) ;
#8825=DIRECTION ( 'NONE',  ( -0.005002170337468016433, -0.7660444431189770143, 0.6427681459581293666 ) ) ;
#8826=DIRECTION ( 'NONE',  ( 0.5364919789714477361, 0.6444004775717706579, 0.5449076811759711036 ) ) ;
#8827=ORIENTED_EDGE ( 'NONE', *, *, #1850, .T. ) ;
#8829=LINE ( 'NONE', #38332, #21026 ) ;
#8830=FACE_OUTER_BOUND ( 'NONE', #11920, .T. ) ;
#8831=LINE ( 'NONE', #3429, #33060 ) ;
#8832=EDGE_CURVE ( 'NONE', #41466, #23008, #52867, .T. ) ;
#8833=DIRECTION ( 'NONE',  ( -0.9999697198139514409, -0.000000000000000000, -0.007781995580013368816 ) ) ;
#8834=CARTESIAN_POINT ( 'NONE',  ( -13.63673279712320507, -0.1191753592594197858, 12.22739664767016521 ) ) ;
#8835=PLANE ( 'NONE',  #20374 ) ;
#8836=CARTESIAN_POINT ( 'NONE',  ( -8.875996589204540044, 0.000000000000000000, 10.41778544861944233 ) ) ;
#8837=EDGE_CURVE ( 'NONE', #11293, #51591, #35557, .T. ) ;
#8838=CARTESIAN_POINT ( 'NONE',  ( -11.27023153255588284, -0.1191753592594177180, 6.679362954920378570 ) ) ;
#8839=LINE ( 'NONE', #26143, #16817 ) ;
#8841=EDGE_CURVE ( 'NONE', #21438, #55768, #9745, .T. ) ;
#8842=DIRECTION ( 'NONE',  ( 0.5364919789714477361, 0.6444004775717706579, 0.5449076811759711036 ) ) ;
#8843=ORIENTED_EDGE ( 'NONE', *, *, #27748, .F. ) ;
#8844=DIRECTION ( 'NONE',  ( -0.8531650599175527594, 0.4028455766673922356, 0.3313982828793700652 ) ) ;
#8845=DIRECTION ( 'NONE',  ( -0.5364919789714478471, 0.6444004775717705469, -0.5449076811759709926 ) ) ;
#8846=ADVANCED_FACE ( 'NONE', ( #44360 ), #8125, .F. ) ;
#8847=CARTESIAN_POINT ( 'NONE',  ( -29.86197018149027116, 0.000000000000000000, 8.281335066757780083 ) ) ;
#8848=LINE ( 'NONE', #39188, #7888 ) ;
#8849=CARTESIAN_POINT ( 'NONE',  ( -14.10280672071693431, -0.1191753592594197858, 12.40843558753103792 ) ) ;
#8850=ORIENTED_EDGE ( 'NONE', *, *, #10807, .T. ) ;
#8851=VECTOR ( 'NONE', #28230, 1000.000000000000227 ) ;
#8852=ORIENTED_EDGE ( 'NONE', *, *, #33743, .F. ) ;
#8853=LINE ( 'NONE', #43463, #24090 ) ;
#8854=DIRECTION ( 'NONE',  ( 0.8531650599175527594, 0.4028455766673922356, -0.3313982828793700652 ) ) ;
#8855=ORIENTED_EDGE ( 'NONE', *, *, #37906, .T. ) ;
#8856=CARTESIAN_POINT ( 'NONE',  ( -14.46888367232926420, 0.000000000000000000, 12.59025272694991315 ) ) ;
#8857=AXIS2_PLACEMENT_3D ( 'NONE', #46722, #3560, #55506 ) ;
#8858=ORIENTED_EDGE ( 'NONE', *, *, #52601, .T. ) ;
#8859=CARTESIAN_POINT ( 'NONE',  ( -19.91360065290022519, -5.375054281893163477, 13.23843028808050981 ) ) ;
#8860=ORIENTED_EDGE ( 'NONE', *, *, #49996, .T. ) ;
#8861=FACE_OUTER_BOUND ( 'NONE', #55273, .T. ) ;
#8862=VERTEX_POINT ( 'NONE', #31600 ) ;
#8863=ORIENTED_EDGE ( 'NONE', *, *, #16499, .F. ) ;
#8864=ORIENTED_EDGE ( 'NONE', *, *, #11237, .T. ) ;
#8865=FACE_OUTER_BOUND ( 'NONE', #3686, .T. ) ;
#8866=CARTESIAN_POINT ( 'NONE',  ( -12.33850799832341849, 0.000000000000000000, 11.68350162852954632 ) ) ;
#8867=DIRECTION ( 'NONE',  ( 0.9999697198139515519, 0.000000000000000000, 0.007781995580013368816 ) ) ;
#8868=FACE_OUTER_BOUND ( 'NONE', #53846, .T. ) ;
#8869=ORIENTED_EDGE ( 'NONE', *, *, #42354, .F. ) ;
#8870=EDGE_CURVE ( 'NONE', #31757, #25455, #5742, .T. ) ;
#8871=ORIENTED_EDGE ( 'NONE', *, *, #28830, .F. ) ;
#8872=EDGE_LOOP ( 'NONE', ( #26246, #26589, #9553, #44748 ) ) ;
#8873=EDGE_CURVE ( 'NONE', #14416, #54500, #31856, .T. ) ;
#8874=CARTESIAN_POINT ( 'NONE',  ( -18.66354898467281132, 0.000000000000000000, 14.21960318569776582 ) ) ;
#8875=EDGE_LOOP ( 'NONE', ( #9908, #53592, #49225, #388 ) ) ;
#8877=VERTEX_POINT ( 'NONE', #45208 ) ;
#8878=FACE_OUTER_BOUND ( 'NONE', #29743, .T. ) ;
#8879=CARTESIAN_POINT ( 'NONE',  ( -11.87243407472968926, 0.000000000000000000, 11.50246268866867361 ) ) ;
#8880=EDGE_CURVE ( 'NONE', #1004, #40111, #7147, .T. ) ;
#8881=EDGE_CURVE ( 'NONE', #24619, #50967, #49993, .T. ) ;
#8882=EDGE_CURVE ( 'NONE', #37125, #23998, #23888, .T. ) ;
#8883=ORIENTED_EDGE ( 'NONE', *, *, #44777, .F. ) ;
#8884=DIRECTION ( 'NONE',  ( 0.9999697198139515519, 0.000000000000000000, 0.007781995580013368816 ) ) ;
#8885=ORIENTED_EDGE ( 'NONE', *, *, #20979, .F. ) ;
#8886=ADVANCED_FACE ( 'NONE', ( #50287 ), #6575, .F. ) ;
#8887=VECTOR ( 'NONE', #42559, 1000.000000000000000 ) ;
#8888=CARTESIAN_POINT ( 'NONE',  ( -21.97156659400807044, 4.819660872929010687, 13.32570833076115946 ) ) ;
#8889=ORIENTED_EDGE ( 'NONE', *, *, #53359, .T. ) ;
#8890=CARTESIAN_POINT ( 'NONE',  ( -9.956977639035045513, 0.000000000000000000, 4.204261539843453299 ) ) ;
#8891=LINE ( 'NONE', #52320, #42014 ) ;
#8892=LINE ( 'NONE', #48041, #38247 ) ;
#8893=VERTEX_POINT ( 'NONE', #15635 ) ;
#8894=LINE ( 'NONE', #8598, #11126 ) ;
#8895=AXIS2_PLACEMENT_3D ( 'NONE', #44998, #19963, #54586 ) ;
#8896=DIRECTION ( 'NONE',  ( 0.000000000000000000, -1.000000000000000000, 0.000000000000000000 ) ) ;
#8897=DIRECTION ( 'NONE',  ( -0.6427681459581293666, -0.7660444431189770143, -0.005002170337467561935 ) ) ;
#8898=DIRECTION ( 'NONE',  ( 0.5449076811759707706, 0.6444004775717708799, -0.5364919789714476250 ) ) ;
#8899=DIRECTION ( 'NONE',  ( -0.6246952433987894571, 0.7422098413412802076, 0.2426528472758539834 ) ) ;
#8900=DIRECTION ( 'NONE',  ( -0.2426528472758542054, 0.7422098413412800966, -0.6246952433987894571 ) ) ;
#8901=EDGE_CURVE ( 'NONE', #13096, #21986, #36393, .T. ) ;
#8902=DIRECTION ( 'NONE',  ( 0.9999697198139515519, 0.000000000000000000, 0.007781995580013368816 ) ) ;
#8903=ORIENTED_EDGE ( 'NONE', *, *, #40879, .T. ) ;
#8904=DIRECTION ( 'NONE',  ( -0.005961354470445682716, -0.6427876096865404731, 0.7660212471507180654 ) ) ;
#8906=EDGE_CURVE ( 'NONE', #14383, #54636, #53444, .T. ) ;
#8907=DIRECTION ( 'NONE',  ( 0.5364919789714477361, 0.6444004775717706579, 0.5449076811759711036 ) ) ;
#8908=ORIENTED_EDGE ( 'NONE', *, *, #36382, .T. ) ;
#8909=LINE ( 'NONE', #21929, #3933 ) ;
#8910=ORIENTED_EDGE ( 'NONE', *, *, #11620, .F. ) ;
#8911=PLANE ( 'NONE',  #47949 ) ;
#8912=ADVANCED_FACE ( 'NONE', ( #45744 ), #2311, .F. ) ;
#8913=LINE ( 'NONE', #5464, #42060 ) ;
#8914=CARTESIAN_POINT ( 'NONE',  ( -21.47341775636118655, -0.1191753592594197858, 5.122631121243466090 ) ) ;
#8915=EDGE_CURVE ( 'NONE', #34779, #35810, #27607, .T. ) ;
#8916=LINE ( 'NONE', #22523, #4804 ) ;
#8917=ORIENTED_EDGE ( 'NONE', *, *, #51725, .T. ) ;
#8918=ORIENTED_EDGE ( 'NONE', *, *, #36572, .T. ) ;
#8919=DIRECTION ( 'NONE',  ( 0.007781995580012663651, 0.000000000000000000, -0.9999697198139515519 ) ) ;
#8920=LINE ( 'NONE', #31609, #28633 ) ;
#8921=DIRECTION ( 'NONE',  ( 0.007781995580012662783, 0.000000000000000000, -0.9999697198139514409 ) ) ;
#8922=CARTESIAN_POINT ( 'NONE',  ( -26.13493519185646008, 0.000000000000000000, 7.033017491833586377 ) ) ;
#8923=CARTESIAN_POINT ( 'NONE',  ( -22.40556560354864146, -0.1191753592594197858, 5.484709000965211523 ) ) ;
#8924=CARTESIAN_POINT ( 'NONE',  ( -15.40600537535590142, -3.917936722690661178, 9.096149048148156169 ) ) ;
#8925=ORIENTED_EDGE ( 'NONE', *, *, #46253, .T. ) ;
#8926=CARTESIAN_POINT ( 'NONE',  ( -18.39746900504187010, 0.000000000000000000, 14.03700784672088808 ) ) ;
#8929=CARTESIAN_POINT ( 'NONE',  ( -15.10091574723437802, 0.000000000000000000, 8.396209005525733460 ) ) ;
#8930=DIRECTION ( 'NONE',  ( 0.5449076811759707706, 0.6444004775717708799, -0.5364919789714476250 ) ) ;
#8931=CARTESIAN_POINT ( 'NONE',  ( -12.13851405436063047, 0.000000000000000000, 11.68505802764555135 ) ) ;
#8932=ORIENTED_EDGE ( 'NONE', *, *, #40884, .F. ) ;
#8933=VECTOR ( 'NONE', #25019, 999.9999999999998863 ) ;
#8934=CARTESIAN_POINT ( 'NONE',  ( -19.22961988024793101, -0.1191753592594177458, 14.39986392600063603 ) ) ;
#8935=ORIENTED_EDGE ( 'NONE', *, *, #7006, .F. ) ;
#8936=ORIENTED_EDGE ( 'NONE', *, *, #44246, .T. ) ;
#8937=ORIENTED_EDGE ( 'NONE', *, *, #29156, .T. ) ;
#8938=EDGE_LOOP ( 'NONE', ( #29865, #52081, #53566, #15654 ) ) ;
#8939=DIRECTION ( 'NONE',  ( 0.000000000000000000, -1.000000000000000000, 0.000000000000000000 ) ) ;
#8942=EDGE_CURVE ( 'NONE', #53450, #21341, #19347, .T. ) ;
#8944=DIRECTION ( 'NONE',  ( -0.6427681459581293666, -0.7660444431189770143, -0.005002170337467561935 ) ) ;
#8946=DIRECTION ( 'NONE',  ( 0.007781995580012663651, -3.146120232559066537E-19, -0.9999697198139514409 ) ) ;
#8948=EDGE_CURVE ( 'NONE', #2320, #45947, #19647, .T. ) ;
#8949=EDGE_CURVE ( 'NONE', #49206, #9950, #49168, .T. ) ;
#8950=PLANE ( 'NONE',  #1184 ) ;
#8951=CARTESIAN_POINT ( 'NONE',  ( -17.59067451224156642, 1.905425754524006532, 3.453954036298156005 ) ) ;
#8952=LINE ( 'NONE', #47257, #50326 ) ;
#8953=DIRECTION ( 'NONE',  ( -0.9999697198139514409, -0.000000000000000000, -0.007781995580013368816 ) ) ;
#8954=LINE ( 'NONE', #26255, #46441 ) ;
#8955=ORIENTED_EDGE ( 'NONE', *, *, #28545, .F. ) ;
#8956=ORIENTED_EDGE ( 'NONE', *, *, #53156, .F. ) ;
#8957=CARTESIAN_POINT ( 'NONE',  ( -9.771353962598668730, 0.000000000000000000, 6.052366455248280097 ) ) ;
#8958=CARTESIAN_POINT ( 'NONE',  ( -11.32921355590532109, 0.000000000000000000, 1.408251937772285300 ) ) ;
#8959=CARTESIAN_POINT ( 'NONE',  ( -15.95701152500570608, -0.03739765774599677212, 3.018190368296854498 ) ) ;
#8960=DIRECTION ( 'NONE',  ( -0.5364919789714478471, 0.6444004775717705469, -0.5449076811759709926 ) ) ;
#8961=CARTESIAN_POINT ( 'NONE',  ( 2.072287782118878319, 0.000000000000000000, -2.950529333540147015 ) ) ;
#8962=LINE ( 'NONE', #52397, #30485 ) ;
#8964=DIRECTION ( 'NONE',  ( 0.5364919789714477361, 0.6444004775717706579, 0.5449076811759711036 ) ) ;
#8967=AXIS2_PLACEMENT_3D ( 'NONE', #8059, #3770, #34189 ) ;
#8968=FACE_OUTER_BOUND ( 'NONE', #12976, .T. ) ;
#8970=CARTESIAN_POINT ( 'NONE',  ( -12.09873015469866253, 0.000000000000000000, 6.572912358960970813 ) ) ;
#8971=EDGE_CURVE ( 'NONE', #35486, #11724, #23613, .T. ) ;
#8972=DIRECTION ( 'NONE',  ( 0.9999697198139515519, 0.000000000000000000, 0.007781995580013368816 ) ) ;
#8973=DIRECTION ( 'NONE',  ( 0.5364919789714477361, 0.6444004775717706579, 0.5449076811759711036 ) ) ;
#8974=EDGE_LOOP ( 'NONE', ( #4960, #8088, #41504 ) ) ;
#8975=ADVANCED_FACE ( 'NONE', ( #6044 ), #19907, .F. ) ;
#8976=VERTEX_POINT ( 'NONE', #36143 ) ;
#8977=CARTESIAN_POINT ( 'NONE',  ( -14.00280974873554030, 0.000000000000000000, 12.40921378708904044 ) ) ;
#8978=DIRECTION ( 'NONE',  ( 0.5364919789714477361, 0.6444004775717706579, 0.5449076811759711036 ) ) ;
#8979=DIRECTION ( 'NONE',  ( 0.5364919789714477361, 0.6444004775717706579, 0.5449076811759711036 ) ) ;
#8980=FACE_OUTER_BOUND ( 'NONE', #25387, .T. ) ;
#8981=ADVANCED_FACE ( 'NONE', ( #15370 ), #36684, .F. ) ;
#8984=PLANE ( 'NONE',  #28397 ) ;
#8985=ORIENTED_EDGE ( 'NONE', *, *, #9455, .T. ) ;
#8986=LINE ( 'NONE', #26287, #30520 ) ;
#8987=DIRECTION ( 'NONE',  ( 0.007781995580012662783, 0.000000000000000000, -0.9999697198139514409 ) ) ;
#8988=VERTEX_POINT ( 'NONE', #1748 ) ;
#8989=DIRECTION ( 'NONE',  ( 0.005961354470445682716, -0.6427876096865404731, -0.7660212471507180654 ) ) ;
#8993=CARTESIAN_POINT ( 'NONE',  ( -20.54049170961573267, 0.000000000000000000, 4.660556269540326646 ) ) ;
#8995=VERTEX_POINT ( 'NONE', #19070 ) ;
#8996=EDGE_LOOP ( 'NONE', ( #615, #32549, #31545, #48006 ) ) ;
#8997=VERTEX_POINT ( 'NONE', #14821 ) ;
#8998=ORIENTED_EDGE ( 'NONE', *, *, #16462, .F. ) ;
#9000=DIRECTION ( 'NONE',  ( -0.5449076811759708816, 0.6444004775717707689, 0.5364919789714475140 ) ) ;
#9001=DIRECTION ( 'NONE',  ( -0.9999697198139514409, -0.000000000000000000, -0.007781995580013368816 ) ) ;
#9002=EDGE_CURVE ( 'NONE', #2126, #44201, #32149, .T. ) ;
#9003=PLANE ( 'NONE',  #26743 ) ;
#9004=VERTEX_POINT ( 'NONE', #37814 ) ;
#9005=CARTESIAN_POINT ( 'NONE',  ( -8.063280706518755281, 0.000000000000000000, 6.234985089866581731 ) ) ;
#9006=VERTEX_POINT ( 'NONE', #3440 ) ;
#9007=ORIENTED_EDGE ( 'NONE', *, *, #23512, .T. ) ;
#9008=ADVANCED_FACE ( 'NONE', ( #51125 ), #34384, .F. ) ;
#9010=DIRECTION ( 'NONE',  ( -0.7660212471507179544, -0.6427876096865405842, -0.005961354470445141482 ) ) ;
#9011=DIRECTION ( 'NONE',  ( 0.9999697198139515519, 0.000000000000000000, 0.007781995580013368816 ) ) ;
#9012=VERTEX_POINT ( 'NONE', #34112 ) ;
#9013=CARTESIAN_POINT ( 'NONE',  ( -16.95814568020944435, 0.000000000000000000, 8.212429599158721061 ) ) ;
#9014=ORIENTED_EDGE ( 'NONE', *, *, #2184, .F. ) ;
#9015=DIRECTION ( 'NONE',  ( 0.005002170337468016433, -0.7660444431189770143, -0.6427681459581293666 ) ) ;
#9016=CARTESIAN_POINT ( 'NONE',  ( -15.40103151951671734, 0.000000000000000000, 12.95233060667165681 ) ) ;
#9017=ADVANCED_FACE ( 'NONE', ( #29849 ), #54828, .F. ) ;
#9018=CARTESIAN_POINT ( 'NONE',  ( -14.46888367232926420, 0.000000000000000000, 12.59025272694991315 ) ) ;
#9019=CARTESIAN_POINT ( 'NONE',  ( -17.28938333041720554, 2.067327705546507133, 6.989941716411668615 ) ) ;
#9020=CARTESIAN_POINT ( 'NONE',  ( -13.69838289619527494, 0.000000000000000000, 7.299127631056469667 ) ) ;
#9022=DIRECTION ( 'NONE',  ( 0.6246952433987893460, 0.7422098413412802076, -0.2426528472758539279 ) ) ;
#9024=ORIENTED_EDGE ( 'NONE', *, *, #20232, .F. ) ;
#9025=DIRECTION ( 'NONE',  ( 0.007781995580012663651, 0.000000000000000000, -0.9999697198139515519 ) ) ;
#9026=DIRECTION ( 'NONE',  ( 0.000000000000000000, -0.000000000000000000, -1.000000000000000000 ) ) ;
#9027=CARTESIAN_POINT ( 'NONE',  ( -20.06177075545399191, 0.000000000000000000, 14.76272000528038220 ) ) ;
#9028=CARTESIAN_POINT ( 'NONE',  ( -8.318202594104366909, -8.005327475259342407, 0.01269879923549658424 ) ) ;
#9029=CARTESIAN_POINT ( 'NONE',  ( 2.072287782118878319, 0.000000000000000000, -2.950529333540147015 ) ) ;
#9030=DIRECTION ( 'NONE',  ( -0.6427681459581293666, -0.7660444431189770143, -0.005002170337467561935 ) ) ;
#9031=FACE_OUTER_BOUND ( 'NONE', #2109, .T. ) ;
#9032=CARTESIAN_POINT ( 'NONE',  ( -27.99923088623136636, 0.000000000000000000, 7.757173251277078130 ) ) ;
#9033=ORIENTED_EDGE ( 'NONE', *, *, #12521, .F. ) ;
#9034=DIRECTION ( 'NONE',  ( 0.007781995580012662783, 0.000000000000000000, -0.9999697198139514409 ) ) ;
#9035=PLANE ( 'NONE',  #3164 ) ;
#9036=DIRECTION ( 'NONE',  ( 0.005961354470445682716, -0.6427876096865404731, -0.7660212471507180654 ) ) ;
#9038=DIRECTION ( 'NONE',  ( -0.9999697198139514409, -0.000000000000000000, -0.007781995580013368816 ) ) ;
#9039=EDGE_CURVE ( 'NONE', #21762, #23836, #2842, .T. ) ;
#9040=LINE ( 'NONE', #13317, #33036 ) ;
#9042=DIRECTION ( 'NONE',  ( 0.5449076811759707706, 0.6444004775717708799, -0.5364919789714476250 ) ) ;
#9043=DIRECTION ( 'NONE',  ( -0.2426528472758542054, 0.7422098413412800966, -0.6246952433987894571 ) ) ;
#9044=EDGE_LOOP ( 'NONE', ( #16926, #18672, #23571, #3270 ) ) ;
#9045=DIRECTION ( 'NONE',  ( 0.9999697198139515519, 0.000000000000000000, 0.007781995580013368816 ) ) ;
#9046=EDGE_CURVE ( 'NONE', #56189, #17210, #51687, .T. ) ;
#9047=EDGE_LOOP ( 'NONE', ( #54406, #54994, #35135, #38059 ) ) ;
#9048=EDGE_CURVE ( 'NONE', #18658, #11310, #12531, .T. ) ;
#9050=VERTEX_POINT ( 'NONE', #42885 ) ;
#9052=ORIENTED_EDGE ( 'NONE', *, *, #26458, .T. ) ;
#9053=ORIENTED_EDGE ( 'NONE', *, *, #25183, .T. ) ;
#9054=LINE ( 'NONE', #51917, #12423 ) ;
#9056=FACE_OUTER_BOUND ( 'NONE', #2396, .T. ) ;
#9057=EDGE_LOOP ( 'NONE', ( #32793, #41873, #28124, #16894 ) ) ;
#9058=EDGE_CURVE ( 'NONE', #10554, #3178, #21321, .T. ) ;
#9059=EDGE_LOOP ( 'NONE', ( #51760, #45692, #22280, #48158 ) ) ;
#9060=EDGE_CURVE ( 'NONE', #54876, #34978, #16778, .T. ) ;
#9061=FACE_OUTER_BOUND ( 'NONE', #34598, .T. ) ;
#9062=ORIENTED_EDGE ( 'NONE', *, *, #107, .T. ) ;
#9064=CARTESIAN_POINT ( 'NONE',  ( -15.88130887279446490, 0.000000000000000000, 3.050160814894388839 ) ) ;
#9065=VERTEX_POINT ( 'NONE', #3701 ) ;
#9066=DIRECTION ( 'NONE',  ( 0.005002170337468016433, -0.7660444431189770143, -0.6427681459581293666 ) ) ;
#9067=ADVANCED_FACE ( 'NONE', ( #33810 ), #7993, .F. ) ;
#9068=ORIENTED_EDGE ( 'NONE', *, *, #9896, .T. ) ;
#9069=LINE ( 'NONE', #42586, #1918 ) ;
#9070=ADVANCED_FACE ( 'NONE', ( #12792 ), #25303, .F. ) ;
#9071=DIRECTION ( 'NONE',  ( 0.5449076811759707706, 0.6444004775717708799, -0.5364919789714476250 ) ) ;
#9072=FACE_OUTER_BOUND ( 'NONE', #12106, .T. ) ;
#9073=ORIENTED_EDGE ( 'NONE', *, *, #14413, .T. ) ;
#9074=DIRECTION ( 'NONE',  ( -0.5364919789714478471, 0.6444004775717705469, -0.5449076811759709926 ) ) ;
#9075=DIRECTION ( 'NONE',  ( -0.7660212471507179544, -0.6427876096865405842, -0.005961354470445141482 ) ) ;
#9076=CARTESIAN_POINT ( 'NONE',  ( 0.000000000000000000, -1.000000000000000000, 2.125000000000000000 ) ) ;
#9078=LINE ( 'NONE', #30679, #47375 ) ;
#9079=EDGE_LOOP ( 'NONE', ( #41764, #30926, #43119, #51582 ) ) ;
#9080=CARTESIAN_POINT ( 'NONE',  ( -13.17065887352947762, -0.1191753592594197858, 12.04635770780929427 ) ) ;
#9081=CARTESIAN_POINT ( 'NONE',  ( -10.40568786923371469, 0.000000000000000000, 2.154103167823834042 ) ) ;
#9083=DIRECTION ( 'NONE',  ( 0.007781995580012663651, 0.000000000000000000, -0.9999697198139515519 ) ) ;
#9085=CARTESIAN_POINT ( 'NONE',  ( -16.33317936670417225, 0.000000000000000000, 13.31440848639340224 ) ) ;
#9086=CARTESIAN_POINT ( 'NONE',  ( -11.70612789434414402, -0.1191753592594183703, 2.982650010574726451 ) ) ;
#9087=CARTESIAN_POINT ( 'NONE',  ( -13.07066190154808361, 0.000000000000000000, 12.04713590736729678 ) ) ;
#9088=DIRECTION ( 'NONE',  ( 0.5449076811759707706, 0.6444004775717708799, -0.5364919789714476250 ) ) ;
#9089=VERTEX_POINT ( 'NONE', #20172 ) ;
#9090=DIRECTION ( 'NONE',  ( 0.9999697198139515519, 0.000000000000000000, 0.007781995580013368816 ) ) ;
#9091=FACE_OUTER_BOUND ( 'NONE', #215, .T. ) ;
#9092=DIRECTION ( 'NONE',  ( 0.000000000000000000, -1.000000000000000000, 0.000000000000000000 ) ) ;
#9093=CARTESIAN_POINT ( 'NONE',  ( -9.568213099748072992, 0.000000000000000000, 2.360626646347695257 ) ) ;
#9094=EDGE_CURVE ( 'NONE', #35036, #13331, #20757, .T. ) ;
#9095=DIRECTION ( 'NONE',  ( -0.005961354470445682716, -0.6427876096865404731, 0.7660212471507180654 ) ) ;
#9096=CARTESIAN_POINT ( 'NONE',  ( -17.93139508144814442, 0.000000000000000000, 13.85596890686001537 ) ) ;
#9097=VERTEX_POINT ( 'NONE', #38072 ) ;
#9098=VECTOR ( 'NONE', #19163, 999.9999999999998863 ) ;
#9099=ORIENTED_EDGE ( 'NONE', *, *, #55382, .F. ) ;
#9100=PLANE ( 'NONE',  #45858 ) ;
#9101=CARTESIAN_POINT ( 'NONE',  ( -13.12303101290966545, -0.1191753592594181482, 5.926279901332813793 ) ) ;
#9102=EDGE_LOOP ( 'NONE', ( #43894, #7159, #32465, #48009 ) ) ;
#9103=EDGE_CURVE ( 'NONE', #40648, #14557, #7399, .T. ) ;
#9104=EDGE_CURVE ( 'NONE', #4182, #29456, #3145, .T. ) ;
#9105=DIRECTION ( 'NONE',  ( 0.000000000000000000, -0.000000000000000000, -1.000000000000000000 ) ) ;
#9106=VERTEX_POINT ( 'NONE', #46579 ) ;
#9107=DIRECTION ( 'NONE',  ( 0.005961354470445682716, -0.6427876096865404731, -0.7660212471507180654 ) ) ;
#9108=ORIENTED_EDGE ( 'NONE', *, *, #44510, .T. ) ;
#9109=DIRECTION ( 'NONE',  ( 0.5449076811759707706, 0.6444004775717708799, -0.5364919789714476250 ) ) ;
#9110=EDGE_CURVE ( 'NONE', #26525, #44524, #7698, .T. ) ;
#9111=ORIENTED_EDGE ( 'NONE', *, *, #20318, .T. ) ;
#9112=VERTEX_POINT ( 'NONE', #26992 ) ;
#9113=ORIENTED_EDGE ( 'NONE', *, *, #54915, .T. ) ;
#9114=DIRECTION ( 'NONE',  ( 0.005961354470445682716, -0.6427876096865404731, -0.7660212471507180654 ) ) ;
#9116=CARTESIAN_POINT ( 'NONE',  ( -10.27421835998572064, 0.000000000000000000, 10.96090226820206048 ) ) ;
#9117=CARTESIAN_POINT ( 'NONE',  ( -20.84899999561040573, -2.137015261443159009, 4.911598775153488639 ) ) ;
#9118=ADVANCED_FACE ( 'NONE', ( #5137 ), #39488, .F. ) ;
#9119=EDGE_LOOP ( 'NONE', ( #24399, #24303, #18799, #44028 ) ) ;
#9120=ORIENTED_EDGE ( 'NONE', *, *, #28862, .T. ) ;
#9121=EDGE_CURVE ( 'NONE', #18181, #51395, #43455, .T. ) ;
#9122=PLANE ( 'NONE',  #15508 ) ;
#9123=ORIENTED_EDGE ( 'NONE', *, *, #21047, .F. ) ;
#9124=CARTESIAN_POINT ( 'NONE',  ( -18.23403687816160712, -0.1191753592594172323, 5.886504871884708834 ) ) ;
#9125=ORIENTED_EDGE ( 'NONE', *, *, #37405, .F. ) ;
#9126=FACE_OUTER_BOUND ( 'NONE', #20305, .T. ) ;
#9127=CARTESIAN_POINT ( 'NONE',  ( -30.79567442779373110, 0.000000000000000000, 8.843406890442315316 ) ) ;
#9128=EDGE_CURVE ( 'NONE', #46056, #44974, #40026, .T. ) ;
#9129=EDGE_LOOP ( 'NONE', ( #24949, #23083, #19995, #46392 ) ) ;
#9130=VECTOR ( 'NONE', #10820, 1000.000000000000227 ) ;
#9131=DIRECTION ( 'NONE',  ( 0.5364919789714477361, 0.6444004775717706579, 0.5449076811759711036 ) ) ;
#9132=VERTEX_POINT ( 'NONE', #48848 ) ;
#9133=VECTOR ( 'NONE', #55671, 999.9999999999998863 ) ;
#9134=CARTESIAN_POINT ( 'NONE',  ( -18.59215049645273510, 0.000000000000000000, 5.045050781177780941 ) ) ;
#9136=LINE ( 'NONE', #48613, #33110 ) ;
#9137=DIRECTION ( 'NONE',  ( 0.9999697198139515519, 0.000000000000000000, 0.007781995580013368816 ) ) ;
#9138=LINE ( 'NONE', #39811, #21020 ) ;
#9139=ORIENTED_EDGE ( 'NONE', *, *, #21364, .T. ) ;
#9140=CARTESIAN_POINT ( 'NONE',  ( -15.88053067323646417, -0.1191753592594197858, 2.950163842912994383 ) ) ;
#9141=CARTESIAN_POINT ( 'NONE',  ( -13.08486533123210194, 0.000000000000000000, 1.963927175729152541 ) ) ;
#9142=PLANE ( 'NONE',  #22194 ) ;
#9144=FACE_OUTER_BOUND ( 'NONE', #9059, .T. ) ;
#9145=DIRECTION ( 'NONE',  ( 0.000000000000000000, 0.000000000000000000, -1.000000000000000000 ) ) ;
#9146=PRESENTATION_STYLE_ASSIGNMENT (( #26459 ) ) ;
#9147=ORIENTED_EDGE ( 'NONE', *, *, #30358, .F. ) ;
#9148=CARTESIAN_POINT ( 'NONE',  ( -26.13493519185646008, 0.000000000000000000, 7.033017491833586377 ) ) ;
#9149=PLANE ( 'NONE',  #493 ) ;
#9150=CARTESIAN_POINT ( 'NONE',  ( -17.93139508144814442, 0.000000000000000000, 13.85596890686001537 ) ) ;
#9151=ORIENTED_EDGE ( 'NONE', *, *, #22186, .F. ) ;
#9152=DIRECTION ( 'NONE',  ( -0.6427681459581293666, -0.7660444431189770143, -0.005002170337467561935 ) ) ;
#9153=CARTESIAN_POINT ( 'NONE',  ( -19.59569683186026268, 0.000000000000000000, 14.58168106541950948 ) ) ;
#9154=ORIENTED_EDGE ( 'NONE', *, *, #4706, .T. ) ;
#9155=ADVANCED_FACE ( 'NONE', ( #26691 ), #5403, .F. ) ;
#9156=DIRECTION ( 'NONE',  ( 0.6427681459581294776, -0.7660444431189769032, 0.005002170337467562802 ) ) ;
#9157=VECTOR ( 'NONE', #40642, 1000.000000000000114 ) ;
#9158=DIRECTION ( 'NONE',  ( 0.000000000000000000, -1.000000000000000000, 0.000000000000000000 ) ) ;
#9159=EDGE_CURVE ( 'NONE', #23847, #3660, #271, .T. ) ;
#9160=PLANE ( 'NONE',  #4244 ) ;
#9162=VERTEX_POINT ( 'NONE', #26147 ) ;
#9163=VERTEX_POINT ( 'NONE', #35237 ) ;
#9164=ADVANCED_FACE ( 'NONE', ( #9091 ), #22459, .F. ) ;
#9165=LINE ( 'NONE', #9451, #11303 ) ;
#9166=CARTESIAN_POINT ( 'NONE',  ( -22.40634380310664397, 0.000000000000000000, 5.584705972946605534 ) ) ;
#9167=LINE ( 'NONE', #12330, #52285 ) ;
#9168=EDGE_CURVE ( 'NONE', #36770, #24378, #44013, .T. ) ;
#9169=ADVANCED_FACE ( 'NONE', ( #4552 ), #9677, .F. ) ;
#9170=EDGE_CURVE ( 'NONE', #5706, #6357, #35489, .T. ) ;
#9172=DIRECTION ( 'NONE',  ( 0.000000000000000000, -1.000000000000000000, 0.000000000000000000 ) ) ;
#9173=VECTOR ( 'NONE', #43690, 1000.000000000000227 ) ;
#9174=DIRECTION ( 'NONE',  ( -0.005002170337468016433, -0.7660444431189770143, 0.6427681459581293666 ) ) ;
#9176=EDGE_CURVE ( 'NONE', #37711, #42922, #30409, .T. ) ;
#9177=CARTESIAN_POINT ( 'NONE',  ( -19.32961685222932147, 0.000000000000000000, 14.39908572644263351 ) ) ;
#9178=AXIS2_PLACEMENT_3D ( 'NONE', #8468, #4768, #25797 ) ;
#9179=FACE_OUTER_BOUND ( 'NONE', #24666, .T. ) ;
#9180=VERTEX_POINT ( 'NONE', #21865 ) ;
#9182=DIRECTION ( 'NONE',  ( 0.7660212471507180654, -0.6427876096865404731, 0.005961354470445141482 ) ) ;
#9183=CARTESIAN_POINT ( 'NONE',  ( -17.18829999102435124, 0.000000000000000000, 3.778653647413541261 ) ) ;
#9184=ORIENTED_EDGE ( 'NONE', *, *, #5299, .T. ) ;
#9185=LINE ( 'NONE', #18254, #13074 ) ;
#9186=ADVANCED_FACE ( 'NONE', ( #39767 ), #17614, .F. ) ;
#9187=ORIENTED_EDGE ( 'NONE', *, *, #11569, .T. ) ;
#9188=EDGE_CURVE ( 'NONE', #50536, #14368, #34954, .T. ) ;
#9190=ORIENTED_EDGE ( 'NONE', *, *, #12247, .T. ) ;
#9191=EDGE_CURVE ( 'NONE', #55170, #547, #4299, .T. ) ;
#9192=ORIENTED_EDGE ( 'NONE', *, *, #20954, .F. ) ;
#9193=CARTESIAN_POINT ( 'NONE',  ( -15.68624088420942542, -3.756034771668162797, 2.854552609374020999 ) ) ;
#9194=EDGE_LOOP ( 'NONE', ( #31975, #8812, #51814, #6619 ) ) ;
#9196=VECTOR ( 'NONE', #3075, 1000.000000000000227 ) ;
#9197=EDGE_CURVE ( 'NONE', #34282, #49846, #25870, .T. ) ;
#9198=VECTOR ( 'NONE', #39997, 1000.000000000000227 ) ;
#9199=ORIENTED_EDGE ( 'NONE', *, *, #9176, .F. ) ;
#9200=PLANE ( 'NONE',  #51300 ) ;
#9201=VERTEX_POINT ( 'NONE', #48561 ) ;
#9202=FACE_OUTER_BOUND ( 'NONE', #52144, .T. ) ;
#9203=VERTEX_POINT ( 'NONE', #26400 ) ;
#9204=EDGE_CURVE ( 'NONE', #4025, #6097, #43716, .T. ) ;
#9205=DIRECTION ( 'NONE',  ( 0.007781995580012662783, 0.000000000000000000, -0.9999697198139514409 ) ) ;
#9206=PLANE ( 'NONE',  #7831 ) ;
#9207=CARTESIAN_POINT ( 'NONE',  ( 1.086233639165236964, 0.000000000000000000, 2.796443541562362078 ) ) ;
#9208=FACE_OUTER_BOUND ( 'NONE', #9391, .T. ) ;
#9209=DIRECTION ( 'NONE',  ( 0.9999697198139515519, 0.000000000000000000, 0.007781995580013368816 ) ) ;
#9210=VERTEX_POINT ( 'NONE', #4832 ) ;
#9211=ORIENTED_EDGE ( 'NONE', *, *, #1371, .F. ) ;
#9212=LINE ( 'NONE', #8676, #444 ) ;
#9213=CARTESIAN_POINT ( 'NONE',  ( -12.80458192191714595, 0.000000000000000000, 11.86454056839041726 ) ) ;
#9214=AXIS2_PLACEMENT_3D ( 'NONE', #39988, #5099, #23258 ) ;
#9215=DIRECTION ( 'NONE',  ( -0.9999697198139514409, -0.000000000000000000, -0.007781995580013368816 ) ) ;
#9216=CARTESIAN_POINT ( 'NONE',  ( -18.86354292863559579, 0.000000000000000000, 14.21804678658176080 ) ) ;
#9217=CARTESIAN_POINT ( 'NONE',  ( 2.072287782118878319, 0.000000000000000000, -2.950529333540147015 ) ) ;
#9218=LINE ( 'NONE', #26533, #42261 ) ;
#9219=VERTEX_POINT ( 'NONE', #45396 ) ;
#9220=DIRECTION ( 'NONE',  ( -0.6427681459581293666, -0.7660444431189770143, -0.005002170337467561935 ) ) ;
#9221=DIRECTION ( 'NONE',  ( 0.007781995580012663651, -3.146120232559066537E-19, -0.9999697198139514409 ) ) ;
#9222=ORIENTED_EDGE ( 'NONE', *, *, #20271, .T. ) ;
#9223=LINE ( 'NONE', #48406, #44265 ) ;
#9225=CARTESIAN_POINT ( 'NONE',  ( -10.87319881958008772, 0.000000000000000000, 2.519796959313588491 ) ) ;
#9226=CARTESIAN_POINT ( 'NONE',  ( -20.06177075545399191, 0.000000000000000000, 14.76272000528038220 ) ) ;
#9227=DIRECTION ( 'NONE',  ( 0.6427681459581294776, -0.7660444431189769032, 0.005002170337467562802 ) ) ;
#9228=EDGE_LOOP ( 'NONE', ( #45859, #4232, #21048, #35363 ) ) ;
#9229=ORIENTED_EDGE ( 'NONE', *, *, #7382, .F. ) ;
#9230=LINE ( 'NONE', #48719, #17591 ) ;
#9231=PLANE ( 'NONE',  #11360 ) ;
#9232=PLANE ( 'NONE',  #30617 ) ;
#9233=ADVANCED_FACE ( 'NONE', ( #44854 ), #6508, .F. ) ;
#9234=ADVANCED_FACE ( 'NONE', ( #32624 ), #41149, .F. ) ;
#9235=AXIS2_PLACEMENT_3D ( 'NONE', #50721, #3315, #28297 ) ;
#9236=VECTOR ( 'NONE', #52017, 999.9999999999998863 ) ;
#9240=DIRECTION ( 'NONE',  ( 0.007781995580012663651, -3.146120232559066537E-19, -0.9999697198139514409 ) ) ;
#9241=LINE ( 'NONE', #43597, #5712 ) ;
#9242=PLANE ( 'NONE',  #25036 ) ;
#9243=PLANE ( 'NONE',  #7908 ) ;
#9244=VECTOR ( 'NONE', #9240, 1000.000000000000227 ) ;
#9246=DIRECTION ( 'NONE',  ( -0.5364919789714478471, 0.6444004775717705469, -0.5449076811759709926 ) ) ;
#9247=VERTEX_POINT ( 'NONE', #23818 ) ;
#9248=LINE ( 'NONE', #34821, #15056 ) ;
#9249=PLANE ( 'NONE',  #24793 ) ;
#9250=ORIENTED_EDGE ( 'NONE', *, *, #204, .T. ) ;
#9251=VECTOR ( 'NONE', #28268, 999.9999999999998863 ) ;
#9252=ORIENTED_EDGE ( 'NONE', *, *, #13380, .T. ) ;
#9253=VECTOR ( 'NONE', #32039, 1000.000000000000227 ) ;
#9254=ORIENTED_EDGE ( 'NONE', *, *, #3282, .F. ) ;
#9255=ORIENTED_EDGE ( 'NONE', *, *, #11419, .T. ) ;
#9256=EDGE_LOOP ( 'NONE', ( #27414, #43559, #33986, #38953 ) ) ;
#9257=ORIENTED_EDGE ( 'NONE', *, *, #53010, .F. ) ;
#9258=LINE ( 'NONE', #30296, #28613 ) ;
#9259=DIRECTION ( 'NONE',  ( 0.005961354470445682716, -0.6427876096865404731, -0.7660212471507180654 ) ) ;
#9260=CARTESIAN_POINT ( 'NONE',  ( -9.984210658517920223, 9.723509473712979911, 7.096580060653336020 ) ) ;
#9262=CARTESIAN_POINT ( 'NONE',  ( -14.41041842488296076, 0.000000000000000000, 5.077593987089866090 ) ) ;
#9263=EDGE_LOOP ( 'NONE', ( #39020, #43140, #8483, #23922 ) ) ;
#9264=ORIENTED_EDGE ( 'NONE', *, *, #31546, .F. ) ;
#9265=ADVANCED_FACE ( 'NONE', ( #49686 ), #32081, .F. ) ;
#9266=CARTESIAN_POINT ( 'NONE',  ( 2.072287782118878319, 0.000000000000000000, -2.950529333540147015 ) ) ;
#9267=EDGE_CURVE ( 'NONE', #33602, #43397, #18758, .T. ) ;
#9268=DIRECTION ( 'NONE',  ( -0.9999697198139514409, -0.000000000000000000, -0.007781995580013368816 ) ) ;
#9269=LINE ( 'NONE', #9861, #50427 ) ;
#9270=VECTOR ( 'NONE', #20397, 1000.000000000000227 ) ;
#9271=ADVANCED_FACE ( 'NONE', ( #36915 ), #53925, .F. ) ;
#9272=ORIENTED_EDGE ( 'NONE', *, *, #39715, .F. ) ;
#9273=FACE_OUTER_BOUND ( 'NONE', #53647, .T. ) ;
#9274=ORIENTED_EDGE ( 'NONE', *, *, #28972, .F. ) ;
#9275=VECTOR ( 'NONE', #24522, 1000.000000000000227 ) ;
#9276=AXIS2_PLACEMENT_3D ( 'NONE', #9931, #40597, #10766 ) ;
#9277=EDGE_CURVE ( 'NONE', #9097, #42364, #54215, .T. ) ;
#9278=DIRECTION ( 'NONE',  ( 0.9999697198139515519, 0.000000000000000000, 0.007781995580013368816 ) ) ;
#9279=DIRECTION ( 'NONE',  ( 0.000000000000000000, -0.000000000000000000, -1.000000000000000000 ) ) ;
#9280=VECTOR ( 'NONE', #34819, 1000.000000000000227 ) ;
#9281=VECTOR ( 'NONE', #7682, 999.9999999999998863 ) ;
#9282=CARTESIAN_POINT ( 'NONE',  ( -28.92982233430281980, 0.000000000000000000, 7.919257187036034651 ) ) ;
#9283=LINE ( 'NONE', #26604, #33960 ) ;
#9285=CARTESIAN_POINT ( 'NONE',  ( -7.930221204654489320, 7.733889655832618892, 6.298740802997315313 ) ) ;
#9286=LINE ( 'NONE', #1323, #39516 ) ;
#9287=EDGE_LOOP ( 'NONE', ( #17646, #38656, #21828, #30524 ) ) ;
#9288=LINE ( 'NONE', #43929, #30200 ) ;
#9290=DIRECTION ( 'NONE',  ( -0.9999697198139514409, -0.000000000000000000, -0.007781995580013368816 ) ) ;
#9291=FACE_OUTER_BOUND ( 'NONE', #22558, .T. ) ;
#9294=DIRECTION ( 'NONE',  ( -0.7660212471507179544, -0.6427876096865405842, -0.005961354470445141482 ) ) ;
#9295=CARTESIAN_POINT ( 'NONE',  ( -12.07286367315112052, 0.000000000000000000, 3.249125029641091178 ) ) ;
#9296=CARTESIAN_POINT ( 'NONE',  ( -11.05155405620451958, -1.003701604285656579, 2.621975966892176046 ) ) ;
#9297=ORIENTED_EDGE ( 'NONE', *, *, #51275, .T. ) ;
#9298=CARTESIAN_POINT ( 'NONE',  ( 1.086233639165236964, 0.000000000000000000, 2.796443541562362078 ) ) ;
#9300=DIRECTION ( 'NONE',  ( 0.007781995580012662783, 0.000000000000000000, -0.9999697198139514409 ) ) ;
#9301=ADVANCED_FACE ( 'NONE', ( #10780 ), #10515, .F. ) ;
#9302=CARTESIAN_POINT ( 'NONE',  ( -13.43195515176800292, 0.2864062442990031321, 1.890221404860171539 ) ) ;
#9303=DIRECTION ( 'NONE',  ( 0.7660212471507180654, -0.6427876096865404731, 0.005961354470445141482 ) ) ;
#9304=VECTOR ( 'NONE', #18599, 999.9999999999998863 ) ;
#9305=DIRECTION ( 'NONE',  ( 0.9999697198139515519, 0.000000000000000000, 0.007781995580013368816 ) ) ;
#9307=EDGE_CURVE ( 'NONE', #42767, #49508, #28091, .T. ) ;
#9308=LINE ( 'NONE', #26632, #51908 ) ;
#9309=DIRECTION ( 'NONE',  ( 0.000000000000000000, 0.000000000000000000, 1.000000000000000000 ) ) ;
#9310=AXIS2_PLACEMENT_3D ( 'NONE', #6069, #37242, #32700 ) ;
#9311=CARTESIAN_POINT ( 'NONE',  ( -17.74482636761137044, -0.1191753592594197858, 3.674319602356483916 ) ) ;
#9312=VECTOR ( 'NONE', #38018, 1000.000000000000000 ) ;
#9313=VECTOR ( 'NONE', #47075, 1000.000000000000227 ) ;
#9314=ORIENTED_EDGE ( 'NONE', *, *, #55186, .F. ) ;
#9315=EDGE_CURVE ( 'NONE', #36994, #28691, #49929, .T. ) ;
#9316=AXIS2_PLACEMENT_3D ( 'NONE', #45032, #5844, #28240 ) ;
#9317=ORIENTED_EDGE ( 'NONE', *, *, #21870, .F. ) ;
#9318=EDGE_LOOP ( 'NONE', ( #8645, #18320, #8042, #5236 ) ) ;
#9319=VECTOR ( 'NONE', #34027, 999.9999999999998863 ) ;
#9320=EDGE_LOOP ( 'NONE', ( #23931, #34160, #26154, #53874 ) ) ;
#9321=ORIENTED_EDGE ( 'NONE', *, *, #19660, .F. ) ;
#9322=DIRECTION ( 'NONE',  ( 0.007781995580012662783, 0.000000000000000000, -0.9999697198139514409 ) ) ;
#9323=PLANE ( 'NONE',  #53018 ) ;
#9324=VERTEX_POINT ( 'NONE', #11035 ) ;
#9325=ORIENTED_EDGE ( 'NONE', *, *, #53860, .F. ) ;
#9326=AXIS2_PLACEMENT_3D ( 'NONE', #18995, #6230, #27818 ) ;
#9327=VECTOR ( 'NONE', #9704, 999.9999999999998863 ) ;
#9328=FACE_OUTER_BOUND ( 'NONE', #8719, .T. ) ;
#9330=DIRECTION ( 'NONE',  ( 0.005002170337468016433, -0.7660444431189770143, -0.6427681459581293666 ) ) ;
#9331=DIRECTION ( 'NONE',  ( -0.5364919789714478471, 0.6444004775717705469, -0.5449076811759709926 ) ) ;
#9332=ORIENTED_EDGE ( 'NONE', *, *, #40781, .T. ) ;
#9333=PLANE ( 'NONE',  #274 ) ;
#9334=AXIS2_PLACEMENT_3D ( 'NONE', #44280, #39744, #16526 ) ;
#9336=CARTESIAN_POINT ( 'NONE',  ( -15.88053067323646417, -0.1191753592594197858, 2.950163842912994383 ) ) ;
#9337=EDGE_CURVE ( 'NONE', #30427, #24462, #28354, .T. ) ;
#9338=VECTOR ( 'NONE', #1189, 999.9999999999998863 ) ;
#9339=PLANE ( 'NONE',  #33822 ) ;
#9340=DIRECTION ( 'NONE',  ( -0.5364919789714478471, 0.6444004775717705469, -0.5449076811759709926 ) ) ;
#9341=CARTESIAN_POINT ( 'NONE',  ( -22.40478740399063895, 0.000000000000000000, 5.384712028983816623 ) ) ;
#9342=ORIENTED_EDGE ( 'NONE', *, *, #43484, .T. ) ;
#9343=LINE ( 'NONE', #5383, #43079 ) ;
#9344=CARTESIAN_POINT ( 'NONE',  ( -11.40636015113596180, 0.000000000000000000, 11.32142374880780089 ) ) ;
#9345=DIRECTION ( 'NONE',  ( -0.3620778797217455991, 0.000000000000000000, -0.9321478471874540261 ) ) ;
#9346=VECTOR ( 'NONE', #25048, 1000.000000000000227 ) ;
#9347=ORIENTED_EDGE ( 'NONE', *, *, #36689, .T. ) ;
#9348=LINE ( 'NONE', #29831, #11975 ) ;
#9349=ORIENTED_EDGE ( 'NONE', *, *, #40428, .F. ) ;
#9350=ADVANCED_FACE ( 'NONE', ( #24117 ), #49104, .F. ) ;
#9351=AXIS2_PLACEMENT_3D ( 'NONE', #6492, #23799, #54736 ) ;
#9352=VECTOR ( 'NONE', #27964, 1000.000000000000227 ) ;
#9353=FACE_OUTER_BOUND ( 'NONE', #45790, .T. ) ;
#9354=CARTESIAN_POINT ( 'NONE',  ( -11.21901323774118708, 0.000000000000000000, 1.039777472322872098 ) ) ;
#9356=DIRECTION ( 'NONE',  ( 0.9999697198139515519, 0.000000000000000000, 0.007781995580013368816 ) ) ;
#9357=CARTESIAN_POINT ( 'NONE',  ( -13.55892737469792309, -0.1191753592594191197, 2.229566956987161230 ) ) ;
#9358=EDGE_CURVE ( 'NONE', #2279, #47606, #40615, .T. ) ;
#9359=CARTESIAN_POINT ( 'NONE',  ( -4.802685646341279480, -6.704367417419401676, 5.083899780593831963 ) ) ;
#9360=DIRECTION ( 'NONE',  ( -0.005002170337468016433, -0.7660444431189770143, 0.6427681459581293666 ) ) ;
#9361=EDGE_CURVE ( 'NONE', #36569, #5010, #42813, .T. ) ;
#9362=VECTOR ( 'NONE', #54549, 999.9999999999998863 ) ;
#9363=CARTESIAN_POINT ( 'NONE',  ( -12.40300812230242045, 1.257817950434005461, 3.763364223827011745 ) ) ;
#9364=AXIS2_PLACEMENT_3D ( 'NONE', #36392, #14820, #10588 ) ;
#9365=CARTESIAN_POINT ( 'NONE',  ( -12.29585004515617186, 0.000000000000000000, 6.202046256587205875 ) ) ;
#9366=EDGE_LOOP ( 'NONE', ( #32895, #36444, #51302, #38631 ) ) ;
#9367=CARTESIAN_POINT ( 'NONE',  ( -17.93139508144814442, 0.000000000000000000, 13.85596890686001537 ) ) ;
#9369=EDGE_CURVE ( 'NONE', #50871, #394, #3073, .T. ) ;
#9370=CARTESIAN_POINT ( 'NONE',  ( -22.07924021441773377, 3.362543313726510164, 5.150975708369738726 ) ) ;
#9371=CARTESIAN_POINT ( 'NONE',  ( -14.56888064431065821, -0.1191753592594197858, 12.58947452739191064 ) ) ;
#9372=EDGE_CURVE ( 'NONE', #13435, #48572, #16709, .T. ) ;
#9373=PLANE ( 'NONE',  #8260 ) ;
#9374=VECTOR ( 'NONE', #3261, 1000.000000000000114 ) ;
#9375=DIRECTION ( 'NONE',  ( 0.5364919789714477361, 0.6444004775717706579, 0.5449076811759711036 ) ) ;
#9376=EDGE_CURVE ( 'NONE', #48014, #32968, #34039, .T. ) ;
#9377=LINE ( 'NONE', #22717, #11116 ) ;
#9378=ORIENTED_EDGE ( 'NONE', *, *, #19048, .T. ) ;
#9379=EDGE_LOOP ( 'NONE', ( #5876, #8031, #4897, #20875 ) ) ;
#9380=DIRECTION ( 'NONE',  ( 0.007781995580012663651, 0.000000000000000000, -0.9999697198139515519 ) ) ;
#9381=LINE ( 'NONE', #36344, #42214 ) ;
#9382=VECTOR ( 'NONE', #15167, 999.9999999999998863 ) ;
#9383=EDGE_CURVE ( 'NONE', #20306, #21351, #55317, .T. ) ;
#9384=ORIENTED_EDGE ( 'NONE', *, *, #12093, .T. ) ;
#9385=CARTESIAN_POINT ( 'NONE',  ( -14.94838282604900748, -0.1191753592594197858, 2.588085963191248506 ) ) ;
#9386=VECTOR ( 'NONE', #19358, 999.9999999999998863 ) ;
#9387=EDGE_LOOP ( 'NONE', ( #5558, #42314, #48215, #29695 ) ) ;
#9388=CARTESIAN_POINT ( 'NONE',  ( -19.47222345087960704, -3.270328918600661439, 4.340653370440049841 ) ) ;
#9389=ADVANCED_FACE ( 'NONE', ( #46819 ), #24650, .F. ) ;
#9391=EDGE_LOOP ( 'NONE', ( #18919, #24214, #34637, #31822 ) ) ;
#9392=ORIENTED_EDGE ( 'NONE', *, *, #849, .T. ) ;
#9393=FACE_OUTER_BOUND ( 'NONE', #3218, .T. ) ;
#9394=AXIS2_PLACEMENT_3D ( 'NONE', #22871, #40194, #30839 ) ;
#9395=LINE ( 'NONE', #15, #18703 ) ;
#9396=CARTESIAN_POINT ( 'NONE',  ( -19.77031582249948016, 4.495856970884011261, 4.217952423934554496 ) ) ;
#9397=VECTOR ( 'NONE', #40720, 999.9999999999998863 ) ;
#9398=VECTOR ( 'NONE', #21717, 999.9999999999998863 ) ;
#9399=FACE_OUTER_BOUND ( 'NONE', #15601, .T. ) ;
#9400=ORIENTED_EDGE ( 'NONE', *, *, #16222, .T. ) ;
#9401=ORIENTED_EDGE ( 'NONE', *, *, #9267, .F. ) ;
#9402=VECTOR ( 'NONE', #39921, 1000.000000000000227 ) ;
#9403=AXIS2_PLACEMENT_3D ( 'NONE', #24114, #37164, #54213 ) ;
#9404=CARTESIAN_POINT ( 'NONE',  ( -13.19793970290151641, 0.000000000000000000, 2.701711344436330098 ) ) ;
#9405=ORIENTED_EDGE ( 'NONE', *, *, #23320, .T. ) ;
#9406=CARTESIAN_POINT ( 'NONE',  ( -17.68960728864125898, 4.172053068839008283, 10.59961518480473508 ) ) ;
#9407=EDGE_LOOP ( 'NONE', ( #34536, #30595, #8310, #51335 ) ) ;
#9408=CARTESIAN_POINT ( 'NONE',  ( -16.06709938707323460, 0.000000000000000000, 13.13181314741652628 ) ) ;
#9409=LINE ( 'NONE', #27026, #44849 ) ;
#9410=EDGE_LOOP ( 'NONE', ( #1133, #26358, #28326, #11702 ) ) ;
#9411=CARTESIAN_POINT ( 'NONE',  ( -16.06709938707323460, 0.000000000000000000, 13.13181314741652628 ) ) ;
#9412=EDGE_CURVE ( 'NONE', #44511, #18621, #38276, .T. ) ;
#9413=EDGE_LOOP ( 'NONE', ( #26384, #9392, #12048, #21940 ) ) ;
#9414=LINE ( 'NONE', #5441, #41780 ) ;
#9415=VECTOR ( 'NONE', #687, 999.9999999999998863 ) ;
#9416=ORIENTED_EDGE ( 'NONE', *, *, #34002, .T. ) ;
#9417=DIRECTION ( 'NONE',  ( -0.2426528472758542054, 0.7422098413412800966, -0.6246952433987894571 ) ) ;
#9418=LINE ( 'NONE', #19627, #51138 ) ;
#9419=CARTESIAN_POINT ( 'NONE',  ( -18.67775241435682432, 0.000000000000000000, 4.136394454059623804 ) ) ;
#9420=ORIENTED_EDGE ( 'NONE', *, *, #21144, .F. ) ;
#9422=LINE ( 'NONE', #5189, #17505 ) ;
#9423=DIRECTION ( 'NONE',  ( 0.6427681459581294776, -0.7660444431189769032, 0.005002170337467562802 ) ) ;
#9424=CARTESIAN_POINT ( 'NONE',  ( -31.72704407542318350, -0.1191753592594197858, 9.105487798182664960 ) ) ;
#9425=AXIS2_PLACEMENT_3D ( 'NONE', #17242, #22638, #30869 ) ;
#9427=CARTESIAN_POINT ( 'NONE',  ( -12.62536516875885795, -0.1191753592594181482, 1.685747015088036482 ) ) ;
#9428=LINE ( 'NONE', #5195, #3441 ) ;
#9430=CARTESIAN_POINT ( 'NONE',  ( -17.37836304482322802, -5.213152330870664208, 3.465340642280367867 ) ) ;
#9431=ORIENTED_EDGE ( 'NONE', *, *, #11087, .T. ) ;
#9432=LINE ( 'NONE', #2006, #48851 ) ;
#9433=CARTESIAN_POINT ( 'NONE',  ( -22.40634380310664397, 0.000000000000000000, 5.584705972946605534 ) ) ;
#9434=DIRECTION ( 'NONE',  ( -0.9999697198139514409, -0.000000000000000000, -0.007781995580013368816 ) ) ;
#9435=ORIENTED_EDGE ( 'NONE', *, *, #21238, .F. ) ;
#9436=VECTOR ( 'NONE', #2608, 999.9999999999998863 ) ;
#9437=CARTESIAN_POINT ( 'NONE',  ( -10.74029228357944987, 0.000000000000000000, 11.14194120806293320 ) ) ;
#9438=CARTESIAN_POINT ( 'NONE',  ( -13.21964368434966630, -3.594132820645663084, 1.901608010842381624 ) ) ;
#9439=ORIENTED_EDGE ( 'NONE', *, *, #24307, .F. ) ;
#9441=CARTESIAN_POINT ( 'NONE',  ( -16.74665552222552733, 0.000000000000000000, 6.736747185243664227 ) ) ;
#9442=EDGE_CURVE ( 'NONE', #7497, #34473, #20402, .T. ) ;
#9443=FACE_OUTER_BOUND ( 'NONE', #15976, .T. ) ;
#9444=CARTESIAN_POINT ( 'NONE',  ( -12.13851405436063047, 0.000000000000000000, 11.68505802764555135 ) ) ;
#9445=EDGE_CURVE ( 'NONE', #2679, #5744, #11617, .T. ) ;
#9447=ORIENTED_EDGE ( 'NONE', *, *, #39769, .F. ) ;
#9448=AXIS2_PLACEMENT_3D ( 'NONE', #33417, #51294, #12409 ) ;
#9449=VECTOR ( 'NONE', #33411, 999.9999999999998863 ) ;
#9450=ORIENTED_EDGE ( 'NONE', *, *, #2491, .F. ) ;
#9451=CARTESIAN_POINT ( 'NONE',  ( -13.41816968106543939, -2.137015261443158565, 5.401210633846317499 ) ) ;
#9452=DIRECTION ( 'NONE',  ( -0.6427681459581293666, -0.7660444431189770143, -0.005002170337467561935 ) ) ;
#9454=DIRECTION ( 'NONE',  ( 0.9999697198139515519, 0.000000000000000000, 0.007781995580013368816 ) ) ;
#9455=EDGE_CURVE ( 'NONE', #44660, #46401, #38575, .T. ) ;
#9456=CARTESIAN_POINT ( 'NONE',  ( -12.15193928448664629, -0.1191753592594197858, 1.501852324026012209 ) ) ;
#9457=CARTESIAN_POINT ( 'NONE',  ( 2.072287782118878319, 0.000000000000000000, -2.950529333540147015 ) ) ;
#9458=VERTEX_POINT ( 'NONE', #3380 ) ;
#9459=CARTESIAN_POINT ( 'NONE',  ( -14.01701317841955508, 0.000000000000000000, 2.326005055450897085 ) ) ;
#9460=AXIS2_PLACEMENT_3D ( 'NONE', #20731, #42582, #39096 ) ;
#9461=EDGE_CURVE ( 'NONE', #50536, #30787, #55903, .T. ) ;
#9462=DIRECTION ( 'NONE',  ( 0.007781995580012663651, -3.146120232559066537E-19, -0.9999697198139514409 ) ) ;
#9463=ORIENTED_EDGE ( 'NONE', *, *, #20282, .T. ) ;
#9464=DIRECTION ( 'NONE',  ( 0.9321478471874540261, 0.000000000000000000, -0.3620778797217456546 ) ) ;
#9465=CARTESIAN_POINT ( 'NONE',  ( -11.40636015113596180, 0.000000000000000000, 11.32142374880780089 ) ) ;
#9466=VECTOR ( 'NONE', #37279, 999.9999999999998863 ) ;
#9467=DIRECTION ( 'NONE',  ( 0.9999697198139515519, 0.000000000000000000, 0.007781995580013368816 ) ) ;
#9468=EDGE_LOOP ( 'NONE', ( #50421, #27345, #51981, #2332 ) ) ;
#9469=LINE ( 'NONE', #26795, #5825 ) ;
#9470=EDGE_LOOP ( 'NONE', ( #50845, #2571, #40215, #46139 ) ) ;
#9471=ORIENTED_EDGE ( 'NONE', *, *, #33380, .F. ) ;
#9472=VERTEX_POINT ( 'NONE', #29791 ) ;
#9473=VECTOR ( 'NONE', #41362, 999.9999999999998863 ) ;
#9474=ORIENTED_EDGE ( 'NONE', *, *, #21577, .F. ) ;
#9475=VECTOR ( 'NONE', #45110, 1000.000000000000227 ) ;
#9476=CARTESIAN_POINT ( 'NONE',  ( -10.33233557835786698, -0.1191753592594185784, 5.578665668683107093 ) ) ;
#9477=ORIENTED_EDGE ( 'NONE', *, *, #46452, .T. ) ;
#9478=EDGE_CURVE ( 'NONE', #55415, #37296, #20102, .T. ) ;
#9479=CARTESIAN_POINT ( 'NONE',  ( -29.86197018149027116, 0.000000000000000000, 8.281335066757780083 ) ) ;
#9481=VECTOR ( 'NONE', #14131, 1000.000000000000227 ) ;
#9482=ORIENTED_EDGE ( 'NONE', *, *, #35865, .F. ) ;
#9483=DIRECTION ( 'NONE',  ( -0.6427681459581293666, -0.7660444431189770143, -0.005002170337467561935 ) ) ;
#9484=ORIENTED_EDGE ( 'NONE', *, *, #42603, .T. ) ;
#9485=LINE ( 'NONE', #43007, #31168 ) ;
#9486=ADVANCED_FACE ( 'NONE', ( #50778 ), #47087, .F. ) ;
#9487=EDGE_LOOP ( 'NONE', ( #45102, #8415, #2271, #17562 ) ) ;
#9488=VECTOR ( 'NONE', #50384, 999.9999999999998863 ) ;
#9489=DIRECTION ( 'NONE',  ( 0.005002170337468016433, -0.7660444431189770143, -0.6427681459581293666 ) ) ;
#9490=VECTOR ( 'NONE', #15322, 1000.000000000000227 ) ;
#9491=EDGE_CURVE ( 'NONE', #21366, #12842, #28660, .T. ) ;
#9492=CARTESIAN_POINT ( 'NONE',  ( -14.01623497886155256, -0.1191753592594197858, 2.226008083469502630 ) ) ;
#9493=DIRECTION ( 'NONE',  ( -0.5364919789714478471, 0.6444004775717705469, -0.5449076811759709926 ) ) ;
#9494=EDGE_CURVE ( 'NONE', #20216, #13812, #20951, .T. ) ;
#9496=LINE ( 'NONE', #26820, #16020 ) ;
#9497=LINE ( 'NONE', #39874, #10180 ) ;
#9498=ORIENTED_EDGE ( 'NONE', *, *, #37443, .F. ) ;
#9499=ADVANCED_FACE ( 'NONE', ( #29196 ), #15861, .F. ) ;
#9500=EDGE_CURVE ( 'NONE', #19178, #1128, #42278, .T. ) ;
#9501=EDGE_CURVE ( 'NONE', #31769, #17110, #5068, .T. ) ;
#9502=ORIENTED_EDGE ( 'NONE', *, *, #45300, .T. ) ;
#9503=CARTESIAN_POINT ( 'NONE',  ( -19.98761758609199291, 0.000000000000000000, 5.234196989836540581 ) ) ;
#9504=CARTESIAN_POINT ( 'NONE',  ( -9.908141408373387193, -0.1191753592594197858, 10.77908512878318703 ) ) ;
#9505=DIRECTION ( 'NONE',  ( -0.5364919789714478471, 0.6444004775717705469, -0.5449076811759709926 ) ) ;
#9506=AXIS2_PLACEMENT_3D ( 'NONE', #2167, #49043, #10145 ) ;
#9507=LINE ( 'NONE', #48395, #6758 ) ;
#9508=ORIENTED_EDGE ( 'NONE', *, *, #12919, .T. ) ;
#9509=VECTOR ( 'NONE', #38695, 999.9999999999998863 ) ;
#9511=DIRECTION ( 'NONE',  ( -0.5449076811759708816, 0.6444004775717707689, 0.5364919789714475140 ) ) ;
#9512=ORIENTED_EDGE ( 'NONE', *, *, #2591, .T. ) ;
#9513=PLANE ( 'NONE',  #44747 ) ;
#9514=DIRECTION ( 'NONE',  ( 0.007781995580012663651, -3.146120232559066537E-19, -0.9999697198139514409 ) ) ;
#9515=AXIS2_PLACEMENT_3D ( 'NONE', #15104, #6561, #24176 ) ;
#9516=ORIENTED_EDGE ( 'NONE', *, *, #7252, .F. ) ;
#9517=DIRECTION ( 'NONE',  ( 0.5449076811759707706, 0.6444004775717708799, -0.5364919789714476250 ) ) ;
#9518=CARTESIAN_POINT ( 'NONE',  ( -17.49314540066396617, -4.241740624735662379, 3.540919126638463421 ) ) ;
#9519=ADVANCED_FACE ( 'NONE', ( #56175 ), #47661, .F. ) ;
#9520=VECTOR ( 'NONE', #31778, 1000.000000000000227 ) ;
#9521=DIRECTION ( 'NONE',  ( 0.005961354470445682716, -0.6427876096865404731, -0.7660212471507180654 ) ) ;
#9522=PLANE ( 'NONE',  #39588 ) ;
#9523=ADVANCED_FACE ( 'NONE', ( #31166 ), #4235, .F. ) ;
#9524=DIRECTION ( 'NONE',  ( 0.000000000000000000, 1.000000000000000000, 0.000000000000000000 ) ) ;
#9525=ORIENTED_EDGE ( 'NONE', *, *, #11924, .T. ) ;
#9526=AXIS2_PLACEMENT_3D ( 'NONE', #10041, #23111, #36179 ) ;
#9527=AXIS2_PLACEMENT_3D ( 'NONE', #17381, #43508, #1476 ) ;
#9528=EDGE_LOOP ( 'NONE', ( #25202, #23896, #13197, #16758 ) ) ;
#9529=EDGE_CURVE ( 'NONE', #21349, #15160, #8780, .T. ) ;
#9530=VECTOR ( 'NONE', #49852, 1000.000000000000227 ) ;
#9531=AXIS2_PLACEMENT_3D ( 'NONE', #4728, #48153, #9562 ) ;
#9532=CARTESIAN_POINT ( 'NONE',  ( -13.07066190154808361, 0.000000000000000000, 12.04713590736729678 ) ) ;
#9533=CARTESIAN_POINT ( 'NONE',  ( 2.072287782118878319, 0.000000000000000000, -2.950529333540147015 ) ) ;
#9534=CARTESIAN_POINT ( 'NONE',  ( -13.53673582514181106, 0.000000000000000000, 12.22817484722816772 ) ) ;
#9535=VECTOR ( 'NONE', #7390, 1000.000000000000227 ) ;
#9536=ADVANCED_FACE ( 'NONE', ( #22395 ), #17853, .F. ) ;
#9537=CARTESIAN_POINT ( 'NONE',  ( -14.90247820238758969, 0.000000000000000000, 8.597759348604526508 ) ) ;
#9538=CARTESIAN_POINT ( 'NONE',  ( -18.67619601524082285, 0.000000000000000000, 3.936400510096834893 ) ) ;
#9539=ORIENTED_EDGE ( 'NONE', *, *, #42285, .F. ) ;
#9541=PLANE ( 'NONE',  #50120 ) ;
#9542=AXIS2_PLACEMENT_3D ( 'NONE', #36929, #18773, #44575 ) ;
#9543=CARTESIAN_POINT ( 'NONE',  ( -13.48114463120078810, 0.000000000000000000, 5.084825810625885900 ) ) ;
#9544=AXIS2_PLACEMENT_3D ( 'NONE', #1251, #18288, #36453 ) ;
#9545=LINE ( 'NONE', #26038, #20585 ) ;
#9546=ORIENTED_EDGE ( 'NONE', *, *, #12370, .F. ) ;
#9547=LINE ( 'NONE', #43060, #12979 ) ;
#9548=VERTEX_POINT ( 'NONE', #39423 ) ;
#9549=DIRECTION ( 'NONE',  ( 0.000000000000000000, -1.000000000000000000, 0.000000000000000000 ) ) ;
#9550=FACE_OUTER_BOUND ( 'NONE', #47521, .T. ) ;
#9551=ORIENTED_EDGE ( 'NONE', *, *, #50151, .T. ) ;
#9552=PLANE ( 'NONE',  #31763 ) ;
#9553=ORIENTED_EDGE ( 'NONE', *, *, #5717, .T. ) ;
#9554=AXIS2_PLACEMENT_3D ( 'NONE', #14363, #53788, #6658 ) ;
#9555=EDGE_LOOP ( 'NONE', ( #35974, #52410, #10910, #2544 ) ) ;
#9556=ORIENTED_EDGE ( 'NONE', *, *, #27613, .F. ) ;
#9557=LINE ( 'NONE', #17027, #43811 ) ;
#9558=EDGE_LOOP ( 'NONE', ( #38791, #44928, #15594 ) ) ;
#9559=VECTOR ( 'NONE', #36874, 999.9999999999998863 ) ;
#9560=ORIENTED_EDGE ( 'NONE', *, *, #3036, .T. ) ;
#9561=DIRECTION ( 'NONE',  ( -0.7660212471507179544, -0.6427876096865405842, -0.005961354470445141482 ) ) ;
#9562=DIRECTION ( 'NONE',  ( 0.6427681459581294776, -0.7660444431189769032, 0.005002170337467562802 ) ) ;
#9563=AXIS2_PLACEMENT_3D ( 'NONE', #56102, #30257, #8690 ) ;
#9564=ORIENTED_EDGE ( 'NONE', *, *, #16760, .T. ) ;
#9566=ORIENTED_EDGE ( 'NONE', *, *, #7537, .F. ) ;
#9567=CARTESIAN_POINT ( 'NONE',  ( -22.17952184443886665, 5.143464774974014553, 5.133107780287143207 ) ) ;
#9568=ORIENTED_EDGE ( 'NONE', *, *, #28877, .T. ) ;
#9569=AXIS2_PLACEMENT_3D ( 'NONE', #11595, #55043, #21222 ) ;
#9570=ORIENTED_EDGE ( 'NONE', *, *, #45670, .F. ) ;
#9571=VECTOR ( 'NONE', #40905, 999.9999999999998863 ) ;
#9572=EDGE_CURVE ( 'NONE', #12044, #32426, #26933, .T. ) ;
#9573=AXIS2_PLACEMENT_3D ( 'NONE', #9784, #25756, #23108 ) ;
#9574=CARTESIAN_POINT ( 'NONE',  ( -13.46677436367437686, 0.000000000000000000, 3.238277294337062795 ) ) ;
#9576=FACE_OUTER_BOUND ( 'NONE', #48150, .T. ) ;
#9577=CARTESIAN_POINT ( 'NONE',  ( -15.13495153988577968, 0.000000000000000000, 12.76973526769478084 ) ) ;
#9578=ORIENTED_EDGE ( 'NONE', *, *, #31248, .F. ) ;
#9579=CARTESIAN_POINT ( 'NONE',  ( -5.105985705592273050, 4.998162406247122824, 5.201711823720286176 ) ) ;
#9580=ORIENTED_EDGE ( 'NONE', *, *, #48216, .F. ) ;
#9581=AXIS2_PLACEMENT_3D ( 'NONE', #41894, #40807, #33128 ) ;
#9582=ADVANCED_FACE ( 'NONE', ( #30883 ), #43400, .F. ) ;
#9583=EDGE_CURVE ( 'NONE', #4850, #26435, #9610, .T. ) ;
#9584=AXIS2_PLACEMENT_3D ( 'NONE', #48525, #1376, #36302 ) ;
#9585=CARTESIAN_POINT ( 'NONE',  ( -17.89891568791274068, 0.000000000000000000, 9.682436588653759557 ) ) ;
#9586=EDGE_CURVE ( 'NONE', #29013, #3202, #52476, .T. ) ;
#9587=VECTOR ( 'NONE', #51775, 1000.000000000000114 ) ;
#9588=DIRECTION ( 'NONE',  ( 0.007781995580012663651, -3.146120232559066537E-19, -0.9999697198139514409 ) ) ;
#9589=AXIS2_PLACEMENT_3D ( 'NONE', #9433, #44083, #27047 ) ;
#9590=DIRECTION ( 'NONE',  ( 0.000000000000000000, -0.000000000000000000, -1.000000000000000000 ) ) ;
#9591=CARTESIAN_POINT ( 'NONE',  ( -18.80938876144721306, 0.000000000000000000, 7.259352601608363820 ) ) ;
#9593=DIRECTION ( 'NONE',  ( -0.5364919789714478471, 0.6444004775717705469, -0.5449076811759709926 ) ) ;
#9594=LINE ( 'NONE', #39949, #28597 ) ;
#9595=VERTEX_POINT ( 'NONE', #21806 ) ;
#9596=DIRECTION ( 'NONE',  ( 0.007781995580012662783, 0.000000000000000000, -0.9999697198139514409 ) ) ;
#9598=DIRECTION ( 'NONE',  ( 0.007781995580012663651, -3.146120232559066537E-19, -0.9999697198139514409 ) ) ;
#9599=CARTESIAN_POINT ( 'NONE',  ( -20.54204810873173415, 0.000000000000000000, 4.860550213503115558 ) ) ;
#9601=DIRECTION ( 'NONE',  ( -0.005002170337468016433, -0.7660444431189770143, 0.6427681459581293666 ) ) ;
#9602=DIRECTION ( 'NONE',  ( 0.007781995580012662783, 0.000000000000000000, -0.9999697198139514409 ) ) ;
#9603=VECTOR ( 'NONE', #35872, 1000.000000000000227 ) ;
#9604=DIRECTION ( 'NONE',  ( -0.6427681459581293666, -0.7660444431189770143, -0.005002170337467561935 ) ) ;
#9605=AXIS2_PLACEMENT_3D ( 'NONE', #31805, #48267, #17925 ) ;
#9606=VERTEX_POINT ( 'NONE', #52197 ) ;
#9607=EDGE_CURVE ( 'NONE', #12905, #53740, #48192, .T. ) ;
#9608=LINE ( 'NONE', #1339, #42020 ) ;
#9609=DIRECTION ( 'NONE',  ( -0.005002170337468016433, -0.7660444431189770143, 0.6427681459581293666 ) ) ;
#9610=LINE ( 'NONE', #4498, #30017 ) ;
#9611=VECTOR ( 'NONE', #44231, 1000.000000000000227 ) ;
#9612=EDGE_CURVE ( 'NONE', #19197, #4449, #39127, .T. ) ;
#9613=DIRECTION ( 'NONE',  ( -0.6427681459581293666, -0.7660444431189770143, -0.005002170337467561935 ) ) ;
#9614=AXIS2_PLACEMENT_3D ( 'NONE', #21853, #7984, #51115 ) ;
#9615=LINE ( 'NONE', #26630, #45707 ) ;
#9616=FACE_OUTER_BOUND ( 'NONE', #17383, .T. ) ;
#9617=CARTESIAN_POINT ( 'NONE',  ( -25.20278734466900517, 0.000000000000000000, 6.670939612111840944 ) ) ;
#9618=EDGE_CURVE ( 'NONE', #6876, #53403, #17260, .T. ) ;
#9619=AXIS2_PLACEMENT_3D ( 'NONE', #4597, #11985, #46935 ) ;
#9620=LINE ( 'NONE', #52483, #28821 ) ;
#9621=AXIS2_PLACEMENT_3D ( 'NONE', #12070, #38783, #55507 ) ;
#9622=CARTESIAN_POINT ( 'NONE',  ( -18.61382527010571764, 0.000000000000000000, 7.830212647944921223 ) ) ;
#9623=VECTOR ( 'NONE', #50907, 1000.000000000000227 ) ;
#9624=VERTEX_POINT ( 'NONE', #788 ) ;
#9625=VECTOR ( 'NONE', #6701, 1000.000000000000227 ) ;
#9626=AXIS2_PLACEMENT_3D ( 'NONE', #42628, #42912, #47165 ) ;
#9627=VERTEX_POINT ( 'NONE', #17551 ) ;
#9628=AXIS2_PLACEMENT_3D ( 'NONE', #7270, #54991, #55524 ) ;
#9629=ORIENTED_EDGE ( 'NONE', *, *, #18986, .T. ) ;
#9630=VERTEX_POINT ( 'NONE', #13840 ) ;
#9631=ORIENTED_EDGE ( 'NONE', *, *, #52659, .F. ) ;
#9632=LINE ( 'NONE', #26949, #45058 ) ;
#9633=CARTESIAN_POINT ( 'NONE',  ( -19.82178941147031637, -0.1191753592594188838, 6.612812754151981665 ) ) ;
#9634=ORIENTED_EDGE ( 'NONE', *, *, #35877, .T. ) ;
#9635=ORIENTED_EDGE ( 'NONE', *, *, #42688, .T. ) ;
#9636=VECTOR ( 'NONE', #41159, 1000.000000000000227 ) ;
#9638=VERTEX_POINT ( 'NONE', #44245 ) ;
#9639=DIRECTION ( 'NONE',  ( -0.6427681459581293666, -0.7660444431189770143, -0.005002170337467561935 ) ) ;
#9640=CARTESIAN_POINT ( 'NONE',  ( -16.99924723426068951, 0.000000000000000000, 13.49389102713827171 ) ) ;
#9641=VERTEX_POINT ( 'NONE', #34882 ) ;
#9642=VECTOR ( 'NONE', #36199, 999.9999999999998863 ) ;
#9643=CARTESIAN_POINT ( 'NONE',  ( -10.11544336623486728, -9.746244815904656633, 0.7108081496845154446 ) ) ;
#9644=ADVANCED_FACE ( 'NONE', ( #47940 ), #51630, .F. ) ;
#9645=EDGE_LOOP ( 'NONE', ( #26157, #5518, #41978, #39520 ) ) ;
#9646=CARTESIAN_POINT ( 'NONE',  ( -13.58766790975075089, -0.1191753592594177180, 5.922663989564801668 ) ) ;
#9647=AXIS2_PLACEMENT_3D ( 'NONE', #46219, #54746, #23809 ) ;
#9648=DIRECTION ( 'NONE',  ( -0.5364919789714478471, 0.6444004775717705469, -0.5449076811759709926 ) ) ;
#9649=ADVANCED_FACE ( 'NONE', ( #43654 ), #48491, .F. ) ;
#9650=EDGE_CURVE ( 'NONE', #51780, #22414, #34581, .T. ) ;
#9651=DIRECTION ( 'NONE',  ( 0.9999697198139515519, 0.000000000000000000, 0.007781995580013368816 ) ) ;
#9652=CARTESIAN_POINT ( 'NONE',  ( -9.542064456761055524, 0.000000000000000000, 10.59726798936431180 ) ) ;
#9653=VECTOR ( 'NONE', #6784, 999.9999999999998863 ) ;
#9654=VERTEX_POINT ( 'NONE', #5904 ) ;
#9655=PLANE ( 'NONE',  #22200 ) ;
#9656=PLANE ( 'NONE',  #50139 ) ;
#9657=LINE ( 'NONE', #47975, #10340 ) ;
#9658=ORIENTED_EDGE ( 'NONE', *, *, #9103, .F. ) ;
#9659=CARTESIAN_POINT ( 'NONE',  ( -17.76939998132051812, -0.1191753592594194527, 5.890120783652720071 ) ) ;
#9660=ORIENTED_EDGE ( 'NONE', *, *, #29182, .F. ) ;
#9662=VECTOR ( 'NONE', #41804, 1000.000000000000000 ) ;
#9663=DIRECTION ( 'NONE',  ( 0.007781995580012663651, -3.146120232559066537E-19, -0.9999697198139514409 ) ) ;
#9664=CARTESIAN_POINT ( 'NONE',  ( -17.93139508144814442, 0.000000000000000000, 13.85596890686001537 ) ) ;
#9666=LINE ( 'NONE', #26981, #20499 ) ;
#9667=CARTESIAN_POINT ( 'NONE',  ( -12.09453844680409951, 0.000000000000000000, 6.034286896408231904 ) ) ;
#9668=CARTESIAN_POINT ( 'NONE',  ( 2.072287782118878319, 0.000000000000000000, -2.950529333540147015 ) ) ;
#9669=CARTESIAN_POINT ( 'NONE',  ( 2.072287782118878319, 0.000000000000000000, -2.950529333540147015 ) ) ;
#9670=VECTOR ( 'NONE', #27793, 999.9999999999998863 ) ;
#9671=VECTOR ( 'NONE', #7212, 999.9999999999998863 ) ;
#9672=CARTESIAN_POINT ( 'NONE',  ( -15.42609712257811339, -0.1191753592594191752, 3.323032419688414230 ) ) ;
#9674=EDGE_LOOP ( 'NONE', ( #43497, #28710, #27943, #40773 ) ) ;
#9675=CARTESIAN_POINT ( 'NONE',  ( -19.16618472534906203, -0.1191753592594172323, 6.248582751606454266 ) ) ;
#9676=LINE ( 'NONE', #17136, #55751 ) ;
#9677=PLANE ( 'NONE',  #41745 ) ;
#9678=LINE ( 'NONE', #44304, #38538 ) ;
#9679=CARTESIAN_POINT ( 'NONE',  ( -8.380317325580694643, 0.000000000000000000, 6.432523893810073723 ) ) ;
#9680=ADVANCED_FACE ( 'NONE', ( #22929 ), #49044, .F. ) ;
#9681=DIRECTION ( 'NONE',  ( 0.000000000000000000, -0.000000000000000000, -1.000000000000000000 ) ) ;
#9682=DIRECTION ( 'NONE',  ( -0.5364919789714478471, 0.6444004775717705469, -0.5449076811759709926 ) ) ;
#9683=AXIS2_PLACEMENT_3D ( 'NONE', #1097, #4540, #47720 ) ;
#9684=EDGE_LOOP ( 'NONE', ( #4372, #12697, #11855, #52442 ) ) ;
#9685=ORIENTED_EDGE ( 'NONE', *, *, #24653, .F. ) ;
#9686=ADVANCED_FACE ( 'NONE', ( #15258 ), #10731, .F. ) ;
#9687=CARTESIAN_POINT ( 'NONE',  ( -18.36199618563782821, 0.000000000000000000, 9.478826732922961185 ) ) ;
#9688=LINE ( 'NONE', #5414, #15947 ) ;
#9689=VECTOR ( 'NONE', #30692, 999.9999999999998863 ) ;
#9691=FACE_OUTER_BOUND ( 'NONE', #29715, .T. ) ;
#9692=AXIS2_PLACEMENT_3D ( 'NONE', #28238, #27136, #48990 ) ;
#9693=ADVANCED_FACE ( 'NONE', ( #49331 ), #32573, .F. ) ;
#9694=VERTEX_POINT ( 'NONE', #10447 ) ;
#9695=LINE ( 'NONE', #39203, #4811 ) ;
#9696=VECTOR ( 'NONE', #20390, 999.9999999999998863 ) ;
#9697=EDGE_LOOP ( 'NONE', ( #17721, #20213, #10023, #5313 ) ) ;
#9698=ORIENTED_EDGE ( 'NONE', *, *, #45286, .T. ) ;
#9699=ORIENTED_EDGE ( 'NONE', *, *, #2626, .T. ) ;
#9700=LINE ( 'NONE', #44583, #27526 ) ;
#9701=CARTESIAN_POINT ( 'NONE',  ( -20.54204810873173415, 0.000000000000000000, 4.860550213503115558 ) ) ;
#9703=VECTOR ( 'NONE', #55294, 999.9999999999998863 ) ;
#9704=DIRECTION ( 'NONE',  ( 0.9999697198139515519, 0.000000000000000000, 0.007781995580013368816 ) ) ;
#9705=ORIENTED_EDGE ( 'NONE', *, *, #24727, .T. ) ;
#9706=ORIENTED_EDGE ( 'NONE', *, *, #42752, .F. ) ;
#9707=EDGE_CURVE ( 'NONE', #14368, #8086, #9886, .T. ) ;
#9708=VECTOR ( 'NONE', #36570, 999.9999999999998863 ) ;
#9709=VECTOR ( 'NONE', #50222, 1000.000000000000227 ) ;
#9710=DIRECTION ( 'NONE',  ( 0.7660212471507180654, -0.6427876096865404731, 0.005961354470445141482 ) ) ;
#9711=ORIENTED_EDGE ( 'NONE', *, *, #55949, .T. ) ;
#9712=DIRECTION ( 'NONE',  ( -0.6427681459581293666, -0.7660444431189770143, -0.005002170337467561935 ) ) ;
#9713=EDGE_CURVE ( 'NONE', #49012, #37392, #53334, .T. ) ;
#9714=VERTEX_POINT ( 'NONE', #53579 ) ;
#9715=FACE_OUTER_BOUND ( 'NONE', #53712, .T. ) ;
#9716=FACE_OUTER_BOUND ( 'NONE', #30805, .T. ) ;
#9717=ORIENTED_EDGE ( 'NONE', *, *, #54596, .T. ) ;
#9718=EDGE_CURVE ( 'NONE', #32655, #8255, #49875, .T. ) ;
#9720=VERTEX_POINT ( 'NONE', #45342 ) ;
#9721=EDGE_CURVE ( 'NONE', #45468, #2367, #1886, .T. ) ;
#9722=VECTOR ( 'NONE', #48599, 1000.000000000000227 ) ;
#9723=LINE ( 'NONE', #31279, #8234 ) ;
#9724=ORIENTED_EDGE ( 'NONE', *, *, #45985, .T. ) ;
#9725=DIRECTION ( 'NONE',  ( 0.5364919789714477361, 0.6444004775717706579, 0.5449076811759711036 ) ) ;
#9726=DIRECTION ( 'NONE',  ( -0.005961354470445682716, -0.6427876096865404731, 0.7660212471507180654 ) ) ;
#9727=LINE ( 'NONE', #36376, #37387 ) ;
#9728=EDGE_LOOP ( 'NONE', ( #9187, #17400, #10876, #33055 ) ) ;
#9729=CARTESIAN_POINT ( 'NONE',  ( 2.072287782118878319, 0.000000000000000000, -2.950529333540147015 ) ) ;
#9730=LINE ( 'NONE', #1469, #41019 ) ;
#9732=LINE ( 'NONE', #19057, #39432 ) ;
#9734=DIRECTION ( 'NONE',  ( -0.5364919789714478471, 0.6444004775717705469, -0.5449076811759709926 ) ) ;
#9735=PLANE ( 'NONE',  #45162 ) ;
#9736=EDGE_CURVE ( 'NONE', #30096, #49088, #44496, .T. ) ;
#9737=AXIS2_PLACEMENT_3D ( 'NONE', #28575, #2707, #37660 ) ;
#9738=CARTESIAN_POINT ( 'NONE',  ( -14.61647978877039478, 3.848249166794009746, 8.874490732104780122 ) ) ;
#9739=ORIENTED_EDGE ( 'NONE', *, *, #9159, .F. ) ;
#9740=LINE ( 'NONE', #36678, #11664 ) ;
#9742=DIRECTION ( 'NONE',  ( 0.005961354470445682716, -0.6427876096865404731, -0.7660212471507180654 ) ) ;
#9743=ORIENTED_EDGE ( 'NONE', *, *, #55021, .F. ) ;
#9744=PLANE ( 'NONE',  #52896 ) ;
#9745=LINE ( 'NONE', #14289, #7301 ) ;
#9748=CARTESIAN_POINT ( 'NONE',  ( -13.01519007997042188, 0.000000000000000000, 4.919125963098919918 ) ) ;
#9749=VECTOR ( 'NONE', #15771, 1000.000000000000227 ) ;
#9750=DIRECTION ( 'NONE',  ( 0.7660212471507180654, -0.6427876096865404731, 0.005961354470445141482 ) ) ;
#9751=CARTESIAN_POINT ( 'NONE',  ( -14.94916102560700821, 0.000000000000000000, 2.688082935172642962 ) ) ;
#9752=CARTESIAN_POINT ( 'NONE',  ( 2.072287782118878319, 0.000000000000000000, -2.950529333540147015 ) ) ;
#9753=EDGE_LOOP ( 'NONE', ( #22230, #18541, #46254, #39284 ) ) ;
#9754=ORIENTED_EDGE ( 'NONE', *, *, #20347, .F. ) ;
#9755=CARTESIAN_POINT ( 'NONE',  ( -18.19747506107908563, 0.000000000000000000, 14.03856424583689311 ) ) ;
#9756=CARTESIAN_POINT ( 'NONE',  ( -16.53317331066696383, 0.000000000000000000, 13.31285208727739899 ) ) ;
#9757=CARTESIAN_POINT ( 'NONE',  ( -21.47419595591918906, 0.000000000000000000, 5.222628093224860102 ) ) ;
#9758=DIRECTION ( 'NONE',  ( 0.007781995580012662783, 0.000000000000000000, -0.9999697198139514409 ) ) ;
#9759=DIRECTION ( 'NONE',  ( 0.005961354470445682716, -0.6427876096865404731, -0.7660212471507180654 ) ) ;
#9760=CARTESIAN_POINT ( 'NONE',  ( -24.27063949748155380, 0.000000000000000000, 6.308861732390097288 ) ) ;
#9761=EDGE_CURVE ( 'NONE', #11534, #36770, #41379, .T. ) ;
#9762=ORIENTED_EDGE ( 'NONE', *, *, #42814, .T. ) ;
#9763=DIRECTION ( 'NONE',  ( 0.5449076811759707706, 0.6444004775717708799, -0.5364919789714476250 ) ) ;
#9764=CARTESIAN_POINT ( 'NONE',  ( -20.81724602552766612, 3.524445264749009876, 4.655608788014395927 ) ) ;
#9765=VERTEX_POINT ( 'NONE', #14687 ) ;
#9766=PLANE ( 'NONE',  #31988 ) ;
#9767=CARTESIAN_POINT ( 'NONE',  ( -18.81956732107907015, 0.000000000000000000, 8.567275655344447571 ) ) ;
#9768=CARTESIAN_POINT ( 'NONE',  ( -15.50102849149811135, -0.1191753592594197858, 12.95155240711365430 ) ) ;
#9769=ADVANCED_FACE ( 'NONE', ( #36849 ), #18378, .F. ) ;
#9771=CARTESIAN_POINT ( 'NONE',  ( -11.67244013076689946, 0.000000000000000000, 11.50401908778467863 ) ) ;
#9772=ORIENTED_EDGE ( 'NONE', *, *, #42575, .F. ) ;
#9774=EDGE_CURVE ( 'NONE', #8247, #14910, #53858, .T. ) ;
#9775=VERTEX_POINT ( 'NONE', #23498 ) ;
#9776=VECTOR ( 'NONE', #18684, 999.9999999999998863 ) ;
#9777=ORIENTED_EDGE ( 'NONE', *, *, #43530, .T. ) ;
#9778=ORIENTED_EDGE ( 'NONE', *, *, #15125, .T. ) ;
#9779=LINE ( 'NONE', #19101, #14855 ) ;
#9780=ADVANCED_FACE ( 'NONE', ( #23756 ), #53035, .F. ) ;
#9782=ORIENTED_EDGE ( 'NONE', *, *, #9736, .F. ) ;
#9783=LINE ( 'NONE', #31049, #13174 ) ;
#9784=CARTESIAN_POINT ( 'NONE',  ( -14.01545677930355183, 0.000000000000000000, 2.126011111488108174 ) ) ;
#9785=VECTOR ( 'NONE', #48625, 999.9999999999998863 ) ;
#9787=CARTESIAN_POINT ( 'NONE',  ( -20.54204810873173415, 0.000000000000000000, 4.860550213503115558 ) ) ;
#9788=EDGE_CURVE ( 'NONE', #26765, #2694, #19504, .T. ) ;
#9789=EDGE_LOOP ( 'NONE', ( #5837, #19610, #9777, #27933 ) ) ;
#9790=PLANE ( 'NONE',  #9526 ) ;
#9791=ORIENTED_EDGE ( 'NONE', *, *, #29963, .F. ) ;
#9792=EDGE_CURVE ( 'NONE', #29905, #35206, #31477, .T. ) ;
#9793=FACE_OUTER_BOUND ( 'NONE', #34225, .T. ) ;
#9794=DIRECTION ( 'NONE',  ( 0.5449076811759707706, 0.6444004775717708799, -0.5364919789714476250 ) ) ;
#9796=DIRECTION ( 'NONE',  ( -0.9999697198139514409, -0.000000000000000000, -0.007781995580013368816 ) ) ;
#9797=CARTESIAN_POINT ( 'NONE',  ( -23.33771345073609638, -0.1191753592594197858, 5.846786880686956955 ) ) ;
#9798=EDGE_LOOP ( 'NONE', ( #50413, #38046, #39806, #6936 ) ) ;
#9799=ADVANCED_FACE ( 'NONE', ( #36027 ), #54685, .F. ) ;
#9800=ORIENTED_EDGE ( 'NONE', *, *, #18609, .F. ) ;
#9801=FACE_OUTER_BOUND ( 'NONE', #27058, .T. ) ;
#9802=DIRECTION ( 'NONE',  ( 0.000000000000000000, -0.000000000000000000, -1.000000000000000000 ) ) ;
#9803=CARTESIAN_POINT ( 'NONE',  ( -24.26908309836554878, 0.000000000000000000, 6.108867788427308376 ) ) ;
#9804=ADVANCED_FACE ( 'NONE', ( #51292 ), #41634, .F. ) ;
#9805=CARTESIAN_POINT ( 'NONE',  ( -17.76284804600266654, 0.4483081953215033444, 3.567321762835300003 ) ) ;
#9806=ORIENTED_EDGE ( 'NONE', *, *, #51779, .F. ) ;
#9807=FACE_OUTER_BOUND ( 'NONE', #24835, .T. ) ;
#9808=PLANE ( 'NONE',  #41380 ) ;
#9809=ORIENTED_EDGE ( 'NONE', *, *, #47714, .F. ) ;
#9810=DIRECTION ( 'NONE',  ( 0.005961354470445682716, -0.6427876096865404731, -0.7660212471507180654 ) ) ;
#9811=FACE_OUTER_BOUND ( 'NONE', #16558, .T. ) ;
#9813=FACE_OUTER_BOUND ( 'NONE', #29749, .T. ) ;
#9814=LINE ( 'NONE', #23143, #38759 ) ;
#9815=PLANE ( 'NONE',  #22307 ) ;
#9816=DIRECTION ( 'NONE',  ( 0.007781995580012663651, -3.146120232559066537E-19, -0.9999697198139514409 ) ) ;
#9817=DIRECTION ( 'NONE',  ( -0.005961354470445682716, -0.6427876096865404731, 0.7660212471507180654 ) ) ;
#9818=ORIENTED_EDGE ( 'NONE', *, *, #31507, .T. ) ;
#9819=EDGE_LOOP ( 'NONE', ( #46249, #45487, #15328, #12107 ) ) ;
#9820=FACE_OUTER_BOUND ( 'NONE', #18848, .T. ) ;
#9821=CARTESIAN_POINT ( 'NONE',  ( -18.15338008115919521, 0.000000000000000000, 8.372454022265671369 ) ) ;
#9822=DIRECTION ( 'NONE',  ( -0.5364919789714478471, 0.6444004775717705469, -0.5449076811759709926 ) ) ;
#9823=AXIS2_PLACEMENT_3D ( 'NONE', #50366, #50648, #41825 ) ;
#9824=DIRECTION ( 'NONE',  ( -0.6427681459581293666, -0.7660444431189770143, -0.005002170337467561935 ) ) ;
#9825=LINE ( 'NONE', #31678, #4914 ) ;
#9826=ADVANCED_FACE ( 'NONE', ( #55255 ), #42206, .F. ) ;
#9827=ORIENTED_EDGE ( 'NONE', *, *, #11894, .F. ) ;
#9828=DIRECTION ( 'NONE',  ( 0.7660212471507180654, -0.6427876096865404731, 0.005961354470445141482 ) ) ;
#9829=CARTESIAN_POINT ( 'NONE',  ( -16.94823507309948596, -3.594132820645662196, 3.349919529729364687 ) ) ;
#9830=CARTESIAN_POINT ( 'NONE',  ( -24.27063949748155380, 0.000000000000000000, 6.308861732390097288 ) ) ;
#9831=CARTESIAN_POINT ( 'NONE',  ( -19.98474353258670888, 0.000000000000000000, 4.864887286578777115 ) ) ;
#9832=ORIENTED_EDGE ( 'NONE', *, *, #55323, .T. ) ;
#9833=CARTESIAN_POINT ( 'NONE',  ( -7.626921145403491309, -9.440094667004895967, 6.180928759870859324 ) ) ;
#9834=ORIENTED_EDGE ( 'NONE', *, *, #27505, .T. ) ;
#9835=LINE ( 'NONE', #35130, #33168 ) ;
#9836=EDGE_CURVE ( 'NONE', #35036, #33995, #33413, .T. ) ;
#9837=EDGE_CURVE ( 'NONE', #41210, #27148, #54997, .T. ) ;
#9838=FACE_OUTER_BOUND ( 'NONE', #35666, .T. ) ;
#9839=VERTEX_POINT ( 'NONE', #29426 ) ;
#9840=LINE ( 'NONE', #53289, #18127 ) ;
#9841=ORIENTED_EDGE ( 'NONE', *, *, #55015, .F. ) ;
#9842=EDGE_CURVE ( 'NONE', #49209, #10401, #2470, .T. ) ;
#9843=ORIENTED_EDGE ( 'NONE', *, *, #50487, .F. ) ;
#9844=ORIENTED_EDGE ( 'NONE', *, *, #19698, .T. ) ;
#9845=DIRECTION ( 'NONE',  ( -0.005961354470445682716, -0.6427876096865404731, 0.7660212471507180654 ) ) ;
#9846=ORIENTED_EDGE ( 'NONE', *, *, #38868, .T. ) ;
#9847=ORIENTED_EDGE ( 'NONE', *, *, #30952, .F. ) ;
#9848=CARTESIAN_POINT ( 'NONE',  ( -11.17101276013249134, 0.000000000000000000, 6.780138126459778647 ) ) ;
#9849=CARTESIAN_POINT ( 'NONE',  ( -14.25207316155825765, -5.375054281893166142, 2.245817962481531538 ) ) ;
#9850=ORIENTED_EDGE ( 'NONE', *, *, #2551, .F. ) ;
#9851=ORIENTED_EDGE ( 'NONE', *, *, #49432, .T. ) ;
#9852=DIRECTION ( 'NONE',  ( -0.5449076811759708816, 0.6444004775717707689, 0.5364919789714475140 ) ) ;
#9853=EDGE_CURVE ( 'NONE', #33003, #39170, #11811, .T. ) ;
#9854=ORIENTED_EDGE ( 'NONE', *, *, #37587, .T. ) ;
#9855=VERTEX_POINT ( 'NONE', #50720 ) ;
#9856=EDGE_CURVE ( 'NONE', #29873, #41167, #3312, .T. ) ;
#9857=FACE_OUTER_BOUND ( 'NONE', #2100, .T. ) ;
#9858=FACE_OUTER_BOUND ( 'NONE', #45814, .T. ) ;
#9861=CARTESIAN_POINT ( 'NONE',  ( -17.87471697247878311, -4.079838673713161334, 10.32078915421988086 ) ) ;
#9862=VERTEX_POINT ( 'NONE', #24881 ) ;
#9863=PLANE ( 'NONE',  #31914 ) ;
#9864=VERTEX_POINT ( 'NONE', #37948 ) ;
#9866=VECTOR ( 'NONE', #40923, 999.9999999999998863 ) ;
#9867=DIRECTION ( 'NONE',  ( 0.5449076811759707706, 0.6444004775717708799, -0.5364919789714476250 ) ) ;
#9869=CARTESIAN_POINT ( 'NONE',  ( -17.23141079360358674, 0.000000000000000000, 9.318299196280007024 ) ) ;
#9870=PLANE ( 'NONE',  #5883 ) ;
#9871=CARTESIAN_POINT ( 'NONE',  ( -22.40478740399063895, 0.000000000000000000, 5.384712028983816623 ) ) ;
#9872=FACE_OUTER_BOUND ( 'NONE', #25632, .T. ) ;
#9873=EDGE_LOOP ( 'NONE', ( #2340, #5994, #23183, #31447 ) ) ;
#9874=FACE_OUTER_BOUND ( 'NONE', #55620, .T. ) ;
#9875=ORIENTED_EDGE ( 'NONE', *, *, #14772, .F. ) ;
#9876=DIRECTION ( 'NONE',  ( 0.000000000000000000, -0.000000000000000000, -1.000000000000000000 ) ) ;
#9877=LINE ( 'NONE', #6186, #14195 ) ;
#9878=DIRECTION ( 'NONE',  ( -0.6427681459581293666, -0.7660444431189770143, -0.005002170337467561935 ) ) ;
#9880=DIRECTION ( 'NONE',  ( 0.9999697198139515519, 0.000000000000000000, 0.007781995580013368816 ) ) ;
#9881=LINE ( 'NONE', #15254, #15057 ) ;
#9882=DIRECTION ( 'NONE',  ( 0.6427681459581294776, -0.7660444431189769032, 0.005002170337467562802 ) ) ;
#9883=ORIENTED_EDGE ( 'NONE', *, *, #38355, .F. ) ;
#9884=DIRECTION ( 'NONE',  ( -0.5364919789714478471, 0.6444004775717705469, -0.5449076811759709926 ) ) ;
#9885=CARTESIAN_POINT ( 'NONE',  ( -18.86354292863559579, 0.000000000000000000, 14.21804678658176080 ) ) ;
#9886=LINE ( 'NONE', #44791, #1897 ) ;
#9887=EDGE_CURVE ( 'NONE', #52348, #235, #20042, .T. ) ;
#9889=PLANE ( 'NONE',  #29166 ) ;
#9890=DIRECTION ( 'NONE',  ( 0.8531650599175527594, 0.4028455766673922356, -0.3313982828793700652 ) ) ;
#9891=EDGE_CURVE ( 'NONE', #54772, #25841, #20887, .T. ) ;
#9892=DIRECTION ( 'NONE',  ( -0.5364919789714478471, 0.6444004775717705469, -0.5449076811759709926 ) ) ;
#9893=DIRECTION ( 'NONE',  ( 0.5364919789714477361, 0.6444004775717706579, 0.5449076811759711036 ) ) ;
#9895=DIRECTION ( 'NONE',  ( -0.005002170337468016433, -0.7660444431189770143, 0.6427681459581293666 ) ) ;
#9896=EDGE_CURVE ( 'NONE', #3399, #29707, #55531, .T. ) ;
#9897=EDGE_CURVE ( 'NONE', #27291, #32551, #8132, .T. ) ;
#9898=ADVANCED_FACE ( 'NONE', ( #11259 ), #3001, .F. ) ;
#9899=VERTEX_POINT ( 'NONE', #24327 ) ;
#9900=EDGE_CURVE ( 'NONE', #19288, #13109, #37365, .T. ) ;
#9901=ORIENTED_EDGE ( 'NONE', *, *, #51993, .F. ) ;
#9902=ORIENTED_EDGE ( 'NONE', *, *, #17247, .T. ) ;
#9903=ORIENTED_EDGE ( 'NONE', *, *, #6002, .F. ) ;
#9904=EDGE_LOOP ( 'NONE', ( #28379, #37694, #41043, #18644 ) ) ;
#9905=DIRECTION ( 'NONE',  ( 0.6427681459581294776, -0.7660444431189769032, 0.005002170337467562802 ) ) ;
#9906=DIRECTION ( 'NONE',  ( 0.000000000000000000, -1.000000000000000000, 0.000000000000000000 ) ) ;
#9907=ORIENTED_EDGE ( 'NONE', *, *, #12117, .F. ) ;
#9908=ORIENTED_EDGE ( 'NONE', *, *, #54420, .F. ) ;
#9909=VERTEX_POINT ( 'NONE', #50450 ) ;
#9910=EDGE_CURVE ( 'NONE', #15470, #12113, #46173, .T. ) ;
#9911=EDGE_CURVE ( 'NONE', #49710, #3791, #21482, .T. ) ;
#9912=CARTESIAN_POINT ( 'NONE',  ( -32.65997012216863737, 0.000000000000000000, 9.567562649885804404 ) ) ;
#9913=ORIENTED_EDGE ( 'NONE', *, *, #14890, .F. ) ;
#9914=EDGE_CURVE ( 'NONE', #6097, #36758, #434, .T. ) ;
#9916=CARTESIAN_POINT ( 'NONE',  ( -11.27719002838203544, -1.813211359398156919, 4.038164060868105310 ) ) ;
#9918=FACE_OUTER_BOUND ( 'NONE', #17020, .T. ) ;
#9919=VERTEX_POINT ( 'NONE', #56113 ) ;
#9920=ADVANCED_FACE ( 'NONE', ( #22019 ), #52668, .F. ) ;
#9921=DIRECTION ( 'NONE',  ( 0.000000000000000000, -0.000000000000000000, -1.000000000000000000 ) ) ;
#9922=DIRECTION ( 'NONE',  ( -0.7660212471507179544, -0.6427876096865405842, -0.005961354470445141482 ) ) ;
#9923=EDGE_CURVE ( 'NONE', #41467, #25423, #34803, .T. ) ;
#9924=LINE ( 'NONE', #14458, #49966 ) ;
#9925=CARTESIAN_POINT ( 'NONE',  ( -20.26077012639039765, 0.7834091684795615462, 5.482683156939285318 ) ) ;
#9926=ORIENTED_EDGE ( 'NONE', *, *, #9494, .T. ) ;
#9927=DIRECTION ( 'NONE',  ( 0.005961354470445682716, -0.6427876096865404731, -0.7660212471507180654 ) ) ;
#9928=CARTESIAN_POINT ( 'NONE',  ( -19.45180701075420160, 5.143464774974011888, 12.87836550513064537 ) ) ;
#9929=PLANE ( 'NONE',  #30285 ) ;
#9930=VERTEX_POINT ( 'NONE', #12670 ) ;
#9931=CARTESIAN_POINT ( 'NONE',  ( -15.40103151951671734, 0.000000000000000000, 12.95233060667165681 ) ) ;
#9932=ORIENTED_EDGE ( 'NONE', *, *, #20051, .T. ) ;
#9933=DIRECTION ( 'NONE',  ( -0.5449076811759708816, 0.6444004775717707689, 0.5364919789714475140 ) ) ;
#9934=CARTESIAN_POINT ( 'NONE',  ( -10.67476127473329939, 0.000000000000000000, 2.721347302392381096 ) ) ;
#9935=CARTESIAN_POINT ( 'NONE',  ( -11.61972299033116052, 0.000000000000000000, 4.729979754440159390 ) ) ;
#9937=LINE ( 'NONE', #5962, #26873 ) ;
#9938=PLANE ( 'NONE',  #20420 ) ;
#9939=DIRECTION ( 'NONE',  ( -0.8531650599175529814, -0.4028455766673920135, 0.3313982828793697877 ) ) ;
#9940=CARTESIAN_POINT ( 'NONE',  ( -14.46888367232926420, 0.000000000000000000, 12.59025272694991315 ) ) ;
#9941=DIRECTION ( 'NONE',  ( -0.5449076811759708816, 0.6444004775717707689, 0.5364919789714475140 ) ) ;
#9942=VERTEX_POINT ( 'NONE', #35367 ) ;
#9943=CARTESIAN_POINT ( 'NONE',  ( -17.36110980056009723, 3.848249166794009746, 3.302797067581964008 ) ) ;
#9944=CARTESIAN_POINT ( 'NONE',  ( -9.342070512798265725, 0.000000000000000000, 10.59882438848031505 ) ) ;
#9945=DIRECTION ( 'NONE',  ( -0.005002170337468016433, -0.7660444431189770143, 0.6427681459581293666 ) ) ;
#9946=LINE ( 'NONE', #23293, #6943 ) ;
#9947=DIRECTION ( 'NONE',  ( 0.9321478471874540261, 0.000000000000000000, -0.3620778797217456546 ) ) ;
#9949=DIRECTION ( 'NONE',  ( 0.7660212471507180654, -0.6427876096865404731, 0.005961354470445141482 ) ) ;
#9950=VERTEX_POINT ( 'NONE', #17472 ) ;
#9951=ORIENTED_EDGE ( 'NONE', *, *, #52811, .F. ) ;
#9952=CARTESIAN_POINT ( 'NONE',  ( -11.40636015113596180, 0.000000000000000000, 11.32142374880780089 ) ) ;
#9953=CARTESIAN_POINT ( 'NONE',  ( -26.13493519185646008, 0.000000000000000000, 7.033017491833586377 ) ) ;
#9954=EDGE_CURVE ( 'NONE', #34831, #43904, #51571, .T. ) ;
#9955=ORIENTED_EDGE ( 'NONE', *, *, #46752, .F. ) ;
#9956=CARTESIAN_POINT ( 'NONE',  ( -16.43317633868556626, -0.1191753592594197858, 13.31363028683540151 ) ) ;
#9957=ORIENTED_EDGE ( 'NONE', *, *, #52141, .T. ) ;
#9958=DIRECTION ( 'NONE',  ( -0.5449076811759708816, 0.6444004775717707689, 0.5364919789714475140 ) ) ;
#9959=EDGE_CURVE ( 'NONE', #43441, #16665, #42744, .T. ) ;
#9960=EDGE_CURVE ( 'NONE', #41657, #36649, #31093, .T. ) ;
#9961=ORIENTED_EDGE ( 'NONE', *, *, #20430, .T. ) ;
#9962=ORIENTED_EDGE ( 'NONE', *, *, #33468, .F. ) ;
#9964=LINE ( 'NONE', #10540, #7574 ) ;
#9966=DIRECTION ( 'NONE',  ( 0.7660212471507180654, -0.6427876096865404731, 0.005961354470445141482 ) ) ;
#9967=CARTESIAN_POINT ( 'NONE',  ( -11.67244013076689946, 0.000000000000000000, 11.50401908778467863 ) ) ;
#9968=ORIENTED_EDGE ( 'NONE', *, *, #36360, .F. ) ;
#9969=ORIENTED_EDGE ( 'NONE', *, *, #23882, .T. ) ;
#9970=LINE ( 'NONE', #22486, #10977 ) ;
#9971=ORIENTED_EDGE ( 'NONE', *, *, #15719, .T. ) ;
#9972=CARTESIAN_POINT ( 'NONE',  ( -9.808144436391993182, 0.000000000000000000, 10.77986332834118777 ) ) ;
#9973=ORIENTED_EDGE ( 'NONE', *, *, #18610, .F. ) ;
#9974=CARTESIAN_POINT ( 'NONE',  ( -30.79567442779373110, 0.000000000000000000, 8.843406890442315316 ) ) ;
#9975=FACE_OUTER_BOUND ( 'NONE', #28546, .T. ) ;
#9976=ORIENTED_EDGE ( 'NONE', *, *, #37314, .F. ) ;
#9977=DIRECTION ( 'NONE',  ( -0.8531650599175527594, 0.4028455766673922356, 0.3313982828793700652 ) ) ;
#9978=VERTEX_POINT ( 'NONE', #52414 ) ;
#9979=EDGE_CURVE ( 'NONE', #24462, #42825, #26281, .T. ) ;
#9980=DIRECTION ( 'NONE',  ( -0.5449076811759708816, 0.6444004775717707689, 0.5364919789714475140 ) ) ;
#9981=ORIENTED_EDGE ( 'NONE', *, *, #27568, .F. ) ;
#9982=EDGE_CURVE ( 'NONE', #16077, #29459, #47586, .T. ) ;
#9983=LINE ( 'NONE', #22207, #44900 ) ;
#9984=CARTESIAN_POINT ( 'NONE',  ( -13.41745442594840654, 3.038739411681508518, 1.796774992419481798 ) ) ;
#9985=LINE ( 'NONE', #27294, #21960 ) ;
#9986=VERTEX_POINT ( 'NONE', #43877 ) ;
#9987=CARTESIAN_POINT ( 'NONE',  ( -12.57067155766631750, 0.000000000000000000, 7.507909797671279861 ) ) ;
#9988=ADVANCED_FACE ( 'NONE', ( #30572 ), #21174, .F. ) ;
#9989=CARTESIAN_POINT ( 'NONE',  ( -13.30555201101248208, 4.495856970884009485, 9.428116599730730130 ) ) ;
#9990=FACE_OUTER_BOUND ( 'NONE', #19813, .T. ) ;
#9991=CARTESIAN_POINT ( 'NONE',  ( -11.61110082981531377, 0.000000000000000000, 3.622050644666864994 ) ) ;
#9992=CARTESIAN_POINT ( 'NONE',  ( -12.72567141089270315, 0.000000000000000000, 1.724709365947141748 ) ) ;
#9993=AXIS2_PLACEMENT_3D ( 'NONE', #37941, #33405, #24872 ) ;
#9995=ORIENTED_EDGE ( 'NONE', *, *, #26069, .T. ) ;
#9996=FACE_OUTER_BOUND ( 'NONE', #4783, .T. ) ;
#9997=DIRECTION ( 'NONE',  ( 0.007781995580012663651, 0.000000000000000000, -0.9999697198139515519 ) ) ;
#9998=DIRECTION ( 'NONE',  ( 0.7660212471507180654, -0.6427876096865404731, 0.005961354470445141482 ) ) ;
#9999=ORIENTED_EDGE ( 'NONE', *, *, #46888, .F. ) ;
#10000=LINE ( 'NONE', #32441, #6655 ) ;
#10001=LINE ( 'NONE', #9438, #23638 ) ;
#10002=ORIENTED_EDGE ( 'NONE', *, *, #28916, .F. ) ;
#10003=FACE_OUTER_BOUND ( 'NONE', #2081, .T. ) ;
#10004=CARTESIAN_POINT ( 'NONE',  ( -14.97617745865445826, -5.051250379848161387, 10.78915007593705866 ) ) ;
#10005=LINE ( 'NONE', #44628, #7845 ) ;
#10006=CARTESIAN_POINT ( 'NONE',  ( -16.99924723426068951, 0.000000000000000000, 13.49389102713827171 ) ) ;
#10007=ORIENTED_EDGE ( 'NONE', *, *, #2194, .F. ) ;
#10008=ORIENTED_EDGE ( 'NONE', *, *, #41910, .T. ) ;
#10009=CARTESIAN_POINT ( 'NONE',  ( -16.33317936670417225, 0.000000000000000000, 13.31440848639340224 ) ) ;
#10010=DIRECTION ( 'NONE',  ( -0.5364919789714478471, 0.6444004775717705469, -0.5449076811759709926 ) ) ;
#10011=CARTESIAN_POINT ( 'NONE',  ( -20.21988856968611969, -2.460819163488157546, 8.574646605433253299 ) ) ;
#10012=ADVANCED_FACE ( 'NONE', ( #48129 ), #9232, .F. ) ;
#10013=DIRECTION ( 'NONE',  ( -0.5364919789714478471, 0.6444004775717705469, -0.5449076811759709926 ) ) ;
#10014=ADVANCED_FACE ( 'NONE', ( #22321 ), #39648, .F. ) ;
#10015=FACE_OUTER_BOUND ( 'NONE', #954, .T. ) ;
#10016=ORIENTED_EDGE ( 'NONE', *, *, #48568, .T. ) ;
#10017=CARTESIAN_POINT ( 'NONE',  ( -18.29747203306047609, -0.1191753592594177458, 14.03778604627889059 ) ) ;
#10018=VERTEX_POINT ( 'NONE', #18046 ) ;
#10019=DIRECTION ( 'NONE',  ( 0.007781995580012662783, 0.000000000000000000, -0.9999697198139514409 ) ) ;
#10020=EDGE_CURVE ( 'NONE', #51066, #32400, #55831, .T. ) ;
#10021=EDGE_CURVE ( 'NONE', #43180, #28433, #47285, .T. ) ;
#10023=ORIENTED_EDGE ( 'NONE', *, *, #16116, .T. ) ;
#10024=LINE ( 'NONE', #32171, #33801 ) ;
#10025=DIRECTION ( 'NONE',  ( 0.6427681459581294776, -0.7660444431189769032, 0.005002170337467562802 ) ) ;
#10026=CARTESIAN_POINT ( 'NONE',  ( -9.542064456761055524, 0.000000000000000000, 10.59726798936431180 ) ) ;
#10027=ORIENTED_EDGE ( 'NONE', *, *, #26261, .T. ) ;
#10028=DIRECTION ( 'NONE',  ( -0.005961354470445682716, -0.6427876096865404731, 0.7660212471507180654 ) ) ;
#10029=VERTEX_POINT ( 'NONE', #4158 ) ;
#10030=ADVANCED_FACE ( 'NONE', ( #43344 ), #4439, .F. ) ;
#10031=AXIS2_PLACEMENT_3D ( 'NONE', #34642, #846, #30942 ) ;
#10032=EDGE_LOOP ( 'NONE', ( #21358, #46355, #49466, #1162 ) ) ;
#10033=VERTEX_POINT ( 'NONE', #49816 ) ;
#10034=ORIENTED_EDGE ( 'NONE', *, *, #28599, .T. ) ;
#10035=CARTESIAN_POINT ( 'NONE',  ( -14.91176584496347424, -5.051250379848164052, 2.512396043748728491 ) ) ;
#10036=ORIENTED_EDGE ( 'NONE', *, *, #37054, .T. ) ;
#10037=LINE ( 'NONE', #18262, #1360 ) ;
#10038=DIRECTION ( 'NONE',  ( 0.005002170337468016433, -0.7660444431189770143, -0.6427681459581293666 ) ) ;
#10039=EDGE_LOOP ( 'NONE', ( #25666, #11969, #25580, #35457 ) ) ;
#10040=ORIENTED_EDGE ( 'NONE', *, *, #31629, .T. ) ;
#10041=CARTESIAN_POINT ( 'NONE',  ( -10.27421835998572064, 0.000000000000000000, 10.96090226820206048 ) ) ;
#10042=EDGE_LOOP ( 'NONE', ( #48741, #48268, #19912, #55326 ) ) ;
#10043=PLANE ( 'NONE',  #6538 ) ;
#10044=DIRECTION ( 'NONE',  ( 0.000000000000000000, 1.000000000000000000, -0.000000000000000000 ) ) ;
#10045=CARTESIAN_POINT ( 'NONE',  ( -15.50102849149811135, -0.1191753592594197858, 12.95155240711365430 ) ) ;
#10046=LINE ( 'NONE', #6353, #23900 ) ;
#10047=CARTESIAN_POINT ( 'NONE',  ( -10.88756908710649896, 0.000000000000000000, 4.366345475602411597 ) ) ;
#10048=CARTESIAN_POINT ( 'NONE',  ( -12.60458797795435615, 0.000000000000000000, 11.86609696750642229 ) ) ;
#10049=FACE_OUTER_BOUND ( 'NONE', #26422, .T. ) ;
#10050=VERTEX_POINT ( 'NONE', #53789 ) ;
#10051=EDGE_LOOP ( 'NONE', ( #18949, #45120, #10189, #25289 ) ) ;
#10052=VECTOR ( 'NONE', #18191, 999.9999999999998863 ) ;
#10053=CARTESIAN_POINT ( 'NONE',  ( -16.81345671998191449, 0.000000000000000000, 3.412238694616132495 ) ) ;
#10054=EDGE_CURVE ( 'NONE', #23468, #5331, #40483, .T. ) ;
#10055=CARTESIAN_POINT ( 'NONE',  ( -11.30636317915456779, -0.1191753592594197858, 11.32220194836580340 ) ) ;
#10056=DIRECTION ( 'NONE',  ( 0.5364919789714477361, 0.6444004775717706579, 0.5449076811759711036 ) ) ;
#10057=LINE ( 'NONE', #5810, #8638 ) ;
#10059=PLANE ( 'NONE',  #1423 ) ;
#10060=DIRECTION ( 'NONE',  ( 0.9999697198139515519, 0.000000000000000000, 0.007781995580013368816 ) ) ;
#10061=ORIENTED_EDGE ( 'NONE', *, *, #40989, .T. ) ;
#10062=LINE ( 'NONE', #35354, #49243 ) ;
#10063=CARTESIAN_POINT ( 'NONE',  ( -13.49551489872720111, 0.000000000000000000, 6.931374326914707673 ) ) ;
#10064=ORIENTED_EDGE ( 'NONE', *, *, #52482, .T. ) ;
#10065=EDGE_CURVE ( 'NONE', #20837, #18484, #44433, .T. ) ;
#10066=CARTESIAN_POINT ( 'NONE',  ( -10.39706570871786795, 0.000000000000000000, 1.046174058050539646 ) ) ;
#10067=LINE ( 'NONE', #27380, #25138 ) ;
#10068=VECTOR ( 'NONE', #51409, 1000.000000000000227 ) ;
#10069=CARTESIAN_POINT ( 'NONE',  ( -24.26908309836554878, 0.000000000000000000, 6.108867788427308376 ) ) ;
#10070=EDGE_CURVE ( 'NONE', #38527, #16305, #32515, .T. ) ;
#10071=EDGE_CURVE ( 'NONE', #12044, #28099, #49257, .T. ) ;
#10072=DIRECTION ( 'NONE',  ( -0.5364919789714478471, 0.6444004775717705469, -0.5449076811759709926 ) ) ;
#10073=VECTOR ( 'NONE', #43122, 1000.000000000000227 ) ;
#10074=DIRECTION ( 'NONE',  ( 0.5364919789714477361, 0.6444004775717706579, 0.5449076811759711036 ) ) ;
#10075=VERTEX_POINT ( 'NONE', #19145 ) ;
#10076=ORIENTED_EDGE ( 'NONE', *, *, #12950, .T. ) ;
#10077=LINE ( 'NONE', #44711, #31208 ) ;
#10078=DIRECTION ( 'NONE',  ( 0.7660212471507180654, -0.6427876096865404731, 0.005961354470445141482 ) ) ;
#10079=CARTESIAN_POINT ( 'NONE',  ( -17.46532115785441519, 0.000000000000000000, 13.67492996699914265 ) ) ;
#10080=EDGE_CURVE ( 'NONE', #43916, #32205, #1267, .T. ) ;
#10081=CARTESIAN_POINT ( 'NONE',  ( -12.53905696910820744, 0.000000000000000000, 3.445503061835871517 ) ) ;
#10082=EDGE_CURVE ( 'NONE', #23668, #56039, #14364, .T. ) ;
#10083=LINE ( 'NONE', #18904, #1335 ) ;
#10084=EDGE_LOOP ( 'NONE', ( #29690, #5386, #925, #25716 ) ) ;
#10086=CARTESIAN_POINT ( 'NONE',  ( -10.84028925556084388, -0.1191753592594197858, 11.14116300850493246 ) ) ;
#10087=EDGE_CURVE ( 'NONE', #41032, #36837, #41008, .T. ) ;
#10088=DIRECTION ( 'NONE',  ( -0.005961354470445682716, -0.6427876096865404731, 0.7660212471507180654 ) ) ;
#10089=CARTESIAN_POINT ( 'NONE',  ( -16.02599783302199299, 0.000000000000000000, 7.850351719436975628 ) ) ;
#10090=ORIENTED_EDGE ( 'NONE', *, *, #49388, .T. ) ;
#10091=CARTESIAN_POINT ( 'NONE',  ( -16.81267852042391198, -0.1191753592594197858, 3.312241722634738039 ) ) ;
#10092=ORIENTED_EDGE ( 'NONE', *, *, #42107, .T. ) ;
#10093=CARTESIAN_POINT ( 'NONE',  ( -11.87243407472968926, 0.000000000000000000, 11.50246268866867361 ) ) ;
#10094=PLANE ( 'NONE',  #18470 ) ;
#10095=ADVANCED_FACE ( 'NONE', ( #31676 ), #36216, .F. ) ;
#10096=ORIENTED_EDGE ( 'NONE', *, *, #20539, .F. ) ;
#10097=VECTOR ( 'NONE', #2241, 999.9999999999998863 ) ;
#10098=VECTOR ( 'NONE', #47632, 1000.000000000000114 ) ;
#10099=DIRECTION ( 'NONE',  ( 0.007781995580012663651, 0.000000000000000000, -0.9999697198139515519 ) ) ;
#10100=ORIENTED_EDGE ( 'NONE', *, *, #33344, .F. ) ;
#10101=ADVANCED_FACE ( 'NONE', ( #22592 ), #53516, .F. ) ;
#10102=VERTEX_POINT ( 'NONE', #27391 ) ;
#10103=ORIENTED_EDGE ( 'NONE', *, *, #44902, .T. ) ;
#10104=DIRECTION ( 'NONE',  ( 0.9999697198139515519, 0.000000000000000000, 0.007781995580013368816 ) ) ;
#10105=ORIENTED_EDGE ( 'NONE', *, *, #32844, .T. ) ;
#10107=DIRECTION ( 'NONE',  ( -0.005961354470445682716, -0.6427876096865404731, 0.7660212471507180654 ) ) ;
#10108=PLANE ( 'NONE',  #42145 ) ;
#10109=EDGE_LOOP ( 'NONE', ( #45763, #5365, #26947, #3233 ) ) ;
#10110=ORIENTED_EDGE ( 'NONE', *, *, #54058, .T. ) ;
#10111=LINE ( 'NONE', #9567, #43992 ) ;
#10112=VERTEX_POINT ( 'NONE', #14618 ) ;
#10114=AXIS2_PLACEMENT_3D ( 'NONE', #53069, #53355, #43975 ) ;
#10115=DIRECTION ( 'NONE',  ( -0.7660212471507179544, -0.6427876096865405842, -0.005961354470445141482 ) ) ;
#10116=LINE ( 'NONE', #35401, #50263 ) ;
#10117=FACE_OUTER_BOUND ( 'NONE', #49913, .T. ) ;
#10118=PLANE ( 'NONE',  #26844 ) ;
#10119=ORIENTED_EDGE ( 'NONE', *, *, #47743, .F. ) ;
#10120=CARTESIAN_POINT ( 'NONE',  ( -17.09571308368427367, -2.622721114510659035, 7.626819433174508056 ) ) ;
#10121=VERTEX_POINT ( 'NONE', #31937 ) ;
#10122=EDGE_CURVE ( 'NONE', #49177, #1909, #49559, .T. ) ;
#10123=FACE_OUTER_BOUND ( 'NONE', #22525, .T. ) ;
#10124=CARTESIAN_POINT ( 'NONE',  ( -9.808144436391993182, 0.000000000000000000, 10.77986332834118777 ) ) ;
#10126=LINE ( 'NONE', #28021, #34904 ) ;
#10127=LINE ( 'NONE', #23212, #54728 ) ;
#10128=DIRECTION ( 'NONE',  ( 0.000000000000000000, -0.000000000000000000, -1.000000000000000000 ) ) ;
#10129=VERTEX_POINT ( 'NONE', #27127 ) ;
#10130=LINE ( 'NONE', #1325, #35633 ) ;
#10132=ORIENTED_EDGE ( 'NONE', *, *, #45776, .F. ) ;
#10133=VECTOR ( 'NONE', #55258, 1000.000000000000227 ) ;
#10134=VECTOR ( 'NONE', #8440, 1000.000000000000227 ) ;
#10135=FACE_OUTER_BOUND ( 'NONE', #40623, .T. ) ;
#10136=LINE ( 'NONE', #31998, #38670 ) ;
#10137=FACE_OUTER_BOUND ( 'NONE', #43965, .T. ) ;
#10138=CARTESIAN_POINT ( 'NONE',  ( -14.57916698481732887, 1.095915999411504194, 2.310009840857418340 ) ) ;
#10139=EDGE_CURVE ( 'NONE', #39340, #27792, #52958, .T. ) ;
#10140=DIRECTION ( 'NONE',  ( -0.7660212471507179544, -0.6427876096865405842, -0.005961354470445141482 ) ) ;
#10141=LINE ( 'NONE', #5341, #39318 ) ;
#10142=VECTOR ( 'NONE', #42657, 1000.000000000000227 ) ;
#10143=ORIENTED_EDGE ( 'NONE', *, *, #50663, .T. ) ;
#10144=DIRECTION ( 'NONE',  ( 0.005002170337468016433, -0.7660444431189770143, -0.6427681459581293666 ) ) ;
#10145=DIRECTION ( 'NONE',  ( 0.6427681459581294776, -0.7660444431189769032, 0.005002170337467562802 ) ) ;
#10146=DIRECTION ( 'NONE',  ( 0.007781995580012663651, 0.000000000000000000, -0.9999697198139515519 ) ) ;
#10147=DIRECTION ( 'NONE',  ( -0.005961354470445682716, -0.6427876096865404731, 0.7660212471507180654 ) ) ;
#10148=EDGE_CURVE ( 'NONE', #30900, #40325, #18305, .T. ) ;
#10149=VECTOR ( 'NONE', #19249, 999.9999999999998863 ) ;
#10150=LINE ( 'NONE', #17555, #38463 ) ;
#10151=DIRECTION ( 'NONE',  ( 0.9999697198139515519, 0.000000000000000000, 0.007781995580013368816 ) ) ;
#10152=LINE ( 'NONE', #40256, #48294 ) ;
#10153=VECTOR ( 'NONE', #50035, 1000.000000000000227 ) ;
#10154=EDGE_CURVE ( 'NONE', #15763, #20246, #45022, .T. ) ;
#10155=FACE_OUTER_BOUND ( 'NONE', #19533, .T. ) ;
#10156=CARTESIAN_POINT ( 'NONE',  ( -18.37703690296480019, -5.213152330870661544, 12.37586806173053056 ) ) ;
#10157=EDGE_CURVE ( 'NONE', #46689, #9630, #40753, .T. ) ;
#10158=ORIENTED_EDGE ( 'NONE', *, *, #13652, .T. ) ;
#10159=EDGE_CURVE ( 'NONE', #22163, #41757, #2096, .T. ) ;
#10160=ORIENTED_EDGE ( 'NONE', *, *, #25159, .F. ) ;
#10161=ORIENTED_EDGE ( 'NONE', *, *, #48437, .T. ) ;
#10162=EDGE_LOOP ( 'NONE', ( #27007, #2325, #25182, #40699 ) ) ;
#10164=DIRECTION ( 'NONE',  ( 0.005961354470445682716, -0.6427876096865404731, -0.7660212471507180654 ) ) ;
#10165=CARTESIAN_POINT ( 'NONE',  ( -11.63984136486813803, 0.000000000000000000, 7.315147677244509872 ) ) ;
#10166=AXIS2_PLACEMENT_3D ( 'NONE', #38589, #47100, #20966 ) ;
#10167=VECTOR ( 'NONE', #34365, 999.9999999999998863 ) ;
#10168=ORIENTED_EDGE ( 'NONE', *, *, #31169, .F. ) ;
#10169=ORIENTED_EDGE ( 'NONE', *, *, #15766, .F. ) ;
#10170=ORIENTED_EDGE ( 'NONE', *, *, #14215, .T. ) ;
#10171=VECTOR ( 'NONE', #35475, 1000.000000000000114 ) ;
#10172=CARTESIAN_POINT ( 'NONE',  ( -16.93515325216717926, 0.000000000000000000, 5.257951973096605336 ) ) ;
#10173=CARTESIAN_POINT ( 'NONE',  ( -28.93060053386082231, -0.1191753592594197858, 8.019254159017428663 ) ) ;
#10174=CARTESIAN_POINT ( 'NONE',  ( -15.52244184149622264, 0.000000000000000000, 2.852947544891258680 ) ) ;
#10175=ORIENTED_EDGE ( 'NONE', *, *, #12731, .T. ) ;
#10176=LINE ( 'NONE', #32042, #45514 ) ;
#10177=EDGE_CURVE ( 'NONE', #26525, #16077, #45284, .T. ) ;
#10178=ORIENTED_EDGE ( 'NONE', *, *, #1210, .T. ) ;
#10179=DIRECTION ( 'NONE',  ( 0.7660212471507180654, -0.6427876096865404731, 0.005961354470445141482 ) ) ;
#10180=VECTOR ( 'NONE', #52093, 1000.000000000000114 ) ;
#10181=ADVANCED_FACE ( 'NONE', ( #36774 ), #35645, .F. ) ;
#10182=CARTESIAN_POINT ( 'NONE',  ( -27.06708303904391144, 0.000000000000000000, 7.395095371555332697 ) ) ;
#10183=CARTESIAN_POINT ( 'NONE',  ( -20.54204810873173415, 0.000000000000000000, 4.860550213503115558 ) ) ;
#10184=DIRECTION ( 'NONE',  ( 0.6427681459581294776, -0.7660444431189769032, 0.005002170337467562802 ) ) ;
#10185=CARTESIAN_POINT ( 'NONE',  ( -11.79997668751810203, -2.460819163488159766, 1.386319776390585012 ) ) ;
#10187=FACE_OUTER_BOUND ( 'NONE', #654, .T. ) ;
#10188=EDGE_CURVE ( 'NONE', #19170, #33373, #20826, .T. ) ;
#10189=ORIENTED_EDGE ( 'NONE', *, *, #23850, .T. ) ;
#10190=CARTESIAN_POINT ( 'NONE',  ( -9.755427295956252465, 0.000000000000000000, 4.005823994996667636 ) ) ;
#10191=ORIENTED_EDGE ( 'NONE', *, *, #36713, .F. ) ;
#10193=ADVANCED_FACE ( 'NONE', ( #6659 ), #16562, .F. ) ;
#10194=EDGE_CURVE ( 'NONE', #18937, #36080, #10914, .T. ) ;
#10195=DIRECTION ( 'NONE',  ( 0.005961354470445682716, -0.6427876096865404731, -0.7660212471507180654 ) ) ;
#10196=LINE ( 'NONE', #27518, #25993 ) ;
#10198=CARTESIAN_POINT ( 'NONE',  ( -18.46543118150865226, 2.391131607591508335, 3.778242673840852994 ) ) ;
#10199=VECTOR ( 'NONE', #10074, 999.9999999999998863 ) ;
#10200=DIRECTION ( 'NONE',  ( 0.007781995580012663651, -3.146120232559066537E-19, -0.9999697198139514409 ) ) ;
#10201=DIRECTION ( 'NONE',  ( 0.000000000000000000, -0.000000000000000000, -1.000000000000000000 ) ) ;
#10203=FACE_OUTER_BOUND ( 'NONE', #11283, .T. ) ;
#10204=FACE_OUTER_BOUND ( 'NONE', #25137, .T. ) ;
#10206=VECTOR ( 'NONE', #26489, 999.9999999999998863 ) ;
#10207=CARTESIAN_POINT ( 'NONE',  ( -15.83594370396432183, 0.000000000000000000, 9.129152987621246496 ) ) ;
#10208=DIRECTION ( 'NONE',  ( 0.5364919789714477361, 0.6444004775717706579, 0.5449076811759711036 ) ) ;
#10209=CARTESIAN_POINT ( 'NONE',  ( -19.60834386242827776, 0.000000000000000000, 4.298478389818581213 ) ) ;
#10210=DIRECTION ( 'NONE',  ( 0.007781995580012663651, -3.146120232559066537E-19, -0.9999697198139514409 ) ) ;
#10211=VECTOR ( 'NONE', #33140, 1000.000000000000114 ) ;
#10213=CARTESIAN_POINT ( 'NONE',  ( 2.072287782118878319, 0.000000000000000000, -2.950529333540147015 ) ) ;
#10214=EDGE_CURVE ( 'NONE', #26440, #51840, #55194, .T. ) ;
#10215=CARTESIAN_POINT ( 'NONE',  ( -22.40634380310664397, 0.000000000000000000, 5.584705972946605534 ) ) ;
#10216=CARTESIAN_POINT ( 'NONE',  ( -16.37157077545227324, 4.333955019861511992, 2.902929945681169688 ) ) ;
#10217=ORIENTED_EDGE ( 'NONE', *, *, #33425, .F. ) ;
#10218=EDGE_CURVE ( 'NONE', #40214, #41786, #33059, .T. ) ;
#10219=VECTOR ( 'NONE', #39721, 1000.000000000000227 ) ;
#10220=VECTOR ( 'NONE', #49866, 1000.000000000000227 ) ;
#10221=EDGE_LOOP ( 'NONE', ( #391, #3333, #29745, #32440 ) ) ;
#10222=EDGE_CURVE ( 'NONE', #49166, #15338, #19724, .T. ) ;
#10223=CARTESIAN_POINT ( 'NONE',  ( -18.78542079201265125, -1.327505506330656893, 6.157489818200859943 ) ) ;
#10225=EDGE_CURVE ( 'NONE', #34831, #9919, #11489, .T. ) ;
#10226=ORIENTED_EDGE ( 'NONE', *, *, #37599, .F. ) ;
#10227=FACE_OUTER_BOUND ( 'NONE', #12130, .T. ) ;
#10228=VECTOR ( 'NONE', #35918, 1000.000000000000227 ) ;
#10229=ORIENTED_EDGE ( 'NONE', *, *, #27733, .F. ) ;
#10230=CARTESIAN_POINT ( 'NONE',  ( -17.08519138589328179, 4.010151117816509903, 10.09913083817650303 ) ) ;
#10231=AXIS2_PLACEMENT_3D ( 'NONE', #16236, #33553, #50864 ) ;
#10232=EDGE_CURVE ( 'NONE', #12750, #21737, #37049, .T. ) ;
#10233=VERTEX_POINT ( 'NONE', #50379 ) ;
#10234=ORIENTED_EDGE ( 'NONE', *, *, #35725, .T. ) ;
#10235=VERTEX_POINT ( 'NONE', #42130 ) ;
#10237=DIRECTION ( 'NONE',  ( 0.6427681459581294776, -0.7660444431189769032, 0.005002170337467562802 ) ) ;
#10238=PLANE ( 'NONE',  #10336 ) ;
#10239=VECTOR ( 'NONE', #21581, 1000.000000000000227 ) ;
#10240=CARTESIAN_POINT ( 'NONE',  ( -11.60535272280474928, 0.000000000000000000, 2.883431238151338505 ) ) ;
#10241=ORIENTED_EDGE ( 'NONE', *, *, #30459, .T. ) ;
#10242=EDGE_LOOP ( 'NONE', ( #48422, #5780, #52861, #24421 ) ) ;
#10243=VECTOR ( 'NONE', #23299, 1000.000000000000000 ) ;
#10244=CARTESIAN_POINT ( 'NONE',  ( -16.27128914543113680, 2.553033558614006715, 2.920797873763766095 ) ) ;
#10245=ORIENTED_EDGE ( 'NONE', *, *, #40525, .T. ) ;
#10246=AXIS2_PLACEMENT_3D ( 'NONE', #37526, #54845, #33293 ) ;
#10247=DIRECTION ( 'NONE',  ( 0.7660212471507180654, -0.6427876096865404731, 0.005961354470445141482 ) ) ;
#10248=ORIENTED_EDGE ( 'NONE', *, *, #306, .T. ) ;
#10249=FACE_OUTER_BOUND ( 'NONE', #51211, .T. ) ;
#10250=AXIS2_PLACEMENT_3D ( 'NONE', #28641, #36896, #28338 ) ;
#10251=AXIS2_PLACEMENT_3D ( 'NONE', #50644, #11736, #37287 ) ;
#10252=ORIENTED_EDGE ( 'NONE', *, *, #7228, .T. ) ;
#10253=LINE ( 'NONE', #23039, #26786 ) ;
#10254=VERTEX_POINT ( 'NONE', #2927 ) ;
#10255=AXIS2_PLACEMENT_3D ( 'NONE', #16296, #38158, #6972 ) ;
#10256=PLANE ( 'NONE',  #39975 ) ;
#10257=VECTOR ( 'NONE', #53443, 1000.000000000000227 ) ;
#10258=ORIENTED_EDGE ( 'NONE', *, *, #46522, .F. ) ;
#10259=DIRECTION ( 'NONE',  ( -0.7660212471507179544, -0.6427876096865405842, -0.005961354470445141482 ) ) ;
#10260=CARTESIAN_POINT ( 'NONE',  ( -19.42933299877883968, -1.003701604285656579, 4.396310540701692915 ) ) ;
#10261=CARTESIAN_POINT ( 'NONE',  ( -14.42059698451481076, 0.000000000000000000, 6.385517040825948953 ) ) ;
#10262=ORIENTED_EDGE ( 'NONE', *, *, #42309, .T. ) ;
#10263=EDGE_CURVE ( 'NONE', #4466, #31521, #55462, .T. ) ;
#10264=EDGE_CURVE ( 'NONE', #15700, #6398, #24811, .T. ) ;
#10265=DIRECTION ( 'NONE',  ( -0.3620778797217456546, 0.000000000000000000, -0.9321478471874540261 ) ) ;
#10266=CARTESIAN_POINT ( 'NONE',  ( -24.27063949748155380, 0.000000000000000000, 6.308861732390097288 ) ) ;
#10267=FACE_OUTER_BOUND ( 'NONE', #33335, .T. ) ;
#10268=VECTOR ( 'NONE', #43176, 1000.000000000000227 ) ;
#10269=FACE_OUTER_BOUND ( 'NONE', #23418, .T. ) ;
#10270=EDGE_CURVE ( 'NONE', #45526, #27480, #54350, .T. ) ;
#10271=AXIS2_PLACEMENT_3D ( 'NONE', #49285, #27723, #5563 ) ;
#10272=LINE ( 'NONE', #5450, #53943 ) ;
#10273=CARTESIAN_POINT ( 'NONE',  ( -13.85891992762947744, 5.143464774974011888, 10.70589822680017456 ) ) ;
#10275=EDGE_LOOP ( 'NONE', ( #30600, #25520, #28100, #56016 ) ) ;
#10276=FACE_OUTER_BOUND ( 'NONE', #1149, .T. ) ;
#10277=CARTESIAN_POINT ( 'NONE',  ( -22.40556560354864146, -0.1191753592594197858, 5.484709000965211523 ) ) ;
#10279=ORIENTED_EDGE ( 'NONE', *, *, #24220, .T. ) ;
#10280=DIRECTION ( 'NONE',  ( -0.005002170337468016433, -0.7660444431189770143, 0.6427681459581293666 ) ) ;
#10281=DIRECTION ( 'NONE',  ( -0.7660212471507179544, -0.6427876096865405842, -0.005961354470445141482 ) ) ;
#10282=ORIENTED_EDGE ( 'NONE', *, *, #627, .T. ) ;
#10283=VECTOR ( 'NONE', #7449, 999.9999999999998863 ) ;
#10284=DIRECTION ( 'NONE',  ( -0.5364919789714478471, 0.6444004775717705469, -0.5449076811759709926 ) ) ;
#10285=AXIS2_PLACEMENT_3D ( 'NONE', #10295, #18534, #5474 ) ;
#10286=CARTESIAN_POINT ( 'NONE',  ( -13.27065584551087163, 0.000000000000000000, 12.04557950825129176 ) ) ;
#10287=DIRECTION ( 'NONE',  ( 0.000000000000000000, -0.000000000000000000, -1.000000000000000000 ) ) ;
#10289=EDGE_LOOP ( 'NONE', ( #12962, #25822, #4722, #13527 ) ) ;
#10290=EDGE_CURVE ( 'NONE', #10918, #20122, #11189, .T. ) ;
#10291=CARTESIAN_POINT ( 'NONE',  ( -20.54204810873173415, 0.000000000000000000, 4.860550213503115558 ) ) ;
#10292=VECTOR ( 'NONE', #31420, 999.9999999999998863 ) ;
#10294=VECTOR ( 'NONE', #10881, 1000.000000000000000 ) ;
#10295=CARTESIAN_POINT ( 'NONE',  ( -19.60990026154428278, 0.000000000000000000, 4.498472333781370125 ) ) ;
#10296=VECTOR ( 'NONE', #32619, 999.9999999999998863 ) ;
#10297=EDGE_CURVE ( 'NONE', #15470, #38880, #15442, .T. ) ;
#10298=LINE ( 'NONE', #668, #52754 ) ;
#10299=VERTEX_POINT ( 'NONE', #46113 ) ;
#10300=PLANE ( 'NONE',  #55734 ) ;
#10301=VERTEX_POINT ( 'NONE', #28511 ) ;
#10302=FACE_OUTER_BOUND ( 'NONE', #51793, .T. ) ;
#10304=VECTOR ( 'NONE', #51986, 999.9999999999998863 ) ;
#10305=PLANE ( 'NONE',  #44179 ) ;
#10306=AXIS2_PLACEMENT_3D ( 'NONE', #38573, #25242, #51052 ) ;
#10307=EDGE_LOOP ( 'NONE', ( #8350, #52127, #45577, #32414, #28581 ) ) ;
#10309=DIRECTION ( 'NONE',  ( -0.005002170337468016433, -0.7660444431189770143, 0.6427681459581293666 ) ) ;
#10310=DIRECTION ( 'NONE',  ( 0.7660212471507180654, -0.6427876096865404731, 0.005961354470445141482 ) ) ;
#10311=EDGE_CURVE ( 'NONE', #36044, #38766, #2659, .T. ) ;
#10312=PLANE ( 'NONE',  #42998 ) ;
#10313=VERTEX_POINT ( 'NONE', #24519 ) ;
#10315=ADVANCED_FACE ( 'NONE', ( #3236 ), #7793, .F. ) ;
#10316=ORIENTED_EDGE ( 'NONE', *, *, #23588, .F. ) ;
#10317=ORIENTED_EDGE ( 'NONE', *, *, #6426, .T. ) ;
#10318=ORIENTED_EDGE ( 'NONE', *, *, #23176, .T. ) ;
#10319=DIRECTION ( 'NONE',  ( 0.000000000000000000, -0.000000000000000000, -1.000000000000000000 ) ) ;
#10320=AXIS2_PLACEMENT_3D ( 'NONE', #30150, #13116, #42639 ) ;
#10321=ORIENTED_EDGE ( 'NONE', *, *, #2727, .F. ) ;
#10322=DIRECTION ( 'NONE',  ( 0.5364919789714477361, 0.6444004775717706579, 0.5449076811759711036 ) ) ;
#10323=VERTEX_POINT ( 'NONE', #17700 ) ;
#10324=VECTOR ( 'NONE', #24625, 1000.000000000000227 ) ;
#10325=CARTESIAN_POINT ( 'NONE',  ( -10.23886491294503820, 0.000000000000000000, 6.418060246738034991 ) ) ;
#10326=CARTESIAN_POINT ( 'NONE',  ( -13.19506564939623416, 0.000000000000000000, 2.332401641178565299 ) ) ;
#10328=CARTESIAN_POINT ( 'NONE',  ( -16.53317331066696383, 0.000000000000000000, 13.31285208727739899 ) ) ;
#10329=VECTOR ( 'NONE', #9593, 1000.000000000000000 ) ;
#10330=ORIENTED_EDGE ( 'NONE', *, *, #22010, .T. ) ;
#10331=FACE_OUTER_BOUND ( 'NONE', #43244, .T. ) ;
#10332=FACE_OUTER_BOUND ( 'NONE', #28400, .T. ) ;
#10334=DIRECTION ( 'NONE',  ( 0.007781995580012662783, 0.000000000000000000, -0.9999697198139514409 ) ) ;
#10336=AXIS2_PLACEMENT_3D ( 'NONE', #14503, #32652, #40638 ) ;
#10337=CARTESIAN_POINT ( 'NONE',  ( -15.87975247367846166, 0.000000000000000000, 2.850166870931599927 ) ) ;
#10338=PLANE ( 'NONE',  #32000 ) ;
#10339=EDGE_LOOP ( 'NONE', ( #15890, #34009, #28167, #33381 ) ) ;
#10340=VECTOR ( 'NONE', #40298, 1000.000000000000227 ) ;
#10341=EDGE_CURVE ( 'NONE', #5277, #54540, #17403, .T. ) ;
#10342=VERTEX_POINT ( 'NONE', #21412 ) ;
#10343=CARTESIAN_POINT ( 'NONE',  ( -13.53673582514181106, 0.000000000000000000, 12.22817484722816772 ) ) ;
#10344=FACE_OUTER_BOUND ( 'NONE', #1092, .T. ) ;
#10345=ADVANCED_FACE ( 'NONE', ( #13451 ), #12873, .F. ) ;
#10346=ADVANCED_FACE ( 'NONE', ( #25378 ), #4080, .F. ) ;
#10347=PLANE ( 'NONE',  #8895 ) ;
#10348=VECTOR ( 'NONE', #31008, 1000.000000000000114 ) ;
#10349=VECTOR ( 'NONE', #19979, 1000.000000000000227 ) ;
#10350=FACE_OUTER_BOUND ( 'NONE', #36101, .T. ) ;
#10351=EDGE_LOOP ( 'NONE', ( #51359, #44346, #48086, #36876 ) ) ;
#10352=DIRECTION ( 'NONE',  ( 0.7660212471507180654, -0.6427876096865404731, 0.005961354470445141482 ) ) ;
#10353=PLANE ( 'NONE',  #49527 ) ;
#10354=ORIENTED_EDGE ( 'NONE', *, *, #8572, .T. ) ;
#10355=CARTESIAN_POINT ( 'NONE',  ( -19.73291444811881945, 0.000000000000000000, 6.513501371556814412 ) ) ;
#10357=ORIENTED_EDGE ( 'NONE', *, *, #37145, .F. ) ;
#10359=DIRECTION ( 'NONE',  ( 0.9999697198139515519, 0.000000000000000000, 0.007781995580013368816 ) ) ;
#10360=DIRECTION ( 'NONE',  ( 0.007781995580012662783, 0.000000000000000000, -0.9999697198139514409 ) ) ;
#10361=PLANE ( 'NONE',  #14218 ) ;
#10362=DIRECTION ( 'NONE',  ( -0.7660212471507179544, -0.6427876096865405842, -0.005961354470445141482 ) ) ;
#10363=VECTOR ( 'NONE', #7120, 1000.000000000000227 ) ;
#10364=EDGE_LOOP ( 'NONE', ( #684, #13775, #43678, #46694 ) ) ;
#10365=VECTOR ( 'NONE', #40122, 1000.000000000000227 ) ;
#10366=ORIENTED_EDGE ( 'NONE', *, *, #52527, .F. ) ;
#10367=CARTESIAN_POINT ( 'NONE',  ( -11.30636317915456779, -0.1191753592594197858, 11.32220194836580340 ) ) ;
#10368=CARTESIAN_POINT ( 'NONE',  ( -11.61054990949386401, 2.553033558614006715, 1.110408475155038266 ) ) ;
#10369=CARTESIAN_POINT ( 'NONE',  ( -18.83816797531202880, 4.495856970884011261, 3.855874544212809507 ) ) ;
#10370=VECTOR ( 'NONE', #18284, 1000.000000000000227 ) ;
#10371=LINE ( 'NONE', #31096, #53654 ) ;
#10372=LINE ( 'NONE', #54092, #35807 ) ;
#10373=VECTOR ( 'NONE', #54128, 1000.000000000000114 ) ;
#10374=ORIENTED_EDGE ( 'NONE', *, *, #53231, .T. ) ;
#10375=DIRECTION ( 'NONE',  ( 0.6427681459581294776, -0.7660444431189769032, 0.005002170337467562802 ) ) ;
#10376=EDGE_CURVE ( 'NONE', #43104, #4253, #13163, .T. ) ;
#10377=CARTESIAN_POINT ( 'NONE',  ( -9.808144436391993182, 0.000000000000000000, 10.77986332834118777 ) ) ;
#10378=DIRECTION ( 'NONE',  ( 0.3313982828793700097, 0.4028455766673916805, 0.8531650599175528704 ) ) ;
#10379=CARTESIAN_POINT ( 'NONE',  ( -28.92982233430281980, 0.000000000000000000, 7.919257187036034651 ) ) ;
#10381=EDGE_CURVE ( 'NONE', #30922, #22808, #52048, .T. ) ;
#10382=VECTOR ( 'NONE', #39442, 999.9999999999998863 ) ;
#10383=CARTESIAN_POINT ( 'NONE',  ( -20.14641686010442356, -0.1941918491731554619, 4.700677864147936980 ) ) ;
#10384=ORIENTED_EDGE ( 'NONE', *, *, #20693, .T. ) ;
#10385=DIRECTION ( 'NONE',  ( -0.005961354470445682716, -0.6427876096865404731, 0.7660212471507180654 ) ) ;
#10386=DIRECTION ( 'NONE',  ( -0.005002170337468016433, -0.7660444431189770143, 0.6427681459581293666 ) ) ;
#10387=VECTOR ( 'NONE', #38556, 999.9999999999998863 ) ;
#10388=ORIENTED_EDGE ( 'NONE', *, *, #42117, .T. ) ;
#10389=DIRECTION ( 'NONE',  ( 0.6427681459581294776, -0.7660444431189769032, 0.005002170337467562802 ) ) ;
#10390=EDGE_CURVE ( 'NONE', #13096, #18181, #30196, .T. ) ;
#10391=ORIENTED_EDGE ( 'NONE', *, *, #7947, .F. ) ;
#10393=ORIENTED_EDGE ( 'NONE', *, *, #10232, .T. ) ;
#10394=ORIENTED_EDGE ( 'NONE', *, *, #16164, .F. ) ;
#10395=DIRECTION ( 'NONE',  ( 0.5364919789714477361, 0.6444004775717706579, 0.5449076811759711036 ) ) ;
#10396=VECTOR ( 'NONE', #33108, 1000.000000000000000 ) ;
#10398=EDGE_LOOP ( 'NONE', ( #355, #48414, #9762, #55150 ) ) ;
#10400=LINE ( 'NONE', #27419, #49409 ) ;
#10401=VERTEX_POINT ( 'NONE', #47515 ) ;
#10402=EDGE_CURVE ( 'NONE', #22818, #11131, #42679, .T. ) ;
#10404=CARTESIAN_POINT ( 'NONE',  ( -21.47341775636118655, -0.1191753592594197858, 5.122631121243466090 ) ) ;
#10405=VERTEX_POINT ( 'NONE', #66 ) ;
#10406=EDGE_LOOP ( 'NONE', ( #54460, #41231, #37849, #19319, #2729 ) ) ;
#10407=EDGE_CURVE ( 'NONE', #21718, #38033, #9167, .T. ) ;
#10408=VECTOR ( 'NONE', #37743, 1000.000000000000227 ) ;
#10409=CARTESIAN_POINT ( 'NONE',  ( -12.57445172676405143, -1.165603555308157846, 1.728476342015877076 ) ) ;
#10410=AXIS2_PLACEMENT_3D ( 'NONE', #24690, #42013, #25834 ) ;
#10411=CARTESIAN_POINT ( 'NONE',  ( -12.17363884469051527, -0.1191753592594191197, 3.348343802064481789 ) ) ;
#10412=CARTESIAN_POINT ( 'NONE',  ( -10.41299237536028421, 0.000000000000000000, 3.092716518302152551 ) ) ;
#10413=LINE ( 'NONE', #27740, #13314 ) ;
#10414=EDGE_CURVE ( 'NONE', #23836, #42731, #34730, .T. ) ;
#10415=ORIENTED_EDGE ( 'NONE', *, *, #48040, .F. ) ;
#10416=CARTESIAN_POINT ( 'NONE',  ( -16.79925329029790149, 0.000000000000000000, 13.49544742625427496 ) ) ;
#10417=VECTOR ( 'NONE', #51675, 1000.000000000000227 ) ;
#10418=ORIENTED_EDGE ( 'NONE', *, *, #45294, .F. ) ;
#10419=EDGE_CURVE ( 'NONE', #46963, #24466, #43286, .T. ) ;
#10420=DIRECTION ( 'NONE',  ( 0.007781995580012662783, 0.000000000000000000, -0.9999697198139514409 ) ) ;
#10421=VECTOR ( 'NONE', #3682, 1000.000000000000227 ) ;
#10422=EDGE_CURVE ( 'NONE', #26242, #23457, #21102, .T. ) ;
#10423=CARTESIAN_POINT ( 'NONE',  ( -19.17768093937019458, -0.1191753592594166911, 7.725821564637509908 ) ) ;
#10424=CARTESIAN_POINT ( 'NONE',  ( -17.74482636761139531, -0.1191753592594203132, 3.674319602356484804 ) ) ;
#10425=LINE ( 'NONE', #33115, #44861 ) ;
#10426=DIRECTION ( 'NONE',  ( -0.5364919789714478471, 0.6444004775717705469, -0.5449076811759709926 ) ) ;
#10427=VECTOR ( 'NONE', #39925, 999.9999999999998863 ) ;
#10428=LINE ( 'NONE', #52717, #24993 ) ;
#10429=ORIENTED_EDGE ( 'NONE', *, *, #21474, .T. ) ;
#10430=DIRECTION ( 'NONE',  ( 0.007781995580012662783, 0.000000000000000000, -0.9999697198139514409 ) ) ;
#10431=ORIENTED_EDGE ( 'NONE', *, *, #6663, .T. ) ;
#10432=VECTOR ( 'NONE', #46030, 1000.000000000000114 ) ;
#10433=ADVANCED_FACE ( 'NONE', ( #26483 ), #16870, .F. ) ;
#10434=LINE ( 'NONE', #14964, #49253 ) ;
#10435=CARTESIAN_POINT ( 'NONE',  ( -14.46888367232926420, 0.000000000000000000, 12.59025272694991315 ) ) ;
#10436=ADVANCED_FACE ( 'NONE', ( #51215 ), #51764, .F. ) ;
#10437=DIRECTION ( 'NONE',  ( 0.005961354470445682716, -0.6427876096865404731, -0.7660212471507180654 ) ) ;
#10438=DIRECTION ( 'NONE',  ( 0.9999697198139515519, 0.000000000000000000, 0.007781995580013368816 ) ) ;
#10439=LINE ( 'NONE', #1334, #54977 ) ;
#10440=EDGE_CURVE ( 'NONE', #51521, #48984, #8069, .T. ) ;
#10441=VECTOR ( 'NONE', #5835, 999.9999999999998863 ) ;
#10442=DIRECTION ( 'NONE',  ( -0.7660212471507179544, -0.6427876096865405842, -0.005961354470445141482 ) ) ;
#10443=AXIS2_PLACEMENT_3D ( 'NONE', #35625, #1802, #40992 ) ;
#10444=ORIENTED_EDGE ( 'NONE', *, *, #3800, .F. ) ;
#10445=DIRECTION ( 'NONE',  ( 0.000000000000000000, -1.000000000000000000, 0.000000000000000000 ) ) ;
#10446=CARTESIAN_POINT ( 'NONE',  ( -17.73140113748535285, 0.000000000000000000, 13.85752530597602039 ) ) ;
#10447=CARTESIAN_POINT ( 'NONE',  ( -13.22093213094377617, 0.000000000000000000, 5.656188970498445379 ) ) ;
#10448=LINE ( 'NONE', #48793, #40966 ) ;
#10449=DIRECTION ( 'NONE',  ( 0.6427681459581294776, -0.7660444431189769032, 0.005002170337467562802 ) ) ;
#10450=CARTESIAN_POINT ( 'NONE',  ( -15.62927958056622657, 0.1245042932765045296, 3.156596835203342888 ) ) ;
#10451=FACE_OUTER_BOUND ( 'NONE', #35147, .T. ) ;
#10452=VECTOR ( 'NONE', #38801, 1000.000000000000227 ) ;
#10453=CARTESIAN_POINT ( 'NONE',  ( -10.07782610008833757, 0.000000000000000000, 1.048658454501847137 ) ) ;
#10454=DIRECTION ( 'NONE',  ( 0.9999697198139515519, 0.000000000000000000, 0.007781995580013368816 ) ) ;
#10455=VECTOR ( 'NONE', #260, 1000.000000000000227 ) ;
#10456=VERTEX_POINT ( 'NONE', #29669 ) ;
#10457=ADVANCED_FACE ( 'NONE', ( #38431 ), #34201, .F. ) ;
#10458=VECTOR ( 'NONE', #29641, 1000.000000000000227 ) ;
#10459=ORIENTED_EDGE ( 'NONE', *, *, #29882, .F. ) ;
#10461=VECTOR ( 'NONE', #51354, 999.9999999999998863 ) ;
#10462=VECTOR ( 'NONE', #34710, 999.9999999999998863 ) ;
#10463=ORIENTED_EDGE ( 'NONE', *, *, #9529, .T. ) ;
#10464=VECTOR ( 'NONE', #19071, 999.9999999999998863 ) ;
#10465=ORIENTED_EDGE ( 'NONE', *, *, #23803, .F. ) ;
#10466=LINE ( 'NONE', #28052, #20561 ) ;
#10467=LINE ( 'NONE', #24073, #43044 ) ;
#10468=VECTOR ( 'NONE', #50209, 1000.000000000000227 ) ;
#10470=ORIENTED_EDGE ( 'NONE', *, *, #25977, .T. ) ;
#10471=VERTEX_POINT ( 'NONE', #40401 ) ;
#10472=VERTEX_POINT ( 'NONE', #31019 ) ;
#10473=ADVANCED_FACE ( 'NONE', ( #6319 ), #44940, .F. ) ;
#10474=EDGE_CURVE ( 'NONE', #27150, #8639, #18832, .T. ) ;
#10475=VECTOR ( 'NONE', #861, 999.9999999999998863 ) ;
#10476=VECTOR ( 'NONE', #53702, 999.9999999999998863 ) ;
#10478=LINE ( 'NONE', #24084, #3813 ) ;
#10479=CARTESIAN_POINT ( 'NONE',  ( -15.40103151951671734, 0.000000000000000000, 12.95233060667165681 ) ) ;
#10480=VERTEX_POINT ( 'NONE', #1195 ) ;
#10481=LINE ( 'NONE', #27807, #47349 ) ;
#10482=ORIENTED_EDGE ( 'NONE', *, *, #18001, .F. ) ;
#10483=FACE_OUTER_BOUND ( 'NONE', #50034, .T. ) ;
#10484=EDGE_CURVE ( 'NONE', #27583, #47452, #40686, .T. ) ;
#10485=DIRECTION ( 'NONE',  ( 0.9999697198139515519, 0.000000000000000000, 0.007781995580013368816 ) ) ;
#10486=ADVANCED_FACE ( 'NONE', ( #44634 ), #27062, .F. ) ;
#10488=DIRECTION ( 'NONE',  ( -0.5364919789714478471, 0.6444004775717705469, -0.5449076811759709926 ) ) ;
#10489=DIRECTION ( 'NONE',  ( 0.9999697198139515519, 0.000000000000000000, 0.007781995580013368816 ) ) ;
#10490=DIRECTION ( 'NONE',  ( -0.005961354470445682716, -0.6427876096865404731, 0.7660212471507180654 ) ) ;
#10491=LINE ( 'NONE', #10762, #53747 ) ;
#10492=CARTESIAN_POINT ( 'NONE',  ( -10.94028622754223967, 0.000000000000000000, 11.14038480894692995 ) ) ;
#10493=VECTOR ( 'NONE', #45573, 999.9999999999998863 ) ;
#10494=ORIENTED_EDGE ( 'NONE', *, *, #16262, .T. ) ;
#10495=PLANE ( 'NONE',  #34644 ) ;
#10496=VERTEX_POINT ( 'NONE', #31610 ) ;
#10497=AXIS2_PLACEMENT_3D ( 'NONE', #22913, #27755, #10128 ) ;
#10498=EDGE_CURVE ( 'NONE', #19093, #21379, #6059, .T. ) ;
#10499=CARTESIAN_POINT ( 'NONE',  ( -13.27065584551087163, 0.000000000000000000, 12.04557950825129176 ) ) ;
#10500=DIRECTION ( 'NONE',  ( 0.007781995580012663651, -3.146120232559066537E-19, -0.9999697198139514409 ) ) ;
#10501=FACE_OUTER_BOUND ( 'NONE', #32533, .T. ) ;
#10502=FACE_OUTER_BOUND ( 'NONE', #4313, .T. ) ;
#10503=VECTOR ( 'NONE', #38916, 1000.000000000000114 ) ;
#10504=CARTESIAN_POINT ( 'NONE',  ( -17.66531893442506629, -2.784623065533161856, 3.654286853175606975 ) ) ;
#10505=DIRECTION ( 'NONE',  ( 0.000000000000000000, -0.000000000000000000, -1.000000000000000000 ) ) ;
#10506=LINE ( 'NONE', #42194, #40660 ) ;
#10507=EDGE_CURVE ( 'NONE', #19751, #2789, #48340, .T. ) ;
#10508=LINE ( 'NONE', #36609, #33747 ) ;
#10509=VECTOR ( 'NONE', #22749, 1000.000000000000000 ) ;
#10510=VECTOR ( 'NONE', #38531, 1000.000000000000000 ) ;
#10511=DIRECTION ( 'NONE',  ( -0.6427681459581293666, -0.7660444431189770143, -0.005002170337467561935 ) ) ;
#10512=ORIENTED_EDGE ( 'NONE', *, *, #28360, .T. ) ;
#10513=DIRECTION ( 'NONE',  ( 0.007781995580012663651, -3.146120232559066537E-19, -0.9999697198139514409 ) ) ;
#10514=CARTESIAN_POINT ( 'NONE',  ( -28.93137873341882127, 0.000000000000000000, 8.119251130998824451 ) ) ;
#10515=PLANE ( 'NONE',  #45437 ) ;
#10516=CARTESIAN_POINT ( 'NONE',  ( 2.072287782118878319, 0.000000000000000000, -2.950529333540147015 ) ) ;
#10517=VECTOR ( 'NONE', #8508, 1000.000000000000227 ) ;
#10518=CARTESIAN_POINT ( 'NONE',  ( -12.90429806846666061, -1.003701604285656579, 1.861765382649475553 ) ) ;
#10519=AXIS2_PLACEMENT_3D ( 'NONE', #17263, #3927, #38580 ) ;
#10520=DIRECTION ( 'NONE',  ( 0.5449076811759707706, 0.6444004775717708799, -0.5364919789714476250 ) ) ;
#10521=CARTESIAN_POINT ( 'NONE',  ( -28.93137873341882127, 0.000000000000000000, 8.119251130998824451 ) ) ;
#10522=CARTESIAN_POINT ( 'NONE',  ( -3.486932065698848504, -6.851436116247921149, -1.863930744634968883 ) ) ;
#10523=ORIENTED_EDGE ( 'NONE', *, *, #10711, .F. ) ;
#10524=VECTOR ( 'NONE', #20580, 1000.000000000000227 ) ;
#10525=AXIS2_PLACEMENT_3D ( 'NONE', #51891, #40808, #49870 ) ;
#10526=EDGE_LOOP ( 'NONE', ( #44658, #383, #33962, #43554 ) ) ;
#10527=DIRECTION ( 'NONE',  ( 0.9999697198139515519, 0.000000000000000000, 0.007781995580013368816 ) ) ;
#10529=ORIENTED_EDGE ( 'NONE', *, *, #51808, .F. ) ;
#10530=CARTESIAN_POINT ( 'NONE',  ( -12.73212453470555872, -2.460819163488159766, 1.748397656112330667 ) ) ;
#10531=EDGE_CURVE ( 'NONE', #5703, #31643, #14551, .T. ) ;
#10532=ORIENTED_EDGE ( 'NONE', *, *, #107, .F. ) ;
#10535=ORIENTED_EDGE ( 'NONE', *, *, #42059, .T. ) ;
#10536=ORIENTED_EDGE ( 'NONE', *, *, #32826, .F. ) ;
#10537=ADVANCED_FACE ( 'NONE', ( #53714 ), #14834, .F. ) ;
#10538=ORIENTED_EDGE ( 'NONE', *, *, #25966, .F. ) ;
#10539=EDGE_CURVE ( 'NONE', #30584, #16783, #32161, .T. ) ;
#10540=CARTESIAN_POINT ( 'NONE',  ( -20.50469437842130915, -0.007300641194113378224, 4.854714758035273192 ) ) ;
#10541=CARTESIAN_POINT ( 'NONE',  ( -13.59054196325603137, -0.1191753592594179401, 6.291973692822567799 ) ) ;
#10542=VECTOR ( 'NONE', #47567, 999.9999999999998863 ) ;
#10543=LINE ( 'NONE', #19607, #20290 ) ;
#10544=EDGE_CURVE ( 'NONE', #27553, #49693, #40106, .T. ) ;
#10545=EDGE_CURVE ( 'NONE', #33893, #19103, #31866, .T. ) ;
#10547=ORIENTED_EDGE ( 'NONE', *, *, #704, .F. ) ;
#10548=VECTOR ( 'NONE', #36323, 1000.000000000000000 ) ;
#10549=EDGE_LOOP ( 'NONE', ( #3802, #6405, #19149, #11272 ) ) ;
#10550=ADVANCED_FACE ( 'NONE', ( #51637 ), #12482, .F. ) ;
#10551=VECTOR ( 'NONE', #24639, 999.9999999999998863 ) ;
#10552=VECTOR ( 'NONE', #48379, 999.9999999999998863 ) ;
#10553=LINE ( 'NONE', #10244, #996 ) ;
#10554=VERTEX_POINT ( 'NONE', #46518 ) ;
#10555=FACE_OUTER_BOUND ( 'NONE', #26206, .T. ) ;
#10556=ORIENTED_EDGE ( 'NONE', *, *, #35188, .T. ) ;
#10557=PLANE ( 'NONE',  #42072 ) ;
#10558=DIRECTION ( 'NONE',  ( 0.007781995580012663651, 0.000000000000000000, -0.9999697198139515519 ) ) ;
#10559=VECTOR ( 'NONE', #11780, 1000.000000000000000 ) ;
#10560=VERTEX_POINT ( 'NONE', #42290 ) ;
#10561=AXIS2_PLACEMENT_3D ( 'NONE', #50182, #20072, #11587 ) ;
#10562=LINE ( 'NONE', #49144, #34049 ) ;
#10563=EDGE_CURVE ( 'NONE', #18224, #34747, #30061, .T. ) ;
#10564=VECTOR ( 'NONE', #23090, 1000.000000000000114 ) ;
#10565=EDGE_CURVE ( 'NONE', #16295, #47558, #29203, .T. ) ;
#10566=CARTESIAN_POINT ( 'NONE',  ( -8.704071095609336339, 0.000000000000000000, 6.599330380697081999 ) ) ;
#10568=ORIENTED_EDGE ( 'NONE', *, *, #31577, .T. ) ;
#10571=ADVANCED_FACE ( 'NONE', ( #20113 ), #25252, .F. ) ;
#10572=DIRECTION ( 'NONE',  ( -0.5364919789714478471, 0.6444004775717705469, -0.5449076811759709926 ) ) ;
#10573=ORIENTED_EDGE ( 'NONE', *, *, #3302, .F. ) ;
#10574=EDGE_CURVE ( 'NONE', #14055, #44098, #43134, .T. ) ;
#10575=CARTESIAN_POINT ( 'NONE',  ( -19.69569380384165669, -0.1191753592594177458, 14.58090286586150697 ) ) ;
#10576=DIRECTION ( 'NONE',  ( -0.005002170337468016433, -0.7660444431189770143, 0.6427681459581293666 ) ) ;
#10577=DIRECTION ( 'NONE',  ( 0.007781995580012663651, -3.146120232559066537E-19, -0.9999697198139514409 ) ) ;
#10578=PLANE ( 'NONE',  #19567 ) ;
#10579=LINE ( 'NONE', #22765, #21322 ) ;
#10580=CARTESIAN_POINT ( 'NONE',  ( -19.12962290826653700, 0.000000000000000000, 14.40064212555863854 ) ) ;
#10583=ORIENTED_EDGE ( 'NONE', *, *, #12125, .F. ) ;
#10585=LINE ( 'NONE', #31852, #50390 ) ;
#10588=DIRECTION ( 'NONE',  ( 0.6427681459581294776, -0.7660444431189769032, 0.005002170337467562802 ) ) ;
#10589=DIRECTION ( 'NONE',  ( 0.000000000000000000, -1.000000000000000000, 0.000000000000000000 ) ) ;
#10590=AXIS2_PLACEMENT_3D ( 'NONE', #3989, #21317, #37504 ) ;
#10591=AXIS2_PLACEMENT_3D ( 'NONE', #47221, #29923, #664 ) ;
#10592=DIRECTION ( 'NONE',  ( 0.005961354470445682716, -0.6427876096865404731, -0.7660212471507180654 ) ) ;
#10593=LINE ( 'NONE', #44093, #580 ) ;
#10594=PLANE ( 'NONE',  #24738 ) ;
#10595=EDGE_LOOP ( 'NONE', ( #46447, #6066, #33364, #31692 ) ) ;
#10596=AXIS2_PLACEMENT_3D ( 'NONE', #2991, #3838, #42482 ) ;
#10597=ORIENTED_EDGE ( 'NONE', *, *, #11495, .T. ) ;
#10598=LINE ( 'NONE', #32449, #37719 ) ;
#10600=DIRECTION ( 'NONE',  ( 0.005002170337468016433, -0.7660444431189770143, -0.6427681459581293666 ) ) ;
#10601=VECTOR ( 'NONE', #53490, 999.9999999999998863 ) ;
#10602=ORIENTED_EDGE ( 'NONE', *, *, #42906, .T. ) ;
#10603=LINE ( 'NONE', #27920, #42154 ) ;
#10604=ADVANCED_FACE ( 'NONE', ( #16423 ), #50529, .F. ) ;
#10605=ORIENTED_EDGE ( 'NONE', *, *, #24751, .F. ) ;
#10606=CARTESIAN_POINT ( 'NONE',  ( -24.27063949748155380, 0.000000000000000000, 6.308861732390097288 ) ) ;
#10607=AXIS2_PLACEMENT_3D ( 'NONE', #18122, #540, #26360 ) ;
#10608=VECTOR ( 'NONE', #23000, 999.9999999999998863 ) ;
#10609=EDGE_CURVE ( 'NONE', #26301, #50967, #51065, .T. ) ;
#10610=ORIENTED_EDGE ( 'NONE', *, *, #19588, .F. ) ;
#10611=DIRECTION ( 'NONE',  ( 0.7660212471507180654, -0.6427876096865404731, 0.005961354470445141482 ) ) ;
#10612=CARTESIAN_POINT ( 'NONE',  ( -10.94028622754223967, 0.000000000000000000, 11.14038480894692995 ) ) ;
#10613=FACE_OUTER_BOUND ( 'NONE', #10364, .T. ) ;
#10615=EDGE_CURVE ( 'NONE', #44163, #27792, #37448, .T. ) ;
#10616=ADVANCED_FACE ( 'NONE', ( #25807 ), #38285, .F. ) ;
#10617=ORIENTED_EDGE ( 'NONE', *, *, #52180, .T. ) ;
#10618=DIRECTION ( 'NONE',  ( -0.005002170337468016433, -0.7660444431189770143, 0.6427681459581293666 ) ) ;
#10619=ORIENTED_EDGE ( 'NONE', *, *, #48503, .F. ) ;
#10620=EDGE_CURVE ( 'NONE', #8057, #17431, #55612, .T. ) ;
#10621=VECTOR ( 'NONE', #29562, 1000.000000000000114 ) ;
#10622=ORIENTED_EDGE ( 'NONE', *, *, #4348, .F. ) ;
#10624=DIRECTION ( 'NONE',  ( -0.5449076811759708816, 0.6444004775717707689, 0.5364919789714475140 ) ) ;
#10625=ORIENTED_EDGE ( 'NONE', *, *, #42333, .T. ) ;
#10626=FACE_OUTER_BOUND ( 'NONE', #36386, .T. ) ;
#10627=ORIENTED_EDGE ( 'NONE', *, *, #38292, .T. ) ;
#10628=CARTESIAN_POINT ( 'NONE',  ( -17.86730109935463418, 0.000000000000000000, 5.620029852818350768 ) ) ;
#10629=CARTESIAN_POINT ( 'NONE',  ( -20.54204810873173415, 0.000000000000000000, 4.860550213503115558 ) ) ;
#10630=ORIENTED_EDGE ( 'NONE', *, *, #43632, .T. ) ;
#10631=AXIS2_PLACEMENT_3D ( 'NONE', #53281, #14372, #41585 ) ;
#10632=DIRECTION ( 'NONE',  ( 0.5449076811759707706, 0.6444004775717708799, -0.5364919789714476250 ) ) ;
#10633=ORIENTED_EDGE ( 'NONE', *, *, #57, .T. ) ;
#10634=EDGE_CURVE ( 'NONE', #9106, #8391, #34334, .T. ) ;
#10635=VECTOR ( 'NONE', #47575, 1000.000000000000227 ) ;
#10636=DIRECTION ( 'NONE',  ( 0.7660212471507180654, -0.6427876096865404731, 0.005961354470445141482 ) ) ;
#10637=DIRECTION ( 'NONE',  ( 0.6246952433987894571, -0.7422098413412800966, -0.2426528472758541777 ) ) ;
#10638=LINE ( 'NONE', #19693, #37738 ) ;
#10639=CARTESIAN_POINT ( 'NONE',  ( -21.47263955680318404, 0.000000000000000000, 5.022634149262071190 ) ) ;
#10640=EDGE_CURVE ( 'NONE', #28121, #29147, #41982, .T. ) ;
#10641=DIRECTION ( 'NONE',  ( -0.7660212471507179544, -0.6427876096865405842, -0.005961354470445141482 ) ) ;
#10642=CARTESIAN_POINT ( 'NONE',  ( -10.88182098009593446, 0.000000000000000000, 3.627726069086881111 ) ) ;
#10643=CARTESIAN_POINT ( 'NONE',  ( -16.84795344307834597, -1.813211359398159583, 3.367787457811957541 ) ) ;
#10644=EDGE_LOOP ( 'NONE', ( #54429, #10007, #37902, #51704 ) ) ;
#10645=ADVANCED_FACE ( 'NONE', ( #55328 ), #3084, .F. ) ;
#10646=ORIENTED_EDGE ( 'NONE', *, *, #5863, .T. ) ;
#10647=VECTOR ( 'NONE', #49908, 999.9999999999998863 ) ;
#10648=LINE ( 'NONE', #10053, #45469 ) ;
#10649=LINE ( 'NONE', #40151, #22156 ) ;
#10650=LINE ( 'NONE', #23664, #52079 ) ;
#10651=EDGE_CURVE ( 'NONE', #8988, #27291, #47096, .T. ) ;
#10652=LINE ( 'NONE', #41816, #44197 ) ;
#10654=CARTESIAN_POINT ( 'NONE',  ( -15.50102849149811135, -0.1191753592594197858, 12.95155240711365430 ) ) ;
#10655=EDGE_LOOP ( 'NONE', ( #46778, #11000, #25695, #4435 ) ) ;
#10656=DIRECTION ( 'NONE',  ( -0.6427681459581293666, -0.7660444431189770143, -0.005002170337467561935 ) ) ;
#10657=FACE_OUTER_BOUND ( 'NONE', #27131, .T. ) ;
#10658=ORIENTED_EDGE ( 'NONE', *, *, #10725, .F. ) ;
#10659=CARTESIAN_POINT ( 'NONE',  ( -32.65997012216863737, 0.000000000000000000, 9.567562649885804404 ) ) ;
#10660=CARTESIAN_POINT ( 'NONE',  ( -18.39746900504187010, 0.000000000000000000, 14.03700784672088808 ) ) ;
#10661=ORIENTED_EDGE ( 'NONE', *, *, #37111, .F. ) ;
#10662=DIRECTION ( 'NONE',  ( 0.000000000000000000, -1.000000000000000000, 0.000000000000000000 ) ) ;
#10663=DIRECTION ( 'NONE',  ( 0.9999697198139515519, 0.000000000000000000, 0.007781995580013368816 ) ) ;
#10664=PLANE ( 'NONE',  #17765 ) ;
#10665=CARTESIAN_POINT ( 'NONE',  ( -17.56503730440392985, -1.003701604285657911, 3.672154781258202050 ) ) ;
#10666=LINE ( 'NONE', #37295, #7477 ) ;
#10667=ORIENTED_EDGE ( 'NONE', *, *, #27734, .T. ) ;
#10669=DIRECTION ( 'NONE',  ( 0.005961354470445682716, -0.6427876096865404731, -0.7660212471507180654 ) ) ;
#10670=DIRECTION ( 'NONE',  ( 0.7660212471507180654, -0.6427876096865404731, 0.005961354470445141482 ) ) ;
#10671=DIRECTION ( 'NONE',  ( 0.007781995580012662783, 0.000000000000000000, -0.9999697198139514409 ) ) ;
#10673=CARTESIAN_POINT ( 'NONE',  ( -14.16876790004692843, 0.000000000000000000, 8.034131125803988027 ) ) ;
#10674=ORIENTED_EDGE ( 'NONE', *, *, #14688, .T. ) ;
#10675=CARTESIAN_POINT ( 'NONE',  ( -16.95946333459872335, 0.000000000000000000, 8.381745358453697392 ) ) ;
#10676=CARTESIAN_POINT ( 'NONE',  ( -11.67244013076689946, 0.000000000000000000, 11.50401908778467863 ) ) ;
#10677=VECTOR ( 'NONE', #27695, 999.9999999999998863 ) ;
#10678=CARTESIAN_POINT ( 'NONE',  ( -18.14344026625406414, 0.000000000000000000, 7.095209153197401086 ) ) ;
#10679=ORIENTED_EDGE ( 'NONE', *, *, #21719, .F. ) ;
#10680=DIRECTION ( 'NONE',  ( 0.000000000000000000, -1.000000000000000000, 0.000000000000000000 ) ) ;
#10681=ORIENTED_EDGE ( 'NONE', *, *, #38628, .F. ) ;
#10682=PLANE ( 'NONE',  #25920 ) ;
#10683=LINE ( 'NONE', #19993, #22088 ) ;
#10684=ADVANCED_FACE ( 'NONE', ( #50787 ), #42824, .F. ) ;
#10685=ORIENTED_EDGE ( 'NONE', *, *, #41044, .F. ) ;
#10686=VECTOR ( 'NONE', #19124, 1000.000000000000114 ) ;
#10687=CARTESIAN_POINT ( 'NONE',  ( -13.53673582514181106, 0.000000000000000000, 12.22817484722816772 ) ) ;
#10689=ADVANCED_FACE ( 'NONE', ( #5355 ), #39972, .F. ) ;
#10690=EDGE_CURVE ( 'NONE', #54495, #10471, #9620, .T. ) ;
#10691=ORIENTED_EDGE ( 'NONE', *, *, #5500, .F. ) ;
#10692=ORIENTED_EDGE ( 'NONE', *, *, #11758, .T. ) ;
#10693=DIRECTION ( 'NONE',  ( -0.005002170337468016433, -0.7660444431189770143, 0.6427681459581293666 ) ) ;
#10694=VERTEX_POINT ( 'NONE', #5076 ) ;
#10695=ORIENTED_EDGE ( 'NONE', *, *, #32286, .F. ) ;
#10697=ORIENTED_EDGE ( 'NONE', *, *, #28059, .T. ) ;
#10698=ORIENTED_EDGE ( 'NONE', *, *, #2086, .T. ) ;
#10699=DIRECTION ( 'NONE',  ( -0.9999697198139514409, -0.000000000000000000, -0.007781995580013368816 ) ) ;
#10700=VERTEX_POINT ( 'NONE', #1057 ) ;
#10701=ORIENTED_EDGE ( 'NONE', *, *, #37827, .T. ) ;
#10702=CARTESIAN_POINT ( 'NONE',  ( -19.13459676410571220, -3.917936722690661178, 10.54446056703513790 ) ) ;
#10703=DIRECTION ( 'NONE',  ( 0.000000000000000000, -0.000000000000000000, -1.000000000000000000 ) ) ;
#10704=CARTESIAN_POINT ( 'NONE',  ( -17.83139810946674686, -0.1191753592594197858, 13.85674710641801788 ) ) ;
#10705=CARTESIAN_POINT ( 'NONE',  ( -14.69949350034596414, -4.727446477803161073, 10.15025926240234178 ) ) ;
#10707=DIRECTION ( 'NONE',  ( 0.007781995580012662783, 0.000000000000000000, -0.9999697198139514409 ) ) ;
#10709=VERTEX_POINT ( 'NONE', #14161 ) ;
#10710=FACE_OUTER_BOUND ( 'NONE', #19892, .T. ) ;
#10711=EDGE_CURVE ( 'NONE', #36870, #26056, #22101, .T. ) ;
#10712=DIRECTION ( 'NONE',  ( 0.000000000000000000, -0.000000000000000000, -1.000000000000000000 ) ) ;
#10713=CARTESIAN_POINT ( 'NONE',  ( -23.33771345073609638, -0.1191753592594197858, 5.846786880686956955 ) ) ;
#10715=CARTESIAN_POINT ( 'NONE',  ( -14.93495759592298988, 0.000000000000000000, 12.77129166681078409 ) ) ;
#10716=DIRECTION ( 'NONE',  ( 0.007781995580012662783, 0.000000000000000000, -0.9999697198139514409 ) ) ;
#10718=DIRECTION ( 'NONE',  ( 0.2426528472758541499, 0.7422098413412800966, 0.6246952433987894571 ) ) ;
#10719=EDGE_CURVE ( 'NONE', #50938, #47436, #56185, .T. ) ;
#10720=ORIENTED_EDGE ( 'NONE', *, *, #7365, .T. ) ;
#10721=VECTOR ( 'NONE', #44077, 1000.000000000000114 ) ;
#10722=CARTESIAN_POINT ( 'NONE',  ( -24.26986129792355129, -0.1191753592594197858, 6.208864760408702388 ) ) ;
#10724=FACE_OUTER_BOUND ( 'NONE', #20728, .T. ) ;
#10725=EDGE_CURVE ( 'NONE', #6678, #50665, #34590, .T. ) ;
#10726=LINE ( 'NONE', #2709, #46733 ) ;
#10727=CARTESIAN_POINT ( 'NONE',  ( -17.87592325987048270, 0.000000000000000000, 6.727958962591642944 ) ) ;
#10728=ORIENTED_EDGE ( 'NONE', *, *, #35662, .F. ) ;
#10729=DIRECTION ( 'NONE',  ( 0.5449076811759707706, 0.6444004775717708799, -0.5364919789714476250 ) ) ;
#10730=LINE ( 'NONE', #1885, #51209 ) ;
#10731=PLANE ( 'NONE',  #17312 ) ;
#10732=DIRECTION ( 'NONE',  ( 0.6427681459581294776, -0.7660444431189769032, 0.005002170337467562802 ) ) ;
#10733=CARTESIAN_POINT ( 'NONE',  ( -15.30154763612674707, 0.2864062442990046309, 3.295003302109830390 ) ) ;
#10734=CARTESIAN_POINT ( 'NONE',  ( -22.40634380310664397, 0.000000000000000000, 5.584705972946605534 ) ) ;
#10735=DIRECTION ( 'NONE',  ( -0.5449076811759708816, 0.6444004775717707689, 0.5364919789714475140 ) ) ;
#10737=LINE ( 'NONE', #23504, #13818 ) ;
#10738=EDGE_CURVE ( 'NONE', #28378, #18922, #22405, .T. ) ;
#10739=ORIENTED_EDGE ( 'NONE', *, *, #21587, .F. ) ;
#10740=ADVANCED_FACE ( 'NONE', ( #523 ), #39720, .F. ) ;
#10741=ORIENTED_EDGE ( 'NONE', *, *, #23995, .T. ) ;
#10742=ORIENTED_EDGE ( 'NONE', *, *, #55208, .F. ) ;
#10743=ORIENTED_EDGE ( 'NONE', *, *, #2266, .F. ) ;
#10744=ORIENTED_EDGE ( 'NONE', *, *, #36294, .F. ) ;
#10745=DIRECTION ( 'NONE',  ( 0.007781995580012662783, 0.000000000000000000, -0.9999697198139514409 ) ) ;
#10746=LINE ( 'NONE', #20657, #39404 ) ;
#10747=AXIS2_PLACEMENT_3D ( 'NONE', #9669, #35775, #30399 ) ;
#10748=EDGE_LOOP ( 'NONE', ( #48249, #47888, #31824, #23431 ) ) ;
#10749=CARTESIAN_POINT ( 'NONE',  ( -16.96964189423057334, 0.000000000000000000, 9.689668412189776703 ) ) ;
#10750=ORIENTED_EDGE ( 'NONE', *, *, #41456, .F. ) ;
#10751=EDGE_CURVE ( 'NONE', #21963, #49166, #35436, .T. ) ;
#10753=FACE_OUTER_BOUND ( 'NONE', #34600, .T. ) ;
#10754=LINE ( 'NONE', #24616, #19579 ) ;
#10756=DIRECTION ( 'NONE',  ( 0.007781995580012662783, 0.000000000000000000, -0.9999697198139514409 ) ) ;
#10757=DIRECTION ( 'NONE',  ( 0.6427681459581294776, -0.7660444431189769032, 0.005002170337467562802 ) ) ;
#10758=LINE ( 'NONE', #22685, #29369 ) ;
#10759=CARTESIAN_POINT ( 'NONE',  ( -25.20278734466900517, 0.000000000000000000, 6.670939612111840944 ) ) ;
#10760=LINE ( 'NONE', #54444, #9703 ) ;
#10761=LINE ( 'NONE', #23531, #41295 ) ;
#10762=CARTESIAN_POINT ( 'NONE',  ( -9.342070512798265725, 0.000000000000000000, 10.59882438848031505 ) ) ;
#10763=CARTESIAN_POINT ( 'NONE',  ( -20.16176772743538237, -0.1191753592594197858, 14.76194180572237968 ) ) ;
#10764=LINE ( 'NONE', #36593, #14794 ) ;
#10765=VERTEX_POINT ( 'NONE', #43407 ) ;
#10766=DIRECTION ( 'NONE',  ( -0.6427681459581293666, -0.7660444431189770143, -0.005002170337467561935 ) ) ;
#10767=ORIENTED_EDGE ( 'NONE', *, *, #24998, .F. ) ;
#10768=CARTESIAN_POINT ( 'NONE',  ( -11.75290974440948766, -0.1191753592594203132, 7.783602850887407776 ) ) ;
#10769=DIRECTION ( 'NONE',  ( 0.7660212471507180654, -0.6427876096865404731, 0.005961354470445141482 ) ) ;
#10770=LINE ( 'NONE', #15031, #19515 ) ;
#10772=ADVANCED_FACE ( 'NONE', ( #21815 ), #34891, .F. ) ;
#10773=LINE ( 'NONE', #32617, #32313 ) ;
#10774=LINE ( 'NONE', #40860, #54872 ) ;
#10775=PLANE ( 'NONE',  #55158 ) ;
#10776=DIRECTION ( 'NONE',  ( -0.6427681459581293666, -0.7660444431189770143, -0.005002170337467561935 ) ) ;
#10777=CARTESIAN_POINT ( 'NONE',  ( -15.40103151951671734, 0.000000000000000000, 12.95233060667165681 ) ) ;
#10778=CARTESIAN_POINT ( 'NONE',  ( -15.33914129824368011, 2.553033558614008047, 2.558719994042019774 ) ) ;
#10779=DIRECTION ( 'NONE',  ( 0.005961354470445682716, -0.6427876096865404731, -0.7660212471507180654 ) ) ;
#10780=FACE_OUTER_BOUND ( 'NONE', #40651, .T. ) ;
#10781=DIRECTION ( 'NONE',  ( 0.005002170337468016433, -0.7660444431189770143, -0.6427681459581293666 ) ) ;
#10782=EDGE_CURVE ( 'NONE', #9219, #27886, #4774, .T. ) ;
#10783=VECTOR ( 'NONE', #42954, 999.9999999999998863 ) ;
#10784=CARTESIAN_POINT ( 'NONE',  ( -9.808144436391993182, 0.000000000000000000, 10.77986332834118777 ) ) ;
#10785=DIRECTION ( 'NONE',  ( 0.7660212471507180654, -0.6427876096865404731, 0.005961354470445141482 ) ) ;
#10787=DIRECTION ( 'NONE',  ( 0.005961354470445682716, -0.6427876096865404731, -0.7660212471507180654 ) ) ;
#10788=ADVANCED_FACE ( 'NONE', ( #15264 ), #44504, .T. ) ;
#10789=CARTESIAN_POINT ( 'NONE',  ( -17.93139508144814442, 0.000000000000000000, 13.85596890686001537 ) ) ;
#10790=ORIENTED_EDGE ( 'NONE', *, *, #12821, .F. ) ;
#10791=ORIENTED_EDGE ( 'NONE', *, *, #32138, .F. ) ;
#10792=CARTESIAN_POINT ( 'NONE',  ( -25.20278734466900517, 0.000000000000000000, 6.670939612111840944 ) ) ;
#10793=LINE ( 'NONE', #2537, #30352 ) ;
#10794=EDGE_CURVE ( 'NONE', #18005, #294, #53586, .T. ) ;
#10795=ORIENTED_EDGE ( 'NONE', *, *, #15438, .T. ) ;
#10796=EDGE_CURVE ( 'NONE', #32426, #21097, #19794, .T. ) ;
#10797=DIRECTION ( 'NONE',  ( 0.000000000000000000, -0.000000000000000000, -1.000000000000000000 ) ) ;
#10798=ORIENTED_EDGE ( 'NONE', *, *, #40390, .T. ) ;
#10799=CARTESIAN_POINT ( 'NONE',  ( -10.31796531083145219, -0.1191753592594183703, 3.732117152394283099 ) ) ;
#10800=EDGE_CURVE ( 'NONE', #21762, #39658, #11267, .T. ) ;
#10801=ORIENTED_EDGE ( 'NONE', *, *, #5289, .T. ) ;
#10802=ORIENTED_EDGE ( 'NONE', *, *, #50254, .T. ) ;
#10803=ORIENTED_EDGE ( 'NONE', *, *, #25121, .F. ) ;
#10804=CARTESIAN_POINT ( 'NONE',  ( -9.727461976784988806, 9.474806996477934007, 6.996850153446332321 ) ) ;
#10805=DIRECTION ( 'NONE',  ( -0.9999697198139514409, -0.000000000000000000, -0.007781995580013368816 ) ) ;
#10806=DIRECTION ( 'NONE',  ( 0.007781995580012663651, -3.146120232559066537E-19, -0.9999697198139514409 ) ) ;
#10807=EDGE_CURVE ( 'NONE', #21652, #12842, #6202, .T. ) ;
#10808=VERTEX_POINT ( 'NONE', #14435 ) ;
#10809=ORIENTED_EDGE ( 'NONE', *, *, #53891, .F. ) ;
#10810=EDGE_CURVE ( 'NONE', #6267, #11826, #36554, .T. ) ;
#10811=DIRECTION ( 'NONE',  ( 0.6427681459581294776, -0.7660444431189769032, 0.005002170337467562802 ) ) ;
#10812=VERTEX_POINT ( 'NONE', #5614 ) ;
#10813=LINE ( 'NONE', #49961, #1940 ) ;
#10814=ORIENTED_EDGE ( 'NONE', *, *, #1025, .T. ) ;
#10815=DIRECTION ( 'NONE',  ( 0.000000000000000000, -0.000000000000000000, -1.000000000000000000 ) ) ;
#10816=CARTESIAN_POINT ( 'NONE',  ( -16.81190032086591302, 0.000000000000000000, 3.212244750653343583 ) ) ;
#10818=EDGE_LOOP ( 'NONE', ( #39077, #11458, #47894, #28886 ) ) ;
#10819=DIRECTION ( 'NONE',  ( 0.007781995580012663651, 0.000000000000000000, -0.9999697198139515519 ) ) ;
#10820=DIRECTION ( 'NONE',  ( 0.007781995580012662783, 0.000000000000000000, -0.9999697198139514409 ) ) ;
#10821=ORIENTED_EDGE ( 'NONE', *, *, #52566, .F. ) ;
#10822=CARTESIAN_POINT ( 'NONE',  ( -15.42508763604229927, 2.067327705546507133, 6.265785956968178638 ) ) ;
#10823=DIRECTION ( 'NONE',  ( 0.005002170337468016433, -0.7660444431189770143, -0.6427681459581293666 ) ) ;
#10824=DIRECTION ( 'NONE',  ( 0.5364919789714477361, 0.6444004775717706579, 0.5449076811759711036 ) ) ;
#10825=VERTEX_POINT ( 'NONE', #10453 ) ;
#10826=LINE ( 'NONE', #24174, #5630 ) ;
#10827=LINE ( 'NONE', #28136, #54096 ) ;
#10828=FACE_OUTER_BOUND ( 'NONE', #13693, .T. ) ;
#10830=DIRECTION ( 'NONE',  ( 0.6427681459581294776, -0.7660444431189769032, 0.005002170337467562802 ) ) ;
#10831=LINE ( 'NONE', #2300, #12234 ) ;
#10832=DIRECTION ( 'NONE',  ( 0.5364919789714477361, 0.6444004775717706579, 0.5449076811759711036 ) ) ;
#10834=EDGE_LOOP ( 'NONE', ( #20203, #28537, #4936, #45988 ) ) ;
#10835=DIRECTION ( 'NONE',  ( -0.9999697198139514409, -0.000000000000000000, -0.007781995580013368816 ) ) ;
#10836=CARTESIAN_POINT ( 'NONE',  ( 2.072287782118878319, 0.000000000000000000, -2.950529333540147015 ) ) ;
#10838=VERTEX_POINT ( 'NONE', #32578 ) ;
#10839=CARTESIAN_POINT ( 'NONE',  ( -18.67619601524082285, 0.000000000000000000, 3.936400510096834893 ) ) ;
#10840=CARTESIAN_POINT ( 'NONE',  ( -19.68796468072271111, -4.565544526780662693, 11.82224219410458055 ) ) ;
#10841=ADVANCED_FACE ( 'NONE', ( #5910 ), #23503, .F. ) ;
#10842=LINE ( 'NONE', #6312, #32233 ) ;
#10843=DIRECTION ( 'NONE',  ( -0.9999697198139514409, -0.000000000000000000, -0.007781995580013368816 ) ) ;
#10844=EDGE_CURVE ( 'NONE', #25146, #23505, #23237, .T. ) ;
#10845=CARTESIAN_POINT ( 'NONE',  ( -14.43874742113896126, -1.165603555308156514, 2.452632101459367497 ) ) ;
#10846=EDGE_LOOP ( 'NONE', ( #46306, #4705, #4752, #36011 ) ) ;
#10847=ORIENTED_EDGE ( 'NONE', *, *, #48004, .T. ) ;
#10851=ORIENTED_EDGE ( 'NONE', *, *, #11282, .F. ) ;
#10852=EDGE_CURVE ( 'NONE', #29930, #10033, #49883, .T. ) ;
#10853=DIRECTION ( 'NONE',  ( 0.007781995580012663651, 0.000000000000000000, -0.9999697198139515519 ) ) ;
#10854=ORIENTED_EDGE ( 'NONE', *, *, #49354, .T. ) ;
#10856=ADVANCED_FACE ( 'NONE', ( #10155 ), #10982, .F. ) ;
#10857=VERTEX_POINT ( 'NONE', #23763 ) ;
#10858=ORIENTED_EDGE ( 'NONE', *, *, #47969, .T. ) ;
#10859=FACE_OUTER_BOUND ( 'NONE', #3574, .T. ) ;
#10860=DIRECTION ( 'NONE',  ( 0.005961354470445682716, -0.6427876096865404731, -0.7660212471507180654 ) ) ;
#10861=DIRECTION ( 'NONE',  ( 0.000000000000000000, -0.000000000000000000, -1.000000000000000000 ) ) ;
#10862=ORIENTED_EDGE ( 'NONE', *, *, #29832, .T. ) ;
#10863=ADVANCED_FACE ( 'NONE', ( #28304 ), #41087, .F. ) ;
#10864=DIRECTION ( 'NONE',  ( -0.005961354470445682716, -0.6427876096865404731, 0.7660212471507180654 ) ) ;
#10865=ORIENTED_EDGE ( 'NONE', *, *, #52422, .F. ) ;
#10866=ORIENTED_EDGE ( 'NONE', *, *, #11680, .F. ) ;
#10867=ORIENTED_EDGE ( 'NONE', *, *, #48832, .F. ) ;
#10868=CARTESIAN_POINT ( 'NONE',  ( -13.18788971426693557, 4.981562823951513508, 1.645618023703288246 ) ) ;
#10869=ORIENTED_EDGE ( 'NONE', *, *, #44388, .F. ) ;
#10870=DIRECTION ( 'NONE',  ( 0.007781995580012663651, 0.000000000000000000, -0.9999697198139515519 ) ) ;
#10871=ORIENTED_EDGE ( 'NONE', *, *, #29672, .T. ) ;
#10872=PLANE ( 'NONE',  #35834 ) ;
#10873=LINE ( 'NONE', #6913, #46724 ) ;
#10874=EDGE_LOOP ( 'NONE', ( #4815, #19465, #16652, #53535 ) ) ;
#10875=DIRECTION ( 'NONE',  ( -0.6427681459581293666, -0.7660444431189770143, -0.005002170337467561935 ) ) ;
#10876=ORIENTED_EDGE ( 'NONE', *, *, #53485, .F. ) ;
#10877=VECTOR ( 'NONE', #48739, 1000.000000000000227 ) ;
#10878=DIRECTION ( 'NONE',  ( -0.5449076811759708816, 0.6444004775717707689, 0.5364919789714475140 ) ) ;
#10879=PLANE ( 'NONE',  #14822 ) ;
#10880=LINE ( 'NONE', #28191, #42273 ) ;
#10881=DIRECTION ( 'NONE',  ( -0.5364919789714478471, 0.6444004775717705469, -0.5449076811759709926 ) ) ;
#10882=LINE ( 'NONE', #33023, #17857 ) ;
#10883=PLANE ( 'NONE',  #36432 ) ;
#10884=LINE ( 'NONE', #36188, #10228 ) ;
#10885=EDGE_LOOP ( 'NONE', ( #18593, #48165, #157, #52624 ) ) ;
#10886=EDGE_CURVE ( 'NONE', #38808, #37795, #1640, .T. ) ;
#10887=ORIENTED_EDGE ( 'NONE', *, *, #558, .F. ) ;
#10889=CARTESIAN_POINT ( 'NONE',  ( -19.60834386242827776, 0.000000000000000000, 4.298478389818581213 ) ) ;
#10891=CARTESIAN_POINT ( 'NONE',  ( -20.32972687588355853, 2.391131607591508335, 4.502398433284342971 ) ) ;
#10892=CARTESIAN_POINT ( 'NONE',  ( -11.82833909480979884, 0.000000000000000000, 5.836352465097450093 ) ) ;
#10893=DIRECTION ( 'NONE',  ( -0.3620778797217457101, 0.000000000000000000, -0.9321478471874540261 ) ) ;
#10895=EDGE_CURVE ( 'NONE', #27645, #42294, #20645, .T. ) ;
#10896=LINE ( 'NONE', #16269, #12291 ) ;
#10897=PLANE ( 'NONE',  #46804 ) ;
#10898=ORIENTED_EDGE ( 'NONE', *, *, #37762, .F. ) ;
#10899=CARTESIAN_POINT ( 'NONE',  ( -20.63919478859656209, 2.714935509636507316, 9.353956982646346674 ) ) ;
#10900=CARTESIAN_POINT ( 'NONE',  ( -21.47263955680318404, 0.000000000000000000, 5.022634149262071190 ) ) ;
#10901=ORIENTED_EDGE ( 'NONE', *, *, #15268, .T. ) ;
#10902=EDGE_CURVE ( 'NONE', #52808, #25477, #34274, .T. ) ;
#10903=EDGE_CURVE ( 'NONE', #15187, #7720, #54693, .T. ) ;
#10904=ADVANCED_FACE ( 'NONE', ( #7876 ), #41907, .F. ) ;
#10906=CARTESIAN_POINT ( 'NONE',  ( -11.34514022254773735, 0.000000000000000000, 3.454794398023896651 ) ) ;
#10907=DIRECTION ( 'NONE',  ( 0.005002170337468016433, -0.7660444431189770143, -0.6427681459581293666 ) ) ;
#10908=DIRECTION ( 'NONE',  ( 0.6427681459581294776, -0.7660444431189769032, 0.005002170337467562802 ) ) ;
#10910=ORIENTED_EDGE ( 'NONE', *, *, #47125, .T. ) ;
#10911=ORIENTED_EDGE ( 'NONE', *, *, #28773, .T. ) ;
#10912=DIRECTION ( 'NONE',  ( 0.6427681459581294776, -0.7660444431189769032, 0.005002170337467562802 ) ) ;
#10913=DIRECTION ( 'NONE',  ( 0.6427681459581294776, -0.7660444431189769032, 0.005002170337467562802 ) ) ;
#10914=LINE ( 'NONE', #41306, #11551 ) ;
#10915=LINE ( 'NONE', #54352, #24664 ) ;
#10916=ADVANCED_FACE ( 'NONE', ( #55264 ), #3859, .F. ) ;
#10917=CARTESIAN_POINT ( 'NONE',  ( -14.89451260070033456, 3.686347215771511365, 2.349852469050325077 ) ) ;
#10918=VERTEX_POINT ( 'NONE', #45919 ) ;
#10920=VECTOR ( 'NONE', #44303, 999.9999999999998863 ) ;
#10921=ADVANCED_FACE ( 'NONE', ( #7033 ), #24334, .F. ) ;
#10922=DIRECTION ( 'NONE',  ( 0.005961354470445682716, -0.6427876096865404731, -0.7660212471507180654 ) ) ;
#10923=DIRECTION ( 'NONE',  ( 0.5364919789714477361, 0.6444004775717706579, 0.5449076811759711036 ) ) ;
#10924=EDGE_LOOP ( 'NONE', ( #33622, #33102, #54178, #22872 ) ) ;
#10926=FACE_OUTER_BOUND ( 'NONE', #38945, .T. ) ;
#10927=FACE_OUTER_BOUND ( 'NONE', #14815, .T. ) ;
#10928=CARTESIAN_POINT ( 'NONE',  ( -14.72909745882335386, -1.489407457353157049, 4.847584766220364827 ) ) ;
#10929=ORIENTED_EDGE ( 'NONE', *, *, #41415, .F. ) ;
#10930=EDGE_CURVE ( 'NONE', #36112, #7607, #55005, .T. ) ;
#10931=CARTESIAN_POINT ( 'NONE',  ( -23.33693525117809386, 0.000000000000000000, 5.746789908705562944 ) ) ;
#10932=ORIENTED_EDGE ( 'NONE', *, *, #17915, .F. ) ;
#10933=ADVANCED_FACE ( 'NONE', ( #12099 ), #50727, .F. ) ;
#10934=EDGE_LOOP ( 'NONE', ( #39834, #36295, #5484, #17930 ) ) ;
#10935=ORIENTED_EDGE ( 'NONE', *, *, #50571, .T. ) ;
#10937=EDGE_LOOP ( 'NONE', ( #9384, #55618, #23671, #54637, #1742 ) ) ;
#10939=DIRECTION ( 'NONE',  ( 0.007781995580012663651, -3.146120232559066537E-19, -0.9999697198139514409 ) ) ;
#10940=ORIENTED_EDGE ( 'NONE', *, *, #2922, .T. ) ;
#10941=ORIENTED_EDGE ( 'NONE', *, *, #5916, .F. ) ;
#10942=CARTESIAN_POINT ( 'NONE',  ( -16.59339315319826014, -1.489407457353158160, 5.571740525663858357 ) ) ;
#10943=ORIENTED_EDGE ( 'NONE', *, *, #33278, .T. ) ;
#10944=ORIENTED_EDGE ( 'NONE', *, *, #11147, .F. ) ;
#10945=EDGE_LOOP ( 'NONE', ( #18399, #21039, #32060, #32155 ) ) ;
#10946=FACE_OUTER_BOUND ( 'NONE', #7578, .T. ) ;
#10947=LINE ( 'NONE', #50418, #45718 ) ;
#10949=LINE ( 'NONE', #45063, #46775 ) ;
#10950=ORIENTED_EDGE ( 'NONE', *, *, #17940, .F. ) ;
#10951=CARTESIAN_POINT ( 'NONE',  ( -9.510902717614937885, 0.000000000000000000, 6.593051430453025219 ) ) ;
#10952=ORIENTED_EDGE ( 'NONE', *, *, #24223, .F. ) ;
#10953=ORIENTED_EDGE ( 'NONE', *, *, #1905, .F. ) ;
#10954=VECTOR ( 'NONE', #25610, 1000.000000000000227 ) ;
#10955=CARTESIAN_POINT ( 'NONE',  ( -15.50102849149811135, -0.1191753592594197858, 12.95155240711365430 ) ) ;
#10956=AXIS2_PLACEMENT_3D ( 'NONE', #30638, #52734, #22654 ) ;
#10958=FACE_OUTER_BOUND ( 'NONE', #18350, .T. ) ;
#10959=CARTESIAN_POINT ( 'NONE',  ( -16.13292578047435910, 0.000000000000000000, 3.048202673938099849 ) ) ;
#10960=CARTESIAN_POINT ( 'NONE',  ( -20.54126990917373519, -0.1191753592594197858, 4.760553241521720658 ) ) ;
#10961=ORIENTED_EDGE ( 'NONE', *, *, #44269, .F. ) ;
#10963=EDGE_LOOP ( 'NONE', ( #33540, #54874, #15808, #39798 ) ) ;
#10964=EDGE_CURVE ( 'NONE', #44493, #45963, #33421, .T. ) ;
#10965=EDGE_CURVE ( 'NONE', #1437, #38304, #24894, .T. ) ;
#10966=PLANE ( 'NONE',  #22054 ) ;
#10968=CARTESIAN_POINT ( 'NONE',  ( -17.74560456716937296, 0.000000000000000000, 3.774316574337878372 ) ) ;
#10969=DIRECTION ( 'NONE',  ( 0.6427681459581294776, -0.7660444431189769032, 0.005002170337467562802 ) ) ;
#10970=EDGE_CURVE ( 'NONE', #27279, #19226, #30279, .T. ) ;
#10971=CARTESIAN_POINT ( 'NONE',  ( -18.80364065443665211, 0.000000000000000000, 6.520733195092834222 ) ) ;
#10972=EDGE_LOOP ( 'NONE', ( #51164, #16706, #45561, #17942 ) ) ;
#10973=DIRECTION ( 'NONE',  ( 0.9999697198139515519, 0.000000000000000000, 0.007781995580013368816 ) ) ;
#10974=DIRECTION ( 'NONE',  ( -0.005002170337468016433, -0.7660444431189770143, 0.6427681459581293666 ) ) ;
#10976=VECTOR ( 'NONE', #28938, 1000.000000000000000 ) ;
#10977=VECTOR ( 'NONE', #48287, 1000.000000000000227 ) ;
#10978=DIRECTION ( 'NONE',  ( 0.7660212471507180654, -0.6427876096865404731, 0.005961354470445141482 ) ) ;
#10979=LINE ( 'NONE', #6197, #26664 ) ;
#10980=DIRECTION ( 'NONE',  ( 0.007781995580012663651, -3.146120232559066537E-19, -0.9999697198139514409 ) ) ;
#10982=PLANE ( 'NONE',  #51393 ) ;
#10983=LINE ( 'NONE', #1641, #41931 ) ;
#10984=ORIENTED_EDGE ( 'NONE', *, *, #10087, .T. ) ;
#10985=VECTOR ( 'NONE', #43986, 999.9999999999998863 ) ;
#10986=EDGE_CURVE ( 'NONE', #37343, #42711, #21492, .T. ) ;
#10987=VECTOR ( 'NONE', #42552, 1000.000000000000114 ) ;
#10988=VERTEX_POINT ( 'NONE', #8717 ) ;
#10989=VERTEX_POINT ( 'NONE', #30583 ) ;
#10990=VERTEX_POINT ( 'NONE', #13519 ) ;
#10991=ADVANCED_FACE ( 'NONE', ( #30834 ), #22029, .F. ) ;
#10992=EDGE_LOOP ( 'NONE', ( #20906, #37179, #51022, #49441 ) ) ;
#10993=CARTESIAN_POINT ( 'NONE',  ( -9.413091840428602808, -0.1191753592594190225, 6.874738116430744839 ) ) ;
#10994=ADVANCED_FACE ( 'NONE', ( #988 ), #52132, .F. ) ;
#10995=DIRECTION ( 'NONE',  ( -0.8531650599175529814, -0.4028455766673920135, 0.3313982828793697877 ) ) ;
#10996=EDGE_LOOP ( 'NONE', ( #56192, #3901, #36573, #462 ) ) ;
#10997=VERTEX_POINT ( 'NONE', #39354 ) ;
#10998=EDGE_CURVE ( 'NONE', #46093, #54486, #445, .T. ) ;
#10999=ORIENTED_EDGE ( 'NONE', *, *, #54021, .T. ) ;
#11000=ORIENTED_EDGE ( 'NONE', *, *, #44997, .T. ) ;
#11002=CARTESIAN_POINT ( 'NONE',  ( 2.072287782118878319, 0.000000000000000000, -2.950529333540147015 ) ) ;
#11003=CARTESIAN_POINT ( 'NONE',  ( -15.86710544311044302, 0.000000000000000000, 13.13336954653252953 ) ) ;
#11004=EDGE_LOOP ( 'NONE', ( #35504, #26504, #29154, #16225 ) ) ;
#11005=CARTESIAN_POINT ( 'NONE',  ( 1.086233639165236964, 0.000000000000000000, 2.796443541562362078 ) ) ;
#11006=AXIS2_PLACEMENT_3D ( 'NONE', #48722, #44714, #9824 ) ;
#11007=VECTOR ( 'NONE', #27223, 1000.000000000000227 ) ;
#11008=DIRECTION ( 'NONE',  ( 0.9999697198139515519, 0.000000000000000000, 0.007781995580013368816 ) ) ;
#11009=PLANE ( 'NONE',  #25723 ) ;
#11010=CARTESIAN_POINT ( 'NONE',  ( -21.74593062183054926, 4.010151117816509903, 11.90952023678523197 ) ) ;
#11011=CARTESIAN_POINT ( 'NONE',  ( -10.80846868922008497, -0.1191753592594181482, 7.052288569946153274 ) ) ;
#11012=VECTOR ( 'NONE', #20540, 1000.000000000000227 ) ;
#11014=DIRECTION ( 'NONE',  ( 0.6427681459581294776, -0.7660444431189769032, 0.005002170337467562802 ) ) ;
#11015=DIRECTION ( 'NONE',  ( 0.000000000000000000, -0.000000000000000000, -1.000000000000000000 ) ) ;
#11016=FACE_OUTER_BOUND ( 'NONE', #27911, .T. ) ;
#11017=ORIENTED_EDGE ( 'NONE', *, *, #12082, .F. ) ;
#11018=DIRECTION ( 'NONE',  ( 0.005961354470445682716, -0.6427876096865404731, -0.7660212471507180654 ) ) ;
#11020=ADVANCED_FACE ( 'NONE', ( #12679 ), #21757, .F. ) ;
#11021=FACE_OUTER_BOUND ( 'NONE', #5824, .T. ) ;
#11022=LINE ( 'NONE', #19002, #6890 ) ;
#11023=CARTESIAN_POINT ( 'NONE',  ( -15.54830832304376820, 0.000000000000000000, 6.176734874211137871 ) ) ;
#11024=CARTESIAN_POINT ( 'NONE',  ( -15.87635958039733097, 3.686347215771509145, 9.098162144920037164 ) ) ;
#11025=DIRECTION ( 'NONE',  ( 0.007781995580012662783, 0.000000000000000000, -0.9999697198139514409 ) ) ;
#11027=EDGE_CURVE ( 'NONE', #22884, #370, #9545, .T. ) ;
#11028=ADVANCED_FACE ( 'NONE', ( #5000 ), #9243, .F. ) ;
#11029=VECTOR ( 'NONE', #26656, 1000.000000000000227 ) ;
#11030=DIRECTION ( 'NONE',  ( 0.005961354470445682716, -0.6427876096865404731, -0.7660212471507180654 ) ) ;
#11032=CARTESIAN_POINT ( 'NONE',  ( -17.93139508144814442, 0.000000000000000000, 13.85596890686001537 ) ) ;
#11033=LINE ( 'NONE', #11868, #53828 ) ;
#11034=DIRECTION ( 'NONE',  ( 0.007781995580012663651, -3.146120232559066537E-19, -0.9999697198139514409 ) ) ;
#11035=CARTESIAN_POINT ( 'NONE',  ( -12.06136745912998975, 0.000000000000000000, 1.771886216610035092 ) ) ;
#11036=PLANE ( 'NONE',  #16912 ) ;
#11037=PLANE ( 'NONE',  #91 ) ;
#11038=FACE_OUTER_BOUND ( 'NONE', #22742, .T. ) ;
#11039=DIRECTION ( 'NONE',  ( 0.000000000000000000, -0.000000000000000000, -1.000000000000000000 ) ) ;
#11040=LINE ( 'NONE', #10789, #20188 ) ;
#11041=ORIENTED_EDGE ( 'NONE', *, *, #20974, .F. ) ;
#11042=LINE ( 'NONE', #41699, #9490 ) ;
#11043=ORIENTED_EDGE ( 'NONE', *, *, #8329, .T. ) ;
#11044=CARTESIAN_POINT ( 'NONE',  ( -15.80102324005015824, -2.784623065533160524, 2.930131093732116554 ) ) ;
#11045=CARTESIAN_POINT ( 'NONE',  ( -13.67694686726901665, 0.000000000000000000, 4.544643948957142854 ) ) ;
#11047=VECTOR ( 'NONE', #42943, 1000.000000000000227 ) ;
#11048=ORIENTED_EDGE ( 'NONE', *, *, #40485, .T. ) ;
#11049=ORIENTED_EDGE ( 'NONE', *, *, #50599, .T. ) ;
#11050=CARTESIAN_POINT ( 'NONE',  ( -19.60912206198628027, -0.1191753592594197858, 4.398475361799976113 ) ) ;
#11051=ORIENTED_EDGE ( 'NONE', *, *, #27316, .T. ) ;
#11052=ORIENTED_EDGE ( 'NONE', *, *, #13652, .F. ) ;
#11053=VECTOR ( 'NONE', #27887, 999.9999999999998863 ) ;
#11054=ORIENTED_EDGE ( 'NONE', *, *, #52505, .T. ) ;
#11055=CARTESIAN_POINT ( 'NONE',  ( -18.86354292863559579, 0.000000000000000000, 14.21804678658176080 ) ) ;
#11056=CARTESIAN_POINT ( 'NONE',  ( -12.60458797795435615, 0.000000000000000000, 11.86609696750642229 ) ) ;
#11057=DIRECTION ( 'NONE',  ( 0.9999697198139515519, 0.000000000000000000, 0.007781995580013368816 ) ) ;
#11058=VERTEX_POINT ( 'NONE', #12949 ) ;
#11059=EDGE_CURVE ( 'NONE', #12635, #6150, #39910, .T. ) ;
#11060=VECTOR ( 'NONE', #35405, 1000.000000000000114 ) ;
#11061=ORIENTED_EDGE ( 'NONE', *, *, #3840, .T. ) ;
#11062=VECTOR ( 'NONE', #29465, 1000.000000000000114 ) ;
#11063=PLANE ( 'NONE',  #32977 ) ;
#11064=LINE ( 'NONE', #53962, #26374 ) ;
#11065=ORIENTED_EDGE ( 'NONE', *, *, #37015, .F. ) ;
#11066=DIRECTION ( 'NONE',  ( -0.9999697198139514409, -0.000000000000000000, -0.007781995580013368816 ) ) ;
#11067=ORIENTED_EDGE ( 'NONE', *, *, #3587, .F. ) ;
#11068=CARTESIAN_POINT ( 'NONE',  ( -18.32598891683381126, -5.698858183938163791, 13.15316534217173938 ) ) ;
#11069=FACE_OUTER_BOUND ( 'NONE', #19859, .T. ) ;
#11070=ADVANCED_FACE ( 'NONE', ( #43059 ), #35375, .F. ) ;
#11071=EDGE_CURVE ( 'NONE', #46056, #46010, #39071, .T. ) ;
#11072=ORIENTED_EDGE ( 'NONE', *, *, #40665, .F. ) ;
#11074=VECTOR ( 'NONE', #6953, 999.9999999999998863 ) ;
#11075=EDGE_CURVE ( 'NONE', #49206, #5052, #34527, .T. ) ;
#11076=EDGE_CURVE ( 'NONE', #50902, #38693, #47296, .T. ) ;
#11077=CARTESIAN_POINT ( 'NONE',  ( 2.072287782118878319, -1.000000000000000000, -2.950529333540147015 ) ) ;
#11078=ORIENTED_EDGE ( 'NONE', *, *, #2314, .T. ) ;
#11079=CARTESIAN_POINT ( 'NONE',  ( -26.13493519185646008, 0.000000000000000000, 7.033017491833586377 ) ) ;
#11080=FACE_OUTER_BOUND ( 'NONE', #1280, .T. ) ;
#11081=AXIS2_PLACEMENT_3D ( 'NONE', #9940, #1684, #10776 ) ;
#11082=DIRECTION ( 'NONE',  ( 0.005002170337468016433, -0.7660444431189770143, -0.6427681459581293666 ) ) ;
#11083=EDGE_CURVE ( 'NONE', #46790, #51656, #38810, .T. ) ;
#11084=ORIENTED_EDGE ( 'NONE', *, *, #42469, .T. ) ;
#11085=AXIS2_PLACEMENT_3D ( 'NONE', #15800, #55537, #16641 ) ;
#11086=VECTOR ( 'NONE', #25846, 1000.000000000000227 ) ;
#11087=EDGE_CURVE ( 'NONE', #16268, #3020, #34814, .T. ) ;
#11089=FACE_OUTER_BOUND ( 'NONE', #7973, .T. ) ;
#11090=FACE_OUTER_BOUND ( 'NONE', #14178, .T. ) ;
#11091=DIRECTION ( 'NONE',  ( -0.005002170337468016433, -0.7660444431189770143, 0.6427681459581293666 ) ) ;
#11094=DIRECTION ( 'NONE',  ( 0.005961354470445682716, -0.6427876096865404731, -0.7660212471507180654 ) ) ;
#11095=AXIS2_PLACEMENT_3D ( 'NONE', #30064, #47371, #796 ) ;
#11096=DIRECTION ( 'NONE',  ( 0.5449076811759707706, 0.6444004775717708799, -0.5364919789714476250 ) ) ;
#11097=VECTOR ( 'NONE', #3908, 1000.000000000000114 ) ;
#11098=VERTEX_POINT ( 'NONE', #9831 ) ;
#11099=CARTESIAN_POINT ( 'NONE',  ( 2.072287782118878319, 0.000000000000000000, -2.950529333540147015 ) ) ;
#11100=LINE ( 'NONE', #19903, #44066 ) ;
#11102=EDGE_LOOP ( 'NONE', ( #38699, #27287, #40386, #32586 ) ) ;
#11103=CARTESIAN_POINT ( 'NONE',  ( -26.13493519185646008, 0.000000000000000000, 7.033017491833586377 ) ) ;
#11104=DIRECTION ( 'NONE',  ( 0.007781995580012663651, -3.146120232559066537E-19, -0.9999697198139514409 ) ) ;
#11105=EDGE_CURVE ( 'NONE', #33009, #21477, #31684, .T. ) ;
#11106=CARTESIAN_POINT ( 'NONE',  ( -15.54699066865448565, 0.000000000000000000, 6.007419114916161540 ) ) ;
#11107=FACE_OUTER_BOUND ( 'NONE', #2117, .T. ) ;
#11108=LINE ( 'NONE', #54533, #21135 ) ;
#11109=EDGE_CURVE ( 'NONE', #51910, #5412, #52970, .T. ) ;
#11110=ORIENTED_EDGE ( 'NONE', *, *, #393, .F. ) ;
#11111=ORIENTED_EDGE ( 'NONE', *, *, #49199, .F. ) ;
#11113=CARTESIAN_POINT ( 'NONE',  ( -12.19375721922749278, -0.1191753592594181482, 5.933511724868832715 ) ) ;
#11114=EDGE_LOOP ( 'NONE', ( #20554, #4367, #25027, #46130 ) ) ;
#11115=DIRECTION ( 'NONE',  ( 0.5449076811759707706, 0.6444004775717708799, -0.5364919789714476250 ) ) ;
#11116=VECTOR ( 'NONE', #30947, 999.9999999999998863 ) ;
#11117=ORIENTED_EDGE ( 'NONE', *, *, #43314, .F. ) ;
#11118=PLANE ( 'NONE',  #29244 ) ;
#11119=ORIENTED_EDGE ( 'NONE', *, *, #3357, .T. ) ;
#11120=VERTEX_POINT ( 'NONE', #49267 ) ;
#11121=CARTESIAN_POINT ( 'NONE',  ( -15.40103151951671734, 0.000000000000000000, 12.95233060667165681 ) ) ;
#11122=VECTOR ( 'NONE', #17709, 1000.000000000000114 ) ;
#11123=DIRECTION ( 'NONE',  ( -0.005002170337468016433, -0.7660444431189770143, 0.6427681459581293666 ) ) ;
#11124=LINE ( 'NONE', #40949, #12144 ) ;
#11125=EDGE_LOOP ( 'NONE', ( #10961, #16060, #53253, #44672 ) ) ;
#11126=VECTOR ( 'NONE', #4601, 1000.000000000000114 ) ;
#11127=VECTOR ( 'NONE', #8688, 999.9999999999998863 ) ;
#11128=CARTESIAN_POINT ( 'NONE',  ( -16.09911561167002958, 4.010151117816511679, 2.807430147226621209 ) ) ;
#11129=ADVANCED_FACE ( 'NONE', ( #15208 ), #27707, .F. ) ;
#11130=EDGE_LOOP ( 'NONE', ( #26431, #49283, #12169, #16528 ) ) ;
#11131=VERTEX_POINT ( 'NONE', #10089 ) ;
#11132=AXIS2_PLACEMENT_3D ( 'NONE', #52426, #13521, #48431 ) ;
#11133=ORIENTED_EDGE ( 'NONE', *, *, #1593, .T. ) ;
#11135=VECTOR ( 'NONE', #3143, 999.9999999999998863 ) ;
#11136=ORIENTED_EDGE ( 'NONE', *, *, #12958, .F. ) ;
#11137=PLANE ( 'NONE',  #30265 ) ;
#11139=DIRECTION ( 'NONE',  ( 0.007781995580012662783, 0.000000000000000000, -0.9999697198139514409 ) ) ;
#11140=CARTESIAN_POINT ( 'NONE',  ( -16.75815173624665277, 0.000000000000000000, 8.213985998274722533 ) ) ;
#11141=ADVANCED_FACE ( 'NONE', ( #44444 ), #27986, .F. ) ;
#11142=ORIENTED_EDGE ( 'NONE', *, *, #43481, .F. ) ;
#11143=DIRECTION ( 'NONE',  ( 0.007781995580012663651, -3.146120232559066537E-19, -0.9999697198139514409 ) ) ;
#11144=VECTOR ( 'NONE', #31211, 1000.000000000000227 ) ;
#11145=ORIENTED_EDGE ( 'NONE', *, *, #2754, .T. ) ;
#11146=VECTOR ( 'NONE', #48871, 1000.000000000000227 ) ;
#11147=EDGE_CURVE ( 'NONE', #40714, #27501, #32247, .T. ) ;
#11148=CARTESIAN_POINT ( 'NONE',  ( -13.25450402488150203, 4.981562823951511731, 10.20541388017194073 ) ) ;
#11149=FACE_OUTER_BOUND ( 'NONE', #46539, .T. ) ;
#11150=FACE_OUTER_BOUND ( 'NONE', #44521, .T. ) ;
#11151=CARTESIAN_POINT ( 'NONE',  ( -13.27065584551087163, 0.000000000000000000, 12.04557950825129176 ) ) ;
#11152=DIRECTION ( 'NONE',  ( -0.7660212471507179544, -0.6427876096865405842, -0.005961354470445141482 ) ) ;
#11153=DIRECTION ( 'NONE',  ( 0.005002170337468016433, -0.7660444431189770143, -0.6427681459581293666 ) ) ;
#11154=FACE_OUTER_BOUND ( 'NONE', #10924, .T. ) ;
#11155=ORIENTED_EDGE ( 'NONE', *, *, #6427, .F. ) ;
#11156=VECTOR ( 'NONE', #9205, 1000.000000000000227 ) ;
#11157=ORIENTED_EDGE ( 'NONE', *, *, #53206, .T. ) ;
#11158=EDGE_CURVE ( 'NONE', #39217, #49206, #18909, .T. ) ;
#11160=DIRECTION ( 'NONE',  ( -0.5364919789714478471, 0.6444004775717705469, -0.5449076811759709926 ) ) ;
#11161=VECTOR ( 'NONE', #2858, 999.9999999999998863 ) ;
#11162=CARTESIAN_POINT ( 'NONE',  ( -16.06709938707323460, 0.000000000000000000, 13.13181314741652628 ) ) ;
#11164=DIRECTION ( 'NONE',  ( -0.5364919789714478471, 0.6444004775717705469, -0.5449076811759709926 ) ) ;
#11165=CARTESIAN_POINT ( 'NONE',  ( -10.31509125732617171, -0.1191753592594185784, 3.362807449136518745 ) ) ;
#11166=VERTEX_POINT ( 'NONE', #27402 ) ;
#11167=LINE ( 'NONE', #54900, #45846 ) ;
#11168=DIRECTION ( 'NONE',  ( 0.9999697198139515519, 0.000000000000000000, 0.007781995580013368816 ) ) ;
#11169=ORIENTED_EDGE ( 'NONE', *, *, #35516, .F. ) ;
#11170=VECTOR ( 'NONE', #7162, 1000.000000000000114 ) ;
#11171=DIRECTION ( 'NONE',  ( 0.005002170337468016433, -0.7660444431189770143, -0.6427681459581293666 ) ) ;
#11172=LINE ( 'NONE', #50903, #42219 ) ;
#11173=VERTEX_POINT ( 'NONE', #36785 ) ;
#11174=AXIS2_PLACEMENT_3D ( 'NONE', #26034, #39067, #26285 ) ;
#11175=EDGE_CURVE ( 'NONE', #44131, #26974, #53800, .T. ) ;
#11176=VECTOR ( 'NONE', #43861, 999.9999999999998863 ) ;
#11177=DIRECTION ( 'NONE',  ( 0.007781995580012663651, 0.000000000000000000, -0.9999697198139515519 ) ) ;
#11178=FACE_OUTER_BOUND ( 'NONE', #55940, .T. ) ;
#11179=CARTESIAN_POINT ( 'NONE',  ( -3.789478469635834568, -7.588859415764141580, -1.746411446826717340 ) ) ;
#11180=DIRECTION ( 'NONE',  ( 0.000000000000000000, -1.000000000000000000, 0.000000000000000000 ) ) ;
#11181=DIRECTION ( 'NONE',  ( 0.7660212471507180654, -0.6427876096865404731, 0.005961354470445141482 ) ) ;
#11182=EDGE_CURVE ( 'NONE', #27005, #19751, #2408, .T. ) ;
#11183=ORIENTED_EDGE ( 'NONE', *, *, #19735, .T. ) ;
#11185=VECTOR ( 'NONE', #54526, 1000.000000000000000 ) ;
#11186=ORIENTED_EDGE ( 'NONE', *, *, #29565, .F. ) ;
#11187=CARTESIAN_POINT ( 'NONE',  ( -15.86710544311044302, 0.000000000000000000, 13.13336954653252953 ) ) ;
#11188=DIRECTION ( 'NONE',  ( -0.7660212471507179544, -0.6427876096865405842, -0.005961354470445141482 ) ) ;
#11189=LINE ( 'NONE', #37596, #53315 ) ;
#11190=DIRECTION ( 'NONE',  ( 0.007781995580012663651, -3.146120232559066537E-19, -0.9999697198139514409 ) ) ;
#11191=CARTESIAN_POINT ( 'NONE',  ( -16.81345671998191449, 0.000000000000000000, 3.412238694616132495 ) ) ;
#11192=LINE ( 'NONE', #31943, #10441 ) ;
#11193=EDGE_LOOP ( 'NONE', ( #53811, #32851, #46850, #44740 ) ) ;
#11194=CARTESIAN_POINT ( 'NONE',  ( -13.73672976910459909, 0.000000000000000000, 12.22661844811216270 ) ) ;
#11195=FACE_OUTER_BOUND ( 'NONE', #42822, .T. ) ;
#11196=DIRECTION ( 'NONE',  ( 0.000000000000000000, -1.000000000000000000, 0.000000000000000000 ) ) ;
#11197=ORIENTED_EDGE ( 'NONE', *, *, #39971, .T. ) ;
#11198=AXIS2_PLACEMENT_3D ( 'NONE', #43488, #21646, #313 ) ;
#11199=CARTESIAN_POINT ( 'NONE',  ( -9.296538506125733292, 0.000000000000000000, 4.748059313280206695 ) ) ;
#11200=PLANE ( 'NONE',  #30463 ) ;
#11201=VECTOR ( 'NONE', #3484, 1000.000000000000227 ) ;
#11202=FACE_OUTER_BOUND ( 'NONE', #16898, .T. ) ;
#11203=EDGE_LOOP ( 'NONE', ( #17051, #41264, #551, #7576 ) ) ;
#11204=PLANE ( 'NONE',  #11375 ) ;
#11205=EDGE_CURVE ( 'NONE', #25448, #50616, #14086, .T. ) ;
#11206=AXIS2_PLACEMENT_3D ( 'NONE', #27064, #27324, #40406 ) ;
#11207=ORIENTED_EDGE ( 'NONE', *, *, #51450, .F. ) ;
#11208=EDGE_LOOP ( 'NONE', ( #53462, #51161, #12914, #33883 ) ) ;
#11209=VERTEX_POINT ( 'NONE', #10678 ) ;
#11210=EDGE_CURVE ( 'NONE', #29764, #51468, #53525, .T. ) ;
#11211=ORIENTED_EDGE ( 'NONE', *, *, #2240, .T. ) ;
#11212=EDGE_CURVE ( 'NONE', #428, #34236, #19440, .T. ) ;
#11213=ORIENTED_EDGE ( 'NONE', *, *, #11557, .F. ) ;
#11214=VECTOR ( 'NONE', #14920, 1000.000000000000114 ) ;
#11215=CARTESIAN_POINT ( 'NONE',  ( -20.54204810873173415, 0.000000000000000000, 4.860550213503115558 ) ) ;
#11216=ORIENTED_EDGE ( 'NONE', *, *, #47202, .F. ) ;
#11217=ADVANCED_FACE ( 'NONE', ( #14628 ), #31950, .F. ) ;
#11218=ADVANCED_FACE ( 'NONE', ( #18620 ), #35966, .F. ) ;
#11219=EDGE_CURVE ( 'NONE', #52348, #23769, #3249, .T. ) ;
#11220=ORIENTED_EDGE ( 'NONE', *, *, #27054, .T. ) ;
#11221=CARTESIAN_POINT ( 'NONE',  ( -19.12962290826653700, 0.000000000000000000, 14.40064212555863854 ) ) ;
#11222=ORIENTED_EDGE ( 'NONE', *, *, #39773, .T. ) ;
#11223=ORIENTED_EDGE ( 'NONE', *, *, #45570, .T. ) ;
#11224=ORIENTED_EDGE ( 'NONE', *, *, #39015, .F. ) ;
#11225=VECTOR ( 'NONE', #37170, 1000.000000000000227 ) ;
#11226=VECTOR ( 'NONE', #5135, 999.9999999999998863 ) ;
#11227=CARTESIAN_POINT ( 'NONE',  ( -13.17065887352947762, -0.1191753592594197858, 12.04635770780929427 ) ) ;
#11228=FACE_OUTER_BOUND ( 'NONE', #21711, .T. ) ;
#11229=CARTESIAN_POINT ( 'NONE',  ( -15.50102849149811135, -0.1191753592594197858, 12.95155240711365430 ) ) ;
#11230=DIRECTION ( 'NONE',  ( 0.005961354470445682716, -0.6427876096865404731, -0.7660212471507180654 ) ) ;
#11231=PLANE ( 'NONE',  #25579 ) ;
#11232=ORIENTED_EDGE ( 'NONE', *, *, #45277, .F. ) ;
#11233=ORIENTED_EDGE ( 'NONE', *, *, #14094, .T. ) ;
#11234=ADVANCED_FACE ( 'NONE', ( #28822 ), #50669, .F. ) ;
#11235=CARTESIAN_POINT ( 'NONE',  ( -16.29770654730013035, 0.000000000000000000, 8.756227372595473568 ) ) ;
#11236=CARTESIAN_POINT ( 'NONE',  ( -20.18473747654950046, 0.000000000000000000, 4.863330887462772978 ) ) ;
#11237=EDGE_CURVE ( 'NONE', #9210, #49710, #37898, .T. ) ;
#11239=PLANE ( 'NONE',  #27641 ) ;
#11240=VECTOR ( 'NONE', #30440, 999.9999999999998863 ) ;
#11241=EDGE_CURVE ( 'NONE', #6281, #15209, #55205, .T. ) ;
#11242=DIRECTION ( 'NONE',  ( -0.005961354470445682716, -0.6427876096865404731, 0.7660212471507180654 ) ) ;
#11243=CARTESIAN_POINT ( 'NONE',  ( -16.48333022373650536, 0.000000000000000000, 6.908122457190647658 ) ) ;
#11245=DIRECTION ( 'NONE',  ( 0.9999697198139515519, 0.000000000000000000, 0.007781995580013368816 ) ) ;
#11246=AXIS2_PLACEMENT_3D ( 'NONE', #46719, #50124, #33109 ) ;
#11247=EDGE_LOOP ( 'NONE', ( #34547, #49355, #33641, #19086 ) ) ;
#11248=EDGE_CURVE ( 'NONE', #22811, #6333, #25386, .T. ) ;
#11249=DIRECTION ( 'NONE',  ( -0.9999697198139514409, -0.000000000000000000, -0.007781995580013368816 ) ) ;
#11250=PLANE ( 'NONE',  #9737 ) ;
#11251=CARTESIAN_POINT ( 'NONE',  ( -14.99882292130570072, -0.1191753592594177180, 8.127674473807362077 ) ) ;
#11252=AXIS2_PLACEMENT_3D ( 'NONE', #46210, #52716, #772 ) ;
#11253=CARTESIAN_POINT ( 'NONE',  ( -11.83851765444165061, 0.000000000000000000, 7.144275518833531180 ) ) ;
#11254=DIRECTION ( 'NONE',  ( 0.5449076811759707706, 0.6444004775717708799, -0.5364919789714476250 ) ) ;
#11255=ORIENTED_EDGE ( 'NONE', *, *, #19785, .F. ) ;
#11256=VECTOR ( 'NONE', #43542, 999.9999999999998863 ) ;
#11257=DIRECTION ( 'NONE',  ( 0.000000000000000000, -0.000000000000000000, -1.000000000000000000 ) ) ;
#11258=PLANE ( 'NONE',  #37681 ) ;
#11259=FACE_OUTER_BOUND ( 'NONE', #26881, .T. ) ;
#11261=CARTESIAN_POINT ( 'NONE',  ( -14.94760462649100496, 0.000000000000000000, 2.488088991209854051 ) ) ;
#11262=LINE ( 'NONE', #19214, #47550 ) ;
#11263=DIRECTION ( 'NONE',  ( -0.6427681459581293666, -0.7660444431189770143, -0.005002170337467561935 ) ) ;
#11264=PLANE ( 'NONE',  #19317 ) ;
#11265=VECTOR ( 'NONE', #23500, 999.9999999999998863 ) ;
#11266=VECTOR ( 'NONE', #7864, 999.9999999999998863 ) ;
#11267=LINE ( 'NONE', #49634, #25989 ) ;
#11268=DIRECTION ( 'NONE',  ( -0.9999697198139514409, -0.000000000000000000, -0.007781995580013368816 ) ) ;
#11269=ORIENTED_EDGE ( 'NONE', *, *, #23120, .T. ) ;
#11270=EDGE_LOOP ( 'NONE', ( #56160, #10865, #680, #38077 ) ) ;
#11271=VECTOR ( 'NONE', #46997, 999.9999999999998863 ) ;
#11272=ORIENTED_EDGE ( 'NONE', *, *, #23129, .F. ) ;
#11273=ORIENTED_EDGE ( 'NONE', *, *, #29887, .T. ) ;
#11274=ORIENTED_EDGE ( 'NONE', *, *, #47067, .T. ) ;
#11275=VECTOR ( 'NONE', #51930, 1000.000000000000000 ) ;
#11276=EDGE_LOOP ( 'NONE', ( #28444, #9832, #48569, #35141 ) ) ;
#11277=DIRECTION ( 'NONE',  ( 0.007781995580012663651, 0.000000000000000000, -0.9999697198139515519 ) ) ;
#11278=CARTESIAN_POINT ( 'NONE',  ( -10.34523968761605772, -0.1191753592594198830, 7.236815996152489383 ) ) ;
#11280=VECTOR ( 'NONE', #48309, 999.9999999999998863 ) ;
#11281=ADVANCED_FACE ( 'NONE', ( #11760 ), #20273, .F. ) ;
#11282=EDGE_CURVE ( 'NONE', #5725, #11899, #37059, .T. ) ;
#11283=EDGE_LOOP ( 'NONE', ( #31728, #48581, #17399, #29032 ) ) ;
#11284=CARTESIAN_POINT ( 'NONE',  ( -22.40634380310664397, 0.000000000000000000, 5.584705972946605534 ) ) ;
#11285=EDGE_LOOP ( 'NONE', ( #30384, #43766, #40189, #30592 ) ) ;
#11286=EDGE_CURVE ( 'NONE', #10342, #49938, #33067, .T. ) ;
#11287=VERTEX_POINT ( 'NONE', #29076 ) ;
#11288=VECTOR ( 'NONE', #46725, 999.9999999999998863 ) ;
#11290=VECTOR ( 'NONE', #23022, 999.9999999999998863 ) ;
#11291=CARTESIAN_POINT ( 'NONE',  ( -18.14631431975934817, 0.000000000000000000, 7.464518856455165441 ) ) ;
#11292=DIRECTION ( 'NONE',  ( 0.9999697198139515519, 0.000000000000000000, 0.007781995580013368816 ) ) ;
#11293=VERTEX_POINT ( 'NONE', #15453 ) ;
#11294=DIRECTION ( 'NONE',  ( 0.7660212471507180654, -0.6427876096865404731, 0.005961354470445141482 ) ) ;
#11296=AXIS2_PLACEMENT_3D ( 'NONE', #45130, #32055, #49376 ) ;
#11297=LINE ( 'NONE', #20375, #53616 ) ;
#11298=FACE_OUTER_BOUND ( 'NONE', #37330, .T. ) ;
#11299=ADVANCED_FACE ( 'NONE', ( #6970 ), #24277, .F. ) ;
#11301=LINE ( 'NONE', #37146, #13632 ) ;
#11302=PLANE ( 'NONE',  #25145 ) ;
#11303=VECTOR ( 'NONE', #26775, 1000.000000000000114 ) ;
#11305=DIRECTION ( 'NONE',  ( 0.000000000000000000, -1.000000000000000000, 0.000000000000000000 ) ) ;
#11306=LINE ( 'NONE', #45958, #24882 ) ;
#11307=EDGE_CURVE ( 'NONE', #9919, #15150, #16573, .T. ) ;
#11308=DIRECTION ( 'NONE',  ( 0.005961354470445682716, -0.6427876096865404731, -0.7660212471507180654 ) ) ;
#11309=PLANE ( 'NONE',  #10250 ) ;
#11310=VERTEX_POINT ( 'NONE', #24822 ) ;
#11311=CARTESIAN_POINT ( 'NONE',  ( -15.60102546347950536, 0.000000000000000000, 12.95077420755565356 ) ) ;
#11312=EDGE_LOOP ( 'NONE', ( #3646, #48317, #37175, #50405 ) ) ;
#11313=ADVANCED_FACE ( 'NONE', ( #16039 ), #46975, .F. ) ;
#11314=CARTESIAN_POINT ( 'NONE',  ( -18.02786093087172503, -2.622721114510660367, 7.988897312896254377 ) ) ;
#11315=CARTESIAN_POINT ( 'NONE',  ( -11.30636317915456779, -0.1191753592594197858, 11.32220194836580340 ) ) ;
#11316=CARTESIAN_POINT ( 'NONE',  ( -18.21022926198954295, -3.432230869623162928, 3.845286450084705265 ) ) ;
#11318=PLANE ( 'NONE',  #26792 ) ;
#11319=EDGE_CURVE ( 'NONE', #26378, #39170, #50086, .T. ) ;
#11320=VECTOR ( 'NONE', #2525, 999.9999999999998863 ) ;
#11321=CARTESIAN_POINT ( 'NONE',  ( 2.072287782118878319, 0.000000000000000000, -2.950529333540147015 ) ) ;
#11322=VECTOR ( 'NONE', #40518, 1000.000000000000000 ) ;
#11323=ORIENTED_EDGE ( 'NONE', *, *, #35942, .F. ) ;
#11324=PLANE ( 'NONE',  #54602 ) ;
#11326=LINE ( 'NONE', #54756, #24010 ) ;
#11327=CARTESIAN_POINT ( 'NONE',  ( -12.77501498680632608, -4.727446477803164626, 1.692740485850688481 ) ) ;
#11328=VECTOR ( 'NONE', #1557, 1000.000000000000000 ) ;
#11329=DIRECTION ( 'NONE',  ( 0.005002170337468016433, -0.7660444431189770143, -0.6427681459581293666 ) ) ;
#11330=PLANE ( 'NONE',  #5554 ) ;
#11331=VECTOR ( 'NONE', #48535, 999.9999999999998863 ) ;
#11332=DIRECTION ( 'NONE',  ( -0.005002170337468016433, -0.7660444431189770143, 0.6427681459581293666 ) ) ;
#11333=LINE ( 'NONE', #29199, #49596 ) ;
#11334=LINE ( 'NONE', #41451, #53762 ) ;
#11335=EDGE_LOOP ( 'NONE', ( #51249, #44482, #56132, #26658 ) ) ;
#11337=VECTOR ( 'NONE', #11139, 1000.000000000000227 ) ;
#11338=VECTOR ( 'NONE', #13434, 999.9999999999998863 ) ;
#11339=ORIENTED_EDGE ( 'NONE', *, *, #16387, .T. ) ;
#11340=AXIS2_PLACEMENT_3D ( 'NONE', #7700, #25032, #3702 ) ;
#11341=DIRECTION ( 'NONE',  ( -0.6427681459581293666, -0.7660444431189770143, -0.005002170337467561935 ) ) ;
#11342=LINE ( 'NONE', #35876, #27392 ) ;
#11343=AXIS2_PLACEMENT_3D ( 'NONE', #38639, #21603, #12223 ) ;
#11344=VERTEX_POINT ( 'NONE', #12029 ) ;
#11346=DIRECTION ( 'NONE',  ( -0.005002170337468016433, -0.7660444431189770143, 0.6427681459581293666 ) ) ;
#11347=AXIS2_PLACEMENT_3D ( 'NONE', #34970, #17337, #30956 ) ;
#11348=ORIENTED_EDGE ( 'NONE', *, *, #3007, .T. ) ;
#11349=VECTOR ( 'NONE', #41615, 1000.000000000000227 ) ;
#11350=ORIENTED_EDGE ( 'NONE', *, *, #21055, .T. ) ;
#11351=ORIENTED_EDGE ( 'NONE', *, *, #10782, .F. ) ;
#11352=CARTESIAN_POINT ( 'NONE',  ( -25.20278734466900517, 0.000000000000000000, 6.670939612111840944 ) ) ;
#11353=PLANE ( 'NONE',  #1507 ) ;
#11354=LINE ( 'NONE', #5694, #46638 ) ;
#11355=EDGE_CURVE ( 'NONE', #18340, #53438, #2668, .T. ) ;
#11356=ORIENTED_EDGE ( 'NONE', *, *, #48008, .T. ) ;
#11357=ORIENTED_EDGE ( 'NONE', *, *, #8176, .F. ) ;
#11358=ADVANCED_FACE ( 'NONE', ( #19989 ), #7807, .F. ) ;
#11359=EDGE_CURVE ( 'NONE', #27927, #29027, #3526, .T. ) ;
#11360=AXIS2_PLACEMENT_3D ( 'NONE', #5280, #43876, #39900 ) ;
#11361=CARTESIAN_POINT ( 'NONE',  ( -11.15664249260607654, 0.000000000000000000, 4.933589610170957762 ) ) ;
#11362=LINE ( 'NONE', #6539, #18231 ) ;
#11363=AXIS2_PLACEMENT_3D ( 'NONE', #25403, #42712, #55788 ) ;
#11364=ORIENTED_EDGE ( 'NONE', *, *, #23780, .F. ) ;
#11365=DIRECTION ( 'NONE',  ( 0.005002170337468016433, -0.7660444431189770143, -0.6427681459581293666 ) ) ;
#11366=ORIENTED_EDGE ( 'NONE', *, *, #1230, .F. ) ;
#11367=VECTOR ( 'NONE', #10716, 1000.000000000000227 ) ;
#11368=DIRECTION ( 'NONE',  ( -0.005002170337468016433, -0.7660444431189770143, 0.6427681459581293666 ) ) ;
#11369=CARTESIAN_POINT ( 'NONE',  ( -18.39746900504187010, 0.000000000000000000, 14.03700784672088808 ) ) ;
#11370=VERTEX_POINT ( 'NONE', #20836 ) ;
#11371=PLANE ( 'NONE',  #15914 ) ;
#11372=VECTOR ( 'NONE', #4356, 1000.000000000000114 ) ;
#11373=DIRECTION ( 'NONE',  ( -0.7660212471507179544, -0.6427876096865405842, -0.005961354470445141482 ) ) ;
#11374=AXIS2_PLACEMENT_3D ( 'NONE', #1227, #53230, #14329 ) ;
#11375=AXIS2_PLACEMENT_3D ( 'NONE', #10931, #50677, #11766 ) ;
#11376=ORIENTED_EDGE ( 'NONE', *, *, #15292, .F. ) ;
#11378=DIRECTION ( 'NONE',  ( 0.007781995580012663651, -3.146120232559066537E-19, -0.9999697198139514409 ) ) ;
#11379=CARTESIAN_POINT ( 'NONE',  ( -2.207734231944874725, 7.028681301134739989, 4.075932526321295768 ) ) ;
#11380=VERTEX_POINT ( 'NONE', #38156 ) ;
#11381=AXIS2_PLACEMENT_3D ( 'NONE', #18100, #13566, #9601 ) ;
#11383=CARTESIAN_POINT ( 'NONE',  ( -19.32961685222932147, 0.000000000000000000, 14.39908572644263351 ) ) ;
#11384=DIRECTION ( 'NONE',  ( 0.9999697198139515519, 0.000000000000000000, 0.007781995580013368816 ) ) ;
#11385=LINE ( 'NONE', #3129, #25813 ) ;
#11386=FACE_OUTER_BOUND ( 'NONE', #1516, .T. ) ;
#11387=EDGE_CURVE ( 'NONE', #34545, #83, #12346, .T. ) ;
#11388=CARTESIAN_POINT ( 'NONE',  ( -16.09107322271225016, -0.3560938001956550081, 3.516661618153204216 ) ) ;
#11389=CARTESIAN_POINT ( 'NONE',  ( -17.51878260850159563, 5.143464774974012776, 3.322718381678418709 ) ) ;
#11390=AXIS2_PLACEMENT_3D ( 'NONE', #21496, #47302, #8409 ) ;
#11391=AXIS2_PLACEMENT_3D ( 'NONE', #47206, #4064, #51747 ) ;
#11392=FACE_OUTER_BOUND ( 'NONE', #37119, .T. ) ;
#11393=EDGE_LOOP ( 'NONE', ( #30968, #14745, #34254, #42848 ) ) ;
#11395=ADVANCED_FACE ( 'NONE', ( #29929 ), #52058, .F. ) ;
#11396=CARTESIAN_POINT ( 'NONE',  ( -18.67775241435682432, 0.000000000000000000, 4.136394454059623804 ) ) ;
#11398=ORIENTED_EDGE ( 'NONE', *, *, #34825, .T. ) ;
#11399=DIRECTION ( 'NONE',  ( -0.5449076811759708816, 0.6444004775717707689, 0.5364919789714475140 ) ) ;
#11400=CARTESIAN_POINT ( 'NONE',  ( -20.15755334212245842, 3.848249166794009302, 4.389030706747201194 ) ) ;
#11401=EDGE_CURVE ( 'NONE', #37283, #46770, #51772, .T. ) ;
#11402=EDGE_CURVE ( 'NONE', #43237, #36649, #21423, .T. ) ;
#11403=CARTESIAN_POINT ( 'NONE',  ( -12.68505759159693014, -0.1191753592594172878, 8.145680730609152320 ) ) ;
#11404=LINE ( 'NONE', #28734, #13322 ) ;
#11405=DIRECTION ( 'NONE',  ( -0.5364919789714478471, 0.6444004775717705469, -0.5449076811759709926 ) ) ;
#11406=VECTOR ( 'NONE', #29585, 1000.000000000000000 ) ;
#11407=ORIENTED_EDGE ( 'NONE', *, *, #20620, .T. ) ;
#11408=ORIENTED_EDGE ( 'NONE', *, *, #50647, .T. ) ;
#11409=VECTOR ( 'NONE', #37176, 999.9999999999998863 ) ;
#11411=VECTOR ( 'NONE', #35352, 999.9999999999998863 ) ;
#11413=FACE_OUTER_BOUND ( 'NONE', #11843, .T. ) ;
#11414=ORIENTED_EDGE ( 'NONE', *, *, #40533, .T. ) ;
#11415=DIRECTION ( 'NONE',  ( 0.9999697198139515519, 0.000000000000000000, 0.007781995580013368816 ) ) ;
#11416=VECTOR ( 'NONE', #20160, 999.9999999999998863 ) ;
#11417=ORIENTED_EDGE ( 'NONE', *, *, #54971, .F. ) ;
#11418=DIRECTION ( 'NONE',  ( 0.007781995580012662783, 0.000000000000000000, -0.9999697198139514409 ) ) ;
#11419=EDGE_CURVE ( 'NONE', #49166, #3505, #51520, .T. ) ;
#11420=VECTOR ( 'NONE', #46218, 999.9999999999998863 ) ;
#11421=VECTOR ( 'NONE', #38466, 1000.000000000000000 ) ;
#11422=ORIENTED_EDGE ( 'NONE', *, *, #23705, .T. ) ;
#11423=ORIENTED_EDGE ( 'NONE', *, *, #46266, .F. ) ;
#11424=DIRECTION ( 'NONE',  ( 0.007781995580012663651, 0.000000000000000000, -0.9999697198139515519 ) ) ;
#11425=AXIS2_PLACEMENT_3D ( 'NONE', #19192, #1617, #15490 ) ;
#11427=CARTESIAN_POINT ( 'NONE',  ( -18.66354898467281132, 0.000000000000000000, 14.21960318569776582 ) ) ;
#11428=FACE_OUTER_BOUND ( 'NONE', #26675, .T. ) ;
#11429=VECTOR ( 'NONE', #55522, 999.9999999999998863 ) ;
#11430=VERTEX_POINT ( 'NONE', #25969 ) ;
#11431=VECTOR ( 'NONE', #54721, 999.9999999999998863 ) ;
#11432=CARTESIAN_POINT ( 'NONE',  ( -16.85162240165947978, -0.1191753592594174960, 7.374591420219792859 ) ) ;
#11433=EDGE_CURVE ( 'NONE', #16969, #42632, #26491, .T. ) ;
#11434=EDGE_LOOP ( 'NONE', ( #16119, #16902, #24548 ) ) ;
#11436=AXIS2_PLACEMENT_3D ( 'NONE', #27013, #21635, #4857 ) ;
#11437=ORIENTED_EDGE ( 'NONE', *, *, #24733, .F. ) ;
#11438=VECTOR ( 'NONE', #27460, 999.9999999999998863 ) ;
#11439=ORIENTED_EDGE ( 'NONE', *, *, #39599, .T. ) ;
#11440=CARTESIAN_POINT ( 'NONE',  ( 2.072287782118878319, 0.000000000000000000, -2.950529333540147015 ) ) ;
#11441=CARTESIAN_POINT ( 'NONE',  ( -9.894967649688549471, -0.1191753592594202438, 1.519416599161745429 ) ) ;
#11442=VERTEX_POINT ( 'NONE', #47230 ) ;
#11443=CARTESIAN_POINT ( 'NONE',  ( -17.74065527477223725, 3.686347215771509145, 9.822317904363528029 ) ) ;
#11444=VERTEX_POINT ( 'NONE', #39008 ) ;
#11445=PLANE ( 'NONE',  #26738 ) ;
#11446=DIRECTION ( 'NONE',  ( 0.5449076811759707706, 0.6444004775717708799, -0.5364919789714476250 ) ) ;
#11447=ORIENTED_EDGE ( 'NONE', *, *, #40873, .F. ) ;
#11448=CARTESIAN_POINT ( 'NONE',  ( -9.835408328977019110, -0.8172783914120439475, 1.672748508373830045 ) ) ;
#11449=ORIENTED_EDGE ( 'NONE', *, *, #4055, .T. ) ;
#11450=AXIS2_PLACEMENT_3D ( 'NONE', #16642, #37955, #56121 ) ;
#11451=EDGE_CURVE ( 'NONE', #2187, #3168, #44112, .T. ) ;
#11452=DIRECTION ( 'NONE',  ( -0.9999697198139514409, -0.000000000000000000, -0.007781995580013368816 ) ) ;
#11453=DIRECTION ( 'NONE',  ( 0.7660212471507180654, -0.6427876096865404731, 0.005961354470445141482 ) ) ;
#11454=LINE ( 'NONE', #45798, #38623 ) ;
#11455=DIRECTION ( 'NONE',  ( 0.6427681459581294776, -0.7660444431189769032, 0.005002170337467562802 ) ) ;
#11456=CARTESIAN_POINT ( 'NONE',  ( -19.32961685222932147, 0.000000000000000000, 14.39908572644263351 ) ) ;
#11457=VECTOR ( 'NONE', #39180, 1000.000000000000227 ) ;
#11458=ORIENTED_EDGE ( 'NONE', *, *, #45286, .F. ) ;
#11459=ORIENTED_EDGE ( 'NONE', *, *, #40291, .T. ) ;
#11460=CARTESIAN_POINT ( 'NONE',  ( 2.072287782118878319, 0.000000000000000000, -2.950529333540147015 ) ) ;
#11461=VECTOR ( 'NONE', #53341, 1000.000000000000227 ) ;
#11462=LINE ( 'NONE', #7195, #13080 ) ;
#11463=CARTESIAN_POINT ( 'NONE',  ( -17.89448523529146229, 0.000000000000000000, 9.113132941433205403 ) ) ;
#11464=CARTESIAN_POINT ( 'NONE',  ( -21.47263955680318404, 0.000000000000000000, 5.022634149262071190 ) ) ;
#11465=FACE_OUTER_BOUND ( 'NONE', #11866, .T. ) ;
#11466=VECTOR ( 'NONE', #34314, 1000.000000000000227 ) ;
#11467=CARTESIAN_POINT ( 'NONE',  ( -12.15271748404464880, 0.000000000000000000, 1.601849296007406664 ) ) ;
#11468=ORIENTED_EDGE ( 'NONE', *, *, #49746, .F. ) ;
#11469=LINE ( 'NONE', #15426, #44922 ) ;
#11470=CARTESIAN_POINT ( 'NONE',  ( -22.40634380310664397, 0.000000000000000000, 5.584705972946605534 ) ) ;
#11471=ORIENTED_EDGE ( 'NONE', *, *, #20598, .T. ) ;
#11472=DIRECTION ( 'NONE',  ( -0.8531650599175529814, -0.4028455766673920135, 0.3313982828793697877 ) ) ;
#11473=PLANE ( 'NONE',  #44894 ) ;
#11474=ORIENTED_EDGE ( 'NONE', *, *, #23546, .T. ) ;
#11475=AXIS2_PLACEMENT_3D ( 'NONE', #6795, #24119, #15863 ) ;
#11476=CARTESIAN_POINT ( 'NONE',  ( 2.072287782118878319, 0.000000000000000000, -2.950529333540147015 ) ) ;
#11477=DIRECTION ( 'NONE',  ( -0.9999697198139514409, -0.000000000000000000, -0.007781995580013368816 ) ) ;
#11478=VECTOR ( 'NONE', #39620, 1000.000000000000227 ) ;
#11480=DIRECTION ( 'NONE',  ( 0.5449076811759707706, 0.6444004775717708799, -0.5364919789714476250 ) ) ;
#11481=CARTESIAN_POINT ( 'NONE',  ( -14.23481991729512508, 4.010151117816509903, 2.083274387783130788 ) ) ;
#11482=AXIS2_PLACEMENT_3D ( 'NONE', #43673, #13587, #17279 ) ;
#11483=LINE ( 'NONE', #1813, #11074 ) ;
#11484=ORIENTED_EDGE ( 'NONE', *, *, #29853, .T. ) ;
#11485=VECTOR ( 'NONE', #12011, 999.9999999999998863 ) ;
#11487=CARTESIAN_POINT ( 'NONE',  ( -16.93072279954589732, 0.000000000000000000, 4.688648325876052070 ) ) ;
#11488=DIRECTION ( 'NONE',  ( -0.7660212471507179544, -0.6427876096865405842, -0.005961354470445141482 ) ) ;
#11489=LINE ( 'NONE', #16030, #23349 ) ;
#11490=EDGE_CURVE ( 'NONE', #28225, #51442, #4926, .T. ) ;
#11491=CARTESIAN_POINT ( 'NONE',  ( -16.93934496006174228, 0.000000000000000000, 5.796577435649344245 ) ) ;
#11492=CARTESIAN_POINT ( 'NONE',  ( 2.072287782118878319, 0.000000000000000000, -2.950529333540147015 ) ) ;
#11493=LINE ( 'NONE', #55199, #13143 ) ;
#11494=ORIENTED_EDGE ( 'NONE', *, *, #27772, .T. ) ;
#11495=EDGE_CURVE ( 'NONE', #54842, #5666, #30208, .T. ) ;
#11496=DIRECTION ( 'NONE',  ( -0.6427681459581293666, -0.7660444431189770143, -0.005002170337467561935 ) ) ;
#11497=ADVANCED_FACE ( 'NONE', ( #13458 ), #26227, .F. ) ;
#11498=VECTOR ( 'NONE', #32429, 999.9999999999998863 ) ;
#11499=CARTESIAN_POINT ( 'NONE',  ( -13.59341601676131539, -0.1191753592594177180, 6.661283396080332153 ) ) ;
#11500=DIRECTION ( 'NONE',  ( 0.000000000000000000, -0.000000000000000000, -1.000000000000000000 ) ) ;
#11501=ORIENTED_EDGE ( 'NONE', *, *, #37957, .T. ) ;
#11502=PLANE ( 'NONE',  #32910 ) ;
#11503=ADVANCED_FACE ( 'NONE', ( #9179 ), #76, .F. ) ;
#11504=LINE ( 'NONE', #46125, #28619 ) ;
#11505=CARTESIAN_POINT ( 'NONE',  ( -9.110551994824897193, -1.000000000000000000, 3.538847790438064411 ) ) ;
#11506=ORIENTED_EDGE ( 'NONE', *, *, #53734, .T. ) ;
#11507=DIRECTION ( 'NONE',  ( -0.6427681459581293666, -0.7660444431189770143, -0.005002170337467561935 ) ) ;
#11508=EDGE_CURVE ( 'NONE', #6097, #21737, #21697, .T. ) ;
#11509=VECTOR ( 'NONE', #56122, 999.9999999999998863 ) ;
#11510=ORIENTED_EDGE ( 'NONE', *, *, #44814, .F. ) ;
#11511=EDGE_CURVE ( 'NONE', #1661, #21438, #52359, .T. ) ;
#11512=ORIENTED_EDGE ( 'NONE', *, *, #289, .F. ) ;
#11513=VECTOR ( 'NONE', #34256, 999.9999999999998863 ) ;
#11514=ORIENTED_EDGE ( 'NONE', *, *, #4572, .F. ) ;
#11515=ORIENTED_EDGE ( 'NONE', *, *, #54741, .T. ) ;
#11516=ORIENTED_EDGE ( 'NONE', *, *, #32351, .T. ) ;
#11517=CARTESIAN_POINT ( 'NONE',  ( -14.42191463890408798, 0.000000000000000000, 6.554832800120924396 ) ) ;
#11518=ORIENTED_EDGE ( 'NONE', *, *, #15624, .F. ) ;
#11519=EDGE_CURVE ( 'NONE', #33225, #37986, #17992, .T. ) ;
#11520=VECTOR ( 'NONE', #11722, 1000.000000000000227 ) ;
#11521=ORIENTED_EDGE ( 'NONE', *, *, #7885, .T. ) ;
#11523=ORIENTED_EDGE ( 'NONE', *, *, #32351, .F. ) ;
#11524=ORIENTED_EDGE ( 'NONE', *, *, #27785, .F. ) ;
#11525=EDGE_CURVE ( 'NONE', #8997, #26804, #18540, .T. ) ;
#11526=AXIS2_PLACEMENT_3D ( 'NONE', #16781, #9095, #4557 ) ;
#11527=LINE ( 'NONE', #29096, #24732 ) ;
#11528=LINE ( 'NONE', #19471, #33052 ) ;
#11530=CARTESIAN_POINT ( 'NONE',  ( 1.086233639165236964, -1.000000000000000000, 2.796443541562362078 ) ) ;
#11531=EDGE_LOOP ( 'NONE', ( #37842, #43601, #9560, #54347 ) ) ;
#11532=DIRECTION ( 'NONE',  ( 0.000000000000000000, -1.000000000000000000, 0.000000000000000000 ) ) ;
#11533=EDGE_LOOP ( 'NONE', ( #43609, #43808, #34998, #4129 ) ) ;
#11534=VERTEX_POINT ( 'NONE', #44644 ) ;
#11535=CARTESIAN_POINT ( 'NONE',  ( -15.33394411155456716, 0.000000000000000000, 4.331742757038320235 ) ) ;
#11536=PLANE ( 'NONE',  #1268 ) ;
#11538=LINE ( 'NONE', #42471, #26699 ) ;
#11539=CARTESIAN_POINT ( 'NONE',  ( -14.66887761629205222, 0.000000000000000000, 12.58869632783390990 ) ) ;
#11540=CARTESIAN_POINT ( 'NONE',  ( -19.79569077582305070, 0.000000000000000000, 14.58012466630350445 ) ) ;
#11541=EDGE_LOOP ( 'NONE', ( #48361, #25076, #17336, #32794 ) ) ;
#11542=CARTESIAN_POINT ( 'NONE',  ( -10.00813838035478298, 0.000000000000000000, 10.77830692922518452 ) ) ;
#11543=ORIENTED_EDGE ( 'NONE', *, *, #16462, .T. ) ;
#11544=CARTESIAN_POINT ( 'NONE',  ( -20.83449926979080757, -4.889348428825663895, 4.818152362712800674 ) ) ;
#11545=CARTESIAN_POINT ( 'NONE',  ( -32.65997012216863737, 0.000000000000000000, 9.567562649885804404 ) ) ;
#11546=AXIS2_PLACEMENT_3D ( 'NONE', #39589, #43538, #21952 ) ;
#11547=CARTESIAN_POINT ( 'NONE',  ( 2.072287782118878319, 0.000000000000000000, -2.950529333540147015 ) ) ;
#11549=DIRECTION ( 'NONE',  ( 0.007781995580012662783, 0.000000000000000000, -0.9999697198139514409 ) ) ;
#11550=CARTESIAN_POINT ( 'NONE',  ( -12.58811780613994813, -1.165603555308156736, 3.484538193242154414 ) ) ;
#11551=VECTOR ( 'NONE', #25119, 1000.000000000000227 ) ;
#11553=EDGE_LOOP ( 'NONE', ( #38970, #22651, #19678, #34289 ) ) ;
#11554=DIRECTION ( 'NONE',  ( 0.5364919789714477361, 0.6444004775717706579, 0.5449076811759711036 ) ) ;
#11555=PLANE ( 'NONE',  #20437 ) ;
#11556=DIRECTION ( 'NONE',  ( 0.007781995580012662783, 0.000000000000000000, -0.9999697198139514409 ) ) ;
#11557=EDGE_CURVE ( 'NONE', #41770, #37828, #53208, .T. ) ;
#11558=ADVANCED_FACE ( 'NONE', ( #44380 ), #10305, .F. ) ;
#11559=VECTOR ( 'NONE', #7533, 999.9999999999998863 ) ;
#11560=DIRECTION ( 'NONE',  ( -0.5449076811759708816, 0.6444004775717707689, 0.5364919789714475140 ) ) ;
#11561=CARTESIAN_POINT ( 'NONE',  ( -13.21397773654151209, -4.079838673713161334, 8.510399755611151917 ) ) ;
#11562=DIRECTION ( 'NONE',  ( 0.005002170337468016433, -0.7660444431189770143, -0.6427681459581293666 ) ) ;
#11563=DIRECTION ( 'NONE',  ( -0.005961354470445682716, -0.6427876096865404731, 0.7660212471507180654 ) ) ;
#11564=ADVANCED_FACE ( 'NONE', ( #22796 ), #40694, .F. ) ;
#11565=DIRECTION ( 'NONE',  ( 0.005961354470445682716, -0.6427876096865404731, -0.7660212471507180654 ) ) ;
#11567=EDGE_LOOP ( 'NONE', ( #19833, #42700, #55957, #55557 ) ) ;
#11569=EDGE_CURVE ( 'NONE', #27005, #31631, #18248, .T. ) ;
#11570=ORIENTED_EDGE ( 'NONE', *, *, #54005, .F. ) ;
#11571=ORIENTED_EDGE ( 'NONE', *, *, #47299, .F. ) ;
#11572=ORIENTED_EDGE ( 'NONE', *, *, #911, .T. ) ;
#11573=EDGE_CURVE ( 'NONE', #12635, #1853, #31618, .T. ) ;
#11574=ORIENTED_EDGE ( 'NONE', *, *, #26493, .T. ) ;
#11575=FACE_OUTER_BOUND ( 'NONE', #8204, .T. ) ;
#11577=CARTESIAN_POINT ( 'NONE',  ( -16.47339040883137784, 0.000000000000000000, 5.630877588122378263 ) ) ;
#11578=ADVANCED_FACE ( 'NONE', ( #27331 ), #27628, .F. ) ;
#11579=ORIENTED_EDGE ( 'NONE', *, *, #41656, .F. ) ;
#11580=ORIENTED_EDGE ( 'NONE', *, *, #27574, .F. ) ;
#11581=ORIENTED_EDGE ( 'NONE', *, *, #55345, .T. ) ;
#11583=EDGE_LOOP ( 'NONE', ( #44535, #35315, #2258, #53291 ) ) ;
#11584=AXIS2_PLACEMENT_3D ( 'NONE', #36153, #40937, #18530 ) ;
#11586=CARTESIAN_POINT ( 'NONE',  ( -16.43317633868556626, -0.1191753592594197858, 13.31363028683540151 ) ) ;
#11587=DIRECTION ( 'NONE',  ( -0.6427681459581293666, -0.7660444431189770143, -0.005002170337467561935 ) ) ;
#11588=ORIENTED_EDGE ( 'NONE', *, *, #54124, .T. ) ;
#11589=LINE ( 'NONE', #46201, #22875 ) ;
#11591=AXIS2_PLACEMENT_3D ( 'NONE', #30476, #52584, #22510 ) ;
#11592=CARTESIAN_POINT ( 'NONE',  ( -17.35095301433918991, -0.1941918491731536578, 3.740333030968461703 ) ) ;
#11593=DIRECTION ( 'NONE',  ( 0.9999697198139515519, 0.000000000000000000, 0.007781995580013368816 ) ) ;
#11594=CARTESIAN_POINT ( 'NONE',  ( -11.87243407472968926, 0.000000000000000000, 11.50246268866867361 ) ) ;
#11595=CARTESIAN_POINT ( 'NONE',  ( -10.94028622754223967, 0.000000000000000000, 11.14038480894692995 ) ) ;
#11596=DIRECTION ( 'NONE',  ( -0.005961354470445682716, -0.6427876096865404731, 0.7660212471507180654 ) ) ;
#11597=PLANE ( 'NONE',  #51186 ) ;
#11598=DIRECTION ( 'NONE',  ( -0.6427681459581293666, -0.7660444431189770143, -0.005002170337467561935 ) ) ;
#11599=DIRECTION ( 'NONE',  ( -0.2426528472758542054, 0.7422098413412800966, -0.6246952433987894571 ) ) ;
#11600=EDGE_LOOP ( 'NONE', ( #14120, #38128, #28026, #43928 ) ) ;
#11601=CARTESIAN_POINT ( 'NONE',  ( -9.542064456761055524, 0.000000000000000000, 10.59726798936431180 ) ) ;
#11602=ORIENTED_EDGE ( 'NONE', *, *, #1547, .T. ) ;
#11603=ADVANCED_FACE ( 'NONE', ( #924 ), #53461, .F. ) ;
#11604=LINE ( 'NONE', #27825, #8393 ) ;
#11605=PLANE ( 'NONE',  #22390 ) ;
#11606=FACE_OUTER_BOUND ( 'NONE', #32599, .T. ) ;
#11608=CARTESIAN_POINT ( 'NONE',  ( -9.075990533167328067, 0.000000000000000000, 10.41622904950343909 ) ) ;
#11609=DIRECTION ( 'NONE',  ( -0.6427681459581293666, -0.7660444431189770143, -0.005002170337467561935 ) ) ;
#11610=PLANE ( 'NONE',  #53823 ) ;
#11613=EDGE_CURVE ( 'NONE', #41926, #46588, #26389, .T. ) ;
#11614=DIRECTION ( 'NONE',  ( 0.7660212471507180654, -0.6427876096865404731, 0.005961354470445141482 ) ) ;
#11615=CARTESIAN_POINT ( 'NONE',  ( -27.99767448711536133, 0.000000000000000000, 7.557179307314289218 ) ) ;
#11616=DIRECTION ( 'NONE',  ( 0.007781995580012663651, 0.000000000000000000, -0.9999697198139515519 ) ) ;
#11617=LINE ( 'NONE', #11327, #5533 ) ;
#11618=ADVANCED_FACE ( 'NONE', ( #48548 ), #17307, .F. ) ;
#11619=CARTESIAN_POINT ( 'NONE',  ( -16.81190032086591302, 0.000000000000000000, 3.212244750653343583 ) ) ;
#11620=EDGE_CURVE ( 'NONE', #12878, #45628, #43703, .T. ) ;
#11621=ADVANCED_FACE ( 'NONE', ( #35478 ), #4542, .F. ) ;
#11622=CARTESIAN_POINT ( 'NONE',  ( -13.76180149347061032, 0.1245042932765029059, 2.023510445493768906 ) ) ;
#11623=LINE ( 'NONE', #28359, #6696 ) ;
#11624=EDGE_CURVE ( 'NONE', #39606, #27112, #9666, .T. ) ;
#11625=DIRECTION ( 'NONE',  ( -0.005961354470445682716, -0.6427876096865404731, 0.7660212471507180654 ) ) ;
#11626=DIRECTION ( 'NONE',  ( -0.9999697198139514409, -0.000000000000000000, -0.007781995580013368816 ) ) ;
#11627=ORIENTED_EDGE ( 'NONE', *, *, #40754, .T. ) ;
#11628=FACE_OUTER_BOUND ( 'NONE', #15332, .T. ) ;
#11629=DIRECTION ( 'NONE',  ( 0.007781995580012662783, 0.000000000000000000, -0.9999697198139514409 ) ) ;
#11630=ORIENTED_EDGE ( 'NONE', *, *, #1624, .F. ) ;
#11632=DIRECTION ( 'NONE',  ( 0.000000000000000000, -1.000000000000000000, 0.000000000000000000 ) ) ;
#11633=VECTOR ( 'NONE', #1257, 999.9999999999998863 ) ;
#11634=VERTEX_POINT ( 'NONE', #47416 ) ;
#11636=LINE ( 'NONE', #13255, #25690 ) ;
#11637=ADVANCED_FACE ( 'NONE', ( #44294 ), #12780, .F. ) ;
#11638=ORIENTED_EDGE ( 'NONE', *, *, #47373, .F. ) ;
#11639=EDGE_LOOP ( 'NONE', ( #34676, #11072, #8078, #14922 ) ) ;
#11640=ORIENTED_EDGE ( 'NONE', *, *, #19755, .T. ) ;
#11641=EDGE_CURVE ( 'NONE', #46009, #46872, #21852, .T. ) ;
#11642=FACE_OUTER_BOUND ( 'NONE', #1837, .T. ) ;
#11644=CARTESIAN_POINT ( 'NONE',  ( -12.52756075508707667, 0.000000000000000000, 1.968264248804815209 ) ) ;
#11645=EDGE_CURVE ( 'NONE', #41020, #17065, #13367, .T. ) ;
#11646=ORIENTED_EDGE ( 'NONE', *, *, #43413, .F. ) ;
#11647=VERTEX_POINT ( 'NONE', #836 ) ;
#11648=ADVANCED_FACE ( 'NONE', ( #22702 ), #26680, .F. ) ;
#11649=DIRECTION ( 'NONE',  ( 0.000000000000000000, -1.000000000000000000, 0.000000000000000000 ) ) ;
#11650=FACE_OUTER_BOUND ( 'NONE', #33457, .T. ) ;
#11651=ORIENTED_EDGE ( 'NONE', *, *, #27525, .F. ) ;
#11652=CARTESIAN_POINT ( 'NONE',  ( -19.60990026154428278, 0.000000000000000000, 4.498472333781370125 ) ) ;
#11653=ORIENTED_EDGE ( 'NONE', *, *, #20539, .T. ) ;
#11654=DIRECTION ( 'NONE',  ( -0.5449076811759708816, 0.6444004775717707689, 0.5364919789714475140 ) ) ;
#11655=LINE ( 'NONE', #28969, #3122 ) ;
#11656=ORIENTED_EDGE ( 'NONE', *, *, #29719, .F. ) ;
#11657=DIRECTION ( 'NONE',  ( 0.007781995580012663651, 0.000000000000000000, -0.9999697198139515519 ) ) ;
#11658=LINE ( 'NONE', #28973, #43616 ) ;
#11659=ORIENTED_EDGE ( 'NONE', *, *, #22192, .T. ) ;
#11662=DIRECTION ( 'NONE',  ( -0.8531650599175529814, -0.4028455766673920135, 0.3313982828793697877 ) ) ;
#11663=ORIENTED_EDGE ( 'NONE', *, *, #41490, .T. ) ;
#11664=VECTOR ( 'NONE', #14536, 1000.000000000000227 ) ;
#11665=CARTESIAN_POINT ( 'NONE',  ( -31.72626587586518099, 0.000000000000000000, 9.005490826201270949 ) ) ;
#11666=DIRECTION ( 'NONE',  ( 0.005961354470445682716, -0.6427876096865404731, -0.7660212471507180654 ) ) ;
#11667=LINE ( 'NONE', #32430, #13118 ) ;
#11668=DIRECTION ( 'NONE',  ( 0.000000000000000000, -0.000000000000000000, -1.000000000000000000 ) ) ;
#11669=CARTESIAN_POINT ( 'NONE',  ( -9.026147446236871374, 0.000000000000000000, 4.011499419416683310 ) ) ;
#11670=LINE ( 'NONE', #12523, #37903 ) ;
#11672=ORIENTED_EDGE ( 'NONE', *, *, #45827, .F. ) ;
#11673=DIRECTION ( 'NONE',  ( 0.000000000000000000, -1.000000000000000000, 0.000000000000000000 ) ) ;
#11674=DIRECTION ( 'NONE',  ( 0.007781995580012662783, 0.000000000000000000, -0.9999697198139514409 ) ) ;
#11675=CARTESIAN_POINT ( 'NONE',  ( -18.61095121660043361, 0.000000000000000000, 7.460902944687155980 ) ) ;
#11676=EDGE_LOOP ( 'NONE', ( #52611, #36564, #42857 ) ) ;
#11677=CARTESIAN_POINT ( 'NONE',  ( -16.40828346936073245, 1.581621852479006440, 5.850566556248715244 ) ) ;
#11679=EDGE_CURVE ( 'NONE', #48505, #11768, #17602, .T. ) ;
#11680=EDGE_CURVE ( 'NONE', #2289, #4025, #22143, .T. ) ;
#11681=CARTESIAN_POINT ( 'NONE',  ( -17.73140113748535285, 0.000000000000000000, 13.85752530597602039 ) ) ;
#11682=EDGE_CURVE ( 'NONE', #4466, #42667, #44000, .T. ) ;
#11683=CARTESIAN_POINT ( 'NONE',  ( -20.36251083028806619, 2.391131607591507446, 8.715066169111624461 ) ) ;
#11684=DIRECTION ( 'NONE',  ( 0.005002170337468016433, -0.7660444431189770143, -0.6427681459581293666 ) ) ;
#11685=VERTEX_POINT ( 'NONE', #52786 ) ;
#11686=ORIENTED_EDGE ( 'NONE', *, *, #8906, .F. ) ;
#11687=CARTESIAN_POINT ( 'NONE',  ( -27.06708303904391144, 0.000000000000000000, 7.395095371555332697 ) ) ;
#11688=DIRECTION ( 'NONE',  ( -0.005002170337468016433, -0.7660444431189770143, 0.6427681459581293666 ) ) ;
#11690=LINE ( 'NONE', #12252, #33130 ) ;
#11691=ORIENTED_EDGE ( 'NONE', *, *, #50385, .F. ) ;
#11692=CARTESIAN_POINT ( 'NONE',  ( -14.24822155599092888, -3.108426967578160394, 7.317883074450481473 ) ) ;
#11693=ORIENTED_EDGE ( 'NONE', *, *, #18834, .F. ) ;
#11694=ORIENTED_EDGE ( 'NONE', *, *, #7228, .F. ) ;
#11695=ORIENTED_EDGE ( 'NONE', *, *, #3269, .T. ) ;
#11696=DIRECTION ( 'NONE',  ( 0.7660212471507180654, -0.6427876096865404731, 0.005961354470445141482 ) ) ;
#11697=DIRECTION ( 'NONE',  ( 0.9999697198139515519, 0.000000000000000000, 0.007781995580013368816 ) ) ;
#11698=DIRECTION ( 'NONE',  ( 0.005002170337468016433, -0.7660444431189770143, -0.6427681459581293666 ) ) ;
#11699=VERTEX_POINT ( 'NONE', #43187 ) ;
#11700=( GEOMETRIC_REPRESENTATION_CONTEXT ( 3 ) GLOBAL_UNCERTAINTY_ASSIGNED_CONTEXT ( ( #15487 ) ) GLOBAL_UNIT_ASSIGNED_CONTEXT ( ( #40020, #53103, #22454 ) ) REPRESENTATION_CONTEXT ( 'NONE', 'WORKASPACE' ) );
#11701=PLANE ( 'NONE',  #20175 ) ;
#11702=ORIENTED_EDGE ( 'NONE', *, *, #20276, .F. ) ;
#11703=EDGE_CURVE ( 'NONE', #28441, #7819, #51948, .T. ) ;
#11704=VERTEX_POINT ( 'NONE', #39474 ) ;
#11705=ORIENTED_EDGE ( 'NONE', *, *, #8788, .F. ) ;
#11706=CARTESIAN_POINT ( 'NONE',  ( -21.47263955680318404, 0.000000000000000000, 5.022634149262071190 ) ) ;
#11707=EDGE_CURVE ( 'NONE', #12718, #8024, #56218, .T. ) ;
#11708=FACE_OUTER_BOUND ( 'NONE', #46194, .T. ) ;
#11709=ORIENTED_EDGE ( 'NONE', *, *, #37964, .F. ) ;
#11710=DIRECTION ( 'NONE',  ( -0.005961354470445682716, -0.6427876096865404731, 0.7660212471507180654 ) ) ;
#11711=ORIENTED_EDGE ( 'NONE', *, *, #241, .T. ) ;
#11714=ORIENTED_EDGE ( 'NONE', *, *, #12741, .F. ) ;
#11715=EDGE_CURVE ( 'NONE', #2289, #19074, #34371, .T. ) ;
#11716=CARTESIAN_POINT ( 'NONE',  ( -9.808144436391993182, 0.000000000000000000, 10.77986332834118777 ) ) ;
#11717=ORIENTED_EDGE ( 'NONE', *, *, #37989, .F. ) ;
#11718=DIRECTION ( 'NONE',  ( -0.8531650599175527594, 0.4028455766673922356, 0.3313982828793700652 ) ) ;
#11719=DIRECTION ( 'NONE',  ( 0.5449076811759707706, 0.6444004775717708799, -0.5364919789714476250 ) ) ;
#11720=DIRECTION ( 'NONE',  ( 0.000000000000000000, -1.000000000000000000, 0.000000000000000000 ) ) ;
#11721=PLANE ( 'NONE',  #20250 ) ;
#11722=DIRECTION ( 'NONE',  ( -0.5449076811759708816, 0.6444004775717707689, 0.5364919789714475140 ) ) ;
#11723=CARTESIAN_POINT ( 'NONE',  ( -16.53317331066696383, 0.000000000000000000, 13.31285208727739899 ) ) ;
#11724=VERTEX_POINT ( 'NONE', #5124 ) ;
#11725=ORIENTED_EDGE ( 'NONE', *, *, #36419, .T. ) ;
#11726=FACE_OUTER_BOUND ( 'NONE', #28457, .T. ) ;
#11729=CARTESIAN_POINT ( 'NONE',  ( 3.882677180727608590, -1.000000000000000000, 1.710209902397122672 ) ) ;
#11730=CARTESIAN_POINT ( 'NONE',  ( -25.20123094555300369, 0.000000000000000000, 6.470945668149052032 ) ) ;
#11731=DIRECTION ( 'NONE',  ( 0.005002170337468016433, -0.7660444431189770143, -0.6427681459581293666 ) ) ;
#11732=ORIENTED_EDGE ( 'NONE', *, *, #5946, .T. ) ;
#11733=LINE ( 'NONE', #54590, #36784 ) ;
#11734=DIRECTION ( 'NONE',  ( 0.007781995580012662783, 0.000000000000000000, -0.9999697198139514409 ) ) ;
#11735=ORIENTED_EDGE ( 'NONE', *, *, #45155, .T. ) ;
#11736=DIRECTION ( 'NONE',  ( -0.7660212471507179544, -0.6427876096865405842, -0.005961354470445141482 ) ) ;
#11737=EDGE_CURVE ( 'NONE', #5309, #18585, #34630, .T. ) ;
#11738=CARTESIAN_POINT ( 'NONE',  ( -19.69569380384165669, -0.1191753592594177458, 14.58090286586150697 ) ) ;
#11739=ORIENTED_EDGE ( 'NONE', *, *, #9612, .F. ) ;
#11740=EDGE_CURVE ( 'NONE', #5490, #2403, #6239, .T. ) ;
#11742=DIRECTION ( 'NONE',  ( 0.9999697198139515519, 0.000000000000000000, 0.007781995580013368816 ) ) ;
#11743=DIRECTION ( 'NONE',  ( 0.007781995580012663651, 0.000000000000000000, -0.9999697198139515519 ) ) ;
#11744=EDGE_CURVE ( 'NONE', #41657, #37529, #14211, .T. ) ;
#11746=PLANE ( 'NONE',  #47768 ) ;
#11747=DIRECTION ( 'NONE',  ( 0.007781995580012663651, 0.000000000000000000, -0.9999697198139515519 ) ) ;
#11748=ORIENTED_EDGE ( 'NONE', *, *, #40363, .T. ) ;
#11749=EDGE_LOOP ( 'NONE', ( #38603, #35732, #42157 ) ) ;
#11750=DIRECTION ( 'NONE',  ( 0.6427681459581294776, -0.7660444431189769032, 0.005002170337467562802 ) ) ;
#11751=DIRECTION ( 'NONE',  ( -0.005002170337468016433, -0.7660444431189770143, 0.6427681459581293666 ) ) ;
#11753=CARTESIAN_POINT ( 'NONE',  ( -18.73788634529089236, 2.714935509636508204, 3.873742472295404138 ) ) ;
#11754=DIRECTION ( 'NONE',  ( 0.005961354470445682716, -0.6427876096865404731, -0.7660212471507180654 ) ) ;
#11755=CARTESIAN_POINT ( 'NONE',  ( -20.18150129800645587, 0.9810866208979801550, 5.686756014922062619 ) ) ;
#11756=EDGE_LOOP ( 'NONE', ( #14848, #47819, #11581, #14853 ) ) ;
#11757=DIRECTION ( 'NONE',  ( -0.6427681459581293666, -0.7660444431189770143, -0.005002170337467561935 ) ) ;
#11758=EDGE_CURVE ( 'NONE', #10857, #20993, #5656, .T. ) ;
#11759=DIRECTION ( 'NONE',  ( 0.000000000000000000, -1.000000000000000000, 0.000000000000000000 ) ) ;
#11760=FACE_OUTER_BOUND ( 'NONE', #53063, .T. ) ;
#11761=VERTEX_POINT ( 'NONE', #48836 ) ;
#11763=LINE ( 'NONE', #16578, #40427 ) ;
#11764=DIRECTION ( 'NONE',  ( -0.9999697198139514409, -0.000000000000000000, -0.007781995580013368816 ) ) ;
#11766=DIRECTION ( 'NONE',  ( -0.005002170337468016433, -0.7660444431189770143, 0.6427681459581293666 ) ) ;
#11767=ORIENTED_EDGE ( 'NONE', *, *, #36755, .T. ) ;
#11768=VERTEX_POINT ( 'NONE', #53915 ) ;
#11769=ORIENTED_EDGE ( 'NONE', *, *, #38711, .F. ) ;
#11770=VERTEX_POINT ( 'NONE', #1936 ) ;
#11771=CARTESIAN_POINT ( 'NONE',  ( -17.21835818046645628, 0.000000000000000000, 7.641066439286161582 ) ) ;
#11772=VERTEX_POINT ( 'NONE', #44842 ) ;
#11773=ORIENTED_EDGE ( 'NONE', *, *, #35962, .T. ) ;
#11774=DIRECTION ( 'NONE',  ( 0.9999697198139515519, 0.000000000000000000, 0.007781995580013368816 ) ) ;
#11775=ADVANCED_FACE ( 'NONE', ( #36072 ), #19566, .F. ) ;
#11776=VERTEX_POINT ( 'NONE', #5960 ) ;
#11778=DIRECTION ( 'NONE',  ( 0.9999697198139515519, 0.000000000000000000, 0.007781995580013368816 ) ) ;
#11779=DIRECTION ( 'NONE',  ( 0.9321478471874541372, 0.000000000000000000, -0.3620778797217453771 ) ) ;
#11780=DIRECTION ( 'NONE',  ( -0.5364919789714478471, 0.6444004775717705469, -0.5449076811759709926 ) ) ;
#11781=DIRECTION ( 'NONE',  ( -0.5364919789714478471, 0.6444004775717705469, -0.5449076811759709926 ) ) ;
#11782=PLANE ( 'NONE',  #20174 ) ;
#11783=ORIENTED_EDGE ( 'NONE', *, *, #33265, .F. ) ;
#11784=ADVANCED_FACE ( 'NONE', ( #18743 ), #41139, .F. ) ;
#11785=EDGE_LOOP ( 'NONE', ( #7881, #11797, #10697, #27531 ) ) ;
#11787=CARTESIAN_POINT ( 'NONE',  ( -16.72653714768854627, 0.000000000000000000, 4.151579262439313744 ) ) ;
#11788=EDGE_CURVE ( 'NONE', #13281, #22170, #32367, .T. ) ;
#11789=EDGE_CURVE ( 'NONE', #23263, #3650, #27521, .T. ) ;
#11790=DIRECTION ( 'NONE',  ( 0.9999697198139515519, 0.000000000000000000, 0.007781995580013368816 ) ) ;
#11791=CARTESIAN_POINT ( 'NONE',  ( -17.73140113748535285, 0.000000000000000000, 13.85752530597602039 ) ) ;
#11792=FACE_OUTER_BOUND ( 'NONE', #48879, .T. ) ;
#11793=CARTESIAN_POINT ( 'NONE',  ( -16.83811138606217739, 0.4483081953215036219, 4.157565528459807425 ) ) ;
#11794=ORIENTED_EDGE ( 'NONE', *, *, #5289, .F. ) ;
#11795=DIRECTION ( 'NONE',  ( -0.3620778797217457656, 0.000000000000000000, -0.9321478471874539151 ) ) ;
#11796=ADVANCED_FACE ( 'NONE', ( #54207 ), #36905, .F. ) ;
#11797=ORIENTED_EDGE ( 'NONE', *, *, #38784, .F. ) ;
#11798=LINE ( 'NONE', #1939, #21613 ) ;
#11799=FACE_OUTER_BOUND ( 'NONE', #45848, .T. ) ;
#11800=DIRECTION ( 'NONE',  ( 0.007781995580012663651, -3.146120232559066537E-19, -0.9999697198139514409 ) ) ;
#11801=EDGE_CURVE ( 'NONE', #32796, #31826, #23807, .T. ) ;
#11802=CARTESIAN_POINT ( 'NONE',  ( -3.789478469635834568, -7.588859415764141580, -1.746411446826717340 ) ) ;
#11803=CARTESIAN_POINT ( 'NONE',  ( -12.13851405436063047, 0.000000000000000000, 11.68505802764555135 ) ) ;
#11804=EDGE_CURVE ( 'NONE', #46401, #45947, #32615, .T. ) ;
#11805=LINE ( 'NONE', #28870, #35952 ) ;
#11806=AXIS2_PLACEMENT_3D ( 'NONE', #14676, #27761, #49618 ) ;
#11808=ORIENTED_EDGE ( 'NONE', *, *, #54700, .T. ) ;
#11809=DIRECTION ( 'NONE',  ( -0.005002170337468016433, -0.7660444431189770143, 0.6427681459581293666 ) ) ;
#11810=LINE ( 'NONE', #33135, #50354 ) ;
#11811=LINE ( 'NONE', #46746, #41498 ) ;
#11812=ADVANCED_FACE ( 'NONE', ( #10502 ), #28344, .F. ) ;
#11813=CARTESIAN_POINT ( 'NONE',  ( -10.00813838035478298, 0.000000000000000000, 10.77830692922518452 ) ) ;
#11814=CARTESIAN_POINT ( 'NONE',  ( -28.93137873341882127, 0.000000000000000000, 8.119251130998824451 ) ) ;
#11815=LINE ( 'NONE', #26033, #7406 ) ;
#11816=CARTESIAN_POINT ( 'NONE',  ( -14.33979583046189887, 3.524445264749008988, 8.235599918570057909 ) ) ;
#11817=ADVANCED_FACE ( 'NONE', ( #53631 ), #40013, .F. ) ;
#11818=CARTESIAN_POINT ( 'NONE',  ( -16.53317331066696383, 0.000000000000000000, 13.31285208727739899 ) ) ;
#11820=LINE ( 'NONE', #7034, #52806 ) ;
#11821=ORIENTED_EDGE ( 'NONE', *, *, #28999, .T. ) ;
#11822=PLANE ( 'NONE',  #34061 ) ;
#11823=EDGE_LOOP ( 'NONE', ( #14876, #24990, #19629, #39530 ) ) ;
#11824=EDGE_LOOP ( 'NONE', ( #55214, #45054, #13858, #45079 ) ) ;
#11825=ORIENTED_EDGE ( 'NONE', *, *, #17117, .T. ) ;
#11826=VERTEX_POINT ( 'NONE', #32069 ) ;
#11827=EDGE_LOOP ( 'NONE', ( #7233, #29383, #37162, #13745 ) ) ;
#11828=DIRECTION ( 'NONE',  ( -0.005002170337468016433, -0.7660444431189770143, 0.6427681459581293666 ) ) ;
#11829=LINE ( 'NONE', #38233, #47432 ) ;
#11830=CARTESIAN_POINT ( 'NONE',  ( -24.27063949748155380, 0.000000000000000000, 6.308861732390097288 ) ) ;
#11831=ORIENTED_EDGE ( 'NONE', *, *, #8568, .T. ) ;
#11832=CARTESIAN_POINT ( 'NONE',  ( -22.40634380310664397, 0.000000000000000000, 5.584705972946605534 ) ) ;
#11833=ADVANCED_FACE ( 'NONE', ( #18437 ), #35771, .F. ) ;
#11834=VERTEX_POINT ( 'NONE', #51042 ) ;
#11835=CARTESIAN_POINT ( 'NONE',  ( 2.072287782118878319, 0.000000000000000000, -2.950529333540147015 ) ) ;
#11836=VERTEX_POINT ( 'NONE', #7613 ) ;
#11837=VECTOR ( 'NONE', #32442, 1000.000000000000000 ) ;
#11839=DIRECTION ( 'NONE',  ( -0.005961354470445682716, -0.6427876096865404731, 0.7660212471507180654 ) ) ;
#11840=DIRECTION ( 'NONE',  ( 0.9999697198139515519, 0.000000000000000000, 0.007781995580013368816 ) ) ;
#11841=ORIENTED_EDGE ( 'NONE', *, *, #29944, .F. ) ;
#11842=DIRECTION ( 'NONE',  ( 0.9999697198139515519, 0.000000000000000000, 0.007781995580013368816 ) ) ;
#11843=EDGE_LOOP ( 'NONE', ( #8009, #30158, #38851 ) ) ;
#11844=CARTESIAN_POINT ( 'NONE',  ( -21.47263955680318404, 0.000000000000000000, 5.022634149262071190 ) ) ;
#11845=DIRECTION ( 'NONE',  ( 0.007781995580012663651, -3.146120232559066537E-19, -0.9999697198139514409 ) ) ;
#11846=EDGE_CURVE ( 'NONE', #20292, #55275, #37732, .T. ) ;
#11847=CARTESIAN_POINT ( 'NONE',  ( -12.05517860703720778, 1.419719901456504507, 1.319276000146733185 ) ) ;
#11848=CARTESIAN_POINT ( 'NONE',  ( -19.60990026154428278, 0.000000000000000000, 4.498472333781370125 ) ) ;
#11850=DIRECTION ( 'NONE',  ( 0.005961354470445682716, -0.6427876096865404731, -0.7660212471507180654 ) ) ;
#11851=CARTESIAN_POINT ( 'NONE',  ( -18.67697421479882181, -0.1191753592594197858, 4.036397482078229793 ) ) ;
#11852=CARTESIAN_POINT ( 'NONE',  ( -28.93137873341882127, 0.000000000000000000, 8.119251130998824451 ) ) ;
#11853=EDGE_LOOP ( 'NONE', ( #47170, #12003, #37517, #25099 ) ) ;
#11854=DIRECTION ( 'NONE',  ( -0.6427681459581293666, -0.7660444431189770143, -0.005002170337467561935 ) ) ;
#11855=ORIENTED_EDGE ( 'NONE', *, *, #52598, .F. ) ;
#11856=VECTOR ( 'NONE', #49880, 1000.000000000000227 ) ;
#11857=DIRECTION ( 'NONE',  ( 0.007781995580012662783, 0.000000000000000000, -0.9999697198139514409 ) ) ;
#11858=LINE ( 'NONE', #38564, #9696 ) ;
#11859=ADVANCED_FACE ( 'NONE', ( #55055 ), #16144, .F. ) ;
#11860=DIRECTION ( 'NONE',  ( -0.5449076811759708816, 0.6444004775717707689, 0.5364919789714475140 ) ) ;
#11861=CARTESIAN_POINT ( 'NONE',  ( -25.20200914511100265, -0.1191753592594197858, 6.570942640130446932 ) ) ;
#11862=LINE ( 'NONE', #47081, #16824 ) ;
#11863=EDGE_CURVE ( 'NONE', #54767, #24397, #15850, .T. ) ;
#11864=DIRECTION ( 'NONE',  ( 0.000000000000000000, -1.000000000000000000, 0.000000000000000000 ) ) ;
#11866=EDGE_LOOP ( 'NONE', ( #20002, #18329, #29030, #20905 ) ) ;
#11867=DIRECTION ( 'NONE',  ( 0.6246952433987894571, -0.7422098413412800966, -0.2426528472758541777 ) ) ;
#11868=CARTESIAN_POINT ( 'NONE',  ( -9.391748698554145847, 7.045229895792196828, 0.4297005639829583057 ) ) ;
#11869=LINE ( 'NONE', #12729, #6787 ) ;
#11870=DIRECTION ( 'NONE',  ( -0.5449076811759708816, 0.6444004775717707689, 0.5364919789714475140 ) ) ;
#11871=ADVANCED_FACE ( 'NONE', ( #7079 ), #28648, .F. ) ;
#11872=VECTOR ( 'NONE', #16192, 999.9999999999998863 ) ;
#11873=LINE ( 'NONE', #54468, #48179 ) ;
#11874=DIRECTION ( 'NONE',  ( -0.005961354470445682716, -0.6427876096865404731, 0.7660212471507180654 ) ) ;
#11875=FACE_OUTER_BOUND ( 'NONE', #40128, .T. ) ;
#11876=FACE_OUTER_BOUND ( 'NONE', #34332, .T. ) ;
#11877=ORIENTED_EDGE ( 'NONE', *, *, #26754, .F. ) ;
#11878=AXIS2_PLACEMENT_3D ( 'NONE', #18107, #26340, #30341 ) ;
#11879=EDGE_CURVE ( 'NONE', #8877, #2394, #41435, .T. ) ;
#11880=DIRECTION ( 'NONE',  ( 0.6246952433987893460, 0.7422098413412802076, -0.2426528472758539279 ) ) ;
#11881=DIRECTION ( 'NONE',  ( -0.005961354470445682716, -0.6427876096865404731, 0.7660212471507180654 ) ) ;
#11882=ORIENTED_EDGE ( 'NONE', *, *, #17125, .T. ) ;
#11883=ORIENTED_EDGE ( 'NONE', *, *, #8949, .F. ) ;
#11885=ORIENTED_EDGE ( 'NONE', *, *, #52086, .F. ) ;
#11886=ORIENTED_EDGE ( 'NONE', *, *, #44063, .T. ) ;
#11887=DIRECTION ( 'NONE',  ( -0.5449076811759708816, 0.6444004775717707689, 0.5364919789714475140 ) ) ;
#11888=ORIENTED_EDGE ( 'NONE', *, *, #54239, .T. ) ;
#11889=EDGE_LOOP ( 'NONE', ( #6368, #44574, #41343, #2950 ) ) ;
#11890=ORIENTED_EDGE ( 'NONE', *, *, #21220, .F. ) ;
#11891=CARTESIAN_POINT ( 'NONE',  ( -17.70179579745524023, 0.000000000000000000, 10.05330269102752716 ) ) ;
#11892=LINE ( 'NONE', #8211, #22403 ) ;
#11893=DIRECTION ( 'NONE',  ( 0.5364919789714477361, 0.6444004775717706579, 0.5449076811759711036 ) ) ;
#11894=EDGE_CURVE ( 'NONE', #29513, #18849, #2517, .T. ) ;
#11895=VECTOR ( 'NONE', #24652, 1000.000000000000227 ) ;
#11896=AXIS2_PLACEMENT_3D ( 'NONE', #25479, #42527, #9015 ) ;
#11897=EDGE_LOOP ( 'NONE', ( #11571, #36923, #30928, #53469 ) ) ;
#11898=ADVANCED_FACE ( 'NONE', ( #11606 ), #38005, .F. ) ;
#11899=VERTEX_POINT ( 'NONE', #15557 ) ;
#11900=ADVANCED_FACE ( 'NONE', ( #24943 ), #32888, .F. ) ;
#11901=CARTESIAN_POINT ( 'NONE',  ( -11.09739355201212163, -0.5179957512181557755, 1.175398865385032465 ) ) ;
#11902=FACE_OUTER_BOUND ( 'NONE', #53032, .T. ) ;
#11903=ORIENTED_EDGE ( 'NONE', *, *, #28371, .T. ) ;
#11904=ADVANCED_FACE ( 'NONE', ( #19837 ), #33725, .F. ) ;
#11905=DIRECTION ( 'NONE',  ( 0.9999697198139515519, 0.000000000000000000, 0.007781995580013368816 ) ) ;
#11906=ORIENTED_EDGE ( 'NONE', *, *, #29677, .T. ) ;
#11907=CARTESIAN_POINT ( 'NONE',  ( -11.20636620717317378, 0.000000000000000000, 11.32298014792380414 ) ) ;
#11909=EDGE_CURVE ( 'NONE', #4790, #18162, #37421, .T. ) ;
#11910=EDGE_CURVE ( 'NONE', #54304, #30596, #50207, .T. ) ;
#11911=EDGE_CURVE ( 'NONE', #19103, #7431, #20690, .T. ) ;
#11912=ORIENTED_EDGE ( 'NONE', *, *, #34594, .T. ) ;
#11913=DIRECTION ( 'NONE',  ( 0.005961354470445682716, -0.6427876096865404731, -0.7660212471507180654 ) ) ;
#11914=AXIS2_PLACEMENT_3D ( 'NONE', #1452, #23329, #5174 ) ;
#11915=PLANE ( 'NONE',  #12776 ) ;
#11916=ORIENTED_EDGE ( 'NONE', *, *, #6079, .T. ) ;
#11917=CARTESIAN_POINT ( 'NONE',  ( -21.31610270512911143, 5.143464774974011888, 13.60252126457413624 ) ) ;
#11918=PLANE ( 'NONE',  #7610 ) ;
#11919=DIRECTION ( 'NONE',  ( -0.9999697198139514409, -0.000000000000000000, -0.007781995580013368816 ) ) ;
#11920=EDGE_LOOP ( 'NONE', ( #4020, #51555, #11948, #41936 ) ) ;
#11921=FACE_OUTER_BOUND ( 'NONE', #16799, .T. ) ;
#11922=CARTESIAN_POINT ( 'NONE',  ( -3.184385661761863773, -6.114012816731704270, -1.981450042443219539 ) ) ;
#11923=CARTESIAN_POINT ( 'NONE',  ( -10.68182703613314644, 0.000000000000000000, 3.629282468202884804 ) ) ;
#11924=EDGE_CURVE ( 'NONE', #43321, #30466, #29486, .T. ) ;
#11925=DIRECTION ( 'NONE',  ( 0.5449076811759707706, 0.6444004775717708799, -0.5364919789714476250 ) ) ;
#11926=DIRECTION ( 'NONE',  ( -0.005002170337468016433, -0.7660444431189770143, 0.6427681459581293666 ) ) ;
#11927=PLANE ( 'NONE',  #22504 ) ;
#11928=EDGE_CURVE ( 'NONE', #5052, #33685, #7924, .T. ) ;
#11929=LINE ( 'NONE', #50278, #26739 ) ;
#11930=ORIENTED_EDGE ( 'NONE', *, *, #30971, .T. ) ;
#11931=PLANE ( 'NONE',  #47088 ) ;
#11932=EDGE_CURVE ( 'NONE', #15628, #23911, #3633, .T. ) ;
#11934=ORIENTED_EDGE ( 'NONE', *, *, #50033, .F. ) ;
#11935=FACE_OUTER_BOUND ( 'NONE', #13631, .T. ) ;
#11936=DIRECTION ( 'NONE',  ( 0.000000000000000000, -1.000000000000000000, 0.000000000000000000 ) ) ;
#11937=VECTOR ( 'NONE', #41311, 1000.000000000000000 ) ;
#11938=EDGE_CURVE ( 'NONE', #51942, #3988, #3061, .T. ) ;
#11939=AXIS2_PLACEMENT_3D ( 'NONE', #32201, #14591, #6104 ) ;
#11940=DIRECTION ( 'NONE',  ( -0.7660212471507179544, -0.6427876096865405842, -0.005961354470445141482 ) ) ;
#11941=CARTESIAN_POINT ( 'NONE',  ( -11.23861694399777633, -0.1191753592594189115, 2.616956219084973334 ) ) ;
#11942=LINE ( 'NONE', #17073, #55590 ) ;
#11943=ORIENTED_EDGE ( 'NONE', *, *, #51679, .F. ) ;
#11944=AXIS2_PLACEMENT_3D ( 'NONE', #19402, #14879, #36743 ) ;
#11945=ORIENTED_EDGE ( 'NONE', *, *, #24663, .F. ) ;
#11946=CARTESIAN_POINT ( 'NONE',  ( -10.74029228357944987, 0.000000000000000000, 11.14194120806293320 ) ) ;
#11947=PLANE ( 'NONE',  #4849 ) ;
#11948=ORIENTED_EDGE ( 'NONE', *, *, #48040, .T. ) ;
#11949=LINE ( 'NONE', #3161, #39498 ) ;
#11950=VECTOR ( 'NONE', #21781, 1000.000000000000114 ) ;
#11951=ORIENTED_EDGE ( 'NONE', *, *, #41587, .T. ) ;
#11952=PLANE ( 'NONE',  #37429 ) ;
#11953=VECTOR ( 'NONE', #45118, 1000.000000000000227 ) ;
#11954=EDGE_LOOP ( 'NONE', ( #17493, #14990, #9405, #26622 ) ) ;
#11955=ORIENTED_EDGE ( 'NONE', *, *, #24551, .T. ) ;
#11956=ORIENTED_EDGE ( 'NONE', *, *, #32420, .T. ) ;
#11957=CARTESIAN_POINT ( 'NONE',  ( -9.342070512798265725, 0.000000000000000000, 10.59882438848031505 ) ) ;
#11958=CARTESIAN_POINT ( 'NONE',  ( 2.072287782118878319, 0.000000000000000000, -2.950529333540147015 ) ) ;
#11959=LINE ( 'NONE', #51153, #18512 ) ;
#11960=LINE ( 'NONE', #29608, #30306 ) ;
#11961=EDGE_LOOP ( 'NONE', ( #48692, #16461, #27139, #42486 ) ) ;
#11962=EDGE_LOOP ( 'NONE', ( #6899, #12890, #36401, #46262 ) ) ;
#11963=EDGE_LOOP ( 'NONE', ( #17016, #38725, #51683, #36362 ) ) ;
#11964=DIRECTION ( 'NONE',  ( -0.7660212471507179544, -0.6427876096865405842, -0.005961354470445141482 ) ) ;
#11966=ORIENTED_EDGE ( 'NONE', *, *, #34585, .F. ) ;
#11967=VECTOR ( 'NONE', #8946, 1000.000000000000227 ) ;
#11968=CARTESIAN_POINT ( 'NONE',  ( -17.57195112297145556, 2.945294577023091609, 12.40488687576302773 ) ) ;
#11969=ORIENTED_EDGE ( 'NONE', *, *, #36689, .F. ) ;
#11970=DIRECTION ( 'NONE',  ( -0.7660212471507179544, -0.6427876096865405842, -0.005961354470445141482 ) ) ;
#11971=DIRECTION ( 'NONE',  ( 0.007781995580012662783, 0.000000000000000000, -0.9999697198139514409 ) ) ;
#11972=EDGE_CURVE ( 'NONE', #11534, #5052, #16699, .T. ) ;
#11973=EDGE_CURVE ( 'NONE', #29528, #38022, #49675, .T. ) ;
#11974=AXIS2_PLACEMENT_3D ( 'NONE', #38147, #13167, #38741 ) ;
#11975=VECTOR ( 'NONE', #48236, 1000.000000000000000 ) ;
#11976=ORIENTED_EDGE ( 'NONE', *, *, #45559, .T. ) ;
#11977=LINE ( 'NONE', #28469, #21353 ) ;
#11978=ORIENTED_EDGE ( 'NONE', *, *, #7537, .T. ) ;
#11979=EDGE_CURVE ( 'NONE', #44660, #46056, #54205, .T. ) ;
#11980=VECTOR ( 'NONE', #9246, 1000.000000000000000 ) ;
#11981=CARTESIAN_POINT ( 'NONE',  ( -16.65852666505410795, 1.905425754524007642, 3.091876156576410128 ) ) ;
#11983=VECTOR ( 'NONE', #16843, 1000.000000000000227 ) ;
#11984=VERTEX_POINT ( 'NONE', #15556 ) ;
#11985=DIRECTION ( 'NONE',  ( 0.000000000000000000, -1.000000000000000000, 0.000000000000000000 ) ) ;
#11986=CARTESIAN_POINT ( 'NONE',  ( -17.41292333033276307, 3.848249166794008413, 9.960724371270012867 ) ) ;
#11987=PLANE ( 'NONE',  #2388 ) ;
#11989=ORIENTED_EDGE ( 'NONE', *, *, #42422, .F. ) ;
#11990=ORIENTED_EDGE ( 'NONE', *, *, #53589, .F. ) ;
#11991=DIRECTION ( 'NONE',  ( 0.9999697198139515519, 0.000000000000000000, 0.007781995580013368816 ) ) ;
#11992=CARTESIAN_POINT ( 'NONE',  ( -11.33364400852660658, 0.000000000000000000, 1.977555584992839455 ) ) ;
#11993=VECTOR ( 'NONE', #54966, 999.9999999999998863 ) ;
#11995=DIRECTION ( 'NONE',  ( 0.9999697198139515519, 0.000000000000000000, 0.007781995580013368816 ) ) ;
#11996=DIRECTION ( 'NONE',  ( 0.007781995580012663651, 0.000000000000000000, -0.9999697198139515519 ) ) ;
#11997=ADVANCED_FACE ( 'NONE', ( #19265 ), #32067, .F. ) ;
#11998=DIRECTION ( 'NONE',  ( -0.5449076811759708816, 0.6444004775717707689, 0.5364919789714475140 ) ) ;
#11999=EDGE_LOOP ( 'NONE', ( #36793, #295, #47154, #11351 ) ) ;
#12000=DIRECTION ( 'NONE',  ( -0.7660212471507179544, -0.6427876096865405842, -0.005961354470445141482 ) ) ;
#12001=EDGE_CURVE ( 'NONE', #2953, #50886, #28343, .T. ) ;
#12002=DIRECTION ( 'NONE',  ( 0.5364919789714477361, 0.6444004775717706579, 0.5449076811759711036 ) ) ;
#12003=ORIENTED_EDGE ( 'NONE', *, *, #12741, .T. ) ;
#12004=DIRECTION ( 'NONE',  ( 0.6427681459581294776, -0.7660444431189769032, 0.005002170337467562802 ) ) ;
#12005=VERTEX_POINT ( 'NONE', #2515 ) ;
#12006=FACE_OUTER_BOUND ( 'NONE', #44665, .T. ) ;
#12007=DIRECTION ( 'NONE',  ( 0.007781995580012663651, 0.000000000000000000, -0.9999697198139515519 ) ) ;
#12008=ADVANCED_FACE ( 'NONE', ( #18741 ), #14469, .F. ) ;
#12009=PLANE ( 'NONE',  #45884 ) ;
#12010=AXIS2_PLACEMENT_3D ( 'NONE', #36912, #37163, #14221 ) ;
#12011=DIRECTION ( 'NONE',  ( 0.9999697198139515519, 0.000000000000000000, 0.007781995580013368816 ) ) ;
#12013=ORIENTED_EDGE ( 'NONE', *, *, #20693, .F. ) ;
#12014=ORIENTED_EDGE ( 'NONE', *, *, #45332, .T. ) ;
#12017=AXIS2_PLACEMENT_3D ( 'NONE', #31945, #27702, #6137 ) ;
#12019=EDGE_CURVE ( 'NONE', #54483, #3178, #19564, .T. ) ;
#12020=VECTOR ( 'NONE', #16418, 999.9999999999998863 ) ;
#12021=CARTESIAN_POINT ( 'NONE',  ( -9.500962902709808588, 0.000000000000000000, 5.315806561384757600 ) ) ;
#12022=VECTOR ( 'NONE', #6714, 1000.000000000000227 ) ;
#12023=DIRECTION ( 'NONE',  ( 0.005961354470445682716, -0.6427876096865404731, -0.7660212471507180654 ) ) ;
#12024=CARTESIAN_POINT ( 'NONE',  ( 2.072287782118878319, 0.000000000000000000, -2.950529333540147015 ) ) ;
#12025=ORIENTED_EDGE ( 'NONE', *, *, #8084, .T. ) ;
#12026=DIRECTION ( 'NONE',  ( 0.000000000000000000, -1.000000000000000000, 0.000000000000000000 ) ) ;
#12027=DIRECTION ( 'NONE',  ( -0.9999697198139514409, -0.000000000000000000, -0.007781995580013368816 ) ) ;
#12028=AXIS2_PLACEMENT_3D ( 'NONE', #27924, #35579, #14311 ) ;
#12029=CARTESIAN_POINT ( 'NONE',  ( -18.72166620304495410, -0.1191753592594162470, 8.837366586178813321 ) ) ;
#12030=VECTOR ( 'NONE', #16697, 1000.000000000000227 ) ;
#12031=ORIENTED_EDGE ( 'NONE', *, *, #13023, .T. ) ;
#12032=LINE ( 'NONE', #50671, #6605 ) ;
#12033=CARTESIAN_POINT ( 'NONE',  ( -8.351072905600126717, 0.000000000000000000, 5.494081284814476440 ) ) ;
#12034=PLANE ( 'NONE',  #31163 ) ;
#12036=DIRECTION ( 'NONE',  ( 0.005961354470445682716, -0.6427876096865404731, -0.7660212471507180654 ) ) ;
#12037=VECTOR ( 'NONE', #14198, 1000.000000000000114 ) ;
#12038=EDGE_LOOP ( 'NONE', ( #21513, #54935, #7587, #49279 ) ) ;
#12039=VECTOR ( 'NONE', #2611, 1000.000000000000227 ) ;
#12040=ORIENTED_EDGE ( 'NONE', *, *, #55092, .F. ) ;
#12041=ORIENTED_EDGE ( 'NONE', *, *, #50497, .F. ) ;
#12042=ORIENTED_EDGE ( 'NONE', *, *, #18230, .F. ) ;
#12043=CARTESIAN_POINT ( 'NONE',  ( -12.56624110504503022, 0.000000000000000000, 6.938606150450726595 ) ) ;
#12044=VERTEX_POINT ( 'NONE', #53374 ) ;
#12045=VECTOR ( 'NONE', #19181, 1000.000000000000227 ) ;
#12046=LINE ( 'NONE', #51787, #47623 ) ;
#12047=EDGE_CURVE ( 'NONE', #31757, #54495, #19836, .T. ) ;
#12048=ORIENTED_EDGE ( 'NONE', *, *, #29606, .T. ) ;
#12049=DIRECTION ( 'NONE',  ( 0.5364919789714477361, 0.6444004775717706579, 0.5449076811759711036 ) ) ;
#12050=ORIENTED_EDGE ( 'NONE', *, *, #49637, .F. ) ;
#12051=AXIS2_PLACEMENT_3D ( 'NONE', #51690, #25035, #8253 ) ;
#12052=VERTEX_POINT ( 'NONE', #15303 ) ;
#12053=EDGE_CURVE ( 'NONE', #42246, #35922, #28647, .T. ) ;
#12054=EDGE_CURVE ( 'NONE', #41830, #39497, #11022, .T. ) ;
#12056=DIRECTION ( 'NONE',  ( -0.7660212471507179544, -0.6427876096865405842, -0.005961354470445141482 ) ) ;
#12057=DIRECTION ( 'NONE',  ( 0.7660212471507180654, -0.6427876096865404731, 0.005961354470445141482 ) ) ;
#12059=VECTOR ( 'NONE', #44949, 1000.000000000000227 ) ;
#12060=CARTESIAN_POINT ( 'NONE',  ( -9.935302865382064752, 0.000000000000000000, 1.419099673076315016 ) ) ;
#12061=EDGE_LOOP ( 'NONE', ( #50807, #2614, #21953, #43063 ) ) ;
#12062=VECTOR ( 'NONE', #48424, 999.9999999999998863 ) ;
#12063=VECTOR ( 'NONE', #8381, 999.9999999999998863 ) ;
#12064=VERTEX_POINT ( 'NONE', #15030 ) ;
#12065=CARTESIAN_POINT ( 'NONE',  ( -8.409922665610809034, 0.000000000000000000, 10.23674650875856962 ) ) ;
#12066=LINE ( 'NONE', #54660, #40273 ) ;
#12067=DIRECTION ( 'NONE',  ( 0.007781995580012662783, 0.000000000000000000, -0.9999697198139514409 ) ) ;
#12068=VECTOR ( 'NONE', #44879, 1000.000000000000227 ) ;
#12069=VECTOR ( 'NONE', #16477, 1000.000000000000227 ) ;
#12070=CARTESIAN_POINT ( 'NONE',  ( -17.46532115785441519, 0.000000000000000000, 13.67492996699914265 ) ) ;
#12071=DIRECTION ( 'NONE',  ( 0.005961354470445682716, -0.6427876096865404731, -0.7660212471507180654 ) ) ;
#12072=CARTESIAN_POINT ( 'NONE',  ( -14.12721349658369085, 0.000000000000000000, 2.694479520900311620 ) ) ;
#12073=ORIENTED_EDGE ( 'NONE', *, *, #43420, .T. ) ;
#12074=DIRECTION ( 'NONE',  ( 0.5449076811759707706, 0.6444004775717708799, -0.5364919789714476250 ) ) ;
#12075=CARTESIAN_POINT ( 'NONE',  ( -17.19780905594623732, -1.651309408375658538, 6.072224872292091291 ) ) ;
#12076=ORIENTED_EDGE ( 'NONE', *, *, #46266, .T. ) ;
#12077=FACE_OUTER_BOUND ( 'NONE', #38151, .T. ) ;
#12078=LINE ( 'NONE', #50137, #17846 ) ;
#12079=DIRECTION ( 'NONE',  ( 0.9999697198139515519, 0.000000000000000000, 0.007781995580013368816 ) ) ;
#12080=CARTESIAN_POINT ( 'NONE',  ( -20.54204810873173415, 0.000000000000000000, 4.860550213503115558 ) ) ;
#12081=VECTOR ( 'NONE', #29754, 1000.000000000000000 ) ;
#12082=EDGE_CURVE ( 'NONE', #16969, #5084, #45666, .T. ) ;
#12083=DIRECTION ( 'NONE',  ( 0.7660212471507180654, -0.6427876096865404731, 0.005961354470445141482 ) ) ;
#12084=ORIENTED_EDGE ( 'NONE', *, *, #55919, .F. ) ;
#12085=ADVANCED_FACE ( 'NONE', ( #2222 ), #32365, .F. ) ;
#12086=EDGE_LOOP ( 'NONE', ( #50003, #37908, #27018, #6304 ) ) ;
#12087=LINE ( 'NONE', #17470, #52986 ) ;
#12088=CARTESIAN_POINT ( 'NONE',  ( -13.53673582514181106, 0.000000000000000000, 12.22817484722816772 ) ) ;
#12089=DIRECTION ( 'NONE',  ( -0.005961354470445682716, -0.6427876096865404731, 0.7660212471507180654 ) ) ;
#12090=EDGE_CURVE ( 'NONE', #16969, #42927, #28078, .T. ) ;
#12091=AXIS2_PLACEMENT_3D ( 'NONE', #27356, #10044, #14333 ) ;
#12092=DIRECTION ( 'NONE',  ( 0.007781995580012662783, 0.000000000000000000, -0.9999697198139514409 ) ) ;
#12093=EDGE_CURVE ( 'NONE', #41034, #1167, #49381, .T. ) ;
#12094=DIRECTION ( 'NONE',  ( -0.005961354470445682716, -0.6427876096865404731, 0.7660212471507180654 ) ) ;
#12095=AXIS2_PLACEMENT_3D ( 'NONE', #40938, #48919, #10600 ) ;
#12096=DIRECTION ( 'NONE',  ( -0.9999697198139514409, -0.000000000000000000, -0.007781995580013368816 ) ) ;
#12097=FACE_OUTER_BOUND ( 'NONE', #17370, .T. ) ;
#12098=CARTESIAN_POINT ( 'NONE',  ( -21.52029464965303518, 3.200641362704007786, 10.49333214280930093 ) ) ;
#12099=FACE_OUTER_BOUND ( 'NONE', #2616, .T. ) ;
#12100=AXIS2_PLACEMENT_3D ( 'NONE', #6674, #45555, #36790 ) ;
#12101=LINE ( 'NONE', #3324, #21964 ) ;
#12102=ORIENTED_EDGE ( 'NONE', *, *, #48544, .F. ) ;
#12105=AXIS2_PLACEMENT_3D ( 'NONE', #18679, #10442, #9882 ) ;
#12106=EDGE_LOOP ( 'NONE', ( #21816, #43293, #33467, #30516 ) ) ;
#12107=ORIENTED_EDGE ( 'NONE', *, *, #5673, .F. ) ;
#12108=ADVANCED_FACE ( 'NONE', ( #53629 ), #5653, .F. ) ;
#12109=AXIS2_PLACEMENT_3D ( 'NONE', #30346, #11874, #25246 ) ;
#12110=EDGE_LOOP ( 'NONE', ( #54085, #878, #4937, #38221 ) ) ;
#12111=ORIENTED_EDGE ( 'NONE', *, *, #18771, .T. ) ;
#12112=AXIS2_PLACEMENT_3D ( 'NONE', #19275, #36614, #53923 ) ;
#12113=VERTEX_POINT ( 'NONE', #41137 ) ;
#12114=ORIENTED_EDGE ( 'NONE', *, *, #4685, .T. ) ;
#12115=LINE ( 'NONE', #42508, #38686 ) ;
#12116=CARTESIAN_POINT ( 'NONE',  ( -21.47263955680318404, 0.000000000000000000, 5.022634149262071190 ) ) ;
#12117=EDGE_CURVE ( 'NONE', #17901, #48104, #1394, .T. ) ;
#12118=DIRECTION ( 'NONE',  ( 0.9999697198139515519, 0.000000000000000000, 0.007781995580013368816 ) ) ;
#12119=ORIENTED_EDGE ( 'NONE', *, *, #41163, .T. ) ;
#12120=EDGE_CURVE ( 'NONE', #28372, #24636, #10196, .T. ) ;
#12121=LINE ( 'NONE', #20914, #15856 ) ;
#12122=EDGE_LOOP ( 'NONE', ( #32534, #421, #7692, #40158 ) ) ;
#12123=DIRECTION ( 'NONE',  ( 0.5449076811759707706, 0.6444004775717708799, -0.5364919789714476250 ) ) ;
#12124=ORIENTED_EDGE ( 'NONE', *, *, #51420, .T. ) ;
#12125=EDGE_CURVE ( 'NONE', #31757, #46955, #5958, .T. ) ;
#12127=AXIS2_PLACEMENT_3D ( 'NONE', #939, #14020, #31633 ) ;
#12128=DIRECTION ( 'NONE',  ( -0.005002170337468016433, -0.7660444431189770143, 0.6427681459581293666 ) ) ;
#12130=EDGE_LOOP ( 'NONE', ( #25970, #46764, #51985, #29232 ) ) ;
#12131=CARTESIAN_POINT ( 'NONE',  ( -11.00050607007353776, -1.489407457353157049, 3.399273247333383985 ) ) ;
#12132=VECTOR ( 'NONE', #9278, 999.9999999999998863 ) ;
#12133=ORIENTED_EDGE ( 'NONE', *, *, #37949, .T. ) ;
#12134=ADVANCED_FACE ( 'NONE', ( #29781 ), #46806, .F. ) ;
#12135=LINE ( 'NONE', #7907, #21915 ) ;
#12136=LINE ( 'NONE', #55573, #23890 ) ;
#12137=VECTOR ( 'NONE', #33717, 1000.000000000000227 ) ;
#12138=EDGE_CURVE ( 'NONE', #27027, #34052, #42264, .T. ) ;
#12139=DIRECTION ( 'NONE',  ( 0.6427681459581294776, -0.7660444431189769032, 0.005002170337467562802 ) ) ;
#12140=DIRECTION ( 'NONE',  ( 0.007781995580012663651, 0.000000000000000000, -0.9999697198139515519 ) ) ;
#12141=LINE ( 'NONE', #43100, #41071 ) ;
#12142=CARTESIAN_POINT ( 'NONE',  ( -18.67775241435682432, 0.000000000000000000, 4.136394454059623804 ) ) ;
#12143=DIRECTION ( 'NONE',  ( -0.9999697198139514409, -0.000000000000000000, -0.007781995580013368816 ) ) ;
#12144=VECTOR ( 'NONE', #15145, 1000.000000000000227 ) ;
#12145=LINE ( 'NONE', #43103, #7776 ) ;
#12146=ORIENTED_EDGE ( 'NONE', *, *, #13053, .T. ) ;
#12147=CARTESIAN_POINT ( 'NONE',  ( 2.072287782118878319, 0.000000000000000000, -2.950529333540147015 ) ) ;
#12148=ORIENTED_EDGE ( 'NONE', *, *, #36620, .T. ) ;
#12150=CARTESIAN_POINT ( 'NONE',  ( -18.70442188201326061, -0.1191753592594160388, 6.621508366632224529 ) ) ;
#12151=DIRECTION ( 'NONE',  ( -0.005961354470445682716, -0.6427876096865404731, 0.7660212471507180654 ) ) ;
#12152=DIRECTION ( 'NONE',  ( -0.6427681459581293666, -0.7660444431189770143, -0.005002170337467561935 ) ) ;
#12153=PLANE ( 'NONE',  #46808 ) ;
#12154=LINE ( 'NONE', #43394, #4145 ) ;
#12155=CIRCLE ( 'NONE', #15802, 6.999999999999999112 ) ;
#12157=VECTOR ( 'NONE', #49814, 999.9999999999998863 ) ;
#12159=ORIENTED_EDGE ( 'NONE', *, *, #32639, .F. ) ;
#12162=CARTESIAN_POINT ( 'NONE',  ( -22.40556560354864146, -0.1191753592594197858, 5.484709000965211523 ) ) ;
#12163=CARTESIAN_POINT ( 'NONE',  ( -32.65997012216863737, 0.000000000000000000, 9.567562649885804404 ) ) ;
#12164=DIRECTION ( 'NONE',  ( 0.9999697198139515519, 0.000000000000000000, 0.007781995580013368816 ) ) ;
#12165=EDGE_CURVE ( 'NONE', #48572, #29343, #37731, .T. ) ;
#12166=DIRECTION ( 'NONE',  ( 0.7660212471507180654, -0.6427876096865404731, 0.005961354470445141482 ) ) ;
#12167=CARTESIAN_POINT ( 'NONE',  ( -11.87243407472968926, 0.000000000000000000, 11.50246268866867361 ) ) ;
#12168=CARTESIAN_POINT ( 'NONE',  ( -32.47108885958310509, 0.000000000000000000, 15.83124721154520387 ) ) ;
#12169=ORIENTED_EDGE ( 'NONE', *, *, #2698, .T. ) ;
#12170=AXIS2_PLACEMENT_3D ( 'NONE', #31444, #18932, #19182 ) ;
#12171=CARTESIAN_POINT ( 'NONE',  ( -17.93139508144814442, 0.000000000000000000, 13.85596890686001537 ) ) ;
#12173=ORIENTED_EDGE ( 'NONE', *, *, #43466, .T. ) ;
#12174=VECTOR ( 'NONE', #34468, 999.9999999999998863 ) ;
#12175=EDGE_LOOP ( 'NONE', ( #54070, #24289, #3808, #47227 ) ) ;
#12176=CARTESIAN_POINT ( 'NONE',  ( -16.46764230182081334, 0.000000000000000000, 4.892258181606849554 ) ) ;
#12177=VECTOR ( 'NONE', #12916, 1000.000000000000114 ) ;
#12178=EDGE_CURVE ( 'NONE', #8704, #50967, #16996, .T. ) ;
#12179=VERTEX_POINT ( 'NONE', #25235 ) ;
#12180=FACE_OUTER_BOUND ( 'NONE', #54385, .T. ) ;
#12181=ADVANCED_FACE ( 'NONE', ( #7612 ), #11605, .F. ) ;
#12182=EDGE_CURVE ( 'NONE', #27886, #27953, #12720, .T. ) ;
#12183=ORIENTED_EDGE ( 'NONE', *, *, #6216, .T. ) ;
#12184=ORIENTED_EDGE ( 'NONE', *, *, #48013, .T. ) ;
#12185=ORIENTED_EDGE ( 'NONE', *, *, #53984, .T. ) ;
#12186=DIRECTION ( 'NONE',  ( -0.005961354470445682716, -0.6427876096865404731, 0.7660212471507180654 ) ) ;
#12187=AXIS2_PLACEMENT_3D ( 'NONE', #36354, #15336, #49423 ) ;
#12189=DIRECTION ( 'NONE',  ( -0.6427681459581293666, -0.7660444431189770143, -0.005002170337467561935 ) ) ;
#12190=VECTOR ( 'NONE', #2371, 1000.000000000000000 ) ;
#12191=ADVANCED_FACE ( 'NONE', ( #21233 ), #55054, .F. ) ;
#12192=ORIENTED_EDGE ( 'NONE', *, *, #55303, .T. ) ;
#12193=ORIENTED_EDGE ( 'NONE', *, *, #42887, .F. ) ;
#12194=EDGE_CURVE ( 'NONE', #53603, #32511, #33194, .T. ) ;
#12195=VECTOR ( 'NONE', #51768, 1000.000000000000114 ) ;
#12196=VECTOR ( 'NONE', #51762, 1000.000000000000227 ) ;
#12197=CARTESIAN_POINT ( 'NONE',  ( 2.072287782118878319, 0.000000000000000000, -2.950529333540147015 ) ) ;
#12198=DIRECTION ( 'NONE',  ( 0.000000000000000000, -1.000000000000000000, 0.000000000000000000 ) ) ;
#12199=VERTEX_POINT ( 'NONE', #3370 ) ;
#12200=LINE ( 'NONE', #47394, #51807 ) ;
#12201=LINE ( 'NONE', #51402, #33160 ) ;
#12202=VERTEX_POINT ( 'NONE', #20940 ) ;
#12203=CARTESIAN_POINT ( 'NONE',  ( -19.30682298318506085, 0.6102101463440048335, 5.382205634531532112 ) ) ;
#12204=PLANE ( 'NONE',  #43026 ) ;
#12205=EDGE_CURVE ( 'NONE', #11344, #39446, #3632, .T. ) ;
#12206=ORIENTED_EDGE ( 'NONE', *, *, #3269, .F. ) ;
#12207=PLANE ( 'NONE',  #21880 ) ;
#12208=VECTOR ( 'NONE', #19788, 1000.000000000000227 ) ;
#12209=EDGE_CURVE ( 'NONE', #56036, #695, #41954, .T. ) ;
#12210=DIRECTION ( 'NONE',  ( -0.6427681459581293666, -0.7660444431189770143, -0.005002170337467561935 ) ) ;
#12211=EDGE_LOOP ( 'NONE', ( #36866, #9539, #43610, #50816, #35988 ) ) ;
#12212=CARTESIAN_POINT ( 'NONE',  ( -11.79540685186240800, 0.000000000000000000, 1.604629969967065195 ) ) ;
#12213=CARTESIAN_POINT ( 'NONE',  ( -23.33849165029409889, 0.000000000000000000, 5.946783852668351855 ) ) ;
#12214=CARTESIAN_POINT ( 'NONE',  ( -13.37731649229117181, -4.889348428825665671, 1.921529324938835437 ) ) ;
#12215=VECTOR ( 'NONE', #19290, 1000.000000000000114 ) ;
#12216=LINE ( 'NONE', #49974, #30155 ) ;
#12217=ORIENTED_EDGE ( 'NONE', *, *, #29841, .T. ) ;
#12218=VECTOR ( 'NONE', #17116, 1000.000000000000227 ) ;
#12219=CARTESIAN_POINT ( 'NONE',  ( -19.60834386242827776, 0.000000000000000000, 4.298478389818581213 ) ) ;
#12221=VECTOR ( 'NONE', #6552, 1000.000000000000227 ) ;
#12222=FACE_OUTER_BOUND ( 'NONE', #28212, .T. ) ;
#12223=DIRECTION ( 'NONE',  ( 0.6427681459581294776, -0.7660444431189769032, 0.005002170337467562802 ) ) ;
#12224=DIRECTION ( 'NONE',  ( 0.9999697198139515519, 0.000000000000000000, 0.007781995580013368816 ) ) ;
#12225=VECTOR ( 'NONE', #36176, 1000.000000000000227 ) ;
#12227=AXIS2_PLACEMENT_3D ( 'NONE', #42342, #38066, #33269 ) ;
#12228=ORIENTED_EDGE ( 'NONE', *, *, #5869, .F. ) ;
#12229=DIRECTION ( 'NONE',  ( 0.6427681459581294776, -0.7660444431189769032, 0.005002170337467562802 ) ) ;
#12230=ORIENTED_EDGE ( 'NONE', *, *, #7507, .F. ) ;
#12231=VECTOR ( 'NONE', #55704, 999.9999999999998863 ) ;
#12234=VECTOR ( 'NONE', #53991, 1000.000000000000114 ) ;
#12235=FACE_OUTER_BOUND ( 'NONE', #13401, .T. ) ;
#12236=ADVANCED_FACE ( 'NONE', ( #51619 ), #50769, .F. ) ;
#12237=CARTESIAN_POINT ( 'NONE',  ( -31.72704407542318350, -0.1191753592594197858, 9.105487798182664960 ) ) ;
#12239=ORIENTED_EDGE ( 'NONE', *, *, #52216, .T. ) ;
#12240=VECTOR ( 'NONE', #14839, 1000.000000000000114 ) ;
#12241=VECTOR ( 'NONE', #12388, 999.9999999999998863 ) ;
#12242=EDGE_CURVE ( 'NONE', #54113, #37795, #24371, .T. ) ;
#12243=ORIENTED_EDGE ( 'NONE', *, *, #35806, .T. ) ;
#12244=DIRECTION ( 'NONE',  ( -0.005002170337468016433, -0.7660444431189770143, 0.6427681459581293666 ) ) ;
#12245=DIRECTION ( 'NONE',  ( -0.005002170337468016433, -0.7660444431189770143, 0.6427681459581293666 ) ) ;
#12246=ORIENTED_EDGE ( 'NONE', *, *, #38700, .F. ) ;
#12247=EDGE_CURVE ( 'NONE', #35835, #43081, #42800, .T. ) ;
#12248=EDGE_CURVE ( 'NONE', #24292, #1300, #41682, .T. ) ;
#12249=EDGE_CURVE ( 'NONE', #21318, #30294, #33723, .T. ) ;
#12250=LINE ( 'NONE', #7710, #43835 ) ;
#12251=VERTEX_POINT ( 'NONE', #28926 ) ;
#12252=CARTESIAN_POINT ( 'NONE',  ( -16.81190032086591302, 0.000000000000000000, 3.212244750653343583 ) ) ;
#12253=EDGE_LOOP ( 'NONE', ( #47893, #38887, #15228, #50105 ) ) ;
#12254=LINE ( 'NONE', #11692, #22043 ) ;
#12255=EDGE_CURVE ( 'NONE', #29153, #20285, #11858, .T. ) ;
#12256=VECTOR ( 'NONE', #12939, 999.9999999999998863 ) ;
#12257=EDGE_LOOP ( 'NONE', ( #17899, #25073, #11769, #23168 ) ) ;
#12258=ORIENTED_EDGE ( 'NONE', *, *, #31174, .F. ) ;
#12259=VERTEX_POINT ( 'NONE', #46216 ) ;
#12260=VECTOR ( 'NONE', #39677, 999.9999999999998863 ) ;
#12261=DIRECTION ( 'NONE',  ( 0.5449076811759707706, 0.6444004775717708799, -0.5364919789714476250 ) ) ;
#12262=DIRECTION ( 'NONE',  ( 0.007781995580012663651, 0.000000000000000000, -0.9999697198139515519 ) ) ;
#12264=LINE ( 'NONE', #25323, #22118 ) ;
#12265=PLANE ( 'NONE',  #4794 ) ;
#12266=EDGE_CURVE ( 'NONE', #39740, #28953, #7325, .T. ) ;
#12267=VECTOR ( 'NONE', #7196, 999.9999999999998863 ) ;
#12268=ORIENTED_EDGE ( 'NONE', *, *, #44272, .F. ) ;
#12269=EDGE_CURVE ( 'NONE', #56078, #14391, #5056, .T. ) ;
#12270=ORIENTED_EDGE ( 'NONE', *, *, #53050, .T. ) ;
#12271=ORIENTED_EDGE ( 'NONE', *, *, #31806, .T. ) ;
#12272=VECTOR ( 'NONE', #21368, 1000.000000000000114 ) ;
#12273=PLANE ( 'NONE',  #29520 ) ;
#12274=AXIS2_PLACEMENT_3D ( 'NONE', #24349, #16666, #37979 ) ;
#12275=LINE ( 'NONE', #29616, #14594 ) ;
#12276=EDGE_CURVE ( 'NONE', #31601, #26572, #39411, .T. ) ;
#12277=ORIENTED_EDGE ( 'NONE', *, *, #40844, .T. ) ;
#12278=VECTOR ( 'NONE', #1751, 1000.000000000000114 ) ;
#12279=DIRECTION ( 'NONE',  ( -0.5449076811759708816, 0.6444004775717707689, 0.5364919789714475140 ) ) ;
#12281=PLANE ( 'NONE',  #21476 ) ;
#12282=PLANE ( 'NONE',  #6789 ) ;
#12283=VECTOR ( 'NONE', #43648, 1000.000000000000114 ) ;
#12284=EDGE_CURVE ( 'NONE', #6407, #23847, #26921, .T. ) ;
#12285=ORIENTED_EDGE ( 'NONE', *, *, #19801, .T. ) ;
#12286=VECTOR ( 'NONE', #12968, 1000.000000000000000 ) ;
#12287=DIRECTION ( 'NONE',  ( -0.6427681459581293666, -0.7660444431189770143, -0.005002170337467561935 ) ) ;
#12288=ORIENTED_EDGE ( 'NONE', *, *, #50732, .F. ) ;
#12290=CARTESIAN_POINT ( 'NONE',  ( -18.81801092196306513, 0.000000000000000000, 8.367281711381659548 ) ) ;
#12291=VECTOR ( 'NONE', #19709, 1000.000000000000227 ) ;
#12292=LINE ( 'NONE', #25079, #51976 ) ;
#12293=VERTEX_POINT ( 'NONE', #502 ) ;
#12294=SHAPE_REPRESENTATION ( 'Integrated Nail File & Cleaner Flip-Out', ( #2610 ), #48882 ) ;
#12295=CARTESIAN_POINT ( 'NONE',  ( -12.15271748404464880, 0.000000000000000000, 1.601849296007406664 ) ) ;
#12296=DIRECTION ( 'NONE',  ( 0.7660212471507180654, -0.6427876096865404731, 0.005961354470445141482 ) ) ;
#12297=CARTESIAN_POINT ( 'NONE',  ( -20.27233569796318946, 2.876837460659008361, 4.464609191105296304 ) ) ;
#12298=DIRECTION ( 'NONE',  ( 0.5449076811759707706, 0.6444004775717708799, -0.5364919789714476250 ) ) ;
#12299=EDGE_LOOP ( 'NONE', ( #53970, #12505, #44953, #38103 ) ) ;
#12300=EDGE_LOOP ( 'NONE', ( #1302, #55084, #26289, #36249 ) ) ;
#12301=DIRECTION ( 'NONE',  ( 0.5364919789714477361, 0.6444004775717706579, 0.5449076811759711036 ) ) ;
#12302=DIRECTION ( 'NONE',  ( -0.6427681459581293666, -0.7660444431189770143, -0.005002170337467561935 ) ) ;
#12303=DIRECTION ( 'NONE',  ( 0.7660212471507180654, -0.6427876096865404731, 0.005961354470445141482 ) ) ;
#12304=DIRECTION ( 'NONE',  ( -0.005002170337468016433, -0.7660444431189770143, 0.6427681459581293666 ) ) ;
#12305=LINE ( 'NONE', #43261, #35199 ) ;
#12306=VECTOR ( 'NONE', #8001, 999.9999999999998863 ) ;
#12307=CARTESIAN_POINT ( 'NONE',  ( -10.94028622754223967, 0.000000000000000000, 11.14038480894692995 ) ) ;
#12308=EDGE_LOOP ( 'NONE', ( #37152, #48214, #52904, #45171 ) ) ;
#12309=VECTOR ( 'NONE', #13733, 999.9999999999998863 ) ;
#12310=CARTESIAN_POINT ( 'NONE',  ( -13.93296765963146733, 0.000000000000000000, 3.434655326531841357 ) ) ;
#12311=CARTESIAN_POINT ( 'NONE',  ( -17.66000264926527663, 0.000000000000000000, 4.682972901456035508 ) ) ;
#12312=ORIENTED_EDGE ( 'NONE', *, *, #20555, .F. ) ;
#12313=LINE ( 'NONE', #21087, #15028 ) ;
#12314=AXIS2_PLACEMENT_3D ( 'NONE', #25634, #42960, #4068 ) ;
#12315=VERTEX_POINT ( 'NONE', #43645 ) ;
#12316=EDGE_CURVE ( 'NONE', #33009, #28898, #21540, .T. ) ;
#12317=CARTESIAN_POINT ( 'NONE',  ( -18.86354292863559579, 0.000000000000000000, 14.21804678658176080 ) ) ;
#12318=LINE ( 'NONE', #20817, #53233 ) ;
#12319=VECTOR ( 'NONE', #26681, 999.9999999999998863 ) ;
#12320=ADVANCED_FACE ( 'NONE', ( #34870 ), #22384, .F. ) ;
#12321=LINE ( 'NONE', #7784, #15047 ) ;
#12322=FACE_OUTER_BOUND ( 'NONE', #18823, .T. ) ;
#12324=EDGE_LOOP ( 'NONE', ( #3342, #8932, #10374, #15342 ) ) ;
#12325=VECTOR ( 'NONE', #12839, 999.9999999999998863 ) ;
#12326=VECTOR ( 'NONE', #3255, 999.9999999999998863 ) ;
#12327=ORIENTED_EDGE ( 'NONE', *, *, #34822, .T. ) ;
#12329=DIRECTION ( 'NONE',  ( 0.6427681459581294776, -0.7660444431189769032, 0.005002170337467562802 ) ) ;
#12330=CARTESIAN_POINT ( 'NONE',  ( -14.20280369269832832, 0.000000000000000000, 12.40765738797303719 ) ) ;
#12331=ADVANCED_FACE ( 'NONE', ( #22644 ), #47648, .F. ) ;
#12332=AXIS2_PLACEMENT_3D ( 'NONE', #2650, #37292, #54601 ) ;
#12333=ADVANCED_FACE ( 'NONE', ( #30327 ), #5335, .F. ) ;
#12334=ADVANCED_FACE ( 'NONE', ( #26085 ), #1040, .F. ) ;
#12335=LINE ( 'NONE', #7795, #42366 ) ;
#12336=VECTOR ( 'NONE', #46474, 1000.000000000000227 ) ;
#12337=CARTESIAN_POINT ( 'NONE',  ( -30.79489622823572859, -0.1191753592594197858, 8.743409918460921304 ) ) ;
#12338=DIRECTION ( 'NONE',  ( -0.005961354470445682716, -0.6427876096865404731, 0.7660212471507180654 ) ) ;
#12339=VECTOR ( 'NONE', #22097, 1000.000000000000000 ) ;
#12340=ORIENTED_EDGE ( 'NONE', *, *, #42529, .F. ) ;
#12342=DIRECTION ( 'NONE',  ( 0.000000000000000000, -0.000000000000000000, -1.000000000000000000 ) ) ;
#12343=VECTOR ( 'NONE', #30213, 999.9999999999998863 ) ;
#12344=CARTESIAN_POINT ( 'NONE',  ( -20.54126990917373519, -0.1191753592594197858, 4.760553241521720658 ) ) ;
#12345=AXIS2_PLACEMENT_3D ( 'NONE', #54523, #49739, #2838 ) ;
#12346=LINE ( 'NONE', #17151, #38755 ) ;
#12347=EDGE_LOOP ( 'NONE', ( #41857, #23866, #30000, #16819 ) ) ;
#12349=CARTESIAN_POINT ( 'NONE',  ( -12.80458192191714595, 0.000000000000000000, 11.86454056839041726 ) ) ;
#12350=DIRECTION ( 'NONE',  ( 0.007781995580012663651, -3.146120232559066537E-19, -0.9999697198139514409 ) ) ;
#12351=ORIENTED_EDGE ( 'NONE', *, *, #26354, .F. ) ;
#12352=CARTESIAN_POINT ( 'NONE',  ( -18.67619601524082285, 0.000000000000000000, 3.936400510096834893 ) ) ;
#12353=ORIENTED_EDGE ( 'NONE', *, *, #23718, .T. ) ;
#12354=ADVANCED_FACE ( 'NONE', ( #17839 ), #35171, .F. ) ;
#12355=VECTOR ( 'NONE', #45687, 1000.000000000000227 ) ;
#12356=ORIENTED_EDGE ( 'NONE', *, *, #47474, .T. ) ;
#12357=ORIENTED_EDGE ( 'NONE', *, *, #8340, .F. ) ;
#12358=ADVANCED_FACE ( 'NONE', ( #190 ), #52465, .F. ) ;
#12359=VERTEX_POINT ( 'NONE', #48182 ) ;
#12360=DIRECTION ( 'NONE',  ( -0.005961354470445682716, -0.6427876096865404731, 0.7660212471507180654 ) ) ;
#12361=AXIS2_PLACEMENT_3D ( 'NONE', #19412, #37285, #49802 ) ;
#12362=ORIENTED_EDGE ( 'NONE', *, *, #23846, .F. ) ;
#12364=EDGE_CURVE ( 'NONE', #17653, #45526, #25784, .T. ) ;
#12365=ORIENTED_EDGE ( 'NONE', *, *, #22339, .T. ) ;
#12366=CARTESIAN_POINT ( 'NONE',  ( -19.12962290826653700, 0.000000000000000000, 14.40064212555863854 ) ) ;
#12367=ORIENTED_EDGE ( 'NONE', *, *, #12266, .T. ) ;
#12368=VECTOR ( 'NONE', #19568, 1000.000000000000227 ) ;
#12370=EDGE_CURVE ( 'NONE', #20361, #45048, #38853, .T. ) ;
#12371=AXIS2_PLACEMENT_3D ( 'NONE', #25855, #39757, #47984 ) ;
#12372=VECTOR ( 'NONE', #41801, 1000.000000000000227 ) ;
#12373=DIRECTION ( 'NONE',  ( 0.9999697198139515519, 0.000000000000000000, 0.007781995580013368816 ) ) ;
#12374=DIRECTION ( 'NONE',  ( -0.9999697198139514409, -0.000000000000000000, -0.007781995580013368816 ) ) ;
#12375=LINE ( 'NONE', #43318, #23152 ) ;
#12376=DIRECTION ( 'NONE',  ( 0.000000000000000000, -0.000000000000000000, -1.000000000000000000 ) ) ;
#12378=VERTEX_POINT ( 'NONE', #43932 ) ;
#12379=VECTOR ( 'NONE', #33100, 999.9999999999998863 ) ;
#12380=ORIENTED_EDGE ( 'NONE', *, *, #1843, .T. ) ;
#12381=AXIS2_PLACEMENT_3D ( 'NONE', #19694, #2362, #6923 ) ;
#12382=DIRECTION ( 'NONE',  ( -0.6427681459581293666, -0.7660444431189770143, -0.005002170337467561935 ) ) ;
#12383=PLANE ( 'NONE',  #53881 ) ;
#12385=CARTESIAN_POINT ( 'NONE',  ( -18.66354898467281132, 0.000000000000000000, 14.21960318569776582 ) ) ;
#12386=VECTOR ( 'NONE', #54082, 1000.000000000000114 ) ;
#12387=DIRECTION ( 'NONE',  ( 0.007781995580012663651, 0.000000000000000000, -0.9999697198139515519 ) ) ;
#12388=DIRECTION ( 'NONE',  ( 0.5364919789714477361, 0.6444004775717706579, 0.5449076811759711036 ) ) ;
#12389=DIRECTION ( 'NONE',  ( 0.9999697198139515519, 0.000000000000000000, 0.007781995580013368816 ) ) ;
#12390=ORIENTED_EDGE ( 'NONE', *, *, #24149, .F. ) ;
#12391=CARTESIAN_POINT ( 'NONE',  ( -21.47419595591918906, 0.000000000000000000, 5.222628093224860102 ) ) ;
#12392=PLANE ( 'NONE',  #53047 ) ;
#12393=EDGE_LOOP ( 'NONE', ( #47804, #13207, #4412, #8143 ) ) ;
#12394=CARTESIAN_POINT ( 'NONE',  ( -17.36532418587302473, -0.1191753592594177458, 13.67570816655714516 ) ) ;
#12395=DIRECTION ( 'NONE',  ( 0.000000000000000000, -0.000000000000000000, -1.000000000000000000 ) ) ;
#12396=DIRECTION ( 'NONE',  ( 0.5364919789714477361, 0.6444004775717706579, 0.5449076811759711036 ) ) ;
#12397=DIRECTION ( 'NONE',  ( 0.007781995580012663651, -3.146120232559066537E-19, -0.9999697198139514409 ) ) ;
#12398=PLANE ( 'NONE',  #37707 ) ;
#12399=VECTOR ( 'NONE', #20744, 1000.000000000000227 ) ;
#12400=ORIENTED_EDGE ( 'NONE', *, *, #3666, .F. ) ;
#12401=ORIENTED_EDGE ( 'NONE', *, *, #1583, .T. ) ;
#12402=CARTESIAN_POINT ( 'NONE',  ( -18.79082678602624057, 0.000000000000000000, 4.874178622766801361 ) ) ;
#12403=DIRECTION ( 'NONE',  ( -0.7660212471507179544, -0.6427876096865405842, -0.005961354470445141482 ) ) ;
#12404=DIRECTION ( 'NONE',  ( -0.5449076811759708816, 0.6444004775717707689, 0.5364919789714475140 ) ) ;
#12405=AXIS2_PLACEMENT_3D ( 'NONE', #44084, #9998, #31001 ) ;
#12406=ADVANCED_FACE ( 'NONE', ( #39700 ), #52724, .F. ) ;
#12408=VECTOR ( 'NONE', #41842, 1000.000000000000227 ) ;
#12409=DIRECTION ( 'NONE',  ( 0.005002170337468016433, -0.7660444431189770143, -0.6427681459581293666 ) ) ;
#12410=EDGE_CURVE ( 'NONE', #49806, #22744, #17249, .T. ) ;
#12411=PLANE ( 'NONE',  #51837 ) ;
#12412=EDGE_CURVE ( 'NONE', #21743, #52239, #2157, .T. ) ;
#12413=PLANE ( 'NONE',  #21103 ) ;
#12414=CARTESIAN_POINT ( 'NONE',  ( -8.898634305293546376, -0.08571482049900724931, 4.084417208347257855 ) ) ;
#12415=AXIS2_PLACEMENT_3D ( 'NONE', #13829, #39954, #31155 ) ;
#12416=CARTESIAN_POINT ( 'NONE',  ( -30.79567442779373110, 0.000000000000000000, 8.843406890442315316 ) ) ;
#12417=FACE_OUTER_BOUND ( 'NONE', #24610, .T. ) ;
#12418=ORIENTED_EDGE ( 'NONE', *, *, #47573, .T. ) ;
#12419=DIRECTION ( 'NONE',  ( 0.007781995580012663651, 0.000000000000000000, -0.9999697198139515519 ) ) ;
#12420=ORIENTED_EDGE ( 'NONE', *, *, #30848, .T. ) ;
#12421=VECTOR ( 'NONE', #1316, 999.9999999999998863 ) ;
#12422=EDGE_LOOP ( 'NONE', ( #49865, #19031, #49649, #38823 ) ) ;
#12423=VECTOR ( 'NONE', #47688, 1000.000000000000227 ) ;
#12424=ORIENTED_EDGE ( 'NONE', *, *, #47031, .F. ) ;
#12425=AXIS2_PLACEMENT_3D ( 'NONE', #44858, #13910, #40031 ) ;
#12426=ORIENTED_EDGE ( 'NONE', *, *, #28155, .F. ) ;
#12428=ORIENTED_EDGE ( 'NONE', *, *, #16396, .T. ) ;
#12429=CARTESIAN_POINT ( 'NONE',  ( -20.29244006095147412, 0.000000000000000000, 5.401150804439980746 ) ) ;
#12430=PLANE ( 'NONE',  #3894 ) ;
#12431=CARTESIAN_POINT ( 'NONE',  ( -12.33850799832341849, 0.000000000000000000, 11.68350162852954632 ) ) ;
#12432=VERTEX_POINT ( 'NONE', #1627 ) ;
#12433=CARTESIAN_POINT ( 'NONE',  ( -0.08953432831225546784, -3.865803998196977176, 3.253151749378868640 ) ) ;
#12434=ORIENTED_EDGE ( 'NONE', *, *, #21921, .T. ) ;
#12435=CARTESIAN_POINT ( 'NONE',  ( -19.03250079184375210, -4.889348428825662118, 12.09905512791755555 ) ) ;
#12437=EDGE_CURVE ( 'NONE', #12832, #15388, #44486, .T. ) ;
#12438=VECTOR ( 'NONE', #33565, 1000.000000000000000 ) ;
#12439=PLANE ( 'NONE',  #34719 ) ;
#12440=EDGE_CURVE ( 'NONE', #32724, #43237, #19494, .T. ) ;
#12441=DIRECTION ( 'NONE',  ( 0.007781995580012663651, -3.146120232559066537E-19, -0.9999697198139514409 ) ) ;
#12443=EDGE_CURVE ( 'NONE', #30915, #26710, #45081, .T. ) ;
#12444=ORIENTED_EDGE ( 'NONE', *, *, #44847, .T. ) ;
#12445=DIRECTION ( 'NONE',  ( 0.7660212471507180654, -0.6427876096865404731, 0.005961354470445141482 ) ) ;
#12446=ORIENTED_EDGE ( 'NONE', *, *, #44847, .F. ) ;
#12447=CARTESIAN_POINT ( 'NONE',  ( -17.74560456716937296, 0.000000000000000000, 3.774316574337878372 ) ) ;
#12448=VECTOR ( 'NONE', #47822, 1000.000000000000227 ) ;
#12449=EDGE_CURVE ( 'NONE', #55206, #46834, #45334, .T. ) ;
#12450=LINE ( 'NONE', #7311, #34805 ) ;
#12451=CARTESIAN_POINT ( 'NONE',  ( -25.20200914511100265, -0.1191753592594197858, 6.570942640130446932 ) ) ;
#12452=VECTOR ( 'NONE', #29059, 1000.000000000000227 ) ;
#12453=DIRECTION ( 'NONE',  ( -0.005961354470445682716, -0.6427876096865404731, 0.7660212471507180654 ) ) ;
#12454=DIRECTION ( 'NONE',  ( -0.5364919789714478471, 0.6444004775717705469, -0.5449076811759709926 ) ) ;
#12455=DIRECTION ( 'NONE',  ( -0.005002170337468016433, -0.7660444431189770143, 0.6427681459581293666 ) ) ;
#12456=LINE ( 'NONE', #51033, #7599 ) ;
#12457=DIRECTION ( 'NONE',  ( -0.005961354470445682716, -0.6427876096865404731, 0.7660212471507180654 ) ) ;
#12458=ORIENTED_EDGE ( 'NONE', *, *, #46552, .T. ) ;
#12459=CARTESIAN_POINT ( 'NONE',  ( -19.60912206198628027, -0.1191753592594197858, 4.398475361799976113 ) ) ;
#12460=EDGE_LOOP ( 'NONE', ( #52919, #52718, #12703, #14349, #21656 ) ) ;
#12461=VECTOR ( 'NONE', #35927, 1000.000000000000227 ) ;
#12462=DIRECTION ( 'NONE',  ( 0.5449076811759707706, 0.6444004775717708799, -0.5364919789714476250 ) ) ;
#12463=CARTESIAN_POINT ( 'NONE',  ( -15.96710241509184058, -0.1191753592594218814, 13.13259134697452879 ) ) ;
#12464=DIRECTION ( 'NONE',  ( 0.000000000000000000, -1.000000000000000000, 0.000000000000000000 ) ) ;
#12465=LINE ( 'NONE', #29783, #15872 ) ;
#12466=LINE ( 'NONE', #20692, #8692 ) ;
#12467=CARTESIAN_POINT ( 'NONE',  ( -18.89843909413720624, 4.495856970884009485, 11.60058387806120273 ) ) ;
#12469=ORIENTED_EDGE ( 'NONE', *, *, #17190, .F. ) ;
#12470=DIRECTION ( 'NONE',  ( -0.9999697198139514409, -0.000000000000000000, -0.007781995580013368816 ) ) ;
#12471=LINE ( 'NONE', #21244, #1347 ) ;
#12472=EDGE_CURVE ( 'NONE', #35002, #41926, #19780, .T. ) ;
#12474=EDGE_CURVE ( 'NONE', #44163, #52435, #23748, .T. ) ;
#12475=FACE_OUTER_BOUND ( 'NONE', #24600, .T. ) ;
#12477=CARTESIAN_POINT ( 'NONE',  ( 2.072287782118878319, 0.000000000000000000, -2.950529333540147015 ) ) ;
#12478=EDGE_CURVE ( 'NONE', #41818, #7991, #5595, .T. ) ;
#12479=DIRECTION ( 'NONE',  ( 0.007781995580012663651, -3.146120232559066537E-19, -0.9999697198139514409 ) ) ;
#12480=ORIENTED_EDGE ( 'NONE', *, *, #55712, .T. ) ;
#12481=CARTESIAN_POINT ( 'NONE',  ( -14.61771687497231653, 0.000000000000000000, 6.014650938452181350 ) ) ;
#12482=PLANE ( 'NONE',  #49577 ) ;
#12483=ORIENTED_EDGE ( 'NONE', *, *, #41415, .T. ) ;
#12484=ORIENTED_EDGE ( 'NONE', *, *, #9442, .F. ) ;
#12485=DIRECTION ( 'NONE',  ( 0.005961354470445682716, -0.6427876096865404731, -0.7660212471507180654 ) ) ;
#12486=ORIENTED_EDGE ( 'NONE', *, *, #26071, .T. ) ;
#12487=EDGE_CURVE ( 'NONE', #26117, #30596, #10136, .T. ) ;
#12489=EDGE_LOOP ( 'NONE', ( #20501, #39140, #24285, #34960 ) ) ;
#12490=EDGE_LOOP ( 'NONE', ( #23406, #18410, #3307, #4350 ) ) ;
#12492=DIRECTION ( 'NONE',  ( -0.005002170337468016433, -0.7660444431189770143, 0.6427681459581293666 ) ) ;
#12493=LINE ( 'NONE', #25266, #5170 ) ;
#12494=DIRECTION ( 'NONE',  ( 0.005002170337468016433, -0.7660444431189770143, -0.6427681459581293666 ) ) ;
#12495=VECTOR ( 'NONE', #45452, 999.9999999999998863 ) ;
#12496=EDGE_LOOP ( 'NONE', ( #48702, #50376, #48646, #34538 ) ) ;
#12497=EDGE_LOOP ( 'NONE', ( #39158, #4250, #38101, #12960 ) ) ;
#12498=LINE ( 'NONE', #8807, #27466 ) ;
#12499=LINE ( 'NONE', #46853, #20938 ) ;
#12500=VERTEX_POINT ( 'NONE', #36272 ) ;
#12501=FACE_OUTER_BOUND ( 'NONE', #28683, .T. ) ;
#12502=LINE ( 'NONE', #26370, #36776 ) ;
#12503=EDGE_LOOP ( 'NONE', ( #710, #50096, #10170, #52663 ) ) ;
#12504=LINE ( 'NONE', #38313, #4969 ) ;
#12505=ORIENTED_EDGE ( 'NONE', *, *, #52272, .T. ) ;
#12506=CARTESIAN_POINT ( 'NONE',  ( -11.83121314831507931, 0.000000000000000000, 6.205662168355214448 ) ) ;
#12507=ADVANCED_FACE ( 'NONE', ( #49319 ), #6443, .F. ) ;
#12508=CARTESIAN_POINT ( 'NONE',  ( -17.39147930267917275, 1.095915999411505082, 5.435347155529250962 ) ) ;
#12509=VERTEX_POINT ( 'NONE', #44779 ) ;
#12510=DIRECTION ( 'NONE',  ( 0.9999697198139515519, 0.000000000000000000, 0.007781995580013368816 ) ) ;
#12511=LINE ( 'NONE', #21295, #27489 ) ;
#12512=CARTESIAN_POINT ( 'NONE',  ( -17.76077782080467315, -0.1191753592594195638, 4.782191673879427007 ) ) ;
#12513=LINE ( 'NONE', #26383, #11086 ) ;
#12514=ORIENTED_EDGE ( 'NONE', *, *, #44107, .T. ) ;
#12517=DIRECTION ( 'NONE',  ( -0.6427681459581293666, -0.7660444431189770143, -0.005002170337467561935 ) ) ;
#12518=CARTESIAN_POINT ( 'NONE',  ( -17.32488145901641374, -0.1191753592594153865, 8.478904618225078238 ) ) ;
#12519=FACE_OUTER_BOUND ( 'NONE', #2155, .T. ) ;
#12520=CARTESIAN_POINT ( 'NONE',  ( -18.67697421479883602, -0.1191753592594185784, 4.036397482078228904 ) ) ;
#12521=EDGE_CURVE ( 'NONE', #32241, #50224, #40805, .T. ) ;
#12522=FACE_OUTER_BOUND ( 'NONE', #33133, .T. ) ;
#12523=CARTESIAN_POINT ( 'NONE',  ( -9.442067484779661513, -0.1191753592594197858, 10.59804618892231254 ) ) ;
#12524=EDGE_CURVE ( 'NONE', #27823, #2633, #1878, .T. ) ;
#12525=DIRECTION ( 'NONE',  ( -0.5449076811759708816, 0.6444004775717707689, 0.5364919789714475140 ) ) ;
#12526=ORIENTED_EDGE ( 'NONE', *, *, #32056, .T. ) ;
#12528=ORIENTED_EDGE ( 'NONE', *, *, #22411, .T. ) ;
#12529=DIRECTION ( 'NONE',  ( 0.7660212471507180654, -0.6427876096865404731, 0.005961354470445141482 ) ) ;
#12530=ADVANCED_FACE ( 'NONE', ( #41370 ), #45604, .F. ) ;
#12531=LINE ( 'NONE', #47145, #3694 ) ;
#12532=AXIS2_PLACEMENT_3D ( 'NONE', #43333, #20876, #38198 ) ;
#12533=EDGE_CURVE ( 'NONE', #12359, #38932, #36532, .T. ) ;
#12534=CARTESIAN_POINT ( 'NONE',  ( -17.85867893883878565, 0.000000000000000000, 4.512100743045057705 ) ) ;
#12535=FACE_OUTER_BOUND ( 'NONE', #16900, .T. ) ;
#12536=EDGE_CURVE ( 'NONE', #26517, #3186, #9877, .T. ) ;
#12538=ORIENTED_EDGE ( 'NONE', *, *, #13491, .F. ) ;
#12539=ORIENTED_EDGE ( 'NONE', *, *, #17856, .F. ) ;
#12540=DIRECTION ( 'NONE',  ( 0.7660212471507180654, -0.6427876096865404731, 0.005961354470445141482 ) ) ;
#12541=DIRECTION ( 'NONE',  ( 0.7660212471507180654, -0.6427876096865404731, 0.005961354470445141482 ) ) ;
#12542=ORIENTED_EDGE ( 'NONE', *, *, #22951, .F. ) ;
#12543=LINE ( 'NONE', #16791, #30234 ) ;
#12544=EDGE_CURVE ( 'NONE', #35256, #40645, #32301, .T. ) ;
#12545=ORIENTED_EDGE ( 'NONE', *, *, #5224, .F. ) ;
#12547=ORIENTED_EDGE ( 'NONE', *, *, #42390, .T. ) ;
#12548=DIRECTION ( 'NONE',  ( 0.5364919789714477361, 0.6444004775717706579, 0.5449076811759711036 ) ) ;
#12549=EDGE_CURVE ( 'NONE', #22074, #4830, #14421, .T. ) ;
#12550=VERTEX_POINT ( 'NONE', #49033 ) ;
#12551=ORIENTED_EDGE ( 'NONE', *, *, #9529, .F. ) ;
#12552=ORIENTED_EDGE ( 'NONE', *, *, #2312, .T. ) ;
#12553=DIRECTION ( 'NONE',  ( 0.007781995580012663651, 0.000000000000000000, -0.9999697198139515519 ) ) ;
#12554=PLANE ( 'NONE',  #13276 ) ;
#12555=CARTESIAN_POINT ( 'NONE',  ( -11.25586126502947337, -0.1191753592594179401, 4.832814438631556797 ) ) ;
#12556=DIRECTION ( 'NONE',  ( 0.007781995580012663651, 0.000000000000000000, -0.9999697198139515519 ) ) ;
#12557=ORIENTED_EDGE ( 'NONE', *, *, #17194, .F. ) ;
#12558=ORIENTED_EDGE ( 'NONE', *, *, #46702, .T. ) ;
#12559=ORIENTED_EDGE ( 'NONE', *, *, #2563, .F. ) ;
#12560=CARTESIAN_POINT ( 'NONE',  ( -12.52654812221797442, 3.038739411681507185, 6.734146878685358217 ) ) ;
#12561=CARTESIAN_POINT ( 'NONE',  ( -9.489466688688677820, 0.000000000000000000, 3.838567748353698850 ) ) ;
#12562=ORIENTED_EDGE ( 'NONE', *, *, #11519, .T. ) ;
#12563=CARTESIAN_POINT ( 'NONE',  ( -12.91543455048469369, 4.657758921906512306, 1.550118225248739101 ) ) ;
#12564=VERTEX_POINT ( 'NONE', #15497 ) ;
#12565=DIRECTION ( 'NONE',  ( 0.9999697198139515519, 0.000000000000000000, 0.007781995580013368816 ) ) ;
#12566=LINE ( 'NONE', #30455, #39430 ) ;
#12567=VECTOR ( 'NONE', #11177, 999.9999999999998863 ) ;
#12568=EDGE_LOOP ( 'NONE', ( #46939, #7165, #33075, #51824 ) ) ;
#12569=FACE_OUTER_BOUND ( 'NONE', #31918, .T. ) ;
#12570=ADVANCED_FACE ( 'NONE', ( #7267 ), #24318, .F. ) ;
#12571=VERTEX_POINT ( 'NONE', #29120 ) ;
#12572=CARTESIAN_POINT ( 'NONE',  ( -10.82591808402700551, -0.1941918491731536578, 1.205787872916244341 ) ) ;
#12573=DIRECTION ( 'NONE',  ( -0.9999697198139514409, -0.000000000000000000, -0.007781995580013368816 ) ) ;
#12574=VERTEX_POINT ( 'NONE', #55246 ) ;
#12575=DIRECTION ( 'NONE',  ( -0.005961354470445682716, -0.6427876096865404731, 0.7660212471507180654 ) ) ;
#12576=LINE ( 'NONE', #30468, #17552 ) ;
#12578=PLANE ( 'NONE',  #136 ) ;
#12579=EDGE_LOOP ( 'NONE', ( #984, #8749, #312, #41465 ) ) ;
#12580=ADVANCED_FACE ( 'NONE', ( #24871 ), #50971, .F. ) ;
#12581=PLANE ( 'NONE',  #27357 ) ;
#12582=PLANE ( 'NONE',  #41241 ) ;
#12583=FACE_OUTER_BOUND ( 'NONE', #554, .T. ) ;
#12584=DIRECTION ( 'NONE',  ( -0.005002170337468016433, -0.7660444431189770143, 0.6427681459581293666 ) ) ;
#12585=PLANE ( 'NONE',  #47878 ) ;
#12586=ADVANCED_FACE ( 'NONE', ( #47019 ), #15781, .F. ) ;
#12587=DIRECTION ( 'NONE',  ( 0.3313982828793700097, 0.4028455766673916805, 0.8531650599175528704 ) ) ;
#12588=EDGE_LOOP ( 'NONE', ( #55360, #52892, #10241, #21289 ) ) ;
#12589=CARTESIAN_POINT ( 'NONE',  ( -21.17348044452715783, -5.213152330870663320, 13.46210170089576508 ) ) ;
#12590=FACE_OUTER_BOUND ( 'NONE', #49118, .T. ) ;
#12591=FACE_OUTER_BOUND ( 'NONE', #54135, .T. ) ;
#12592=ORIENTED_EDGE ( 'NONE', *, *, #19549, .T. ) ;
#12593=CARTESIAN_POINT ( 'NONE',  ( -17.75790376729938913, -0.1191753592594196193, 4.412881970621663541 ) ) ;
#12594=ORIENTED_EDGE ( 'NONE', *, *, #5523, .F. ) ;
#12595=DIRECTION ( 'NONE',  ( -0.6427681459581293666, -0.7660444431189770143, -0.005002170337467561935 ) ) ;
#12596=DIRECTION ( 'NONE',  ( -0.7660212471507179544, -0.6427876096865405842, -0.005961354470445141482 ) ) ;
#12597=EDGE_CURVE ( 'NONE', #21470, #31183, #32823, .T. ) ;
#12598=LINE ( 'NONE', #48061, #41397 ) ;
#12599=EDGE_CURVE ( 'NONE', #33755, #14988, #16335, .T. ) ;
#12601=ORIENTED_EDGE ( 'NONE', *, *, #39939, .F. ) ;
#12602=ORIENTED_EDGE ( 'NONE', *, *, #6549, .F. ) ;
#12604=DIRECTION ( 'NONE',  ( 0.6427681459581294776, -0.7660444431189769032, 0.005002170337467562802 ) ) ;
#12605=DIRECTION ( 'NONE',  ( -0.7660212471507179544, -0.6427876096865405842, -0.005961354470445141482 ) ) ;
#12606=LINE ( 'NONE', #29924, #13922 ) ;
#12607=EDGE_CURVE ( 'NONE', #15806, #37866, #33126, .T. ) ;
#12608=VECTOR ( 'NONE', #55184, 1000.000000000000227 ) ;
#12609=PLANE ( 'NONE',  #1993 ) ;
#12610=CARTESIAN_POINT ( 'NONE',  ( -20.35841145877394354, 0.000000000000000000, 5.231311386181617173 ) ) ;
#12611=ORIENTED_EDGE ( 'NONE', *, *, #11355, .T. ) ;
#12612=DIRECTION ( 'NONE',  ( 0.9999697198139515519, 0.000000000000000000, 0.007781995580013368816 ) ) ;
#12613=EDGE_CURVE ( 'NONE', #5013, #28164, #20877, .T. ) ;
#12614=CARTESIAN_POINT ( 'NONE',  ( -16.71693315311381767, -3.270328918600659218, 8.542523180522204385 ) ) ;
#12615=EDGE_LOOP ( 'NONE', ( #40946, #30822, #28320, #35744 ) ) ;
#12616=LINE ( 'NONE', #25663, #4781 ) ;
#12617=CARTESIAN_POINT ( 'NONE',  ( -15.54124256164392293, 0.000000000000000000, 5.268799708400632831 ) ) ;
#12618=CARTESIAN_POINT ( 'NONE',  ( -10.91056151514876049, 0.000000000000000000, 7.320823101664526433 ) ) ;
#12619=ORIENTED_EDGE ( 'NONE', *, *, #46255, .T. ) ;
#12620=DIRECTION ( 'NONE',  ( 0.7660212471507180654, -0.6427876096865404731, 0.005961354470445141482 ) ) ;
#12621=ORIENTED_EDGE ( 'NONE', *, *, #48483, .T. ) ;
#12622=ORIENTED_EDGE ( 'NONE', *, *, #43984, .F. ) ;
#12623=VERTEX_POINT ( 'NONE', #3570 ) ;
#12624=EDGE_LOOP ( 'NONE', ( #31781, #10248, #49327, #10229 ) ) ;
#12625=DIRECTION ( 'NONE',  ( 0.000000000000000000, -1.000000000000000000, 0.000000000000000000 ) ) ;
#12627=ORIENTED_EDGE ( 'NONE', *, *, #26257, .T. ) ;
#12628=ADVANCED_FACE ( 'NONE', ( #41891 ), #54674, .F. ) ;
#12629=PLANE ( 'NONE',  #53974 ) ;
#12630=ORIENTED_EDGE ( 'NONE', *, *, #34700, .F. ) ;
#12631=LINE ( 'NONE', #3809, #5064 ) ;
#12632=ORIENTED_EDGE ( 'NONE', *, *, #14826, .F. ) ;
#12633=PLANE ( 'NONE',  #32852 ) ;
#12634=EDGE_CURVE ( 'NONE', #55568, #44513, #25174, .T. ) ;
#12635=VERTEX_POINT ( 'NONE', #55519 ) ;
#12636=DIRECTION ( 'NONE',  ( 0.7660212471507180654, -0.6427876096865404731, 0.005961354470445141482 ) ) ;
#12637=DIRECTION ( 'NONE',  ( 0.9999697198139515519, 0.000000000000000000, 0.007781995580013368816 ) ) ;
#12638=EDGE_CURVE ( 'NONE', #83, #36758, #7545, .T. ) ;
#12639=CARTESIAN_POINT ( 'NONE',  ( -15.86710544311044302, 0.000000000000000000, 13.13336954653252953 ) ) ;
#12640=LINE ( 'NONE', #16601, #43228 ) ;
#12641=DIRECTION ( 'NONE',  ( 0.6427681459581294776, -0.7660444431189769032, 0.005002170337467562802 ) ) ;
#12642=ORIENTED_EDGE ( 'NONE', *, *, #22172, .F. ) ;
#12643=ADVANCED_FACE ( 'NONE', ( #28865 ), #37940, .F. ) ;
#12644=EDGE_CURVE ( 'NONE', #30203, #45792, #12078, .T. ) ;
#12645=ADVANCED_FACE ( 'NONE', ( #29416 ), #7015, .F. ) ;
#12646=VECTOR ( 'NONE', #20752, 1000.000000000000114 ) ;
#12647=ORIENTED_EDGE ( 'NONE', *, *, #16736, .F. ) ;
#12648=CARTESIAN_POINT ( 'NONE',  ( -13.63673279712320507, -0.1191753592594197858, 12.22739664767016521 ) ) ;
#12649=CARTESIAN_POINT ( 'NONE',  ( -11.87243407472968926, 0.000000000000000000, 11.50246268866867361 ) ) ;
#12650=LINE ( 'NONE', #26010, #41471 ) ;
#12652=LINE ( 'NONE', #43027, #23116 ) ;
#12653=CARTESIAN_POINT ( 'NONE',  ( -14.01701317841955508, 0.000000000000000000, 2.326005055450897085 ) ) ;
#12654=EDGE_LOOP ( 'NONE', ( #10622, #14090, #40823, #12258 ) ) ;
#12655=PLANE ( 'NONE',  #40210 ) ;
#12656=CARTESIAN_POINT ( 'NONE',  ( -16.43317633868556626, -0.1191753592594197858, 13.31363028683540151 ) ) ;
#12657=ORIENTED_EDGE ( 'NONE', *, *, #10640, .F. ) ;
#12658=CARTESIAN_POINT ( 'NONE',  ( -11.82702144042051984, 0.000000000000000000, 5.667036705802473762 ) ) ;
#12659=CARTESIAN_POINT ( 'NONE',  ( -13.21362762481721020, 0.000000000000000000, 4.717575620020126870 ) ) ;
#12660=ADVANCED_FACE ( 'NONE', ( #21165 ), #11250, .F. ) ;
#12662=EDGE_CURVE ( 'NONE', #2262, #19938, #20033, .T. ) ;
#12663=DIRECTION ( 'NONE',  ( -0.3313982828793700652, 0.4028455766673916250, -0.8531650599175529814 ) ) ;
#12664=ADVANCED_FACE ( 'NONE', ( #47868 ), #12931, .F. ) ;
#12665=EDGE_LOOP ( 'NONE', ( #15752, #37726, #25275, #44776 ) ) ;
#12666=VERTEX_POINT ( 'NONE', #26843 ) ;
#12667=EDGE_CURVE ( 'NONE', #38691, #32780, #30260, .T. ) ;
#12668=CARTESIAN_POINT ( 'NONE',  ( -16.84047315302936454, -5.051250379848161387, 11.51330583538055130 ) ) ;
#12669=CARTESIAN_POINT ( 'NONE',  ( -11.35795409095814712, 0.000000000000000000, 5.101348970349929068 ) ) ;
#12670=CARTESIAN_POINT ( 'NONE',  ( -15.79726335400637183, 0.000000000000000000, 4.158811085975333555 ) ) ;
#12671=EDGE_CURVE ( 'NONE', #39021, #883, #25711, .T. ) ;
#12672=DIRECTION ( 'NONE',  ( 0.000000000000000000, -1.000000000000000000, 0.000000000000000000 ) ) ;
#12673=DIRECTION ( 'NONE',  ( 0.5364919789714477361, 0.6444004775717706579, 0.5449076811759711036 ) ) ;
#12674=CARTESIAN_POINT ( 'NONE',  ( -24.26986129792355129, -0.1191753592594197858, 6.208864760408702388 ) ) ;
#12675=PLANE ( 'NONE',  #11174 ) ;
#12676=EDGE_CURVE ( 'NONE', #12635, #12199, #8694, .T. ) ;
#12677=VERTEX_POINT ( 'NONE', #17767 ) ;
#12678=FACE_OUTER_BOUND ( 'NONE', #54792, .T. ) ;
#12679=FACE_OUTER_BOUND ( 'NONE', #43523, .T. ) ;
#12680=CARTESIAN_POINT ( 'NONE',  ( -18.67775241435682432, 0.000000000000000000, 4.136394454059623804 ) ) ;
#12682=LINE ( 'NONE', #7880, #37706 ) ;
#12685=ORIENTED_EDGE ( 'NONE', *, *, #6546, .F. ) ;
#12686=ORIENTED_EDGE ( 'NONE', *, *, #141, .T. ) ;
#12687=ORIENTED_EDGE ( 'NONE', *, *, #5348, .T. ) ;
#12688=EDGE_LOOP ( 'NONE', ( #40683, #20850, #3959, #25054 ) ) ;
#12689=EDGE_LOOP ( 'NONE', ( #47404, #55466, #16359, #40454 ) ) ;
#12690=CARTESIAN_POINT ( 'NONE',  ( -18.34507117752021088, 3.848249166794009746, 10.32280225099176185 ) ) ;
#12691=LINE ( 'NONE', #39673, #7550 ) ;
#12692=DIRECTION ( 'NONE',  ( 0.007781995580012662783, 0.000000000000000000, -0.9999697198139514409 ) ) ;
#12693=ORIENTED_EDGE ( 'NONE', *, *, #45271, .T. ) ;
#12694=CARTESIAN_POINT ( 'NONE',  ( -14.20280369269832832, 0.000000000000000000, 12.40765738797303719 ) ) ;
#12695=ORIENTED_EDGE ( 'NONE', *, *, #18408, .F. ) ;
#12697=ORIENTED_EDGE ( 'NONE', *, *, #52905, .T. ) ;
#12698=CARTESIAN_POINT ( 'NONE',  ( -19.59569683186026268, 0.000000000000000000, 14.58168106541950948 ) ) ;
#12699=CARTESIAN_POINT ( 'NONE',  ( -20.18761906488554914, -0.7980104508677885455, 5.671006189966389499 ) ) ;
#12700=CARTESIAN_POINT ( 'NONE',  ( -17.34043131654819092, 1.581621852479005552, 6.212644435970458900 ) ) ;
#12701=ORIENTED_EDGE ( 'NONE', *, *, #9911, .T. ) ;
#12702=CARTESIAN_POINT ( 'NONE',  ( -27.99923088623136636, 0.000000000000000000, 7.757173251277078130 ) ) ;
#12703=ORIENTED_EDGE ( 'NONE', *, *, #5500, .T. ) ;
#12704=EDGE_CURVE ( 'NONE', #27150, #39340, #122, .T. ) ;
#12706=DIRECTION ( 'NONE',  ( -0.6427681459581293666, -0.7660444431189770143, -0.005002170337467561935 ) ) ;
#12707=CARTESIAN_POINT ( 'NONE',  ( -18.67619601524082285, 0.000000000000000000, 3.936400510096834893 ) ) ;
#12708=EDGE_CURVE ( 'NONE', #46096, #37185, #52404, .T. ) ;
#12709=VECTOR ( 'NONE', #14637, 1000.000000000000227 ) ;
#12710=DIRECTION ( 'NONE',  ( 0.007781995580012662783, 0.000000000000000000, -0.9999697198139514409 ) ) ;
#12711=PLANE ( 'NONE',  #46720 ) ;
#12712=PLANE ( 'NONE',  #6618 ) ;
#12714=LINE ( 'NONE', #47341, #34809 ) ;
#12715=PLANE ( 'NONE',  #41337 ) ;
#12716=EDGE_LOOP ( 'NONE', ( #15741, #32594, #8936, #28617 ) ) ;
#12718=VERTEX_POINT ( 'NONE', #26272 ) ;
#12719=CARTESIAN_POINT ( 'NONE',  ( -14.01545677930355183, 0.000000000000000000, 2.126011111488108174 ) ) ;
#12720=LINE ( 'NONE', #12463, #11466 ) ;
#12721=CARTESIAN_POINT ( 'NONE',  ( -16.06709938707323460, 0.000000000000000000, 13.13181314741652628 ) ) ;
#12722=CARTESIAN_POINT ( 'NONE',  ( -23.33693525117809386, 0.000000000000000000, 5.746789908705562944 ) ) ;
#12723=DIRECTION ( 'NONE',  ( 0.7660212471507180654, -0.6427876096865404731, 0.005961354470445141482 ) ) ;
#12724=DIRECTION ( 'NONE',  ( -0.9321478471874540261, 0.000000000000000000, 0.3620778797217457656 ) ) ;
#12725=LINE ( 'NONE', #8189, #35580 ) ;
#12727=VERTEX_POINT ( 'NONE', #4430 ) ;
#12728=CARTESIAN_POINT ( 'NONE',  ( -23.33693525117809386, 0.000000000000000000, 5.746789908705562944 ) ) ;
#12729=CARTESIAN_POINT ( 'NONE',  ( -18.29747203306047609, -0.1191753592594177458, 14.03778604627889059 ) ) ;
#12730=CARTESIAN_POINT ( 'NONE',  ( -16.79925329029790149, 0.000000000000000000, 13.49544742625427496 ) ) ;
#12731=EDGE_CURVE ( 'NONE', #17974, #54313, #48407, .T. ) ;
#12732=CARTESIAN_POINT ( 'NONE',  ( -20.54126990917373874, 0.000000000000000000, 4.760553241521714440 ) ) ;
#12734=EDGE_CURVE ( 'NONE', #8596, #19207, #22309, .T. ) ;
#12735=CARTESIAN_POINT ( 'NONE',  ( -8.846271876811060864, 0.000000000000000000, 6.598223741337037040 ) ) ;
#12736=CARTESIAN_POINT ( 'NONE',  ( -24.27063949748155380, 0.000000000000000000, 6.308861732390097288 ) ) ;
#12737=VERTEX_POINT ( 'NONE', #51563 ) ;
#12738=CARTESIAN_POINT ( 'NONE',  ( -30.79567442779373110, 0.000000000000000000, 8.843406890442315316 ) ) ;
#12739=DIRECTION ( 'NONE',  ( 0.000000000000000000, -1.000000000000000000, 0.000000000000000000 ) ) ;
#12740=ORIENTED_EDGE ( 'NONE', *, *, #55088, .F. ) ;
#12741=EDGE_CURVE ( 'NONE', #21963, #30486, #43334, .T. ) ;
#12742=EDGE_LOOP ( 'NONE', ( #22355, #9484, #7046, #24675 ) ) ;
#12743=CARTESIAN_POINT ( 'NONE',  ( 2.072287782118878319, 0.000000000000000000, -2.950529333540147015 ) ) ;
#12744=EDGE_CURVE ( 'NONE', #38231, #14055, #55819, .T. ) ;
#12745=ORIENTED_EDGE ( 'NONE', *, *, #37662, .F. ) ;
#12746=ADVANCED_FACE ( 'NONE', ( #35103 ), #43865, .F. ) ;
#12747=VECTOR ( 'NONE', #20034, 1000.000000000000227 ) ;
#12748=ORIENTED_EDGE ( 'NONE', *, *, #38213, .T. ) ;
#12750=VERTEX_POINT ( 'NONE', #38793 ) ;
#12751=CARTESIAN_POINT ( 'NONE',  ( -13.08486533123210194, 0.000000000000000000, 1.963927175729152541 ) ) ;
#12752=ORIENTED_EDGE ( 'NONE', *, *, #11789, .T. ) ;
#12754=LINE ( 'NONE', #24404, #18557 ) ;
#12755=VERTEX_POINT ( 'NONE', #4689 ) ;
#12756=ORIENTED_EDGE ( 'NONE', *, *, #19225, .T. ) ;
#12757=LINE ( 'NONE', #52497, #37512 ) ;
#12758=ORIENTED_EDGE ( 'NONE', *, *, #50347, .F. ) ;
#12759=CARTESIAN_POINT ( 'NONE',  ( -12.15271748404464880, 0.000000000000000000, 1.601849296007406664 ) ) ;
#12760=LINE ( 'NONE', #42580, #5039 ) ;
#12761=ORIENTED_EDGE ( 'NONE', *, *, #48405, .T. ) ;
#12762=LINE ( 'NONE', #21586, #22064 ) ;
#12763=EDGE_CURVE ( 'NONE', #40825, #41994, #16932, .T. ) ;
#12764=ORIENTED_EDGE ( 'NONE', *, *, #9959, .T. ) ;
#12765=VECTOR ( 'NONE', #41182, 1000.000000000000227 ) ;
#12766=PLANE ( 'NONE',  #41810 ) ;
#12767=ADVANCED_FACE ( 'NONE', ( #39052 ), #34794, .F. ) ;
#12768=EDGE_CURVE ( 'NONE', #21349, #22899, #35358, .T. ) ;
#12769=CARTESIAN_POINT ( 'NONE',  ( -17.74482636761137044, -0.1191753592594197858, 3.674319602356483916 ) ) ;
#12770=ORIENTED_EDGE ( 'NONE', *, *, #55046, .F. ) ;
#12771=DIRECTION ( 'NONE',  ( 0.7660212471507180654, -0.6427876096865404731, 0.005961354470445141482 ) ) ;
#12772=CARTESIAN_POINT ( 'NONE',  ( -12.13851405436063047, 0.000000000000000000, 11.68505802764555135 ) ) ;
#12773=CARTESIAN_POINT ( 'NONE',  ( -21.10098843074258923, -2.946525016555658016, 9.714021765596209335 ) ) ;
#12774=CARTESIAN_POINT ( 'NONE',  ( -8.828121567967061267, 0.000000000000000000, 4.265948033562787955 ) ) ;
#12775=VERTEX_POINT ( 'NONE', #12659 ) ;
#12776=AXIS2_PLACEMENT_3D ( 'NONE', #42019, #46021, #24423 ) ;
#12777=DIRECTION ( 'NONE',  ( 0.007781995580012663651, -3.146120232559066537E-19, -0.9999697198139514409 ) ) ;
#12778=DIRECTION ( 'NONE',  ( -0.005961354470445682716, -0.6427876096865404731, 0.7660212471507180654 ) ) ;
#12779=PLANE ( 'NONE',  #44855 ) ;
#12780=PLANE ( 'NONE',  #41387 ) ;
#12781=LINE ( 'NONE', #47417, #35033 ) ;
#12782=CARTESIAN_POINT ( 'NONE',  ( -15.34256627207041390, 0.000000000000000000, 5.439671866811612411 ) ) ;
#12783=DIRECTION ( 'NONE',  ( 0.6427681459581294776, -0.7660444431189769032, 0.005002170337467562802 ) ) ;
#12784=EDGE_CURVE ( 'NONE', #21737, #26746, #29975, .T. ) ;
#12785=VECTOR ( 'NONE', #25501, 1000.000000000000227 ) ;
#12786=LINE ( 'NONE', #4547, #3923 ) ;
#12787=DIRECTION ( 'NONE',  ( 0.5364919789714477361, 0.6444004775717706579, 0.5449076811759711036 ) ) ;
#12788=ORIENTED_EDGE ( 'NONE', *, *, #33158, .F. ) ;
#12790=ORIENTED_EDGE ( 'NONE', *, *, #25608, .T. ) ;
#12791=LINE ( 'NONE', #29848, #8433 ) ;
#12792=FACE_OUTER_BOUND ( 'NONE', #20434, .T. ) ;
#12795=EDGE_CURVE ( 'NONE', #38515, #17105, #49245, .T. ) ;
#12796=CARTESIAN_POINT ( 'NONE',  ( -10.70062775628084495, 0.000000000000000000, 6.045134631712261175 ) ) ;
#12797=DIRECTION ( 'NONE',  ( 0.5364919789714477361, 0.6444004775717706579, 0.5449076811759711036 ) ) ;
#12798=ORIENTED_EDGE ( 'NONE', *, *, #14701, .F. ) ;
#12799=ORIENTED_EDGE ( 'NONE', *, *, #53807, .T. ) ;
#12800=DIRECTION ( 'NONE',  ( 0.6427681459581294776, -0.7660444431189769032, 0.005002170337467562802 ) ) ;
#12801=DIRECTION ( 'NONE',  ( 0.005961354470445682716, -0.6427876096865404731, -0.7660212471507180654 ) ) ;
#12802=ORIENTED_EDGE ( 'NONE', *, *, #26576, .F. ) ;
#12803=PLANE ( 'NONE',  #32933 ) ;
#12804=VECTOR ( 'NONE', #52271, 1000.000000000000227 ) ;
#12805=VECTOR ( 'NONE', #22126, 1000.000000000000227 ) ;
#12806=ORIENTED_EDGE ( 'NONE', *, *, #6944, .T. ) ;
#12807=DIRECTION ( 'NONE',  ( -0.7660212471507179544, -0.6427876096865405842, -0.005961354470445141482 ) ) ;
#12808=ADVANCED_FACE ( 'NONE', ( #27118 ), #22582, .F. ) ;
#12809=VERTEX_POINT ( 'NONE', #27681 ) ;
#12810=DIRECTION ( 'NONE',  ( 0.5449076811759707706, 0.6444004775717708799, -0.5364919789714476250 ) ) ;
#12811=ORIENTED_EDGE ( 'NONE', *, *, #51082, .T. ) ;
#12812=EDGE_LOOP ( 'NONE', ( #26808, #32387, #55816, #51381 ) ) ;
#12813=ORIENTED_EDGE ( 'NONE', *, *, #17369, .T. ) ;
#12814=CARTESIAN_POINT ( 'NONE',  ( -22.40478740399063895, 0.000000000000000000, 5.384712028983816623 ) ) ;
#12815=DIRECTION ( 'NONE',  ( -0.005961354470445682716, -0.6427876096865404731, 0.7660212471507180654 ) ) ;
#12816=CARTESIAN_POINT ( 'NONE',  ( -15.50102849149811135, -0.1191753592594197858, 12.95155240711365430 ) ) ;
#12817=ADVANCED_FACE ( 'NONE', ( #32223 ), #53261, .F. ) ;
#12818=CARTESIAN_POINT ( 'NONE',  ( -16.11251725036584048, -3.108426967578159061, 8.042038833893970562 ) ) ;
#12820=EDGE_LOOP ( 'NONE', ( #45005, #33824, #47047, #41399 ) ) ;
#12821=EDGE_CURVE ( 'NONE', #39352, #37185, #14607, .T. ) ;
#12822=EDGE_CURVE ( 'NONE', #28898, #52574, #52949, .T. ) ;
#12823=VECTOR ( 'NONE', #40353, 999.9999999999998863 ) ;
#12824=ORIENTED_EDGE ( 'NONE', *, *, #5529, .T. ) ;
#12825=DIRECTION ( 'NONE',  ( 0.000000000000000000, -0.000000000000000000, -1.000000000000000000 ) ) ;
#12826=ORIENTED_EDGE ( 'NONE', *, *, #14952, .F. ) ;
#12828=EDGE_CURVE ( 'NONE', #54772, #12635, #2085, .T. ) ;
#12829=ORIENTED_EDGE ( 'NONE', *, *, #21989, .F. ) ;
#12830=PLANE ( 'NONE',  #6081 ) ;
#12831=LINE ( 'NONE', #30153, #19470 ) ;
#12832=VERTEX_POINT ( 'NONE', #19419 ) ;
#12833=ADVANCED_FACE ( 'NONE', ( #23426 ), #36207, .F. ) ;
#12834=DIRECTION ( 'NONE',  ( 0.005961354470445682716, -0.6427876096865404731, -0.7660212471507180654 ) ) ;
#12835=ORIENTED_EDGE ( 'NONE', *, *, #49629, .F. ) ;
#12837=DIRECTION ( 'NONE',  ( -0.005961354470445682716, -0.6427876096865404731, 0.7660212471507180654 ) ) ;
#12838=ORIENTED_EDGE ( 'NONE', *, *, #26190, .F. ) ;
#12839=DIRECTION ( 'NONE',  ( 0.9999697198139515519, 0.000000000000000000, 0.007781995580013368816 ) ) ;
#12840=CARTESIAN_POINT ( 'NONE',  ( -17.93139508144814442, 0.000000000000000000, 13.85596890686001537 ) ) ;
#12841=DIRECTION ( 'NONE',  ( 0.007781995580012663651, 0.000000000000000000, -0.9999697198139515519 ) ) ;
#12842=VERTEX_POINT ( 'NONE', #10906 ) ;
#12843=ADVANCED_FACE ( 'NONE', ( #45529 ), #40742, .F. ) ;
#12844=VECTOR ( 'NONE', #46439, 1000.000000000000114 ) ;
#12845=CARTESIAN_POINT ( 'NONE',  ( -11.89954417724882774, 0.000000000000000000, 1.403813493000912294 ) ) ;
#12846=VECTOR ( 'NONE', #53428, 1000.000000000000227 ) ;
#12847=EDGE_CURVE ( 'NONE', #52707, #27319, #10067, .T. ) ;
#12848=DIRECTION ( 'NONE',  ( 0.000000000000000000, -0.000000000000000000, -1.000000000000000000 ) ) ;
#12849=CARTESIAN_POINT ( 'NONE',  ( -18.58795878855817207, 0.000000000000000000, 4.506425318625041143 ) ) ;
#12850=LINE ( 'NONE', #47490, #28602 ) ;
#12851=DIRECTION ( 'NONE',  ( 0.007781995580012662783, 0.000000000000000000, -0.9999697198139514409 ) ) ;
#12852=DIRECTION ( 'NONE',  ( 0.7660212471507180654, -0.6427876096865404731, 0.005961354470445141482 ) ) ;
#12853=EDGE_CURVE ( 'NONE', #3505, #25279, #971, .T. ) ;
#12854=CARTESIAN_POINT ( 'NONE',  ( -19.69569380384165669, -0.1191753592594177458, 14.58090286586150697 ) ) ;
#12855=VECTOR ( 'NONE', #51738, 1000.000000000000114 ) ;
#12856=ORIENTED_EDGE ( 'NONE', *, *, #9923, .F. ) ;
#12858=DIRECTION ( 'NONE',  ( 0.007781995580012663651, -3.146120232559066537E-19, -0.9999697198139514409 ) ) ;
#12859=LINE ( 'NONE', #51200, #27770 ) ;
#12860=EDGE_LOOP ( 'NONE', ( #14671, #10465, #18249 ) ) ;
#12861=CARTESIAN_POINT ( 'NONE',  ( -20.01569662516219239, -4.403642575758160760, 11.68383572719809216 ) ) ;
#12862=CARTESIAN_POINT ( 'NONE',  ( -13.62236162558936847, -0.1941918491731548790, 2.292021512081481305 ) ) ;
#12863=VERTEX_POINT ( 'NONE', #19135 ) ;
#12864=CARTESIAN_POINT ( 'NONE',  ( -16.33317936670417225, 0.000000000000000000, 13.31440848639340224 ) ) ;
#12865=CARTESIAN_POINT ( 'NONE',  ( -12.13851405436063047, 0.000000000000000000, 11.68505802764555135 ) ) ;
#12866=FACE_OUTER_BOUND ( 'NONE', #54438, .T. ) ;
#12867=VECTOR ( 'NONE', #44143, 1000.000000000000227 ) ;
#12869=ORIENTED_EDGE ( 'NONE', *, *, #14509, .T. ) ;
#12870=VERTEX_POINT ( 'NONE', #14060 ) ;
#12871=CARTESIAN_POINT ( 'NONE',  ( -16.81345671998191449, 0.000000000000000000, 3.412238694616132495 ) ) ;
#12872=LINE ( 'NONE', #26220, #5993 ) ;
#12873=PLANE ( 'NONE',  #33362 ) ;
#12874=DIRECTION ( 'NONE',  ( 0.000000000000000000, -0.000000000000000000, -1.000000000000000000 ) ) ;
#12875=LINE ( 'NONE', #8923, #6557 ) ;
#12876=FACE_OUTER_BOUND ( 'NONE', #40045, .T. ) ;
#12877=EDGE_CURVE ( 'NONE', #23301, #20373, #40166, .T. ) ;
#12878=VERTEX_POINT ( 'NONE', #35944 ) ;
#12879=DIRECTION ( 'NONE',  ( 0.000000000000000000, -0.000000000000000000, -1.000000000000000000 ) ) ;
#12880=DIRECTION ( 'NONE',  ( -0.005002170337468016433, -0.7660444431189770143, 0.6427681459581293666 ) ) ;
#12881=EDGE_LOOP ( 'NONE', ( #4567, #54110, #42295, #7108 ) ) ;
#12882=DIRECTION ( 'NONE',  ( 0.007781995580012663651, 0.000000000000000000, -0.9999697198139515519 ) ) ;
#12883=DIRECTION ( 'NONE',  ( -0.5449076811759708816, 0.6444004775717707689, 0.5364919789714475140 ) ) ;
#12884=CARTESIAN_POINT ( 'NONE',  ( -19.60834386242827776, 0.000000000000000000, 4.298478389818581213 ) ) ;
#12885=EDGE_CURVE ( 'NONE', #54227, #41918, #7021, .T. ) ;
#12886=EDGE_LOOP ( 'NONE', ( #37417, #3445, #2703, #39308 ) ) ;
#12887=VECTOR ( 'NONE', #42293, 1000.000000000000227 ) ;
#12888=VECTOR ( 'NONE', #11662, 999.9999999999998863 ) ;
#12889=LINE ( 'NONE', #21703, #1263 ) ;
#12890=ORIENTED_EDGE ( 'NONE', *, *, #31640, .T. ) ;
#12891=ADVANCED_FACE ( 'NONE', ( #27968 ), #36460, .F. ) ;
#12892=ORIENTED_EDGE ( 'NONE', *, *, #45533, .F. ) ;
#12893=ORIENTED_EDGE ( 'NONE', *, *, #32056, .F. ) ;
#12894=AXIS2_PLACEMENT_3D ( 'NONE', #35768, #18150, #40302 ) ;
#12895=ORIENTED_EDGE ( 'NONE', *, *, #51380, .F. ) ;
#12896=CARTESIAN_POINT ( 'NONE',  ( -13.19219159589095192, 0.000000000000000000, 1.963091937920801833 ) ) ;
#12897=ORIENTED_EDGE ( 'NONE', *, *, #1134, .F. ) ;
#12898=DIRECTION ( 'NONE',  ( -0.5364919789714478471, 0.6444004775717705469, -0.5449076811759709926 ) ) ;
#12899=EDGE_LOOP ( 'NONE', ( #37467, #45008, #8228, #10418 ) ) ;
#12900=FACE_OUTER_BOUND ( 'NONE', #38587, .T. ) ;
#12901=EDGE_CURVE ( 'NONE', #21477, #12052, #9814, .T. ) ;
#12902=ORIENTED_EDGE ( 'NONE', *, *, #35255, .T. ) ;
#12904=VECTOR ( 'NONE', #10756, 1000.000000000000227 ) ;
#12905=VERTEX_POINT ( 'NONE', #18889 ) ;
#12906=EDGE_CURVE ( 'NONE', #11836, #45158, #45820, .T. ) ;
#12907=CARTESIAN_POINT ( 'NONE',  ( -9.442067484779661513, -0.1191753592594197858, 10.59804618892231254 ) ) ;
#12908=LINE ( 'NONE', #4408, #4925 ) ;
#12909=CARTESIAN_POINT ( 'NONE',  ( -23.33693525117809386, 0.000000000000000000, 5.746789908705562944 ) ) ;
#12910=PLANE ( 'NONE',  #26004 ) ;
#12911=FACE_OUTER_BOUND ( 'NONE', #10221, .T. ) ;
#12912=ORIENTED_EDGE ( 'NONE', *, *, #55113, .F. ) ;
#12913=EDGE_CURVE ( 'NONE', #23729, #11761, #15433, .T. ) ;
#12914=ORIENTED_EDGE ( 'NONE', *, *, #44745, .T. ) ;
#12915=CARTESIAN_POINT ( 'NONE',  ( -14.39892221086183000, 0.000000000000000000, 3.600355174058808672 ) ) ;
#12916=DIRECTION ( 'NONE',  ( 0.5449076811759707706, 0.6444004775717708799, -0.5364919789714476250 ) ) ;
#12918=CARTESIAN_POINT ( 'NONE',  ( -15.03495456790438389, -0.1191753592594197858, 12.77051346725278158 ) ) ;
#12919=EDGE_CURVE ( 'NONE', #3230, #37945, #20557, .T. ) ;
#12920=LINE ( 'NONE', #21731, #45736 ) ;
#12921=DIRECTION ( 'NONE',  ( 0.000000000000000000, -0.000000000000000000, -1.000000000000000000 ) ) ;
#12922=FACE_OUTER_BOUND ( 'NONE', #11954, .T. ) ;
#12923=EDGE_LOOP ( 'NONE', ( #52677, #20716, #37591, #27093 ) ) ;
#12924=VECTOR ( 'NONE', #17408, 1000.000000000000227 ) ;
#12925=CARTESIAN_POINT ( 'NONE',  ( -19.60990026154428278, 0.000000000000000000, 4.498472333781370125 ) ) ;
#12926=CARTESIAN_POINT ( 'NONE',  ( -15.81738172854334934, 0.000000000000000000, 6.743979008779684037 ) ) ;
#12927=EDGE_LOOP ( 'NONE', ( #46191, #49951, #43598, #39911 ) ) ;
#12928=VECTOR ( 'NONE', #31175, 999.9999999999998863 ) ;
#12929=VECTOR ( 'NONE', #28410, 1000.000000000000114 ) ;
#12930=DIRECTION ( 'NONE',  ( -0.7660212471507179544, -0.6427876096865405842, -0.005961354470445141482 ) ) ;
#12931=PLANE ( 'NONE',  #40551 ) ;
#12932=LINE ( 'NONE', #51284, #52213 ) ;
#12933=FACE_OUTER_BOUND ( 'NONE', #39044, .T. ) ;
#12934=ORIENTED_EDGE ( 'NONE', *, *, #28869, .F. ) ;
#12935=AXIS2_PLACEMENT_3D ( 'NONE', #26567, #22332, #26865 ) ;
#12936=AXIS2_PLACEMENT_3D ( 'NONE', #7077, #55053, #28925 ) ;
#12937=ORIENTED_EDGE ( 'NONE', *, *, #37714, .F. ) ;
#12938=DIRECTION ( 'NONE',  ( 0.007781995580012663651, -3.146120232559066537E-19, -0.9999697198139514409 ) ) ;
#12939=DIRECTION ( 'NONE',  ( 0.007781995580012663651, 0.000000000000000000, -0.9999697198139515519 ) ) ;
#12940=DIRECTION ( 'NONE',  ( 0.000000000000000000, -1.000000000000000000, 0.000000000000000000 ) ) ;
#12941=DIRECTION ( 'NONE',  ( -0.005002170337468016433, -0.7660444431189770143, 0.6427681459581293666 ) ) ;
#12942=VECTOR ( 'NONE', #14037, 999.9999999999998863 ) ;
#12943=CARTESIAN_POINT ( 'NONE',  ( -14.94760462649100496, 0.000000000000000000, 2.488088991209854051 ) ) ;
#12944=EDGE_CURVE ( 'NONE', #41786, #1716, #6649, .T. ) ;
#12945=LINE ( 'NONE', #43052, #34606 ) ;
#12946=PLANE ( 'NONE',  #21145 ) ;
#12947=ORIENTED_EDGE ( 'NONE', *, *, #32980, .T. ) ;
#12948=DIRECTION ( 'NONE',  ( 0.9999697198139515519, 0.000000000000000000, 0.007781995580013368816 ) ) ;
#12949=CARTESIAN_POINT ( 'NONE',  ( -17.67437291679169320, 0.000000000000000000, 6.529521417744858169 ) ) ;
#12950=EDGE_CURVE ( 'NONE', #29873, #46828, #38135, .T. ) ;
#12951=EDGE_CURVE ( 'NONE', #34537, #35206, #42418, .T. ) ;
#12952=ORIENTED_EDGE ( 'NONE', *, *, #5787, .T. ) ;
#12953=DIRECTION ( 'NONE',  ( 0.5364919789714477361, 0.6444004775717706579, 0.5449076811759711036 ) ) ;
#12954=ORIENTED_EDGE ( 'NONE', *, *, #34145, .T. ) ;
#12955=CARTESIAN_POINT ( 'NONE',  ( -17.38641064682997595, 0.000000000000000000, 3.535098764555870243 ) ) ;
#12956=EDGE_CURVE ( 'NONE', #40957, #33373, #46658, .T. ) ;
#12957=VECTOR ( 'NONE', #34293, 1000.000000000000227 ) ;
#12958=EDGE_CURVE ( 'NONE', #41874, #35444, #12318, .T. ) ;
#12959=ADVANCED_FACE ( 'NONE', ( #11178 ), #37583, .F. ) ;
#12960=ORIENTED_EDGE ( 'NONE', *, *, #43699, .F. ) ;
#12961=AXIS2_PLACEMENT_3D ( 'NONE', #34389, #7997, #11684 ) ;
#12962=ORIENTED_EDGE ( 'NONE', *, *, #33353, .F. ) ;
#12963=ORIENTED_EDGE ( 'NONE', *, *, #331, .F. ) ;
#12964=VERTEX_POINT ( 'NONE', #37291 ) ;
#12966=ORIENTED_EDGE ( 'NONE', *, *, #38667, .T. ) ;
#12967=VECTOR ( 'NONE', #21338, 1000.000000000000227 ) ;
#12968=DIRECTION ( 'NONE',  ( -0.5364919789714478471, 0.6444004775717705469, -0.5449076811759709926 ) ) ;
#12969=LINE ( 'NONE', #26583, #54679 ) ;
#12970=DIRECTION ( 'NONE',  ( -0.005961354470445682716, -0.6427876096865404731, 0.7660212471507180654 ) ) ;
#12971=AXIS2_PLACEMENT_3D ( 'NONE', #9729, #22503, #51736 ) ;
#12972=VECTOR ( 'NONE', #10718, 1000.000000000000114 ) ;
#12973=ORIENTED_EDGE ( 'NONE', *, *, #21623, .T. ) ;
#12975=ADVANCED_FACE ( 'NONE', ( #33048 ), #50062, .F. ) ;
#12976=EDGE_LOOP ( 'NONE', ( #5557, #9875, #18120, #34310 ) ) ;
#12977=ORIENTED_EDGE ( 'NONE', *, *, #5821, .F. ) ;
#12978=EDGE_CURVE ( 'NONE', #45114, #18340, #54909, .T. ) ;
#12979=VECTOR ( 'NONE', #12953, 999.9999999999998863 ) ;
#12980=AXIS2_PLACEMENT_3D ( 'NONE', #51429, #30112, #17319 ) ;
#12981=PLANE ( 'NONE',  #44813 ) ;
#12982=EDGE_CURVE ( 'NONE', #14805, #37070, #55185, .T. ) ;
#12983=CARTESIAN_POINT ( 'NONE',  ( -23.33693525117809386, 0.000000000000000000, 5.746789908705562944 ) ) ;
#12984=ORIENTED_EDGE ( 'NONE', *, *, #36623, .T. ) ;
#12985=DIRECTION ( 'NONE',  ( 0.007781995580012662783, 0.000000000000000000, -0.9999697198139514409 ) ) ;
#12986=ORIENTED_EDGE ( 'NONE', *, *, #8540, .T. ) ;
#12988=DIRECTION ( 'NONE',  ( 0.5364919789714477361, 0.6444004775717706579, 0.5449076811759711036 ) ) ;
#12989=VECTOR ( 'NONE', #44286, 1000.000000000000000 ) ;
#12990=PLANE ( 'NONE',  #35706 ) ;
#12991=VECTOR ( 'NONE', #50738, 999.9999999999998863 ) ;
#12992=DIRECTION ( 'NONE',  ( -0.9999697198139514409, -0.000000000000000000, -0.007781995580013368816 ) ) ;
#12993=LINE ( 'NONE', #47638, #21350 ) ;
#12994=LINE ( 'NONE', #47639, #48310 ) ;
#12995=CARTESIAN_POINT ( 'NONE',  ( -17.85424848621750016, 0.000000000000000000, 3.942797095824502662 ) ) ;
#12996=CARTESIAN_POINT ( 'NONE',  ( -19.02484223489273063, 0.2864062442990042978, 4.062688683190644134 ) ) ;
#12997=DIRECTION ( 'NONE',  ( 0.007781995580012662783, 0.000000000000000000, -0.9999697198139514409 ) ) ;
#12999=DIRECTION ( 'NONE',  ( 0.5449076811759707706, 0.6444004775717708799, -0.5364919789714476250 ) ) ;
#13000=VECTOR ( 'NONE', #42089, 999.9999999999998863 ) ;
#13001=PLANE ( 'NONE',  #15627 ) ;
#13002=DIRECTION ( 'NONE',  ( -0.005961354470445682716, -0.6427876096865404731, 0.7660212471507180654 ) ) ;
#13003=CARTESIAN_POINT ( 'NONE',  ( -14.36939978893929570, 0.2864062442990022439, 2.932925422388083181 ) ) ;
#13004=VECTOR ( 'NONE', #54538, 999.9999999999998863 ) ;
#13005=CARTESIAN_POINT ( 'NONE',  ( -12.76779144812382327, 0.000000000000000000, 7.137043695297512258 ) ) ;
#13006=LINE ( 'NONE', #7926, #41308 ) ;
#13007=LINE ( 'NONE', #26620, #28670 ) ;
#13008=DIRECTION ( 'NONE',  ( -0.005961354470445682716, -0.6427876096865404731, 0.7660212471507180654 ) ) ;
#13010=ORIENTED_EDGE ( 'NONE', *, *, #24384, .F. ) ;
#13011=AXIS2_PLACEMENT_3D ( 'NONE', #42438, #3530, #21118 ) ;
#13012=PLANE ( 'NONE',  #10306 ) ;
#13013=DIRECTION ( 'NONE',  ( -0.5364919789714478471, 0.6444004775717705469, -0.5449076811759709926 ) ) ;
#13014=DIRECTION ( 'NONE',  ( 0.9999697198139515519, 0.000000000000000000, 0.007781995580013368816 ) ) ;
#13015=VECTOR ( 'NONE', #35916, 1000.000000000000114 ) ;
#13016=VECTOR ( 'NONE', #11472, 999.9999999999998863 ) ;
#13018=CARTESIAN_POINT ( 'NONE',  ( -14.59759850043533724, 0.000000000000000000, 3.429483015647829092 ) ) ;
#13019=DIRECTION ( 'NONE',  ( -0.9999697198139514409, -0.000000000000000000, -0.007781995580013368816 ) ) ;
#13020=LINE ( 'NONE', #39131, #54611 ) ;
#13021=AXIS2_PLACEMENT_3D ( 'NONE', #868, #35259, #13647 ) ;
#13022=PLANE ( 'NONE',  #33037 ) ;
#13023=EDGE_CURVE ( 'NONE', #48933, #9978, #33343, .T. ) ;
#13024=VECTOR ( 'NONE', #19502, 999.9999999999998863 ) ;
#13026=EDGE_LOOP ( 'NONE', ( #6926, #2681, #35342, #28596 ) ) ;
#13027=DIRECTION ( 'NONE',  ( 0.5364919789714477361, 0.6444004775717706579, 0.5449076811759711036 ) ) ;
#13028=EDGE_CURVE ( 'NONE', #29379, #32268, #7475, .T. ) ;
#13030=EDGE_CURVE ( 'NONE', #43836, #43824, #7210, .T. ) ;
#13031=ORIENTED_EDGE ( 'NONE', *, *, #48937, .F. ) ;
#13032=EDGE_CURVE ( 'NONE', #5134, #12666, #24508, .T. ) ;
#13033=VERTEX_POINT ( 'NONE', #33595 ) ;
#13034=ORIENTED_EDGE ( 'NONE', *, *, #24814, .F. ) ;
#13035=ORIENTED_EDGE ( 'NONE', *, *, #21749, .F. ) ;
#13036=AXIS2_PLACEMENT_3D ( 'NONE', #55783, #8939, #51784 ) ;
#13038=LINE ( 'NONE', #804, #19667 ) ;
#13039=DIRECTION ( 'NONE',  ( -0.5449076811759708816, 0.6444004775717707689, 0.5364919789714475140 ) ) ;
#13040=VECTOR ( 'NONE', #18989, 1000.000000000000227 ) ;
#13042=AXIS2_PLACEMENT_3D ( 'NONE', #43425, #35202, #34916 ) ;
#13043=EDGE_CURVE ( 'NONE', #55101, #31910, #50906, .T. ) ;
#13045=ORIENTED_EDGE ( 'NONE', *, *, #17869, .T. ) ;
#13046=EDGE_CURVE ( 'NONE', #33948, #1716, #38730, .T. ) ;
#13047=DIRECTION ( 'NONE',  ( 0.6427681459581294776, -0.7660444431189769032, 0.005002170337467562802 ) ) ;
#13048=LINE ( 'NONE', #34080, #6854 ) ;
#13049=ORIENTED_EDGE ( 'NONE', *, *, #25328, .T. ) ;
#13050=CARTESIAN_POINT ( 'NONE',  ( 2.072287782118878319, 0.000000000000000000, -2.950529333540147015 ) ) ;
#13051=VECTOR ( 'NONE', #13955, 999.9999999999998863 ) ;
#13052=ORIENTED_EDGE ( 'NONE', *, *, #7928, .F. ) ;
#13053=EDGE_CURVE ( 'NONE', #34537, #41034, #38422, .T. ) ;
#13054=LINE ( 'NONE', #51407, #28245 ) ;
#13055=EDGE_CURVE ( 'NONE', #34036, #52834, #40315, .T. ) ;
#13056=VECTOR ( 'NONE', #27415, 1000.000000000000227 ) ;
#13057=CARTESIAN_POINT ( 'NONE',  ( -16.36775718102074606, -0.6798977022406563764, 4.155552431687926429 ) ) ;
#13058=VECTOR ( 'NONE', #2468, 999.9999999999998863 ) ;
#13059=EDGE_LOOP ( 'NONE', ( #10316, #42258, #32563, #31151 ) ) ;
#13060=FACE_OUTER_BOUND ( 'NONE', #37311, .T. ) ;
#13061=LINE ( 'NONE', #47406, #10268 ) ;
#13062=CARTESIAN_POINT ( 'NONE',  ( -11.61840533594187974, 0.000000000000000000, 4.560663995145184835 ) ) ;
#13063=DIRECTION ( 'NONE',  ( 0.9999697198139515519, 0.000000000000000000, 0.007781995580013368816 ) ) ;
#13065=DIRECTION ( 'NONE',  ( 0.7660212471507180654, -0.6427876096865404731, 0.005961354470445141482 ) ) ;
#13066=PLANE ( 'NONE',  #48668 ) ;
#13067=DIRECTION ( 'NONE',  ( 0.005961354470445682716, -0.6427876096865404731, -0.7660212471507180654 ) ) ;
#13068=DIRECTION ( 'NONE',  ( 0.007781995580012663651, 0.000000000000000000, -0.9999697198139515519 ) ) ;
#13069=LINE ( 'NONE', #8238, #10503 ) ;
#13070=CARTESIAN_POINT ( 'NONE',  ( -3.033487535867088081, 3.746215373297818729, -2.040063999062676103 ) ) ;
#13071=DIRECTION ( 'NONE',  ( 0.9999697198139515519, 0.000000000000000000, 0.007781995580013368816 ) ) ;
#13072=FACE_OUTER_BOUND ( 'NONE', #48907, .T. ) ;
#13073=LINE ( 'NONE', #4548, #44952 ) ;
#13074=VECTOR ( 'NONE', #6078, 1000.000000000000227 ) ;
#13075=ORIENTED_EDGE ( 'NONE', *, *, #28923, .T. ) ;
#13076=DIRECTION ( 'NONE',  ( 0.9999697198139515519, 0.000000000000000000, 0.007781995580013368816 ) ) ;
#13077=ORIENTED_EDGE ( 'NONE', *, *, #35316, .T. ) ;
#13078=CARTESIAN_POINT ( 'NONE',  ( -20.54049170961573267, 0.000000000000000000, 4.660556269540326646 ) ) ;
#13079=DIRECTION ( 'NONE',  ( 0.5364919789714477361, 0.6444004775717706579, 0.5449076811759711036 ) ) ;
#13080=VECTOR ( 'NONE', #24494, 1000.000000000000114 ) ;
#13081=DIRECTION ( 'NONE',  ( 0.9999697198139515519, 0.000000000000000000, 0.007781995580013368816 ) ) ;
#13082=AXIS2_PLACEMENT_3D ( 'NONE', #31765, #32341, #19244 ) ;
#13083=CARTESIAN_POINT ( 'NONE',  ( -19.60834386242827776, 0.000000000000000000, 4.298478389818581213 ) ) ;
#13084=LINE ( 'NONE', #48855, #22037 ) ;
#13085=ORIENTED_EDGE ( 'NONE', *, *, #15330, .T. ) ;
#13086=VERTEX_POINT ( 'NONE', #27246 ) ;
#13087=CARTESIAN_POINT ( 'NONE',  ( -22.40634380310664397, 0.000000000000000000, 5.584705972946605534 ) ) ;
#13088=VECTOR ( 'NONE', #50739, 1000.000000000000227 ) ;
#13089=CARTESIAN_POINT ( 'NONE',  ( -17.36532418587302473, -0.1191753592594177458, 13.67570816655714516 ) ) ;
#13090=EDGE_LOOP ( 'NONE', ( #31639, #22040, #46019, #17162 ) ) ;
#13091=AXIS2_PLACEMENT_3D ( 'NONE', #4057, #8047, #21079 ) ;
#13092=FACE_OUTER_BOUND ( 'NONE', #23697, .T. ) ;
#13093=ADVANCED_FACE ( 'NONE', ( #52796 ), #53107, .F. ) ;
#13094=ORIENTED_EDGE ( 'NONE', *, *, #15076, .F. ) ;
#13095=PLANE ( 'NONE',  #44022 ) ;
#13096=VERTEX_POINT ( 'NONE', #48847 ) ;
#13097=CARTESIAN_POINT ( 'NONE',  ( -15.86710544311044302, 0.000000000000000000, 13.13336954653252953 ) ) ;
#13098=EDGE_CURVE ( 'NONE', #51326, #19370, #18756, .T. ) ;
#13100=VECTOR ( 'NONE', #42208, 999.9999999999998863 ) ;
#13101=EDGE_LOOP ( 'NONE', ( #38439, #37907, #32058, #46340 ) ) ;
#13102=VECTOR ( 'NONE', #30060, 1000.000000000000227 ) ;
#13103=ORIENTED_EDGE ( 'NONE', *, *, #734, .T. ) ;
#13104=ORIENTED_EDGE ( 'NONE', *, *, #1654, .T. ) ;
#13105=CARTESIAN_POINT ( 'NONE',  ( -15.07947971830811795, 0.000000000000000000, 5.641725323426407535 ) ) ;
#13106=DIRECTION ( 'NONE',  ( 0.9999697198139515519, 0.000000000000000000, 0.007781995580013368816 ) ) ;
#13107=LINE ( 'NONE', #30438, #54735 ) ;
#13108=DIRECTION ( 'NONE',  ( -0.5364919789714478471, 0.6444004775717705469, -0.5449076811759709926 ) ) ;
#13109=VERTEX_POINT ( 'NONE', #29915 ) ;
#13110=ORIENTED_EDGE ( 'NONE', *, *, #27505, .F. ) ;
#13111=AXIS2_PLACEMENT_3D ( 'NONE', #6282, #32661, #49963 ) ;
#13112=ORIENTED_EDGE ( 'NONE', *, *, #42814, .F. ) ;
#13113=CARTESIAN_POINT ( 'NONE',  ( -10.70924991679669169, 0.000000000000000000, 7.153063741485553351 ) ) ;
#13114=AXIS2_PLACEMENT_3D ( 'NONE', #16823, #34417, #51720 ) ;
#13115=ORIENTED_EDGE ( 'NONE', *, *, #30895, .F. ) ;
#13116=DIRECTION ( 'NONE',  ( 0.7660212471507180654, -0.6427876096865404731, 0.005961354470445141482 ) ) ;
#13117=VERTEX_POINT ( 'NONE', #8060 ) ;
#13118=VECTOR ( 'NONE', #41741, 1000.000000000000227 ) ;
#13119=DIRECTION ( 'NONE',  ( 0.000000000000000000, -0.000000000000000000, -1.000000000000000000 ) ) ;
#13120=DIRECTION ( 'NONE',  ( 0.005002170337468016433, -0.7660444431189770143, -0.6427681459581293666 ) ) ;
#13121=ORIENTED_EDGE ( 'NONE', *, *, #16828, .T. ) ;
#13122=CARTESIAN_POINT ( 'NONE',  ( -17.22069023688172607, -3.917936722690662066, 3.445419328183913610 ) ) ;
#13123=ORIENTED_EDGE ( 'NONE', *, *, #42005, .F. ) ;
#13124=EDGE_CURVE ( 'NONE', #14373, #7205, #5136, .T. ) ;
#13125=FACE_OUTER_BOUND ( 'NONE', #22944, .T. ) ;
#13126=VECTOR ( 'NONE', #26012, 1000.000000000000227 ) ;
#13127=EDGE_LOOP ( 'NONE', ( #1183, #41249, #46616, #55562 ) ) ;
#13128=ADVANCED_FACE ( 'NONE', ( #36082 ), #53384, .F. ) ;
#13129=DIRECTION ( 'NONE',  ( -0.9999697198139514409, -0.000000000000000000, -0.007781995580013368816 ) ) ;
#13130=DIRECTION ( 'NONE',  ( 0.007781995580012663651, -3.146120232559066537E-19, -0.9999697198139514409 ) ) ;
#13131=VECTOR ( 'NONE', #35391, 1000.000000000000114 ) ;
#13132=CARTESIAN_POINT ( 'NONE',  ( -15.48567762416715077, -0.1941918491731566832, 2.890288465539208929 ) ) ;
#13133=EDGE_CURVE ( 'NONE', #31427, #40934, #8319, .T. ) ;
#13135=AXIS2_PLACEMENT_3D ( 'NONE', #44076, #31847, #23347 ) ;
#13136=LINE ( 'NONE', #9140, #1152 ) ;
#13137=LINE ( 'NONE', #30472, #5602 ) ;
#13138=ADVANCED_FACE ( 'NONE', ( #18447 ), #1111, .F. ) ;
#13139=DIRECTION ( 'NONE',  ( -0.005961354470445682716, -0.6427876096865404731, 0.7660212471507180654 ) ) ;
#13140=CARTESIAN_POINT ( 'NONE',  ( -11.30636317915456779, -0.1191753592594197858, 11.32220194836580340 ) ) ;
#13141=DIRECTION ( 'NONE',  ( -0.5449076811759708816, 0.6444004775717707689, 0.5364919789714475140 ) ) ;
#13142=CARTESIAN_POINT ( 'NONE',  ( -19.60990026154428278, 0.000000000000000000, 4.498472333781370125 ) ) ;
#13143=VECTOR ( 'NONE', #20830, 999.9999999999998863 ) ;
#13144=AXIS2_PLACEMENT_3D ( 'NONE', #44161, #35932, #10656 ) ;
#13145=CARTESIAN_POINT ( 'NONE',  ( -13.12590506641494592, -0.1191753592594172878, 6.295589604590576371 ) ) ;
#13146=ORIENTED_EDGE ( 'NONE', *, *, #25672, .F. ) ;
#13148=CARTESIAN_POINT ( 'NONE',  ( -14.62346498198288280, 0.000000000000000000, 6.753270344967709171 ) ) ;
#13149=LINE ( 'NONE', #47801, #6045 ) ;
#13150=ORIENTED_EDGE ( 'NONE', *, *, #51623, .T. ) ;
#13151=DIRECTION ( 'NONE',  ( -0.7660212471507179544, -0.6427876096865405842, -0.005961354470445141482 ) ) ;
#13152=EDGE_LOOP ( 'NONE', ( #4729, #11468, #34501, #53950 ) ) ;
#13153=CARTESIAN_POINT ( 'NONE',  ( -21.12243245839617956, -5.698858183938163791, 14.23939898133697568 ) ) ;
#13154=DIRECTION ( 'NONE',  ( 0.5364919789714477361, 0.6444004775717706579, 0.5449076811759711036 ) ) ;
#13155=FACE_OUTER_BOUND ( 'NONE', #47156, .T. ) ;
#13157=AXIS2_PLACEMENT_3D ( 'NONE', #21091, #42965, #40025 ) ;
#13158=ORIENTED_EDGE ( 'NONE', *, *, #44957, .F. ) ;
#13159=VERTEX_POINT ( 'NONE', #21400 ) ;
#13161=CARTESIAN_POINT ( 'NONE',  ( -19.60912206198628027, -0.1191753592594197858, 4.398475361799976113 ) ) ;
#13162=DIRECTION ( 'NONE',  ( 0.5364919789714477361, 0.6444004775717706579, 0.5449076811759711036 ) ) ;
#13163=LINE ( 'NONE', #35042, #1488 ) ;
#13164=EDGE_CURVE ( 'NONE', #55170, #55582, #9676, .T. ) ;
#13165=AXIS2_PLACEMENT_3D ( 'NONE', #10900, #37879, #24505 ) ;
#13166=LINE ( 'NONE', #43532, #9386 ) ;
#13167=DIRECTION ( 'NONE',  ( -0.005961354470445682716, -0.6427876096865404731, 0.7660212471507180654 ) ) ;
#13168=DIRECTION ( 'NONE',  ( 0.6427681459581294776, -0.7660444431189769032, 0.005002170337467562802 ) ) ;
#13169=AXIS2_PLACEMENT_3D ( 'NONE', #822, #22689, #43989 ) ;
#13170=ORIENTED_EDGE ( 'NONE', *, *, #21204, .F. ) ;
#13171=DIRECTION ( 'NONE',  ( 0.007781995580012663651, -3.146120232559066537E-19, -0.9999697198139514409 ) ) ;
#13172=ADVANCED_FACE ( 'NONE', ( #25371 ), #22711, .F. ) ;
#13174=VECTOR ( 'NONE', #31894, 1000.000000000000227 ) ;
#13175=ORIENTED_EDGE ( 'NONE', *, *, #29640, .F. ) ;
#13176=VECTOR ( 'NONE', #55674, 999.9999999999998863 ) ;
#13177=CARTESIAN_POINT ( 'NONE',  ( -18.67775241435682432, 0.000000000000000000, 4.136394454059623804 ) ) ;
#13178=DIRECTION ( 'NONE',  ( 0.007781995580012663651, 0.000000000000000000, -0.9999697198139515519 ) ) ;
#13179=CARTESIAN_POINT ( 'NONE',  ( -14.01545677930355183, 0.000000000000000000, 2.126011111488108174 ) ) ;
#13180=AXIS2_PLACEMENT_3D ( 'NONE', #49921, #28929, #27830 ) ;
#13181=EDGE_LOOP ( 'NONE', ( #51915, #23721, #31115, #21886 ) ) ;
#13182=DIRECTION ( 'NONE',  ( 0.005961354470445682716, -0.6427876096865404731, -0.7660212471507180654 ) ) ;
#13183=ORIENTED_EDGE ( 'NONE', *, *, #7365, .F. ) ;
#13184=EDGE_CURVE ( 'NONE', #54636, #49471, #4071, .T. ) ;
#13185=AXIS2_PLACEMENT_3D ( 'NONE', #32391, #5685, #23009 ) ;
#13186=ORIENTED_EDGE ( 'NONE', *, *, #48281, .F. ) ;
#13187=VECTOR ( 'NONE', #45812, 1000.000000000000000 ) ;
#13188=VERTEX_POINT ( 'NONE', #5669 ) ;
#13189=ORIENTED_EDGE ( 'NONE', *, *, #2491, .T. ) ;
#13190=LINE ( 'NONE', #9193, #24824 ) ;
#13191=ORIENTED_EDGE ( 'NONE', *, *, #41489, .T. ) ;
#13192=DIRECTION ( 'NONE',  ( 0.007781995580012663651, -3.146120232559066537E-19, -0.9999697198139514409 ) ) ;
#13194=LINE ( 'NONE', #4662, #2321 ) ;
#13195=EDGE_LOOP ( 'NONE', ( #26833, #11572, #22367, #5311 ) ) ;
#13196=CARTESIAN_POINT ( 'NONE',  ( -20.24133259733970291, -5.213152330870663320, 13.10002382117402320 ) ) ;
#13197=ORIENTED_EDGE ( 'NONE', *, *, #9774, .T. ) ;
#13198=VECTOR ( 'NONE', #25720, 1000.000000000000227 ) ;
#13199=CARTESIAN_POINT ( 'NONE',  ( -14.06954912762353338, -0.1191753592594177180, 8.134906297343379222 ) ) ;
#13200=AXIS2_PLACEMENT_3D ( 'NONE', #34654, #12541, #4308 ) ;
#13201=CARTESIAN_POINT ( 'NONE',  ( -10.47421230394850866, 0.000000000000000000, 10.95934586908605723 ) ) ;
#13202=DIRECTION ( 'NONE',  ( -0.005002170337468016433, -0.7660444431189770143, 0.6427681459581293666 ) ) ;
#13203=LINE ( 'NONE', #39313, #28704 ) ;
#13204=DIRECTION ( 'NONE',  ( 0.5364919789714477361, 0.6444004775717706579, 0.5449076811759711036 ) ) ;
#13205=VECTOR ( 'NONE', #50132, 1000.000000000000114 ) ;
#13206=ORIENTED_EDGE ( 'NONE', *, *, #27272, .F. ) ;
#13207=ORIENTED_EDGE ( 'NONE', *, *, #26735, .T. ) ;
#13208=LINE ( 'NONE', #38779, #33132 ) ;
#13209=EDGE_CURVE ( 'NONE', #8976, #5703, #26690, .T. ) ;
#13210=FACE_OUTER_BOUND ( 'NONE', #53415, .T. ) ;
#13211=VECTOR ( 'NONE', #23479, 1000.000000000000114 ) ;
#13212=DIRECTION ( 'NONE',  ( -0.7660212471507179544, -0.6427876096865405842, -0.005961354470445141482 ) ) ;
#13213=VECTOR ( 'NONE', #8884, 999.9999999999998863 ) ;
#13214=AXIS2_PLACEMENT_3D ( 'NONE', #16472, #37217, #54521 ) ;
#13215=LINE ( 'NONE', #962, #21264 ) ;
#13216=DIRECTION ( 'NONE',  ( 0.000000000000000000, -1.000000000000000000, 0.000000000000000000 ) ) ;
#13217=LINE ( 'NONE', #35096, #29588 ) ;
#13218=ORIENTED_EDGE ( 'NONE', *, *, #6742, .T. ) ;
#13219=LINE ( 'NONE', #29970, #12063 ) ;
#13221=ORIENTED_EDGE ( 'NONE', *, *, #48203, .F. ) ;
#13222=EDGE_CURVE ( 'NONE', #53048, #50265, #51755, .T. ) ;
#13223=DIRECTION ( 'NONE',  ( -0.9999697198139514409, -0.000000000000000000, -0.007781995580013368816 ) ) ;
#13224=DIRECTION ( 'NONE',  ( -0.005961354470445682716, -0.6427876096865404731, 0.7660212471507180654 ) ) ;
#13225=VECTOR ( 'NONE', #44971, 999.9999999999998863 ) ;
#13226=VECTOR ( 'NONE', #21104, 999.9999999999998863 ) ;
#13227=CARTESIAN_POINT ( 'NONE',  ( -17.88586307477561022, 0.000000000000000000, 8.005203831659914115 ) ) ;
#13228=ADVANCED_FACE ( 'NONE', ( #35783 ), #51505, .F. ) ;
#13229=EDGE_CURVE ( 'NONE', #13159, #11166, #36332, .T. ) ;
#13231=VECTOR ( 'NONE', #39359, 999.9999999999998863 ) ;
#13232=PLANE ( 'NONE',  #23808 ) ;
#13233=ORIENTED_EDGE ( 'NONE', *, *, #40064, .T. ) ;
#13234=AXIS2_PLACEMENT_3D ( 'NONE', #4763, #30332, #52187 ) ;
#13235=ORIENTED_EDGE ( 'NONE', *, *, #7038, .T. ) ;
#13236=LINE ( 'NONE', #30570, #28491 ) ;
#13237=PLANE ( 'NONE',  #32211 ) ;
#13238=CARTESIAN_POINT ( 'NONE',  ( -18.49821513591315991, 2.391131607591507446, 7.990910409668134484 ) ) ;
#13239=EDGE_CURVE ( 'NONE', #2673, #9548, #11326, .T. ) ;
#13240=CARTESIAN_POINT ( 'NONE',  ( -21.82894433340611684, -4.889348428825662118, 13.18528876708279185 ) ) ;
#13241=ADVANCED_FACE ( 'NONE', ( #31795 ), #45676, .F. ) ;
#13243=FACE_OUTER_BOUND ( 'NONE', #660, .T. ) ;
#13244=CARTESIAN_POINT ( 'NONE',  ( 2.072287782118878319, 0.000000000000000000, -2.950529333540147015 ) ) ;
#13245=EDGE_CURVE ( 'NONE', #45223, #5769, #19013, .T. ) ;
#13246=VERTEX_POINT ( 'NONE', #24381 ) ;
#13247=AXIS2_PLACEMENT_3D ( 'NONE', #38999, #16869, #5215 ) ;
#13248=CARTESIAN_POINT ( 'NONE',  ( -23.33693525117809386, 0.000000000000000000, 5.746789908705562944 ) ) ;
#13249=CARTESIAN_POINT ( 'NONE',  ( -20.70076447251854290, -0.8417996532631553119, 6.104348297203140206 ) ) ;
#13250=EDGE_LOOP ( 'NONE', ( #7397, #42150, #10016, #8843 ) ) ;
#13251=PLANE ( 'NONE',  #41017 ) ;
#13253=CARTESIAN_POINT ( 'NONE',  ( -12.93745269883482152, 0.000000000000000000, 8.243719561634259563 ) ) ;
#13254=AXIS2_PLACEMENT_3D ( 'NONE', #25704, #42186, #24864 ) ;
#13255=CARTESIAN_POINT ( 'NONE',  ( -13.74730076765101217, 2.876837460659009693, 1.930064033053078498 ) ) ;
#13256=ADVANCED_FACE ( 'NONE', ( #54214 ), #27838, .F. ) ;
#13257=EDGE_LOOP ( 'NONE', ( #27354, #38298, #21998, #32918 ) ) ;
#13258=VECTOR ( 'NONE', #20746, 999.9999999999998863 ) ;
#13259=ORIENTED_EDGE ( 'NONE', *, *, #22066, .F. ) ;
#13260=EDGE_CURVE ( 'NONE', #485, #2545, #28089, .T. ) ;
#13261=ORIENTED_EDGE ( 'NONE', *, *, #28161, .F. ) ;
#13262=AXIS2_PLACEMENT_3D ( 'NONE', #46496, #33195, #33461 ) ;
#13263=ORIENTED_EDGE ( 'NONE', *, *, #36947, .F. ) ;
#13264=AXIS2_PLACEMENT_3D ( 'NONE', #15993, #2895, #20223 ) ;
#13265=EDGE_LOOP ( 'NONE', ( #8614, #18476, #43568, #50333 ) ) ;
#13266=VERTEX_POINT ( 'NONE', #32623 ) ;
#13267=DIRECTION ( 'NONE',  ( -0.5449076811759708816, 0.6444004775717707689, 0.5364919789714475140 ) ) ;
#13268=CARTESIAN_POINT ( 'NONE',  ( -21.47419595591918906, 0.000000000000000000, 5.222628093224860102 ) ) ;
#13270=VECTOR ( 'NONE', #46409, 999.9999999999998863 ) ;
#13271=VECTOR ( 'NONE', #1077, 1000.000000000000227 ) ;
#13272=VERTEX_POINT ( 'NONE', #23817 ) ;
#13273=CARTESIAN_POINT ( 'NONE',  ( -17.74482636761137044, -0.1191753592594197858, 3.674319602356483916 ) ) ;
#13274=ORIENTED_EDGE ( 'NONE', *, *, #30573, .F. ) ;
#13275=ORIENTED_EDGE ( 'NONE', *, *, #29654, .T. ) ;
#13276=AXIS2_PLACEMENT_3D ( 'NONE', #11958, #29289, #46608 ) ;
#13277=VECTOR ( 'NONE', #42673, 999.9999999999998863 ) ;
#13278=DIRECTION ( 'NONE',  ( 0.000000000000000000, -0.000000000000000000, -1.000000000000000000 ) ) ;
#13279=PLANE ( 'NONE',  #18539 ) ;
#13281=VERTEX_POINT ( 'NONE', #2776 ) ;
#13282=FACE_OUTER_BOUND ( 'NONE', #18014, .T. ) ;
#13283=EDGE_LOOP ( 'NONE', ( #52045, #10523, #31813, #22614, #25904 ) ) ;
#13284=CARTESIAN_POINT ( 'NONE',  ( -13.89904558389786438, -0.5179957512181551094, 2.930912325616202629 ) ) ;
#13285=ADVANCED_FACE ( 'NONE', ( #45395 ), #23291, .F. ) ;
#13286=CARTESIAN_POINT ( 'NONE',  ( -27.99923088623136636, 0.000000000000000000, 7.757173251277078130 ) ) ;
#13289=CARTESIAN_POINT ( 'NONE',  ( -18.79501849392080359, 0.000000000000000000, 5.412804085319542047 ) ) ;
#13290=DIRECTION ( 'NONE',  ( -0.005961354470445682716, -0.6427876096865404731, 0.7660212471507180654 ) ) ;
#13291=LINE ( 'NONE', #39106, #9481 ) ;
#13292=PLANE ( 'NONE',  #18462 ) ;
#13293=CARTESIAN_POINT ( 'NONE',  ( -16.01162756549557287, 0.000000000000000000, 6.003803203148152967 ) ) ;
#13294=ORIENTED_EDGE ( 'NONE', *, *, #13425, .F. ) ;
#13295=DIRECTION ( 'NONE',  ( 0.000000000000000000, -0.000000000000000000, -1.000000000000000000 ) ) ;
#13296=PRODUCT_DEFINITION_SHAPE ( 'NONE', 'NONE',  #27394 ) ;
#13297=VECTOR ( 'NONE', #20169, 999.9999999999998863 ) ;
#13298=EDGE_CURVE ( 'NONE', #34545, #55928, #41148, .T. ) ;
#13299=EDGE_CURVE ( 'NONE', #24514, #43824, #49927, .T. ) ;
#13300=PLANE ( 'NONE',  #32865 ) ;
#13301=DIRECTION ( 'NONE',  ( 0.005002170337468016433, -0.7660444431189770143, -0.6427681459581293666 ) ) ;
#13303=CARTESIAN_POINT ( 'NONE',  ( -12.09741250030938176, 0.000000000000000000, 6.403596599665996258 ) ) ;
#13305=CARTESIAN_POINT ( 'NONE',  ( -17.26532721389163072, 0.000000000000000000, 13.67648636611514590 ) ) ;
#13306=ADVANCED_FACE ( 'NONE', ( #41444 ), #37431, .F. ) ;
#13308=VECTOR ( 'NONE', #49616, 999.9999999999998863 ) ;
#13309=CARTESIAN_POINT ( 'NONE',  ( -17.80101456987863173, -0.1191753592594181482, 9.952527519488127083 ) ) ;
#13311=DIRECTION ( 'NONE',  ( -0.5364919789714478471, 0.6444004775717705469, -0.5449076811759709926 ) ) ;
#13312=LINE ( 'NONE', #17852, #27669 ) ;
#13313=CARTESIAN_POINT ( 'NONE',  ( -25.20123094555300369, 0.000000000000000000, 6.470945668149052032 ) ) ;
#13314=VECTOR ( 'NONE', #51800, 1000.000000000000227 ) ;
#13315=CARTESIAN_POINT ( 'NONE',  ( -15.30390940309393599, -4.889348428825662118, 10.65074360903057382 ) ) ;
#13316=EDGE_CURVE ( 'NONE', #52307, #5827, #28658, .T. ) ;
#13317=CARTESIAN_POINT ( 'NONE',  ( -11.20636620717317378, 0.000000000000000000, 11.32298014792380414 ) ) ;
#13318=DIRECTION ( 'NONE',  ( -0.005002170337468016433, -0.7660444431189770143, 0.6427681459581293666 ) ) ;
#13319=DIRECTION ( 'NONE',  ( 0.000000000000000000, -1.000000000000000000, 0.000000000000000000 ) ) ;
#13320=AXIS2_PLACEMENT_3D ( 'NONE', #13334, #47956, #52751 ) ;
#13321=EDGE_CURVE ( 'NONE', #7193, #21470, #14748, .T. ) ;
#13322=VECTOR ( 'NONE', #46044, 999.9999999999998863 ) ;
#13323=LINE ( 'NONE', #52207, #4060 ) ;
#13324=DIRECTION ( 'NONE',  ( -0.6427681459581293666, -0.7660444431189770143, -0.005002170337467561935 ) ) ;
#13326=CARTESIAN_POINT ( 'NONE',  ( -14.09440035361675747, -4.079838673713161334, 2.225896648385081278 ) ) ;
#13327=ADVANCED_FACE ( 'NONE', ( #24115 ), #40613, .F. ) ;
#13329=AXIS2_PLACEMENT_3D ( 'NONE', #34157, #4336, #16517 ) ;
#13330=ORIENTED_EDGE ( 'NONE', *, *, #12919, .F. ) ;
#13331=VERTEX_POINT ( 'NONE', #45977 ) ;
#13332=ORIENTED_EDGE ( 'NONE', *, *, #42834, .T. ) ;
#13333=ORIENTED_EDGE ( 'NONE', *, *, #10407, .F. ) ;
#13334=CARTESIAN_POINT ( 'NONE',  ( 2.072287782118878319, 0.000000000000000000, -2.950529333540147015 ) ) ;
#13335=LINE ( 'NONE', #30655, #17626 ) ;
#13336=ORIENTED_EDGE ( 'NONE', *, *, #20054, .F. ) ;
#13337=VECTOR ( 'NONE', #40761, 1000.000000000000227 ) ;
#13338=ORIENTED_EDGE ( 'NONE', *, *, #31131, .T. ) ;
#13339=VECTOR ( 'NONE', #43036, 1000.000000000000114 ) ;
#13340=LINE ( 'NONE', #22424, #379 ) ;
#13341=VERTEX_POINT ( 'NONE', #49395 ) ;
#13343=CARTESIAN_POINT ( 'NONE',  ( -14.20280369269832832, 0.000000000000000000, 12.40765738797303719 ) ) ;
#13344=ORIENTED_EDGE ( 'NONE', *, *, #24733, .T. ) ;
#13345=FACE_OUTER_BOUND ( 'NONE', #46642, .T. ) ;
#13346=EDGE_CURVE ( 'NONE', #9458, #6017, #19276, .T. ) ;
#13347=ORIENTED_EDGE ( 'NONE', *, *, #10381, .F. ) ;
#13348=AXIS2_PLACEMENT_3D ( 'NONE', #9652, #14459, #31777 ) ;
#13349=DIRECTION ( 'NONE',  ( 0.005961354470445682716, -0.6427876096865404731, -0.7660212471507180654 ) ) ;
#13350=EDGE_CURVE ( 'NONE', #55970, #49405, #1946, .T. ) ;
#13351=CARTESIAN_POINT ( 'NONE',  ( -2.881839257824877265, -5.376589517215482950, -2.098969340251471305 ) ) ;
#13352=AXIS2_PLACEMENT_3D ( 'NONE', #46296, #54833, #28998 ) ;
#13353=EDGE_LOOP ( 'NONE', ( #37000, #12480, #18287, #3111, #52691 ) ) ;
#13354=CARTESIAN_POINT ( 'NONE',  ( -13.47695292330622507, 0.000000000000000000, 4.546200348073146991 ) ) ;
#13355=DIRECTION ( 'NONE',  ( -0.5449076811759708816, 0.6444004775717707689, 0.5364919789714475140 ) ) ;
#13356=LINE ( 'NONE', #1387, #25782 ) ;
#13357=EDGE_CURVE ( 'NONE', #49206, #6706, #49685, .T. ) ;
#13358=ORIENTED_EDGE ( 'NONE', *, *, #53580, .T. ) ;
#13359=CARTESIAN_POINT ( 'NONE',  ( -19.15687783499660313, -0.6798977022406558213, 4.300810742247143104 ) ) ;
#13360=EDGE_LOOP ( 'NONE', ( #6328, #19020, #2247, #40397 ) ) ;
#13361=EDGE_CURVE ( 'NONE', #55490, #48977, #38275, .T. ) ;
#13362=EDGE_CURVE ( 'NONE', #26758, #17816, #11869, .T. ) ;
#13363=EDGE_CURVE ( 'NONE', #55993, #48862, #33735, .T. ) ;
#13364=CARTESIAN_POINT ( 'NONE',  ( -11.67244013076689946, 0.000000000000000000, 11.50401908778467863 ) ) ;
#13365=PLANE ( 'NONE',  #18765 ) ;
#13367=LINE ( 'NONE', #575, #46811 ) ;
#13368=DIRECTION ( 'NONE',  ( 0.6427681459581294776, -0.7660444431189769032, 0.005002170337467562802 ) ) ;
#13369=ADVANCED_FACE ( 'NONE', ( #3920 ), #55598, .F. ) ;
#13370=FACE_OUTER_BOUND ( 'NONE', #29421, .T. ) ;
#13371=FACE_OUTER_BOUND ( 'NONE', #33122, .T. ) ;
#13372=DIRECTION ( 'NONE',  ( 0.000000000000000000, -1.000000000000000000, 0.000000000000000000 ) ) ;
#13373=DIRECTION ( 'NONE',  ( 0.000000000000000000, 0.000000000000000000, 1.000000000000000000 ) ) ;
#13374=DIRECTION ( 'NONE',  ( 0.007781995580012662783, 0.000000000000000000, -0.9999697198139514409 ) ) ;
#13375=ORIENTED_EDGE ( 'NONE', *, *, #44348, .T. ) ;
#13376=DIRECTION ( 'NONE',  ( 0.005961354470445682716, -0.6427876096865404731, -0.7660212471507180654 ) ) ;
#13377=DIRECTION ( 'NONE',  ( 0.9999697198139515519, 0.000000000000000000, 0.007781995580013368816 ) ) ;
#13378=CARTESIAN_POINT ( 'NONE',  ( -22.40478740399063895, 0.000000000000000000, 5.384712028983816623 ) ) ;
#13379=DIRECTION ( 'NONE',  ( -0.5364919789714478471, 0.6444004775717705469, -0.5449076811759709926 ) ) ;
#13380=EDGE_CURVE ( 'NONE', #26525, #41032, #12471, .T. ) ;
#13381=CARTESIAN_POINT ( 'NONE',  ( -29.86352658060627618, 0.000000000000000000, 8.481329010720569883 ) ) ;
#13382=DIRECTION ( 'NONE',  ( -0.7660212471507179544, -0.6427876096865405842, -0.005961354470445141482 ) ) ;
#13383=VERTEX_POINT ( 'NONE', #47357 ) ;
#13384=EDGE_CURVE ( 'NONE', #54774, #18119, #20401, .T. ) ;
#13385=VECTOR ( 'NONE', #10671, 1000.000000000000227 ) ;
#13386=ORIENTED_EDGE ( 'NONE', *, *, #4207, .F. ) ;
#13387=EDGE_CURVE ( 'NONE', #39017, #51326, #29195, .T. ) ;
#13388=CARTESIAN_POINT ( 'NONE',  ( -22.40634380310664397, 0.000000000000000000, 5.584705972946605534 ) ) ;
#13389=CARTESIAN_POINT ( 'NONE',  ( -15.87975247367846166, 0.000000000000000000, 2.850166870931599927 ) ) ;
#13391=VERTEX_POINT ( 'NONE', #38013 ) ;
#13392=FACE_OUTER_BOUND ( 'NONE', #4396, .T. ) ;
#13393=EDGE_CURVE ( 'NONE', #10405, #36484, #25500, .T. ) ;
#13394=VECTOR ( 'NONE', #9505, 1000.000000000000000 ) ;
#13395=ORIENTED_EDGE ( 'NONE', *, *, #19953, .F. ) ;
#13396=LINE ( 'NONE', #48576, #28579 ) ;
#13397=ORIENTED_EDGE ( 'NONE', *, *, #29720, .F. ) ;
#13399=EDGE_CURVE ( 'NONE', #28247, #48080, #4234, .T. ) ;
#13400=ORIENTED_EDGE ( 'NONE', *, *, #39415, .F. ) ;
#13401=EDGE_LOOP ( 'NONE', ( #50201, #53055, #28967, #44465 ) ) ;
#13402=ORIENTED_EDGE ( 'NONE', *, *, #36149, .T. ) ;
#13403=DIRECTION ( 'NONE',  ( 0.005961354470445682716, -0.6427876096865404731, -0.7660212471507180654 ) ) ;
#13404=FACE_OUTER_BOUND ( 'NONE', #34281, .T. ) ;
#13405=PLANE ( 'NONE',  #33024 ) ;
#13406=DIRECTION ( 'NONE',  ( 0.007781995580012663651, 0.000000000000000000, -0.9999697198139515519 ) ) ;
#13407=ORIENTED_EDGE ( 'NONE', *, *, #52068, .T. ) ;
#13408=ORIENTED_EDGE ( 'NONE', *, *, #25478, .T. ) ;
#13409=CARTESIAN_POINT ( 'NONE',  ( -19.23990622075459811, 1.095915999411505526, 4.120399239466145502 ) ) ;
#13410=ORIENTED_EDGE ( 'NONE', *, *, #31957, .T. ) ;
#13411=LINE ( 'NONE', #21899, #18456 ) ;
#13412=ORIENTED_EDGE ( 'NONE', *, *, #33353, .T. ) ;
#13413=DIRECTION ( 'NONE',  ( 0.005002170337468016433, -0.7660444431189770143, -0.6427681459581293666 ) ) ;
#13414=CARTESIAN_POINT ( 'NONE',  ( -9.135000016821216207, 6.796527418557151812, 0.3299706567759553844 ) ) ;
#13415=ORIENTED_EDGE ( 'NONE', *, *, #19761, .T. ) ;
#13416=CARTESIAN_POINT ( 'NONE',  ( -19.12962290826653700, 0.000000000000000000, 14.40064212555863854 ) ) ;
#13417=ORIENTED_EDGE ( 'NONE', *, *, #7626, .F. ) ;
#13418=DIRECTION ( 'NONE',  ( -0.9999697198139514409, -0.000000000000000000, -0.007781995580013368816 ) ) ;
#13419=ORIENTED_EDGE ( 'NONE', *, *, #30358, .T. ) ;
#13420=DIRECTION ( 'NONE',  ( 0.7660212471507180654, -0.6427876096865404731, 0.005961354470445141482 ) ) ;
#13421=PLANE ( 'NONE',  #22979 ) ;
#13422=CARTESIAN_POINT ( 'NONE',  ( -16.81190032086591302, 0.000000000000000000, 3.212244750653343583 ) ) ;
#13423=ORIENTED_EDGE ( 'NONE', *, *, #23407, .F. ) ;
#13424=EDGE_CURVE ( 'NONE', #41178, #34966, #33471, .T. ) ;
#13425=EDGE_CURVE ( 'NONE', #55458, #25319, #17004, .T. ) ;
#13426=DIRECTION ( 'NONE',  ( 0.9999697198139515519, 0.000000000000000000, 0.007781995580013368816 ) ) ;
#13427=VECTOR ( 'NONE', #7987, 1000.000000000000000 ) ;
#13428=DIRECTION ( 'NONE',  ( 0.000000000000000000, -0.000000000000000000, -1.000000000000000000 ) ) ;
#13429=LINE ( 'NONE', #47198, #14009 ) ;
#13430=LINE ( 'NONE', #30746, #6004 ) ;
#13431=ADVANCED_FACE ( 'NONE', ( #51629 ), #55316, .F. ) ;
#13432=CARTESIAN_POINT ( 'NONE',  ( -13.06083377814856483, -5.536956232915664522, 10.84229159693478017 ) ) ;
#13434=DIRECTION ( 'NONE',  ( 0.007781995580012663651, 0.000000000000000000, -0.9999697198139515519 ) ) ;
#13435=VERTEX_POINT ( 'NONE', #46505 ) ;
#13436=FACE_OUTER_BOUND ( 'NONE', #41344, .T. ) ;
#13437=DIRECTION ( 'NONE',  ( 0.000000000000000000, -0.000000000000000000, -1.000000000000000000 ) ) ;
#13438=CARTESIAN_POINT ( 'NONE',  ( -15.29625084614291097, 0.2864062442990042978, 2.614377164303661960 ) ) ;
#13439=VERTEX_POINT ( 'NONE', #16411 ) ;
#13440=CARTESIAN_POINT ( 'NONE',  ( 2.072287782118878319, 0.000000000000000000, -2.950529333540147015 ) ) ;
#13441=LINE ( 'NONE', #30758, #15451 ) ;
#13442=ORIENTED_EDGE ( 'NONE', *, *, #36294, .T. ) ;
#13443=CARTESIAN_POINT ( 'NONE',  ( -10.84028925556084388, -0.1191753592594197858, 11.14116300850493246 ) ) ;
#13444=LINE ( 'NONE', #10004, #30290 ) ;
#13445=CARTESIAN_POINT ( 'NONE',  ( -15.86710544311044302, 0.000000000000000000, 13.13336954653252953 ) ) ;
#13446=LINE ( 'NONE', #52876, #28307 ) ;
#13447=VERTEX_POINT ( 'NONE', #3379 ) ;
#13448=ORIENTED_EDGE ( 'NONE', *, *, #39865, .F. ) ;
#13449=CARTESIAN_POINT ( 'NONE',  ( -11.59673056228890076, 0.000000000000000000, 1.775502128378044331 ) ) ;
#13450=DIRECTION ( 'NONE',  ( 0.005961354470445682716, -0.6427876096865404731, -0.7660212471507180654 ) ) ;
#13451=FACE_OUTER_BOUND ( 'NONE', #29226, .T. ) ;
#13453=DIRECTION ( 'NONE',  ( 0.007781995580012663651, 0.000000000000000000, -0.9999697198139515519 ) ) ;
#13454=CARTESIAN_POINT ( 'NONE',  ( -21.47263955680318404, 0.000000000000000000, 5.022634149262071190 ) ) ;
#13455=VERTEX_POINT ( 'NONE', #33207 ) ;
#13456=LINE ( 'NONE', #31617, #17454 ) ;
#13457=ADVANCED_FACE ( 'NONE', ( #16151 ), #3640, .F. ) ;
#13458=FACE_OUTER_BOUND ( 'NONE', #53737, .T. ) ;
#13459=ORIENTED_EDGE ( 'NONE', *, *, #42571, .F. ) ;
#13460=EDGE_CURVE ( 'NONE', #30608, #37937, #8192, .T. ) ;
#13462=LINE ( 'NONE', #39848, #55824 ) ;
#13463=EDGE_CURVE ( 'NONE', #54313, #19601, #42551, .T. ) ;
#13464=LINE ( 'NONE', #44651, #4005 ) ;
#13465=ORIENTED_EDGE ( 'NONE', *, *, #34896, .T. ) ;
#13466=VECTOR ( 'NONE', #24572, 1000.000000000000114 ) ;
#13467=PLANE ( 'NONE',  #32275 ) ;
#13468=EDGE_CURVE ( 'NONE', #9720, #10560, #28935, .T. ) ;
#13469=ORIENTED_EDGE ( 'NONE', *, *, #42029, .T. ) ;
#13470=VERTEX_POINT ( 'NONE', #24952 ) ;
#13471=ORIENTED_EDGE ( 'NONE', *, *, #49514, .F. ) ;
#13472=ORIENTED_EDGE ( 'NONE', *, *, #34068, .F. ) ;
#13473=CARTESIAN_POINT ( 'NONE',  ( -18.03805572822844283, -4.889348428825663895, 3.731918723547563932 ) ) ;
#13474=ORIENTED_EDGE ( 'NONE', *, *, #36107, .F. ) ;
#13475=FACE_OUTER_BOUND ( 'NONE', #41529, .T. ) ;
#13476=VERTEX_POINT ( 'NONE', #20699 ) ;
#13477=CARTESIAN_POINT ( 'NONE',  ( -14.94760462649100496, 0.000000000000000000, 2.488088991209854051 ) ) ;
#13478=ORIENTED_EDGE ( 'NONE', *, *, #51458, .F. ) ;
#13479=CARTESIAN_POINT ( 'NONE',  ( -14.01545677930355183, 0.000000000000000000, 2.126011111488108174 ) ) ;
#13480=EDGE_LOOP ( 'NONE', ( #12952, #51075, #2431, #33302 ) ) ;
#13481=DIRECTION ( 'NONE',  ( 0.007781995580012663651, 0.000000000000000000, -0.9999697198139515519 ) ) ;
#13482=PLANE ( 'NONE',  #28654 ) ;
#13483=DIRECTION ( 'NONE',  ( 0.007781995580012663651, -3.146120232559066537E-19, -0.9999697198139514409 ) ) ;
#13484=LINE ( 'NONE', #31649, #20558 ) ;
#13485=FACE_OUTER_BOUND ( 'NONE', #8872, .T. ) ;
#13486=EDGE_LOOP ( 'NONE', ( #25605, #48872, #318, #29235 ) ) ;
#13487=EDGE_CURVE ( 'NONE', #17790, #6537, #48791, .T. ) ;
#13488=ORIENTED_EDGE ( 'NONE', *, *, #8239, .F. ) ;
#13489=LINE ( 'NONE', #51805, #36734 ) ;
#13490=DIRECTION ( 'NONE',  ( -0.5449076811759708816, 0.6444004775717707689, 0.5364919789714475140 ) ) ;
#13491=EDGE_CURVE ( 'NONE', #1421, #394, #35430, .T. ) ;
#13493=DIRECTION ( 'NONE',  ( -0.005961354470445682716, -0.6427876096865404731, 0.7660212471507180654 ) ) ;
#13494=DIRECTION ( 'NONE',  ( -0.9999697198139514409, -0.000000000000000000, -0.007781995580013368816 ) ) ;
#13495=LINE ( 'NONE', #115, #16785 ) ;
#13496=CARTESIAN_POINT ( 'NONE',  ( -18.16200224167504373, 0.000000000000000000, 9.480383132038964433 ) ) ;
#13497=ORIENTED_EDGE ( 'NONE', *, *, #22266, .T. ) ;
#13498=PLANE ( 'NONE',  #48343 ) ;
#13499=LINE ( 'NONE', #38790, #5912 ) ;
#13500=ORIENTED_EDGE ( 'NONE', *, *, #48843, .F. ) ;
#13501=VECTOR ( 'NONE', #47799, 1000.000000000000227 ) ;
#13502=PLANE ( 'NONE',  #34300 ) ;
#13503=CARTESIAN_POINT ( 'NONE',  ( -17.74560456716937296, 0.000000000000000000, 3.774316574337878372 ) ) ;
#13504=FACE_OUTER_BOUND ( 'NONE', #26107, .T. ) ;
#13506=EDGE_CURVE ( 'NONE', #42368, #6114, #17550, .T. ) ;
#13507=LINE ( 'NONE', #52662, #29238 ) ;
#13508=ORIENTED_EDGE ( 'NONE', *, *, #55272, .F. ) ;
#13509=VERTEX_POINT ( 'NONE', #22090 ) ;
#13510=DIRECTION ( 'NONE',  ( -0.6427681459581293666, -0.7660444431189770143, -0.005002170337467561935 ) ) ;
#13511=CARTESIAN_POINT ( 'NONE',  ( 2.072287782118878319, 0.000000000000000000, -2.950529333540147015 ) ) ;
#13512=CARTESIAN_POINT ( 'NONE',  ( -16.81345671998191449, 0.000000000000000000, 3.412238694616132495 ) ) ;
#13513=CARTESIAN_POINT ( 'NONE',  ( 2.072287782118878319, 0.000000000000000000, -2.950529333540147015 ) ) ;
#13514=LINE ( 'NONE', #9538, #27616 ) ;
#13516=DIRECTION ( 'NONE',  ( 0.000000000000000000, -0.000000000000000000, -1.000000000000000000 ) ) ;
#13518=DIRECTION ( 'NONE',  ( -0.5364919789714478471, 0.6444004775717705469, -0.5449076811759709926 ) ) ;
#13519=CARTESIAN_POINT ( 'NONE',  ( -15.81295127592206207, 0.000000000000000000, 6.174675361559132547 ) ) ;
#13520=ORIENTED_EDGE ( 'NONE', *, *, #52466, .T. ) ;
#13521=DIRECTION ( 'NONE',  ( -0.005961354470445682716, -0.6427876096865404731, 0.7660212471507180654 ) ) ;
#13522=ORIENTED_EDGE ( 'NONE', *, *, #26190, .T. ) ;
#13523=DIRECTION ( 'NONE',  ( 0.5449076811759707706, 0.6444004775717708799, -0.5364919789714476250 ) ) ;
#13524=DIRECTION ( 'NONE',  ( -0.5364919789714478471, 0.6444004775717705469, -0.5449076811759709926 ) ) ;
#13525=ORIENTED_EDGE ( 'NONE', *, *, #36149, .F. ) ;
#13526=EDGE_CURVE ( 'NONE', #34394, #55847, #31165, .T. ) ;
#13527=ORIENTED_EDGE ( 'NONE', *, *, #50191, .T. ) ;
#13528=ORIENTED_EDGE ( 'NONE', *, *, #53716, .F. ) ;
#13529=ORIENTED_EDGE ( 'NONE', *, *, #39668, .T. ) ;
#13530=EDGE_LOOP ( 'NONE', ( #3350, #27718, #15271 ) ) ;
#13531=VERTEX_POINT ( 'NONE', #48490 ) ;
#13532=LINE ( 'NONE', #47048, #7745 ) ;
#13533=FACE_OUTER_BOUND ( 'NONE', #39035, .T. ) ;
#13534=PLANE ( 'NONE',  #9531 ) ;
#13535=EDGE_CURVE ( 'NONE', #2679, #49846, #13312, .T. ) ;
#13536=ORIENTED_EDGE ( 'NONE', *, *, #16953, .T. ) ;
#13537=FACE_OUTER_BOUND ( 'NONE', #19354, .T. ) ;
#13538=ORIENTED_EDGE ( 'NONE', *, *, #9170, .F. ) ;
#13539=ADVANCED_FACE ( 'NONE', ( #52733 ), #30637, .F. ) ;
#13540=ORIENTED_EDGE ( 'NONE', *, *, #53904, .T. ) ;
#13541=ADVANCED_FACE ( 'NONE', ( #35719 ), #26094, .F. ) ;
#13542=DIRECTION ( 'NONE',  ( 0.000000000000000000, -0.000000000000000000, -1.000000000000000000 ) ) ;
#13543=CARTESIAN_POINT ( 'NONE',  ( -13.08486533123210194, 0.000000000000000000, 1.963927175729152541 ) ) ;
#13544=LINE ( 'NONE', #26313, #32285 ) ;
#13545=ADVANCED_FACE ( 'NONE', ( #51896 ), #9035, .F. ) ;
#13546=ORIENTED_EDGE ( 'NONE', *, *, #38039, .F. ) ;
#13547=LINE ( 'NONE', #24018, #9251 ) ;
#13548=EDGE_LOOP ( 'NONE', ( #26724, #5008, #27900, #18767 ) ) ;
#13549=DIRECTION ( 'NONE',  ( 0.000000000000000000, -0.000000000000000000, -1.000000000000000000 ) ) ;
#13550=ADVANCED_FACE ( 'NONE', ( #4767 ), #43399, .F. ) ;
#13551=DIRECTION ( 'NONE',  ( 0.6427681459581294776, -0.7660444431189769032, 0.005002170337467562802 ) ) ;
#13552=ADVANCED_FACE ( 'NONE', ( #202 ), #26625, .F. ) ;
#13553=LINE ( 'NONE', #36006, #38731 ) ;
#13554=DIRECTION ( 'NONE',  ( -0.5449076811759708816, 0.6444004775717707689, 0.5364919789714475140 ) ) ;
#13555=DIRECTION ( 'NONE',  ( 0.5364919789714477361, 0.6444004775717706579, 0.5449076811759711036 ) ) ;
#13557=CARTESIAN_POINT ( 'NONE',  ( -19.96568551101100297, -0.1191753592594195360, 6.242360851625931240 ) ) ;
#13558=DIRECTION ( 'NONE',  ( 0.007781995580012663651, -3.146120232559066537E-19, -0.9999697198139514409 ) ) ;
#13559=ORIENTED_EDGE ( 'NONE', *, *, #32626, .T. ) ;
#13560=PLANE ( 'NONE',  #219 ) ;
#13561=ADVANCED_FACE ( 'NONE', ( #5067 ), #39711, .F. ) ;
#13562=CARTESIAN_POINT ( 'NONE',  ( -24.26986129792355129, -0.1191753592594197858, 6.208864760408702388 ) ) ;
#13563=DIRECTION ( 'NONE',  ( -0.005961354470445682716, -0.6427876096865404731, 0.7660212471507180654 ) ) ;
#13564=DIRECTION ( 'NONE',  ( 0.6246952433987894571, -0.7422098413412800966, -0.2426528472758541777 ) ) ;
#13566=DIRECTION ( 'NONE',  ( 0.005961354470445682716, -0.6427876096865404731, -0.7660212471507180654 ) ) ;
#13567=DIRECTION ( 'NONE',  ( 0.007781995580012663651, 0.000000000000000000, -0.9999697198139515519 ) ) ;
#13568=ADVANCED_FACE ( 'NONE', ( #47939 ), #43653, .F. ) ;
#13569=CARTESIAN_POINT ( 'NONE',  ( -8.373012819454125122, 0.000000000000000000, 5.493910543331755214 ) ) ;
#13570=VERTEX_POINT ( 'NONE', #27190 ) ;
#13571=DIRECTION ( 'NONE',  ( 0.005961354470445682716, -0.6427876096865404731, -0.7660212471507180654 ) ) ;
#13572=DIRECTION ( 'NONE',  ( -0.005961354470445682716, -0.6427876096865404731, 0.7660212471507180654 ) ) ;
#13573=DIRECTION ( 'NONE',  ( -0.5364919789714478471, 0.6444004775717705469, -0.5449076811759709926 ) ) ;
#13576=CARTESIAN_POINT ( 'NONE',  ( -4.092399949646539525, 6.327196921604587132, -1.628746456733796588 ) ) ;
#13577=CARTESIAN_POINT ( 'NONE',  ( -11.16239059961664282, 0.000000000000000000, 5.672209016686486471 ) ) ;
#13578=FACE_OUTER_BOUND ( 'NONE', #18712, .T. ) ;
#13581=VERTEX_POINT ( 'NONE', #18106 ) ;
#13582=ADVANCED_FACE ( 'NONE', ( #48191 ), #13839, .F. ) ;
#13583=ORIENTED_EDGE ( 'NONE', *, *, #43562, .T. ) ;
#13584=ORIENTED_EDGE ( 'NONE', *, *, #4207, .T. ) ;
#13585=VERTEX_POINT ( 'NONE', #39964 ) ;
#13586=ORIENTED_EDGE ( 'NONE', *, *, #13750, .F. ) ;
#13587=DIRECTION ( 'NONE',  ( -0.005961354470445682716, -0.6427876096865404731, 0.7660212471507180654 ) ) ;
#13588=CARTESIAN_POINT ( 'NONE',  ( 2.072287782118878319, 0.000000000000000000, -2.950529333540147015 ) ) ;
#13589=ORIENTED_EDGE ( 'NONE', *, *, #13981, .T. ) ;
#13590=ORIENTED_EDGE ( 'NONE', *, *, #39887, .T. ) ;
#13591=ADVANCED_FACE ( 'NONE', ( #28583 ), #14975, .F. ) ;
#13592=CARTESIAN_POINT ( 'NONE',  ( -13.01075962734913816, 0.000000000000000000, 4.349822315878366652 ) ) ;
#13593=ORIENTED_EDGE ( 'NONE', *, *, #38818, .F. ) ;
#13594=CARTESIAN_POINT ( 'NONE',  ( -10.94028622754223967, 0.000000000000000000, 11.14038480894692995 ) ) ;
#13595=FACE_OUTER_BOUND ( 'NONE', #45166, .T. ) ;
#13596=ORIENTED_EDGE ( 'NONE', *, *, #44046, .F. ) ;
#13597=CARTESIAN_POINT ( 'NONE',  ( -13.07066190154808361, 0.000000000000000000, 12.04713590736729678 ) ) ;
#13598=ORIENTED_EDGE ( 'NONE', *, *, #13909, .F. ) ;
#13599=CARTESIAN_POINT ( 'NONE',  ( -14.00280974873554030, 0.000000000000000000, 12.40921378708904044 ) ) ;
#13600=ADVANCED_FACE ( 'NONE', ( #49330 ), #23755, .F. ) ;
#13601=CARTESIAN_POINT ( 'NONE',  ( -9.908559390481867624, 0.8026771090238171702, 1.484425475346726531 ) ) ;
#13602=ADVANCED_FACE ( 'NONE', ( #45341 ), #45907, .F. ) ;
#13603=LINE ( 'NONE', #1383, #48154 ) ;
#13604=LINE ( 'NONE', #15995, #11520 ) ;
#13605=EDGE_LOOP ( 'NONE', ( #38883, #26444, #43453, #9739 ) ) ;
#13606=CARTESIAN_POINT ( 'NONE',  ( -19.59569683186026268, 0.000000000000000000, 14.58168106541950948 ) ) ;
#13608=CARTESIAN_POINT ( 'NONE',  ( -24.26986129792355129, -0.1191753592594197858, 6.208864760408702388 ) ) ;
#13609=EDGE_LOOP ( 'NONE', ( #37087, #15934, #10252, #50325 ) ) ;
#13610=CARTESIAN_POINT ( 'NONE',  ( -9.808144436391993182, 0.000000000000000000, 10.77986332834118777 ) ) ;
#13611=ORIENTED_EDGE ( 'NONE', *, *, #34885, .T. ) ;
#13612=EDGE_CURVE ( 'NONE', #36877, #17353, #41077, .T. ) ;
#13613=DIRECTION ( 'NONE',  ( 0.9999697198139515519, 0.000000000000000000, 0.007781995580013368816 ) ) ;
#13614=DIRECTION ( 'NONE',  ( 0.9999697198139515519, 0.000000000000000000, 0.007781995580013368816 ) ) ;
#13615=CARTESIAN_POINT ( 'NONE',  ( -12.12632416399392277, 0.9340140483890049250, 3.124473410292289977 ) ) ;
#13616=DIRECTION ( 'NONE',  ( 0.007781995580012662783, 0.000000000000000000, -0.9999697198139514409 ) ) ;
#13617=LINE ( 'NONE', #5658, #12319 ) ;
#13618=DIRECTION ( 'NONE',  ( 0.9321478471874541372, 0.000000000000000000, -0.3620778797217453771 ) ) ;
#13619=DIRECTION ( 'NONE',  ( -0.6427681459581293666, -0.7660444431189770143, -0.005002170337467561935 ) ) ;
#13620=EDGE_CURVE ( 'NONE', #52907, #21716, #27768, .T. ) ;
#13621=CARTESIAN_POINT ( 'NONE',  ( -16.71867036141801677, -5.536956232915664522, 3.198762561013173578 ) ) ;
#13622=LINE ( 'NONE', #26397, #35972 ) ;
#13623=ORIENTED_EDGE ( 'NONE', *, *, #33996, .F. ) ;
#13624=DIRECTION ( 'NONE',  ( -0.9999697198139514409, -0.000000000000000000, -0.007781995580013368816 ) ) ;
#13625=DIRECTION ( 'NONE',  ( 0.007781995580012663651, -3.146120232559066537E-19, -0.9999697198139514409 ) ) ;
#13627=CARTESIAN_POINT ( 'NONE',  ( -10.37421533196711465, -0.1191753592594197858, 10.96012406864405975 ) ) ;
#13629=CARTESIAN_POINT ( 'NONE',  ( 2.072287782118878319, 0.000000000000000000, -2.950529333540147015 ) ) ;
#13630=FACE_OUTER_BOUND ( 'NONE', #50473, .T. ) ;
#13631=EDGE_LOOP ( 'NONE', ( #41595, #45974, #702, #39846, #5372 ) ) ;
#13632=VECTOR ( 'NONE', #32603, 1000.000000000000227 ) ;
#13633=ORIENTED_EDGE ( 'NONE', *, *, #1326, .T. ) ;
#13634=DIRECTION ( 'NONE',  ( 0.007781995580012662783, 0.000000000000000000, -0.9999697198139514409 ) ) ;
#13635=DIRECTION ( 'NONE',  ( 0.005961354470445682716, -0.6427876096865404731, -0.7660212471507180654 ) ) ;
#13636=EDGE_CURVE ( 'NONE', #29728, #21771, #1340, .T. ) ;
#13637=ORIENTED_EDGE ( 'NONE', *, *, #45357, .F. ) ;
#13638=CARTESIAN_POINT ( 'NONE',  ( -13.53673582514181106, 0.000000000000000000, 12.22817484722816772 ) ) ;
#13639=EDGE_CURVE ( 'NONE', #34394, #36809, #14429, .T. ) ;
#13640=ORIENTED_EDGE ( 'NONE', *, *, #47235, .T. ) ;
#13641=DIRECTION ( 'NONE',  ( 0.007781995580012663651, 0.000000000000000000, -0.9999697198139515519 ) ) ;
#13642=ORIENTED_EDGE ( 'NONE', *, *, #9842, .T. ) ;
#13643=ORIENTED_EDGE ( 'NONE', *, *, #13650, .F. ) ;
#13644=ADVANCED_FACE ( 'NONE', ( #27464 ), #37108, .F. ) ;
#13645=ORIENTED_EDGE ( 'NONE', *, *, #52981, .F. ) ;
#13646=ADVANCED_FACE ( 'NONE', ( #18962 ), #28294, .F. ) ;
#13647=DIRECTION ( 'NONE',  ( -0.6427681459581293666, -0.7660444431189770143, -0.005002170337467561935 ) ) ;
#13648=DIRECTION ( 'NONE',  ( -0.005002170337468016433, -0.7660444431189770143, 0.6427681459581293666 ) ) ;
#13650=EDGE_CURVE ( 'NONE', #26046, #18030, #10730, .T. ) ;
#13651=ADVANCED_FACE ( 'NONE', ( #23228 ), #19209, .F. ) ;
#13652=EDGE_CURVE ( 'NONE', #50299, #55191, #36279, .T. ) ;
#13653=CARTESIAN_POINT ( 'NONE',  ( -1.148821818165424169, 4.447699752827971587, 3.664614983992416697 ) ) ;
#13654=VERTEX_POINT ( 'NONE', #41378 ) ;
#13655=ORIENTED_EDGE ( 'NONE', *, *, #46961, .T. ) ;
#13656=FACE_OUTER_BOUND ( 'NONE', #30693, .T. ) ;
#13657=ORIENTED_EDGE ( 'NONE', *, *, #48211, .F. ) ;
#13658=CARTESIAN_POINT ( 'NONE',  ( -15.03495456790438389, -0.1191753592594197858, 12.77051346725278158 ) ) ;
#13659=ORIENTED_EDGE ( 'NONE', *, *, #2622, .T. ) ;
#13660=PLANE ( 'NONE',  #5181 ) ;
#13661=PLANE ( 'NONE',  #38481 ) ;
#13663=VECTOR ( 'NONE', #43764, 1000.000000000000000 ) ;
#13664=LINE ( 'NONE', #30980, #20453 ) ;
#13665=EDGE_CURVE ( 'NONE', #9855, #50386, #53333, .T. ) ;
#13666=ORIENTED_EDGE ( 'NONE', *, *, #46538, .T. ) ;
#13667=VECTOR ( 'NONE', #37508, 1000.000000000000000 ) ;
#13668=EDGE_CURVE ( 'NONE', #33376, #49938, #14686, .T. ) ;
#13669=DIRECTION ( 'NONE',  ( 0.5449076811759707706, 0.6444004775717708799, -0.5364919789714476250 ) ) ;
#13670=ORIENTED_EDGE ( 'NONE', *, *, #54894, .F. ) ;
#13671=DIRECTION ( 'NONE',  ( -0.5364919789714478471, 0.6444004775717705469, -0.5449076811759709926 ) ) ;
#13672=LINE ( 'NONE', #39810, #14835 ) ;
#13673=ADVANCED_FACE ( 'NONE', ( #45612 ), #11258, .F. ) ;
#13674=LINE ( 'NONE', #30166, #1959 ) ;
#13675=ORIENTED_EDGE ( 'NONE', *, *, #36843, .T. ) ;
#13676=DIRECTION ( 'NONE',  ( 0.6246952433987893460, 0.7422098413412802076, -0.2426528472758539279 ) ) ;
#13677=EDGE_CURVE ( 'NONE', #49612, #38385, #36026, .T. ) ;
#13678=CARTESIAN_POINT ( 'NONE',  ( -26.13337879274045505, 0.000000000000000000, 6.833023547870798353 ) ) ;
#13679=CARTESIAN_POINT ( 'NONE',  ( -16.01608722591203104, -3.594132820645663084, 2.987841650007617922 ) ) ;
#13680=DIRECTION ( 'NONE',  ( -0.005002170337468016433, -0.7660444431189770143, 0.6427681459581293666 ) ) ;
#13681=CARTESIAN_POINT ( 'NONE',  ( -13.27065584551087163, 0.000000000000000000, 12.04557950825129176 ) ) ;
#13682=CARTESIAN_POINT ( 'NONE',  ( -23.33771345073609638, -0.1191753592594197858, 5.846786880686956955 ) ) ;
#13683=FACE_OUTER_BOUND ( 'NONE', #34715, .T. ) ;
#13684=ORIENTED_EDGE ( 'NONE', *, *, #97, .T. ) ;
#13685=CARTESIAN_POINT ( 'NONE',  ( -1.086233639165236964, 0.000000000000000000, -2.796443541562362078 ) ) ;
#13686=FACE_OUTER_BOUND ( 'NONE', #7393, .T. ) ;
#13687=CARTESIAN_POINT ( 'NONE',  ( -8.378760926464691394, 0.000000000000000000, 6.232529949847283923 ) ) ;
#13688=ORIENTED_EDGE ( 'NONE', *, *, #19549, .F. ) ;
#13689=ADVANCED_FACE ( 'NONE', ( #41633 ), #29425, .F. ) ;
#13690=DIRECTION ( 'NONE',  ( 0.5364919789714477361, 0.6444004775717706579, 0.5449076811759711036 ) ) ;
#13691=DIRECTION ( 'NONE',  ( 0.7660212471507180654, -0.6427876096865404731, 0.005961354470445141482 ) ) ;
#13693=EDGE_LOOP ( 'NONE', ( #45961, #27960, #11273, #39598 ) ) ;
#13694=CARTESIAN_POINT ( 'NONE',  ( -31.72782227498118601, 0.000000000000000000, 9.205484770164058972 ) ) ;
#13695=AXIS2_PLACEMENT_3D ( 'NONE', #8847, #44017, #22461 ) ;
#13697=CARTESIAN_POINT ( 'NONE',  ( -21.47419595591918906, 0.000000000000000000, 5.222628093224860102 ) ) ;
#13698=LINE ( 'NONE', #26215, #35054 ) ;
#13699=CARTESIAN_POINT ( 'NONE',  ( -11.40636015113596180, 0.000000000000000000, 11.32142374880780089 ) ) ;
#13700=ORIENTED_EDGE ( 'NONE', *, *, #51420, .F. ) ;
#13701=ORIENTED_EDGE ( 'NONE', *, *, #52407, .F. ) ;
#13702=LINE ( 'NONE', #10009, #45753 ) ;
#13703=FACE_OUTER_BOUND ( 'NONE', #8353, .T. ) ;
#13705=CARTESIAN_POINT ( 'NONE',  ( -14.84211576094791418, 4.657758921906509642, 10.29067882608070761 ) ) ;
#13706=CARTESIAN_POINT ( 'NONE',  ( -17.83139810946674686, -0.1191753592594197858, 13.85674710641801788 ) ) ;
#13707=VECTOR ( 'NONE', #52509, 1000.000000000000227 ) ;
#13708=FACE_OUTER_BOUND ( 'NONE', #32863, .T. ) ;
#13709=ORIENTED_EDGE ( 'NONE', *, *, #46692, .F. ) ;
#13710=LINE ( 'NONE', #9459, #10206 ) ;
#13711=AXIS2_PLACEMENT_3D ( 'NONE', #1410, #41445, #2526 ) ;
#13712=CARTESIAN_POINT ( 'NONE',  ( -13.63673279712320507, -0.1191753592594197858, 12.22739664767016521 ) ) ;
#13713=EDGE_LOOP ( 'NONE', ( #31241, #20141, #13643, #50398 ) ) ;
#13714=CARTESIAN_POINT ( 'NONE',  ( -15.34124861768113135, 0.000000000000000000, 5.270356107516636968 ) ) ;
#13715=DIRECTION ( 'NONE',  ( 0.007781995580012662783, 0.000000000000000000, -0.9999697198139514409 ) ) ;
#13716=DIRECTION ( 'NONE',  ( 0.007781995580012663651, -3.146120232559066537E-19, -0.9999697198139514409 ) ) ;
#13718=EDGE_CURVE ( 'NONE', #52808, #34831, #25185, .T. ) ;
#13719=ORIENTED_EDGE ( 'NONE', *, *, #41312, .T. ) ;
#13720=LINE ( 'NONE', #49197, #29267 ) ;
#13721=ORIENTED_EDGE ( 'NONE', *, *, #2027, .F. ) ;
#13722=EDGE_CURVE ( 'NONE', #39978, #308, #38208, .T. ) ;
#13723=ORIENTED_EDGE ( 'NONE', *, *, #31406, .T. ) ;
#13724=ORIENTED_EDGE ( 'NONE', *, *, #24417, .T. ) ;
#13726=CARTESIAN_POINT ( 'NONE',  ( -14.71120258492120136, -1.489407457353158160, 2.548131899913917309 ) ) ;
#13727=ORIENTED_EDGE ( 'NONE', *, *, #21238, .T. ) ;
#13728=DIRECTION ( 'NONE',  ( 0.000000000000000000, -0.000000000000000000, -1.000000000000000000 ) ) ;
#13729=LINE ( 'NONE', #31050, #32231 ) ;
#13730=AXIS2_PLACEMENT_3D ( 'NONE', #38927, #26150, #26996 ) ;
#13731=AXIS2_PLACEMENT_3D ( 'NONE', #7671, #11913, #50260 ) ;
#13732=ORIENTED_EDGE ( 'NONE', *, *, #39892, .T. ) ;
#13733=DIRECTION ( 'NONE',  ( 0.9999697198139515519, 0.000000000000000000, 0.007781995580013368816 ) ) ;
#13734=ORIENTED_EDGE ( 'NONE', *, *, #14316, .F. ) ;
#13735=LINE ( 'NONE', #39613, #2129 ) ;
#13736=EDGE_LOOP ( 'NONE', ( #22471, #13386, #31384, #51170 ) ) ;
#13737=PLANE ( 'NONE',  #21037 ) ;
#13738=CARTESIAN_POINT ( 'NONE',  ( -23.33771345073609638, -0.1191753592594197858, 5.846786880686956955 ) ) ;
#13739=VECTOR ( 'NONE', #22861, 1000.000000000000227 ) ;
#13740=LINE ( 'NONE', #950, #10552 ) ;
#13742=EDGE_CURVE ( 'NONE', #52840, #33489, #37947, .T. ) ;
#13743=CARTESIAN_POINT ( 'NONE',  ( -15.50102849149811135, -0.1191753592594197858, 12.95155240711365430 ) ) ;
#13744=CARTESIAN_POINT ( 'NONE',  ( -11.19417631680646963, 0.9340140483890049250, 2.762395530570545432 ) ) ;
#13745=ORIENTED_EDGE ( 'NONE', *, *, #41169, .F. ) ;
#13746=EDGE_CURVE ( 'NONE', #17943, #41770, #34263, .T. ) ;
#13748=LINE ( 'NONE', #31067, #24932 ) ;
#13749=DIRECTION ( 'NONE',  ( 0.6427681459581294776, -0.7660444431189769032, 0.005002170337467562802 ) ) ;
#13750=EDGE_CURVE ( 'NONE', #49112, #18253, #11810, .T. ) ;
#13751=AXIS2_PLACEMENT_3D ( 'NONE', #23855, #20140, #37473 ) ;
#13752=CARTESIAN_POINT ( 'NONE',  ( -15.55405643005433269, 0.000000000000000000, 6.915354280726666580 ) ) ;
#13753=FACE_OUTER_BOUND ( 'NONE', #5721, .T. ) ;
#13754=ORIENTED_EDGE ( 'NONE', *, *, #21921, .F. ) ;
#13755=LINE ( 'NONE', #38482, #17680 ) ;
#13756=DIRECTION ( 'NONE',  ( -0.6427681459581293666, -0.7660444431189770143, -0.005002170337467561935 ) ) ;
#13757=EDGE_LOOP ( 'NONE', ( #48526, #31106, #18793, #7022 ) ) ;
#13758=CARTESIAN_POINT ( 'NONE',  ( -3.335658863730355694, -6.482724466489810489, -1.922690393539094433 ) ) ;
#13759=DIRECTION ( 'NONE',  ( 0.7660212471507180654, -0.6427876096865404731, 0.005961354470445141482 ) ) ;
#13760=ORIENTED_EDGE ( 'NONE', *, *, #21688, .F. ) ;
#13761=DIRECTION ( 'NONE',  ( -0.5364919789714478471, 0.6444004775717705469, -0.5449076811759709926 ) ) ;
#13762=DIRECTION ( 'NONE',  ( 0.5449076811759707706, 0.6444004775717708799, -0.5364919789714476250 ) ) ;
#13763=DIRECTION ( 'NONE',  ( 0.007781995580012663651, -3.146120232559066537E-19, -0.9999697198139514409 ) ) ;
#13764=CARTESIAN_POINT ( 'NONE',  ( -18.80519705355265003, 0.000000000000000000, 6.720727139055624022 ) ) ;
#13766=ORIENTED_EDGE ( 'NONE', *, *, #13718, .T. ) ;
#13767=ORIENTED_EDGE ( 'NONE', *, *, #14949, .T. ) ;
#13768=DIRECTION ( 'NONE',  ( -0.5364919789714478471, 0.6444004775717705469, -0.5449076811759709926 ) ) ;
#13770=DIRECTION ( 'NONE',  ( -0.6427681459581293666, -0.7660444431189770143, -0.005002170337467561935 ) ) ;
#13771=VECTOR ( 'NONE', #40816, 1000.000000000000227 ) ;
#13772=VECTOR ( 'NONE', #52577, 1000.000000000000114 ) ;
#13773=LINE ( 'NONE', #1573, #54528 ) ;
#13774=CARTESIAN_POINT ( 'NONE',  ( 2.072287782118878319, 0.000000000000000000, -2.950529333540147015 ) ) ;
#13775=ORIENTED_EDGE ( 'NONE', *, *, #20888, .F. ) ;
#13776=CARTESIAN_POINT ( 'NONE',  ( -18.26849638870942272, -0.1191753592594162470, 10.31447797378732645 ) ) ;
#13777=LINE ( 'NONE', #47293, #26585 ) ;
#13779=DIRECTION ( 'NONE',  ( -0.005002170337468016433, -0.7660444431189770143, 0.6427681459581293666 ) ) ;
#13780=VECTOR ( 'NONE', #30274, 999.9999999999998863 ) ;
#13781=VERTEX_POINT ( 'NONE', #12669 ) ;
#13782=FACE_OUTER_BOUND ( 'NONE', #23856, .T. ) ;
#13783=ORIENTED_EDGE ( 'NONE', *, *, #19698, .F. ) ;
#13784=DIRECTION ( 'NONE',  ( 0.007781995580012662783, 0.000000000000000000, -0.9999697198139514409 ) ) ;
#13785=DIRECTION ( 'NONE',  ( 0.005002170337468016433, -0.7660444431189770143, -0.6427681459581293666 ) ) ;
#13786=ADVANCED_FACE ( 'NONE', ( #54996 ), #47284, .F. ) ;
#13787=ORIENTED_EDGE ( 'NONE', *, *, #5747, .T. ) ;
#13788=CARTESIAN_POINT ( 'NONE',  ( -15.87975247367846166, 0.000000000000000000, 2.850166870931599927 ) ) ;
#13789=VECTOR ( 'NONE', #2143, 999.9999999999998863 ) ;
#13790=ORIENTED_EDGE ( 'NONE', *, *, #49126, .F. ) ;
#13791=ADVANCED_FACE ( 'NONE', ( #29129 ), #11555, .F. ) ;
#13792=ADVANCED_FACE ( 'NONE', ( #24583 ), #16634, .F. ) ;
#13793=VECTOR ( 'NONE', #36182, 1000.000000000000227 ) ;
#13794=ORIENTED_EDGE ( 'NONE', *, *, #30562, .F. ) ;
#13795=ORIENTED_EDGE ( 'NONE', *, *, #49122, .F. ) ;
#13796=DIRECTION ( 'NONE',  ( 0.7660212471507180654, -0.6427876096865404731, 0.005961354470445141482 ) ) ;
#13797=ORIENTED_EDGE ( 'NONE', *, *, #30848, .F. ) ;
#13798=ORIENTED_EDGE ( 'NONE', *, *, #56000, .T. ) ;
#13799=DIRECTION ( 'NONE',  ( -0.5364919789714478471, 0.6444004775717705469, -0.5449076811759709926 ) ) ;
#13800=CARTESIAN_POINT ( 'NONE',  ( -19.60495096914714708, 3.686347215771508257, 10.54647366380701712 ) ) ;
#13801=VERTEX_POINT ( 'NONE', #55254 ) ;
#13802=ORIENTED_EDGE ( 'NONE', *, *, #40713, .T. ) ;
#13803=LINE ( 'NONE', #40213, #43069 ) ;
#13804=ORIENTED_EDGE ( 'NONE', *, *, #41368, .F. ) ;
#13805=ORIENTED_EDGE ( 'NONE', *, *, #32454, .F. ) ;
#13806=PLANE ( 'NONE',  #22034 ) ;
#13807=CARTESIAN_POINT ( 'NONE',  ( -32.10901097986136676, -1.000000000000000000, 16.76339505873265168 ) ) ;
#13808=DIRECTION ( 'NONE',  ( 0.007781995580012663651, 0.000000000000000000, -0.9999697198139515519 ) ) ;
#13809=AXIS2_PLACEMENT_3D ( 'NONE', #5965, #36327, #55594 ) ;
#13810=ORIENTED_EDGE ( 'NONE', *, *, #21630, .T. ) ;
#13811=CARTESIAN_POINT ( 'NONE',  ( -13.27065584551087163, 0.000000000000000000, 12.04557950825129176 ) ) ;
#13812=VERTEX_POINT ( 'NONE', #50981 ) ;
#13813=VECTOR ( 'NONE', #8072, 999.9999999999998863 ) ;
#13814=VECTOR ( 'NONE', #23801, 1000.000000000000227 ) ;
#13816=ADVANCED_FACE ( 'NONE', ( #29732 ), #46172, .F. ) ;
#13817=PLANE ( 'NONE',  #46942 ) ;
#13818=VECTOR ( 'NONE', #54167, 1000.000000000000114 ) ;
#13819=VECTOR ( 'NONE', #5726, 1000.000000000000227 ) ;
#13820=LINE ( 'NONE', #26910, #22247 ) ;
#13821=CARTESIAN_POINT ( 'NONE',  ( -14.85263745873890606, -3.270328918600659218, 7.818367421078713519 ) ) ;
#13822=EDGE_CURVE ( 'NONE', #46922, #51942, #47029, .T. ) ;
#13824=DIRECTION ( 'NONE',  ( 0.9999697198139515519, 0.000000000000000000, 0.007781995580013368816 ) ) ;
#13825=DIRECTION ( 'NONE',  ( 0.5449076811759707706, 0.6444004775717708799, -0.5364919789714476250 ) ) ;
#13826=ORIENTED_EDGE ( 'NONE', *, *, #38926, .T. ) ;
#13827=PLANE ( 'NONE',  #32903 ) ;
#13828=CARTESIAN_POINT ( 'NONE',  ( -28.92982233430281980, 0.000000000000000000, 7.919257187036034651 ) ) ;
#13829=CARTESIAN_POINT ( 'NONE',  ( -27.06552663992790997, 0.000000000000000000, 7.195101427592543786 ) ) ;
#13830=DIRECTION ( 'NONE',  ( 0.8531650599175527594, 0.4028455766673922356, -0.3313982828793700652 ) ) ;
#13831=EDGE_CURVE ( 'NONE', #55458, #31864, #20332, .T. ) ;
#13832=AXIS2_PLACEMENT_3D ( 'NONE', #26522, #4411, #51801 ) ;
#13834=CARTESIAN_POINT ( 'NONE',  ( -15.13495153988577968, 0.000000000000000000, 12.76973526769478084 ) ) ;
#13835=CARTESIAN_POINT ( 'NONE',  ( -24.26908309836554878, 0.000000000000000000, 6.108867788427308376 ) ) ;
#13836=PLANE ( 'NONE',  #46553 ) ;
#13837=ORIENTED_EDGE ( 'NONE', *, *, #3032, .T. ) ;
#13838=PLANE ( 'NONE',  #19369 ) ;
#13839=PLANE ( 'NONE',  #14939 ) ;
#13840=CARTESIAN_POINT ( 'NONE',  ( -19.26695989688845501, 0.000000000000000000, 6.347801524029851095 ) ) ;
#13841=CARTESIAN_POINT ( 'NONE',  ( -16.99924723426068951, 0.000000000000000000, 13.49389102713827171 ) ) ;
#13842=CARTESIAN_POINT ( 'NONE',  ( -13.07066190154808361, 0.000000000000000000, 12.04713590736729678 ) ) ;
#13843=AXIS2_PLACEMENT_3D ( 'NONE', #22850, #48715, #9227 ) ;
#13844=DIRECTION ( 'NONE',  ( 0.005961354470445682716, -0.6427876096865404731, -0.7660212471507180654 ) ) ;
#13845=EDGE_CURVE ( 'NONE', #37525, #4654, #24880, .T. ) ;
#13846=LINE ( 'NONE', #43405, #38330 ) ;
#13847=DIRECTION ( 'NONE',  ( -0.5449076811759708816, 0.6444004775717707689, 0.5364919789714475140 ) ) ;
#13848=AXIS2_PLACEMENT_3D ( 'NONE', #47228, #16291, #20270 ) ;
#13849=CARTESIAN_POINT ( 'NONE',  ( -17.27808141480208803, -3.432230869623162928, 3.483208570362961609 ) ) ;
#13850=EDGE_CURVE ( 'NONE', #28121, #13117, #26554, .T. ) ;
#13851=AXIS2_PLACEMENT_3D ( 'NONE', #50458, #46753, #38216 ) ;
#13852=VECTOR ( 'NONE', #31995, 999.9999999999998863 ) ;
#13854=ADVANCED_FACE ( 'NONE', ( #21746 ), #17779, .F. ) ;
#13855=EDGE_CURVE ( 'NONE', #14660, #10075, #26028, .T. ) ;
#13856=VECTOR ( 'NONE', #12882, 999.9999999999998863 ) ;
#13858=ORIENTED_EDGE ( 'NONE', *, *, #18487, .F. ) ;
#13859=EDGE_LOOP ( 'NONE', ( #23475, #28499, #33601, #31873 ) ) ;
#13861=FACE_OUTER_BOUND ( 'NONE', #36055, .T. ) ;
#13862=PLANE ( 'NONE',  #21267 ) ;
#13864=ORIENTED_EDGE ( 'NONE', *, *, #6636, .T. ) ;
#13865=VECTOR ( 'NONE', #34931, 999.9999999999998863 ) ;
#13866=VECTOR ( 'NONE', #37972, 1000.000000000000114 ) ;
#13867=EDGE_CURVE ( 'NONE', #12052, #4182, #17471, .T. ) ;
#13868=DIRECTION ( 'NONE',  ( -0.6427681459581293666, -0.7660444431189770143, -0.005002170337467561935 ) ) ;
#13869=EDGE_LOOP ( 'NONE', ( #3205, #15959, #6526, #45416 ) ) ;
#13870=FACE_OUTER_BOUND ( 'NONE', #53071, .T. ) ;
#13871=DIRECTION ( 'NONE',  ( 0.5449076811759707706, 0.6444004775717708799, -0.5364919789714476250 ) ) ;
#13872=EDGE_LOOP ( 'NONE', ( #55138, #3777, #8181, #13478 ) ) ;
#13873=DIRECTION ( 'NONE',  ( -0.7660212471507179544, -0.6427876096865405842, -0.005961354470445141482 ) ) ;
#13874=VECTOR ( 'NONE', #21720, 1000.000000000000114 ) ;
#13875=ORIENTED_EDGE ( 'NONE', *, *, #5092, .F. ) ;
#13876=CARTESIAN_POINT ( 'NONE',  ( -18.19747506107908563, 0.000000000000000000, 14.03856424583689311 ) ) ;
#13877=VECTOR ( 'NONE', #11405, 1000.000000000000000 ) ;
#13878=FACE_OUTER_BOUND ( 'NONE', #47947, .T. ) ;
#13879=CARTESIAN_POINT ( 'NONE',  ( -14.53367362947859753, -0.1117717739993928788, 8.863745978987285667 ) ) ;
#13880=LINE ( 'NONE', #31207, #50508 ) ;
#13881=ORIENTED_EDGE ( 'NONE', *, *, #9039, .T. ) ;
#13882=CARTESIAN_POINT ( 'NONE',  ( -12.57486326556087697, 0.000000000000000000, 8.046535260224020547 ) ) ;
#13883=LINE ( 'NONE', #35216, #12989 ) ;
#13884=CARTESIAN_POINT ( 'NONE',  ( -26.13337879274045505, 0.000000000000000000, 6.833023547870798353 ) ) ;
#13885=ORIENTED_EDGE ( 'NONE', *, *, #13850, .T. ) ;
#13886=CARTESIAN_POINT ( 'NONE',  ( -16.01869332689541991, 0.000000000000000000, 6.911738368958656231 ) ) ;
#13887=ORIENTED_EDGE ( 'NONE', *, *, #17362, .F. ) ;
#13888=AXIS2_PLACEMENT_3D ( 'NONE', #8136, #25442, #32838 ) ;
#13889=VECTOR ( 'NONE', #6643, 1000.000000000000000 ) ;
#13890=CARTESIAN_POINT ( 'NONE',  ( -16.26896601224730432, 0.000000000000000000, 5.063130340017827358 ) ) ;
#13891=FACE_OUTER_BOUND ( 'NONE', #35329, .T. ) ;
#13892=CARTESIAN_POINT ( 'NONE',  ( -16.61838873139687678, -3.756034771668162797, 3.216630489095766876 ) ) ;
#13894=ADVANCED_FACE ( 'NONE', ( #52957 ), #13237, .F. ) ;
#13895=PLANE ( 'NONE',  #36853 ) ;
#13896=PLANE ( 'NONE',  #42149 ) ;
#13897=DIRECTION ( 'NONE',  ( 0.9321478471874541372, 0.000000000000000000, -0.3620778797217453771 ) ) ;
#13898=VECTOR ( 'NONE', #29602, 999.9999999999998863 ) ;
#13899=CARTESIAN_POINT ( 'NONE',  ( -31.72626587586518099, 0.000000000000000000, 9.005490826201270949 ) ) ;
#13900=VECTOR ( 'NONE', #42347, 1000.000000000000227 ) ;
#13901=CARTESIAN_POINT ( 'NONE',  ( -22.10562829171461274, -5.213152330870663320, 13.82417958061751051 ) ) ;
#13902=ORIENTED_EDGE ( 'NONE', *, *, #8837, .T. ) ;
#13903=CARTESIAN_POINT ( 'NONE',  ( -15.87975247367846166, 0.000000000000000000, 2.850166870931599927 ) ) ;
#13904=CARTESIAN_POINT ( 'NONE',  ( -12.65008812213352485, 4.819660872929010687, 9.704929533543706910 ) ) ;
#13905=DIRECTION ( 'NONE',  ( -0.005002170337468016433, -0.7660444431189770143, 0.6427681459581293666 ) ) ;
#13906=PLANE ( 'NONE',  #16773 ) ;
#13907=ADVANCED_FACE ( 'NONE', ( #43589 ), #725, .F. ) ;
#13908=LINE ( 'NONE', #4834, #21879 ) ;
#13909=EDGE_CURVE ( 'NONE', #12870, #40212, #21481, .T. ) ;
#13910=DIRECTION ( 'NONE',  ( 0.005961354470445682716, -0.6427876096865404731, -0.7660212471507180654 ) ) ;
#13911=EDGE_CURVE ( 'NONE', #35631, #43670, #26854, .T. ) ;
#13912=DIRECTION ( 'NONE',  ( 0.005002170337468016433, -0.7660444431189770143, -0.6427681459581293666 ) ) ;
#13913=ORIENTED_EDGE ( 'NONE', *, *, #41797, .F. ) ;
#13914=EDGE_LOOP ( 'NONE', ( #38235, #3763, #46133 ) ) ;
#13915=PLANE ( 'NONE',  #40492 ) ;
#13917=ADVANCED_FACE ( 'NONE', ( #47876 ), #22320, .F. ) ;
#13918=AXIS2_PLACEMENT_3D ( 'NONE', #1026, #23205, #18355 ) ;
#13920=EDGE_CURVE ( 'NONE', #21318, #25308, #35113, .T. ) ;
#13921=CARTESIAN_POINT ( 'NONE',  ( -18.19747506107908563, 0.000000000000000000, 14.03856424583689311 ) ) ;
#13922=VECTOR ( 'NONE', #43803, 999.9999999999998863 ) ;
#13923=EDGE_LOOP ( 'NONE', ( #11, #25574, #25803, #9903 ) ) ;
#13924=CARTESIAN_POINT ( 'NONE',  ( -18.62532148412685018, 0.000000000000000000, 9.307451460975977753 ) ) ;
#13926=ORIENTED_EDGE ( 'NONE', *, *, #43235, .T. ) ;
#13927=EDGE_LOOP ( 'NONE', ( #37831, #34663, #16727, #52980 ) ) ;
#13928=EDGE_LOOP ( 'NONE', ( #12312, #691, #19905, #1295 ) ) ;
#13929=FACE_OUTER_BOUND ( 'NONE', #39780, .T. ) ;
#13930=VECTOR ( 'NONE', #35661, 1000.000000000000114 ) ;
#13931=LINE ( 'NONE', #30137, #46829 ) ;
#13932=CARTESIAN_POINT ( 'NONE',  ( -8.480943993241147894, -0.1191753592594194527, 6.512660236708999406 ) ) ;
#13933=VECTOR ( 'NONE', #33862, 1000.000000000000227 ) ;
#13934=EDGE_CURVE ( 'NONE', #44596, #56081, #48128, .T. ) ;
#13935=VECTOR ( 'NONE', #197, 1000.000000000000114 ) ;
#13936=LINE ( 'NONE', #5428, #17524 ) ;
#13938=ORIENTED_EDGE ( 'NONE', *, *, #47578, .F. ) ;
#13939=ADVANCED_FACE ( 'NONE', ( #44176 ), #9231, .F. ) ;
#13940=VECTOR ( 'NONE', #18066, 1000.000000000000227 ) ;
#13941=VECTOR ( 'NONE', #35487, 1000.000000000000000 ) ;
#13943=ORIENTED_EDGE ( 'NONE', *, *, #3204, .T. ) ;
#13944=FACE_OUTER_BOUND ( 'NONE', #13713, .T. ) ;
#13945=ORIENTED_EDGE ( 'NONE', *, *, #49315, .T. ) ;
#13946=DIRECTION ( 'NONE',  ( -0.005961354470445682716, -0.6427876096865404731, 0.7660212471507180654 ) ) ;
#13947=PLANE ( 'NONE',  #46666 ) ;
#13948=ORIENTED_EDGE ( 'NONE', *, *, #31451, .T. ) ;
#13949=DIRECTION ( 'NONE',  ( -0.7660212471507179544, -0.6427876096865405842, -0.005961354470445141482 ) ) ;
#13950=ORIENTED_EDGE ( 'NONE', *, *, #18053, .F. ) ;
#13951=DIRECTION ( 'NONE',  ( -0.005961354470445682716, -0.6427876096865404731, 0.7660212471507180654 ) ) ;
#13952=AXIS2_PLACEMENT_3D ( 'NONE', #45785, #45491, #28461 ) ;
#13953=ORIENTED_EDGE ( 'NONE', *, *, #7804, .F. ) ;
#13954=CARTESIAN_POINT ( 'NONE',  ( -9.808144436391993182, 0.000000000000000000, 10.77986332834118777 ) ) ;
#13955=DIRECTION ( 'NONE',  ( 0.5364919789714477361, 0.6444004775717706579, 0.5449076811759711036 ) ) ;
#13956=CARTESIAN_POINT ( 'NONE',  ( -12.44516864510371512, -4.889348428825665671, 1.559451445217089560 ) ) ;
#13958=ORIENTED_EDGE ( 'NONE', *, *, #43837, .F. ) ;
#13959=VECTOR ( 'NONE', #28486, 1000.000000000000227 ) ;
#13960=CARTESIAN_POINT ( 'NONE',  ( -19.60990026154428278, 0.000000000000000000, 4.498472333781370125 ) ) ;
#13961=DIRECTION ( 'NONE',  ( -0.6427681459581293666, -0.7660444431189770143, -0.005002170337467561935 ) ) ;
#13962=CARTESIAN_POINT ( 'NONE',  ( -30.79489622823572859, -0.1191753592594197858, 8.743409918460921304 ) ) ;
#13963=EDGE_CURVE ( 'NONE', #20216, #32474, #4990, .T. ) ;
#13964=EDGE_CURVE ( 'NONE', #83, #17803, #35644, .T. ) ;
#13965=VECTOR ( 'NONE', #48774, 999.9999999999998863 ) ;
#13966=CARTESIAN_POINT ( 'NONE',  ( -8.024318355659660895, 0.000000000000000000, 6.335291332000425157 ) ) ;
#13967=CARTESIAN_POINT ( 'NONE',  ( -11.22056963685719211, 0.000000000000000000, 1.239771416285661010 ) ) ;
#13969=CARTESIAN_POINT ( 'NONE',  ( -16.99924723426068951, 0.000000000000000000, 13.49389102713827171 ) ) ;
#13970=ORIENTED_EDGE ( 'NONE', *, *, #33491, .T. ) ;
#13971=LINE ( 'NONE', #23352, #45273 ) ;
#13972=CARTESIAN_POINT ( 'NONE',  ( -13.24358169501890714, -0.8417996532631553119, 3.207725259429178077 ) ) ;
#13973=LINE ( 'NONE', #31304, #43213 ) ;
#13974=ORIENTED_EDGE ( 'NONE', *, *, #44450, .F. ) ;
#13975=VECTOR ( 'NONE', #44041, 999.9999999999998863 ) ;
#13976=FACE_OUTER_BOUND ( 'NONE', #36976, .T. ) ;
#13978=ORIENTED_EDGE ( 'NONE', *, *, #47979, .T. ) ;
#13979=EDGE_CURVE ( 'NONE', #27886, #25181, #4157, .T. ) ;
#13981=EDGE_CURVE ( 'NONE', #50871, #21762, #30268, .T. ) ;
#13982=VECTOR ( 'NONE', #1728, 1000.000000000000114 ) ;
#13983=LINE ( 'NONE', #26767, #45232 ) ;
#13984=DIRECTION ( 'NONE',  ( 0.000000000000000000, -1.000000000000000000, 0.000000000000000000 ) ) ;
#13985=LINE ( 'NONE', #9751, #37794 ) ;
#13986=EDGE_CURVE ( 'NONE', #32747, #48737, #2398, .T. ) ;
#13987=DIRECTION ( 'NONE',  ( 0.000000000000000000, -0.000000000000000000, -1.000000000000000000 ) ) ;
#13988=VERTEX_POINT ( 'NONE', #27975 ) ;
#13989=VECTOR ( 'NONE', #9890, 999.9999999999998863 ) ;
#13990=VECTOR ( 'NONE', #52412, 1000.000000000000000 ) ;
#13991=EDGE_LOOP ( 'NONE', ( #51649, #42016, #13412, #43000 ) ) ;
#13992=CARTESIAN_POINT ( 'NONE',  ( -12.73074006674189995, 1.095915999411505082, 3.624957756920523355 ) ) ;
#13993=CARTESIAN_POINT ( 'NONE',  ( -20.77710809187043850, -5.375054281893166142, 4.780363120533749566 ) ) ;
#13995=DIRECTION ( 'NONE',  ( 0.007781995580012663651, 0.000000000000000000, -0.9999697198139515519 ) ) ;
#13996=DIRECTION ( 'NONE',  ( -0.9999697198139514409, -0.000000000000000000, -0.007781995580013368816 ) ) ;
#13997=ADVANCED_FACE ( 'NONE', ( #15441 ), #2095, .F. ) ;
#13998=CARTESIAN_POINT ( 'NONE',  ( -13.51773605596954120, 4.819660872929013351, 1.778907064336885391 ) ) ;
#13999=VERTEX_POINT ( 'NONE', #14617 ) ;
#14000=FACE_OUTER_BOUND ( 'NONE', #31900, .T. ) ;
#14001=EDGE_CURVE ( 'NONE', #33244, #38668, #31936, .T. ) ;
#14002=AXIS2_PLACEMENT_3D ( 'NONE', #53830, #14942, #5317 ) ;
#14003=CARTESIAN_POINT ( 'NONE',  ( -13.08330893211609869, 0.000000000000000000, 1.763933231766363630 ) ) ;
#14004=ORIENTED_EDGE ( 'NONE', *, *, #29654, .F. ) ;
#14005=VECTOR ( 'NONE', #880, 999.9999999999998863 ) ;
#14006=EDGE_CURVE ( 'NONE', #9106, #33688, #19429, .T. ) ;
#14007=DIRECTION ( 'NONE',  ( 0.9999697198139515519, 0.000000000000000000, 0.007781995580013368816 ) ) ;
#14008=CARTESIAN_POINT ( 'NONE',  ( -12.33850799832341849, 0.000000000000000000, 11.68350162852954632 ) ) ;
#14009=VECTOR ( 'NONE', #7761, 999.9999999999998863 ) ;
#14010=CARTESIAN_POINT ( 'NONE',  ( -19.52298068925090746, 0.000000000000000000, 5.237812901604549154 ) ) ;
#14011=ORIENTED_EDGE ( 'NONE', *, *, #38548, .T. ) ;
#14012=EDGE_CURVE ( 'NONE', #51326, #45566, #6386, .T. ) ;
#14013=FACE_OUTER_BOUND ( 'NONE', #9407, .T. ) ;
#14014=ORIENTED_EDGE ( 'NONE', *, *, #6847, .T. ) ;
#14015=ORIENTED_EDGE ( 'NONE', *, *, #447, .T. ) ;
#14016=ORIENTED_EDGE ( 'NONE', *, *, #30026, .F. ) ;
#14017=AXIS2_PLACEMENT_3D ( 'NONE', #20024, #19772, #53839 ) ;
#14018=ORIENTED_EDGE ( 'NONE', *, *, #15907, .T. ) ;
#14019=VECTOR ( 'NONE', #21270, 1000.000000000000000 ) ;
#14020=DIRECTION ( 'NONE',  ( -0.7660212471507179544, -0.6427876096865405842, -0.005961354470445141482 ) ) ;
#14021=EDGE_LOOP ( 'NONE', ( #26351, #14480, #45188 ) ) ;
#14022=DIRECTION ( 'NONE',  ( 0.007781995580012663651, -3.146120232559066537E-19, -0.9999697198139514409 ) ) ;
#14024=VECTOR ( 'NONE', #37995, 999.9999999999998863 ) ;
#14025=EDGE_LOOP ( 'NONE', ( #13104, #53545, #8198, #15663 ) ) ;
#14026=FACE_OUTER_BOUND ( 'NONE', #8000, .T. ) ;
#14027=ORIENTED_EDGE ( 'NONE', *, *, #15032, .T. ) ;
#14028=LINE ( 'NONE', #48948, #54917 ) ;
#14029=ORIENTED_EDGE ( 'NONE', *, *, #32844, .F. ) ;
#14030=VECTOR ( 'NONE', #10853, 999.9999999999998863 ) ;
#14031=CARTESIAN_POINT ( 'NONE',  ( -18.67619601524082285, 0.000000000000000000, 3.936400510096834893 ) ) ;
#14032=VECTOR ( 'NONE', #8067, 999.9999999999998863 ) ;
#14033=DIRECTION ( 'NONE',  ( 0.6427681459581294776, -0.7660444431189769032, 0.005002170337467562802 ) ) ;
#14034=CARTESIAN_POINT ( 'NONE',  ( -21.47341775636118655, -0.1191753592594197858, 5.122631121243466090 ) ) ;
#14035=DIRECTION ( 'NONE',  ( 0.007781995580012663651, 0.000000000000000000, -0.9999697198139515519 ) ) ;
#14036=PLANE ( 'NONE',  #51365 ) ;
#14037=DIRECTION ( 'NONE',  ( 0.5364919789714477361, 0.6444004775717706579, 0.5449076811759711036 ) ) ;
#14038=EDGE_LOOP ( 'NONE', ( #15985, #10119, #38131, #49581 ) ) ;
#14039=ADVANCED_FACE ( 'NONE', ( #19144 ), #32235, .F. ) ;
#14040=ORIENTED_EDGE ( 'NONE', *, *, #714, .F. ) ;
#14041=DIRECTION ( 'NONE',  ( 0.000000000000000000, -1.000000000000000000, 0.000000000000000000 ) ) ;
#14042=PLANE ( 'NONE',  #49351 ) ;
#14043=ADVANCED_FACE ( 'NONE', ( #23687 ), #31675, .F. ) ;
#14044=DIRECTION ( 'NONE',  ( 0.9999697198139515519, 0.000000000000000000, 0.007781995580013368816 ) ) ;
#14045=VECTOR ( 'NONE', #40867, 1000.000000000000227 ) ;
#14046=LINE ( 'NONE', #1249, #43042 ) ;
#14047=ORIENTED_EDGE ( 'NONE', *, *, #7076, .F. ) ;
#14048=AXIS2_PLACEMENT_3D ( 'NONE', #10816, #53677, #32941 ) ;
#14049=PLANE ( 'NONE',  #9544 ) ;
#14050=LINE ( 'NONE', #4680, #4172 ) ;
#14051=VERTEX_POINT ( 'NONE', #9821 ) ;
#14052=CARTESIAN_POINT ( 'NONE',  ( -10.94028622754223967, 0.000000000000000000, 11.14038480894692995 ) ) ;
#14053=DIRECTION ( 'NONE',  ( -0.9999697198139514409, -0.000000000000000000, -0.007781995580013368816 ) ) ;
#14054=VECTOR ( 'NONE', #7851, 999.9999999999998863 ) ;
#14055=VERTEX_POINT ( 'NONE', #19723 ) ;
#14056=ADVANCED_FACE ( 'NONE', ( #54349 ), #27126, .F. ) ;
#14057=ADVANCED_FACE ( 'NONE', ( #18606 ), #45021, .F. ) ;
#14058=ADVANCED_FACE ( 'NONE', ( #1818 ), #23154, .F. ) ;
#14059=CARTESIAN_POINT ( 'NONE',  ( -13.96745630169485786, 0.000000000000000000, 7.866371765625014945 ) ) ;
#14060=CARTESIAN_POINT ( 'NONE',  ( -14.04943075308655587, -0.1191753592594183703, 5.549738374539030517 ) ) ;
#14061=AXIS2_PLACEMENT_3D ( 'NONE', #3120, #55105, #50817 ) ;
#14062=CARTESIAN_POINT ( 'NONE',  ( -1.086233639165236964, 0.000000000000000000, -2.796443541562362078 ) ) ;
#14064=PLANE ( 'NONE',  #6071 ) ;
#14065=CARTESIAN_POINT ( 'NONE',  ( -16.85737050867004783, -0.1191753592594190225, 8.113210826735326009 ) ) ;
#14066=VERTEX_POINT ( 'NONE', #40752 ) ;
#14067=VECTOR ( 'NONE', #54309, 1000.000000000000227 ) ;
#14069=VERTEX_POINT ( 'NONE', #36468 ) ;
#14070=VECTOR ( 'NONE', #46581, 999.9999999999998863 ) ;
#14071=VECTOR ( 'NONE', #28763, 1000.000000000000000 ) ;
#14072=PLANE ( 'NONE',  #47511 ) ;
#14073=DIRECTION ( 'NONE',  ( -0.005961354470445682716, -0.6427876096865404731, 0.7660212471507180654 ) ) ;
#14074=CARTESIAN_POINT ( 'NONE',  ( -16.33317936670417225, 0.000000000000000000, 13.31440848639340224 ) ) ;
#14075=VECTOR ( 'NONE', #12851, 1000.000000000000227 ) ;
#14076=LINE ( 'NONE', #52962, #28244 ) ;
#14077=DIRECTION ( 'NONE',  ( -0.9999697198139514409, -0.000000000000000000, -0.007781995580013368816 ) ) ;
#14078=VERTEX_POINT ( 'NONE', #45537 ) ;
#14079=DIRECTION ( 'NONE',  ( 0.007781995580012663651, 0.000000000000000000, -0.9999697198139515519 ) ) ;
#14080=DIRECTION ( 'NONE',  ( 0.9999697198139515519, 0.000000000000000000, 0.007781995580013368816 ) ) ;
#14081=ADVANCED_FACE ( 'NONE', ( #23970 ), #5538, .F. ) ;
#14082=AXIS2_PLACEMENT_3D ( 'NONE', #25578, #12807, #55989 ) ;
#14083=ADVANCED_FACE ( 'NONE', ( #1266 ), #48979, .F. ) ;
#14084=DIRECTION ( 'NONE',  ( -0.7660212471507179544, -0.6427876096865405842, -0.005961354470445141482 ) ) ;
#14085=VECTOR ( 'NONE', #50123, 1000.000000000000227 ) ;
#14086=LINE ( 'NONE', #1276, #3355 ) ;
#14087=EDGE_CURVE ( 'NONE', #18849, #12775, #2658, .T. ) ;
#14088=ORIENTED_EDGE ( 'NONE', *, *, #23588, .T. ) ;
#14089=DIRECTION ( 'NONE',  ( 0.5364919789714477361, 0.6444004775717706579, 0.5449076811759711036 ) ) ;
#14090=ORIENTED_EDGE ( 'NONE', *, *, #38202, .F. ) ;
#14091=LINE ( 'NONE', #26867, #13231 ) ;
#14092=CARTESIAN_POINT ( 'NONE',  ( -25.20123094555300369, 0.000000000000000000, 6.470945668149052032 ) ) ;
#14094=EDGE_CURVE ( 'NONE', #22899, #50665, #25377, .T. ) ;
#14095=LINE ( 'NONE', #31422, #10877 ) ;
#14096=ORIENTED_EDGE ( 'NONE', *, *, #10290, .T. ) ;
#14098=AXIS2_PLACEMENT_3D ( 'NONE', #54608, #42129, #7792 ) ;
#14099=ORIENTED_EDGE ( 'NONE', *, *, #24436, .T. ) ;
#14100=ORIENTED_EDGE ( 'NONE', *, *, #17134, .T. ) ;
#14101=PLANE ( 'NONE',  #45671 ) ;
#14102=ORIENTED_EDGE ( 'NONE', *, *, #9002, .T. ) ;
#14103=AXIS2_PLACEMENT_3D ( 'NONE', #34288, #51322, #55282 ) ;
#14106=DIRECTION ( 'NONE',  ( -0.5364919789714478471, 0.6444004775717705469, -0.5449076811759709926 ) ) ;
#14107=VECTOR ( 'NONE', #21396, 999.9999999999998863 ) ;
#14108=EDGE_LOOP ( 'NONE', ( #1296, #6222, #18080, #32457 ) ) ;
#14109=ORIENTED_EDGE ( 'NONE', *, *, #276, .F. ) ;
#14110=DIRECTION ( 'NONE',  ( 0.9999697198139515519, 0.000000000000000000, 0.007781995580013368816 ) ) ;
#14111=ORIENTED_EDGE ( 'NONE', *, *, #53812, .F. ) ;
#14112=AXIS2_PLACEMENT_3D ( 'NONE', #18360, #39104, #9590 ) ;
#14113=VERTEX_POINT ( 'NONE', #21100 ) ;
#14114=VECTOR ( 'NONE', #11657, 999.9999999999998863 ) ;
#14116=DIRECTION ( 'NONE',  ( 0.6427681459581294776, -0.7660444431189769032, 0.005002170337467562802 ) ) ;
#14117=CARTESIAN_POINT ( 'NONE',  ( -11.14227222507966530, 0.000000000000000000, 3.087041093882136433 ) ) ;
#14118=DIRECTION ( 'NONE',  ( 0.005002170337468016433, -0.7660444431189770143, -0.6427681459581293666 ) ) ;
#14119=LINE ( 'NONE', #49018, #51320 ) ;
#14120=ORIENTED_EDGE ( 'NONE', *, *, #46873, .F. ) ;
#14121=DIRECTION ( 'NONE',  ( -0.9999697198139514409, -0.000000000000000000, -0.007781995580013368816 ) ) ;
#14122=ORIENTED_EDGE ( 'NONE', *, *, #27472, .F. ) ;
#14123=AXIS2_PLACEMENT_3D ( 'NONE', #2227, #45387, #45669 ) ;
#14124=AXIS2_PLACEMENT_3D ( 'NONE', #49203, #45237, #19380 ) ;
#14125=DIRECTION ( 'NONE',  ( -0.9999697198139514409, -0.000000000000000000, -0.007781995580013368816 ) ) ;
#14126=VECTOR ( 'NONE', #46760, 1000.000000000000227 ) ;
#14127=DIRECTION ( 'NONE',  ( -0.7660212471507179544, -0.6427876096865405842, -0.005961354470445141482 ) ) ;
#14128=VECTOR ( 'NONE', #51199, 1000.000000000000000 ) ;
#14129=DIRECTION ( 'NONE',  ( 0.000000000000000000, -0.000000000000000000, -1.000000000000000000 ) ) ;
#14130=DIRECTION ( 'NONE',  ( 0.6427681459581294776, -0.7660444431189769032, 0.005002170337467562802 ) ) ;
#14131=DIRECTION ( 'NONE',  ( 0.007781995580012662783, 0.000000000000000000, -0.9999697198139514409 ) ) ;
#14132=CARTESIAN_POINT ( 'NONE',  ( -28.92982233430281980, 0.000000000000000000, 7.919257187036034651 ) ) ;
#14133=FACE_OUTER_BOUND ( 'NONE', #51143, .T. ) ;
#14134=EDGE_LOOP ( 'NONE', ( #46691, #18431, #14720, #15523 ) ) ;
#14135=DIRECTION ( 'NONE',  ( 0.005002170337468016433, -0.7660444431189770143, -0.6427681459581293666 ) ) ;
#14136=EDGE_CURVE ( 'NONE', #53080, #56036, #46371, .T. ) ;
#14137=DIRECTION ( 'NONE',  ( -0.005961354470445682716, -0.6427876096865404731, 0.7660212471507180654 ) ) ;
#14138=CARTESIAN_POINT ( 'NONE',  ( -15.60102546347950536, 0.000000000000000000, 12.95077420755565356 ) ) ;
#14139=DIRECTION ( 'NONE',  ( -0.7660212471507179544, -0.6427876096865405842, -0.005961354470445141482 ) ) ;
#14141=DIRECTION ( 'NONE',  ( 0.007781995580012662783, 0.000000000000000000, -0.9999697198139514409 ) ) ;
#14142=EDGE_CURVE ( 'NONE', #12775, #17469, #29356, .T. ) ;
#14143=ADVANCED_FACE ( 'NONE', ( #33604 ), #41833, .F. ) ;
#14144=CARTESIAN_POINT ( 'NONE',  ( -11.44573815241757764, 9.034849713672558735, 1.227539821638981010 ) ) ;
#14145=AXIS2_PLACEMENT_3D ( 'NONE', #19077, #44633, #14550 ) ;
#14146=DIRECTION ( 'NONE',  ( -0.7660212471507179544, -0.6427876096865405842, -0.005961354470445141482 ) ) ;
#14148=AXIS2_PLACEMENT_3D ( 'NONE', #15226, #32541, #16057 ) ;
#14149=ORIENTED_EDGE ( 'NONE', *, *, #12090, .F. ) ;
#14150=CARTESIAN_POINT ( 'NONE',  ( -18.60364671047386409, 0.000000000000000000, 6.522289594208837471 ) ) ;
#14151=DIRECTION ( 'NONE',  ( 0.000000000000000000, -0.000000000000000000, -1.000000000000000000 ) ) ;
#14152=CARTESIAN_POINT ( 'NONE',  ( 2.072287782118878319, 0.000000000000000000, -2.950529333540147015 ) ) ;
#14153=AXIS2_PLACEMENT_3D ( 'NONE', #6644, #41565, #37288 ) ;
#14154=PLANE ( 'NONE',  #19198 ) ;
#14155=VECTOR ( 'NONE', #44550, 1000.000000000000227 ) ;
#14156=PLANE ( 'NONE',  #8560 ) ;
#14157=LINE ( 'NONE', #31744, #17769 ) ;
#14158=DIRECTION ( 'NONE',  ( 0.000000000000000000, -0.000000000000000000, -1.000000000000000000 ) ) ;
#14159=VECTOR ( 'NONE', #49919, 1000.000000000000227 ) ;
#14160=AXIS2_PLACEMENT_3D ( 'NONE', #54051, #14870, #45504 ) ;
#14161=CARTESIAN_POINT ( 'NONE',  ( -19.92672316015189082, 0.000000000000000000, 6.342667093759775554 ) ) ;
#14162=AXIS2_PLACEMENT_3D ( 'NONE', #39327, #114, #21995 ) ;
#14163=CARTESIAN_POINT ( 'NONE',  ( -18.33900375759556667, 0.000000000000000000, 6.524349106860843683 ) ) ;
#14164=VECTOR ( 'NONE', #43717, 1000.000000000000114 ) ;
#14165=EDGE_LOOP ( 'NONE', ( #24000, #19887, #49958, #27032 ) ) ;
#14166=VECTOR ( 'NONE', #15760, 999.9999999999998863 ) ;
#14167=ADVANCED_FACE ( 'NONE', ( #51214 ), #7483, .F. ) ;
#14168=VECTOR ( 'NONE', #53957, 999.9999999999998863 ) ;
#14169=ORIENTED_EDGE ( 'NONE', *, *, #22476, .F. ) ;
#14170=VECTOR ( 'NONE', #53853, 1000.000000000000227 ) ;
#14171=ORIENTED_EDGE ( 'NONE', *, *, #12478, .F. ) ;
#14173=ADVANCED_FACE ( 'NONE', ( #37299 ), #32764, .F. ) ;
#14174=EDGE_LOOP ( 'NONE', ( #54025, #21840, #21280, #39919 ) ) ;
#14175=DIRECTION ( 'NONE',  ( 0.9999697198139515519, 0.000000000000000000, 0.007781995580013368816 ) ) ;
#14176=DIRECTION ( 'NONE',  ( 0.005002170337468016433, -0.7660444431189770143, -0.6427681459581293666 ) ) ;
#14177=ORIENTED_EDGE ( 'NONE', *, *, #27192, .F. ) ;
#14178=EDGE_LOOP ( 'NONE', ( #9846, #16605, #49300, #12893 ) ) ;
#14179=ADVANCED_FACE ( 'NONE', ( #33898 ), #29066, .F. ) ;
#14180=EDGE_LOOP ( 'NONE', ( #54365, #43742, #14499, #25746 ) ) ;
#14181=VECTOR ( 'NONE', #35124, 999.9999999999998863 ) ;
#14182=FACE_OUTER_BOUND ( 'NONE', #30050, .T. ) ;
#14183=ORIENTED_EDGE ( 'NONE', *, *, #38408, .T. ) ;
#14184=DIRECTION ( 'NONE',  ( 0.007781995580012663651, 0.000000000000000000, -0.9999697198139515519 ) ) ;
#14185=DIRECTION ( 'NONE',  ( 0.5449076811759707706, 0.6444004775717708799, -0.5364919789714476250 ) ) ;
#14186=ORIENTED_EDGE ( 'NONE', *, *, #38633, .F. ) ;
#14187=VECTOR ( 'NONE', #38415, 999.9999999999998863 ) ;
#14188=DIRECTION ( 'NONE',  ( 0.9999697198139515519, 0.000000000000000000, 0.007781995580013368816 ) ) ;
#14189=EDGE_LOOP ( 'NONE', ( #21435, #10901, #325, #14662 ) ) ;
#14190=PLANE ( 'NONE',  #24586 ) ;
#14191=AXIS2_PLACEMENT_3D ( 'NONE', #14302, #19078, #53452 ) ;
#14192=CARTESIAN_POINT ( 'NONE',  ( -13.00656791945457513, 0.000000000000000000, 3.811196853325626854 ) ) ;
#14193=DIRECTION ( 'NONE',  ( 0.007781995580012662783, 0.000000000000000000, -0.9999697198139514409 ) ) ;
#14194=CARTESIAN_POINT ( 'NONE',  ( -13.82194518983451736, -3.756034771668161909, 2.130396849930530134 ) ) ;
#14195=VECTOR ( 'NONE', #36016, 999.9999999999998863 ) ;
#14196=ORIENTED_EDGE ( 'NONE', *, *, #18140, .F. ) ;
#14197=LINE ( 'NONE', #18425, #42136 ) ;
#14198=DIRECTION ( 'NONE',  ( 0.5449076811759707706, 0.6444004775717708799, -0.5364919789714476250 ) ) ;
#14200=ORIENTED_EDGE ( 'NONE', *, *, #7060, .T. ) ;
#14201=DIRECTION ( 'NONE',  ( 0.007781995580012663651, -3.146120232559066537E-19, -0.9999697198139514409 ) ) ;
#14202=ADVANCED_FACE ( 'NONE', ( #20825 ), #55756, .F. ) ;
#14204=ORIENTED_EDGE ( 'NONE', *, *, #24731, .F. ) ;
#14205=VECTOR ( 'NONE', #1411, 1000.000000000000227 ) ;
#14206=EDGE_CURVE ( 'NONE', #19740, #23008, #25118, .T. ) ;
#14207=VECTOR ( 'NONE', #3488, 1000.000000000000000 ) ;
#14208=CARTESIAN_POINT ( 'NONE',  ( -13.57131363945838487, -0.6798977022406551551, 3.069318792522690575 ) ) ;
#14209=CARTESIAN_POINT ( 'NONE',  ( -19.66637125327706670, -0.08393247865673328367, 7.012927507599523658 ) ) ;
#14210=DIRECTION ( 'NONE',  ( -0.9999697198139514409, -0.000000000000000000, -0.007781995580013368816 ) ) ;
#14211=LINE ( 'NONE', #10198, #15078 ) ;
#14212=LINE ( 'NONE', #4822, #48591 ) ;
#14213=FACE_OUTER_BOUND ( 'NONE', #2959, .T. ) ;
#14214=ADVANCED_FACE ( 'NONE', ( #3235 ), #28510, .F. ) ;
#14215=EDGE_CURVE ( 'NONE', #1477, #29979, #42426, .T. ) ;
#14216=DIRECTION ( 'NONE',  ( 0.6427681459581294776, -0.7660444431189769032, 0.005002170337467562802 ) ) ;
#14217=VECTOR ( 'NONE', #11277, 999.9999999999998863 ) ;
#14218=AXIS2_PLACEMENT_3D ( 'NONE', #5532, #49550, #31670 ) ;
#14219=LINE ( 'NONE', #14743, #23770 ) ;
#14221=DIRECTION ( 'NONE',  ( 0.6427681459581294776, -0.7660444431189769032, 0.005002170337467562802 ) ) ;
#14222=ORIENTED_EDGE ( 'NONE', *, *, #35132, .T. ) ;
#14223=DIRECTION ( 'NONE',  ( 0.005002170337468016433, -0.7660444431189770143, -0.6427681459581293666 ) ) ;
#14224=DIRECTION ( 'NONE',  ( 0.007781995580012663651, 0.000000000000000000, -0.9999697198139515519 ) ) ;
#14225=CARTESIAN_POINT ( 'NONE',  ( -15.88053067323646417, -0.1191753592594197858, 2.950163842912994383 ) ) ;
#14226=CARTESIAN_POINT ( 'NONE',  ( -14.06311187215340297, 3.200641362704009119, 7.596709105035338361 ) ) ;
#14227=DIRECTION ( 'NONE',  ( 0.5364919789714477361, 0.6444004775717706579, 0.5449076811759711036 ) ) ;
#14228=DIRECTION ( 'NONE',  ( 0.000000000000000000, -1.000000000000000000, 0.000000000000000000 ) ) ;
#14229=LINE ( 'NONE', #35792, #244 ) ;
#14230=VECTOR ( 'NONE', #21599, 1000.000000000000114 ) ;
#14231=EDGE_CURVE ( 'NONE', #6270, #3791, #46966, .T. ) ;
#14232=EDGE_LOOP ( 'NONE', ( #2558, #2732, #5566, #38370 ) ) ;
#14233=EDGE_LOOP ( 'NONE', ( #33286, #9349, #33928, #35869, #3401, #47912, #51791 ) ) ;
#14234=LINE ( 'NONE', #44569, #2357 ) ;
#14235=CARTESIAN_POINT ( 'NONE',  ( -13.09429047785683942, -0.1191753592594188005, 2.233182868755169803 ) ) ;
#14236=ORIENTED_EDGE ( 'NONE', *, *, #47960, .F. ) ;
#14237=FACE_OUTER_BOUND ( 'NONE', #15463, .T. ) ;
#14238=VECTOR ( 'NONE', #41639, 999.9999999999998863 ) ;
#14239=EDGE_LOOP ( 'NONE', ( #26228, #30726, #35219, #49169 ) ) ;
#14240=CARTESIAN_POINT ( 'NONE',  ( -24.26908309836554878, 0.000000000000000000, 6.108867788427308376 ) ) ;
#14241=VECTOR ( 'NONE', #40999, 1000.000000000000227 ) ;
#14242=ORIENTED_EDGE ( 'NONE', *, *, #10782, .T. ) ;
#14243=ORIENTED_EDGE ( 'NONE', *, *, #39865, .T. ) ;
#14244=EDGE_LOOP ( 'NONE', ( #45509, #22153, #48231, #53266 ) ) ;
#14245=CARTESIAN_POINT ( 'NONE',  ( -12.43497384774700265, -2.622721114510659035, 5.816430034565780005 ) ) ;
#14246=FACE_OUTER_BOUND ( 'NONE', #9674, .T. ) ;
#14247=DIRECTION ( 'NONE',  ( 0.5364919789714477361, 0.6444004775717706579, 0.5449076811759711036 ) ) ;
#14248=VECTOR ( 'NONE', #35158, 999.9999999999998863 ) ;
#14249=FACE_OUTER_BOUND ( 'NONE', #10748, .T. ) ;
#14250=ORIENTED_EDGE ( 'NONE', *, *, #42068, .T. ) ;
#14251=EDGE_CURVE ( 'NONE', #21588, #22086, #41575, .T. ) ;
#14252=ORIENTED_EDGE ( 'NONE', *, *, #28368, .F. ) ;
#14253=VECTOR ( 'NONE', #54004, 1000.000000000000227 ) ;
#14254=LINE ( 'NONE', #1145, #22778 ) ;
#14255=EDGE_LOOP ( 'NONE', ( #22914, #3812, #44266, #21872 ) ) ;
#14256=LINE ( 'NONE', #18792, #25717 ) ;
#14257=ORIENTED_EDGE ( 'NONE', *, *, #45073, .T. ) ;
#14258=FACE_OUTER_BOUND ( 'NONE', #52147, .T. ) ;
#14259=DIRECTION ( 'NONE',  ( -0.6246952433987893460, -0.7422098413412802076, 0.2426528472758542054 ) ) ;
#14260=EDGE_CURVE ( 'NONE', #38668, #23390, #16560, .T. ) ;
#14261=ORIENTED_EDGE ( 'NONE', *, *, #2189, .F. ) ;
#14262=FACE_OUTER_BOUND ( 'NONE', #43436, .T. ) ;
#14263=VERTEX_POINT ( 'NONE', #4375 ) ;
#14264=EDGE_CURVE ( 'NONE', #56189, #21908, #51763, .T. ) ;
#14265=ADVANCED_FACE ( 'NONE', ( #13703 ), #21686, .F. ) ;
#14266=DIRECTION ( 'NONE',  ( 0.007781995580012663651, 0.000000000000000000, -0.9999697198139515519 ) ) ;
#14267=EDGE_LOOP ( 'NONE', ( #21704, #48508, #33653, #52133 ) ) ;
#14268=DIRECTION ( 'NONE',  ( -0.6427681459581293666, -0.7660444431189770143, -0.005002170337467561935 ) ) ;
#14269=CARTESIAN_POINT ( 'NONE',  ( -19.95699008208018199, 0.2864062442990042978, 4.424766562912388679 ) ) ;
#14270=CARTESIAN_POINT ( 'NONE',  ( -11.40636015113596180, 0.000000000000000000, 11.32142374880780089 ) ) ;
#14271=EDGE_CURVE ( 'NONE', #10033, #34166, #34200, .T. ) ;
#14272=ORIENTED_EDGE ( 'NONE', *, *, #19595, .T. ) ;
#14273=ADVANCED_FACE ( 'NONE', ( #17699 ), #25645, .F. ) ;
#14274=FACE_OUTER_BOUND ( 'NONE', #41014, .T. ) ;
#14275=AXIS2_PLACEMENT_3D ( 'NONE', #4089, #47524, #17409 ) ;
#14276=FACE_OUTER_BOUND ( 'NONE', #12038, .T. ) ;
#14278=FACE_OUTER_BOUND ( 'NONE', #3260, .T. ) ;
#14279=EDGE_CURVE ( 'NONE', #15160, #21771, #35041, .T. ) ;
#14280=FACE_OUTER_BOUND ( 'NONE', #10051, .T. ) ;
#14281=VECTOR ( 'NONE', #54600, 999.9999999999998863 ) ;
#14283=VERTEX_POINT ( 'NONE', #26776 ) ;
#14285=LINE ( 'NONE', #31303, #31345 ) ;
#14286=DIRECTION ( 'NONE',  ( 0.9999697198139515519, 0.000000000000000000, 0.007781995580013368816 ) ) ;
#14287=ORIENTED_EDGE ( 'NONE', *, *, #35606, .F. ) ;
#14288=CARTESIAN_POINT ( 'NONE',  ( -13.73672976910459909, 0.000000000000000000, 12.22661844811216270 ) ) ;
#14289=CARTESIAN_POINT ( 'NONE',  ( -26.13493519185646008, 0.000000000000000000, 7.033017491833586377 ) ) ;
#14290=ORIENTED_EDGE ( 'NONE', *, *, #10852, .F. ) ;
#14292=CARTESIAN_POINT ( 'NONE',  ( -16.33317936670417225, 0.000000000000000000, 13.31440848639340224 ) ) ;
#14293=VECTOR ( 'NONE', #5516, 1000.000000000000114 ) ;
#14294=CARTESIAN_POINT ( 'NONE',  ( -11.12790195755325229, 0.000000000000000000, 1.240492577593313550 ) ) ;
#14295=LINE ( 'NONE', #22522, #50514 ) ;
#14296=LINE ( 'NONE', #31013, #47361 ) ;
#14297=EDGE_CURVE ( 'NONE', #41331, #5666, #52047, .T. ) ;
#14298=ORIENTED_EDGE ( 'NONE', *, *, #51998, .T. ) ;
#14299=EDGE_LOOP ( 'NONE', ( #23315, #35898, #40764, #36508 ) ) ;
#14300=LINE ( 'NONE', #48337, #41224 ) ;
#14301=FACE_OUTER_BOUND ( 'NONE', #1895, .T. ) ;
#14302=CARTESIAN_POINT ( 'NONE',  ( -31.72626587586518099, 0.000000000000000000, 9.005490826201270949 ) ) ;
#14303=DIRECTION ( 'NONE',  ( -0.6427681459581293666, -0.7660444431189770143, -0.005002170337467561935 ) ) ;
#14304=DIRECTION ( 'NONE',  ( 0.9999697198139515519, 0.000000000000000000, 0.007781995580013368816 ) ) ;
#14305=ORIENTED_EDGE ( 'NONE', *, *, #24384, .T. ) ;
#14306=DIRECTION ( 'NONE',  ( 0.5449076811759707706, 0.6444004775717708799, -0.5364919789714476250 ) ) ;
#14307=VERTEX_POINT ( 'NONE', #48338 ) ;
#14308=CARTESIAN_POINT ( 'NONE',  ( -9.483718581678113324, 0.000000000000000000, 3.099948341838171029 ) ) ;
#14310=VERTEX_POINT ( 'NONE', #22240 ) ;
#14311=DIRECTION ( 'NONE',  ( 0.000000000000000000, -0.000000000000000000, -1.000000000000000000 ) ) ;
#14312=CARTESIAN_POINT ( 'NONE',  ( -17.39286377064282618, -2.460819163488160655, 3.558787054721057608 ) ) ;
#14313=FACE_OUTER_BOUND ( 'NONE', #42703, .T. ) ;
#14314=ORIENTED_EDGE ( 'NONE', *, *, #32674, .F. ) ;
#14315=DIRECTION ( 'NONE',  ( 0.7660212471507180654, -0.6427876096865404731, 0.005961354470445141482 ) ) ;
#14316=EDGE_CURVE ( 'NONE', #52765, #19601, #12872, .T. ) ;
#14317=ORIENTED_EDGE ( 'NONE', *, *, #21708, .F. ) ;
#14318=ORIENTED_EDGE ( 'NONE', *, *, #40133, .T. ) ;
#14319=AXIS2_PLACEMENT_3D ( 'NONE', #9534, #47877, #13770 ) ;
#14320=ORIENTED_EDGE ( 'NONE', *, *, #46120, .T. ) ;
#14321=ORIENTED_EDGE ( 'NONE', *, *, #30611, .F. ) ;
#14322=PLANE ( 'NONE',  #12127 ) ;
#14323=ORIENTED_EDGE ( 'NONE', *, *, #19241, .T. ) ;
#14324=FACE_OUTER_BOUND ( 'NONE', #49652, .T. ) ;
#14325=CARTESIAN_POINT ( 'NONE',  ( 2.072287782118878319, 0.000000000000000000, -2.950529333540147015 ) ) ;
#14326=VECTOR ( 'NONE', #38718, 999.9999999999998863 ) ;
#14327=ORIENTED_EDGE ( 'NONE', *, *, #40443, .F. ) ;
#14328=ORIENTED_EDGE ( 'NONE', *, *, #39049, .T. ) ;
#14329=DIRECTION ( 'NONE',  ( 0.005002170337468016433, -0.7660444431189770143, -0.6427681459581293666 ) ) ;
#14330=ORIENTED_EDGE ( 'NONE', *, *, #29223, .T. ) ;
#14331=ADVANCED_FACE ( 'NONE', ( #39271 ), #52352, .F. ) ;
#14332=PLANE ( 'NONE',  #48228 ) ;
#14333=DIRECTION ( 'NONE',  ( 0.000000000000000000, 0.000000000000000000, -1.000000000000000000 ) ) ;
#14334=LINE ( 'NONE', #31647, #54961 ) ;
#14335=DIRECTION ( 'NONE',  ( 0.9999697198139515519, 0.000000000000000000, 0.007781995580013368816 ) ) ;
#14336=CARTESIAN_POINT ( 'NONE',  ( -27.99767448711536133, 0.000000000000000000, 7.557179307314289218 ) ) ;
#14337=DIRECTION ( 'NONE',  ( 0.9999697198139515519, 0.000000000000000000, 0.007781995580013368816 ) ) ;
#14338=EDGE_LOOP ( 'NONE', ( #33561, #26955, #50024, #48742 ) ) ;
#14339=ORIENTED_EDGE ( 'NONE', *, *, #7271, .F. ) ;
#14340=ADVANCED_FACE ( 'NONE', ( #52606 ), #42975, .F. ) ;
#14341=DIRECTION ( 'NONE',  ( 0.7660212471507180654, -0.6427876096865404731, 0.005961354470445141482 ) ) ;
#14342=CARTESIAN_POINT ( 'NONE',  ( -10.87188116519080694, 0.000000000000000000, 2.350481200018612160 ) ) ;
#14343=ADVANCED_FACE ( 'NONE', ( #43527 ), #51511, .F. ) ;
#14344=CARTESIAN_POINT ( 'NONE',  ( -16.93227919866189879, 0.000000000000000000, 4.888642269838840093 ) ) ;
#14345=PLANE ( 'NONE',  #15874 ) ;
#14346=EDGE_LOOP ( 'NONE', ( #51862, #26308, #33275, #27783 ) ) ;
#14348=DIRECTION ( 'NONE',  ( -0.9999697198139514409, -0.000000000000000000, -0.007781995580013368816 ) ) ;
#14349=ORIENTED_EDGE ( 'NONE', *, *, #11909, .T. ) ;
#14350=DIRECTION ( 'NONE',  ( 0.7660212471507180654, -0.6427876096865404731, 0.005961354470445141482 ) ) ;
#14351=CARTESIAN_POINT ( 'NONE',  ( -25.20278734466900517, 0.000000000000000000, 6.670939612111840944 ) ) ;
#14352=VERTEX_POINT ( 'NONE', #21411 ) ;
#14353=ADVANCED_FACE ( 'NONE', ( #47514 ), #4079, .F. ) ;
#14355=DIRECTION ( 'NONE',  ( 0.5364919789714477361, 0.6444004775717706579, 0.5449076811759711036 ) ) ;
#14356=CARTESIAN_POINT ( 'NONE',  ( -20.21494452004282394, 3.362543313726509719, 4.426819948926248749 ) ) ;
#14357=PLANE ( 'NONE',  #30510 ) ;
#14358=LINE ( 'NONE', #31086, #35573 ) ;
#14359=EDGE_CURVE ( 'NONE', #31186, #51745, #47814, .T. ) ;
#14360=ORIENTED_EDGE ( 'NONE', *, *, #22632, .T. ) ;
#14361=VERTEX_POINT ( 'NONE', #39575 ) ;
#14362=CARTESIAN_POINT ( 'NONE',  ( -11.25873531853475384, -0.1191753592594179401, 5.202124141889320263 ) ) ;
#14363=CARTESIAN_POINT ( 'NONE',  ( -18.86354292863559579, 0.000000000000000000, 14.21804678658176080 ) ) ;
#14364=LINE ( 'NONE', #18607, #36970 ) ;
#14365=AXIS2_PLACEMENT_3D ( 'NONE', #31926, #36206, #5818 ) ;
#14366=CARTESIAN_POINT ( 'NONE',  ( -9.746805135440405721, 0.000000000000000000, 2.897894885223375461 ) ) ;
#14367=DIRECTION ( 'NONE',  ( 0.9999697198139515519, 0.000000000000000000, 0.007781995580013368816 ) ) ;
#14368=VERTEX_POINT ( 'NONE', #17142 ) ;
#14370=DIRECTION ( 'NONE',  ( 0.5449076811759707706, 0.6444004775717708799, -0.5364919789714476250 ) ) ;
#14371=DIRECTION ( 'NONE',  ( -0.6427681459581293666, -0.7660444431189770143, -0.005002170337467561935 ) ) ;
#14372=DIRECTION ( 'NONE',  ( 0.005961354470445682716, -0.6427876096865404731, -0.7660212471507180654 ) ) ;
#14373=VERTEX_POINT ( 'NONE', #8626 ) ;
#14374=LINE ( 'NONE', #27988, #25659 ) ;
#14375=ORIENTED_EDGE ( 'NONE', *, *, #56069, .F. ) ;
#14376=PLANE ( 'NONE',  #6862 ) ;
#14377=EDGE_CURVE ( 'NONE', #41210, #16962, #17985, .T. ) ;
#14378=DIRECTION ( 'NONE',  ( 0.6427681459581294776, -0.7660444431189769032, 0.005002170337467562802 ) ) ;
#14380=FACE_OUTER_BOUND ( 'NONE', #47605, .T. ) ;
#14381=EDGE_CURVE ( 'NONE', #22565, #38766, #8920, .T. ) ;
#14382=ORIENTED_EDGE ( 'NONE', *, *, #15105, .F. ) ;
#14383=VERTEX_POINT ( 'NONE', #53195 ) ;
#14384=ORIENTED_EDGE ( 'NONE', *, *, #30299, .T. ) ;
#14386=ORIENTED_EDGE ( 'NONE', *, *, #51082, .F. ) ;
#14388=VERTEX_POINT ( 'NONE', #48916 ) ;
#14389=FACE_OUTER_BOUND ( 'NONE', #43151, .T. ) ;
#14390=DIRECTION ( 'NONE',  ( 0.007781995580012663651, 0.000000000000000000, -0.9999697198139515519 ) ) ;
#14391=VERTEX_POINT ( 'NONE', #5472 ) ;
#14392=ADVANCED_FACE ( 'NONE', ( #48648 ), #22786, .F. ) ;
#14393=EDGE_CURVE ( 'NONE', #44862, #18734, #49179, .T. ) ;
#14394=ADVANCED_FACE ( 'NONE', ( #1496 ), #27619, .F. ) ;
#14397=ORIENTED_EDGE ( 'NONE', *, *, #19755, .F. ) ;
#14398=ORIENTED_EDGE ( 'NONE', *, *, #25470, .F. ) ;
#14399=LINE ( 'NONE', #31711, #51038 ) ;
#14400=CARTESIAN_POINT ( 'NONE',  ( -15.60102546347950536, 0.000000000000000000, 12.95077420755565356 ) ) ;
#14401=CARTESIAN_POINT ( 'NONE',  ( -12.75342118059741026, 0.000000000000000000, 5.290495179008689597 ) ) ;
#14402=CARTESIAN_POINT ( 'NONE',  ( -16.36686713028141682, -0.1191753592594189115, 4.793039409183453614 ) ) ;
#14403=VERTEX_POINT ( 'NONE', #27913 ) ;
#14404=LINE ( 'NONE', #6998, #44671 ) ;
#14405=ORIENTED_EDGE ( 'NONE', *, *, #5787, .F. ) ;
#14406=AXIS2_PLACEMENT_3D ( 'NONE', #27053, #44362, #655 ) ;
#14407=EDGE_CURVE ( 'NONE', #28407, #35510, #27322, .T. ) ;
#14408=DIRECTION ( 'NONE',  ( 0.6427681459581294776, -0.7660444431189769032, 0.005002170337467562802 ) ) ;
#14409=EDGE_CURVE ( 'NONE', #27150, #45223, #44939, .T. ) ;
#14410=DIRECTION ( 'NONE',  ( -0.9999697198139514409, -0.000000000000000000, -0.007781995580013368816 ) ) ;
#14411=DIRECTION ( 'NONE',  ( 0.9999697198139515519, 0.000000000000000000, 0.007781995580013368816 ) ) ;
#14412=DIRECTION ( 'NONE',  ( 0.007781995580012663651, 0.000000000000000000, -0.9999697198139515519 ) ) ;
#14413=EDGE_CURVE ( 'NONE', #2309, #18910, #10598, .T. ) ;
#14414=CARTESIAN_POINT ( 'NONE',  ( -13.69131713479542967, 0.000000000000000000, 6.391192465245965515 ) ) ;
#14415=CARTESIAN_POINT ( 'NONE',  ( -27.99923088623136636, 0.000000000000000000, 7.757173251277078130 ) ) ;
#14416=VERTEX_POINT ( 'NONE', #2020 ) ;
#14417=CARTESIAN_POINT ( 'NONE',  ( -19.60834386242827776, 0.000000000000000000, 4.298478389818581213 ) ) ;
#14418=ORIENTED_EDGE ( 'NONE', *, *, #8216, .T. ) ;
#14419=ADVANCED_FACE ( 'NONE', ( #31865 ), #6058, .F. ) ;
#14420=CARTESIAN_POINT ( 'NONE',  ( -15.90510428694561718, -0.1191753592594205907, 5.165965024209228318 ) ) ;
#14421=LINE ( 'NONE', #53570, #18730 ) ;
#14422=CARTESIAN_POINT ( 'NONE',  ( -19.32568712495613639, 5.629170628041515023, 4.009084898942861130 ) ) ;
#14423=FACE_OUTER_BOUND ( 'NONE', #48996, .T. ) ;
#14424=ADVANCED_FACE ( 'NONE', ( #36402 ), #45471, .F. ) ;
#14425=CARTESIAN_POINT ( 'NONE',  ( -9.075990533167328067, 0.000000000000000000, 10.41622904950343909 ) ) ;
#14427=ORIENTED_EDGE ( 'NONE', *, *, #246, .F. ) ;
#14429=LINE ( 'NONE', #6193, #12208 ) ;
#14430=DIRECTION ( 'NONE',  ( 0.6427681459581294776, -0.7660444431189769032, 0.005002170337467562802 ) ) ;
#14431=CARTESIAN_POINT ( 'NONE',  ( -29.86352658060627618, 0.000000000000000000, 8.481329010720569883 ) ) ;
#14432=DIRECTION ( 'NONE',  ( 0.9999697198139515519, 0.000000000000000000, 0.007781995580013368816 ) ) ;
#14433=CARTESIAN_POINT ( 'NONE',  ( -10.94028622754223967, 0.000000000000000000, 11.14038480894692995 ) ) ;
#14434=LINE ( 'NONE', #14981, #3835 ) ;
#14435=CARTESIAN_POINT ( 'NONE',  ( -17.18579816256228554, 0.000000000000000000, 3.457174062837659712 ) ) ;
#14436=CARTESIAN_POINT ( 'NONE',  ( 2.072287782118878319, 0.000000000000000000, -2.950529333540147015 ) ) ;
#14437=ORIENTED_EDGE ( 'NONE', *, *, #15621, .F. ) ;
#14438=VERTEX_POINT ( 'NONE', #1757 ) ;
#14439=ORIENTED_EDGE ( 'NONE', *, *, #55422, .F. ) ;
#14440=ORIENTED_EDGE ( 'NONE', *, *, #19188, .T. ) ;
#14441=ORIENTED_EDGE ( 'NONE', *, *, #52843, .F. ) ;
#14442=LINE ( 'NONE', #6469, #9670 ) ;
#14443=CARTESIAN_POINT ( 'NONE',  ( -8.575880816922197170, 0.000000000000000000, 5.861663847473516320 ) ) ;
#14444=ADVANCED_FACE ( 'NONE', ( #14301 ), #23621, .F. ) ;
#14446=EDGE_LOOP ( 'NONE', ( #7319, #1070, #45576, #37626 ) ) ;
#14447=ORIENTED_EDGE ( 'NONE', *, *, #1863, .T. ) ;
#14448=EDGE_LOOP ( 'NONE', ( #43822, #14513, #29833, #51984, #56125 ) ) ;
#14449=EDGE_CURVE ( 'NONE', #43897, #12199, #40936, .T. ) ;
#14450=FACE_OUTER_BOUND ( 'NONE', #10162, .T. ) ;
#14451=LINE ( 'NONE', #27494, #21895 ) ;
#14452=PLANE ( 'NONE',  #22310 ) ;
#14453=VERTEX_POINT ( 'NONE', #6582 ) ;
#14454=DIRECTION ( 'NONE',  ( 0.005961354470445682716, -0.6427876096865404731, -0.7660212471507180654 ) ) ;
#14455=ORIENTED_EDGE ( 'NONE', *, *, #25709, .F. ) ;
#14456=DIRECTION ( 'NONE',  ( 0.5364919789714477361, 0.6444004775717706579, 0.5449076811759711036 ) ) ;
#14457=CARTESIAN_POINT ( 'NONE',  ( -27.06552663992790997, 0.000000000000000000, 7.195101427592543786 ) ) ;
#14458=CARTESIAN_POINT ( 'NONE',  ( -9.110551994824897193, 0.000000000000000000, 3.538847790438064411 ) ) ;
#14459=DIRECTION ( 'NONE',  ( -0.7660212471507179544, -0.6427876096865405842, -0.005961354470445141482 ) ) ;
#14460=CARTESIAN_POINT ( 'NONE',  ( -20.76273478851211607, 4.495856970884009485, 12.32473963750469359 ) ) ;
#14461=CARTESIAN_POINT ( 'NONE',  ( -18.16733880988877914, -1.165603555308156514, 3.900943620346350116 ) ) ;
#14462=DIRECTION ( 'NONE',  ( -0.5364919789714478471, 0.6444004775717705469, -0.5449076811759709926 ) ) ;
#14463=ORIENTED_EDGE ( 'NONE', *, *, #18114, .T. ) ;
#14464=LINE ( 'NONE', #36316, #7441 ) ;
#14465=ORIENTED_EDGE ( 'NONE', *, *, #34594, .F. ) ;
#14466=EDGE_LOOP ( 'NONE', ( #49061, #37905, #27081, #21159 ) ) ;
#14467=EDGE_CURVE ( 'NONE', #41178, #5706, #23898, .T. ) ;
#14468=DIRECTION ( 'NONE',  ( 0.7660212471507180654, -0.6427876096865404731, 0.005961354470445141482 ) ) ;
#14469=PLANE ( 'NONE',  #561 ) ;
#14470=DIRECTION ( 'NONE',  ( 0.5449076811759707706, 0.6444004775717708799, -0.5364919789714476250 ) ) ;
#14472=CARTESIAN_POINT ( 'NONE',  ( -20.91752765554880966, 5.305366725996514710, 4.637740859931800408 ) ) ;
#14473=EDGE_CURVE ( 'NONE', #51439, #9864, #52881, .T. ) ;
#14474=CARTESIAN_POINT ( 'NONE',  ( -23.33849165029409889, 0.000000000000000000, 5.946783852668351855 ) ) ;
#14476=FACE_OUTER_BOUND ( 'NONE', #9528, .T. ) ;
#14477=( NAMED_UNIT ( * ) SI_UNIT ( $, .STERADIAN. ) SOLID_ANGLE_UNIT ( ) );
#14478=ADVANCED_FACE ( 'NONE', ( #44369 ), #1193, .F. ) ;
#14479=LINE ( 'NONE', #19844, #46846 ) ;
#14480=ORIENTED_EDGE ( 'NONE', *, *, #7427, .T. ) ;
#14481=CARTESIAN_POINT ( 'NONE',  ( -15.03495456790438389, -0.1191753592594197858, 12.77051346725278158 ) ) ;
#14484=EDGE_CURVE ( 'NONE', #6551, #8206, #32983, .T. ) ;
#14485=DIRECTION ( 'NONE',  ( 0.007781995580012663651, -3.146120232559066537E-19, -0.9999697198139514409 ) ) ;
#14486=EDGE_CURVE ( 'NONE', #31864, #46689, #16220, .T. ) ;
#14487=CARTESIAN_POINT ( 'NONE',  ( -20.28887480193589354, 0.000000000000000000, 4.662514410496616968 ) ) ;
#14488=CARTESIAN_POINT ( 'NONE',  ( 2.072287782118878319, 0.000000000000000000, -2.950529333540147015 ) ) ;
#14489=DIRECTION ( 'NONE',  ( -0.5449076811759708816, 0.6444004775717707689, 0.5364919789714475140 ) ) ;
#14490=ORIENTED_EDGE ( 'NONE', *, *, #41667, .F. ) ;
#14491=ORIENTED_EDGE ( 'NONE', *, *, #26090, .T. ) ;
#14493=DIRECTION ( 'NONE',  ( -0.6427681459581293666, -0.7660444431189770143, -0.005002170337467561935 ) ) ;
#14494=ORIENTED_EDGE ( 'NONE', *, *, #17975, .F. ) ;
#14495=PLANE ( 'NONE',  #24976 ) ;
#14496=EDGE_LOOP ( 'NONE', ( #8817, #38861, #19699, #40208 ) ) ;
#14497=DIRECTION ( 'NONE',  ( 0.5449076811759707706, 0.6444004775717708799, -0.5364919789714476250 ) ) ;
#14498=ORIENTED_EDGE ( 'NONE', *, *, #13468, .T. ) ;
#14499=ORIENTED_EDGE ( 'NONE', *, *, #27808, .T. ) ;
#14500=ORIENTED_EDGE ( 'NONE', *, *, #18748, .F. ) ;
#14501=LINE ( 'NONE', #14245, #14798 ) ;
#14502=DIRECTION ( 'NONE',  ( 0.007781995580012663651, -3.146120232559066537E-19, -0.9999697198139514409 ) ) ;
#14503=CARTESIAN_POINT ( 'NONE',  ( -16.33317936670417225, 0.000000000000000000, 13.31440848639340224 ) ) ;
#14504=EDGE_CURVE ( 'NONE', #883, #37296, #55390, .T. ) ;
#14505=CARTESIAN_POINT ( 'NONE',  ( -10.68050938174386566, 0.000000000000000000, 3.459966708907908473 ) ) ;
#14506=ORIENTED_EDGE ( 'NONE', *, *, #49719, .T. ) ;
#14507=ORIENTED_EDGE ( 'NONE', *, *, #33185, .F. ) ;
#14509=EDGE_CURVE ( 'NONE', #48572, #21088, #46899, .T. ) ;
#14510=DIRECTION ( 'NONE',  ( -0.9999697198139514409, -0.000000000000000000, -0.007781995580013368816 ) ) ;
#14511=ORIENTED_EDGE ( 'NONE', *, *, #19422, .T. ) ;
#14512=PLANE ( 'NONE',  #23723 ) ;
#14513=ORIENTED_EDGE ( 'NONE', *, *, #20725, .T. ) ;
#14515=FACE_OUTER_BOUND ( 'NONE', #49183, .T. ) ;
#14516=ORIENTED_EDGE ( 'NONE', *, *, #20459, .T. ) ;
#14518=ORIENTED_EDGE ( 'NONE', *, *, #22764, .T. ) ;
#14521=ORIENTED_EDGE ( 'NONE', *, *, #15449, .F. ) ;
#14522=CARTESIAN_POINT ( 'NONE',  ( -18.39746900504187010, 0.000000000000000000, 14.03700784672088808 ) ) ;
#14523=PLANE ( 'NONE',  #32064 ) ;
#14524=CARTESIAN_POINT ( 'NONE',  ( -13.99298162533602152, -5.536956232915663634, 11.20436947665652561 ) ) ;
#14525=ORIENTED_EDGE ( 'NONE', *, *, #21246, .T. ) ;
#14526=CARTESIAN_POINT ( 'NONE',  ( -14.53418602446461705, -0.1191753592594185784, 8.131290385575372426 ) ) ;
#14527=LINE ( 'NONE', #10266, #46839 ) ;
#14528=DIRECTION ( 'NONE',  ( -0.9999697198139514409, -0.000000000000000000, -0.007781995580013368816 ) ) ;
#14530=EDGE_CURVE ( 'NONE', #31964, #16497, #3447, .T. ) ;
#14531=DIRECTION ( 'NONE',  ( 0.005002170337468016433, -0.7660444431189770143, -0.6427681459581293666 ) ) ;
#14532=LINE ( 'NONE', #49159, #30656 ) ;
#14533=VECTOR ( 'NONE', #13830, 999.9999999999998863 ) ;
#14535=VERTEX_POINT ( 'NONE', #16489 ) ;
#14536=DIRECTION ( 'NONE',  ( 0.007781995580012662783, 0.000000000000000000, -0.9999697198139514409 ) ) ;
#14537=ADVANCED_FACE ( 'NONE', ( #41226 ), #29272, .F. ) ;
#14538=LINE ( 'NONE', #22770, #18665 ) ;
#14540=ORIENTED_EDGE ( 'NONE', *, *, #46673, .F. ) ;
#14541=LINE ( 'NONE', #22773, #10257 ) ;
#14542=DIRECTION ( 'NONE',  ( 0.005961354470445682716, -0.6427876096865404731, -0.7660212471507180654 ) ) ;
#14543=ORIENTED_EDGE ( 'NONE', *, *, #44578, .F. ) ;
#14544=EDGE_CURVE ( 'NONE', #98, #23644, #36987, .T. ) ;
#14545=DIRECTION ( 'NONE',  ( -0.8531650599175527594, 0.4028455766673922356, 0.3313982828793700652 ) ) ;
#14546=DIRECTION ( 'NONE',  ( 0.9999697198139515519, 0.000000000000000000, 0.007781995580013368816 ) ) ;
#14548=ORIENTED_EDGE ( 'NONE', *, *, #4648, .T. ) ;
#14549=ORIENTED_EDGE ( 'NONE', *, *, #28827, .T. ) ;
#14550=DIRECTION ( 'NONE',  ( 0.000000000000000000, -0.000000000000000000, -1.000000000000000000 ) ) ;
#14551=LINE ( 'NONE', #35306, #23265 ) ;
#14553=CARTESIAN_POINT ( 'NONE',  ( -13.35659999714346391, 4.010151117816509903, 8.650819319289523079 ) ) ;
#14554=CARTESIAN_POINT ( 'NONE',  ( -27.06552663992790997, 0.000000000000000000, 7.195101427592543786 ) ) ;
#14555=ORIENTED_EDGE ( 'NONE', *, *, #45635, .F. ) ;
#14556=CARTESIAN_POINT ( 'NONE',  ( -14.10280672071693431, -0.1191753592594197858, 12.40843558753103792 ) ) ;
#14557=VERTEX_POINT ( 'NONE', #15643 ) ;
#14558=ADVANCED_FACE ( 'NONE', ( #50848 ), #42050, .F. ) ;
#14560=ADVANCED_FACE ( 'NONE', ( #41759 ), #28434, .F. ) ;
#14562=ORIENTED_EDGE ( 'NONE', *, *, #33488, .T. ) ;
#14563=DIRECTION ( 'NONE',  ( 0.9999697198139515519, 0.000000000000000000, 0.007781995580013368816 ) ) ;
#14564=EDGE_CURVE ( 'NONE', #35585, #50536, #46589, .T. ) ;
#14565=CARTESIAN_POINT ( 'NONE',  ( -12.16214263066938628, -0.1191753592594194527, 1.871104989033428145 ) ) ;
#14566=DIRECTION ( 'NONE',  ( 0.005002170337468016433, -0.7660444431189770143, -0.6427681459581293666 ) ) ;
#14567=EDGE_LOOP ( 'NONE', ( #17519, #15163, #8552, #40935 ) ) ;
#14568=PLANE ( 'NONE',  #23044 ) ;
#14569=EDGE_CURVE ( 'NONE', #15522, #4593, #25039, .T. ) ;
#14570=VERTEX_POINT ( 'NONE', #7408 ) ;
#14571=ADVANCED_FACE ( 'NONE', ( #54537 ), #46301, .F. ) ;
#14572=VECTOR ( 'NONE', #36978, 1000.000000000000000 ) ;
#14573=VERTEX_POINT ( 'NONE', #55132 ) ;
#14574=EDGE_LOOP ( 'NONE', ( #31349, #18424, #23126, #15081 ) ) ;
#14575=CARTESIAN_POINT ( 'NONE',  ( -13.79019121975177953, 5.143464774974014553, 1.874406862791435868 ) ) ;
#14576=ORIENTED_EDGE ( 'NONE', *, *, #41013, .F. ) ;
#14577=CARTESIAN_POINT ( 'NONE',  ( 2.072287782118878319, 0.000000000000000000, -2.950529333540147015 ) ) ;
#14578=ORIENTED_EDGE ( 'NONE', *, *, #31657, .T. ) ;
#14579=PLANE ( 'NONE',  #22204 ) ;
#14580=FACE_OUTER_BOUND ( 'NONE', #739, .T. ) ;
#14581=ADVANCED_FACE ( 'NONE', ( #7155 ), #15948, .F. ) ;
#14582=VERTEX_POINT ( 'NONE', #8549 ) ;
#14583=PLANE ( 'NONE',  #5920 ) ;
#14584=ORIENTED_EDGE ( 'NONE', *, *, #39050, .F. ) ;
#14585=ADVANCED_FACE ( 'NONE', ( #26155 ), #51440, .F. ) ;
#14586=FACE_OUTER_BOUND ( 'NONE', #45585, .T. ) ;
#14587=LINE ( 'NONE', #949, #21129 ) ;
#14588=DIRECTION ( 'NONE',  ( -0.9999697198139514409, -0.000000000000000000, -0.007781995580013368816 ) ) ;
#14589=CARTESIAN_POINT ( 'NONE',  ( -12.80458192191714595, 0.000000000000000000, 11.86454056839041726 ) ) ;
#14591=DIRECTION ( 'NONE',  ( 0.000000000000000000, -1.000000000000000000, 0.000000000000000000 ) ) ;
#14592=EDGE_LOOP ( 'NONE', ( #40508, #17564, #50492, #16722, #47042 ) ) ;
#14593=ORIENTED_EDGE ( 'NONE', *, *, #6603, .F. ) ;
#14594=VECTOR ( 'NONE', #8021, 1000.000000000000227 ) ;
#14595=LINE ( 'NONE', #10343, #35509 ) ;
#14596=PLANE ( 'NONE',  #23051 ) ;
#14597=CARTESIAN_POINT ( 'NONE',  ( -8.563136055001720592, -0.006715909454105468447, 4.948137389168624445 ) ) ;
#14598=FACE_OUTER_BOUND ( 'NONE', #3552, .T. ) ;
#14599=ORIENTED_EDGE ( 'NONE', *, *, #22202, .T. ) ;
#14600=LINE ( 'NONE', #6115, #34018 ) ;
#14601=CARTESIAN_POINT ( 'NONE',  ( -8.700467249853277352, 8.479997087537753941, 6.597930524618322856 ) ) ;
#14602=ORIENTED_EDGE ( 'NONE', *, *, #47322, .T. ) ;
#14603=DIRECTION ( 'NONE',  ( -0.5364919789714478471, 0.6444004775717705469, -0.5449076811759709926 ) ) ;
#14604=DIRECTION ( 'NONE',  ( 0.9999697198139515519, 0.000000000000000000, 0.007781995580013368816 ) ) ;
#14605=ORIENTED_EDGE ( 'NONE', *, *, #22656, .T. ) ;
#14606=CARTESIAN_POINT ( 'NONE',  ( -18.95295033115275984, 3.524445264749009876, 3.931453028570905062 ) ) ;
#14607=LINE ( 'NONE', #14894, #645 ) ;
#14608=AXIS2_PLACEMENT_3D ( 'NONE', #49445, #1986, #27290 ) ;
#14609=ADVANCED_FACE ( 'NONE', ( #47744 ), #25882, .F. ) ;
#14610=CARTESIAN_POINT ( 'NONE',  ( -20.72220850017212612, -3.594132820645660420, 10.62972551294390655 ) ) ;
#14611=DIRECTION ( 'NONE',  ( -0.5364919789714478471, 0.6444004775717705469, -0.5449076811759709926 ) ) ;
#14612=VECTOR ( 'NONE', #6194, 1000.000000000000227 ) ;
#14613=LINE ( 'NONE', #721, #10199 ) ;
#14614=ORIENTED_EDGE ( 'NONE', *, *, #10082, .F. ) ;
#14615=ORIENTED_EDGE ( 'NONE', *, *, #38186, .T. ) ;
#14616=DIRECTION ( 'NONE',  ( 0.007781995580012663651, 0.000000000000000000, -0.9999697198139515519 ) ) ;
#14617=CARTESIAN_POINT ( 'NONE',  ( -14.61903452936159553, 0.000000000000000000, 6.183966697747157681 ) ) ;
#14618=CARTESIAN_POINT ( 'NONE',  ( -16.93359685305117779, 0.000000000000000000, 5.057958029133816424 ) ) ;
#14619=ADVANCED_FACE ( 'NONE', ( #43210 ), #47152, .F. ) ;
#14620=DIRECTION ( 'NONE',  ( -0.5364919789714478471, 0.6444004775717705469, -0.5449076811759709926 ) ) ;
#14622=ORIENTED_EDGE ( 'NONE', *, *, #15972, .F. ) ;
#14623=ADVANCED_FACE ( 'NONE', ( #3707 ), #16787, .F. ) ;
#14625=CARTESIAN_POINT ( 'NONE',  ( -14.01701317841955508, 0.000000000000000000, 2.326005055450897085 ) ) ;
#14626=ADVANCED_FACE ( 'NONE', ( #21874 ), #9100, .F. ) ;
#14627=DIRECTION ( 'NONE',  ( -0.9999697198139514409, -0.000000000000000000, -0.007781995580013368816 ) ) ;
#14628=FACE_OUTER_BOUND ( 'NONE', #12299, .T. ) ;
#14629=ORIENTED_EDGE ( 'NONE', *, *, #5408, .T. ) ;
#14630=DIRECTION ( 'NONE',  ( -0.6427681459581293666, -0.7660444431189770143, -0.005002170337467561935 ) ) ;
#14631=EDGE_LOOP ( 'NONE', ( #22682, #30445, #37276, #54148 ) ) ;
#14632=PLANE ( 'NONE',  #38594 ) ;
#14633=DIRECTION ( 'NONE',  ( 0.005961354470445682716, -0.6427876096865404731, -0.7660212471507180654 ) ) ;
#14634=ORIENTED_EDGE ( 'NONE', *, *, #10222, .T. ) ;
#14636=VECTOR ( 'NONE', #37404, 999.9999999999998863 ) ;
#14637=DIRECTION ( 'NONE',  ( -0.5449076811759708816, 0.6444004775717707689, 0.5364919789714475140 ) ) ;
#14638=EDGE_CURVE ( 'NONE', #52700, #7363, #4004, .T. ) ;
#14639=ORIENTED_EDGE ( 'NONE', *, *, #4568, .F. ) ;
#14641=EDGE_LOOP ( 'NONE', ( #7295, #23252, #34923, #13459 ) ) ;
#14642=ORIENTED_EDGE ( 'NONE', *, *, #9911, .F. ) ;
#14643=CARTESIAN_POINT ( 'NONE',  ( -15.87975247367846166, 0.000000000000000000, 2.850166870931599927 ) ) ;
#14644=ORIENTED_EDGE ( 'NONE', *, *, #26199, .F. ) ;
#14645=ORIENTED_EDGE ( 'NONE', *, *, #45225, .F. ) ;
#14646=DIRECTION ( 'NONE',  ( 0.9999697198139515519, 0.000000000000000000, 0.007781995580013368816 ) ) ;
#14647=LINE ( 'NONE', #7176, #16776 ) ;
#14648=EDGE_LOOP ( 'NONE', ( #18775, #4101, #5259, #4853 ) ) ;
#14649=EDGE_CURVE ( 'NONE', #4593, #33120, #4842, .T. ) ;
#14650=ORIENTED_EDGE ( 'NONE', *, *, #25851, .F. ) ;
#14651=DIRECTION ( 'NONE',  ( 0.5364919789714477361, 0.6444004775717706579, 0.5449076811759711036 ) ) ;
#14652=VERTEX_POINT ( 'NONE', #17076 ) ;
#14653=ORIENTED_EDGE ( 'NONE', *, *, #51519, .T. ) ;
#14654=VECTOR ( 'NONE', #26118, 1000.000000000000000 ) ;
#14655=ADVANCED_FACE ( 'NONE', ( #30704 ), #30123, .F. ) ;
#14657=DIRECTION ( 'NONE',  ( -0.9999697198139514409, -0.000000000000000000, -0.007781995580013368816 ) ) ;
#14658=LINE ( 'NONE', #6421, #50464 ) ;
#14659=CARTESIAN_POINT ( 'NONE',  ( -15.50102849149811135, -0.1191753592594197858, 12.95155240711365430 ) ) ;
#14660=VERTEX_POINT ( 'NONE', #48001 ) ;
#14661=LINE ( 'NONE', #6424, #23790 ) ;
#14662=ORIENTED_EDGE ( 'NONE', *, *, #447, .F. ) ;
#14663=LINE ( 'NONE', #31452, #52913 ) ;
#14664=CARTESIAN_POINT ( 'NONE',  ( -14.17164195355221246, 0.000000000000000000, 8.403440829061754158 ) ) ;
#14665=LINE ( 'NONE', #33331, #24063 ) ;
#14666=CARTESIAN_POINT ( 'NONE',  ( -11.80247261326225505, 0.000000000000000000, 2.512565135777569569 ) ) ;
#14667=DIRECTION ( 'NONE',  ( 0.5364919789714477361, 0.6444004775717706579, 0.5449076811759711036 ) ) ;
#14668=LINE ( 'NONE', #5888, #16858 ) ;
#14669=ORIENTED_EDGE ( 'NONE', *, *, #8092, .F. ) ;
#14670=CARTESIAN_POINT ( 'NONE',  ( -17.74404816805336793, 0.000000000000000000, 3.574322630375089460 ) ) ;
#14671=ORIENTED_EDGE ( 'NONE', *, *, #12209, .F. ) ;
#14672=VECTOR ( 'NONE', #41635, 1000.000000000000114 ) ;
#14673=AXIS2_PLACEMENT_3D ( 'NONE', #7756, #24238, #37560 ) ;
#14674=DIRECTION ( 'NONE',  ( -0.6427681459581293666, -0.7660444431189770143, -0.005002170337467561935 ) ) ;
#14675=CARTESIAN_POINT ( 'NONE',  ( -11.52752152373586192, -2.137015261443160341, 1.290819977936035423 ) ) ;
#14676=CARTESIAN_POINT ( 'NONE',  ( -14.20280369269832832, 0.000000000000000000, 12.40765738797303719 ) ) ;
#14678=CARTESIAN_POINT ( 'NONE',  ( -22.40478740399063895, 0.000000000000000000, 5.384712028983816623 ) ) ;
#14679=CARTESIAN_POINT ( 'NONE',  ( -9.110551994824897193, 0.000000000000000000, 3.538847790438064411 ) ) ;
#14681=EDGE_CURVE ( 'NONE', #14310, #27973, #42896, .T. ) ;
#14682=AXIS2_PLACEMENT_3D ( 'NONE', #48389, #6362, #44153 ) ;
#14683=ORIENTED_EDGE ( 'NONE', *, *, #36430, .F. ) ;
#14684=ADVANCED_FACE ( 'NONE', ( #34653 ), #38657, .F. ) ;
#14685=CARTESIAN_POINT ( 'NONE',  ( -24.27063949748155380, 0.000000000000000000, 6.308861732390097288 ) ) ;
#14686=LINE ( 'NONE', #32008, #15896 ) ;
#14687=CARTESIAN_POINT ( 'NONE',  ( -10.42868029727597801, 0.000000000000000000, 5.108580793885948879 ) ) ;
#14688=EDGE_CURVE ( 'NONE', #41032, #7012, #8853, .T. ) ;
#14689=EDGE_CURVE ( 'NONE', #39029, #12809, #4563, .T. ) ;
#14690=EDGE_CURVE ( 'NONE', #15779, #31243, #30950, .T. ) ;
#14691=LINE ( 'NONE', #54162, #13771 ) ;
#14692=VECTOR ( 'NONE', #40585, 1000.000000000000227 ) ;
#14693=CARTESIAN_POINT ( 'NONE',  ( -24.26908309836554878, 0.000000000000000000, 6.108867788427308376 ) ) ;
#14694=CARTESIAN_POINT ( 'NONE',  ( -8.609916609573598834, 0.000000000000000000, 10.23519010964256637 ) ) ;
#14695=VECTOR ( 'NONE', #21066, 999.9999999999998863 ) ;
#14696=DIRECTION ( 'NONE',  ( -0.5364919789714478471, 0.6444004775717705469, -0.5449076811759709926 ) ) ;
#14697=DIRECTION ( 'NONE',  ( 0.007781995580012663651, 0.000000000000000000, -0.9999697198139515519 ) ) ;
#14698=ORIENTED_EDGE ( 'NONE', *, *, #2406, .F. ) ;
#14699=ORIENTED_EDGE ( 'NONE', *, *, #3711, .F. ) ;
#14700=EDGE_CURVE ( 'NONE', #24619, #24312, #53122, .T. ) ;
#14701=EDGE_CURVE ( 'NONE', #5503, #12315, #27543, .T. ) ;
#14702=ORIENTED_EDGE ( 'NONE', *, *, #51993, .T. ) ;
#14703=VERTEX_POINT ( 'NONE', #23303 ) ;
#14704=ORIENTED_EDGE ( 'NONE', *, *, #528, .T. ) ;
#14705=EDGE_CURVE ( 'NONE', #21025, #41679, #53940, .T. ) ;
#14706=ORIENTED_EDGE ( 'NONE', *, *, #12248, .T. ) ;
#14707=LINE ( 'NONE', #53348, #42323 ) ;
#14708=DIRECTION ( 'NONE',  ( 0.005002170337468016433, -0.7660444431189770143, -0.6427681459581293666 ) ) ;
#14709=VECTOR ( 'NONE', #3938, 999.9999999999998863 ) ;
#14710=EDGE_CURVE ( 'NONE', #11058, #47950, #18768, .T. ) ;
#14711=VECTOR ( 'NONE', #31782, 1000.000000000000227 ) ;
#14712=ORIENTED_EDGE ( 'NONE', *, *, #10020, .T. ) ;
#14713=ORIENTED_EDGE ( 'NONE', *, *, #39584, .T. ) ;
#14714=ORIENTED_EDGE ( 'NONE', *, *, #18085, .F. ) ;
#14715=VECTOR ( 'NONE', #43355, 999.9999999999998863 ) ;
#14716=AXIS2_PLACEMENT_3D ( 'NONE', #19001, #14468, #52783 ) ;
#14717=FACE_OUTER_BOUND ( 'NONE', #18628, .T. ) ;
#14718=PLANE ( 'NONE',  #112 ) ;
#14719=CARTESIAN_POINT ( 'NONE',  ( -9.442067484779661513, -0.1191753592594197858, 10.59804618892231254 ) ) ;
#14720=ORIENTED_EDGE ( 'NONE', *, *, #10895, .T. ) ;
#14721=DIRECTION ( 'NONE',  ( -0.005961354470445682716, -0.6427876096865404731, 0.7660212471507180654 ) ) ;
#14722=ORIENTED_EDGE ( 'NONE', *, *, #16608, .F. ) ;
#14723=DIRECTION ( 'NONE',  ( 0.9999697198139515519, 0.000000000000000000, 0.007781995580013368816 ) ) ;
#14724=AXIS2_PLACEMENT_3D ( 'NONE', #18020, #38775, #52930 ) ;
#14725=CARTESIAN_POINT ( 'NONE',  ( -13.53673582514181106, 0.000000000000000000, 12.22817484722816772 ) ) ;
#14726=LINE ( 'NONE', #32050, #23678 ) ;
#14727=LINE ( 'NONE', #49082, #43276 ) ;
#14728=FACE_OUTER_BOUND ( 'NONE', #8017, .T. ) ;
#14729=DIRECTION ( 'NONE',  ( -0.5364919789714478471, 0.6444004775717705469, -0.5449076811759709926 ) ) ;
#14730=FACE_OUTER_BOUND ( 'NONE', #23081, .T. ) ;
#14731=ORIENTED_EDGE ( 'NONE', *, *, #48013, .F. ) ;
#14732=PLANE ( 'NONE',  #41888 ) ;
#14733=ORIENTED_EDGE ( 'NONE', *, *, #26406, .T. ) ;
#14734=CARTESIAN_POINT ( 'NONE',  ( -16.21389796751076773, 3.038739411681508518, 2.883008631584717207 ) ) ;
#14735=DIRECTION ( 'NONE',  ( -0.5449076811759708816, 0.6444004775717707689, 0.5364919789714475140 ) ) ;
#14736=DIRECTION ( 'NONE',  ( 0.9999697198139515519, 0.000000000000000000, 0.007781995580013368816 ) ) ;
#14737=DIRECTION ( 'NONE',  ( -0.5364919789714478471, 0.6444004775717705469, -0.5449076811759709926 ) ) ;
#14738=EDGE_CURVE ( 'NONE', #3988, #46922, #1956, .T. ) ;
#14739=AXIS2_PLACEMENT_3D ( 'NONE', #10777, #49392, #10511 ) ;
#14740=LINE ( 'NONE', #32070, #42266 ) ;
#14741=PLANE ( 'NONE',  #40373 ) ;
#14742=CARTESIAN_POINT ( 'NONE',  ( -13.66964236114244891, 0.000000000000000000, 3.606030598478824789 ) ) ;
#14743=CARTESIAN_POINT ( 'NONE',  ( -10.47421230394850866, 0.000000000000000000, 10.95934586908605723 ) ) ;
#14744=LINE ( 'NONE', #54212, #39605 ) ;
#14745=ORIENTED_EDGE ( 'NONE', *, *, #26199, .T. ) ;
#14746=VECTOR ( 'NONE', #2938, 999.9999999999998863 ) ;
#14747=DIRECTION ( 'NONE',  ( 0.007781995580012663651, 0.000000000000000000, -0.9999697198139515519 ) ) ;
#14748=LINE ( 'NONE', #44853, #37630 ) ;
#14750=EDGE_CURVE ( 'NONE', #48012, #50620, #31547, .T. ) ;
#14751=DIRECTION ( 'NONE',  ( 0.000000000000000000, -1.000000000000000000, 0.000000000000000000 ) ) ;
#14753=ADVANCED_FACE ( 'NONE', ( #1698 ), #13915, .F. ) ;
#14754=VECTOR ( 'NONE', #44795, 1000.000000000000114 ) ;
#14756=LINE ( 'NONE', #1415, #28200 ) ;
#14757=EDGE_CURVE ( 'NONE', #7759, #3022, #44026, .T. ) ;
#14758=DIRECTION ( 'NONE',  ( -0.005961354470445682716, -0.6427876096865404731, 0.7660212471507180654 ) ) ;
#14759=LINE ( 'NONE', #19853, #5701 ) ;
#14760=ORIENTED_EDGE ( 'NONE', *, *, #13362, .F. ) ;
#14761=VECTOR ( 'NONE', #46977, 999.9999999999998863 ) ;
#14762=AXIS2_PLACEMENT_3D ( 'NONE', #41369, #6442, #32564 ) ;
#14763=ORIENTED_EDGE ( 'NONE', *, *, #7252, .T. ) ;
#14765=LINE ( 'NONE', #45160, #48498 ) ;
#14766=VERTEX_POINT ( 'NONE', #36092 ) ;
#14767=DIRECTION ( 'NONE',  ( 0.7660212471507180654, -0.6427876096865404731, 0.005961354470445141482 ) ) ;
#14768=VECTOR ( 'NONE', #3971, 1000.000000000000000 ) ;
#14769=EDGE_LOOP ( 'NONE', ( #32335, #32394, #39109, #29441 ) ) ;
#14770=CARTESIAN_POINT ( 'NONE',  ( -18.15140093078727901, -4.403642575758160760, 10.95967996775459952 ) ) ;
#14771=VECTOR ( 'NONE', #15147, 1000.000000000000227 ) ;
#14772=EDGE_CURVE ( 'NONE', #13654, #16888, #53395, .T. ) ;
#14773=ORIENTED_EDGE ( 'NONE', *, *, #11707, .T. ) ;
#14774=EDGE_LOOP ( 'NONE', ( #48799, #19345, #51333, #11459 ) ) ;
#14775=ORIENTED_EDGE ( 'NONE', *, *, #20794, .T. ) ;
#14777=EDGE_CURVE ( 'NONE', #42084, #20292, #48573, .T. ) ;
#14778=PLANE ( 'NONE',  #28404 ) ;
#14779=LINE ( 'NONE', #44880, #8743 ) ;
#14781=VECTOR ( 'NONE', #52761, 999.9999999999998863 ) ;
#14782=EDGE_CURVE ( 'NONE', #8988, #28441, #53649, .T. ) ;
#14783=VERTEX_POINT ( 'NONE', #9687 ) ;
#14784=ORIENTED_EDGE ( 'NONE', *, *, #45841, .F. ) ;
#14785=VECTOR ( 'NONE', #7703, 1000.000000000000227 ) ;
#14787=CARTESIAN_POINT ( 'NONE',  ( -19.60834386242827776, 0.000000000000000000, 4.298478389818581213 ) ) ;
#14788=ORIENTED_EDGE ( 'NONE', *, *, #20035, .T. ) ;
#14789=VECTOR ( 'NONE', #26293, 999.9999999999998863 ) ;
#14790=CARTESIAN_POINT ( 'NONE',  ( -13.07066190154808361, 0.000000000000000000, 12.04713590736729678 ) ) ;
#14792=DIRECTION ( 'NONE',  ( 0.005961354470445682716, -0.6427876096865404731, -0.7660212471507180654 ) ) ;
#14793=LINE ( 'NONE', #40647, #40311 ) ;
#14794=VECTOR ( 'NONE', #53905, 1000.000000000000227 ) ;
#14795=VECTOR ( 'NONE', #47273, 1000.000000000000114 ) ;
#14796=ORIENTED_EDGE ( 'NONE', *, *, #6740, .F. ) ;
#14797=DIRECTION ( 'NONE',  ( 0.000000000000000000, -1.000000000000000000, 0.000000000000000000 ) ) ;
#14798=VECTOR ( 'NONE', #39514, 1000.000000000000114 ) ;
#14799=LINE ( 'NONE', #18492, #25462 ) ;
#14800=VECTOR ( 'NONE', #9090, 999.9999999999998863 ) ;
#14801=ORIENTED_EDGE ( 'NONE', *, *, #30217, .T. ) ;
#14802=PLANE ( 'NONE',  #44097 ) ;
#14803=FACE_OUTER_BOUND ( 'NONE', #304, .T. ) ;
#14804=DIRECTION ( 'NONE',  ( -0.9999697198139514409, -0.000000000000000000, -0.007781995580013368816 ) ) ;
#14805=VERTEX_POINT ( 'NONE', #45159 ) ;
#14806=CARTESIAN_POINT ( 'NONE',  ( -9.075990533167328067, 0.000000000000000000, 10.41622904950343909 ) ) ;
#14807=LINE ( 'NONE', #20157, #11498 ) ;
#14808=DIRECTION ( 'NONE',  ( 0.005961354470445682716, -0.6427876096865404731, -0.7660212471507180654 ) ) ;
#14809=VECTOR ( 'NONE', #31199, 1000.000000000000114 ) ;
#14810=DIRECTION ( 'NONE',  ( 0.007781995580012663651, 0.000000000000000000, -0.9999697198139515519 ) ) ;
#14811=VECTOR ( 'NONE', #752, 1000.000000000000227 ) ;
#14812=CARTESIAN_POINT ( 'NONE',  ( -11.51026827947273112, 0.7721120973665037690, 1.128276403237633563 ) ) ;
#14813=DIRECTION ( 'NONE',  ( 0.2426528472758542054, 0.7422098413412800966, 0.6246952433987894571 ) ) ;
#14815=EDGE_LOOP ( 'NONE', ( #40149, #53222, #6120, #56061, #14122 ) ) ;
#14816=CARTESIAN_POINT ( 'NONE',  ( 2.072287782118878319, 0.000000000000000000, -2.950529333540147015 ) ) ;
#14817=CARTESIAN_POINT ( 'NONE',  ( -13.66257659974260186, 0.000000000000000000, 2.698095432668320637 ) ) ;
#14819=VERTEX_POINT ( 'NONE', #32093 ) ;
#14820=DIRECTION ( 'NONE',  ( -0.7660212471507179544, -0.6427876096865405842, -0.005961354470445141482 ) ) ;
#14821=CARTESIAN_POINT ( 'NONE',  ( -12.55055318312933643, 0.000000000000000000, 4.922741874866930267 ) ) ;
#14822=AXIS2_PLACEMENT_3D ( 'NONE', #23937, #37017, #32483 ) ;
#14823=EDGE_CURVE ( 'NONE', #21642, #13331, #49408, .T. ) ;
#14824=CARTESIAN_POINT ( 'NONE',  ( -14.62205743691809801, 3.362543313726510164, 2.254352670595775265 ) ) ;
#14825=VECTOR ( 'NONE', #24200, 999.9999999999998863 ) ;
#14826=EDGE_CURVE ( 'NONE', #15779, #30378, #22723, .T. ) ;
#14827=EDGE_CURVE ( 'NONE', #44163, #5769, #14234, .T. ) ;
#14828=DIRECTION ( 'NONE',  ( -0.6427681459581293666, -0.7660444431189770143, -0.005002170337467561935 ) ) ;
#14830=ORIENTED_EDGE ( 'NONE', *, *, #1072, .F. ) ;
#14831=EDGE_LOOP ( 'NONE', ( #35627, #4113, #47204, #18258 ) ) ;
#14833=AXIS2_PLACEMENT_3D ( 'NONE', #17488, #33753, #16169 ) ;
#14834=PLANE ( 'NONE',  #45913 ) ;
#14835=VECTOR ( 'NONE', #1164, 999.9999999999998863 ) ;
#14836=PLANE ( 'NONE',  #50154 ) ;
#14837=VECTOR ( 'NONE', #39706, 1000.000000000000227 ) ;
#14838=ORIENTED_EDGE ( 'NONE', *, *, #41988, .T. ) ;
#14839=DIRECTION ( 'NONE',  ( 0.5449076811759707706, 0.6444004775717708799, -0.5364919789714476250 ) ) ;
#14843=VECTOR ( 'NONE', #37672, 999.9999999999998863 ) ;
#14844=ORIENTED_EDGE ( 'NONE', *, *, #22781, .T. ) ;
#14845=PLANE ( 'NONE',  #2043 ) ;
#14846=PLANE ( 'NONE',  #45889 ) ;
#14847=FACE_OUTER_BOUND ( 'NONE', #43495, .T. ) ;
#14848=ORIENTED_EDGE ( 'NONE', *, *, #9650, .F. ) ;
#14849=DIRECTION ( 'NONE',  ( 0.005961354470445682716, -0.6427876096865404731, -0.7660212471507180654 ) ) ;
#14850=EDGE_LOOP ( 'NONE', ( #23495, #9926, #32115, #9968 ) ) ;
#14851=EDGE_CURVE ( 'NONE', #51400, #20591, #5682, .T. ) ;
#14852=ORIENTED_EDGE ( 'NONE', *, *, #544, .T. ) ;
#14853=ORIENTED_EDGE ( 'NONE', *, *, #6691, .F. ) ;
#14854=CARTESIAN_POINT ( 'NONE',  ( -25.20123094555300369, 0.000000000000000000, 6.470945668149052032 ) ) ;
#14855=VECTOR ( 'NONE', #22550, 1000.000000000000114 ) ;
#14856=ADVANCED_FACE ( 'NONE', ( #32388 ), #33975, .F. ) ;
#14857=ORIENTED_EDGE ( 'NONE', *, *, #52194, .F. ) ;
#14858=PLANE ( 'NONE',  #8492 ) ;
#14860=AXIS2_PLACEMENT_3D ( 'NONE', #49080, #18419, #54192 ) ;
#14861=CARTESIAN_POINT ( 'NONE',  ( -16.99924723426068951, 0.000000000000000000, 13.49389102713827171 ) ) ;
#14863=ORIENTED_EDGE ( 'NONE', *, *, #8349, .T. ) ;
#14864=ADVANCED_FACE ( 'NONE', ( #8137 ), #21183, .F. ) ;
#14865=DIRECTION ( 'NONE',  ( 0.6427681459581294776, -0.7660444431189769032, 0.005002170337467562802 ) ) ;
#14866=VECTOR ( 'NONE', #14956, 1000.000000000000227 ) ;
#14867=EDGE_LOOP ( 'NONE', ( #28677, #36190, #50935, #24287 ) ) ;
#14868=DIRECTION ( 'NONE',  ( 0.005961354470445682716, -0.6427876096865404731, -0.7660212471507180654 ) ) ;
#14869=LINE ( 'NONE', #36438, #40193 ) ;
#14870=DIRECTION ( 'NONE',  ( -0.7660212471507179544, -0.6427876096865405842, -0.005961354470445141482 ) ) ;
#14871=CARTESIAN_POINT ( 'NONE',  ( -10.74029228357944987, 0.000000000000000000, 11.14194120806293320 ) ) ;
#14872=CARTESIAN_POINT ( 'NONE',  ( -9.743931081935125249, 0.000000000000000000, 2.528585181965609774 ) ) ;
#14873=VECTOR ( 'NONE', #20506, 1000.000000000000114 ) ;
#14874=DIRECTION ( 'NONE',  ( 0.7660212471507180654, -0.6427876096865404731, 0.005961354470445141482 ) ) ;
#14876=ORIENTED_EDGE ( 'NONE', *, *, #40168, .T. ) ;
#14877=AXIS2_PLACEMENT_3D ( 'NONE', #17298, #16459, #56211 ) ;
#14878=ORIENTED_EDGE ( 'NONE', *, *, #49399, .T. ) ;
#14879=DIRECTION ( 'NONE',  ( -0.7660212471507179544, -0.6427876096865405842, -0.005961354470445141482 ) ) ;
#14880=FACE_OUTER_BOUND ( 'NONE', #7405, .T. ) ;
#14881=CARTESIAN_POINT ( 'NONE',  ( -14.40467031787239449, 0.000000000000000000, 4.338974580574337381 ) ) ;
#14882=VECTOR ( 'NONE', #38599, 999.9999999999998863 ) ;
#14883=AXIS2_PLACEMENT_3D ( 'NONE', #16344, #51825, #50980 ) ;
#14885=VERTEX_POINT ( 'NONE', #33680 ) ;
#14886=DIRECTION ( 'NONE',  ( -0.7660212471507179544, -0.6427876096865405842, -0.005961354470445141482 ) ) ;
#14887=DIRECTION ( 'NONE',  ( 0.000000000000000000, -1.000000000000000000, 0.000000000000000000 ) ) ;
#14888=EDGE_LOOP ( 'NONE', ( #22548, #37622, #16752, #48402 ) ) ;
#14889=LINE ( 'NONE', #6372, #2976 ) ;
#14890=EDGE_CURVE ( 'NONE', #17736, #6150, #42212, .T. ) ;
#14891=LINE ( 'NONE', #26838, #38525 ) ;
#14892=EDGE_LOOP ( 'NONE', ( #43845, #2482, #53668, #7960 ) ) ;
#14893=CARTESIAN_POINT ( 'NONE',  ( -14.71857576103236198, 2.876837460659007473, 7.319896171222362469 ) ) ;
#14894=CARTESIAN_POINT ( 'NONE',  ( -15.29900336458644894, -4.403642575758165201, 2.683474326561374745 ) ) ;
#14895=CARTESIAN_POINT ( 'NONE',  ( -33.59211796935609584, 0.000000000000000000, 9.929640529607549837 ) ) ;
#14896=ADVANCED_FACE ( 'NONE', ( #17207 ), #2252, .F. ) ;
#14897=PLANE ( 'NONE',  #21463 ) ;
#14898=LINE ( 'NONE', #45825, #45575 ) ;
#14899=AXIS2_PLACEMENT_3D ( 'NONE', #48759, #27738, #10703 ) ;
#14900=ORIENTED_EDGE ( 'NONE', *, *, #393, .T. ) ;
#14901=VECTOR ( 'NONE', #6001, 999.9999999999998863 ) ;
#14902=ORIENTED_EDGE ( 'NONE', *, *, #41119, .F. ) ;
#14903=DIRECTION ( 'NONE',  ( -0.7660212471507179544, -0.6427876096865405842, -0.005961354470445141482 ) ) ;
#14904=CARTESIAN_POINT ( 'NONE',  ( -26.13493519185646008, 0.000000000000000000, 7.033017491833586377 ) ) ;
#14905=DIRECTION ( 'NONE',  ( 0.007781995580012663651, -3.146120232559066537E-19, -0.9999697198139514409 ) ) ;
#14906=AXIS2_PLACEMENT_3D ( 'NONE', #24561, #2979, #2445 ) ;
#14907=LINE ( 'NONE', #53273, #17371 ) ;
#14908=CARTESIAN_POINT ( 'NONE',  ( -18.67697421479882181, -0.1191753592594197858, 4.036397482078229793 ) ) ;
#14909=VECTOR ( 'NONE', #11778, 999.9999999999998863 ) ;
#14910=VERTEX_POINT ( 'NONE', #36926 ) ;
#14911=PLANE ( 'NONE',  #21999 ) ;
#14912=EDGE_CURVE ( 'NONE', #34828, #35980, #50988, .T. ) ;
#14913=FACE_OUTER_BOUND ( 'NONE', #46185, .T. ) ;
#14914=CARTESIAN_POINT ( 'NONE',  ( -25.20200914511100265, -0.1191753592594197858, 6.570942640130446932 ) ) ;
#14915=ORIENTED_EDGE ( 'NONE', *, *, #51726, .F. ) ;
#14916=VECTOR ( 'NONE', #3101, 999.9999999999998863 ) ;
#14917=DIRECTION ( 'NONE',  ( 0.000000000000000000, -0.000000000000000000, -1.000000000000000000 ) ) ;
#14918=ORIENTED_EDGE ( 'NONE', *, *, #43946, .F. ) ;
#14919=LINE ( 'NONE', #41845, #50388 ) ;
#14920=DIRECTION ( 'NONE',  ( 0.5449076811759707706, 0.6444004775717708799, -0.5364919789714476250 ) ) ;
#14922=ORIENTED_EDGE ( 'NONE', *, *, #2260, .F. ) ;
#14923=DIRECTION ( 'NONE',  ( 0.7660212471507180654, -0.6427876096865404731, 0.005961354470445141482 ) ) ;
#14924=VERTEX_POINT ( 'NONE', #49942 ) ;
#14926=ORIENTED_EDGE ( 'NONE', *, *, #39444, .F. ) ;
#14927=ORIENTED_EDGE ( 'NONE', *, *, #10751, .F. ) ;
#14928=DIRECTION ( 'NONE',  ( 0.005961354470445682716, -0.6427876096865404731, -0.7660212471507180654 ) ) ;
#14929=VECTOR ( 'NONE', #56048, 1000.000000000000227 ) ;
#14930=VERTEX_POINT ( 'NONE', #12414 ) ;
#14931=ORIENTED_EDGE ( 'NONE', *, *, #50994, .T. ) ;
#14932=CARTESIAN_POINT ( 'NONE',  ( -26.13337879274045505, 0.000000000000000000, 6.833023547870798353 ) ) ;
#14933=ORIENTED_EDGE ( 'NONE', *, *, #27520, .T. ) ;
#14934=ORIENTED_EDGE ( 'NONE', *, *, #18167, .T. ) ;
#14935=CARTESIAN_POINT ( 'NONE',  ( -15.09844010454417429, -0.8417996532631562001, 2.719210182726563119 ) ) ;
#14936=EDGE_CURVE ( 'NONE', #1131, #33580, #25733, .T. ) ;
#14937=EDGE_LOOP ( 'NONE', ( #27847, #2891, #9570, #15299 ) ) ;
#14938=ORIENTED_EDGE ( 'NONE', *, *, #7360, .F. ) ;
#14939=AXIS2_PLACEMENT_3D ( 'NONE', #26932, #5346, #22653 ) ;
#14940=LINE ( 'NONE', #36250, #36545 ) ;
#14941=VECTOR ( 'NONE', #2282, 1000.000000000000227 ) ;
#14942=DIRECTION ( 'NONE',  ( 0.000000000000000000, -1.000000000000000000, 0.000000000000000000 ) ) ;
#14943=CARTESIAN_POINT ( 'NONE',  ( -20.54204810873173415, 0.000000000000000000, 4.860550213503115558 ) ) ;
#14944=DIRECTION ( 'NONE',  ( 0.007781995580012663651, -3.146120232559066537E-19, -0.9999697198139514409 ) ) ;
#14945=ORIENTED_EDGE ( 'NONE', *, *, #23281, .F. ) ;
#14946=FACE_OUTER_BOUND ( 'NONE', #41411, .T. ) ;
#14947=VECTOR ( 'NONE', #15925, 999.9999999999998863 ) ;
#14948=ORIENTED_EDGE ( 'NONE', *, *, #42402, .T. ) ;
#14949=EDGE_CURVE ( 'NONE', #52494, #33064, #42495, .T. ) ;
#14950=CARTESIAN_POINT ( 'NONE',  ( -13.36712169493445579, -2.622721114510659035, 6.178507914287525438 ) ) ;
#14951=AXIS2_PLACEMENT_3D ( 'NONE', #6848, #27883, #36374 ) ;
#14952=EDGE_CURVE ( 'NONE', #8247, #18922, #55838, .T. ) ;
#14953=EDGE_CURVE ( 'NONE', #40596, #6333, #20644, .T. ) ;
#14954=DIRECTION ( 'NONE',  ( -0.005002170337468016433, -0.7660444431189770143, 0.6427681459581293666 ) ) ;
#14955=CARTESIAN_POINT ( 'NONE',  ( 3.004435629306332345, 0.000000000000000000, -3.312607213261892003 ) ) ;
#14956=DIRECTION ( 'NONE',  ( -0.9999697198139514409, -0.000000000000000000, -0.007781995580013368816 ) ) ;
#14957=VECTOR ( 'NONE', #21357, 1000.000000000000000 ) ;
#14958=CARTESIAN_POINT ( 'NONE',  ( -18.82594708035263764, 2.229229656569007290, 7.852503942761646982 ) ) ;
#14959=ORIENTED_EDGE ( 'NONE', *, *, #8881, .F. ) ;
#14960=CARTESIAN_POINT ( 'NONE',  ( -19.71200609458190911, -1.984075165378300865, 6.895443337863062183 ) ) ;
#14961=ADVANCED_FACE ( 'NONE', ( #28101 ), #6519, .F. ) ;
#14962=ORIENTED_EDGE ( 'NONE', *, *, #35003, .F. ) ;
#14963=VECTOR ( 'NONE', #25555, 1000.000000000000114 ) ;
#14964=CARTESIAN_POINT ( 'NONE',  ( -27.06708303904391144, 0.000000000000000000, 7.395095371555332697 ) ) ;
#14965=DIRECTION ( 'NONE',  ( -0.9999697198139514409, -0.000000000000000000, -0.007781995580013368816 ) ) ;
#14966=EDGE_CURVE ( 'NONE', #52332, #45792, #21490, .T. ) ;
#14967=CARTESIAN_POINT ( 'NONE',  ( -25.20200914511100265, -0.1191753592594197858, 6.570942640130446932 ) ) ;
#14968=FACE_OUTER_BOUND ( 'NONE', #27788, .T. ) ;
#14969=ADVANCED_FACE ( 'NONE', ( #12678 ), #15324, .F. ) ;
#14970=CARTESIAN_POINT ( 'NONE',  ( -9.542064456761055524, 0.000000000000000000, 10.59726798936431180 ) ) ;
#14971=AXIS2_PLACEMENT_3D ( 'NONE', #12024, #51219, #3521 ) ;
#14972=VECTOR ( 'NONE', #8377, 1000.000000000000227 ) ;
#14973=ORIENTED_EDGE ( 'NONE', *, *, #26735, .F. ) ;
#14974=LINE ( 'NONE', #19787, #7619 ) ;
#14975=PLANE ( 'NONE',  #46663 ) ;
#14976=DIRECTION ( 'NONE',  ( -0.005961354470445682716, -0.6427876096865404731, 0.7660212471507180654 ) ) ;
#14977=EDGE_CURVE ( 'NONE', #24834, #25732, #29989, .T. ) ;
#14978=LINE ( 'NONE', #33137, #24621 ) ;
#14979=FACE_OUTER_BOUND ( 'NONE', #14831, .T. ) ;
#14980=CARTESIAN_POINT ( 'NONE',  ( -13.66545065324788411, 0.000000000000000000, 3.067405135926084103 ) ) ;
#14981=CARTESIAN_POINT ( 'NONE',  ( -18.92804305261459774, 1.257817950434005461, 6.297909381879228441 ) ) ;
#14982=VECTOR ( 'NONE', #54921, 999.9999999999998863 ) ;
#14983=EDGE_CURVE ( 'NONE', #10480, #18734, #32637, .T. ) ;
#14985=AXIS2_PLACEMENT_3D ( 'NONE', #50741, #15280, #24078 ) ;
#14986=LINE ( 'NONE', #5911, #27442 ) ;
#14987=VECTOR ( 'NONE', #14210, 1000.000000000000227 ) ;
#14988=VERTEX_POINT ( 'NONE', #3321 ) ;
#14989=VECTOR ( 'NONE', #50195, 999.9999999999998863 ) ;
#14990=ORIENTED_EDGE ( 'NONE', *, *, #17536, .T. ) ;
#14991=ORIENTED_EDGE ( 'NONE', *, *, #20753, .F. ) ;
#14992=AXIS2_PLACEMENT_3D ( 'NONE', #48784, #34872, #26333 ) ;
#14994=ORIENTED_EDGE ( 'NONE', *, *, #1927, .T. ) ;
#14995=VECTOR ( 'NONE', #50841, 999.9999999999998863 ) ;
#14996=ORIENTED_EDGE ( 'NONE', *, *, #35473, .F. ) ;
#14997=DIRECTION ( 'NONE',  ( -0.005961354470445682716, -0.6427876096865404731, 0.7660212471507180654 ) ) ;
#14998=CARTESIAN_POINT ( 'NONE',  ( -27.06708303904391144, 0.000000000000000000, 7.395095371555332697 ) ) ;
#14999=AXIS2_PLACEMENT_3D ( 'NONE', #49036, #47933, #5059 ) ;
#15000=VECTOR ( 'NONE', #24219, 999.9999999999998863 ) ;
#15001=ORIENTED_EDGE ( 'NONE', *, *, #48184, .T. ) ;
#15002=CARTESIAN_POINT ( 'NONE',  ( -10.79984652870423822, -0.1191753592594181482, 5.944359460172861098 ) ) ;
#15003=EDGE_CURVE ( 'NONE', #32474, #29764, #55263, .T. ) ;
#15004=ORIENTED_EDGE ( 'NONE', *, *, #12364, .F. ) ;
#15005=VECTOR ( 'NONE', #38084, 1000.000000000000227 ) ;
#15006=VECTOR ( 'NONE', #48902, 1000.000000000000227 ) ;
#15007=CARTESIAN_POINT ( 'NONE',  ( -20.59866850025657925, -1.813211359398156919, 7.658942858085559635 ) ) ;
#15008=DIRECTION ( 'NONE',  ( 0.5364919789714477361, 0.6444004775717706579, 0.5449076811759711036 ) ) ;
#15009=DIRECTION ( 'NONE',  ( 0.007781995580012663651, -3.146120232559066537E-19, -0.9999697198139514409 ) ) ;
#15010=ORIENTED_EDGE ( 'NONE', *, *, #4512, .F. ) ;
#15011=DIRECTION ( 'NONE',  ( -0.005961354470445682716, -0.6427876096865404731, 0.7660212471507180654 ) ) ;
#15012=EDGE_CURVE ( 'NONE', #54304, #9862, #20894, .T. ) ;
#15014=PLANE ( 'NONE',  #51790 ) ;
#15015=CARTESIAN_POINT ( 'NONE',  ( -14.98445265377928770, -0.1191753592594174960, 6.281125957518538527 ) ) ;
#15016=ADVANCED_FACE ( 'NONE', ( #48426 ), #5290, .F. ) ;
#15018=DIRECTION ( 'NONE',  ( -0.005961354470445682716, -0.6427876096865404731, 0.7660212471507180654 ) ) ;
#15019=FACE_OUTER_BOUND ( 'NONE', #15323, .T. ) ;
#15021=DIRECTION ( 'NONE',  ( 0.6427681459581294776, -0.7660444431189769032, 0.005002170337467562802 ) ) ;
#15022=CARTESIAN_POINT ( 'NONE',  ( -11.87243407472968926, 0.000000000000000000, 11.50246268866867361 ) ) ;
#15023=VECTOR ( 'NONE', #11774, 999.9999999999998863 ) ;
#15024=DIRECTION ( 'NONE',  ( -0.005961354470445682716, -0.6427876096865404731, 0.7660212471507180654 ) ) ;
#15025=ORIENTED_EDGE ( 'NONE', *, *, #3679, .T. ) ;
#15026=DIRECTION ( 'NONE',  ( 0.000000000000000000, -0.000000000000000000, -1.000000000000000000 ) ) ;
#15027=ORIENTED_EDGE ( 'NONE', *, *, #29720, .T. ) ;
#15028=VECTOR ( 'NONE', #16857, 999.9999999999998863 ) ;
#15029=PLANE ( 'NONE',  #49204 ) ;
#15030=CARTESIAN_POINT ( 'NONE',  ( -13.20368780991208268, 0.000000000000000000, 3.440330750951857031 ) ) ;
#15031=CARTESIAN_POINT ( 'NONE',  ( -11.30636317915456779, -0.1191753592594197858, 11.32220194836580340 ) ) ;
#15032=EDGE_CURVE ( 'NONE', #42375, #39726, #17788, .T. ) ;
#15034=VECTOR ( 'NONE', #42873, 1000.000000000000114 ) ;
#15035=DIRECTION ( 'NONE',  ( 0.005961354470445682716, -0.6427876096865404731, -0.7660212471507180654 ) ) ;
#15036=PLANE ( 'NONE',  #40420 ) ;
#15037=DIRECTION ( 'NONE',  ( 0.000000000000000000, -1.000000000000000000, 0.000000000000000000 ) ) ;
#15038=ADVANCED_FACE ( 'NONE', ( #443 ), #5546, .F. ) ;
#15039=DIRECTION ( 'NONE',  ( 0.007781995580012662783, 0.000000000000000000, -0.9999697198139514409 ) ) ;
#15040=AXIS2_PLACEMENT_3D ( 'NONE', #15676, #3191, #15987 ) ;
#15041=VECTOR ( 'NONE', #24535, 1000.000000000000227 ) ;
#15042=DIRECTION ( 'NONE',  ( 0.005002170337468016433, -0.7660444431189770143, -0.6427681459581293666 ) ) ;
#15043=PLANE ( 'NONE',  #12112 ) ;
#15044=DIRECTION ( 'NONE',  ( 0.9999697198139515519, 0.000000000000000000, 0.007781995580013368816 ) ) ;
#15045=CARTESIAN_POINT ( 'NONE',  ( -14.46333583037745107, 5.305366725996512045, 11.20638257342840660 ) ) ;
#15046=PLANE ( 'NONE',  #5119 ) ;
#15047=VECTOR ( 'NONE', #11743, 999.9999999999998863 ) ;
#15048=EDGE_CURVE ( 'NONE', #10989, #6706, #735, .T. ) ;
#15049=VECTOR ( 'NONE', #37084, 1000.000000000000227 ) ;
#15050=DIRECTION ( 'NONE',  ( 0.007781995580012663651, 0.000000000000000000, -0.9999697198139515519 ) ) ;
#15051=VECTOR ( 'NONE', #17556, 1000.000000000000227 ) ;
#15052=DIRECTION ( 'NONE',  ( -0.6246952433987894571, 0.7422098413412802076, 0.2426528472758539834 ) ) ;
#15053=FACE_OUTER_BOUND ( 'NONE', #2536, .T. ) ;
#15054=LINE ( 'NONE', #19585, #40120 ) ;
#15055=ORIENTED_EDGE ( 'NONE', *, *, #12412, .T. ) ;
#15056=VECTOR ( 'NONE', #13784, 1000.000000000000227 ) ;
#15057=VECTOR ( 'NONE', #1881, 999.9999999999998863 ) ;
#15058=VERTEX_POINT ( 'NONE', #9543 ) ;
#15059=DIRECTION ( 'NONE',  ( 0.9999697198139515519, 0.000000000000000000, 0.007781995580013368816 ) ) ;
#15060=DIRECTION ( 'NONE',  ( 0.5449076811759707706, 0.6444004775717708799, -0.5364919789714476250 ) ) ;
#15061=ORIENTED_EDGE ( 'NONE', *, *, #42046, .T. ) ;
#15062=PLANE ( 'NONE',  #13185 ) ;
#15063=ORIENTED_EDGE ( 'NONE', *, *, #9170, .T. ) ;
#15064=CARTESIAN_POINT ( 'NONE',  ( -18.68645613183151610, -0.07073876987044309950, 9.535660383697532438 ) ) ;
#15065=VECTOR ( 'NONE', #25194, 1000.000000000000227 ) ;
#15066=ORIENTED_EDGE ( 'NONE', *, *, #29239, .T. ) ;
#15067=VERTEX_POINT ( 'NONE', #22864 ) ;
#15068=ORIENTED_EDGE ( 'NONE', *, *, #47064, .T. ) ;
#15069=LINE ( 'NONE', #15891, #22990 ) ;
#15070=DIRECTION ( 'NONE',  ( -0.7660212471507179544, -0.6427876096865405842, -0.005961354470445141482 ) ) ;
#15071=VECTOR ( 'NONE', #14348, 1000.000000000000227 ) ;
#15073=EDGE_CURVE ( 'NONE', #30649, #12259, #39070, .T. ) ;
#15074=ORIENTED_EDGE ( 'NONE', *, *, #44815, .F. ) ;
#15075=VECTOR ( 'NONE', #41684, 999.9999999999998863 ) ;
#15076=EDGE_CURVE ( 'NONE', #7467, #24071, #35374, .T. ) ;
#15077=ORIENTED_EDGE ( 'NONE', *, *, #54244, .T. ) ;
#15078=VECTOR ( 'NONE', #14737, 1000.000000000000000 ) ;
#15080=CARTESIAN_POINT ( 'NONE',  ( -18.66354898467281132, 0.000000000000000000, 14.21960318569776582 ) ) ;
#15081=ORIENTED_EDGE ( 'NONE', *, *, #5466, .T. ) ;
#15083=CARTESIAN_POINT ( 'NONE',  ( -11.87243407472968926, 0.000000000000000000, 11.50246268866867361 ) ) ;
#15084=EDGE_LOOP ( 'NONE', ( #21560, #39163, #22190, #26461 ) ) ;
#15085=CARTESIAN_POINT ( 'NONE',  ( -9.042720045137619067, -2.794052915596232367, 3.713477088201619924 ) ) ;
#15086=LINE ( 'NONE', #28700, #27630 ) ;
#15087=EDGE_CURVE ( 'NONE', #6080, #15150, #30833, .T. ) ;
#15088=AXIS2_PLACEMENT_3D ( 'NONE', #10516, #14751, #40616 ) ;
#15089=EDGE_CURVE ( 'NONE', #32268, #54774, #26862, .T. ) ;
#15090=ADVANCED_FACE ( 'NONE', ( #26036 ), #8716, .F. ) ;
#15091=ORIENTED_EDGE ( 'NONE', *, *, #7464, .F. ) ;
#15092=VECTOR ( 'NONE', #31906, 1000.000000000000000 ) ;
#15093=LINE ( 'NONE', #49721, #6844 ) ;
#15094=AXIS2_PLACEMENT_3D ( 'NONE', #52822, #4577, #8566 ) ;
#15095=PLANE ( 'NONE',  #16369 ) ;
#15096=AXIS2_PLACEMENT_3D ( 'NONE', #39641, #30263, #52113 ) ;
#15097=EDGE_LOOP ( 'NONE', ( #27404, #11061, #14857, #34718 ) ) ;
#15098=PLANE ( 'NONE',  #55762 ) ;
#15100=CARTESIAN_POINT ( 'NONE',  ( -21.47341775636118655, -0.1191753592594197858, 5.122631121243466090 ) ) ;
#15101=EDGE_LOOP ( 'NONE', ( #43830, #33587, #29277, #16895 ) ) ;
#15102=CARTESIAN_POINT ( 'NONE',  ( 2.072287782118878319, 0.000000000000000000, -2.950529333540147015 ) ) ;
#15103=DIRECTION ( 'NONE',  ( 0.005961354470445682716, -0.6427876096865404731, -0.7660212471507180654 ) ) ;
#15104=CARTESIAN_POINT ( 'NONE',  ( -17.73140113748535285, 0.000000000000000000, 13.85752530597602039 ) ) ;
#15105=EDGE_CURVE ( 'NONE', #15287, #10033, #34526, .T. ) ;
#15106=CARTESIAN_POINT ( 'NONE',  ( -13.23305999722791171, 2.229229656569007290, 5.680036664431174387 ) ) ;
#15107=CARTESIAN_POINT ( 'NONE',  ( -22.40478740399063895, 0.000000000000000000, 5.384712028983816623 ) ) ;
#15108=PLANE ( 'NONE',  #39733 ) ;
#15109=AXIS2_PLACEMENT_3D ( 'NONE', #7805, #11759, #33905 ) ;
#15110=ADVANCED_FACE ( 'NONE', ( #44185 ), #9242, .F. ) ;
#15112=EDGE_LOOP ( 'NONE', ( #38817, #22425, #46980, #53512 ) ) ;
#15113=FACE_OUTER_BOUND ( 'NONE', #55845, .T. ) ;
#15114=FACE_OUTER_BOUND ( 'NONE', #39213, .T. ) ;
#15115=ADVANCED_FACE ( 'NONE', ( #39353 ), #26563, .F. ) ;
#15117=EDGE_LOOP ( 'NONE', ( #22273, #42675, #43370, #31762 ) ) ;
#15119=CARTESIAN_POINT ( 'NONE',  ( -25.20200914511100265, -0.1191753592594197858, 6.570942640130446932 ) ) ;
#15120=VECTOR ( 'NONE', #9941, 1000.000000000000227 ) ;
#15121=EDGE_CURVE ( 'NONE', #29959, #41646, #39655, .T. ) ;
#15122=VECTOR ( 'NONE', #23622, 1000.000000000000227 ) ;
#15123=LINE ( 'NONE', #42043, #19525 ) ;
#15124=FACE_OUTER_BOUND ( 'NONE', #20907, .T. ) ;
#15125=EDGE_CURVE ( 'NONE', #47950, #41108, #52130, .T. ) ;
#15126=DIRECTION ( 'NONE',  ( -0.5449076811759708816, 0.6444004775717707689, 0.5364919789714475140 ) ) ;
#15127=ORIENTED_EDGE ( 'NONE', *, *, #32947, .T. ) ;
#15128=VECTOR ( 'NONE', #5894, 1000.000000000000114 ) ;
#15129=ORIENTED_EDGE ( 'NONE', *, *, #23717, .T. ) ;
#15131=CARTESIAN_POINT ( 'NONE',  ( -17.93139508144814442, 0.000000000000000000, 13.85596890686001537 ) ) ;
#15133=CARTESIAN_POINT ( 'NONE',  ( -13.53673582514181106, 0.000000000000000000, 12.22817484722816772 ) ) ;
#15134=VECTOR ( 'NONE', #8756, 1000.000000000000000 ) ;
#15135=EDGE_LOOP ( 'NONE', ( #10463, #1704, #1310, #16242 ) ) ;
#15136=FACE_OUTER_BOUND ( 'NONE', #24912, .T. ) ;
#15137=ORIENTED_EDGE ( 'NONE', *, *, #24928, .T. ) ;
#15138=LINE ( 'NONE', #50010, #39218 ) ;
#15139=VECTOR ( 'NONE', #37695, 999.9999999999998863 ) ;
#15140=AXIS2_PLACEMENT_3D ( 'NONE', #28361, #15573, #20108 ) ;
#15142=EDGE_LOOP ( 'NONE', ( #20855, #38822, #24971, #23511 ) ) ;
#15143=CARTESIAN_POINT ( 'NONE',  ( -16.45614608779968080, 0.000000000000000000, 3.415019368575790804 ) ) ;
#15144=DIRECTION ( 'NONE',  ( 0.005002170337468016433, -0.7660444431189770143, -0.6427681459581293666 ) ) ;
#15145=DIRECTION ( 'NONE',  ( -0.9999697198139514409, -0.000000000000000000, -0.007781995580013368816 ) ) ;
#15146=ORIENTED_EDGE ( 'NONE', *, *, #52752, .F. ) ;
#15147=DIRECTION ( 'NONE',  ( -0.9999697198139514409, -0.000000000000000000, -0.007781995580013368816 ) ) ;
#15148=ORIENTED_EDGE ( 'NONE', *, *, #53108, .T. ) ;
#15149=VECTOR ( 'NONE', #39801, 999.9999999999998863 ) ;
#15150=VERTEX_POINT ( 'NONE', #44443 ) ;
#15151=ORIENTED_EDGE ( 'NONE', *, *, #27912, .T. ) ;
#15152=CARTESIAN_POINT ( 'NONE',  ( -19.43036298310061483, 2.391131607591507446, 8.352988289389880805 ) ) ;
#15153=ORIENTED_EDGE ( 'NONE', *, *, #13229, .F. ) ;
#15154=DIRECTION ( 'NONE',  ( -0.5449076811759708816, 0.6444004775717707689, 0.5364919789714475140 ) ) ;
#15155=ORIENTED_EDGE ( 'NONE', *, *, #7068, .F. ) ;
#15156=LINE ( 'NONE', #23929, #28563 ) ;
#15157=DIRECTION ( 'NONE',  ( 0.005002170337468016433, -0.7660444431189770143, -0.6427681459581293666 ) ) ;
#15158=EDGE_CURVE ( 'NONE', #1353, #40267, #40187, .T. ) ;
#15159=EDGE_CURVE ( 'NONE', #50596, #33190, #8986, .T. ) ;
#15160=VERTEX_POINT ( 'NONE', #45029 ) ;
#15161=VECTOR ( 'NONE', #29990, 1000.000000000000227 ) ;
#15162=CARTESIAN_POINT ( 'NONE',  ( -10.94028622754223967, 0.000000000000000000, 11.14038480894692995 ) ) ;
#15163=ORIENTED_EDGE ( 'NONE', *, *, #38819, .F. ) ;
#15164=ADVANCED_FACE ( 'NONE', ( #32521 ), #45547, .F. ) ;
#15165=AXIS2_PLACEMENT_3D ( 'NONE', #28217, #49546, #49808 ) ;
#15166=DIRECTION ( 'NONE',  ( 0.005961354470445682716, -0.6427876096865404731, -0.7660212471507180654 ) ) ;
#15167=DIRECTION ( 'NONE',  ( 0.007781995580012663651, 0.000000000000000000, -0.9999697198139515519 ) ) ;
#15168=CARTESIAN_POINT ( 'NONE',  ( -12.70113610826450845, 4.333955019861509328, 8.927632253102496307 ) ) ;
#15169=CARTESIAN_POINT ( 'NONE',  ( -18.67775241435682432, 0.000000000000000000, 4.136394454059623804 ) ) ;
#15170=CARTESIAN_POINT ( 'NONE',  ( -12.30028049777745558, 0.000000000000000000, 6.771349903807757364 ) ) ;
#15171=LINE ( 'NONE', #22063, #24622 ) ;
#15172=CARTESIAN_POINT ( 'NONE',  ( -21.47263955680318404, 0.000000000000000000, 5.022634149262071190 ) ) ;
#15173=ORIENTED_EDGE ( 'NONE', *, *, #48624, .F. ) ;
#15175=VECTOR ( 'NONE', #28276, 1000.000000000000114 ) ;
#15176=CARTESIAN_POINT ( 'NONE',  ( -11.67244013076689946, 0.000000000000000000, 11.50401908778467863 ) ) ;
#15177=FACE_OUTER_BOUND ( 'NONE', #14631, .T. ) ;
#15178=CARTESIAN_POINT ( 'NONE',  ( -10.70637586329141122, 0.000000000000000000, 6.783754038227788108 ) ) ;
#15179=DIRECTION ( 'NONE',  ( -0.5364919789714478471, 0.6444004775717705469, -0.5449076811759709926 ) ) ;
#15180=LINE ( 'NONE', #53499, #19484 ) ;
#15181=VERTEX_POINT ( 'NONE', #28237 ) ;
#15182=FACE_OUTER_BOUND ( 'NONE', #32262, .T. ) ;
#15183=DIRECTION ( 'NONE',  ( 0.007781995580012662783, 0.000000000000000000, -0.9999697198139514409 ) ) ;
#15184=ORIENTED_EDGE ( 'NONE', *, *, #24070, .F. ) ;
#15185=CARTESIAN_POINT ( 'NONE',  ( -15.13495153988577968, 0.000000000000000000, 12.76973526769478084 ) ) ;
#15187=VERTEX_POINT ( 'NONE', #1826 ) ;
#15188=CARTESIAN_POINT ( 'NONE',  ( -18.61801697800028066, 0.000000000000000000, 8.368838110497661020 ) ) ;
#15189=CARTESIAN_POINT ( 'NONE',  ( -15.60102546347950536, 0.000000000000000000, 12.95077420755565356 ) ) ;
#15190=DIRECTION ( 'NONE',  ( 0.6427681459581294776, -0.7660444431189769032, 0.005002170337467562802 ) ) ;
#15191=EDGE_CURVE ( 'NONE', #37975, #2305, #19439, .T. ) ;
#15192=PLANE ( 'NONE',  #54086 ) ;
#15193=DIRECTION ( 'NONE',  ( -0.5449076811759708816, 0.6444004775717707689, 0.5364919789714475140 ) ) ;
#15194=ORIENTED_EDGE ( 'NONE', *, *, #30670, .F. ) ;
#15195=ADVANCED_FACE ( 'NONE', ( #19151 ), #54097, .F. ) ;
#15196=VERTEX_POINT ( 'NONE', #53524 ) ;
#15197=LINE ( 'NONE', #49557, #51147 ) ;
#15199=CARTESIAN_POINT ( 'NONE',  ( -15.85841441797052731, -2.298917212465658721, 2.967920335911165886 ) ) ;
#15200=EDGE_CURVE ( 'NONE', #51439, #12052, #18618, .T. ) ;
#15201=DIRECTION ( 'NONE',  ( 0.5449076811759707706, 0.6444004775717708799, -0.5364919789714476250 ) ) ;
#15202=EDGE_CURVE ( 'NONE', #6270, #12635, #15206, .T. ) ;
#15203=LINE ( 'NONE', #37055, #15836 ) ;
#15204=VERTEX_POINT ( 'NONE', #53799 ) ;
#15205=CARTESIAN_POINT ( 'NONE',  ( -14.41904058539880751, 0.000000000000000000, 6.185523096863160042 ) ) ;
#15206=LINE ( 'NONE', #6969, #48626 ) ;
#15207=VECTOR ( 'NONE', #33136, 999.9999999999998863 ) ;
#15208=FACE_OUTER_BOUND ( 'NONE', #9470, .T. ) ;
#15209=VERTEX_POINT ( 'NONE', #53279 ) ;
#15210=DIRECTION ( 'NONE',  ( -0.5364919789714478471, 0.6444004775717705469, -0.5449076811759709926 ) ) ;
#15211=DIRECTION ( 'NONE',  ( -0.7660212471507179544, -0.6427876096865405842, -0.005961354470445141482 ) ) ;
#15212=FACE_OUTER_BOUND ( 'NONE', #11583, .T. ) ;
#15213=ORIENTED_EDGE ( 'NONE', *, *, #29841, .F. ) ;
#15214=VECTOR ( 'NONE', #48465, 999.9999999999998863 ) ;
#15215=LINE ( 'NONE', #32529, #5077 ) ;
#15216=ORIENTED_EDGE ( 'NONE', *, *, #16007, .F. ) ;
#15217=ORIENTED_EDGE ( 'NONE', *, *, #1015, .F. ) ;
#15219=FACE_OUTER_BOUND ( 'NONE', #13872, .T. ) ;
#15221=ORIENTED_EDGE ( 'NONE', *, *, #7986, .T. ) ;
#15222=DIRECTION ( 'NONE',  ( 0.5364919789714477361, 0.6444004775717706579, 0.5449076811759711036 ) ) ;
#15223=EDGE_LOOP ( 'NONE', ( #22179, #33695, #23316, #41400 ) ) ;
#15224=ADVANCED_FACE ( 'NONE', ( #14913 ), #23981, .F. ) ;
#15225=ORIENTED_EDGE ( 'NONE', *, *, #40811, .F. ) ;
#15226=CARTESIAN_POINT ( 'NONE',  ( -22.40634380310664397, 0.000000000000000000, 5.584705972946605534 ) ) ;
#15227=ORIENTED_EDGE ( 'NONE', *, *, #34209, .F. ) ;
#15228=ORIENTED_EDGE ( 'NONE', *, *, #51527, .T. ) ;
#15229=ADVANCED_FACE ( 'NONE', ( #50084 ), #49567, .F. ) ;
#15230=ADVANCED_FACE ( 'NONE', ( #11195 ), #49824, .F. ) ;
#15231=ORIENTED_EDGE ( 'NONE', *, *, #24483, .T. ) ;
#15232=LINE ( 'NONE', #54962, #2960 ) ;
#15233=DIRECTION ( 'NONE',  ( 0.6427681459581294776, -0.7660444431189769032, 0.005002170337467562802 ) ) ;
#15235=LINE ( 'NONE', #24555, #5081 ) ;
#15236=ORIENTED_EDGE ( 'NONE', *, *, #9372, .T. ) ;
#15238=ORIENTED_EDGE ( 'NONE', *, *, #21385, .F. ) ;
#15239=ORIENTED_EDGE ( 'NONE', *, *, #54873, .T. ) ;
#15240=FACE_OUTER_BOUND ( 'NONE', #10644, .T. ) ;
#15241=EDGE_CURVE ( 'NONE', #13117, #56078, #27401, .T. ) ;
#15243=LINE ( 'NONE', #40538, #3136 ) ;
#15244=DIRECTION ( 'NONE',  ( 0.007781995580012663651, 0.000000000000000000, -0.9999697198139515519 ) ) ;
#15245=CARTESIAN_POINT ( 'NONE',  ( -13.63328395545196159, 4.333955019861509328, 9.289710132824241740 ) ) ;
#15246=EDGE_LOOP ( 'NONE', ( #36455, #47686, #15817, #49005 ) ) ;
#15247=DIRECTION ( 'NONE',  ( 0.7660212471507180654, -0.6427876096865404731, 0.005961354470445141482 ) ) ;
#15248=ORIENTED_EDGE ( 'NONE', *, *, #31142, .F. ) ;
#15249=VECTOR ( 'NONE', #20808, 999.9999999999998863 ) ;
#15250=FACE_OUTER_BOUND ( 'NONE', #38258, .T. ) ;
#15251=DIRECTION ( 'NONE',  ( 0.5364919789714477361, 0.6444004775717706579, 0.5449076811759711036 ) ) ;
#15252=CARTESIAN_POINT ( 'NONE',  ( -9.952547186413761793, 0.000000000000000000, 3.634957892622900033 ) ) ;
#15253=DIRECTION ( 'NONE',  ( 0.005961354470445682716, -0.6427876096865404731, -0.7660212471507180654 ) ) ;
#15254=CARTESIAN_POINT ( 'NONE',  ( -15.25611291248567980, -2.137015261443160341, 2.739131496823017375 ) ) ;
#15255=VERTEX_POINT ( 'NONE', #19731 ) ;
#15257=DIRECTION ( 'NONE',  ( 0.9999697198139515519, 0.000000000000000000, 0.007781995580013368816 ) ) ;
#15258=FACE_OUTER_BOUND ( 'NONE', #45696, .T. ) ;
#15260=ADVANCED_FACE ( 'NONE', ( #40760 ), #44722, .F. ) ;
#15261=DIRECTION ( 'NONE',  ( 0.000000000000000000, -1.000000000000000000, 0.000000000000000000 ) ) ;
#15262=CARTESIAN_POINT ( 'NONE',  ( -9.442067484779661513, -0.1191753592594197858, 10.59804618892231254 ) ) ;
#15263=CARTESIAN_POINT ( 'NONE',  ( -14.46888367232926420, 0.000000000000000000, 12.59025272694991315 ) ) ;
#15264=FACE_OUTER_BOUND ( 'NONE', #21369, .T. ) ;
#15265=CARTESIAN_POINT ( 'NONE',  ( -20.19048558356006495, 0.000000000000000000, 5.601950293978301687 ) ) ;
#15266=EDGE_CURVE ( 'NONE', #33543, #27412, #15452, .T. ) ;
#15267=ORIENTED_EDGE ( 'NONE', *, *, #5344, .F. ) ;
#15268=EDGE_CURVE ( 'NONE', #51780, #2633, #28519, .T. ) ;
#15269=EDGE_CURVE ( 'NONE', #44507, #48671, #18908, .T. ) ;
#15270=ORIENTED_EDGE ( 'NONE', *, *, #33779, .F. ) ;
#15271=ORIENTED_EDGE ( 'NONE', *, *, #50850, .F. ) ;
#15272=ORIENTED_EDGE ( 'NONE', *, *, #40795, .F. ) ;
#15273=ORIENTED_EDGE ( 'NONE', *, *, #3482, .T. ) ;
#15274=CARTESIAN_POINT ( 'NONE',  ( -20.67682646184930206, -3.594132820645662196, 4.798231048616345085 ) ) ;
#15275=EDGE_CURVE ( 'NONE', #13570, #36235, #31948, .T. ) ;
#15276=CARTESIAN_POINT ( 'NONE',  ( -1.753914626039396296, 5.922546351860411562, 3.899653579608918896 ) ) ;
#15277=AXIS2_PLACEMENT_3D ( 'NONE', #34255, #21164, #51562 ) ;
#15278=ORIENTED_EDGE ( 'NONE', *, *, #1371, .T. ) ;
#15279=EDGE_CURVE ( 'NONE', #12863, #17764, #28820, .T. ) ;
#15280=DIRECTION ( 'NONE',  ( 0.005961354470445682716, -0.6427876096865404731, -0.7660212471507180654 ) ) ;
#15282=ORIENTED_EDGE ( 'NONE', *, *, #7716, .T. ) ;
#15283=ADVANCED_FACE ( 'NONE', ( #38155 ), #46681, .F. ) ;
#15285=CARTESIAN_POINT ( 'NONE',  ( -8.443718568120347712, 8.231294610302708037, 6.498200617411320934 ) ) ;
#15286=LINE ( 'NONE', #11003, #16874 ) ;
#15287=VERTEX_POINT ( 'NONE', #11499 ) ;
#15288=CARTESIAN_POINT ( 'NONE',  ( -20.52784467904771759, 0.000000000000000000, 14.94375894514125491 ) ) ;
#15289=EDGE_CURVE ( 'NONE', #8713, #44261, #24528, .T. ) ;
#15290=DIRECTION ( 'NONE',  ( -0.7660212471507179544, -0.6427876096865405842, -0.005961354470445141482 ) ) ;
#15291=LINE ( 'NONE', #53895, #42945 ) ;
#15292=EDGE_CURVE ( 'NONE', #54772, #43897, #2667, .T. ) ;
#15293=DIRECTION ( 'NONE',  ( 0.007781995580012663651, 0.000000000000000000, -0.9999697198139515519 ) ) ;
#15294=DIRECTION ( 'NONE',  ( -0.5364919789714478471, 0.6444004775717705469, -0.5449076811759709926 ) ) ;
#15296=DIRECTION ( 'NONE',  ( -0.7660212471507179544, -0.6427876096865405842, -0.005961354470445141482 ) ) ;
#15297=PLANE ( 'NONE',  #42052 ) ;
#15298=DIRECTION ( 'NONE',  ( -0.5449076811759708816, 0.6444004775717707689, 0.5364919789714475140 ) ) ;
#15299=ORIENTED_EDGE ( 'NONE', *, *, #20054, .T. ) ;
#15300=FACE_OUTER_BOUND ( 'NONE', #54624, .T. ) ;
#15301=ORIENTED_EDGE ( 'NONE', *, *, #16576, .F. ) ;
#15302=CARTESIAN_POINT ( 'NONE',  ( 1.086233639165236964, 0.000000000000000000, 2.796443541562362078 ) ) ;
#15303=CARTESIAN_POINT ( 'NONE',  ( -16.39848171883952332, -0.1191753592594198830, 8.855446145018868620 ) ) ;
#15304=PLANE ( 'NONE',  #29499 ) ;
#15305=DIRECTION ( 'NONE',  ( 0.005002170337468016433, -0.7660444431189770143, -0.6427681459581293666 ) ) ;
#15306=CARTESIAN_POINT ( 'NONE',  ( -26.13337879274045505, 0.000000000000000000, 6.833023547870798353 ) ) ;
#15307=CARTESIAN_POINT ( 'NONE',  ( -15.83019559695375911, 0.000000000000000000, 8.390533581105717786 ) ) ;
#15308=DIRECTION ( 'NONE',  ( 0.005002170337468016433, -0.7660444431189770143, -0.6427681459581293666 ) ) ;
#15310=DIRECTION ( 'NONE',  ( 0.007781995580012663651, -3.146120232559066537E-19, -0.9999697198139514409 ) ) ;
#15312=CARTESIAN_POINT ( 'NONE',  ( -20.54049170961573267, 0.000000000000000000, 4.660556269540326646 ) ) ;
#15313=CARTESIAN_POINT ( 'NONE',  ( -20.42542555003737093, -0.2049780936125319142, 5.058787616018051381 ) ) ;
#15314=LINE ( 'NONE', #45678, #54077 ) ;
#15315=AXIS2_PLACEMENT_3D ( 'NONE', #14816, #22513, #44082 ) ;
#15316=FACE_OUTER_BOUND ( 'NONE', #43747, .T. ) ;
#15317=ADVANCED_FACE ( 'NONE', ( #20835 ), #55204, .F. ) ;
#15318=PLANE ( 'NONE',  #27564 ) ;
#15319=DIRECTION ( 'NONE',  ( 0.000000000000000000, -1.000000000000000000, 0.000000000000000000 ) ) ;
#15320=LINE ( 'NONE', #53646, #45586 ) ;
#15321=VERTEX_POINT ( 'NONE', #29678 ) ;
#15322=DIRECTION ( 'NONE',  ( 0.007781995580012662783, 0.000000000000000000, -0.9999697198139514409 ) ) ;
#15323=EDGE_LOOP ( 'NONE', ( #46477, #33424, #34494 ) ) ;
#15324=PLANE ( 'NONE',  #5096 ) ;
#15325=CARTESIAN_POINT ( 'NONE',  ( -14.17413731849972613, 0.000000000000000000, 8.724089865898580598 ) ) ;
#15326=VERTEX_POINT ( 'NONE', #25127 ) ;
#15327=CARTESIAN_POINT ( 'NONE',  ( -18.28310086152664127, -0.1941918491731536578, 4.102410910690207579 ) ) ;
#15328=ORIENTED_EDGE ( 'NONE', *, *, #51503, .F. ) ;
#15330=EDGE_CURVE ( 'NONE', #10233, #24902, #16038, .T. ) ;
#15331=ORIENTED_EDGE ( 'NONE', *, *, #3822, .F. ) ;
#15332=EDGE_LOOP ( 'NONE', ( #42274, #50101, #22133, #39367 ) ) ;
#15333=ORIENTED_EDGE ( 'NONE', *, *, #16068, .T. ) ;
#15334=FACE_OUTER_BOUND ( 'NONE', #28828, .T. ) ;
#15335=CARTESIAN_POINT ( 'NONE',  ( -12.23851102634202448, -0.1191753592594197858, 11.68427982808754884 ) ) ;
#15336=DIRECTION ( 'NONE',  ( 0.005961354470445682716, -0.6427876096865404731, -0.7660212471507180654 ) ) ;
#15337=EDGE_CURVE ( 'NONE', #33548, #33876, #20576, .T. ) ;
#15338=VERTEX_POINT ( 'NONE', #41841 ) ;
#15339=ORIENTED_EDGE ( 'NONE', *, *, #33475, .F. ) ;
#15340=EDGE_CURVE ( 'NONE', #30955, #40959, #29075, .T. ) ;
#15342=ORIENTED_EDGE ( 'NONE', *, *, #20590, .F. ) ;
#15343=CARTESIAN_POINT ( 'NONE',  ( -15.62609718784551838, 0.1245042932765041271, 2.747666204937259771 ) ) ;
#15344=ORIENTED_EDGE ( 'NONE', *, *, #4103, .F. ) ;
#15345=CARTESIAN_POINT ( 'NONE',  ( -18.39611916365119271, 3.362543313726509719, 9.545504970550553026 ) ) ;
#15346=LINE ( 'NONE', #33248, #16756 ) ;
#15347=ADVANCED_FACE ( 'NONE', ( #25385 ), #2939, .F. ) ;
#15348=AXIS2_PLACEMENT_3D ( 'NONE', #11099, #11673, #49987 ) ;
#15349=ORIENTED_EDGE ( 'NONE', *, *, #53064, .F. ) ;
#15350=CARTESIAN_POINT ( 'NONE',  ( -15.36555870011267366, 0.000000000000000000, 8.394149492873728136 ) ) ;
#15351=EDGE_CURVE ( 'NONE', #49806, #29206, #42140, .T. ) ;
#15352=CARTESIAN_POINT ( 'NONE',  ( -18.72630217577924583, -0.1191753592594160666, 9.433079126556494387 ) ) ;
#15353=ORIENTED_EDGE ( 'NONE', *, *, #37623, .F. ) ;
#15354=DIRECTION ( 'NONE',  ( 0.000000000000000000, -1.000000000000000000, 0.000000000000000000 ) ) ;
#15355=CARTESIAN_POINT ( 'NONE',  ( -16.81345671998191449, 0.000000000000000000, 3.412238694616132495 ) ) ;
#15356=ORIENTED_EDGE ( 'NONE', *, *, #42390, .F. ) ;
#15357=DIRECTION ( 'NONE',  ( -0.5449076811759708816, 0.6444004775717707689, 0.5364919789714475140 ) ) ;
#15358=LINE ( 'NONE', #49155, #16037 ) ;
#15359=DIRECTION ( 'NONE',  ( -0.9321478471874540261, 0.000000000000000000, 0.3620778797217457656 ) ) ;
#15360=DIRECTION ( 'NONE',  ( -0.6427681459581293666, -0.7660444431189770143, -0.005002170337467561935 ) ) ;
#15361=DIRECTION ( 'NONE',  ( 0.9999697198139515519, 0.000000000000000000, 0.007781995580013368816 ) ) ;
#15362=CARTESIAN_POINT ( 'NONE',  ( -28.92982233430281980, 0.000000000000000000, 7.919257187036034651 ) ) ;
#15364=VERTEX_POINT ( 'NONE', #46380 ) ;
#15365=PLANE ( 'NONE',  #27116 ) ;
#15366=CARTESIAN_POINT ( 'NONE',  ( -21.47263955680318404, 0.000000000000000000, 5.022634149262071190 ) ) ;
#15368=ORIENTED_EDGE ( 'NONE', *, *, #54714, .F. ) ;
#15369=DIRECTION ( 'NONE',  ( -0.005002170337468016433, -0.7660444431189770143, 0.6427681459581293666 ) ) ;
#15370=FACE_OUTER_BOUND ( 'NONE', #11600, .T. ) ;
#15372=EDGE_CURVE ( 'NONE', #41034, #19170, #54620, .T. ) ;
#15373=PLANE ( 'NONE',  #29665 ) ;
#15374=CARTESIAN_POINT ( 'NONE',  ( -13.20345603875051665, 5.467268677019013090, 10.98271116061314956 ) ) ;
#15375=ORIENTED_EDGE ( 'NONE', *, *, #7002, .T. ) ;
#15376=EDGE_CURVE ( 'NONE', #32426, #41467, #33613, .T. ) ;
#15377=ORIENTED_EDGE ( 'NONE', *, *, #17837, .F. ) ;
#15378=EDGE_CURVE ( 'NONE', #45628, #98, #42433, .T. ) ;
#15379=CARTESIAN_POINT ( 'NONE',  ( -21.47419595591918906, 0.000000000000000000, 5.222628093224860102 ) ) ;
#15380=EDGE_CURVE ( 'NONE', #17338, #34543, #3789, .T. ) ;
#15381=EDGE_CURVE ( 'NONE', #44617, #54969, #50389, .T. ) ;
#15382=ADVANCED_FACE ( 'NONE', ( #19333 ), #15618, .F. ) ;
#15383=CARTESIAN_POINT ( 'NONE',  ( 2.072287782118878319, 0.000000000000000000, -2.950529333540147015 ) ) ;
#15384=VERTEX_POINT ( 'NONE', #28718 ) ;
#15385=FACE_OUTER_BOUND ( 'NONE', #29354, .T. ) ;
#15386=ORIENTED_EDGE ( 'NONE', *, *, #50894, .F. ) ;
#15387=LINE ( 'NONE', #40943, #2926 ) ;
#15388=VERTEX_POINT ( 'NONE', #2830 ) ;
#15389=ORIENTED_EDGE ( 'NONE', *, *, #17009, .F. ) ;
#15390=CARTESIAN_POINT ( 'NONE',  ( -9.941050972392631024, 0.000000000000000000, 2.157719079591843059 ) ) ;
#15391=FACE_OUTER_BOUND ( 'NONE', #49064, .T. ) ;
#15392=DIRECTION ( 'NONE',  ( 0.9999697198139515519, 0.000000000000000000, 0.007781995580013368816 ) ) ;
#15394=CARTESIAN_POINT ( 'NONE',  ( -13.22955429145962469, 0.000000000000000000, 6.764118080271738442 ) ) ;
#15395=ADVANCED_FACE ( 'NONE', ( #11089 ), #36671, .F. ) ;
#15396=ORIENTED_EDGE ( 'NONE', *, *, #30363, .T. ) ;
#15397=ADVANCED_FACE ( 'NONE', ( #53431 ), #19633, .F. ) ;
#15398=ORIENTED_EDGE ( 'NONE', *, *, #5228, .F. ) ;
#15399=ORIENTED_EDGE ( 'NONE', *, *, #32306, .T. ) ;
#15400=DIRECTION ( 'NONE',  ( 0.5449076811759707706, 0.6444004775717708799, -0.5364919789714476250 ) ) ;
#15401=EDGE_CURVE ( 'NONE', #45158, #54577, #14527, .T. ) ;
#15402=EDGE_LOOP ( 'NONE', ( #4663, #34833, #13218, #46300 ) ) ;
#15403=DIRECTION ( 'NONE',  ( 0.000000000000000000, -0.000000000000000000, -1.000000000000000000 ) ) ;
#15404=EDGE_LOOP ( 'NONE', ( #5101, #4318, #50292, #42505 ) ) ;
#15405=CARTESIAN_POINT ( 'NONE',  ( -19.32961685222932147, 0.000000000000000000, 14.39908572644263351 ) ) ;
#15407=ADVANCED_FACE ( 'NONE', ( #40915 ), #1996, .F. ) ;
#15408=ORIENTED_EDGE ( 'NONE', *, *, #13346, .T. ) ;
#15409=DIRECTION ( 'NONE',  ( 0.000000000000000000, -0.000000000000000000, -1.000000000000000000 ) ) ;
#15410=VERTEX_POINT ( 'NONE', #54265 ) ;
#15411=VECTOR ( 'NONE', #44198, 999.9999999999998863 ) ;
#15412=CARTESIAN_POINT ( 'NONE',  ( -23.33771345073609638, -0.1191753592594197858, 5.846786880686956955 ) ) ;
#15413=CARTESIAN_POINT ( 'NONE',  ( -19.60912206198628027, -0.1191753592594197858, 4.398475361799976113 ) ) ;
#15414=DIRECTION ( 'NONE',  ( -0.6427681459581293666, -0.7660444431189770143, -0.005002170337467561935 ) ) ;
#15415=FACE_OUTER_BOUND ( 'NONE', #41105, .T. ) ;
#15416=CARTESIAN_POINT ( 'NONE',  ( -18.67775241435682432, 0.000000000000000000, 4.136394454059623804 ) ) ;
#15417=LINE ( 'NONE', #37022, #4758 ) ;
#15418=ORIENTED_EDGE ( 'NONE', *, *, #8767, .T. ) ;
#15419=ORIENTED_EDGE ( 'NONE', *, *, #51725, .F. ) ;
#15420=DIRECTION ( 'NONE',  ( -0.7660212471507179544, -0.6427876096865405842, -0.005961354470445141482 ) ) ;
#15421=DIRECTION ( 'NONE',  ( -0.7660212471507179544, -0.6427876096865405842, -0.005961354470445141482 ) ) ;
#15422=LINE ( 'NONE', #37280, #47544 ) ;
#15423=FACE_OUTER_BOUND ( 'NONE', #5851, .T. ) ;
#15424=DIRECTION ( 'NONE',  ( 0.007781995580012662783, 0.000000000000000000, -0.9999697198139514409 ) ) ;
#15425=ORIENTED_EDGE ( 'NONE', *, *, #18551, .T. ) ;
#15426=CARTESIAN_POINT ( 'NONE',  ( -16.43317633868556626, -0.1191753592594197858, 13.31363028683540151 ) ) ;
#15427=DIRECTION ( 'NONE',  ( 0.000000000000000000, -0.000000000000000000, -1.000000000000000000 ) ) ;
#15429=DIRECTION ( 'NONE',  ( -0.6427681459581293666, -0.7660444431189770143, -0.005002170337467561935 ) ) ;
#15430=CARTESIAN_POINT ( 'NONE',  ( -22.40634380310664397, 0.000000000000000000, 5.584705972946605534 ) ) ;
#15431=EDGE_LOOP ( 'NONE', ( #13787, #49812, #41003, #17341 ) ) ;
#15432=FACE_OUTER_BOUND ( 'NONE', #36267, .T. ) ;
#15433=LINE ( 'NONE', #3223, #24232 ) ;
#15434=CARTESIAN_POINT ( 'NONE',  ( -26.13493519185646008, 0.000000000000000000, 7.033017491833586377 ) ) ;
#15435=PLANE ( 'NONE',  #23286 ) ;
#15436=DIRECTION ( 'NONE',  ( 0.007781995580012663651, 0.000000000000000000, -0.9999697198139515519 ) ) ;
#15437=ORIENTED_EDGE ( 'NONE', *, *, #28594, .T. ) ;
#15438=EDGE_CURVE ( 'NONE', #3168, #55625, #10827, .T. ) ;
#15439=ORIENTED_EDGE ( 'NONE', *, *, #43049, .F. ) ;
#15440=LINE ( 'NONE', #23969, #52044 ) ;
#15441=FACE_OUTER_BOUND ( 'NONE', #48811, .T. ) ;
#15442=LINE ( 'NONE', #32765, #32349 ) ;
#15443=EDGE_CURVE ( 'NONE', #9714, #1292, #24430, .T. ) ;
#15444=ADVANCED_FACE ( 'NONE', ( #6031 ), #6560, .F. ) ;
#15445=CARTESIAN_POINT ( 'NONE',  ( -13.61720543878437439, -0.1191753592594146788, 8.507758610330894200 ) ) ;
#15446=CARTESIAN_POINT ( 'NONE',  ( -21.47693870893288093, 3.200641362704010007, 4.922186869281591548 ) ) ;
#15447=LINE ( 'NONE', #28515, #27655 ) ;
#15448=EDGE_LOOP ( 'NONE', ( #15225, #14490, #18398 ) ) ;
#15449=EDGE_CURVE ( 'NONE', #18021, #25146, #14807, .T. ) ;
#15450=DIRECTION ( 'NONE',  ( -0.005961354470445682716, -0.6427876096865404731, 0.7660212471507180654 ) ) ;
#15451=VECTOR ( 'NONE', #51282, 1000.000000000000227 ) ;
#15452=LINE ( 'NONE', #32773, #25077 ) ;
#15453=CARTESIAN_POINT ( 'NONE',  ( -19.99180929398655593, 0.000000000000000000, 5.772822452389281267 ) ) ;
#15454=ORIENTED_EDGE ( 'NONE', *, *, #31695, .F. ) ;
#15455=CARTESIAN_POINT ( 'NONE',  ( -14.40136551438387436, -1.651309408375657428, 4.985991233126853217 ) ) ;
#15456=CARTESIAN_POINT ( 'NONE',  ( -14.87086361382948141, 0.000000000000000000, 4.535352612769118608 ) ) ;
#15457=DIRECTION ( 'NONE',  ( -0.5364919789714478471, 0.6444004775717705469, -0.5449076811759709926 ) ) ;
#15458=ORIENTED_EDGE ( 'NONE', *, *, #2792, .T. ) ;
#15459=CARTESIAN_POINT ( 'NONE',  ( -18.67775241435682432, 0.000000000000000000, 4.136394454059623804 ) ) ;
#15460=VERTEX_POINT ( 'NONE', #31843 ) ;
#15461=EDGE_CURVE ( 'NONE', #17816, #19391, #15358, .T. ) ;
#15462=ORIENTED_EDGE ( 'NONE', *, *, #8653, .T. ) ;
#15463=EDGE_LOOP ( 'NONE', ( #13953, #13330, #36458, #30076 ) ) ;
#15464=ORIENTED_EDGE ( 'NONE', *, *, #2520, .F. ) ;
#15465=EDGE_CURVE ( 'NONE', #27011, #36001, #1734, .T. ) ;
#15466=EDGE_LOOP ( 'NONE', ( #3438, #48031, #35825, #39855 ) ) ;
#15467=DIRECTION ( 'NONE',  ( 0.007781995580012663651, -3.146120232559066537E-19, -0.9999697198139514409 ) ) ;
#15468=ORIENTED_EDGE ( 'NONE', *, *, #44825, .T. ) ;
#15469=ADVANCED_FACE ( 'NONE', ( #49978 ), #45728, .F. ) ;
#15470=VERTEX_POINT ( 'NONE', #36379 ) ;
#15472=EDGE_LOOP ( 'NONE', ( #18736, #46857, #28168, #12973 ) ) ;
#15473=ORIENTED_EDGE ( 'NONE', *, *, #27573, .T. ) ;
#15474=EDGE_CURVE ( 'NONE', #883, #45963, #23872, .T. ) ;
#15475=ORIENTED_EDGE ( 'NONE', *, *, #34804, .F. ) ;
#15476=CARTESIAN_POINT ( 'NONE',  ( -19.22540549493500350, 3.848249166794009302, 4.026952827025455761 ) ) ;
#15477=LINE ( 'NONE', #55796, #11271 ) ;
#15479=DIRECTION ( 'NONE',  ( 0.9999697198139515519, 0.000000000000000000, 0.007781995580013368816 ) ) ;
#15480=ORIENTED_EDGE ( 'NONE', *, *, #53130, .F. ) ;
#15481=CARTESIAN_POINT ( 'NONE',  ( -18.25415525269858463, -0.1191753592594158168, 8.471672794689057540 ) ) ;
#15482=VERTEX_POINT ( 'NONE', #45195 ) ;
#15483=ORIENTED_EDGE ( 'NONE', *, *, #47711, .F. ) ;
#15485=LINE ( 'NONE', #3286, #23075 ) ;
#15486=CARTESIAN_POINT ( 'NONE',  ( -9.908141408373387193, -0.1191753592594197858, 10.77908512878318703 ) ) ;
#15487=UNCERTAINTY_MEASURE_WITH_UNIT (LENGTH_MEASURE( 1.000000000000000082E-05 ), #40020, 'distance_accuracy_value', 'NONE');
#15489=DIRECTION ( 'NONE',  ( 0.000000000000000000, -1.000000000000000000, 0.000000000000000000 ) ) ;
#15490=DIRECTION ( 'NONE',  ( 0.005002170337468016433, -0.7660444431189770143, -0.6427681459581293666 ) ) ;
#15491=FACE_OUTER_BOUND ( 'NONE', #42158, .T. ) ;
#15492=PLANE ( 'NONE',  #18639 ) ;
#15493=ORIENTED_EDGE ( 'NONE', *, *, #55348, .F. ) ;
#15494=DIRECTION ( 'NONE',  ( 0.007781995580012663651, 0.000000000000000000, -0.9999697198139515519 ) ) ;
#15495=ORIENTED_EDGE ( 'NONE', *, *, #35106, .F. ) ;
#15496=DIRECTION ( 'NONE',  ( 0.005002170337468016433, -0.7660444431189770143, -0.6427681459581293666 ) ) ;
#15497=CARTESIAN_POINT ( 'NONE',  ( -9.955421239919042264, 0.000000000000000000, 4.004267595880665276 ) ) ;
#15499=PLANE ( 'NONE',  #9581 ) ;
#15500=DIRECTION ( 'NONE',  ( 0.007781995580012662783, 0.000000000000000000, -0.9999697198139514409 ) ) ;
#15501=ORIENTED_EDGE ( 'NONE', *, *, #43021, .F. ) ;
#15502=DIRECTION ( 'NONE',  ( 0.9999697198139515519, 0.000000000000000000, 0.007781995580013368816 ) ) ;
#15503=DIRECTION ( 'NONE',  ( 0.000000000000000000, -0.000000000000000000, -1.000000000000000000 ) ) ;
#15504=CARTESIAN_POINT ( 'NONE',  ( -15.23885966822254368, 0.7721120973665037690, 2.576587922124613517 ) ) ;
#15506=EDGE_CURVE ( 'NONE', #36899, #3799, #19895, .T. ) ;
#15508=AXIS2_PLACEMENT_3D ( 'NONE', #26722, #9710, #36109 ) ;
#15509=CARTESIAN_POINT ( 'NONE',  ( -19.08498593125663234, -3.917936722690662954, 4.169575087627404031 ) ) ;
#15510=DIRECTION ( 'NONE',  ( 0.9999697198139515519, 0.000000000000000000, 0.007781995580013368816 ) ) ;
#15511=EDGE_CURVE ( 'NONE', #24571, #50552, #50272, .T. ) ;
#15512=PLANE ( 'NONE',  #45421 ) ;
#15513=ADVANCED_FACE ( 'NONE', ( #3689 ), #37492, .F. ) ;
#15514=DIRECTION ( 'NONE',  ( 0.6427681459581294776, -0.7660444431189769032, 0.005002170337467562802 ) ) ;
#15515=CARTESIAN_POINT ( 'NONE',  ( -22.40634380310664397, 0.000000000000000000, 5.584705972946605534 ) ) ;
#15516=DIRECTION ( 'NONE',  ( 0.007781995580012663651, -3.146120232559066537E-19, -0.9999697198139514409 ) ) ;
#15517=ORIENTED_EDGE ( 'NONE', *, *, #50755, .F. ) ;
#15519=AXIS2_PLACEMENT_3D ( 'NONE', #21282, #38897, #4525 ) ;
#15520=ORIENTED_EDGE ( 'NONE', *, *, #52011, .F. ) ;
#15521=ORIENTED_EDGE ( 'NONE', *, *, #5581, .F. ) ;
#15522=VERTEX_POINT ( 'NONE', #12518 ) ;
#15523=ORIENTED_EDGE ( 'NONE', *, *, #26643, .F. ) ;
#15524=DIRECTION ( 'NONE',  ( 0.007781995580012663651, 0.000000000000000000, -0.9999697198139515519 ) ) ;
#15525=CARTESIAN_POINT ( 'NONE',  ( -21.75645231962154824, -2.622721114510657703, 9.437208831783232554 ) ) ;
#15526=DIRECTION ( 'NONE',  ( -0.005961354470445682716, -0.6427876096865404731, 0.7660212471507180654 ) ) ;
#15527=EDGE_LOOP ( 'NONE', ( #51783, #19382, #47102, #32026 ) ) ;
#15528=ORIENTED_EDGE ( 'NONE', *, *, #28403, .F. ) ;
#15529=VERTEX_POINT ( 'NONE', #25552 ) ;
#15530=ORIENTED_EDGE ( 'NONE', *, *, #480, .T. ) ;
#15531=ADVANCED_FACE ( 'NONE', ( #15924 ), #42027, .F. ) ;
#15533=ADVANCED_FACE ( 'NONE', ( #55959 ), #34100, .F. ) ;
#15534=CARTESIAN_POINT ( 'NONE',  ( -14.56888064431065821, -0.1191753592594197858, 12.58947452739191064 ) ) ;
#15535=DIRECTION ( 'NONE',  ( 0.7660212471507180654, -0.6427876096865404731, 0.005961354470445141482 ) ) ;
#15536=ORIENTED_EDGE ( 'NONE', *, *, #19834, .F. ) ;
#15537=DIRECTION ( 'NONE',  ( 0.9321478471874541372, 0.000000000000000000, -0.3620778797217453771 ) ) ;
#15538=VERTEX_POINT ( 'NONE', #3428 ) ;
#15539=VECTOR ( 'NONE', #22594, 999.9999999999998863 ) ;
#15540=VECTOR ( 'NONE', #29168, 1000.000000000000114 ) ;
#15541=CARTESIAN_POINT ( 'NONE',  ( -13.55751301594631286, -0.1191753592594181482, 2.047824894809781249 ) ) ;
#15542=ADVANCED_FACE ( 'NONE', ( #50570 ), #20465, .F. ) ;
#15543=CARTESIAN_POINT ( 'NONE',  ( -12.28722788464031979, 0.000000000000000000, 5.094117146813910146 ) ) ;
#15544=DIRECTION ( 'NONE',  ( 0.005961354470445682716, -0.6427876096865404731, -0.7660212471507180654 ) ) ;
#15545=CARTESIAN_POINT ( 'NONE',  ( -11.37675481110584741, 0.000000000000000000, 7.517201133859304996 ) ) ;
#15546=VECTOR ( 'NONE', #11991, 999.9999999999998863 ) ;
#15549=LINE ( 'NONE', #32879, #23990 ) ;
#15550=CARTESIAN_POINT ( 'NONE',  ( -9.302286613136297788, 0.000000000000000000, 5.486678719795735404 ) ) ;
#15551=PLANE ( 'NONE',  #48341 ) ;
#15552=VERTEX_POINT ( 'NONE', #38061 ) ;
#15554=EDGE_LOOP ( 'NONE', ( #42809, #34608, #20537, #3721 ) ) ;
#15555=DIRECTION ( 'NONE',  ( 0.000000000000000000, -1.000000000000000000, 0.000000000000000000 ) ) ;
#15556=CARTESIAN_POINT ( 'NONE',  ( -10.67895298262786241, 0.000000000000000000, 3.259972764945120005 ) ) ;
#15557=CARTESIAN_POINT ( 'NONE',  ( -13.70568740232184091, 0.000000000000000000, 8.237740981534788176 ) ) ;
#15558=FACE_OUTER_BOUND ( 'NONE', #25343, .T. ) ;
#15559=DIRECTION ( 'NONE',  ( -0.7660212471507179544, -0.6427876096865405842, -0.005961354470445141482 ) ) ;
#15560=ADVANCED_FACE ( 'NONE', ( #50826 ), #8236, .F. ) ;
#15561=VECTOR ( 'NONE', #37137, 1000.000000000000227 ) ;
#15562=LINE ( 'NONE', #55310, #10296 ) ;
#15563=EDGE_LOOP ( 'NONE', ( #18192, #20595, #2144, #36863 ) ) ;
#15564=CARTESIAN_POINT ( 'NONE',  ( -9.742613427545842697, 0.000000000000000000, 2.359269422670635219 ) ) ;
#15565=CARTESIAN_POINT ( 'NONE',  ( 2.072287782118878319, 0.000000000000000000, -2.950529333540147015 ) ) ;
#15567=EDGE_CURVE ( 'NONE', #15599, #34233, #55110, .T. ) ;
#15568=CARTESIAN_POINT ( 'NONE',  ( -9.342070512798265725, 0.000000000000000000, 10.59882438848031505 ) ) ;
#15569=DIRECTION ( 'NONE',  ( 0.005961354470445682716, -0.6427876096865404731, -0.7660212471507180654 ) ) ;
#15570=ADVANCED_FACE ( 'NONE', ( #33262 ), #25292, .F. ) ;
#15571=LINE ( 'NONE', #7627, #37275 ) ;
#15572=DIRECTION ( 'NONE',  ( 0.005961354470445682716, -0.6427876096865404731, -0.7660212471507180654 ) ) ;
#15573=DIRECTION ( 'NONE',  ( -0.005961354470445682716, -0.6427876096865404731, 0.7660212471507180654 ) ) ;
#15574=EDGE_CURVE ( 'NONE', #40214, #5277, #34369, .T. ) ;
#15575=DIRECTION ( 'NONE',  ( 0.9999697198139515519, 0.000000000000000000, 0.007781995580013368816 ) ) ;
#15576=ORIENTED_EDGE ( 'NONE', *, *, #11744, .T. ) ;
#15577=DIRECTION ( 'NONE',  ( 0.005961354470445682716, -0.6427876096865404731, -0.7660212471507180654 ) ) ;
#15578=ORIENTED_EDGE ( 'NONE', *, *, #25928, .T. ) ;
#15579=DIRECTION ( 'NONE',  ( 0.007781995580012663651, -3.146120232559066537E-19, -0.9999697198139514409 ) ) ;
#15580=DIRECTION ( 'NONE',  ( 0.6427681459581294776, -0.7660444431189769032, 0.005002170337467562802 ) ) ;
#15581=VECTOR ( 'NONE', #27325, 1000.000000000000227 ) ;
#15582=VECTOR ( 'NONE', #36739, 1000.000000000000227 ) ;
#15583=ORIENTED_EDGE ( 'NONE', *, *, #30628, .F. ) ;
#15584=ORIENTED_EDGE ( 'NONE', *, *, #51804, .F. ) ;
#15585=DIRECTION ( 'NONE',  ( 0.7660212471507180654, -0.6427876096865404731, 0.005961354470445141482 ) ) ;
#15586=EDGE_CURVE ( 'NONE', #18997, #33290, #30098, .T. ) ;
#15587=EDGE_LOOP ( 'NONE', ( #38447, #4394, #153, #45778 ) ) ;
#15588=ORIENTED_EDGE ( 'NONE', *, *, #37628, .F. ) ;
#15590=ORIENTED_EDGE ( 'NONE', *, *, #24722, .T. ) ;
#15591=DIRECTION ( 'NONE',  ( 0.6427681459581294776, -0.7660444431189769032, 0.005002170337467562802 ) ) ;
#15592=CARTESIAN_POINT ( 'NONE',  ( -13.95152963505244159, 0.000000000000000000, 5.819829305373406036 ) ) ;
#15593=FACE_OUTER_BOUND ( 'NONE', #47542, .T. ) ;
#15594=ORIENTED_EDGE ( 'NONE', *, *, #29078, .T. ) ;
#15595=VECTOR ( 'NONE', #40839, 1000.000000000000114 ) ;
#15596=EDGE_LOOP ( 'NONE', ( #49767, #42721, #55990, #40677 ) ) ;
#15597=PLANE ( 'NONE',  #30273 ) ;
#15598=DIRECTION ( 'NONE',  ( -0.005961354470445682716, -0.6427876096865404731, 0.7660212471507180654 ) ) ;
#15599=VERTEX_POINT ( 'NONE', #51113 ) ;
#15600=CARTESIAN_POINT ( 'NONE',  ( -26.13337879274045505, 0.000000000000000000, 6.833023547870798353 ) ) ;
#15601=EDGE_LOOP ( 'NONE', ( #31755, #3865, #14712, #51173 ) ) ;
#15602=CARTESIAN_POINT ( 'NONE',  ( -10.20281987176564442, 0.000000000000000000, 1.786349863682072936 ) ) ;
#15603=DIRECTION ( 'NONE',  ( -0.005002170337468016433, -0.7660444431189770143, 0.6427681459581293666 ) ) ;
#15604=ORIENTED_EDGE ( 'NONE', *, *, #29886, .F. ) ;
#15605=LINE ( 'NONE', #32664, #8682 ) ;
#15606=ADVANCED_FACE ( 'NONE', ( #43184 ), #42335, .F. ) ;
#15607=VECTOR ( 'NONE', #28656, 999.9999999999998863 ) ;
#15608=CYLINDRICAL_SURFACE ( 'NONE', #34542, 1.000000000000000444 ) ;
#15610=DIRECTION ( 'NONE',  ( -0.5449076811759708816, 0.6444004775717707689, 0.5364919789714475140 ) ) ;
#15611=AXIS2_PLACEMENT_3D ( 'NONE', #19729, #2666, #10375 ) ;
#15612=CARTESIAN_POINT ( 'NONE',  ( -20.54049170961573267, 0.000000000000000000, 4.660556269540326646 ) ) ;
#15613=EDGE_LOOP ( 'NONE', ( #29144, #16247, #16208, #4637 ) ) ;
#15614=EDGE_CURVE ( 'NONE', #35268, #8997, #16201, .T. ) ;
#15615=AXIS2_PLACEMENT_3D ( 'NONE', #7938, #54762, #38281 ) ;
#15616=VECTOR ( 'NONE', #35220, 999.9999999999998863 ) ;
#15618=PLANE ( 'NONE',  #4252 ) ;
#15619=LINE ( 'NONE', #49732, #14947 ) ;
#15620=LINE ( 'NONE', #54518, #36808 ) ;
#15621=EDGE_CURVE ( 'NONE', #3020, #26788, #25013, .T. ) ;
#15622=CARTESIAN_POINT ( 'NONE',  ( -27.06630483948590893, -0.1191753592594197858, 7.295098399573937797 ) ) ;
#15623=LINE ( 'NONE', #11389, #40627 ) ;
#15624=EDGE_CURVE ( 'NONE', #32592, #4309, #47134, .T. ) ;
#15625=VECTOR ( 'NONE', #33978, 1000.000000000000000 ) ;
#15626=FACE_OUTER_BOUND ( 'NONE', #23335, .T. ) ;
#15627=AXIS2_PLACEMENT_3D ( 'NONE', #42799, #7611, #7922 ) ;
#15628=VERTEX_POINT ( 'NONE', #16466 ) ;
#15632=ORIENTED_EDGE ( 'NONE', *, *, #49629, .T. ) ;
#15633=CARTESIAN_POINT ( 'NONE',  ( -24.26986129792355129, -0.1191753592594197858, 6.208864760408702388 ) ) ;
#15635=CARTESIAN_POINT ( 'NONE',  ( -13.92434549911562058, 0.000000000000000000, 2.326726216758550514 ) ) ;
#15636=EDGE_CURVE ( 'NONE', #21767, #34530, #51418, .T. ) ;
#15637=FACE_BOUND ( 'NONE', #54536, .T. ) ;
#15638=LINE ( 'NONE', #32978, #6993 ) ;
#15639=EDGE_CURVE ( 'NONE', #33398, #54767, #31218, .T. ) ;
#15641=EDGE_LOOP ( 'NONE', ( #11686, #42539, #30899, #18132 ) ) ;
#15642=ORIENTED_EDGE ( 'NONE', *, *, #15380, .F. ) ;
#15643=CARTESIAN_POINT ( 'NONE',  ( -12.76623504900782180, 0.000000000000000000, 6.937049751334724235 ) ) ;
#15644=FACE_OUTER_BOUND ( 'NONE', #34312, .T. ) ;
#15645=EDGE_CURVE ( 'NONE', #713, #9548, #259, .T. ) ;
#15646=DIRECTION ( 'NONE',  ( 0.005961354470445682716, -0.6427876096865404731, -0.7660212471507180654 ) ) ;
#15647=ORIENTED_EDGE ( 'NONE', *, *, #44506, .F. ) ;
#15648=DIRECTION ( 'NONE',  ( 0.9999697198139515519, 0.000000000000000000, 0.007781995580013368816 ) ) ;
#15649=VECTOR ( 'NONE', #28431, 999.9999999999998863 ) ;
#15650=EDGE_LOOP ( 'NONE', ( #40575, #15129, #39882, #43212 ) ) ;
#15651=CYLINDRICAL_SURFACE ( 'NONE', #25646, 1.000000000000000222 ) ;
#15652=ADVANCED_FACE ( 'NONE', ( #8830 ), #52520, .F. ) ;
#15653=EDGE_LOOP ( 'NONE', ( #26650, #19400, #12954, #1779 ) ) ;
#15654=ORIENTED_EDGE ( 'NONE', *, *, #40263, .F. ) ;
#15655=LINE ( 'NONE', #7722, #42018 ) ;
#15656=VECTOR ( 'NONE', #28376, 999.9999999999998863 ) ;
#15657=CARTESIAN_POINT ( 'NONE',  ( -10.32371341784202023, -0.1191753592594179401, 4.470736558909812253 ) ) ;
#15658=DIRECTION ( 'NONE',  ( -0.005002170337468016433, -0.7660444431189770143, 0.6427681459581293666 ) ) ;
#15659=VERTEX_POINT ( 'NONE', #9081 ) ;
#15660=VECTOR ( 'NONE', #38971, 1000.000000000000114 ) ;
#15661=AXIS2_PLACEMENT_3D ( 'NONE', #5890, #40802, #53321 ) ;
#15662=DIRECTION ( 'NONE',  ( 0.6427681459581294776, -0.7660444431189769032, 0.005002170337467562802 ) ) ;
#15663=ORIENTED_EDGE ( 'NONE', *, *, #1417, .F. ) ;
#15664=ORIENTED_EDGE ( 'NONE', *, *, #37190, .T. ) ;
#15665=AXIS2_PLACEMENT_3D ( 'NONE', #21699, #30779, #56062 ) ;
#15666=ORIENTED_EDGE ( 'NONE', *, *, #5406, .T. ) ;
#15667=PLANE ( 'NONE',  #21367 ) ;
#15668=AXIS2_PLACEMENT_3D ( 'NONE', #2310, #20480, #36977 ) ;
#15669=DIRECTION ( 'NONE',  ( -0.7660212471507179544, -0.6427876096865405842, -0.005961354470445141482 ) ) ;
#15670=ORIENTED_EDGE ( 'NONE', *, *, #50925, .T. ) ;
#15671=PLANE ( 'NONE',  #23924 ) ;
#15672=ORIENTED_EDGE ( 'NONE', *, *, #54541, .T. ) ;
#15674=DIRECTION ( 'NONE',  ( -0.005961354470445682716, -0.6427876096865404731, 0.7660212471507180654 ) ) ;
#15675=ORIENTED_EDGE ( 'NONE', *, *, #10148, .F. ) ;
#15676=CARTESIAN_POINT ( 'NONE',  ( -14.00280974873554030, 0.000000000000000000, 12.40921378708904044 ) ) ;
#15677=VECTOR ( 'NONE', #23657, 1000.000000000000227 ) ;
#15678=EDGE_CURVE ( 'NONE', #36899, #5305, #39755, .T. ) ;
#15679=ORIENTED_EDGE ( 'NONE', *, *, #6131, .T. ) ;
#15680=VECTOR ( 'NONE', #2958, 1000.000000000000227 ) ;
#15681=DIRECTION ( 'NONE',  ( 0.007781995580012663651, 0.000000000000000000, -0.9999697198139515519 ) ) ;
#15682=DIRECTION ( 'NONE',  ( 0.2426528472758542054, 0.7422098413412800966, 0.6246952433987894571 ) ) ;
#15683=PLANE ( 'NONE',  #6008 ) ;
#15684=DIRECTION ( 'NONE',  ( -0.5364919789714478471, 0.6444004775717705469, -0.5449076811759709926 ) ) ;
#15685=CARTESIAN_POINT ( 'NONE',  ( -21.47263955680318404, 0.000000000000000000, 5.022634149262071190 ) ) ;
#15686=DIRECTION ( 'NONE',  ( -0.005002170337468016433, -0.7660444431189770143, 0.6427681459581293666 ) ) ;
#15687=EDGE_LOOP ( 'NONE', ( #46985, #35852, #49604, #24713 ) ) ;
#15688=EDGE_CURVE ( 'NONE', #53048, #26165, #44292, .T. ) ;
#15689=VECTOR ( 'NONE', #41345, 1000.000000000000000 ) ;
#15690=EDGE_CURVE ( 'NONE', #36809, #41926, #38912, .T. ) ;
#15691=ORIENTED_EDGE ( 'NONE', *, *, #19245, .T. ) ;
#15692=FACE_OUTER_BOUND ( 'NONE', #19679, .T. ) ;
#15693=CARTESIAN_POINT ( 'NONE',  ( -9.175487151985130652, -0.1191753592594191058, 3.371676111792005770 ) ) ;
#15694=AXIS2_PLACEMENT_3D ( 'NONE', #38663, #17079, #8554 ) ;
#15695=CARTESIAN_POINT ( 'NONE',  ( -19.60834386242827776, 0.000000000000000000, 4.298478389818581213 ) ) ;
#15696=PLANE ( 'NONE',  #22168 ) ;
#15697=CARTESIAN_POINT ( 'NONE',  ( -16.81267852042391198, -0.1191753592594197858, 3.312241722634738039 ) ) ;
#15698=ADVANCED_FACE ( 'NONE', ( #5391 ), #5122, .F. ) ;
#15699=DIRECTION ( 'NONE',  ( -0.005961354470445682716, -0.6427876096865404731, 0.7660212471507180654 ) ) ;
#15700=VERTEX_POINT ( 'NONE', #30931 ) ;
#15701=LINE ( 'NONE', #28793, #24978 ) ;
#15704=AXIS2_PLACEMENT_3D ( 'NONE', #39013, #43296, #51525 ) ;
#15705=DIRECTION ( 'NONE',  ( -0.6246952433987893460, -0.7422098413412802076, 0.2426528472758542054 ) ) ;
#15706=DIRECTION ( 'NONE',  ( 0.9999697198139515519, 0.000000000000000000, 0.007781995580013368816 ) ) ;
#15707=ORIENTED_EDGE ( 'NONE', *, *, #26796, .F. ) ;
#15708=VECTOR ( 'NONE', #31385, 999.9999999999998863 ) ;
#15709=PLANE ( 'NONE',  #9823 ) ;
#15710=CARTESIAN_POINT ( 'NONE',  ( -22.40478740399063895, 0.000000000000000000, 5.384712028983816623 ) ) ;
#15711=EDGE_CURVE ( 'NONE', #9919, #47750, #573, .T. ) ;
#15712=CARTESIAN_POINT ( 'NONE',  ( -9.749679188945689745, 0.000000000000000000, 3.267204588481138927 ) ) ;
#15713=DIRECTION ( 'NONE',  ( 0.000000000000000000, -0.000000000000000000, -1.000000000000000000 ) ) ;
#15714=EDGE_CURVE ( 'NONE', #50133, #41831, #26678, .T. ) ;
#15715=CARTESIAN_POINT ( 'NONE',  ( -11.73199437589168781, -0.1191753592594185784, 6.306437339894606531 ) ) ;
#15716=EDGE_LOOP ( 'NONE', ( #9844, #29796, #18490, #50803 ) ) ;
#15718=ORIENTED_EDGE ( 'NONE', *, *, #39138, .F. ) ;
#15719=EDGE_CURVE ( 'NONE', #48671, #35152, #39472, .T. ) ;
#15720=DIRECTION ( 'NONE',  ( 0.007781995580012663651, 0.000000000000000000, -0.9999697198139515519 ) ) ;
#15721=DIRECTION ( 'NONE',  ( 0.9999697198139515519, 0.000000000000000000, 0.007781995580013368816 ) ) ;
#15723=FACE_OUTER_BOUND ( 'NONE', #52357, .T. ) ;
#15724=ADVANCED_FACE ( 'NONE', ( #17305 ), #13066, .F. ) ;
#15727=ORIENTED_EDGE ( 'NONE', *, *, #50033, .T. ) ;
#15728=DIRECTION ( 'NONE',  ( -0.7660212471507179544, -0.6427876096865405842, -0.005961354470445141482 ) ) ;
#15729=DIRECTION ( 'NONE',  ( 0.007781995580012663651, 0.000000000000000000, -0.9999697198139515519 ) ) ;
#15730=CARTESIAN_POINT ( 'NONE',  ( 2.072287782118878319, 0.000000000000000000, -2.950529333540147015 ) ) ;
#15731=ORIENTED_EDGE ( 'NONE', *, *, #2561, .F. ) ;
#15732=VECTOR ( 'NONE', #47836, 999.9999999999998863 ) ;
#15733=DIRECTION ( 'NONE',  ( 0.000000000000000000, -0.000000000000000000, -1.000000000000000000 ) ) ;
#15734=DIRECTION ( 'NONE',  ( 0.007781995580012663651, -3.146120232559066537E-19, -0.9999697198139514409 ) ) ;
#15735=AXIS2_PLACEMENT_3D ( 'NONE', #36585, #53076, #5944 ) ;
#15736=DIRECTION ( 'NONE',  ( 0.7660212471507180654, -0.6427876096865404731, 0.005961354470445141482 ) ) ;
#15737=VERTEX_POINT ( 'NONE', #14209 ) ;
#15738=DIRECTION ( 'NONE',  ( 0.7660212471507180654, -0.6427876096865404731, 0.005961354470445141482 ) ) ;
#15740=EDGE_LOOP ( 'NONE', ( #22617, #37455, #24581, #7667 ) ) ;
#15741=ORIENTED_EDGE ( 'NONE', *, *, #11387, .F. ) ;
#15742=ORIENTED_EDGE ( 'NONE', *, *, #34059, .T. ) ;
#15743=ORIENTED_EDGE ( 'NONE', *, *, #322, .T. ) ;
#15744=ORIENTED_EDGE ( 'NONE', *, *, #23710, .F. ) ;
#15746=DIRECTION ( 'NONE',  ( -0.6427681459581293666, -0.7660444431189770143, -0.005002170337467561935 ) ) ;
#15747=EDGE_LOOP ( 'NONE', ( #46901, #2543, #47568, #16786, #40826, #55078, #5234 ) ) ;
#15748=EDGE_CURVE ( 'NONE', #7193, #223, #53091, .T. ) ;
#15749=AXIS2_PLACEMENT_3D ( 'NONE', #53369, #5951, #44834 ) ;
#15750=VERTEX_POINT ( 'NONE', #9934 ) ;
#15751=PLANE ( 'NONE',  #23134 ) ;
#15752=ORIENTED_EDGE ( 'NONE', *, *, #37827, .F. ) ;
#15753=EDGE_CURVE ( 'NONE', #10299, #15737, #39172, .T. ) ;
#15754=ORIENTED_EDGE ( 'NONE', *, *, #20395, .F. ) ;
#15755=VECTOR ( 'NONE', #20975, 999.9999999999998863 ) ;
#15756=AXIS2_PLACEMENT_3D ( 'NONE', #5279, #5828, #1570 ) ;
#15757=PLANE ( 'NONE',  #49226 ) ;
#15758=CARTESIAN_POINT ( 'NONE',  ( 1.086233639165236964, 0.000000000000000000, 2.796443541562362078 ) ) ;
#15759=CARTESIAN_POINT ( 'NONE',  ( -13.08486533123210194, 0.000000000000000000, 1.963927175729152541 ) ) ;
#15760=DIRECTION ( 'NONE',  ( 0.9999697198139515519, 0.000000000000000000, 0.007781995580013368816 ) ) ;
#15761=ORIENTED_EDGE ( 'NONE', *, *, #27351, .T. ) ;
#15762=CARTESIAN_POINT ( 'NONE',  ( -23.33771345073609638, -0.1191753592594197858, 5.846786880686956955 ) ) ;
#15763=VERTEX_POINT ( 'NONE', #35476 ) ;
#15764=EDGE_CURVE ( 'NONE', #5026, #19711, #56216, .T. ) ;
#15765=ADVANCED_FACE ( 'NONE', ( #13891 ), #13365, .F. ) ;
#15766=EDGE_CURVE ( 'NONE', #2545, #46574, #17903, .T. ) ;
#15767=EDGE_LOOP ( 'NONE', ( #52236, #9981, #37002, #32843 ) ) ;
#15768=LINE ( 'NONE', #46150, #10396 ) ;
#15769=CARTESIAN_POINT ( 'NONE',  ( -21.47263955680318404, 0.000000000000000000, 5.022634149262071190 ) ) ;
#15770=ADVANCED_FACE ( 'NONE', ( #29309 ), #56011, .F. ) ;
#15771=DIRECTION ( 'NONE',  ( 0.007781995580012663651, -3.146120232559066537E-19, -0.9999697198139514409 ) ) ;
#15772=DIRECTION ( 'NONE',  ( 0.007781995580012663651, 0.000000000000000000, -0.9999697198139515519 ) ) ;
#15773=AXIS2_PLACEMENT_3D ( 'NONE', #30216, #13182, #17417 ) ;
#15774=DIRECTION ( 'NONE',  ( 0.005002170337468016433, -0.7660444431189770143, -0.6427681459581293666 ) ) ;
#15775=DIRECTION ( 'NONE',  ( -0.7660212471507179544, -0.6427876096865405842, -0.005961354470445141482 ) ) ;
#15776=ORIENTED_EDGE ( 'NONE', *, *, #21979, .T. ) ;
#15777=LINE ( 'NONE', #14960, #12972 ) ;
#15778=AXIS2_PLACEMENT_3D ( 'NONE', #7258, #54388, #24305 ) ;
#15779=VERTEX_POINT ( 'NONE', #46625 ) ;
#15780=DIRECTION ( 'NONE',  ( -0.005002170337468016433, -0.7660444431189770143, 0.6427681459581293666 ) ) ;
#15781=PLANE ( 'NONE',  #53192 ) ;
#15782=DIRECTION ( 'NONE',  ( 0.000000000000000000, -1.000000000000000000, 0.000000000000000000 ) ) ;
#15783=AXIS2_PLACEMENT_3D ( 'NONE', #39152, #51398, #8218 ) ;
#15784=CARTESIAN_POINT ( 'NONE',  ( -16.79925329029790149, 0.000000000000000000, 13.49544742625427496 ) ) ;
#15785=ADVANCED_FACE ( 'NONE', ( #4036 ), #38104, .F. ) ;
#15786=DIRECTION ( 'NONE',  ( 0.5449076811759707706, 0.6444004775717708799, -0.5364919789714476250 ) ) ;
#15787=EDGE_CURVE ( 'NONE', #16128, #45114, #38694, .T. ) ;
#15788=ORIENTED_EDGE ( 'NONE', *, *, #6050, .T. ) ;
#15789=ORIENTED_EDGE ( 'NONE', *, *, #12472, .T. ) ;
#15790=ADVANCED_FACE ( 'NONE', ( #17102 ), #12281, .F. ) ;
#15791=VECTOR ( 'NONE', #53880, 999.9999999999998863 ) ;
#15792=LINE ( 'NONE', #33134, #33933 ) ;
#15793=DIRECTION ( 'NONE',  ( 0.007781995580012663651, -3.146120232559066537E-19, -0.9999697198139514409 ) ) ;
#15794=CARTESIAN_POINT ( 'NONE',  ( -1.086233639165236964, 0.000000000000000000, -2.796443541562362078 ) ) ;
#15795=VECTOR ( 'NONE', #39947, 1000.000000000000227 ) ;
#15796=ADVANCED_FACE ( 'NONE', ( #8025 ), #12830, .F. ) ;
#15797=FACE_OUTER_BOUND ( 'NONE', #12503, .T. ) ;
#15798=PLANE ( 'NONE',  #19407 ) ;
#15799=DIRECTION ( 'NONE',  ( 0.7660212471507180654, -0.6427876096865404731, 0.005961354470445141482 ) ) ;
#15800=CARTESIAN_POINT ( 'NONE',  ( -11.22056963685719211, 0.000000000000000000, 1.239771416285661010 ) ) ;
#15801=EDGE_CURVE ( 'NONE', #9624, #46898, #21361, .T. ) ;
#15802=AXIS2_PLACEMENT_3D ( 'NONE', #45616, #6731, #28878 ) ;
#15803=VECTOR ( 'NONE', #54972, 1000.000000000000227 ) ;
#15805=DIRECTION ( 'NONE',  ( 0.5364919789714477361, 0.6444004775717706579, 0.5449076811759711036 ) ) ;
#15806=VERTEX_POINT ( 'NONE', #34683 ) ;
#15807=VECTOR ( 'NONE', #22894, 1000.000000000000227 ) ;
#15808=ORIENTED_EDGE ( 'NONE', *, *, #20447, .T. ) ;
#15809=VERTEX_POINT ( 'NONE', #3187 ) ;
#15810=ORIENTED_EDGE ( 'NONE', *, *, #4873, .T. ) ;
#15811=VECTOR ( 'NONE', #15060, 1000.000000000000114 ) ;
#15814=DIRECTION ( 'NONE',  ( -0.5449076811759708816, 0.6444004775717707689, 0.5364919789714475140 ) ) ;
#15815=CARTESIAN_POINT ( 'NONE',  ( -14.66887761629205222, 0.000000000000000000, 12.58869632783390990 ) ) ;
#15816=VECTOR ( 'NONE', #21917, 1000.000000000000227 ) ;
#15817=ORIENTED_EDGE ( 'NONE', *, *, #21440, .T. ) ;
#15818=FACE_OUTER_BOUND ( 'NONE', #44331, .T. ) ;
#15819=EDGE_LOOP ( 'NONE', ( #19747, #46329, #20612, #19517 ) ) ;
#15820=DIRECTION ( 'NONE',  ( 0.9999697198139515519, 0.000000000000000000, 0.007781995580013368816 ) ) ;
#15821=EDGE_LOOP ( 'NONE', ( #54698, #27244, #54440, #1700 ) ) ;
#15822=AXIS2_PLACEMENT_3D ( 'NONE', #46416, #28856, #29404 ) ;
#15825=PLANE ( 'NONE',  #1016 ) ;
#15826=DIRECTION ( 'NONE',  ( 0.5364919789714477361, 0.6444004775717706579, 0.5449076811759711036 ) ) ;
#15827=EDGE_LOOP ( 'NONE', ( #47477, #46814, #6142, #39279 ) ) ;
#15828=LINE ( 'NONE', #3616, #50945 ) ;
#15829=VERTEX_POINT ( 'NONE', #30152 ) ;
#15830=VECTOR ( 'NONE', #17058, 1000.000000000000227 ) ;
#15831=ADVANCED_FACE ( 'NONE', ( #43240 ), #20521, .F. ) ;
#15833=CARTESIAN_POINT ( 'NONE',  ( 1.086233639165236964, 0.000000000000000000, 2.796443541562362078 ) ) ;
#15834=CARTESIAN_POINT ( 'NONE',  ( -20.70246366968693508, 4.495856970884011261, 4.580030303656299928 ) ) ;
#15835=ADVANCED_FACE ( 'NONE', ( #37850 ), #50874, .F. ) ;
#15836=VECTOR ( 'NONE', #27981, 999.9999999999998863 ) ;
#15837=DIRECTION ( 'NONE',  ( -0.5449076811759708816, 0.6444004775717707689, 0.5364919789714475140 ) ) ;
#15838=LINE ( 'NONE', #37409, #19661 ) ;
#15839=AXIS2_PLACEMENT_3D ( 'NONE', #8961, #26264, #25421 ) ;
#15841=CARTESIAN_POINT ( 'NONE',  ( -17.13623937202426362, 3.524445264749008100, 9.321833557735295983 ) ) ;
#15842=DIRECTION ( 'NONE',  ( 0.9999697198139515519, 0.000000000000000000, 0.007781995580013368816 ) ) ;
#15843=CARTESIAN_POINT ( 'NONE',  ( -22.40478740399063895, 0.000000000000000000, 5.384712028983816623 ) ) ;
#15844=DIRECTION ( 'NONE',  ( -0.5449076811759708816, 0.6444004775717707689, 0.5364919789714475140 ) ) ;
#15845=ORIENTED_EDGE ( 'NONE', *, *, #27074, .F. ) ;
#15848=LINE ( 'NONE', #32364, #28366 ) ;
#15849=DIRECTION ( 'NONE',  ( 0.5364919789714477361, 0.6444004775717706579, 0.5449076811759711036 ) ) ;
#15850=LINE ( 'NONE', #24373, #55850 ) ;
#15851=CARTESIAN_POINT ( 'NONE',  ( -15.02486367781824939, -0.03739765774599677212, 2.656112488575108621 ) ) ;
#15852=CARTESIAN_POINT ( 'NONE',  ( -0.3920807322492407820, -4.603227297713195831, 3.370671047187119296 ) ) ;
#15853=VECTOR ( 'NONE', #50520, 1000.000000000000227 ) ;
#15856=VECTOR ( 'NONE', #29757, 1000.000000000000227 ) ;
#15857=ORIENTED_EDGE ( 'NONE', *, *, #24049, .T. ) ;
#15858=PLANE ( 'NONE',  #16554 ) ;
#15859=CARTESIAN_POINT ( 'NONE',  ( -18.19747506107908563, 0.000000000000000000, 14.03856424583689311 ) ) ;
#15860=DIRECTION ( 'NONE',  ( -0.6427681459581293666, -0.7660444431189770143, -0.005002170337467561935 ) ) ;
#15861=PLANE ( 'NONE',  #16420 ) ;
#15862=VECTOR ( 'NONE', #16331, 1000.000000000000227 ) ;
#15863=DIRECTION ( 'NONE',  ( -0.6427681459581293666, -0.7660444431189770143, -0.005002170337467561935 ) ) ;
#15864=CARTESIAN_POINT ( 'NONE',  ( -23.33849165029409889, 0.000000000000000000, 5.946783852668351855 ) ) ;
#15865=VECTOR ( 'NONE', #12510, 999.9999999999998863 ) ;
#15866=DIRECTION ( 'NONE',  ( 0.005961354470445682716, -0.6427876096865404731, -0.7660212471507180654 ) ) ;
#15867=EDGE_CURVE ( 'NONE', #34537, #36412, #25, .T. ) ;
#15868=PLANE ( 'NONE',  #46866 ) ;
#15869=CARTESIAN_POINT ( 'NONE',  ( -12.17271348132147679, -4.565544526780664469, 1.463951646762539971 ) ) ;
#15870=EDGE_LOOP ( 'NONE', ( #37320, #15227, #32743, #28626 ) ) ;
#15871=LINE ( 'NONE', #6516, #53899 ) ;
#15872=VECTOR ( 'NONE', #38566, 999.9999999999998863 ) ;
#15873=DIRECTION ( 'NONE',  ( 0.005002170337468016433, -0.7660444431189770143, -0.6427681459581293666 ) ) ;
#15874=AXIS2_PLACEMENT_3D ( 'NONE', #23667, #31917, #10893 ) ;
#15875=ORIENTED_EDGE ( 'NONE', *, *, #30008, .T. ) ;
#15876=ADVANCED_FACE ( 'NONE', ( #51469 ), #25338, .F. ) ;
#15877=VECTOR ( 'NONE', #16908, 1000.000000000000114 ) ;
#15878=CARTESIAN_POINT ( 'NONE',  ( -15.25286141696295594, -5.375054281893161701, 11.42804088947178087 ) ) ;
#15880=EDGE_CURVE ( 'NONE', #42286, #9201, #29880, .T. ) ;
#15881=VECTOR ( 'NONE', #26682, 999.9999999999998863 ) ;
#15882=ORIENTED_EDGE ( 'NONE', *, *, #49337, .T. ) ;
#15883=EDGE_CURVE ( 'NONE', #44182, #19378, #3737, .T. ) ;
#15884=ORIENTED_EDGE ( 'NONE', *, *, #34913, .T. ) ;
#15885=LINE ( 'NONE', #33226, #42958 ) ;
#15886=AXIS2_PLACEMENT_3D ( 'NONE', #4012, #30128, #43216 ) ;
#15887=ORIENTED_EDGE ( 'NONE', *, *, #2810, .F. ) ;
#15889=ORIENTED_EDGE ( 'NONE', *, *, #18388, .F. ) ;
#15890=ORIENTED_EDGE ( 'NONE', *, *, #50485, .T. ) ;
#15891=CARTESIAN_POINT ( 'NONE',  ( -22.40556560354864146, -0.1191753592594197858, 5.484709000965211523 ) ) ;
#15892=PLANE ( 'NONE',  #29662 ) ;
#15893=CARTESIAN_POINT ( 'NONE',  ( -18.16487629518032065, 0.000000000000000000, 9.849692835296727011 ) ) ;
#15894=ORIENTED_EDGE ( 'NONE', *, *, #44531, .F. ) ;
#15895=ORIENTED_EDGE ( 'NONE', *, *, #38271, .T. ) ;
#15896=VECTOR ( 'NONE', #32572, 999.9999999999998863 ) ;
#15897=FACE_OUTER_BOUND ( 'NONE', #55691, .T. ) ;
#15898=CARTESIAN_POINT ( 'NONE',  ( -15.53968616252791790, 0.000000000000000000, 5.068805764437843919 ) ) ;
#15900=ORIENTED_EDGE ( 'NONE', *, *, #39788, .T. ) ;
#15901=CARTESIAN_POINT ( 'NONE',  ( -27.06552663992790997, 0.000000000000000000, 7.195101427592543786 ) ) ;
#15903=ORIENTED_EDGE ( 'NONE', *, *, #3656, .F. ) ;
#15904=VECTOR ( 'NONE', #3900, 999.9999999999998863 ) ;
#15905=FACE_OUTER_BOUND ( 'NONE', #3141, .T. ) ;
#15906=LINE ( 'NONE', #11369, #53921 ) ;
#15907=EDGE_CURVE ( 'NONE', #16052, #51781, #51168, .T. ) ;
#15908=EDGE_LOOP ( 'NONE', ( #9450, #16249, #49694, #12428, #25978 ) ) ;
#15909=DIRECTION ( 'NONE',  ( -0.9999697198139514409, -0.000000000000000000, -0.007781995580013368816 ) ) ;
#15910=VECTOR ( 'NONE', #49909, 1000.000000000000227 ) ;
#15911=EDGE_CURVE ( 'NONE', #31521, #19558, #27282, .T. ) ;
#15912=EDGE_CURVE ( 'NONE', #1446, #21607, #43755, .T. ) ;
#15913=DIRECTION ( 'NONE',  ( 0.007781995580012662783, 0.000000000000000000, -0.9999697198139514409 ) ) ;
#15914=AXIS2_PLACEMENT_3D ( 'NONE', #20449, #19883, #54252 ) ;
#15915=AXIS2_PLACEMENT_3D ( 'NONE', #2620, #2051, #45494 ) ;
#15916=ORIENTED_EDGE ( 'NONE', *, *, #2735, .F. ) ;
#15917=CARTESIAN_POINT ( 'NONE',  ( -18.34475186460612761, 0.000000000000000000, 7.262968513376373281 ) ) ;
#15918=DIRECTION ( 'NONE',  ( 0.5364919789714477361, 0.6444004775717706579, 0.5449076811759711036 ) ) ;
#15919=CARTESIAN_POINT ( 'NONE',  ( -19.73541775872651272, 0.000000000000000000, 6.835171408663078374 ) ) ;
#15920=EDGE_LOOP ( 'NONE', ( #54177, #36834, #15027, #39073 ) ) ;
#15921=VECTOR ( 'NONE', #838, 1000.000000000000114 ) ;
#15922=AXIS2_PLACEMENT_3D ( 'NONE', #43071, #36172, #465 ) ;
#15923=LINE ( 'NONE', #49730, #23783 ) ;
#15924=FACE_OUTER_BOUND ( 'NONE', #14774, .T. ) ;
#15925=DIRECTION ( 'NONE',  ( 0.9999697198139515519, 0.000000000000000000, 0.007781995580013368816 ) ) ;
#15927=CARTESIAN_POINT ( 'NONE',  ( -9.509585063225655333, 0.000000000000000000, 6.423735671158050664 ) ) ;
#15928=PLANE ( 'NONE',  #32190 ) ;
#15929=CARTESIAN_POINT ( 'NONE',  ( -14.93495759592298988, 0.000000000000000000, 12.77129166681078409 ) ) ;
#15930=ADVANCED_FACE ( 'NONE', ( #35526 ), #44332, .F. ) ;
#15931=VECTOR ( 'NONE', #18544, 999.9999999999998863 ) ;
#15932=AXIS2_PLACEMENT_3D ( 'NONE', #27372, #14886, #964 ) ;
#15934=ORIENTED_EDGE ( 'NONE', *, *, #11911, .T. ) ;
#15935=DIRECTION ( 'NONE',  ( -0.005002170337468016433, -0.7660444431189770143, 0.6427681459581293666 ) ) ;
#15936=LINE ( 'NONE', #19343, #21422 ) ;
#15937=LINE ( 'NONE', #55969, #8764 ) ;
#15938=ORIENTED_EDGE ( 'NONE', *, *, #38408, .F. ) ;
#15939=CARTESIAN_POINT ( 'NONE',  ( -18.97909103874558312, 0.7721120973665051013, 5.520612101438020503 ) ) ;
#15940=CARTESIAN_POINT ( 'NONE',  ( 2.072287782118878319, 0.000000000000000000, -2.950529333540147015 ) ) ;
#15941=PLANE ( 'NONE',  #481 ) ;
#15942=FACE_OUTER_BOUND ( 'NONE', #38471, .T. ) ;
#15943=CARTESIAN_POINT ( 'NONE',  ( -14.56888064431065821, -0.1191753592594197858, 12.58947452739191064 ) ) ;
#15944=VECTOR ( 'NONE', #21943, 1000.000000000000227 ) ;
#15945=ORIENTED_EDGE ( 'NONE', *, *, #35156, .T. ) ;
#15946=ORIENTED_EDGE ( 'NONE', *, *, #26719, .T. ) ;
#15947=VECTOR ( 'NONE', #5683, 1000.000000000000227 ) ;
#15948=PLANE ( 'NONE',  #5062 ) ;
#15949=VECTOR ( 'NONE', #18883, 1000.000000000000227 ) ;
#15950=PLANE ( 'NONE',  #38405 ) ;
#15951=EDGE_LOOP ( 'NONE', ( #48093, #40040, #53256, #47611 ) ) ;
#15952=FACE_OUTER_BOUND ( 'NONE', #29651, .T. ) ;
#15953=EDGE_CURVE ( 'NONE', #31401, #26710, #40061, .T. ) ;
#15954=AXIS2_PLACEMENT_3D ( 'NONE', #26391, #44002, #31788 ) ;
#15956=CARTESIAN_POINT ( 'NONE',  ( -16.26477430435274130, 0.000000000000000000, 4.524504877465088448 ) ) ;
#15957=VECTOR ( 'NONE', #28927, 1000.000000000000114 ) ;
#15958=AXIS2_PLACEMENT_3D ( 'NONE', #37860, #11720, #29036 ) ;
#15959=ORIENTED_EDGE ( 'NONE', *, *, #12120, .T. ) ;
#15960=ORIENTED_EDGE ( 'NONE', *, *, #17011, .T. ) ;
#15961=ORIENTED_EDGE ( 'NONE', *, *, #21161, .F. ) ;
#15962=LINE ( 'NONE', #37245, #9362 ) ;
#15963=PLANE ( 'NONE',  #22360 ) ;
#15964=FACE_OUTER_BOUND ( 'NONE', #10963, .T. ) ;
#15966=EDGE_CURVE ( 'NONE', #47675, #16451, #5707, .T. ) ;
#15967=ORIENTED_EDGE ( 'NONE', *, *, #18408, .T. ) ;
#15968=VECTOR ( 'NONE', #14185, 1000.000000000000114 ) ;
#15969=DIRECTION ( 'NONE',  ( -0.7660212471507179544, -0.6427876096865405842, -0.005961354470445141482 ) ) ;
#15970=ORIENTED_EDGE ( 'NONE', *, *, #23243, .T. ) ;
#15971=ADVANCED_FACE ( 'NONE', ( #52564 ), #13660, .F. ) ;
#15972=EDGE_CURVE ( 'NONE', #31317, #33602, #39221, .T. ) ;
#15973=VECTOR ( 'NONE', #53464, 1000.000000000000000 ) ;
#15974=ORIENTED_EDGE ( 'NONE', *, *, #27525, .T. ) ;
#15975=VECTOR ( 'NONE', #15786, 1000.000000000000114 ) ;
#15976=EDGE_LOOP ( 'NONE', ( #14622, #46732, #7728, #23830, #1142 ) ) ;
#15977=LINE ( 'NONE', #38689, #44962 ) ;
#15978=CARTESIAN_POINT ( 'NONE',  ( -15.56267859057018121, 0.000000000000000000, 8.023283390499960532 ) ) ;
#15979=VERTEX_POINT ( 'NONE', #5436 ) ;
#15980=PLANE ( 'NONE',  #51119 ) ;
#15982=ORIENTED_EDGE ( 'NONE', *, *, #30523, .T. ) ;
#15983=FACE_OUTER_BOUND ( 'NONE', #41462, .T. ) ;
#15984=CARTESIAN_POINT ( 'NONE',  ( -11.40636015113596180, 0.000000000000000000, 11.32142374880780089 ) ) ;
#15985=ORIENTED_EDGE ( 'NONE', *, *, #42815, .F. ) ;
#15986=ADVANCED_FACE ( 'NONE', ( #14258 ), #30454, .F. ) ;
#15987=DIRECTION ( 'NONE',  ( -0.6427681459581293666, -0.7660444431189770143, -0.005002170337467561935 ) ) ;
#15989=ADVANCED_FACE ( 'NONE', ( #9126 ), #36113, .F. ) ;
#15990=VECTOR ( 'NONE', #31804, 1000.000000000000227 ) ;
#15991=CARTESIAN_POINT ( 'NONE',  ( -31.72704407542318350, -0.1191753592594197858, 9.105487798182664960 ) ) ;
#15992=LINE ( 'NONE', #54050, #8453 ) ;
#15993=CARTESIAN_POINT ( 'NONE',  ( -17.26532721389163072, 0.000000000000000000, 13.67648636611514590 ) ) ;
#15994=DIRECTION ( 'NONE',  ( -0.7660212471507179544, -0.6427876096865405842, -0.005961354470445141482 ) ) ;
#15995=CARTESIAN_POINT ( 'NONE',  ( -16.75745944145380406, 4.172053068839010059, 10.23753730508299142 ) ) ;
#15996=LINE ( 'NONE', #2631, #35543 ) ;
#15997=VECTOR ( 'NONE', #43198, 1000.000000000000227 ) ;
#15998=ORIENTED_EDGE ( 'NONE', *, *, #28197, .T. ) ;
#15999=ADVANCED_FACE ( 'NONE', ( #8878 ), #316, .F. ) ;
#16000=ORIENTED_EDGE ( 'NONE', *, *, #11359, .T. ) ;
#16001=DIRECTION ( 'NONE',  ( 0.5364919789714477361, 0.6444004775717706579, 0.5449076811759711036 ) ) ;
#16002=VECTOR ( 'NONE', #4631, 999.9999999999998863 ) ;
#16003=CARTESIAN_POINT ( 'NONE',  ( -21.47341775636118655, -0.1191753592594197858, 5.122631121243466090 ) ) ;
#16006=DIRECTION ( 'NONE',  ( -0.005961354470445682716, -0.6427876096865404731, 0.7660212471507180654 ) ) ;
#16007=EDGE_CURVE ( 'NONE', #39014, #30987, #5176, .T. ) ;
#16008=VECTOR ( 'NONE', #3909, 999.9999999999998863 ) ;
#16009=CARTESIAN_POINT ( 'NONE',  ( -32.65841372305263235, 0.000000000000000000, 9.367568705923016381 ) ) ;
#16010=VERTEX_POINT ( 'NONE', #26438 ) ;
#16011=FACE_OUTER_BOUND ( 'NONE', #8413, .T. ) ;
#16012=DIRECTION ( 'NONE',  ( 0.000000000000000000, 0.000000000000000000, 1.000000000000000000 ) ) ;
#16013=ORIENTED_EDGE ( 'NONE', *, *, #36568, .F. ) ;
#16014=LINE ( 'NONE', #19414, #28398 ) ;
#16015=CARTESIAN_POINT ( 'NONE',  ( -18.68717756098156713, -0.1191753592594176070, 4.405650147085642843 ) ) ;
#16019=DIRECTION ( 'NONE',  ( -0.6427681459581293666, -0.7660444431189770143, -0.005002170337467561935 ) ) ;
#16020=VECTOR ( 'NONE', #43842, 1000.000000000000114 ) ;
#16021=CARTESIAN_POINT ( 'NONE',  ( -11.20636620717317378, 0.000000000000000000, 11.32298014792380414 ) ) ;
#16022=CARTESIAN_POINT ( 'NONE',  ( -14.00280974873554030, 0.000000000000000000, 12.40921378708904044 ) ) ;
#16023=AXIS2_PLACEMENT_3D ( 'NONE', #28313, #6749, #24072 ) ;
#16024=CARTESIAN_POINT ( 'NONE',  ( -19.12962290826653700, 0.000000000000000000, 14.40064212555863854 ) ) ;
#16025=EDGE_LOOP ( 'NONE', ( #49086, #3467, #30591, #10701 ) ) ;
#16026=AXIS2_PLACEMENT_3D ( 'NONE', #50652, #50908, #37884 ) ;
#16028=FACE_OUTER_BOUND ( 'NONE', #14641, .T. ) ;
#16030=CARTESIAN_POINT ( 'NONE',  ( -16.81267852042391198, -0.1191753592594197858, 3.312241722634738039 ) ) ;
#16032=LINE ( 'NONE', #28814, #11937 ) ;
#16033=CARTESIAN_POINT ( 'NONE',  ( -22.40478740399063895, 0.000000000000000000, 5.384712028983816623 ) ) ;
#16034=EDGE_CURVE ( 'NONE', #52765, #42667, #22195, .T. ) ;
#16035=EDGE_LOOP ( 'NONE', ( #2522, #55916, #1601, #16719 ) ) ;
#16036=FACE_OUTER_BOUND ( 'NONE', #12665, .T. ) ;
#16037=VECTOR ( 'NONE', #40662, 1000.000000000000000 ) ;
#16038=LINE ( 'NONE', #19988, #2405 ) ;
#16039=FACE_OUTER_BOUND ( 'NONE', #18147, .T. ) ;
#16041=DIRECTION ( 'NONE',  ( 0.000000000000000000, -1.000000000000000000, 0.000000000000000000 ) ) ;
#16042=PLANE ( 'NONE',  #3246 ) ;
#16043=CARTESIAN_POINT ( 'NONE',  ( -13.71629766702752562, -5.213152330870663320, 10.56547866312180339 ) ) ;
#16044=EDGE_LOOP ( 'NONE', ( #42074, #14927, #20416, #40092 ) ) ;
#16045=CARTESIAN_POINT ( 'NONE',  ( -17.93139508144814442, 0.000000000000000000, 13.85596890686001537 ) ) ;
#16046=VECTOR ( 'NONE', #46122, 1000.000000000000227 ) ;
#16047=ORIENTED_EDGE ( 'NONE', *, *, #39003, .T. ) ;
#16048=ADVANCED_FACE ( 'NONE', ( #35269 ), #48292, .F. ) ;
#16049=ORIENTED_EDGE ( 'NONE', *, *, #42701, .F. ) ;
#16050=AXIS2_PLACEMENT_3D ( 'NONE', #44558, #22458, #46957 ) ;
#16051=ORIENTED_EDGE ( 'NONE', *, *, #42193, .F. ) ;
#16052=VERTEX_POINT ( 'NONE', #18195 ) ;
#16053=PLANE ( 'NONE',  #2103 ) ;
#16054=ORIENTED_EDGE ( 'NONE', *, *, #23216, .F. ) ;
#16056=ORIENTED_EDGE ( 'NONE', *, *, #52128, .F. ) ;
#16057=DIRECTION ( 'NONE',  ( 0.005002170337468016433, -0.7660444431189770143, -0.6427681459581293666 ) ) ;
#16058=EDGE_CURVE ( 'NONE', #9638, #11120, #27025, .T. ) ;
#16059=ORIENTED_EDGE ( 'NONE', *, *, #34070, .T. ) ;
#16060=ORIENTED_EDGE ( 'NONE', *, *, #3462, .T. ) ;
#16061=ADVANCED_FACE ( 'NONE', ( #9715 ), #41479, .F. ) ;
#16062=AXIS2_PLACEMENT_3D ( 'NONE', #14488, #14228, #9681 ) ;
#16063=LINE ( 'NONE', #42167, #10373 ) ;
#16064=DIRECTION ( 'NONE',  ( -0.6246952433987894571, 0.7422098413412802076, 0.2426528472758539834 ) ) ;
#16065=FACE_OUTER_BOUND ( 'NONE', #16550, .T. ) ;
#16066=FACE_OUTER_BOUND ( 'NONE', #47999, .T. ) ;
#16067=ORIENTED_EDGE ( 'NONE', *, *, #16736, .T. ) ;
#16068=EDGE_CURVE ( 'NONE', #43321, #48873, #19315, .T. ) ;
#16069=VERTEX_POINT ( 'NONE', #15602 ) ;
#16070=CARTESIAN_POINT ( 'NONE',  ( -8.207176806059445440, 0.000000000000000000, 5.864533187340529530 ) ) ;
#16071=CARTESIAN_POINT ( 'NONE',  ( -13.68844308129014564, 0.000000000000000000, 6.021882761988201160 ) ) ;
#16072=DIRECTION ( 'NONE',  ( 0.007781995580012663651, 0.000000000000000000, -0.9999697198139515519 ) ) ;
#16073=EDGE_CURVE ( 'NONE', #10456, #17295, #19043, .T. ) ;
#16074=CARTESIAN_POINT ( 'NONE',  ( 2.072287782118878319, 0.000000000000000000, -2.950529333540147015 ) ) ;
#16075=CARTESIAN_POINT ( 'NONE',  ( -13.27065584551087163, 0.000000000000000000, 12.04557950825129176 ) ) ;
#16076=DIRECTION ( 'NONE',  ( 0.9999697198139515519, 0.000000000000000000, 0.007781995580013368816 ) ) ;
#16077=VERTEX_POINT ( 'NONE', #32118 ) ;
#16078=DIRECTION ( 'NONE',  ( -0.6427681459581293666, -0.7660444431189770143, -0.005002170337467561935 ) ) ;
#16079=EDGE_LOOP ( 'NONE', ( #13688, #2422, #43692, #5542 ) ) ;
#16080=FACE_OUTER_BOUND ( 'NONE', #33039, .T. ) ;
#16081=DIRECTION ( 'NONE',  ( 0.007781995580012663651, 0.000000000000000000, -0.9999697198139515519 ) ) ;
#16082=DIRECTION ( 'NONE',  ( 0.5449076811759707706, 0.6444004775717708799, -0.5364919789714476250 ) ) ;
#16083=DIRECTION ( 'NONE',  ( 0.000000000000000000, -0.000000000000000000, -1.000000000000000000 ) ) ;
#16084=DIRECTION ( 'NONE',  ( 0.007781995580012662783, 0.000000000000000000, -0.9999697198139514409 ) ) ;
#16085=LINE ( 'NONE', #54680, #15975 ) ;
#16086=VECTOR ( 'NONE', #42490, 1000.000000000000227 ) ;
#16087=ORIENTED_EDGE ( 'NONE', *, *, #25360, .T. ) ;
#16088=ORIENTED_EDGE ( 'NONE', *, *, #1356, .T. ) ;
#16090=DIRECTION ( 'NONE',  ( 0.5449076811759707706, 0.6444004775717708799, -0.5364919789714476250 ) ) ;
#16091=DIRECTION ( 'NONE',  ( 0.9999697198139515519, 0.000000000000000000, 0.007781995580013368816 ) ) ;
#16092=EDGE_CURVE ( 'NONE', #14416, #16426, #46017, .T. ) ;
#16093=VECTOR ( 'NONE', #34247, 1000.000000000000114 ) ;
#16094=LINE ( 'NONE', #32834, #12844 ) ;
#16095=DIRECTION ( 'NONE',  ( 0.007781995580012663651, 0.000000000000000000, -0.9999697198139515519 ) ) ;
#16096=ADVANCED_FACE ( 'NONE', ( #24415 ), #36658, .F. ) ;
#16097=LINE ( 'NONE', #46177, #29091 ) ;
#16098=DIRECTION ( 'NONE',  ( -0.6246952433987894571, 0.7422098413412802076, 0.2426528472758539834 ) ) ;
#16099=DIRECTION ( 'NONE',  ( 0.005002170337468016433, -0.7660444431189770143, -0.6427681459581293666 ) ) ;
#16100=ADVANCED_FACE ( 'NONE', ( #53968 ), #2816, .F. ) ;
#16101=DIRECTION ( 'NONE',  ( 0.5449076811759707706, 0.6444004775717708799, -0.5364919789714476250 ) ) ;
#16102=ORIENTED_EDGE ( 'NONE', *, *, #3841, .F. ) ;
#16103=EDGE_CURVE ( 'NONE', #3799, #39923, #2559, .T. ) ;
#16104=ADVANCED_FACE ( 'NONE', ( #19617 ), #10557, .F. ) ;
#16105=EDGE_CURVE ( 'NONE', #8484, #12293, #28122, .T. ) ;
#16106=ORIENTED_EDGE ( 'NONE', *, *, #1876, .F. ) ;
#16107=EDGE_LOOP ( 'NONE', ( #37545, #55397, #28056, #50976 ) ) ;
#16108=ORIENTED_EDGE ( 'NONE', *, *, #19215, .F. ) ;
#16109=ORIENTED_EDGE ( 'NONE', *, *, #23738, .T. ) ;
#16110=ORIENTED_EDGE ( 'NONE', *, *, #24347, .F. ) ;
#16111=LINE ( 'NONE', #33431, #6952 ) ;
#16112=PLANE ( 'NONE',  #18407 ) ;
#16113=FACE_OUTER_BOUND ( 'NONE', #2997, .T. ) ;
#16115=DIRECTION ( 'NONE',  ( 0.005002170337468016433, -0.7660444431189770143, -0.6427681459581293666 ) ) ;
#16116=EDGE_CURVE ( 'NONE', #48743, #33120, #40901, .T. ) ;
#16117=ORIENTED_EDGE ( 'NONE', *, *, #22696, .T. ) ;
#16119=ORIENTED_EDGE ( 'NONE', *, *, #12662, .F. ) ;
#16121=AXIS2_PLACEMENT_3D ( 'NONE', #17561, #52209, #13324 ) ;
#16123=EDGE_CURVE ( 'NONE', #51745, #18836, #20142, .T. ) ;
#16124=FACE_OUTER_BOUND ( 'NONE', #41594, .T. ) ;
#16125=DIRECTION ( 'NONE',  ( -0.6427681459581293666, -0.7660444431189770143, -0.005002170337467561935 ) ) ;
#16126=ORIENTED_EDGE ( 'NONE', *, *, #5419, .F. ) ;
#16127=CARTESIAN_POINT ( 'NONE',  ( -9.110551994824897193, 0.000000000000000000, 3.538847790438064411 ) ) ;
#16128=VERTEX_POINT ( 'NONE', #23331 ) ;
#16129=ADVANCED_FACE ( 'NONE', ( #36365 ), #40646, .F. ) ;
#16130=VECTOR ( 'NONE', #21384, 1000.000000000000114 ) ;
#16131=DIRECTION ( 'NONE',  ( -0.9999697198139514409, -0.000000000000000000, -0.007781995580013368816 ) ) ;
#16132=DIRECTION ( 'NONE',  ( -0.5364919789714478471, 0.6444004775717705469, -0.5449076811759709926 ) ) ;
#16133=DIRECTION ( 'NONE',  ( 0.5364919789714477361, 0.6444004775717706579, 0.5449076811759711036 ) ) ;
#16134=DIRECTION ( 'NONE',  ( 0.005002170337468016433, -0.7660444431189770143, -0.6427681459581293666 ) ) ;
#16135=LINE ( 'NONE', #33451, #31242 ) ;
#16136=DIRECTION ( 'NONE',  ( 0.007781995580012662783, 0.000000000000000000, -0.9999697198139514409 ) ) ;
#16137=DIRECTION ( 'NONE',  ( 0.9999697198139515519, 0.000000000000000000, 0.007781995580013368816 ) ) ;
#16138=CARTESIAN_POINT ( 'NONE',  ( 2.072287782118878319, 0.000000000000000000, -2.950529333540147015 ) ) ;
#16139=ORIENTED_EDGE ( 'NONE', *, *, #25618, .T. ) ;
#16140=DIRECTION ( 'NONE',  ( -0.005002170337468016433, -0.7660444431189770143, 0.6427681459581293666 ) ) ;
#16141=EDGE_LOOP ( 'NONE', ( #11521, #5922, #54281, #2908, #49070 ) ) ;
#16142=PLANE ( 'NONE',  #6608 ) ;
#16143=DIRECTION ( 'NONE',  ( -0.005002170337468016433, -0.7660444431189770143, 0.6427681459581293666 ) ) ;
#16144=PLANE ( 'NONE',  #53143 ) ;
#16145=DIRECTION ( 'NONE',  ( -0.005002170337468016433, -0.7660444431189770143, 0.6427681459581293666 ) ) ;
#16146=CARTESIAN_POINT ( 'NONE',  ( -18.29747203306047609, -0.1191753592594177458, 14.03778604627889059 ) ) ;
#16147=CARTESIAN_POINT ( 'NONE',  ( -16.89925026227929195, -0.1191753592594197858, 13.49466922669627422 ) ) ;
#16148=ORIENTED_EDGE ( 'NONE', *, *, #18745, .T. ) ;
#16149=CARTESIAN_POINT ( 'NONE',  ( -14.66887761629205222, 0.000000000000000000, 12.58869632783390990 ) ) ;
#16151=FACE_OUTER_BOUND ( 'NONE', #38000, .T. ) ;
#16152=DIRECTION ( 'NONE',  ( 0.007781995580012662783, 0.000000000000000000, -0.9999697198139514409 ) ) ;
#16153=LINE ( 'NONE', #49930, #36862 ) ;
#16154=DIRECTION ( 'NONE',  ( 0.000000000000000000, -0.000000000000000000, -1.000000000000000000 ) ) ;
#16155=DIRECTION ( 'NONE',  ( 0.9999697198139515519, 0.000000000000000000, 0.007781995580013368816 ) ) ;
#16156=CARTESIAN_POINT ( 'NONE',  ( -21.47419595591918906, 0.000000000000000000, 5.222628093224860102 ) ) ;
#16157=PLANE ( 'NONE',  #17458 ) ;
#16158=ORIENTED_EDGE ( 'NONE', *, *, #35191, .F. ) ;
#16159=DIRECTION ( 'NONE',  ( 0.9999697198139515519, 0.000000000000000000, 0.007781995580013368816 ) ) ;
#16161=ORIENTED_EDGE ( 'NONE', *, *, #38681, .F. ) ;
#16162=ORIENTED_EDGE ( 'NONE', *, *, #5655, .F. ) ;
#16163=CARTESIAN_POINT ( 'NONE',  ( -24.27063949748155380, 0.000000000000000000, 6.308861732390097288 ) ) ;
#16164=EDGE_CURVE ( 'NONE', #39726, #20170, #6836, .T. ) ;
#16165=EDGE_CURVE ( 'NONE', #32592, #28407, #24160, .T. ) ;
#16166=VECTOR ( 'NONE', #25860, 1000.000000000000000 ) ;
#16167=ORIENTED_EDGE ( 'NONE', *, *, #173, .F. ) ;
#16168=ORIENTED_EDGE ( 'NONE', *, *, #41803, .F. ) ;
#16169=DIRECTION ( 'NONE',  ( 0.6427681459581294776, -0.7660444431189769032, 0.005002170337467562802 ) ) ;
#16170=ADVANCED_FACE ( 'NONE', ( #44895 ), #1717, .F. ) ;
#16171=EDGE_LOOP ( 'NONE', ( #50562, #27604, #20436, #9850 ) ) ;
#16172=ORIENTED_EDGE ( 'NONE', *, *, #45511, .T. ) ;
#16173=ORIENTED_EDGE ( 'NONE', *, *, #26618, .F. ) ;
#16174=PLANE ( 'NONE',  #31132 ) ;
#16175=DIRECTION ( 'NONE',  ( 0.6427681459581294776, -0.7660444431189769032, 0.005002170337467562802 ) ) ;
#16176=CARTESIAN_POINT ( 'NONE',  ( -10.84028925556084388, -0.1191753592594197858, 11.14116300850493246 ) ) ;
#16177=ORIENTED_EDGE ( 'NONE', *, *, #28616, .T. ) ;
#16178=ORIENTED_EDGE ( 'NONE', *, *, #52405, .T. ) ;
#16179=ADVANCED_FACE ( 'NONE', ( #55355 ), #46263, .F. ) ;
#16180=CARTESIAN_POINT ( 'NONE',  ( -20.54204810873173415, 0.000000000000000000, 4.860550213503115558 ) ) ;
#16181=CARTESIAN_POINT ( 'NONE',  ( -20.54049170961573267, 0.000000000000000000, 4.660556269540326646 ) ) ;
#16182=ORIENTED_EDGE ( 'NONE', *, *, #34736, .F. ) ;
#16183=EDGE_CURVE ( 'NONE', #44937, #29422, #37784, .T. ) ;
#16184=DIRECTION ( 'NONE',  ( 0.005961354470445682716, -0.6427876096865404731, -0.7660212471507180654 ) ) ;
#16185=ORIENTED_EDGE ( 'NONE', *, *, #27727, .F. ) ;
#16186=DIRECTION ( 'NONE',  ( 0.000000000000000000, -0.000000000000000000, -1.000000000000000000 ) ) ;
#16187=DIRECTION ( 'NONE',  ( -0.9321478471874540261, 0.000000000000000000, 0.3620778797217457656 ) ) ;
#16188=ORIENTED_EDGE ( 'NONE', *, *, #25767, .F. ) ;
#16189=EDGE_CURVE ( 'NONE', #16632, #23911, #46549, .T. ) ;
#16190=CARTESIAN_POINT ( 'NONE',  ( -24.26908309836554878, 0.000000000000000000, 6.108867788427308376 ) ) ;
#16191=ADVANCED_FACE ( 'NONE', ( #3674 ), #54795, .F. ) ;
#16192=DIRECTION ( 'NONE',  ( 0.9999697198139515519, 0.000000000000000000, 0.007781995580013368816 ) ) ;
#16193=EDGE_LOOP ( 'NONE', ( #43696, #36961, #26419, #47109 ) ) ;
#16194=DIRECTION ( 'NONE',  ( -0.5449076811759708816, 0.6444004775717707689, 0.5364919789714475140 ) ) ;
#16195=CARTESIAN_POINT ( 'NONE',  ( -0.9975486161969306931, 4.078988103069860038, 3.605855335088290925 ) ) ;
#16196=CARTESIAN_POINT ( 'NONE',  ( -23.33771345073609638, -0.1191753592594197858, 5.846786880686956955 ) ) ;
#16197=ADVANCED_FACE ( 'NONE', ( #42012 ), #16448, .F. ) ;
#16198=EDGE_LOOP ( 'NONE', ( #27332, #49885, #55378, #8777 ) ) ;
#16199=VECTOR ( 'NONE', #39262, 1000.000000000000227 ) ;
#16200=CARTESIAN_POINT ( 'NONE',  ( -15.80145506190093130, 0.000000000000000000, 4.697436548528074240 ) ) ;
#16201=LINE ( 'NONE', #29251, #44123 ) ;
#16202=EDGE_CURVE ( 'NONE', #17993, #24549, #3112, .T. ) ;
#16204=PLANE ( 'NONE',  #8725 ) ;
#16205=LINE ( 'NONE', #24708, #41261 ) ;
#16206=LINE ( 'NONE', #3133, #3477 ) ;
#16208=ORIENTED_EDGE ( 'NONE', *, *, #28803, .T. ) ;
#16209=LINE ( 'NONE', #38068, #3554 ) ;
#16210=CARTESIAN_POINT ( 'NONE',  ( -19.75809492754008900, 2.229229656569007290, 8.214581822483392415 ) ) ;
#16211=LINE ( 'NONE', #46885, #40499 ) ;
#16212=EDGE_LOOP ( 'NONE', ( #43106, #52290, #22978, #14088 ) ) ;
#16213=DIRECTION ( 'NONE',  ( 0.007781995580012662783, 0.000000000000000000, -0.9999697198139514409 ) ) ;
#16214=CARTESIAN_POINT ( 'NONE',  ( -12.15271748404464880, 0.000000000000000000, 1.601849296007406664 ) ) ;
#16215=CARTESIAN_POINT ( 'NONE',  ( -14.06264638353402141, 5.467268677019013978, 1.969906661245985457 ) ) ;
#16216=PLANE ( 'NONE',  #55059 ) ;
#16218=ORIENTED_EDGE ( 'NONE', *, *, #6200, .T. ) ;
#16219=ORIENTED_EDGE ( 'NONE', *, *, #12901, .F. ) ;
#16220=LINE ( 'NONE', #33819, #8714 ) ;
#16222=EDGE_CURVE ( 'NONE', #15181, #17295, #33775, .T. ) ;
#16223=ORIENTED_EDGE ( 'NONE', *, *, #11433, .F. ) ;
#16224=LINE ( 'NONE', #25314, #55778 ) ;
#16225=ORIENTED_EDGE ( 'NONE', *, *, #24040, .F. ) ;
#16226=LINE ( 'NONE', #2864, #44695 ) ;
#16227=ADVANCED_FACE ( 'NONE', ( #15905 ), #30856, .F. ) ;
#16228=ADVANCED_FACE ( 'NONE', ( #35150 ), #46858, .F. ) ;
#16229=ORIENTED_EDGE ( 'NONE', *, *, #54546, .T. ) ;
#16230=ORIENTED_EDGE ( 'NONE', *, *, #13229, .T. ) ;
#16231=ORIENTED_EDGE ( 'NONE', *, *, #31592, .T. ) ;
#16232=DIRECTION ( 'NONE',  ( -0.005002170337468016433, -0.7660444431189770143, 0.6427681459581293666 ) ) ;
#16233=FACE_OUTER_BOUND ( 'NONE', #33818, .T. ) ;
#16234=CARTESIAN_POINT ( 'NONE',  ( -10.40149616133915345, 0.000000000000000000, 1.615477705271093800 ) ) ;
#16236=CARTESIAN_POINT ( 'NONE',  ( -14.46888367232926420, 0.000000000000000000, 12.59025272694991315 ) ) ;
#16237=ORIENTED_EDGE ( 'NONE', *, *, #26059, .T. ) ;
#16238=EDGE_LOOP ( 'NONE', ( #45089, #55752, #15903, #23568 ) ) ;
#16239=ORIENTED_EDGE ( 'NONE', *, *, #5337, .T. ) ;
#16240=CARTESIAN_POINT ( 'NONE',  ( -10.00813838035478298, 0.000000000000000000, 10.77830692922518452 ) ) ;
#16241=LINE ( 'NONE', #20785, #43964 ) ;
#16242=ORIENTED_EDGE ( 'NONE', *, *, #6459, .F. ) ;
#16243=DIRECTION ( 'NONE',  ( 0.005002170337468016433, -0.7660444431189770143, -0.6427681459581293666 ) ) ;
#16244=ORIENTED_EDGE ( 'NONE', *, *, #23325, .T. ) ;
#16246=CARTESIAN_POINT ( 'NONE',  ( -18.76354595665420177, -0.1191753592594177458, 14.21882498613976331 ) ) ;
#16247=ORIENTED_EDGE ( 'NONE', *, *, #26889, .F. ) ;
#16248=DIRECTION ( 'NONE',  ( -0.5364919789714478471, 0.6444004775717705469, -0.5449076811759709926 ) ) ;
#16249=ORIENTED_EDGE ( 'NONE', *, *, #38708, .F. ) ;
#16250=ADVANCED_FACE ( 'NONE', ( #20445 ), #7371, .F. ) ;
#16251=CARTESIAN_POINT ( 'NONE',  ( -8.844954222421781864, 0.000000000000000000, 6.428907982042063374 ) ) ;
#16252=CARTESIAN_POINT ( 'NONE',  ( -8.932676780824044371, -0.1191753592594177180, 4.850893997471606767 ) ) ;
#16253=EDGE_CURVE ( 'NONE', #47896, #55726, #30606, .T. ) ;
#16255=DIRECTION ( 'NONE',  ( 0.005002170337468016433, -0.7660444431189770143, -0.6427681459581293666 ) ) ;
#16256=FACE_OUTER_BOUND ( 'NONE', #7071, .T. ) ;
#16257=LINE ( 'NONE', #38399, #6522 ) ;
#16259=ORIENTED_EDGE ( 'NONE', *, *, #48083, .F. ) ;
#16260=ORIENTED_EDGE ( 'NONE', *, *, #4556, .F. ) ;
#16262=EDGE_CURVE ( 'NONE', #15067, #14438, #42317, .T. ) ;
#16263=LINE ( 'NONE', #50048, #50232 ) ;
#16265=CARTESIAN_POINT ( 'NONE',  ( -21.53432988685325356, 2.714935509636508204, 4.959976111460639103 ) ) ;
#16266=CARTESIAN_POINT ( 'NONE',  ( -12.60458797795435615, 0.000000000000000000, 11.86609696750642229 ) ) ;
#16267=DIRECTION ( 'NONE',  ( -0.7660212471507179544, -0.6427876096865405842, -0.005961354470445141482 ) ) ;
#16268=VERTEX_POINT ( 'NONE', #52445 ) ;
#16269=CARTESIAN_POINT ( 'NONE',  ( -10.00813838035478298, 0.000000000000000000, 10.77830692922518452 ) ) ;
#16270=FACE_OUTER_BOUND ( 'NONE', #20219, .T. ) ;
#16271=ORIENTED_EDGE ( 'NONE', *, *, #27733, .T. ) ;
#16272=FACE_OUTER_BOUND ( 'NONE', #43754, .T. ) ;
#16273=ORIENTED_EDGE ( 'NONE', *, *, #10965, .T. ) ;
#16274=LINE ( 'NONE', #34443, #47051 ) ;
#16276=CARTESIAN_POINT ( 'NONE',  ( -18.62819553763212710, 0.000000000000000000, 9.676761164233743884 ) ) ;
#16277=ADVANCED_FACE ( 'NONE', ( #4734 ), #25276, .F. ) ;
#16278=DIRECTION ( 'NONE',  ( 0.007781995580012663651, 0.000000000000000000, -0.9999697198139515519 ) ) ;
#16280=ORIENTED_EDGE ( 'NONE', *, *, #31297, .F. ) ;
#16281=ORIENTED_EDGE ( 'NONE', *, *, #3465, .F. ) ;
#16282=LINE ( 'NONE', #33603, #14929 ) ;
#16284=DIRECTION ( 'NONE',  ( -0.9999697198139514409, -0.000000000000000000, -0.007781995580013368816 ) ) ;
#16285=EDGE_CURVE ( 'NONE', #43426, #41524, #28968, .T. ) ;
#16286=FACE_OUTER_BOUND ( 'NONE', #15740, .T. ) ;
#16287=DIRECTION ( 'NONE',  ( -0.5364919789714478471, 0.6444004775717705469, -0.5449076811759709926 ) ) ;
#16288=ADVANCED_FACE ( 'NONE', ( #34847 ), #13279, .F. ) ;
#16289=CARTESIAN_POINT ( 'NONE',  ( -8.460163181381084030, -0.1064616600236961419, 5.213234893987049645 ) ) ;
#16290=EDGE_LOOP ( 'NONE', ( #47185, #54712, #1755, #36233 ) ) ;
#16291=DIRECTION ( 'NONE',  ( 0.000000000000000000, -1.000000000000000000, 0.000000000000000000 ) ) ;
#16292=EDGE_CURVE ( 'NONE', #10480, #40212, #43911, .T. ) ;
#16293=CARTESIAN_POINT ( 'NONE',  ( -11.59440027503052129, 3.038739411681507185, 6.372068998963611897 ) ) ;
#16294=CARTESIAN_POINT ( 'NONE',  ( 2.072287782118878319, 0.000000000000000000, -2.950529333540147015 ) ) ;
#16295=VERTEX_POINT ( 'NONE', #45316 ) ;
#16296=CARTESIAN_POINT ( 'NONE',  ( 2.072287782118878319, 0.000000000000000000, -2.950529333540147015 ) ) ;
#16297=CARTESIAN_POINT ( 'NONE',  ( -17.74482636761137044, -0.1191753592594197858, 3.674319602356483916 ) ) ;
#16299=EDGE_CURVE ( 'NONE', #19103, #31662, #10116, .T. ) ;
#16300=EDGE_LOOP ( 'NONE', ( #49502, #38230, #16419, #1595 ) ) ;
#16301=EDGE_CURVE ( 'NONE', #41698, #31162, #40526, .T. ) ;
#16302=CARTESIAN_POINT ( 'NONE',  ( -22.40478740399063895, 0.000000000000000000, 5.384712028983816623 ) ) ;
#16303=ORIENTED_EDGE ( 'NONE', *, *, #45150, .T. ) ;
#16304=EDGE_CURVE ( 'NONE', #40075, #51697, #27428, .T. ) ;
#16305=VERTEX_POINT ( 'NONE', #1607 ) ;
#16306=ORIENTED_EDGE ( 'NONE', *, *, #31634, .T. ) ;
#16307=EDGE_LOOP ( 'NONE', ( #17911, #39298, #18042, #4271 ) ) ;
#16308=LINE ( 'NONE', #11215, #22956 ) ;
#16309=ORIENTED_EDGE ( 'NONE', *, *, #38562, .F. ) ;
#16310=DIRECTION ( 'NONE',  ( -0.005961354470445682716, -0.6427876096865404731, 0.7660212471507180654 ) ) ;
#16311=ORIENTED_EDGE ( 'NONE', *, *, #52884, .F. ) ;
#16312=FACE_OUTER_BOUND ( 'NONE', #26538, .T. ) ;
#16313=ORIENTED_EDGE ( 'NONE', *, *, #2556, .T. ) ;
#16314=VERTEX_POINT ( 'NONE', #14117 ) ;
#16315=CARTESIAN_POINT ( 'NONE',  ( -15.33837456417585088, 0.000000000000000000, 4.901046404258871725 ) ) ;
#16316=CARTESIAN_POINT ( 'NONE',  ( -9.408809891686260585, -0.1191753592594168437, 6.324516898734651171 ) ) ;
#16317=LINE ( 'NONE', #11229, #9530 ) ;
#16318=PLANE ( 'NONE',  #18739 ) ;
#16319=LINE ( 'NONE', #50953, #26516 ) ;
#16320=ORIENTED_EDGE ( 'NONE', *, *, #29886, .T. ) ;
#16321=ORIENTED_EDGE ( 'NONE', *, *, #41190, .T. ) ;
#16322=CARTESIAN_POINT ( 'NONE',  ( -9.195139935026407585, 2.581774180789586648, 3.321081197191737555 ) ) ;
#16324=DIRECTION ( 'NONE',  ( -0.9999697198139514409, -0.000000000000000000, -0.007781995580013368816 ) ) ;
#16325=LINE ( 'NONE', #55807, #46904 ) ;
#16326=PLANE ( 'NONE',  #42142 ) ;
#16327=CARTESIAN_POINT ( 'NONE',  ( -27.06552663992790997, 0.000000000000000000, 7.195101427592543786 ) ) ;
#16328=CARTESIAN_POINT ( 'NONE',  ( -29.86352658060627618, 0.000000000000000000, 8.481329010720569883 ) ) ;
#16330=CARTESIAN_POINT ( 'NONE',  ( -15.32687835015472011, 0.000000000000000000, 3.423807591227812530 ) ) ;
#16331=DIRECTION ( 'NONE',  ( -0.9999697198139514409, -0.000000000000000000, -0.007781995580013368816 ) ) ;
#16332=ORIENTED_EDGE ( 'NONE', *, *, #42982, .T. ) ;
#16333=ADVANCED_FACE ( 'NONE', ( #22364 ), #49016, .F. ) ;
#16334=CARTESIAN_POINT ( 'NONE',  ( -12.80458192191714595, 0.000000000000000000, 11.86454056839041726 ) ) ;
#16335=LINE ( 'NONE', #46163, #35079 ) ;
#16336=DIRECTION ( 'NONE',  ( 0.000000000000000000, -1.000000000000000000, 0.000000000000000000 ) ) ;
#16337=DIRECTION ( 'NONE',  ( 0.9999697198139515519, 0.000000000000000000, 0.007781995580013368816 ) ) ;
#16338=ADVANCED_FACE ( 'NONE', ( #18078 ), #49297, .T. ) ;
#16339=EDGE_CURVE ( 'NONE', #43960, #12251, #1856, .T. ) ;
#16340=DIRECTION ( 'NONE',  ( -0.5364919789714478471, 0.6444004775717705469, -0.5449076811759709926 ) ) ;
#16341=VECTOR ( 'NONE', #10099, 999.9999999999998863 ) ;
#16342=ORIENTED_EDGE ( 'NONE', *, *, #53909, .T. ) ;
#16343=VERTEX_POINT ( 'NONE', #10411 ) ;
#16344=CARTESIAN_POINT ( 'NONE',  ( -30.79411802867772607, 0.000000000000000000, 8.643412946479525516 ) ) ;
#16345=DIRECTION ( 'NONE',  ( -0.005002170337468016433, -0.7660444431189770143, 0.6427681459581293666 ) ) ;
#16346=DIRECTION ( 'NONE',  ( 0.005961354470445682716, -0.6427876096865404731, -0.7660212471507180654 ) ) ;
#16347=FACE_OUTER_BOUND ( 'NONE', #36949, .T. ) ;
#16348=ADVANCED_FACE ( 'NONE', ( #39933 ), #48457, .F. ) ;
#16349=FACE_OUTER_BOUND ( 'NONE', #3190, .T. ) ;
#16350=CARTESIAN_POINT ( 'NONE',  ( -21.98208829179906232, -3.432230869623159819, 10.85339692575916537 ) ) ;
#16351=DIRECTION ( 'NONE',  ( 0.9999697198139515519, 0.000000000000000000, 0.007781995580013368816 ) ) ;
#16352=ADVANCED_FACE ( 'NONE', ( #26899 ), #23470, .F. ) ;
#16353=CARTESIAN_POINT ( 'NONE',  ( -11.30636317915456779, -0.1191753592594197858, 11.32220194836580340 ) ) ;
#16354=DIRECTION ( 'NONE',  ( -0.005961354470445682716, -0.6427876096865404731, 0.7660212471507180654 ) ) ;
#16355=CARTESIAN_POINT ( 'NONE',  ( -13.73672976910459909, 0.000000000000000000, 12.22661844811216270 ) ) ;
#16357=CARTESIAN_POINT ( 'NONE',  ( -20.23219776430595829, -4.727446477803164626, 4.589363523624652608 ) ) ;
#16358=ADVANCED_FACE ( 'NONE', ( #9858 ), #40221, .F. ) ;
#16359=ORIENTED_EDGE ( 'NONE', *, *, #11210, .T. ) ;
#16360=ORIENTED_EDGE ( 'NONE', *, *, #4325, .F. ) ;
#16362=ORIENTED_EDGE ( 'NONE', *, *, #16464, .F. ) ;
#16363=ORIENTED_EDGE ( 'NONE', *, *, #54763, .F. ) ;
#16364=ORIENTED_EDGE ( 'NONE', *, *, #7197, .F. ) ;
#16365=ORIENTED_EDGE ( 'NONE', *, *, #2551, .T. ) ;
#16366=CARTESIAN_POINT ( 'NONE',  ( -31.72704407542318350, -0.1191753592594197858, 9.105487798182664960 ) ) ;
#16367=CARTESIAN_POINT ( 'NONE',  ( -28.93137873341882127, 0.000000000000000000, 8.119251130998824451 ) ) ;
#16368=CARTESIAN_POINT ( 'NONE',  ( -23.33693525117809386, 0.000000000000000000, 5.746789908705562944 ) ) ;
#16369=AXIS2_PLACEMENT_3D ( 'NONE', #25000, #33513, #37483 ) ;
#16370=VERTEX_POINT ( 'NONE', #32277 ) ;
#16371=PLANE ( 'NONE',  #45811 ) ;
#16372=ORIENTED_EDGE ( 'NONE', *, *, #17932, .F. ) ;
#16373=PLANE ( 'NONE',  #1404 ) ;
#16374=VERTEX_POINT ( 'NONE', #49598 ) ;
#16377=CARTESIAN_POINT ( 'NONE',  ( -19.60990026154428278, 0.000000000000000000, 4.498472333781370125 ) ) ;
#16379=ORIENTED_EDGE ( 'NONE', *, *, #38227, .T. ) ;
#16380=PLANE ( 'NONE',  #44627 ) ;
#16381=EDGE_CURVE ( 'NONE', #37296, #55481, #28009, .T. ) ;
#16382=VERTEX_POINT ( 'NONE', #18346 ) ;
#16383=LINE ( 'NONE', #33709, #47333 ) ;
#16384=ADVANCED_FACE ( 'NONE', ( #35687 ), #27163, .F. ) ;
#16385=DIRECTION ( 'NONE',  ( 0.007781995580012663651, -3.146120232559066537E-19, -0.9999697198139514409 ) ) ;
#16387=EDGE_CURVE ( 'NONE', #41466, #24940, #10947, .T. ) ;
#16388=DIRECTION ( 'NONE',  ( 0.005002170337468016433, -0.7660444431189770143, -0.6427681459581293666 ) ) ;
#16389=DIRECTION ( 'NONE',  ( 0.000000000000000000, -1.000000000000000000, 0.000000000000000000 ) ) ;
#16390=CARTESIAN_POINT ( 'NONE',  ( -10.00813838035478298, 0.000000000000000000, 10.77830692922518452 ) ) ;
#16391=CARTESIAN_POINT ( 'NONE',  ( -18.69579972149740854, -0.1191753592594173433, 5.513579256858934130 ) ) ;
#16392=CARTESIAN_POINT ( 'NONE',  ( -8.875996589204540044, 0.000000000000000000, 10.41778544861944233 ) ) ;
#16393=ORIENTED_EDGE ( 'NONE', *, *, #8880, .T. ) ;
#16396=EDGE_CURVE ( 'NONE', #43993, #8713, #54380, .T. ) ;
#16397=ADVANCED_FACE ( 'NONE', ( #11228 ), #41607, .F. ) ;
#16399=VECTOR ( 'NONE', #1713, 1000.000000000000000 ) ;
#16400=PLANE ( 'NONE',  #55564 ) ;
#16401=DIRECTION ( 'NONE',  ( -0.005961354470445682716, -0.6427876096865404731, 0.7660212471507180654 ) ) ;
#16402=CARTESIAN_POINT ( 'NONE',  ( -19.44088468089161026, -1.003701604285655469, 5.880676884387883163 ) ) ;
#16403=LINE ( 'NONE', #46809, #2249 ) ;
#16404=DIRECTION ( 'NONE',  ( -0.7660212471507179544, -0.6427876096865405842, -0.005961354470445141482 ) ) ;
#16406=LINE ( 'NONE', #37426, #6688 ) ;
#16408=ORIENTED_EDGE ( 'NONE', *, *, #26064, .F. ) ;
#16409=CARTESIAN_POINT ( 'NONE',  ( -29.86197018149027116, 0.000000000000000000, 8.281335066757780083 ) ) ;
#16411=CARTESIAN_POINT ( 'NONE',  ( -16.94377541268302778, 0.000000000000000000, 6.365881082869898400 ) ) ;
#16412=DIRECTION ( 'NONE',  ( -0.9999697198139514409, -0.000000000000000000, -0.007781995580013368816 ) ) ;
#16414=CARTESIAN_POINT ( 'NONE',  ( -10.14100915727248164, 0.000000000000000000, 7.157485922469027706 ) ) ;
#16415=ADVANCED_FACE ( 'NONE', ( #28550 ), #32546, .F. ) ;
#16416=DIRECTION ( 'NONE',  ( 0.005002170337468016433, -0.7660444431189770143, -0.6427681459581293666 ) ) ;
#16417=CARTESIAN_POINT ( 'NONE',  ( -20.57654483182816918, -1.813211359398158029, 4.816098976698940604 ) ) ;
#16418=DIRECTION ( 'NONE',  ( 0.9999697198139515519, 0.000000000000000000, 0.007781995580013368816 ) ) ;
#16419=ORIENTED_EDGE ( 'NONE', *, *, #25838, .T. ) ;
#16420=AXIS2_PLACEMENT_3D ( 'NONE', #46506, #50521, #24954 ) ;
#16421=EDGE_CURVE ( 'NONE', #27552, #23390, #29393, .T. ) ;
#16422=PLANE ( 'NONE',  #2212 ) ;
#16423=FACE_OUTER_BOUND ( 'NONE', #39356, .T. ) ;
#16424=ORIENTED_EDGE ( 'NONE', *, *, #49170, .F. ) ;
#16425=EDGE_CURVE ( 'NONE', #41830, #28682, #11528, .T. ) ;
#16426=VERTEX_POINT ( 'NONE', #55229 ) ;
#16427=FACE_OUTER_BOUND ( 'NONE', #52709, .T. ) ;
#16428=EDGE_CURVE ( 'NONE', #16370, #31087, #29097, .T. ) ;
#16429=EDGE_LOOP ( 'NONE', ( #51865, #13150, #12701, #17225 ) ) ;
#16430=ORIENTED_EDGE ( 'NONE', *, *, #31397, .T. ) ;
#16431=PLANE ( 'NONE',  #14833 ) ;
#16432=ORIENTED_EDGE ( 'NONE', *, *, #24683, .T. ) ;
#16433=ORIENTED_EDGE ( 'NONE', *, *, #36359, .T. ) ;
#16434=ORIENTED_EDGE ( 'NONE', *, *, #30905, .T. ) ;
#16435=DIRECTION ( 'NONE',  ( -0.6427681459581293666, -0.7660444431189770143, -0.005002170337467561935 ) ) ;
#16436=DIRECTION ( 'NONE',  ( 0.007781995580012663651, -3.146120232559066537E-19, -0.9999697198139514409 ) ) ;
#16437=CARTESIAN_POINT ( 'NONE',  ( -16.00719711287428737, 0.000000000000000000, 5.434499555927599701 ) ) ;
#16438=AXIS2_PLACEMENT_3D ( 'NONE', #3381, #29197, #41694 ) ;
#16439=VECTOR ( 'NONE', #14723, 999.9999999999998863 ) ;
#16440=VERTEX_POINT ( 'NONE', #50111 ) ;
#16441=ORIENTED_EDGE ( 'NONE', *, *, #32645, .T. ) ;
#16442=DIRECTION ( 'NONE',  ( 0.007781995580012663651, -3.146120232559066537E-19, -0.9999697198139514409 ) ) ;
#16443=CARTESIAN_POINT ( 'NONE',  ( 2.072287782118878319, 0.000000000000000000, -2.950529333540147015 ) ) ;
#16444=ORIENTED_EDGE ( 'NONE', *, *, #53364, .F. ) ;
#16445=FACE_OUTER_BOUND ( 'NONE', #803, .T. ) ;
#16446=DIRECTION ( 'NONE',  ( 0.007781995580012662783, 0.000000000000000000, -0.9999697198139514409 ) ) ;
#16447=ORIENTED_EDGE ( 'NONE', *, *, #30736, .F. ) ;
#16448=PLANE ( 'NONE',  #16715 ) ;
#16449=PLANE ( 'NONE',  #29448 ) ;
#16450=EDGE_CURVE ( 'NONE', #29013, #24466, #54649, .T. ) ;
#16451=VERTEX_POINT ( 'NONE', #6699 ) ;
#16452=CARTESIAN_POINT ( 'NONE',  ( -19.25070634120488222, 0.000000000000000000, 4.259254523999361552 ) ) ;
#16453=EDGE_CURVE ( 'NONE', #41032, #24619, #20012, .T. ) ;
#16454=AXIS2_PLACEMENT_3D ( 'NONE', #15901, #16184, #28120 ) ;
#16455=LINE ( 'NONE', #33783, #39089 ) ;
#16456=ORIENTED_EDGE ( 'NONE', *, *, #41617, .F. ) ;
#16457=LINE ( 'NONE', #1089, #33999 ) ;
#16458=PLANE ( 'NONE',  #5728 ) ;
#16459=DIRECTION ( 'NONE',  ( 0.005961354470445682716, -0.6427876096865404731, -0.7660212471507180654 ) ) ;
#16460=LINE ( 'NONE', #33789, #15616 ) ;
#16461=ORIENTED_EDGE ( 'NONE', *, *, #718, .F. ) ;
#16462=EDGE_CURVE ( 'NONE', #31624, #24198, #54963, .T. ) ;
#16463=EDGE_CURVE ( 'NONE', #21299, #35152, #37337, .T. ) ;
#16464=EDGE_CURVE ( 'NONE', #44511, #46096, #33099, .T. ) ;
#16465=CARTESIAN_POINT ( 'NONE',  ( -18.76354595665420177, -0.1191753592594177458, 14.21882498613976331 ) ) ;
#16466=CARTESIAN_POINT ( 'NONE',  ( -10.21012437789221217, 0.000000000000000000, 2.724963214160391445 ) ) ;
#16467=DIRECTION ( 'NONE',  ( -0.5449076811759708816, 0.6444004775717707689, 0.5364919789714475140 ) ) ;
#16468=CARTESIAN_POINT ( 'NONE',  ( -14.94760462649100496, 0.000000000000000000, 2.488088991209854051 ) ) ;
#16469=EDGE_CURVE ( 'NONE', #53596, #27982, #3274, .T. ) ;
#16470=DIRECTION ( 'NONE',  ( 0.7660212471507180654, -0.6427876096865404731, 0.005961354470445141482 ) ) ;
#16471=DIRECTION ( 'NONE',  ( 0.5364919789714477361, 0.6444004775717706579, 0.5449076811759711036 ) ) ;
#16472=CARTESIAN_POINT ( 'NONE',  ( 2.072287782118878319, 0.000000000000000000, -2.950529333540147015 ) ) ;
#16473=ORIENTED_EDGE ( 'NONE', *, *, #48624, .T. ) ;
#16475=PLANE ( 'NONE',  #2413 ) ;
#16476=VERTEX_POINT ( 'NONE', #16316 ) ;
#16477=DIRECTION ( 'NONE',  ( -0.5449076811759708816, 0.6444004775717707689, 0.5364919789714475140 ) ) ;
#16478=CARTESIAN_POINT ( 'NONE',  ( -17.88038292028693732, -3.594132820645663084, 3.711997409451107455 ) ) ;
#16480=VECTOR ( 'NONE', #27361, 999.9999999999998863 ) ;
#16481=CARTESIAN_POINT ( 'NONE',  ( -19.79569077582305070, 0.000000000000000000, 14.58012466630350445 ) ) ;
#16482=PLANE ( 'NONE',  #13352 ) ;
#16483=ADVANCED_FACE ( 'NONE', ( #33635 ), #50949, .F. ) ;
#16484=LINE ( 'NONE', #20486, #25638 ) ;
#16485=ORIENTED_EDGE ( 'NONE', *, *, #1085, .F. ) ;
#16486=VECTOR ( 'NONE', #40150, 999.9999999999998863 ) ;
#16487=EDGE_LOOP ( 'NONE', ( #12559, #7411, #25415, #39860 ) ) ;
#16488=ADVANCED_FACE ( 'NONE', ( #23726 ), #2139, .F. ) ;
#16489=CARTESIAN_POINT ( 'NONE',  ( -12.10028655381466578, 0.000000000000000000, 6.772906302923760613 ) ) ;
#16491=ORIENTED_EDGE ( 'NONE', *, *, #10402, .T. ) ;
#16492=CARTESIAN_POINT ( 'NONE',  ( -9.876320842032628278, -0.1191753592594181482, 6.690210690224407841 ) ) ;
#16493=EDGE_CURVE ( 'NONE', #54483, #38787, #15477, .T. ) ;
#16494=ORIENTED_EDGE ( 'NONE', *, *, #52345, .T. ) ;
#16495=LINE ( 'NONE', #24458, #53993 ) ;
#16496=AXIS2_PLACEMENT_3D ( 'NONE', #38544, #12445, #43089 ) ;
#16497=VERTEX_POINT ( 'NONE', #17437 ) ;
#16498=CARTESIAN_POINT ( 'NONE',  ( -15.03495456790438389, -0.1191753592594197858, 12.77051346725278158 ) ) ;
#16499=EDGE_CURVE ( 'NONE', #43061, #23916, #12908, .T. ) ;
#16500=VECTOR ( 'NONE', #43086, 1000.000000000000227 ) ;
#16502=VERTEX_POINT ( 'NONE', #51798 ) ;
#16503=ORIENTED_EDGE ( 'NONE', *, *, #53331, .F. ) ;
#16504=LINE ( 'NONE', #4576, #10304 ) ;
#16505=DIRECTION ( 'NONE',  ( -0.7660212471507179544, -0.6427876096865405842, -0.005961354470445141482 ) ) ;
#16506=CARTESIAN_POINT ( 'NONE',  ( -13.88852388610687250, 1.905425754524005200, 5.403223730618197607 ) ) ;
#16507=PLANE ( 'NONE',  #10231 ) ;
#16508=ORIENTED_EDGE ( 'NONE', *, *, #37671, .F. ) ;
#16509=EDGE_LOOP ( 'NONE', ( #867, #9634, #1377, #16792 ) ) ;
#16510=EDGE_LOOP ( 'NONE', ( #19452, #8003, #37825, #37098 ) ) ;
#16511=DIRECTION ( 'NONE',  ( -0.5449076811759708816, 0.6444004775717707689, 0.5364919789714475140 ) ) ;
#16512=LINE ( 'NONE', #24760, #24920 ) ;
#16513=EDGE_LOOP ( 'NONE', ( #31563, #8852, #32722, #48708 ) ) ;
#16514=VECTOR ( 'NONE', #28653, 999.9999999999998863 ) ;
#16515=CARTESIAN_POINT ( 'NONE',  ( -12.82965364628315719, 0.1245042932765029059, 1.661432565772024361 ) ) ;
#16516=ORIENTED_EDGE ( 'NONE', *, *, #15159, .T. ) ;
#16517=DIRECTION ( 'NONE',  ( 0.005002170337468016433, -0.7660444431189770143, -0.6427681459581293666 ) ) ;
#16518=DIRECTION ( 'NONE',  ( 0.9999697198139515519, 0.000000000000000000, 0.007781995580013368816 ) ) ;
#16519=AXIS2_PLACEMENT_3D ( 'NONE', #2934, #11754, #36777 ) ;
#16520=VECTOR ( 'NONE', #27035, 1000.000000000000227 ) ;
#16521=ORIENTED_EDGE ( 'NONE', *, *, #29536, .F. ) ;
#16522=CARTESIAN_POINT ( 'NONE',  ( -17.20554431205604828, 0.000000000000000000, 5.994511866960127833 ) ) ;
#16524=VECTOR ( 'NONE', #21817, 999.9999999999998863 ) ;
#16525=DIRECTION ( 'NONE',  ( -0.5449076811759708816, 0.6444004775717707689, 0.5364919789714475140 ) ) ;
#16526=DIRECTION ( 'NONE',  ( -0.005002170337468016433, -0.7660444431189770143, 0.6427681459581293666 ) ) ;
#16528=ORIENTED_EDGE ( 'NONE', *, *, #42472, .F. ) ;
#16529=PLANE ( 'NONE',  #48593 ) ;
#16530=FACE_OUTER_BOUND ( 'NONE', #4536, .T. ) ;
#16531=CARTESIAN_POINT ( 'NONE',  ( -17.32200740551113327, -0.1191753592594158168, 8.109594914967312107 ) ) ;
#16532=LINE ( 'NONE', #11456, #22857 ) ;
#16533=ORIENTED_EDGE ( 'NONE', *, *, #24889, .T. ) ;
#16534=EDGE_CURVE ( 'NONE', #42137, #25299, #47256, .T. ) ;
#16535=ORIENTED_EDGE ( 'NONE', *, *, #43197, .T. ) ;
#16536=DIRECTION ( 'NONE',  ( 0.9999697198139515519, 0.000000000000000000, 0.007781995580013368816 ) ) ;
#16537=PLANE ( 'NONE',  #30355 ) ;
#16538=VECTOR ( 'NONE', #22827, 999.9999999999998863 ) ;
#16539=DIRECTION ( 'NONE',  ( -0.9999697198139514409, -0.000000000000000000, -0.007781995580013368816 ) ) ;
#16540=EDGE_CURVE ( 'NONE', #593, #24779, #55495, .T. ) ;
#16541=EDGE_CURVE ( 'NONE', #10709, #50934, #16907, .T. ) ;
#16542=LINE ( 'NONE', #6634, #29427 ) ;
#16543=FACE_OUTER_BOUND ( 'NONE', #55024, .T. ) ;
#16544=LINE ( 'NONE', #24788, #55767 ) ;
#16545=ORIENTED_EDGE ( 'NONE', *, *, #36954, .T. ) ;
#16546=DIRECTION ( 'NONE',  ( -0.6427681459581293666, -0.7660444431189770143, -0.005002170337467561935 ) ) ;
#16547=DIRECTION ( 'NONE',  ( 0.007781995580012663651, -3.146120232559066537E-19, -0.9999697198139514409 ) ) ;
#16548=ORIENTED_EDGE ( 'NONE', *, *, #40899, .F. ) ;
#16549=DIRECTION ( 'NONE',  ( -0.6427681459581293666, -0.7660444431189770143, -0.005002170337467561935 ) ) ;
#16550=EDGE_LOOP ( 'NONE', ( #1010, #46002, #7287, #55995 ) ) ;
#16552=CARTESIAN_POINT ( 'NONE',  ( -16.79925329029790149, 0.000000000000000000, 13.49544742625427496 ) ) ;
#16553=CARTESIAN_POINT ( 'NONE',  ( -19.60990026154428278, 0.000000000000000000, 4.498472333781370125 ) ) ;
#16554=AXIS2_PLACEMENT_3D ( 'NONE', #16149, #24950, #7332 ) ;
#16555=FACE_OUTER_BOUND ( 'NONE', #11823, .T. ) ;
#16557=VERTEX_POINT ( 'NONE', #43012 ) ;
#16558=EDGE_LOOP ( 'NONE', ( #18082, #55705, #45299, #49447 ) ) ;
#16559=DIRECTION ( 'NONE',  ( -0.005961354470445682716, -0.6427876096865404731, 0.7660212471507180654 ) ) ;
#16560=LINE ( 'NONE', #24518, #43115 ) ;
#16561=AXIS2_PLACEMENT_3D ( 'NONE', #11194, #15728, #23979 ) ;
#16562=PLANE ( 'NONE',  #36049 ) ;
#16563=AXIS2_PLACEMENT_3D ( 'NONE', #14694, #23502, #15514 ) ;
#16564=LINE ( 'NONE', #46374, #17894 ) ;
#16565=AXIS2_PLACEMENT_3D ( 'NONE', #37416, #54201, #11854 ) ;
#16566=PLANE ( 'NONE',  #36472 ) ;
#16567=CARTESIAN_POINT ( 'NONE',  ( -21.47419595591918906, 0.000000000000000000, 5.222628093224860102 ) ) ;
#16568=ORIENTED_EDGE ( 'NONE', *, *, #52068, .F. ) ;
#16569=DIRECTION ( 'NONE',  ( 0.007781995580012662783, 0.000000000000000000, -0.9999697198139514409 ) ) ;
#16570=ADVANCED_FACE ( 'NONE', ( #34239 ), #13482, .F. ) ;
#16571=DIRECTION ( 'NONE',  ( 0.005961354470445682716, -0.6427876096865404731, -0.7660212471507180654 ) ) ;
#16572=VECTOR ( 'NONE', #34743, 1000.000000000000000 ) ;
#16573=LINE ( 'NONE', #32774, #17879 ) ;
#16574=VECTOR ( 'NONE', #11857, 1000.000000000000227 ) ;
#16575=ORIENTED_EDGE ( 'NONE', *, *, #39853, .F. ) ;
#16576=EDGE_CURVE ( 'NONE', #37968, #11293, #21138, .T. ) ;
#16577=CARTESIAN_POINT ( 'NONE',  ( -14.62700148656139199, -2.460819163488158878, 6.402179327102785145 ) ) ;
#16578=CARTESIAN_POINT ( 'NONE',  ( -17.73140113748535285, 0.000000000000000000, 13.85752530597602039 ) ) ;
#16579=DIRECTION ( 'NONE',  ( 0.5364919789714477361, 0.6444004775717706579, 0.5449076811759711036 ) ) ;
#16581=CARTESIAN_POINT ( 'NONE',  ( -11.33076995502132256, 0.000000000000000000, 1.608245881735075100 ) ) ;
#16582=EDGE_CURVE ( 'NONE', #29241, #30062, #4121, .T. ) ;
#16583=VECTOR ( 'NONE', #26129, 999.9999999999998863 ) ;
#16585=VECTOR ( 'NONE', #54709, 999.9999999999998863 ) ;
#16587=EDGE_LOOP ( 'NONE', ( #34902, #26886, #18173, #30353 ) ) ;
#16588=ORIENTED_EDGE ( 'NONE', *, *, #14823, .T. ) ;
#16589=CARTESIAN_POINT ( 'NONE',  ( -14.94838282604900748, -0.1191753592594197858, 2.588085963191248506 ) ) ;
#16590=ORIENTED_EDGE ( 'NONE', *, *, #40754, .F. ) ;
#16591=AXIS2_PLACEMENT_3D ( 'NONE', #22822, #52637, #14033 ) ;
#16592=CARTESIAN_POINT ( 'NONE',  ( -26.13493519185646008, 0.000000000000000000, 7.033017491833586377 ) ) ;
#16593=EDGE_LOOP ( 'NONE', ( #43611, #40346, #40034, #48628 ) ) ;
#16594=DIRECTION ( 'NONE',  ( -0.6427681459581293666, -0.7660444431189770143, -0.005002170337467561935 ) ) ;
#16595=ORIENTED_EDGE ( 'NONE', *, *, #50157, .F. ) ;
#16596=AXIS2_PLACEMENT_3D ( 'NONE', #44630, #5468, #52602 ) ;
#16597=ORIENTED_EDGE ( 'NONE', *, *, #11490, .T. ) ;
#16598=CARTESIAN_POINT ( 'NONE',  ( -9.075990533167328067, 0.000000000000000000, 10.41622904950343909 ) ) ;
#16599=CARTESIAN_POINT ( 'NONE',  ( -13.68269497427957937, 0.000000000000000000, 5.283263355472670675 ) ) ;
#16600=FACE_OUTER_BOUND ( 'NONE', #12253, .T. ) ;
#16601=CARTESIAN_POINT ( 'NONE',  ( -18.91005987905199603, 1.257817950434005683, 3.987110198832547248 ) ) ;
#16602=AXIS2_PLACEMENT_3D ( 'NONE', #21884, #17634, #23311 ) ;
#16603=EDGE_CURVE ( 'NONE', #27953, #30961, #39311, .T. ) ;
#16604=CARTESIAN_POINT ( 'NONE',  ( -17.86574470023862560, 0.000000000000000000, 5.420035908855560969 ) ) ;
#16605=ORIENTED_EDGE ( 'NONE', *, *, #17975, .T. ) ;
#16606=VECTOR ( 'NONE', #43502, 1000.000000000000114 ) ;
#16607=VECTOR ( 'NONE', #4682, 999.9999999999998863 ) ;
#16608=EDGE_CURVE ( 'NONE', #33688, #1588, #38772, .T. ) ;
#16609=ORIENTED_EDGE ( 'NONE', *, *, #1682, .F. ) ;
#16610=LINE ( 'NONE', #20866, #34915 ) ;
#16611=DIRECTION ( 'NONE',  ( 0.005002170337468016433, -0.7660444431189770143, -0.6427681459581293666 ) ) ;
#16613=EDGE_CURVE ( 'NONE', #6528, #9930, #39031, .T. ) ;
#16614=CARTESIAN_POINT ( 'NONE',  ( -14.02931237854957836, -0.1191753592594187450, 2.964570451734679146 ) ) ;
#16615=AXIS2_PLACEMENT_3D ( 'NONE', #25321, #9114, #21889 ) ;
#16616=AXIS2_PLACEMENT_3D ( 'NONE', #32148, #18513, #40387 ) ;
#16617=PLANE ( 'NONE',  #9621 ) ;
#16618=LINE ( 'NONE', #29713, #43972 ) ;
#16619=DIRECTION ( 'NONE',  ( -0.3620778797217457101, 0.000000000000000000, -0.9321478471874540261 ) ) ;
#16620=ORIENTED_EDGE ( 'NONE', *, *, #21719, .T. ) ;
#16621=CARTESIAN_POINT ( 'NONE',  ( -15.60102546347950536, 0.000000000000000000, 12.95077420755565356 ) ) ;
#16622=DIRECTION ( 'NONE',  ( -0.5449076811759708816, 0.6444004775717707689, 0.5364919789714475140 ) ) ;
#16623=EDGE_LOOP ( 'NONE', ( #49346, #22485, #49113, #8437, #41987 ) ) ;
#16624=LINE ( 'NONE', #12394, #37011 ) ;
#16625=DIRECTION ( 'NONE',  ( 0.2426528472758542054, 0.7422098413412800966, 0.6246952433987894571 ) ) ;
#16626=DIRECTION ( 'NONE',  ( 0.6427681459581294776, -0.7660444431189769032, 0.005002170337467562802 ) ) ;
#16627=LINE ( 'NONE', #11803, #29559 ) ;
#16628=VECTOR ( 'NONE', #15467, 1000.000000000000227 ) ;
#16629=LINE ( 'NONE', #20881, #20473 ) ;
#16630=EDGE_CURVE ( 'NONE', #866, #15209, #401, .T. ) ;
#16631=VERTEX_POINT ( 'NONE', #52385 ) ;
#16632=VERTEX_POINT ( 'NONE', #21721 ) ;
#16633=LINE ( 'NONE', #37946, #37530 ) ;
#16634=PLANE ( 'NONE',  #4118 ) ;
#16635=CARTESIAN_POINT ( 'NONE',  ( -22.40478740399063895, 0.000000000000000000, 5.384712028983816623 ) ) ;
#16636=AXIS2_PLACEMENT_3D ( 'NONE', #33710, #51026, #29472 ) ;
#16637=LINE ( 'NONE', #3580, #42746 ) ;
#16638=CARTESIAN_POINT ( 'NONE',  ( -19.59569683186026268, 0.000000000000000000, 14.58168106541950948 ) ) ;
#16639=VECTOR ( 'NONE', #1499, 999.9999999999998863 ) ;
#16640=CARTESIAN_POINT ( 'NONE',  ( -23.33771345073609638, -0.1191753592594197858, 5.846786880686956955 ) ) ;
#16641=DIRECTION ( 'NONE',  ( 0.005002170337468016433, -0.7660444431189770143, -0.6427681459581293666 ) ) ;
#16642=CARTESIAN_POINT ( 'NONE',  ( 2.072287782118878319, 0.000000000000000000, -2.950529333540147015 ) ) ;
#16644=VECTOR ( 'NONE', #23170, 1000.000000000000000 ) ;
#16645=DIRECTION ( 'NONE',  ( 0.5364919789714477361, 0.6444004775717706579, 0.5449076811759711036 ) ) ;
#16646=EDGE_LOOP ( 'NONE', ( #51178, #14945, #5879, #27341 ) ) ;
#16648=AXIS2_PLACEMENT_3D ( 'NONE', #11151, #15994, #49789 ) ;
#16649=AXIS2_PLACEMENT_3D ( 'NONE', #31531, #35777, #48841 ) ;
#16650=EDGE_LOOP ( 'NONE', ( #42431, #19293, #22002, #9250 ) ) ;
#16651=EDGE_CURVE ( 'NONE', #55479, #48095, #47846, .T. ) ;
#16652=ORIENTED_EDGE ( 'NONE', *, *, #52817, .T. ) ;
#16653=AXIS2_PLACEMENT_3D ( 'NONE', #40509, #40772, #49281 ) ;
#16655=EDGE_LOOP ( 'NONE', ( #50646, #50057, #5080, #3435 ) ) ;
#16656=VECTOR ( 'NONE', #53106, 1000.000000000000000 ) ;
#16657=ORIENTED_EDGE ( 'NONE', *, *, #8753, .F. ) ;
#16658=VERTEX_POINT ( 'NONE', #56088 ) ;
#16659=DIRECTION ( 'NONE',  ( 0.007781995580012662783, 0.000000000000000000, -0.9999697198139514409 ) ) ;
#16660=LINE ( 'NONE', #16367, #12991 ) ;
#16661=PLANE ( 'NONE',  #44817 ) ;
#16662=EDGE_CURVE ( 'NONE', #947, #29012, #17173, .T. ) ;
#16663=ORIENTED_EDGE ( 'NONE', *, *, #32786, .T. ) ;
#16664=DIRECTION ( 'NONE',  ( 0.005961354470445682716, -0.6427876096865404731, -0.7660212471507180654 ) ) ;
#16665=VERTEX_POINT ( 'NONE', #16599 ) ;
#16666=DIRECTION ( 'NONE',  ( -0.005961354470445682716, -0.6427876096865404731, 0.7660212471507180654 ) ) ;
#16667=EDGE_CURVE ( 'NONE', #48671, #40111, #33935, .T. ) ;
#16668=ORIENTED_EDGE ( 'NONE', *, *, #3072, .T. ) ;
#16669=EDGE_CURVE ( 'NONE', #19391, #26974, #17745, .T. ) ;
#16670=LINE ( 'NONE', #166, #46630 ) ;
#16671=VECTOR ( 'NONE', #50872, 1000.000000000000227 ) ;
#16672=DIRECTION ( 'NONE',  ( 0.007781995580012663651, 0.000000000000000000, -0.9999697198139515519 ) ) ;
#16673=CARTESIAN_POINT ( 'NONE',  ( -11.80977711938882280, 0.000000000000000000, 3.451178486255886302 ) ) ;
#16674=EDGE_CURVE ( 'NONE', #50886, #43539, #8102, .T. ) ;
#16675=EDGE_LOOP ( 'NONE', ( #19556, #27255, #56110, #20741 ) ) ;
#16676=DIRECTION ( 'NONE',  ( 0.7660212471507180654, -0.6427876096865404731, 0.005961354470445141482 ) ) ;
#16677=AXIS2_PLACEMENT_3D ( 'NONE', #20675, #51337, #25223 ) ;
#16678=ORIENTED_EDGE ( 'NONE', *, *, #19814, .T. ) ;
#16679=DIRECTION ( 'NONE',  ( -0.5449076811759708816, 0.6444004775717707689, 0.5364919789714475140 ) ) ;
#16680=EDGE_CURVE ( 'NONE', #43283, #40959, #29703, .T. ) ;
#16681=DIRECTION ( 'NONE',  ( -0.5364919789714478471, 0.6444004775717705469, -0.5449076811759709926 ) ) ;
#16682=VECTOR ( 'NONE', #31992, 999.9999999999998863 ) ;
#16683=EDGE_CURVE ( 'NONE', #36712, #30417, #53237, .T. ) ;
#16684=LINE ( 'NONE', #42788, #7883 ) ;
#16686=CARTESIAN_POINT ( 'NONE',  ( -16.15304353870583043, 4.010151117816509903, 9.737052958454759377 ) ) ;
#16687=CARTESIAN_POINT ( 'NONE',  ( -27.99767448711536133, 0.000000000000000000, 7.557179307314289218 ) ) ;
#16689=CARTESIAN_POINT ( 'NONE',  ( -15.06930115867626974, 0.000000000000000000, 4.333802269690326447 ) ) ;
#16690=VECTOR ( 'NONE', #24211, 999.9999999999998863 ) ;
#16691=DIRECTION ( 'NONE',  ( -0.5364919789714478471, 0.6444004775717705469, -0.5449076811759709926 ) ) ;
#16692=ORIENTED_EDGE ( 'NONE', *, *, #7329, .T. ) ;
#16693=PLANE ( 'NONE',  #50121 ) ;
#16694=VERTEX_POINT ( 'NONE', #4956 ) ;
#16695=VECTOR ( 'NONE', #47407, 1000.000000000000114 ) ;
#16696=ADVANCED_FACE ( 'NONE', ( #22824 ), #9206, .F. ) ;
#16697=DIRECTION ( 'NONE',  ( 0.3313982828793700097, 0.4028455766673916805, 0.8531650599175528704 ) ) ;
#16698=CARTESIAN_POINT ( 'NONE',  ( -22.29430420027960125, 4.172053068839010947, 5.208686264645241870 ) ) ;
#16699=LINE ( 'NONE', #34029, #1448 ) ;
#16700=CARTESIAN_POINT ( 'NONE',  ( -29.86352658060627618, 0.000000000000000000, 8.481329010720569883 ) ) ;
#16701=CARTESIAN_POINT ( 'NONE',  ( 2.072287782118878319, 0.000000000000000000, -2.950529333540147015 ) ) ;
#16702=EDGE_CURVE ( 'NONE', #49293, #8255, #13740, .T. ) ;
#16703=VECTOR ( 'NONE', #39903, 1000.000000000000227 ) ;
#16704=CARTESIAN_POINT ( 'NONE',  ( -11.67244013076689946, 0.000000000000000000, 11.50401908778467863 ) ) ;
#16705=VECTOR ( 'NONE', #55529, 999.9999999999998863 ) ;
#16706=ORIENTED_EDGE ( 'NONE', *, *, #10188, .T. ) ;
#16708=DIRECTION ( 'NONE',  ( 0.5364919789714477361, 0.6444004775717706579, 0.5449076811759711036 ) ) ;
#16709=LINE ( 'NONE', #7335, #7343 ) ;
#16710=PLANE ( 'NONE',  #54493 ) ;
#16711=PLANE ( 'NONE',  #46557 ) ;
#16712=CARTESIAN_POINT ( 'NONE',  ( -19.79569077582305070, 0.000000000000000000, 14.58012466630350445 ) ) ;
#16713=DIRECTION ( 'NONE',  ( -0.005961354470445682716, -0.6427876096865404731, 0.7660212471507180654 ) ) ;
#16714=ORIENTED_EDGE ( 'NONE', *, *, #3072, .F. ) ;
#16715=AXIS2_PLACEMENT_3D ( 'NONE', #11907, #7668, #52161 ) ;
#16716=CARTESIAN_POINT ( 'NONE',  ( -9.808144436391993182, 0.000000000000000000, 10.77986332834118777 ) ) ;
#16717=DIRECTION ( 'NONE',  ( 0.5364919789714477361, 0.6444004775717706579, 0.5449076811759711036 ) ) ;
#16718=ORIENTED_EDGE ( 'NONE', *, *, #12247, .F. ) ;
#16719=ORIENTED_EDGE ( 'NONE', *, *, #29084, .F. ) ;
#16720=DIRECTION ( 'NONE',  ( 0.007781995580012663651, 0.000000000000000000, -0.9999697198139515519 ) ) ;
#16721=VECTOR ( 'NONE', #50892, 999.9999999999998863 ) ;
#16722=ORIENTED_EDGE ( 'NONE', *, *, #45221, .T. ) ;
#16725=EDGE_LOOP ( 'NONE', ( #14149, #46623, #52135, #31198 ) ) ;
#16726=VECTOR ( 'NONE', #44413, 1000.000000000000227 ) ;
#16727=ORIENTED_EDGE ( 'NONE', *, *, #44157, .T. ) ;
#16728=LINE ( 'NONE', #5304, #26592 ) ;
#16729=VECTOR ( 'NONE', #12118, 999.9999999999998863 ) ;
#16730=DIRECTION ( 'NONE',  ( 0.005002170337468016433, -0.7660444431189770143, -0.6427681459581293666 ) ) ;
#16731=CARTESIAN_POINT ( 'NONE',  ( -33.59211796935609584, 0.000000000000000000, 9.929640529607549837 ) ) ;
#16732=EDGE_CURVE ( 'NONE', #28952, #41133, #18574, .T. ) ;
#16733=VECTOR ( 'NONE', #11995, 999.9999999999998863 ) ;
#16734=ORIENTED_EDGE ( 'NONE', *, *, #47373, .T. ) ;
#16735=ORIENTED_EDGE ( 'NONE', *, *, #8144, .F. ) ;
#16736=EDGE_CURVE ( 'NONE', #2673, #39913, #27099, .T. ) ;
#16737=VECTOR ( 'NONE', #35572, 999.9999999999998863 ) ;
#16738=AXIS2_PLACEMENT_3D ( 'NONE', #38429, #47513, #46667 ) ;
#16739=CARTESIAN_POINT ( 'NONE',  ( 2.072287782118878319, 0.000000000000000000, -2.950529333540147015 ) ) ;
#16740=DIRECTION ( 'NONE',  ( -0.7660212471507179544, -0.6427876096865405842, -0.005961354470445141482 ) ) ;
#16741=ORIENTED_EDGE ( 'NONE', *, *, #49174, .T. ) ;
#16742=DIRECTION ( 'NONE',  ( 0.9999697198139515519, 0.000000000000000000, 0.007781995580013368816 ) ) ;
#16743=CARTESIAN_POINT ( 'NONE',  ( -26.13415699229845757, -0.1191753592594197858, 6.933020519852192365 ) ) ;
#16744=VERTEX_POINT ( 'NONE', #39618 ) ;
#16745=CARTESIAN_POINT ( 'NONE',  ( -9.283724637715325301, 0.000000000000000000, 3.101504740954174277 ) ) ;
#16746=EDGE_LOOP ( 'NONE', ( #18200, #51773, #54929, #47387, #23684 ) ) ;
#16747=FACE_OUTER_BOUND ( 'NONE', #14592, .T. ) ;
#16748=EDGE_CURVE ( 'NONE', #22478, #47842, #22285, .T. ) ;
#16750=VECTOR ( 'NONE', #25796, 1000.000000000000000 ) ;
#16751=DIRECTION ( 'NONE',  ( -0.5364919789714478471, 0.6444004775717705469, -0.5449076811759709926 ) ) ;
#16752=ORIENTED_EDGE ( 'NONE', *, *, #3159, .T. ) ;
#16753=DIRECTION ( 'NONE',  ( -0.6427681459581293666, -0.7660444431189770143, -0.005002170337467561935 ) ) ;
#16754=LINE ( 'NONE', #47709, #17521 ) ;
#16755=LINE ( 'NONE', #251, #48435 ) ;
#16756=VECTOR ( 'NONE', #28123, 1000.000000000000114 ) ;
#16757=DIRECTION ( 'NONE',  ( 0.5364919789714477361, 0.6444004775717706579, 0.5449076811759711036 ) ) ;
#16758=ORIENTED_EDGE ( 'NONE', *, *, #4706, .F. ) ;
#16759=VECTOR ( 'NONE', #53168, 1000.000000000000227 ) ;
#16760=EDGE_CURVE ( 'NONE', #31029, #38002, #40144, .T. ) ;
#16761=CARTESIAN_POINT ( 'NONE',  ( -21.47419595591918906, 0.000000000000000000, 5.222628093224860102 ) ) ;
#16762=DIRECTION ( 'NONE',  ( 0.6427681459581294776, -0.7660444431189769032, 0.005002170337467562802 ) ) ;
#16763=DIRECTION ( 'NONE',  ( 0.007781995580012663651, 0.000000000000000000, -0.9999697198139515519 ) ) ;
#16764=VECTOR ( 'NONE', #40910, 999.9999999999998863 ) ;
#16765=DIRECTION ( 'NONE',  ( 0.007781995580012662783, 0.000000000000000000, -0.9999697198139514409 ) ) ;
#16766=LINE ( 'NONE', #34103, #16779 ) ;
#16767=DIRECTION ( 'NONE',  ( 0.007781995580012662783, 0.000000000000000000, -0.9999697198139514409 ) ) ;
#16768=VECTOR ( 'NONE', #44978, 999.9999999999998863 ) ;
#16769=DIRECTION ( 'NONE',  ( 0.6427681459581294776, -0.7660444431189769032, 0.005002170337467562802 ) ) ;
#16770=VECTOR ( 'NONE', #11998, 1000.000000000000227 ) ;
#16771=ORIENTED_EDGE ( 'NONE', *, *, #37714, .T. ) ;
#16773=AXIS2_PLACEMENT_3D ( 'NONE', #31538, #36084, #22998 ) ;
#16774=DIRECTION ( 'NONE',  ( 0.007781995580012663651, -3.146120232559066537E-19, -0.9999697198139514409 ) ) ;
#16775=ORIENTED_EDGE ( 'NONE', *, *, #15753, .F. ) ;
#16776=VECTOR ( 'NONE', #14390, 999.9999999999998863 ) ;
#16777=CARTESIAN_POINT ( 'NONE',  ( -24.26908309836554878, 0.000000000000000000, 6.108867788427308376 ) ) ;
#16778=LINE ( 'NONE', #16478, #2744 ) ;
#16779=VECTOR ( 'NONE', #51422, 1000.000000000000227 ) ;
#16780=DIRECTION ( 'NONE',  ( 0.007781995580012662783, 0.000000000000000000, -0.9999697198139514409 ) ) ;
#16781=CARTESIAN_POINT ( 'NONE',  ( -29.86352658060627618, 0.000000000000000000, 8.481329010720569883 ) ) ;
#16782=CARTESIAN_POINT ( 'NONE',  ( -14.22368343527709200, -0.3560938001956543975, 2.394921545183867462 ) ) ;
#16783=VERTEX_POINT ( 'NONE', #48688 ) ;
#16784=VECTOR ( 'NONE', #28105, 999.9999999999998863 ) ;
#16785=VECTOR ( 'NONE', #34787, 999.9999999999998863 ) ;
#16786=ORIENTED_EDGE ( 'NONE', *, *, #23774, .T. ) ;
#16787=PLANE ( 'NONE',  #507 ) ;
#16788=DIRECTION ( 'NONE',  ( -0.6427681459581293666, -0.7660444431189770143, -0.005002170337467561935 ) ) ;
#16789=ORIENTED_EDGE ( 'NONE', *, *, #50634, .T. ) ;
#16791=CARTESIAN_POINT ( 'NONE',  ( -9.110551994824897193, 0.000000000000000000, 3.538847790438064411 ) ) ;
#16792=ORIENTED_EDGE ( 'NONE', *, *, #7091, .F. ) ;
#16794=EDGE_CURVE ( 'NONE', #27421, #51703, #19113, .T. ) ;
#16795=VERTEX_POINT ( 'NONE', #18017 ) ;
#16796=CARTESIAN_POINT ( 'NONE',  ( 2.072287782118878319, 0.000000000000000000, -2.950529333540147015 ) ) ;
#16797=AXIS2_PLACEMENT_3D ( 'NONE', #41900, #24326, #46437 ) ;
#16798=ORIENTED_EDGE ( 'NONE', *, *, #39238, .T. ) ;
#16799=EDGE_LOOP ( 'NONE', ( #34320, #25133, #17466, #37687 ) ) ;
#16800=EDGE_LOOP ( 'NONE', ( #35353, #43363, #27233, #33173 ) ) ;
#16802=EDGE_CURVE ( 'NONE', #33384, #20003, #36440, .T. ) ;
#16803=CARTESIAN_POINT ( 'NONE',  ( -1.086233639165236964, 0.000000000000000000, -2.796443541562362078 ) ) ;
#16804=FACE_OUTER_BOUND ( 'NONE', #9413, .T. ) ;
#16805=VECTOR ( 'NONE', #52106, 1000.000000000000227 ) ;
#16806=LINE ( 'NONE', #18185, #46590 ) ;
#16807=ADVANCED_FACE ( 'NONE', ( #5796 ), #44675, .F. ) ;
#16808=EDGE_CURVE ( 'NONE', #33246, #10129, #5506, .T. ) ;
#16809=ADVANCED_FACE ( 'NONE', ( #5254 ), #22561, .F. ) ;
#16810=DIRECTION ( 'NONE',  ( -0.5364919789714478471, 0.6444004775717705469, -0.5449076811759709926 ) ) ;
#16811=ORIENTED_EDGE ( 'NONE', *, *, #14681, .T. ) ;
#16812=VECTOR ( 'NONE', #494, 1000.000000000000227 ) ;
#16813=ORIENTED_EDGE ( 'NONE', *, *, #25159, .T. ) ;
#16814=ORIENTED_EDGE ( 'NONE', *, *, #36324, .F. ) ;
#16815=AXIS2_PLACEMENT_3D ( 'NONE', #11716, #50032, #50335 ) ;
#16816=DIRECTION ( 'NONE',  ( -0.6427681459581293666, -0.7660444431189770143, -0.005002170337467561935 ) ) ;
#16817=VECTOR ( 'NONE', #17314, 999.9999999999998863 ) ;
#16818=CARTESIAN_POINT ( 'NONE',  ( -18.90896079192820167, -3.108426967578159061, 9.128272473059206860 ) ) ;
#16819=ORIENTED_EDGE ( 'NONE', *, *, #43113, .F. ) ;
#16820=LINE ( 'NONE', #20787, #28459 ) ;
#16821=ORIENTED_EDGE ( 'NONE', *, *, #47892, .F. ) ;
#16822=CARTESIAN_POINT ( 'NONE',  ( -8.609916609573598834, 0.000000000000000000, 10.23519010964256637 ) ) ;
#16823=CARTESIAN_POINT ( 'NONE',  ( -28.92982233430281980, 0.000000000000000000, 7.919257187036034651 ) ) ;
#16824=VECTOR ( 'NONE', #29188, 999.9999999999998863 ) ;
#16825=EDGE_LOOP ( 'NONE', ( #24672, #38196, #47473 ) ) ;
#16826=VECTOR ( 'NONE', #51464, 999.9999999999998863 ) ;
#16827=CARTESIAN_POINT ( 'NONE',  ( -18.15781053378047716, 0.000000000000000000, 8.941757669486225524 ) ) ;
#16828=EDGE_CURVE ( 'NONE', #30507, #29147, #14334, .T. ) ;
#16829=ORIENTED_EDGE ( 'NONE', *, *, #44562, .F. ) ;
#16830=AXIS2_PLACEMENT_3D ( 'NONE', #53211, #17412, #48076 ) ;
#16832=DIRECTION ( 'NONE',  ( -0.005961354470445682716, -0.6427876096865404731, 0.7660212471507180654 ) ) ;
#16833=VECTOR ( 'NONE', #28992, 1000.000000000000000 ) ;
#16835=EDGE_LOOP ( 'NONE', ( #9024, #48517, #11663, #31815 ) ) ;
#16836=CARTESIAN_POINT ( 'NONE',  ( -20.54204810873173415, 0.000000000000000000, 4.860550213503115558 ) ) ;
#16837=DIRECTION ( 'NONE',  ( 0.005961354470445682716, -0.6427876096865404731, -0.7660212471507180654 ) ) ;
#16838=EDGE_CURVE ( 'NONE', #40865, #22139, #19394, .T. ) ;
#16840=FACE_OUTER_BOUND ( 'NONE', #20001, .T. ) ;
#16841=ORIENTED_EDGE ( 'NONE', *, *, #49514, .T. ) ;
#16842=ADVANCED_FACE ( 'NONE', ( #11150 ), #36736, .F. ) ;
#16843=DIRECTION ( 'NONE',  ( -0.9999697198139514409, -0.000000000000000000, -0.007781995580013368816 ) ) ;
#16844=DIRECTION ( 'NONE',  ( 0.5364919789714477361, 0.6444004775717706579, 0.5449076811759711036 ) ) ;
#16845=DIRECTION ( 'NONE',  ( -0.9999697198139514409, -0.000000000000000000, -0.007781995580013368816 ) ) ;
#16846=LINE ( 'NONE', #13432, #35841 ) ;
#16847=ADVANCED_FACE ( 'NONE', ( #32198 ), #27948, .F. ) ;
#16848=CARTESIAN_POINT ( 'NONE',  ( -27.06630483948590893, -0.1191753592594197858, 7.295098399573937797 ) ) ;
#16849=VECTOR ( 'NONE', #24730, 999.9999999999998863 ) ;
#16850=DIRECTION ( 'NONE',  ( 0.9999697198139515519, 0.000000000000000000, 0.007781995580013368816 ) ) ;
#16851=ORIENTED_EDGE ( 'NONE', *, *, #22781, .F. ) ;
#16852=FACE_OUTER_BOUND ( 'NONE', #39372, .T. ) ;
#16853=VECTOR ( 'NONE', #25988, 1000.000000000000227 ) ;
#16854=DIRECTION ( 'NONE',  ( -0.005961354470445682716, -0.6427876096865404731, 0.7660212471507180654 ) ) ;
#16855=DIRECTION ( 'NONE',  ( 0.007781995580012662783, 0.000000000000000000, -0.9999697198139514409 ) ) ;
#16856=EDGE_LOOP ( 'NONE', ( #45716, #6337, #13410, #11155 ) ) ;
#16857=DIRECTION ( 'NONE',  ( 0.5364919789714477361, 0.6444004775717706579, 0.5449076811759711036 ) ) ;
#16858=VECTOR ( 'NONE', #35164, 1000.000000000000114 ) ;
#16859=ORIENTED_EDGE ( 'NONE', *, *, #8213, .T. ) ;
#16860=DIRECTION ( 'NONE',  ( 0.9999697198139515519, 0.000000000000000000, 0.007781995580013368816 ) ) ;
#16861=DIRECTION ( 'NONE',  ( 0.000000000000000000, -1.000000000000000000, 0.000000000000000000 ) ) ;
#16862=VECTOR ( 'NONE', #32137, 1000.000000000000000 ) ;
#16863=DIRECTION ( 'NONE',  ( -0.9999697198139514409, -0.000000000000000000, -0.007781995580013368816 ) ) ;
#16865=ORIENTED_EDGE ( 'NONE', *, *, #40650, .T. ) ;
#16866=VECTOR ( 'NONE', #47553, 999.9999999999998863 ) ;
#16867=ORIENTED_EDGE ( 'NONE', *, *, #48786, .F. ) ;
#16869=DIRECTION ( 'NONE',  ( -0.005961354470445682716, -0.6427876096865404731, 0.7660212471507180654 ) ) ;
#16870=PLANE ( 'NONE',  #22385 ) ;
#16871=VECTOR ( 'NONE', #39400, 1000.000000000000227 ) ;
#16872=VECTOR ( 'NONE', #23145, 1000.000000000000114 ) ;
#16873=LINE ( 'NONE', #11753, #7800 ) ;
#16874=VECTOR ( 'NONE', #46199, 999.9999999999998863 ) ;
#16875=DIRECTION ( 'NONE',  ( 0.000000000000000000, -1.000000000000000000, 0.000000000000000000 ) ) ;
#16877=ORIENTED_EDGE ( 'NONE', *, *, #47590, .F. ) ;
#16878=PLANE ( 'NONE',  #13848 ) ;
#16879=VECTOR ( 'NONE', #34140, 999.9999999999998863 ) ;
#16880=VECTOR ( 'NONE', #26022, 999.9999999999998863 ) ;
#16882=ORIENTED_EDGE ( 'NONE', *, *, #53498, .T. ) ;
#16883=LINE ( 'NONE', #51523, #52844 ) ;
#16884=CARTESIAN_POINT ( 'NONE',  ( -13.69706524180599239, 0.000000000000000000, 7.129811871761492448 ) ) ;
#16885=CARTESIAN_POINT ( 'NONE',  ( -16.86024456217533185, -0.1191753592594181482, 8.482520529993088587 ) ) ;
#16886=ADVANCED_FACE ( 'NONE', ( #46335 ), #23653, .F. ) ;
#16887=ADVANCED_FACE ( 'NONE', ( #6624 ), #23938, .F. ) ;
#16888=VERTEX_POINT ( 'NONE', #54883 ) ;
#16889=FACE_OUTER_BOUND ( 'NONE', #4395, .T. ) ;
#16890=VERTEX_POINT ( 'NONE', #3198 ) ;
#16891=EDGE_CURVE ( 'NONE', #34545, #30649, #24775, .T. ) ;
#16892=VECTOR ( 'NONE', #28369, 999.9999999999998863 ) ;
#16894=ORIENTED_EDGE ( 'NONE', *, *, #20352, .F. ) ;
#16895=ORIENTED_EDGE ( 'NONE', *, *, #48519, .T. ) ;
#16896=DIRECTION ( 'NONE',  ( -0.9999697198139514409, -0.000000000000000000, -0.007781995580013368816 ) ) ;
#16897=VECTOR ( 'NONE', #15183, 1000.000000000000227 ) ;
#16898=EDGE_LOOP ( 'NONE', ( #25592, #26639, #40530, #14760 ) ) ;
#16899=FACE_OUTER_BOUND ( 'NONE', #25909, .T. ) ;
#16900=EDGE_LOOP ( 'NONE', ( #15528, #16951, #8917, #29636 ) ) ;
#16901=CARTESIAN_POINT ( 'NONE',  ( -18.55978481983513717, -0.5179957512181551094, 4.741301724224929792 ) ) ;
#16902=ORIENTED_EDGE ( 'NONE', *, *, #38532, .F. ) ;
#16903=EDGE_LOOP ( 'NONE', ( #18454, #41622, #35195, #27715 ) ) ;
#16904=EDGE_CURVE ( 'NONE', #21366, #37937, #20532, .T. ) ;
#16905=VECTOR ( 'NONE', #20391, 1000.000000000000114 ) ;
#16906=CARTESIAN_POINT ( 'NONE',  ( -14.11415985828438480, 2.714935509636508204, 6.819411824594130422 ) ) ;
#16907=LINE ( 'NONE', #8668, #8730 ) ;
#16908=DIRECTION ( 'NONE',  ( 0.5449076811759707706, 0.6444004775717708799, -0.5364919789714476250 ) ) ;
#16910=FACE_OUTER_BOUND ( 'NONE', #12881, .T. ) ;
#16911=ORIENTED_EDGE ( 'NONE', *, *, #15105, .T. ) ;
#16912=AXIS2_PLACEMENT_3D ( 'NONE', #32380, #49687, #10781 ) ;
#16913=ADVANCED_FACE ( 'NONE', ( #19951 ), #15683, .F. ) ;
#16914=ORIENTED_EDGE ( 'NONE', *, *, #21281, .F. ) ;
#16915=VECTOR ( 'NONE', #8953, 1000.000000000000227 ) ;
#16916=DIRECTION ( 'NONE',  ( 0.000000000000000000, -1.000000000000000000, 0.000000000000000000 ) ) ;
#16917=DIRECTION ( 'NONE',  ( -0.7660212471507179544, -0.6427876096865405842, -0.005961354470445141482 ) ) ;
#16918=EDGE_CURVE ( 'NONE', #6267, #34530, #10638, .T. ) ;
#16919=VECTOR ( 'NONE', #5089, 1000.000000000000000 ) ;
#16920=LINE ( 'NONE', #29964, #27904 ) ;
#16921=VECTOR ( 'NONE', #55748, 999.9999999999998863 ) ;
#16922=DIRECTION ( 'NONE',  ( 0.000000000000000000, -1.000000000000000000, 0.000000000000000000 ) ) ;
#16923=ADVANCED_FACE ( 'NONE', ( #46081 ), #7187, .F. ) ;
#16924=CARTESIAN_POINT ( 'NONE',  ( -16.77330902089484610, 0.9340140483890038148, 3.167454640934507459 ) ) ;
#16925=DIRECTION ( 'NONE',  ( -0.005961354470445682716, -0.6427876096865404731, 0.7660212471507180654 ) ) ;
#16926=ORIENTED_EDGE ( 'NONE', *, *, #44490, .F. ) ;
#16927=CARTESIAN_POINT ( 'NONE',  ( -18.81669326757378613, 0.000000000000000000, 8.197965952086681440 ) ) ;
#16928=EDGE_CURVE ( 'NONE', #41874, #35555, #33323, .T. ) ;
#16929=DIRECTION ( 'NONE',  ( -0.005961354470445682716, -0.6427876096865404731, 0.7660212471507180654 ) ) ;
#16930=ORIENTED_EDGE ( 'NONE', *, *, #14649, .F. ) ;
#16931=CARTESIAN_POINT ( 'NONE',  ( -11.20636620717317378, 0.000000000000000000, 11.32298014792380414 ) ) ;
#16932=LINE ( 'NONE', #18036, #36933 ) ;
#16933=ADVANCED_FACE ( 'NONE', ( #32484 ), #45248, .F. ) ;
#16934=FACE_OUTER_BOUND ( 'NONE', #10351, .T. ) ;
#16935=LINE ( 'NONE', #3304, #27751 ) ;
#16936=VECTOR ( 'NONE', #34628, 999.9999999999998863 ) ;
#16937=ORIENTED_EDGE ( 'NONE', *, *, #5168, .F. ) ;
#16938=ORIENTED_EDGE ( 'NONE', *, *, #31704, .F. ) ;
#16939=LINE ( 'NONE', #12668, #25747 ) ;
#16940=CARTESIAN_POINT ( 'NONE',  ( -16.43317633868556626, -0.1191753592594197858, 13.31363028683540151 ) ) ;
#16941=CARTESIAN_POINT ( 'NONE',  ( -19.60990026154428278, 0.000000000000000000, 4.498472333781370125 ) ) ;
#16943=VECTOR ( 'NONE', #18055, 1000.000000000000227 ) ;
#16944=CARTESIAN_POINT ( 'NONE',  ( -10.66745676860673342, 0.000000000000000000, 1.782733951914063031 ) ) ;
#16945=DIRECTION ( 'NONE',  ( -0.9999697198139514409, -0.000000000000000000, -0.007781995580013368816 ) ) ;
#16946=DIRECTION ( 'NONE',  ( 0.9999697198139515519, 0.000000000000000000, 0.007781995580013368816 ) ) ;
#16947=DIRECTION ( 'NONE',  ( 0.9999697198139515519, 0.000000000000000000, 0.007781995580013368816 ) ) ;
#16948=VECTOR ( 'NONE', #47078, 1000.000000000000000 ) ;
#16950=DIRECTION ( 'NONE',  ( 0.000000000000000000, -0.000000000000000000, -1.000000000000000000 ) ) ;
#16951=ORIENTED_EDGE ( 'NONE', *, *, #55608, .F. ) ;
#16952=FACE_OUTER_BOUND ( 'NONE', #10846, .T. ) ;
#16953=EDGE_CURVE ( 'NONE', #36994, #30666, #50342, .T. ) ;
#16954=VERTEX_POINT ( 'NONE', #50038 ) ;
#16955=VECTOR ( 'NONE', #18944, 1000.000000000000227 ) ;
#16956=EDGE_LOOP ( 'NONE', ( #54643, #38300, #6590, #48856 ) ) ;
#16957=EDGE_CURVE ( 'NONE', #49949, #40825, #10880, .T. ) ;
#16958=EDGE_CURVE ( 'NONE', #40111, #21299, #11454, .T. ) ;
#16959=VERTEX_POINT ( 'NONE', #24235 ) ;
#16960=AXIS2_PLACEMENT_3D ( 'NONE', #3077, #10787, #6799 ) ;
#16961=ORIENTED_EDGE ( 'NONE', *, *, #29239, .F. ) ;
#16962=VERTEX_POINT ( 'NONE', #41546 ) ;
#16963=ORIENTED_EDGE ( 'NONE', *, *, #46221, .F. ) ;
#16964=DIRECTION ( 'NONE',  ( -0.3620778797217457656, 0.000000000000000000, -0.9321478471874539151 ) ) ;
#16965=DIRECTION ( 'NONE',  ( 0.000000000000000000, -1.000000000000000000, 0.000000000000000000 ) ) ;
#16966=FACE_OUTER_BOUND ( 'NONE', #28438, .T. ) ;
#16967=EDGE_LOOP ( 'NONE', ( #52498, #1774, #23310, #36248 ) ) ;
#16968=CARTESIAN_POINT ( 'NONE',  ( -23.33693525117809386, 0.000000000000000000, 5.746789908705562944 ) ) ;
#16969=VERTEX_POINT ( 'NONE', #47191 ) ;
#16972=AXIS2_PLACEMENT_3D ( 'NONE', #27571, #45429, #11368 ) ;
#16973=ADVANCED_FACE ( 'NONE', ( #38396 ), #21070, .F. ) ;
#16974=FACE_OUTER_BOUND ( 'NONE', #38511, .T. ) ;
#16975=CARTESIAN_POINT ( 'NONE',  ( -11.40636015113596180, 0.000000000000000000, 11.32142374880780089 ) ) ;
#16977=ORIENTED_EDGE ( 'NONE', *, *, #18097, .T. ) ;
#16978=DIRECTION ( 'NONE',  ( 0.5449076811759707706, 0.6444004775717708799, -0.5364919789714476250 ) ) ;
#16979=ORIENTED_EDGE ( 'NONE', *, *, #12047, .F. ) ;
#16980=LINE ( 'NONE', #34556, #30954 ) ;
#16982=DIRECTION ( 'NONE',  ( -0.9999697198139514409, -0.000000000000000000, -0.007781995580013368816 ) ) ;
#16983=EDGE_CURVE ( 'NONE', #8639, #21780, #33861, .T. ) ;
#16984=CARTESIAN_POINT ( 'NONE',  ( -29.86274838104827367, -0.1191753592594197858, 8.381332038739175871 ) ) ;
#16985=VECTOR ( 'NONE', #11742, 999.9999999999998863 ) ;
#16986=DIRECTION ( 'NONE',  ( 0.007781995580012662783, 0.000000000000000000, -0.9999697198139514409 ) ) ;
#16987=LINE ( 'NONE', #34306, #30218 ) ;
#16988=FACE_OUTER_BOUND ( 'NONE', #469, .T. ) ;
#16989=LINE ( 'NONE', #9285, #17577 ) ;
#16990=PLANE ( 'NONE',  #44040 ) ;
#16991=ORIENTED_EDGE ( 'NONE', *, *, #17543, .T. ) ;
#16992=DIRECTION ( 'NONE',  ( 0.007781995580012663651, -3.146120232559066537E-19, -0.9999697198139514409 ) ) ;
#16993=ORIENTED_EDGE ( 'NONE', *, *, #45263, .F. ) ;
#16994=VECTOR ( 'NONE', #17448, 1000.000000000000114 ) ;
#16995=CARTESIAN_POINT ( 'NONE',  ( -18.67775241435682432, 0.000000000000000000, 4.136394454059623804 ) ) ;
#16996=LINE ( 'NONE', #55587, #25097 ) ;
#16997=PLANE ( 'NONE',  #899 ) ;
#16998=ADVANCED_FACE ( 'NONE', ( #34167 ), #17366, .T. ) ;
#16999=CARTESIAN_POINT ( 'NONE',  ( -8.409922665610809034, 0.000000000000000000, 10.23674650875856962 ) ) ;
#17000=LINE ( 'NONE', #3635, #50380 ) ;
#17001=LINE ( 'NONE', #47083, #302 ) ;
#17004=LINE ( 'NONE', #34322, #32168 ) ;
#17005=DIRECTION ( 'NONE',  ( -0.9999697198139514409, -0.000000000000000000, -0.007781995580013368816 ) ) ;
#17006=ADVANCED_FACE ( 'NONE', ( #38967 ), #43498, .F. ) ;
#17007=CARTESIAN_POINT ( 'NONE',  ( -21.47341775636118655, -0.1191753592594197858, 5.122631121243466090 ) ) ;
#17008=CARTESIAN_POINT ( 'NONE',  ( -19.53245895536257493, 1.419719901456505395, 6.798393728507462264 ) ) ;
#17009=EDGE_CURVE ( 'NONE', #40102, #22884, #29891, .T. ) ;
#17010=DIRECTION ( 'NONE',  ( 0.000000000000000000, -1.000000000000000000, 0.000000000000000000 ) ) ;
#17011=EDGE_CURVE ( 'NONE', #32502, #29020, #29629, .T. ) ;
#17012=LINE ( 'NONE', #15869, #4777 ) ;
#17013=EDGE_LOOP ( 'NONE', ( #7057, #37089, #46037, #31980 ) ) ;
#17014=FACE_OUTER_BOUND ( 'NONE', #19911, .T. ) ;
#17016=ORIENTED_EDGE ( 'NONE', *, *, #25891, .T. ) ;
#17017=EDGE_LOOP ( 'NONE', ( #44924, #31716, #3940, #20288 ) ) ;
#17018=DIRECTION ( 'NONE',  ( -0.005002170337468016433, -0.7660444431189770143, 0.6427681459581293666 ) ) ;
#17019=EDGE_CURVE ( 'NONE', #20837, #29012, #25615, .T. ) ;
#17020=EDGE_LOOP ( 'NONE', ( #48071, #11439, #39452, #4647 ) ) ;
#17021=EDGE_CURVE ( 'NONE', #26517, #2943, #29321, .T. ) ;
#17022=EDGE_CURVE ( 'NONE', #8862, #3167, #4045, .T. ) ;
#17023=VECTOR ( 'NONE', #51827, 1000.000000000000227 ) ;
#17025=ORIENTED_EDGE ( 'NONE', *, *, #5637, .F. ) ;
#17026=VERTEX_POINT ( 'NONE', #47479 ) ;
#17027=CARTESIAN_POINT ( 'NONE',  ( -19.60834386242827776, 0.000000000000000000, 4.298478389818581213 ) ) ;
#17028=ORIENTED_EDGE ( 'NONE', *, *, #8471, .F. ) ;
#17029=PLANE ( 'NONE',  #13320 ) ;
#17030=PLANE ( 'NONE',  #40327 ) ;
#17031=ADVANCED_FACE ( 'NONE', ( #4346 ), #8592, .F. ) ;
#17032=VECTOR ( 'NONE', #41558, 1000.000000000000227 ) ;
#17033=ORIENTED_EDGE ( 'NONE', *, *, #30026, .T. ) ;
#17034=ORIENTED_EDGE ( 'NONE', *, *, #27090, .F. ) ;
#17035=EDGE_CURVE ( 'NONE', #3617, #4870, #43251, .T. ) ;
#17036=DIRECTION ( 'NONE',  ( 0.000000000000000000, -1.000000000000000000, 0.000000000000000000 ) ) ;
#17037=CARTESIAN_POINT ( 'NONE',  ( -22.40556560354864146, -0.1191753592594197858, 5.484709000965211523 ) ) ;
#17038=EDGE_LOOP ( 'NONE', ( #39636, #16309, #28690, #26348 ) ) ;
#17039=DIRECTION ( 'NONE',  ( 0.5364919789714477361, 0.6444004775717706579, 0.5449076811759711036 ) ) ;
#17040=CARTESIAN_POINT ( 'NONE',  ( -15.96710241509184058, -0.1191753592594218814, 13.13259134697452879 ) ) ;
#17041=VERTEX_POINT ( 'NONE', #21657 ) ;
#17042=LINE ( 'NONE', #25277, #36575 ) ;
#17043=ORIENTED_EDGE ( 'NONE', *, *, #31297, .T. ) ;
#17044=LINE ( 'NONE', #29548, #34569 ) ;
#17045=DIRECTION ( 'NONE',  ( -0.5364919789714478471, 0.6444004775717705469, -0.5449076811759709926 ) ) ;
#17046=ORIENTED_EDGE ( 'NONE', *, *, #26619, .F. ) ;
#17047=DIRECTION ( 'NONE',  ( 0.7660212471507180654, -0.6427876096865404731, 0.005961354470445141482 ) ) ;
#17048=CARTESIAN_POINT ( 'NONE',  ( -14.03506048556014285, -0.1191753592594184813, 3.703189858250206079 ) ) ;
#17049=PLANE ( 'NONE',  #14877 ) ;
#17050=LINE ( 'NONE', #26673, #6558 ) ;
#17051=ORIENTED_EDGE ( 'NONE', *, *, #831, .F. ) ;
#17052=FACE_OUTER_BOUND ( 'NONE', #50109, .T. ) ;
#17053=DIRECTION ( 'NONE',  ( 0.007781995580012663651, 0.000000000000000000, -0.9999697198139515519 ) ) ;
#17054=LINE ( 'NONE', #8525, #24909 ) ;
#17055=DIRECTION ( 'NONE',  ( 0.7660212471507180654, -0.6427876096865404731, 0.005961354470445141482 ) ) ;
#17056=EDGE_CURVE ( 'NONE', #52307, #18978, #34696, .T. ) ;
#17057=CARTESIAN_POINT ( 'NONE',  ( -24.26908309836554878, 0.000000000000000000, 6.108867788427308376 ) ) ;
#17058=DIRECTION ( 'NONE',  ( -0.5449076811759708816, 0.6444004775717707689, 0.5364919789714475140 ) ) ;
#17059=LINE ( 'NONE', #3432, #728 ) ;
#17060=DIRECTION ( 'NONE',  ( -0.7660212471507179544, -0.6427876096865405842, -0.005961354470445141482 ) ) ;
#17061=CARTESIAN_POINT ( 'NONE',  ( -19.37931499696963300, 2.876837460659007473, 9.130285569831087855 ) ) ;
#17062=ORIENTED_EDGE ( 'NONE', *, *, #48105, .T. ) ;
#17064=DIRECTION ( 'NONE',  ( 0.9999697198139515519, 0.000000000000000000, 0.007781995580013368816 ) ) ;
#17065=VERTEX_POINT ( 'NONE', #8890 ) ;
#17066=PLANE ( 'NONE',  #5720 ) ;
#17067=DIRECTION ( 'NONE',  ( 0.007781995580012663651, -3.146120232559066537E-19, -0.9999697198139514409 ) ) ;
#17068=ADVANCED_FACE ( 'NONE', ( #25348 ), #26193, .F. ) ;
#17069=VECTOR ( 'NONE', #55372, 1000.000000000000114 ) ;
#17070=LINE ( 'NONE', #11681, #14995 ) ;
#17071=CARTESIAN_POINT ( 'NONE',  ( -14.99020076078985397, -0.1191753592594185784, 7.019745364034069013 ) ) ;
#17073=CARTESIAN_POINT ( 'NONE',  ( -14.95190377862070541, 3.200641362704010007, 2.387641711229373520 ) ) ;
#17074=EDGE_LOOP ( 'NONE', ( #483, #3367, #45490, #40702 ) ) ;
#17075=ORIENTED_EDGE ( 'NONE', *, *, #32631, .F. ) ;
#17076=CARTESIAN_POINT ( 'NONE',  ( -14.40754437137767674, 0.000000000000000000, 4.708284283832102624 ) ) ;
#17077=DIRECTION ( 'NONE',  ( 0.005002170337468016433, -0.7660444431189770143, -0.6427681459581293666 ) ) ;
#17078=ORIENTED_EDGE ( 'NONE', *, *, #49399, .F. ) ;
#17079=DIRECTION ( 'NONE',  ( -0.005961354470445682716, -0.6427876096865404731, 0.7660212471507180654 ) ) ;
#17080=ORIENTED_EDGE ( 'NONE', *, *, #3982, .T. ) ;
#17081=ADVANCED_FACE ( 'NONE', ( #38115 ), #16529, .F. ) ;
#17082=FACE_OUTER_BOUND ( 'NONE', #51921, .T. ) ;
#17083=EDGE_LOOP ( 'NONE', ( #11630, #41098, #27720, #28015, #2962 ) ) ;
#17084=PLANE ( 'NONE',  #21141 ) ;
#17085=ADVANCED_FACE ( 'NONE', ( #53426 ), #1163, .F. ) ;
#17086=ORIENTED_EDGE ( 'NONE', *, *, #10390, .F. ) ;
#17087=ORIENTED_EDGE ( 'NONE', *, *, #28862, .F. ) ;
#17088=ORIENTED_EDGE ( 'NONE', *, *, #11490, .F. ) ;
#17089=DIRECTION ( 'NONE',  ( 0.9321478471874541372, 0.000000000000000000, -0.3620778797217453771 ) ) ;
#17090=LINE ( 'NONE', #3460, #25967 ) ;
#17091=LINE ( 'NONE', #55404, #14873 ) ;
#17092=ADVANCED_FACE ( 'NONE', ( #22499 ), #39544, .F. ) ;
#17094=VERTEX_POINT ( 'NONE', #52848 ) ;
#17095=ORIENTED_EDGE ( 'NONE', *, *, #38262, .T. ) ;
#17096=ADVANCED_FACE ( 'NONE', ( #39809 ), #35535, .F. ) ;
#17097=ORIENTED_EDGE ( 'NONE', *, *, #15076, .T. ) ;
#17098=PLANE ( 'NONE',  #29464 ) ;
#17099=EDGE_LOOP ( 'NONE', ( #37875, #16332, #16424, #35534 ) ) ;
#17100=DIRECTION ( 'NONE',  ( -0.5364919789714478471, 0.6444004775717705469, -0.5449076811759709926 ) ) ;
#17101=ORIENTED_EDGE ( 'NONE', *, *, #2500, .T. ) ;
#17102=FACE_OUTER_BOUND ( 'NONE', #17414, .T. ) ;
#17103=DIRECTION ( 'NONE',  ( 0.005002170337468016433, -0.7660444431189770143, -0.6427681459581293666 ) ) ;
#17104=AXIS2_PLACEMENT_3D ( 'NONE', #33047, #24257, #2915 ) ;
#17105=VERTEX_POINT ( 'NONE', #35277 ) ;
#17106=FACE_OUTER_BOUND ( 'NONE', #35370, .T. ) ;
#17107=VERTEX_POINT ( 'NONE', #23046 ) ;
#17110=VERTEX_POINT ( 'NONE', #31581 ) ;
#17111=CARTESIAN_POINT ( 'NONE',  ( -19.38983669476062843, -1.489407457353155717, 6.657974164829091990 ) ) ;
#17112=DIRECTION ( 'NONE',  ( -0.005961354470445682716, -0.6427876096865404731, 0.7660212471507180654 ) ) ;
#17113=DIRECTION ( 'NONE',  ( 0.007781995580012663651, 0.000000000000000000, -0.9999697198139515519 ) ) ;
#17114=ORIENTED_EDGE ( 'NONE', *, *, #39639, .T. ) ;
#17115=CARTESIAN_POINT ( 'NONE',  ( -31.72704407542318350, -0.1191753592594197858, 9.105487798182664960 ) ) ;
#17116=DIRECTION ( 'NONE',  ( 0.007781995580012663651, -3.146120232559066537E-19, -0.9999697198139514409 ) ) ;
#17117=EDGE_CURVE ( 'NONE', #43329, #16440, #1465, .T. ) ;
#17118=CARTESIAN_POINT ( 'NONE',  ( -20.54126990917373519, -0.1191753592594197858, 4.760553241521720658 ) ) ;
#17119=LINE ( 'NONE', #51741, #14075 ) ;
#17120=CARTESIAN_POINT ( 'NONE',  ( -14.93495759592298988, 0.000000000000000000, 12.77129166681078409 ) ) ;
#17121=ADVANCED_FACE ( 'NONE', ( #27292 ), #44068, .F. ) ;
#17123=ORIENTED_EDGE ( 'NONE', *, *, #52767, .F. ) ;
#17124=CARTESIAN_POINT ( 'NONE',  ( -14.53706007796989930, -0.1191753592594181482, 8.500600088833135004 ) ) ;
#17125=EDGE_CURVE ( 'NONE', #32968, #7585, #9983, .T. ) ;
#17126=LINE ( 'NONE', #55739, #20427 ) ;
#17127=LINE ( 'NONE', #37877, #52237 ) ;
#17128=ORIENTED_EDGE ( 'NONE', *, *, #45225, .T. ) ;
#17129=PLANE ( 'NONE',  #31133 ) ;
#17130=PLANE ( 'NONE',  #17749 ) ;
#17131=ORIENTED_EDGE ( 'NONE', *, *, #30902, .T. ) ;
#17132=EDGE_CURVE ( 'NONE', #53826, #38778, #52319, .T. ) ;
#17133=EDGE_CURVE ( 'NONE', #43303, #6876, #31283, .T. ) ;
#17134=EDGE_CURVE ( 'NONE', #35736, #5331, #9136, .T. ) ;
#17135=FACE_OUTER_BOUND ( 'NONE', #42386, .T. ) ;
#17136=CARTESIAN_POINT ( 'NONE',  ( -13.00742402505039585, 1.419719901456506728, 4.263848570455246012 ) ) ;
#17137=DIRECTION ( 'NONE',  ( 0.7660212471507180654, -0.6427876096865404731, 0.005961354470445141482 ) ) ;
#17139=ORIENTED_EDGE ( 'NONE', *, *, #21151, .F. ) ;
#17140=ORIENTED_EDGE ( 'NONE', *, *, #130, .T. ) ;
#17141=PLANE ( 'NONE',  #49373 ) ;
#17142=CARTESIAN_POINT ( 'NONE',  ( -13.09716453136212166, -0.1191753592594190225, 2.602492572012935046 ) ) ;
#17143=DIRECTION ( 'NONE',  ( 0.9999697198139515519, 0.000000000000000000, 0.007781995580013368816 ) ) ;
#17144=PLANE ( 'NONE',  #3006 ) ;
#17145=LINE ( 'NONE', #51218, #51868 ) ;
#17146=EDGE_CURVE ( 'NONE', #17736, #17689, #48889, .T. ) ;
#17147=CARTESIAN_POINT ( 'NONE',  ( -10.94028622754223967, 0.000000000000000000, 11.14038480894692995 ) ) ;
#17148=ORIENTED_EDGE ( 'NONE', *, *, #4393, .F. ) ;
#17149=DIRECTION ( 'NONE',  ( -0.5364919789714478471, 0.6444004775717705469, -0.5449076811759709926 ) ) ;
#17150=EDGE_CURVE ( 'NONE', #11098, #16694, #27033, .T. ) ;
#17151=CARTESIAN_POINT ( 'NONE',  ( -10.84028925556084388, -0.1191753592594197858, 11.14116300850493246 ) ) ;
#17152=ORIENTED_EDGE ( 'NONE', *, *, #6415, .T. ) ;
#17153=EDGE_CURVE ( 'NONE', #10765, #3186, #26741, .T. ) ;
#17154=CARTESIAN_POINT ( 'NONE',  ( -27.99923088623136636, 0.000000000000000000, 7.757173251277078130 ) ) ;
#17155=CARTESIAN_POINT ( 'NONE',  ( -19.15367902479211537, 2.067327705546507133, 7.714097475855159480 ) ) ;
#17156=CARTESIAN_POINT ( 'NONE',  ( -29.86352658060627618, 0.000000000000000000, 8.481329010720569883 ) ) ;
#17157=ORIENTED_EDGE ( 'NONE', *, *, #26454, .T. ) ;
#17158=EDGE_CURVE ( 'NONE', #20365, #41108, #43767, .T. ) ;
#17160=ORIENTED_EDGE ( 'NONE', *, *, #25010, .F. ) ;
#17161=ORIENTED_EDGE ( 'NONE', *, *, #16808, .T. ) ;
#17162=ORIENTED_EDGE ( 'NONE', *, *, #11282, .T. ) ;
#17163=ORIENTED_EDGE ( 'NONE', *, *, #15376, .F. ) ;
#17164=DIRECTION ( 'NONE',  ( -0.5449076811759708816, 0.6444004775717707689, 0.5364919789714475140 ) ) ;
#17165=ORIENTED_EDGE ( 'NONE', *, *, #29211, .F. ) ;
#17167=ORIENTED_EDGE ( 'NONE', *, *, #26055, .T. ) ;
#17168=CARTESIAN_POINT ( 'NONE',  ( -19.46808184255099405, 2.760183692663749078, 7.523411736767075197 ) ) ;
#17169=ORIENTED_EDGE ( 'NONE', *, *, #27155, .F. ) ;
#17170=CARTESIAN_POINT ( 'NONE',  ( -17.33350361953226582, -0.1191753592594149563, 9.586833727998367749 ) ) ;
#17171=ORIENTED_EDGE ( 'NONE', *, *, #9315, .F. ) ;
#17172=LINE ( 'NONE', #42459, #24780 ) ;
#17173=LINE ( 'NONE', #30538, #32318 ) ;
#17174=DIRECTION ( 'NONE',  ( 0.9321478471874541372, 0.000000000000000000, -0.3620778797217453771 ) ) ;
#17175=LINE ( 'NONE', #25155, #55905 ) ;
#17176=DIRECTION ( 'NONE',  ( 0.6427681459581294776, -0.7660444431189769032, 0.005002170337467562802 ) ) ;
#17177=VERTEX_POINT ( 'NONE', #18802 ) ;
#17178=ORIENTED_EDGE ( 'NONE', *, *, #30109, .F. ) ;
#17179=CARTESIAN_POINT ( 'NONE',  ( -15.35274483170226389, 0.000000000000000000, 6.747594920547692610 ) ) ;
#17180=LINE ( 'NONE', #51806, #45689 ) ;
#17181=DIRECTION ( 'NONE',  ( -0.5364919789714478471, 0.6444004775717705469, -0.5449076811759709926 ) ) ;
#17182=CARTESIAN_POINT ( 'NONE',  ( -16.18826075967313116, -2.137015261443160341, 3.101209376544761920 ) ) ;
#17183=FACE_OUTER_BOUND ( 'NONE', #23619, .T. ) ;
#17184=LINE ( 'NONE', #3564, #44990 ) ;
#17185=EDGE_LOOP ( 'NONE', ( #29118, #14773, #10695, #2773 ) ) ;
#17186=DIRECTION ( 'NONE',  ( 0.000000000000000000, -1.000000000000000000, 0.000000000000000000 ) ) ;
#17187=CARTESIAN_POINT ( 'NONE',  ( -16.02887188652727701, 0.000000000000000000, 8.219661422694739983 ) ) ;
#17188=VERTEX_POINT ( 'NONE', #39235 ) ;
#17189=ADVANCED_FACE ( 'NONE', ( #4882 ), #632, .F. ) ;
#17190=EDGE_CURVE ( 'NONE', #53080, #1201, #35009, .T. ) ;
#17191=CARTESIAN_POINT ( 'NONE',  ( -19.63369567569543150, -0.1191753592594164690, 6.614276543096206495 ) ) ;
#17192=CARTESIAN_POINT ( 'NONE',  ( -20.86483076077407617, 3.524445264749008100, 10.77014507662227594 ) ) ;
#17193=PLANE ( 'NONE',  #19578 ) ;
#17194=EDGE_CURVE ( 'NONE', #18056, #30132, #30984, .T. ) ;
#17195=DIRECTION ( 'NONE',  ( 0.7660212471507180654, -0.6427876096865404731, 0.005961354470445141482 ) ) ;
#17196=ORIENTED_EDGE ( 'NONE', *, *, #18757, .T. ) ;
#17197=ORIENTED_EDGE ( 'NONE', *, *, #45354, .F. ) ;
#17198=CARTESIAN_POINT ( 'NONE',  ( -22.40478740399063895, 0.000000000000000000, 5.384712028983816623 ) ) ;
#17199=DIRECTION ( 'NONE',  ( 0.000000000000000000, -0.000000000000000000, -1.000000000000000000 ) ) ;
#17200=CARTESIAN_POINT ( 'NONE',  ( -13.73672976910459909, 0.000000000000000000, 12.22661844811216270 ) ) ;
#17201=DIRECTION ( 'NONE',  ( 0.9999697198139515519, 0.000000000000000000, 0.007781995580013368816 ) ) ;
#17202=CARTESIAN_POINT ( 'NONE',  ( -15.78864119349052153, 0.000000000000000000, 3.050881976202041379 ) ) ;
#17203=FACE_OUTER_BOUND ( 'NONE', #52947, .T. ) ;
#17204=DIRECTION ( 'NONE',  ( 0.6427681459581294776, -0.7660444431189769032, 0.005002170337467562802 ) ) ;
#17205=ORIENTED_EDGE ( 'NONE', *, *, #33159, .F. ) ;
#17206=EDGE_CURVE ( 'NONE', #1154, #621, #23338, .T. ) ;
#17207=FACE_OUTER_BOUND ( 'NONE', #12490, .T. ) ;
#17208=CARTESIAN_POINT ( 'NONE',  ( -12.70458494993575194, -0.1191753592594197858, 11.86531876794841978 ) ) ;
#17210=VERTEX_POINT ( 'NONE', #15917 ) ;
#17211=PLANE ( 'NONE',  #29214 ) ;
#17212=ORIENTED_EDGE ( 'NONE', *, *, #7002, .F. ) ;
#17213=DIRECTION ( 'NONE',  ( -0.6246952433987893460, -0.7422098413412802076, 0.2426528472758542054 ) ) ;
#17214=EDGE_LOOP ( 'NONE', ( #31026, #11694, #21675, #47883 ) ) ;
#17215=EDGE_CURVE ( 'NONE', #27257, #1128, #37206, .T. ) ;
#17216=ORIENTED_EDGE ( 'NONE', *, *, #11525, .T. ) ;
#17217=ADVANCED_FACE ( 'NONE', ( #1727 ), #24425, .F. ) ;
#17218=ORIENTED_EDGE ( 'NONE', *, *, #36040, .F. ) ;
#17219=VERTEX_POINT ( 'NONE', #32667 ) ;
#17220=EDGE_LOOP ( 'NONE', ( #8536, #12041, #47368, #25104 ) ) ;
#17221=ORIENTED_EDGE ( 'NONE', *, *, #4792, .T. ) ;
#17222=CARTESIAN_POINT ( 'NONE',  ( -13.07991603883496623, 3.686347215771509145, 8.011928505754800867 ) ) ;
#17223=CARTESIAN_POINT ( 'NONE',  ( -27.06552663992790997, 0.000000000000000000, 7.195101427592543786 ) ) ;
#17224=LINE ( 'NONE', #9260, #13131 ) ;
#17225=ORIENTED_EDGE ( 'NONE', *, *, #14231, .F. ) ;
#17226=CARTESIAN_POINT ( 'NONE',  ( -16.73803336170967526, 0.000000000000000000, 5.628818075470372939 ) ) ;
#17228=DIRECTION ( 'NONE',  ( -0.5449076811759708816, 0.6444004775717707689, 0.5364919789714475140 ) ) ;
#17229=EDGE_LOOP ( 'NONE', ( #1816, #28618, #34649, #18930 ) ) ;
#17230=PLANE ( 'NONE',  #34857 ) ;
#17232=ORIENTED_EDGE ( 'NONE', *, *, #7300, .T. ) ;
#17233=DIRECTION ( 'NONE',  ( 0.6427681459581294776, -0.7660444431189769032, 0.005002170337467562802 ) ) ;
#17234=ORIENTED_EDGE ( 'NONE', *, *, #54597, .T. ) ;
#17235=FACE_OUTER_BOUND ( 'NONE', #4278, .T. ) ;
#17236=CARTESIAN_POINT ( 'NONE',  ( -14.66887761629205222, 0.000000000000000000, 12.58869632783390990 ) ) ;
#17237=AXIS2_PLACEMENT_3D ( 'NONE', #1835, #23173, #10389 ) ;
#17238=FACE_OUTER_BOUND ( 'NONE', #32102, .T. ) ;
#17239=CARTESIAN_POINT ( 'NONE',  ( -17.41547807092396027, 0.000000000000000000, 7.270200336912393091 ) ) ;
#17240=FACE_OUTER_BOUND ( 'NONE', #35291, .T. ) ;
#17241=FACE_OUTER_BOUND ( 'NONE', #23449, .T. ) ;
#17242=CARTESIAN_POINT ( 'NONE',  ( -25.20278734466900517, 0.000000000000000000, 6.670939612111840944 ) ) ;
#17244=ORIENTED_EDGE ( 'NONE', *, *, #12744, .T. ) ;
#17245=LINE ( 'NONE', #30323, #9313 ) ;
#17246=VERTEX_POINT ( 'NONE', #53684 ) ;
#17247=EDGE_CURVE ( 'NONE', #1327, #42332, #28130, .T. ) ;
#17248=FACE_OUTER_BOUND ( 'NONE', #1633, .T. ) ;
#17249=LINE ( 'NONE', #48478, #1494 ) ;
#17250=CARTESIAN_POINT ( 'NONE',  ( -20.16176772743538237, -0.1191753592594197858, 14.76194180572237968 ) ) ;
#17251=CARTESIAN_POINT ( 'NONE',  ( -20.18605513093877946, 0.000000000000000000, 5.032646646757750197 ) ) ;
#17252=FACE_OUTER_BOUND ( 'NONE', #39795, .T. ) ;
#17253=ADVANCED_FACE ( 'NONE', ( #2290 ), #54510, .F. ) ;
#17254=ADVANCED_FACE ( 'NONE', ( #32953 ), #2825, .F. ) ;
#17255=PLANE ( 'NONE',  #10525 ) ;
#17257=ORIENTED_EDGE ( 'NONE', *, *, #51503, .T. ) ;
#17258=DIRECTION ( 'NONE',  ( 0.007781995580012663651, 0.000000000000000000, -0.9999697198139515519 ) ) ;
#17259=DIRECTION ( 'NONE',  ( -0.5449076811759708816, 0.6444004775717707689, 0.5364919789714475140 ) ) ;
#17260=LINE ( 'NONE', #39965, #34548 ) ;
#17261=CARTESIAN_POINT ( 'NONE',  ( -17.62617585138765008, -3.117730071725258956, 12.26528855537868701 ) ) ;
#17262=CARTESIAN_POINT ( 'NONE',  ( -17.68742552992882366, 0.000000000000000000, 8.206754174738705387 ) ) ;
#17263=CARTESIAN_POINT ( 'NONE',  ( -27.99923088623136636, 0.000000000000000000, 7.757173251277078130 ) ) ;
#17264=LINE ( 'NONE', #51902, #35632 ) ;
#17265=ORIENTED_EDGE ( 'NONE', *, *, #29279, .F. ) ;
#17266=DIRECTION ( 'NONE',  ( 0.005002170337468016433, -0.7660444431189770143, -0.6427681459581293666 ) ) ;
#17267=DIRECTION ( 'NONE',  ( -0.5449076811759708816, 0.6444004775717707689, 0.5364919789714475140 ) ) ;
#17268=ORIENTED_EDGE ( 'NONE', *, *, #18890, .T. ) ;
#17269=VERTEX_POINT ( 'NONE', #24170 ) ;
#17270=DIRECTION ( 'NONE',  ( 0.5449076811759707706, 0.6444004775717708799, -0.5364919789714476250 ) ) ;
#17271=ORIENTED_EDGE ( 'NONE', *, *, #7102, .T. ) ;
#17272=ADVANCED_FACE ( 'NONE', ( #41195 ), #15098, .F. ) ;
#17273=VECTOR ( 'NONE', #47734, 1000.000000000000227 ) ;
#17274=ORIENTED_EDGE ( 'NONE', *, *, #51964, .T. ) ;
#17275=ORIENTED_EDGE ( 'NONE', *, *, #40626, .T. ) ;
#17276=VERTEX_POINT ( 'NONE', #33257 ) ;
#17277=EDGE_CURVE ( 'NONE', #16077, #20216, #7126, .T. ) ;
#17278=ORIENTED_EDGE ( 'NONE', *, *, #35052, .F. ) ;
#17279=DIRECTION ( 'NONE',  ( 0.005002170337468016433, -0.7660444431189770143, -0.6427681459581293666 ) ) ;
#17280=ADVANCED_FACE ( 'NONE', ( #32126 ), #14802, .F. ) ;
#17281=DIRECTION ( 'NONE',  ( -0.005961354470445682716, -0.6427876096865404731, 0.7660212471507180654 ) ) ;
#17282=ORIENTED_EDGE ( 'NONE', *, *, #38223, .T. ) ;
#17283=EDGE_CURVE ( 'NONE', #9919, #46009, #49448, .T. ) ;
#17284=CARTESIAN_POINT ( 'NONE',  ( -17.69317363693938816, 0.000000000000000000, 8.945373581254235873 ) ) ;
#17285=ORIENTED_EDGE ( 'NONE', *, *, #37551, .F. ) ;
#17286=CARTESIAN_POINT ( 'NONE',  ( -18.19747506107908563, 0.000000000000000000, 14.03856424583689311 ) ) ;
#17287=DIRECTION ( 'NONE',  ( 0.007781995580012663651, 0.000000000000000000, -0.9999697198139515519 ) ) ;
#17288=VERTEX_POINT ( 'NONE', #37486 ) ;
#17289=LINE ( 'NONE', #7968, #29313 ) ;
#17290=EDGE_LOOP ( 'NONE', ( #6339, #2793, #52826, #42563 ) ) ;
#17291=VECTOR ( 'NONE', #28118, 1000.000000000000114 ) ;
#17292=PLANE ( 'NONE',  #35500 ) ;
#17294=LINE ( 'NONE', #25840, #19136 ) ;
#17295=VERTEX_POINT ( 'NONE', #54805 ) ;
#17297=DIRECTION ( 'NONE',  ( 0.000000000000000000, -1.000000000000000000, 0.000000000000000000 ) ) ;
#17298=CARTESIAN_POINT ( 'NONE',  ( -27.06552663992790997, 0.000000000000000000, 7.195101427592543786 ) ) ;
#17299=DIRECTION ( 'NONE',  ( -0.9999697198139514409, -0.000000000000000000, -0.007781995580013368816 ) ) ;
#17300=EDGE_CURVE ( 'NONE', #7239, #45359, #49972, .T. ) ;
#17302=AXIS2_PLACEMENT_3D ( 'NONE', #26737, #13951, #44599 ) ;
#17303=EDGE_CURVE ( 'NONE', #48501, #24198, #50564, .T. ) ;
#17304=FACE_OUTER_BOUND ( 'NONE', #29192, .T. ) ;
#17305=FACE_OUTER_BOUND ( 'NONE', #16290, .T. ) ;
#17306=DIRECTION ( 'NONE',  ( -0.5364919789714478471, 0.6444004775717705469, -0.5449076811759709926 ) ) ;
#17307=PLANE ( 'NONE',  #49534 ) ;
#17308=CARTESIAN_POINT ( 'NONE',  ( -14.24932064311472146, 1.257817950434004350, 2.176720800223820529 ) ) ;
#17309=LINE ( 'NONE', #47137, #53061 ) ;
#17310=ADVANCED_FACE ( 'NONE', ( #32423 ), #19327, .F. ) ;
#17311=DIRECTION ( 'NONE',  ( 0.9321478471874541372, 0.000000000000000000, -0.3620778797217453771 ) ) ;
#17312=AXIS2_PLACEMENT_3D ( 'NONE', #32009, #14976, #45613 ) ;
#17313=LINE ( 'NONE', #9087, #17506 ) ;
#17314=DIRECTION ( 'NONE',  ( 0.9999697198139515519, 0.000000000000000000, 0.007781995580013368816 ) ) ;
#17315=ORIENTED_EDGE ( 'NONE', *, *, #23614, .F. ) ;
#17317=PLANE ( 'NONE',  #22382 ) ;
#17318=EDGE_LOOP ( 'NONE', ( #30940, #42640, #52000, #53735 ) ) ;
#17319=DIRECTION ( 'NONE',  ( -0.6427681459581293666, -0.7660444431189770143, -0.005002170337467561935 ) ) ;
#17320=DIRECTION ( 'NONE',  ( -0.5449076811759708816, 0.6444004775717707689, 0.5364919789714475140 ) ) ;
#17322=LINE ( 'NONE', #24124, #32734 ) ;
#17323=CARTESIAN_POINT ( 'NONE',  ( -15.43184522958867788, -0.1191753592594192307, 4.061651826203944715 ) ) ;
#17324=CARTESIAN_POINT ( 'NONE',  ( -18.30775837356714675, 1.095915999411505526, 3.758321359744400070 ) ) ;
#17325=ADVANCED_FACE ( 'NONE', ( #29554 ), #25842, .F. ) ;
#17326=ORIENTED_EDGE ( 'NONE', *, *, #5863, .F. ) ;
#17327=ORIENTED_EDGE ( 'NONE', *, *, #10690, .F. ) ;
#17328=DIRECTION ( 'NONE',  ( 0.6427681459581294776, -0.7660444431189769032, 0.005002170337467562802 ) ) ;
#17330=PLANE ( 'NONE',  #13200 ) ;
#17332=VERTEX_POINT ( 'NONE', #7380 ) ;
#17333=CARTESIAN_POINT ( 'NONE',  ( -15.40103151951671734, 0.000000000000000000, 12.95233060667165681 ) ) ;
#17334=VECTOR ( 'NONE', #33212, 999.9999999999998863 ) ;
#17335=VECTOR ( 'NONE', #25837, 1000.000000000000227 ) ;
#17336=ORIENTED_EDGE ( 'NONE', *, *, #38633, .T. ) ;
#17337=DIRECTION ( 'NONE',  ( -0.7660212471507179544, -0.6427876096865405842, -0.005961354470445141482 ) ) ;
#17338=VERTEX_POINT ( 'NONE', #21593 ) ;
#17339=CARTESIAN_POINT ( 'NONE',  ( -13.63673279712320507, -0.1191753592594197858, 12.22739664767016521 ) ) ;
#17340=ORIENTED_EDGE ( 'NONE', *, *, #52670, .T. ) ;
#17341=ORIENTED_EDGE ( 'NONE', *, *, #5613, .T. ) ;
#17342=EDGE_LOOP ( 'NONE', ( #47060, #16185, #26442, #50535 ) ) ;
#17343=CARTESIAN_POINT ( 'NONE',  ( -13.97033035520014010, 0.000000000000000000, 8.235681468882781076 ) ) ;
#17344=PLANE ( 'NONE',  #52261 ) ;
#17345=PLANE ( 'NONE',  #44788 ) ;
#17346=DIRECTION ( 'NONE',  ( -0.7660212471507179544, -0.6427876096865405842, -0.005961354470445141482 ) ) ;
#17347=VERTEX_POINT ( 'NONE', #56209 ) ;
#17348=ADVANCED_FACE ( 'NONE', ( #34362 ), #46868, .F. ) ;
#17349=ORIENTED_EDGE ( 'NONE', *, *, #1210, .F. ) ;
#17350=AXIS2_PLACEMENT_3D ( 'NONE', #53609, #28902, #49900 ) ;
#17351=ORIENTED_EDGE ( 'NONE', *, *, #27592, .F. ) ;
#17352=DIRECTION ( 'NONE',  ( 0.6427681459581294776, -0.7660444431189769032, 0.005002170337467562802 ) ) ;
#17353=VERTEX_POINT ( 'NONE', #43175 ) ;
#17354=PLANE ( 'NONE',  #31185 ) ;
#17355=ORIENTED_EDGE ( 'NONE', *, *, #54011, .T. ) ;
#17356=CARTESIAN_POINT ( 'NONE',  ( -11.67244013076689946, 0.000000000000000000, 11.50401908778467863 ) ) ;
#17357=PLANE ( 'NONE',  #23088 ) ;
#17358=EDGE_CURVE ( 'NONE', #26046, #4586, #3970, .T. ) ;
#17359=ORIENTED_EDGE ( 'NONE', *, *, #14206, .F. ) ;
#17361=VERTEX_POINT ( 'NONE', #12212 ) ;
#17362=EDGE_CURVE ( 'NONE', #50871, #25675, #29828, .T. ) ;
#17363=ADVANCED_FACE ( 'NONE', ( #51412 ), #47128, .F. ) ;
#17365=ORIENTED_EDGE ( 'NONE', *, *, #13535, .F. ) ;
#17366=PLANE ( 'NONE',  #25051 ) ;
#17367=PLANE ( 'NONE',  #50204 ) ;
#17368=DIRECTION ( 'NONE',  ( 0.6427681459581294776, -0.7660444431189769032, 0.005002170337467562802 ) ) ;
#17369=EDGE_CURVE ( 'NONE', #50265, #6886, #33515, .T. ) ;
#17370=EDGE_LOOP ( 'NONE', ( #32570, #35378, #49705, #48778 ) ) ;
#17371=VECTOR ( 'NONE', #48419, 999.9999999999998863 ) ;
#17372=CARTESIAN_POINT ( 'NONE',  ( -15.73373731979538270, -3.756034771668160577, 8.957742581241667779 ) ) ;
#17373=VECTOR ( 'NONE', #50041, 999.9999999999998863 ) ;
#17374=ADVANCED_FACE ( 'NONE', ( #21294 ), #29242, .F. ) ;
#17375=CARTESIAN_POINT ( 'NONE',  ( -19.60912206198628027, -0.1191753592594197858, 4.398475361799976113 ) ) ;
#17376=LINE ( 'NONE', #39243, #50270 ) ;
#17377=LINE ( 'NONE', #38975, #11372 ) ;
#17378=PLANE ( 'NONE',  #34012 ) ;
#17379=EDGE_CURVE ( 'NONE', #54774, #1004, #4279, .T. ) ;
#17380=DIRECTION ( 'NONE',  ( 0.000000000000000000, 1.000000000000000000, -0.000000000000000000 ) ) ;
#17381=CARTESIAN_POINT ( 'NONE',  ( -18.67775241435682432, 0.000000000000000000, 4.136394454059623804 ) ) ;
#17382=VECTOR ( 'NONE', #16536, 999.9999999999998863 ) ;
#17383=EDGE_LOOP ( 'NONE', ( #35452, #48412, #29494, #27732 ) ) ;
#17384=CARTESIAN_POINT ( 'NONE',  ( -7.094024697029445825, 2.107956770024262294, 8.730276719704061605 ) ) ;
#17385=DIRECTION ( 'NONE',  ( 0.9999697198139515519, 0.000000000000000000, 0.007781995580013368816 ) ) ;
#17386=LINE ( 'NONE', #52031, #36883 ) ;
#17387=ORIENTED_EDGE ( 'NONE', *, *, #30073, .F. ) ;
#17388=LINE ( 'NONE', #2990, #7535 ) ;
#17389=CARTESIAN_POINT ( 'NONE',  ( -27.06708303904391144, 0.000000000000000000, 7.395095371555332697 ) ) ;
#17390=ORIENTED_EDGE ( 'NONE', *, *, #6453, .T. ) ;
#17393=CARTESIAN_POINT ( 'NONE',  ( -6.824261881224860993, 4.558205123441750217, -0.5675985080870675770 ) ) ;
#17394=AXIS2_PLACEMENT_3D ( 'NONE', #18722, #21834, #5376 ) ;
#17395=DIRECTION ( 'NONE',  ( -0.6427681459581293666, -0.7660444431189770143, -0.005002170337467561935 ) ) ;
#17396=VECTOR ( 'NONE', #15008, 999.9999999999998863 ) ;
#17398=EDGE_CURVE ( 'NONE', #51697, #18162, #46561, .T. ) ;
#17399=ORIENTED_EDGE ( 'NONE', *, *, #54367, .F. ) ;
#17400=ORIENTED_EDGE ( 'NONE', *, *, #31507, .F. ) ;
#17401=LINE ( 'NONE', #13161, #21276 ) ;
#17402=DIRECTION ( 'NONE',  ( 0.005002170337468016433, -0.7660444431189770143, -0.6427681459581293666 ) ) ;
#17403=LINE ( 'NONE', #8627, #16002 ) ;
#17404=LINE ( 'NONE', #47222, #36586 ) ;
#17405=CARTESIAN_POINT ( 'NONE',  ( -16.28854238969427470, -3.917936722690662954, 3.083341448462168621 ) ) ;
#17406=DIRECTION ( 'NONE',  ( 0.7660212471507180654, -0.6427876096865404731, 0.005961354470445141482 ) ) ;
#17407=EDGE_LOOP ( 'NONE', ( #39259, #14555, #16259, #18245 ) ) ;
#17408=DIRECTION ( 'NONE',  ( 0.007781995580012662783, 0.000000000000000000, -0.9999697198139514409 ) ) ;
#17409=DIRECTION ( 'NONE',  ( 0.005002170337468016433, -0.7660444431189770143, -0.6427681459581293666 ) ) ;
#17410=ORIENTED_EDGE ( 'NONE', *, *, #48428, .F. ) ;
#17411=CARTESIAN_POINT ( 'NONE',  ( -13.03021690632542828, 3.686347215771511365, 1.625696709606834434 ) ) ;
#17412=DIRECTION ( 'NONE',  ( 0.000000000000000000, -1.000000000000000000, 0.000000000000000000 ) ) ;
#17414=EDGE_LOOP ( 'NONE', ( #28047, #12285, #18293, #20998 ) ) ;
#17415=VECTOR ( 'NONE', #3088, 1000.000000000000114 ) ;
#17416=VECTOR ( 'NONE', #31583, 1000.000000000000227 ) ;
#17417=DIRECTION ( 'NONE',  ( -0.005002170337468016433, -0.7660444431189770143, 0.6427681459581293666 ) ) ;
#17418=ADVANCED_FACE ( 'NONE', ( #51666 ), #25546, .F. ) ;
#17420=ORIENTED_EDGE ( 'NONE', *, *, #36355, .F. ) ;
#17421=ORIENTED_EDGE ( 'NONE', *, *, #17153, .T. ) ;
#17422=VECTOR ( 'NONE', #12777, 1000.000000000000227 ) ;
#17423=ORIENTED_EDGE ( 'NONE', *, *, #10218, .F. ) ;
#17424=FACE_OUTER_BOUND ( 'NONE', #1602, .T. ) ;
#17425=ORIENTED_EDGE ( 'NONE', *, *, #3453, .T. ) ;
#17426=ADVANCED_FACE ( 'NONE', ( #13060 ), #37796, .F. ) ;
#17428=EDGE_CURVE ( 'NONE', #33926, #14055, #47405, .T. ) ;
#17429=VERTEX_POINT ( 'NONE', #20737 ) ;
#17430=DIRECTION ( 'NONE',  ( 0.007781995580012662783, 0.000000000000000000, -0.9999697198139514409 ) ) ;
#17431=VERTEX_POINT ( 'NONE', #55361 ) ;
#17432=CARTESIAN_POINT ( 'NONE',  ( -14.45241350051485796, -1.165603555308155626, 4.208693952685643502 ) ) ;
#17433=AXIS2_PLACEMENT_3D ( 'NONE', #56091, #4670, #52641 ) ;
#17434=EDGE_LOOP ( 'NONE', ( #52390, #25197, #21561, #3507 ) ) ;
#17435=EDGE_CURVE ( 'NONE', #9089, #31401, #16457, .T. ) ;
#17436=FACE_OUTER_BOUND ( 'NONE', #37667, .T. ) ;
#17437=CARTESIAN_POINT ( 'NONE',  ( -18.80076660093136809, 0.000000000000000000, 6.151423491835070756 ) ) ;
#17438=FACE_OUTER_BOUND ( 'NONE', #35324, .T. ) ;
#17439=DIRECTION ( 'NONE',  ( 0.9999697198139515519, 0.000000000000000000, 0.007781995580013368816 ) ) ;
#17440=DIRECTION ( 'NONE',  ( 0.007781995580012663651, 0.000000000000000000, -0.9999697198139515519 ) ) ;
#17441=ORIENTED_EDGE ( 'NONE', *, *, #33891, .F. ) ;
#17442=VERTEX_POINT ( 'NONE', #13882 ) ;
#17443=ADVANCED_FACE ( 'NONE', ( #36061 ), #47973, .F. ) ;
#17444=LINE ( 'NONE', #35088, #27657 ) ;
#17445=DIRECTION ( 'NONE',  ( -0.005002170337468016433, -0.7660444431189770143, 0.6427681459581293666 ) ) ;
#17446=AXIS2_PLACEMENT_3D ( 'NONE', #21742, #52114, #22011 ) ;
#17447=ADVANCED_FACE ( 'NONE', ( #39164 ), #52246, .F. ) ;
#17448=DIRECTION ( 'NONE',  ( 0.2426528472758541499, 0.7422098413412800966, 0.6246952433987894571 ) ) ;
#17449=PLANE ( 'NONE',  #48466 ) ;
#17450=EDGE_CURVE ( 'NONE', #32241, #47466, #14197, .T. ) ;
#17451=CARTESIAN_POINT ( 'NONE',  ( -19.89959890415981292, 0.7721120973665049902, 4.386977320733340235 ) ) ;
#17452=DIRECTION ( 'NONE',  ( 0.000000000000000000, -1.000000000000000000, 0.000000000000000000 ) ) ;
#17453=ORIENTED_EDGE ( 'NONE', *, *, #13387, .F. ) ;
#17454=VECTOR ( 'NONE', #10019, 1000.000000000000227 ) ;
#17456=DIRECTION ( 'NONE',  ( 0.007781995580012663651, -3.146120232559066537E-19, -0.9999697198139514409 ) ) ;
#17457=ORIENTED_EDGE ( 'NONE', *, *, #52817, .F. ) ;
#17458=AXIS2_PLACEMENT_3D ( 'NONE', #3928, #55606, #33480 ) ;
#17459=EDGE_CURVE ( 'NONE', #20837, #33148, #31518, .T. ) ;
#17460=VECTOR ( 'NONE', #9596, 1000.000000000000227 ) ;
#17461=PLANE ( 'NONE',  #36128 ) ;
#17462=CARTESIAN_POINT ( 'NONE',  ( -19.20472701092309720, 1.581621852479005552, 6.936800195413949766 ) ) ;
#17463=CARTESIAN_POINT ( 'NONE',  ( -13.17065887352947762, -0.1191753592594197858, 12.04635770780929427 ) ) ;
#17464=LINE ( 'NONE', #34796, #41361 ) ;
#17465=CARTESIAN_POINT ( 'NONE',  ( -25.20200914511100265, -0.1191753592594197858, 6.570942640130446932 ) ) ;
#17466=ORIENTED_EDGE ( 'NONE', *, *, #40263, .T. ) ;
#17467=AXIS2_PLACEMENT_3D ( 'NONE', #24059, #41389, #9895 ) ;
#17468=VECTOR ( 'NONE', #23488, 999.9999999999998863 ) ;
#17469=VERTEX_POINT ( 'NONE', #40003 ) ;
#17470=CARTESIAN_POINT ( 'NONE',  ( -30.79567442779373110, 0.000000000000000000, 8.843406890442315316 ) ) ;
#17471=LINE ( 'NONE', #34802, #53077 ) ;
#17472=CARTESIAN_POINT ( 'NONE',  ( -16.95371522758815885, 0.000000000000000000, 7.643125951938166907 ) ) ;
#17473=LINE ( 'NONE', #30574, #31896 ) ;
#17474=VECTOR ( 'NONE', #14729, 1000.000000000000000 ) ;
#17475=LINE ( 'NONE', #22596, #22221 ) ;
#17477=AXIS2_PLACEMENT_3D ( 'NONE', #24750, #15969, #15662 ) ;
#17478=DIRECTION ( 'NONE',  ( -0.5364919789714478471, 0.6444004775717705469, -0.5449076811759709926 ) ) ;
#17480=CARTESIAN_POINT ( 'NONE',  ( -16.97217308376872325, -0.8417996532631553119, 4.656036778316158475 ) ) ;
#17481=CARTESIAN_POINT ( 'NONE',  ( -26.13493519185646008, 0.000000000000000000, 7.033017491833586377 ) ) ;
#17482=ORIENTED_EDGE ( 'NONE', *, *, #33646, .F. ) ;
#17483=LINE ( 'NONE', #30585, #37445 ) ;
#17484=ORIENTED_EDGE ( 'NONE', *, *, #14484, .T. ) ;
#17486=ADVANCED_FACE ( 'NONE', ( #35762 ), #27228, .F. ) ;
#17487=VECTOR ( 'NONE', #1305, 1000.000000000000000 ) ;
#17488=CARTESIAN_POINT ( 'NONE',  ( -9.075990533167328067, 0.000000000000000000, 10.41622904950343909 ) ) ;
#17489=VERTEX_POINT ( 'NONE', #13354 ) ;
#17490=EDGE_CURVE ( 'NONE', #36296, #24378, #34930, .T. ) ;
#17491=AXIS2_PLACEMENT_3D ( 'NONE', #41154, #1420, #2246 ) ;
#17492=ORIENTED_EDGE ( 'NONE', *, *, #18939, .F. ) ;
#17493=ORIENTED_EDGE ( 'NONE', *, *, #37078, .T. ) ;
#17494=ORIENTED_EDGE ( 'NONE', *, *, #28815, .F. ) ;
#17495=ORIENTED_EDGE ( 'NONE', *, *, #217, .F. ) ;
#17496=EDGE_CURVE ( 'NONE', #31186, #38038, #5646, .T. ) ;
#17497=ORIENTED_EDGE ( 'NONE', *, *, #30324, .F. ) ;
#17498=VECTOR ( 'NONE', #37766, 1000.000000000000114 ) ;
#17499=LINE ( 'NONE', #18852, #54925 ) ;
#17500=DIRECTION ( 'NONE',  ( -0.005961354470445682716, -0.6427876096865404731, 0.7660212471507180654 ) ) ;
#17501=LINE ( 'NONE', #26885, #38539 ) ;
#17502=EDGE_CURVE ( 'NONE', #1004, #29284, #18144, .T. ) ;
#17503=EDGE_CURVE ( 'NONE', #9004, #34934, #8823, .T. ) ;
#17504=EDGE_CURVE ( 'NONE', #24424, #25619, #1385, .T. ) ;
#17505=VECTOR ( 'NONE', #47485, 999.9999999999998863 ) ;
#17506=VECTOR ( 'NONE', #30938, 999.9999999999998863 ) ;
#17507=EDGE_LOOP ( 'NONE', ( #29328, #3109, #7930, #47525 ) ) ;
#17508=CARTESIAN_POINT ( 'NONE',  ( -17.74404816805336793, 0.000000000000000000, 3.574322630375089460 ) ) ;
#17509=EDGE_LOOP ( 'NONE', ( #19, #2623, #37926, #20813 ) ) ;
#17510=ADVANCED_FACE ( 'NONE', ( #53081 ), #26128, .F. ) ;
#17511=ORIENTED_EDGE ( 'NONE', *, *, #31393, .F. ) ;
#17512=AXIS2_PLACEMENT_3D ( 'NONE', #22604, #53283, #1279 ) ;
#17513=AXIS2_PLACEMENT_3D ( 'NONE', #34382, #55670, #42606 ) ;
#17514=DIRECTION ( 'NONE',  ( 0.000000000000000000, -1.000000000000000000, 0.000000000000000000 ) ) ;
#17515=DIRECTION ( 'NONE',  ( 0.5449076811759707706, 0.6444004775717708799, -0.5364919789714476250 ) ) ;
#17516=DIRECTION ( 'NONE',  ( 0.005961354470445682716, -0.6427876096865404731, -0.7660212471507180654 ) ) ;
#17517=ORIENTED_EDGE ( 'NONE', *, *, #48930, .T. ) ;
#17519=ORIENTED_EDGE ( 'NONE', *, *, #4717, .F. ) ;
#17520=DIRECTION ( 'NONE',  ( 0.7660212471507180654, -0.6427876096865404731, 0.005961354470445141482 ) ) ;
#17521=VECTOR ( 'NONE', #34093, 999.9999999999998863 ) ;
#17522=EDGE_CURVE ( 'NONE', #17269, #8995, #43693, .T. ) ;
#17523=DIRECTION ( 'NONE',  ( -0.005961354470445682716, -0.6427876096865404731, 0.7660212471507180654 ) ) ;
#17524=VECTOR ( 'NONE', #5697, 999.9999999999998863 ) ;
#17525=ADVANCED_FACE ( 'NONE', ( #17896 ), #249, .F. ) ;
#17526=PLANE ( 'NONE',  #6108 ) ;
#17527=PLANE ( 'NONE',  #8678 ) ;
#17528=CARTESIAN_POINT ( 'NONE',  ( -16.81345671998191449, 0.000000000000000000, 3.412238694616132495 ) ) ;
#17529=CARTESIAN_POINT ( 'NONE',  ( -15.96710241509184058, -0.1191753592594218814, 13.13259134697452879 ) ) ;
#17530=ADVANCED_FACE ( 'NONE', ( #22134 ), #9655, .F. ) ;
#17531=LINE ( 'NONE', #35415, #51128 ) ;
#17532=CARTESIAN_POINT ( 'NONE',  ( -16.84587429464891173, -0.1191753592594185784, 6.635972013704265926 ) ) ;
#17533=ORIENTED_EDGE ( 'NONE', *, *, #51011, .F. ) ;
#17535=VECTOR ( 'NONE', #28474, 1000.000000000000227 ) ;
#17536=EDGE_CURVE ( 'NONE', #29764, #37770, #9343, .T. ) ;
#17537=DIRECTION ( 'NONE',  ( -0.5449076811759708816, 0.6444004775717707689, 0.5364919789714475140 ) ) ;
#17538=CARTESIAN_POINT ( 'NONE',  ( -25.20278734466900517, 0.000000000000000000, 6.670939612111840944 ) ) ;
#17539=PLANE ( 'NONE',  #46246 ) ;
#17542=CARTESIAN_POINT ( 'NONE',  ( -16.06709938707323460, 0.000000000000000000, 13.13181314741652628 ) ) ;
#17543=EDGE_CURVE ( 'NONE', #13476, #17361, #44285, .T. ) ;
#17544=CARTESIAN_POINT ( 'NONE',  ( -12.10447826170922880, 0.000000000000000000, 7.311531765476501299 ) ) ;
#17545=CARTESIAN_POINT ( 'NONE',  ( -10.40437021484443569, 0.000000000000000000, 1.984787408528857489 ) ) ;
#17547=ORIENTED_EDGE ( 'NONE', *, *, #30009, .F. ) ;
#17548=VECTOR ( 'NONE', #27335, 999.9999999999998863 ) ;
#17549=CARTESIAN_POINT ( 'NONE',  ( -18.35064882566791411, 3.362543313726510164, 3.702664189482756552 ) ) ;
#17550=LINE ( 'NONE', #56173, #29444 ) ;
#17551=CARTESIAN_POINT ( 'NONE',  ( -11.60978317542603300, 0.000000000000000000, 3.452734885371889550 ) ) ;
#17552=VECTOR ( 'NONE', #46936, 999.9999999999998863 ) ;
#17553=VECTOR ( 'NONE', #44298, 999.9999999999998863 ) ;
#17554=CARTESIAN_POINT ( 'NONE',  ( -17.30763713798472025, -0.1191753592594164690, 6.263046398678491222 ) ) ;
#17555=CARTESIAN_POINT ( 'NONE',  ( -15.13495153988577968, 0.000000000000000000, 12.76973526769478084 ) ) ;
#17556=DIRECTION ( 'NONE',  ( 0.007781995580012663651, -3.146120232559066537E-19, -0.9999697198139514409 ) ) ;
#17558=VECTOR ( 'NONE', #2868, 1000.000000000000227 ) ;
#17559=PLANE ( 'NONE',  #7662 ) ;
#17560=VECTOR ( 'NONE', #10513, 1000.000000000000227 ) ;
#17561=CARTESIAN_POINT ( 'NONE',  ( -15.40103151951671734, 0.000000000000000000, 12.95233060667165681 ) ) ;
#17562=ORIENTED_EDGE ( 'NONE', *, *, #13032, .T. ) ;
#17563=CARTESIAN_POINT ( 'NONE',  ( -12.68923408260478958, -0.1941918491731554897, 1.804054826373973519 ) ) ;
#17564=ORIENTED_EDGE ( 'NONE', *, *, #36014, .T. ) ;
#17565=ORIENTED_EDGE ( 'NONE', *, *, #17117, .F. ) ;
#17566=VERTEX_POINT ( 'NONE', #54731 ) ;
#17568=VECTOR ( 'NONE', #29026, 1000.000000000000000 ) ;
#17570=DIRECTION ( 'NONE',  ( 0.9999697198139515519, 0.000000000000000000, 0.007781995580013368816 ) ) ;
#17571=CARTESIAN_POINT ( 'NONE',  ( -13.49838895223248336, 0.000000000000000000, 7.300684030172472028 ) ) ;
#17572=AXIS2_PLACEMENT_3D ( 'NONE', #51871, #30613, #39102 ) ;
#17574=EDGE_CURVE ( 'NONE', #42137, #31963, #41126, .T. ) ;
#17575=EDGE_LOOP ( 'NONE', ( #7035, #14878, #31958, #30210 ) ) ;
#17576=ORIENTED_EDGE ( 'NONE', *, *, #21385, .T. ) ;
#17577=VECTOR ( 'NONE', #9022, 1000.000000000000114 ) ;
#17578=ADVANCED_FACE ( 'NONE', ( #32355 ), #54196, .F. ) ;
#17580=ORIENTED_EDGE ( 'NONE', *, *, #26772, .T. ) ;
#17581=VECTOR ( 'NONE', #32108, 1000.000000000000000 ) ;
#17582=CARTESIAN_POINT ( 'NONE',  ( -19.79569077582305070, 0.000000000000000000, 14.58012466630350445 ) ) ;
#17585=DIRECTION ( 'NONE',  ( 0.000000000000000000, -1.000000000000000000, 0.000000000000000000 ) ) ;
#17586=VECTOR ( 'NONE', #55955, 999.9999999999998863 ) ;
#17587=VERTEX_POINT ( 'NONE', #19550 ) ;
#17588=LINE ( 'NONE', #8513, #12805 ) ;
#17589=VECTOR ( 'NONE', #39263, 1000.000000000000227 ) ;
#17590=LINE ( 'NONE', #20997, #21848 ) ;
#17591=VECTOR ( 'NONE', #40176, 1000.000000000000227 ) ;
#17592=VERTEX_POINT ( 'NONE', #6775 ) ;
#17593=CARTESIAN_POINT ( 'NONE',  ( -18.67619601524082285, 0.000000000000000000, 3.936400510096834893 ) ) ;
#17594=DIRECTION ( 'NONE',  ( -0.6246952433987893460, -0.7422098413412802076, 0.2426528472758542054 ) ) ;
#17595=PLANE ( 'NONE',  #3058 ) ;
#17596=ORIENTED_EDGE ( 'NONE', *, *, #22281, .F. ) ;
#17597=CARTESIAN_POINT ( 'NONE',  ( -10.68338343524914968, 0.000000000000000000, 3.829276412165673715 ) ) ;
#17599=CARTESIAN_POINT ( 'NONE',  ( -14.01545677930355183, 0.000000000000000000, 2.126011111488108174 ) ) ;
#17600=DIRECTION ( 'NONE',  ( 0.007781995580012663651, 0.000000000000000000, -0.9999697198139515519 ) ) ;
#17601=DIRECTION ( 'NONE',  ( 0.000000000000000000, -0.000000000000000000, -1.000000000000000000 ) ) ;
#17602=LINE ( 'NONE', #52523, #26877 ) ;
#17603=FACE_OUTER_BOUND ( 'NONE', #4261, .T. ) ;
#17604=EDGE_CURVE ( 'NONE', #50472, #6087, #10761, .T. ) ;
#17605=LINE ( 'NONE', #4290, #28573 ) ;
#17606=CARTESIAN_POINT ( 'NONE',  ( -15.83175199606975880, 0.000000000000000000, 8.590527525068505810 ) ) ;
#17607=VECTOR ( 'NONE', #1018, 1000.000000000000227 ) ;
#17608=DIRECTION ( 'NONE',  ( -0.9999697198139514409, -0.000000000000000000, -0.007781995580013368816 ) ) ;
#17609=AXIS2_PLACEMENT_3D ( 'NONE', #4328, #38095, #47459 ) ;
#17610=EDGE_CURVE ( 'NONE', #48860, #3963, #2507, .T. ) ;
#17611=CARTESIAN_POINT ( 'NONE',  ( -16.25902619734217680, 0.000000000000000000, 3.785885470949557963 ) ) ;
#17612=ORIENTED_EDGE ( 'NONE', *, *, #33366, .F. ) ;
#17613=CARTESIAN_POINT ( 'NONE',  ( -12.53043480859235892, 0.000000000000000000, 2.337573952062577121 ) ) ;
#17614=PLANE ( 'NONE',  #31802 ) ;
#17615=EDGE_CURVE ( 'NONE', #40689, #6398, #27508, .T. ) ;
#17616=VECTOR ( 'NONE', #50698, 1000.000000000000114 ) ;
#17617=DIRECTION ( 'NONE',  ( 0.007781995580012663651, 0.000000000000000000, -0.9999697198139515519 ) ) ;
#17618=EDGE_CURVE ( 'NONE', #44660, #34834, #40848, .T. ) ;
#17619=CARTESIAN_POINT ( 'NONE',  ( -18.81451671468552789, -0.1191753592594156363, 9.205976071834351515 ) ) ;
#17620=VECTOR ( 'NONE', #36813, 999.9999999999998863 ) ;
#17621=DIRECTION ( 'NONE',  ( 0.9321478471874541372, 0.000000000000000000, -0.3620778797217453771 ) ) ;
#17622=FACE_OUTER_BOUND ( 'NONE', #6401, .T. ) ;
#17623=ORIENTED_EDGE ( 'NONE', *, *, #15586, .F. ) ;
#17624=VERTEX_POINT ( 'NONE', #1924 ) ;
#17625=CARTESIAN_POINT ( 'NONE',  ( -21.22452843065813965, -4.727446477803159297, 12.68480442045455803 ) ) ;
#17626=VECTOR ( 'NONE', #56196, 1000.000000000000227 ) ;
#17627=LINE ( 'NONE', #38658, #18635 ) ;
#17628=ORIENTED_EDGE ( 'NONE', *, *, #9707, .F. ) ;
#17629=VECTOR ( 'NONE', #32357, 999.9999999999998863 ) ;
#17631=ORIENTED_EDGE ( 'NONE', *, *, #55195, .T. ) ;
#17632=FACE_OUTER_BOUND ( 'NONE', #11639, .T. ) ;
#17633=VERTEX_POINT ( 'NONE', #28069 ) ;
#17634=DIRECTION ( 'NONE',  ( -0.7660212471507179544, -0.6427876096865405842, -0.005961354470445141482 ) ) ;
#17635=AXIS2_PLACEMENT_3D ( 'NONE', #19791, #6456, #37112 ) ;
#17636=EDGE_LOOP ( 'NONE', ( #5700, #20566, #46351, #20762 ) ) ;
#17637=AXIS2_PLACEMENT_3D ( 'NONE', #5214, #22785, #1192 ) ;
#17638=EDGE_LOOP ( 'NONE', ( #13724, #51067, #20497, #31893 ) ) ;
#17639=ORIENTED_EDGE ( 'NONE', *, *, #2171, .T. ) ;
#17641=DIRECTION ( 'NONE',  ( 0.6427681459581294776, -0.7660444431189769032, 0.005002170337467562802 ) ) ;
#17642=LINE ( 'NONE', #34983, #34817 ) ;
#17643=EDGE_CURVE ( 'NONE', #24619, #55170, #36589, .T. ) ;
#17644=CARTESIAN_POINT ( 'NONE',  ( -25.20123094555300369, 0.000000000000000000, 6.470945668149052032 ) ) ;
#17645=ORIENTED_EDGE ( 'NONE', *, *, #8915, .F. ) ;
#17646=ORIENTED_EDGE ( 'NONE', *, *, #26995, .T. ) ;
#17647=EDGE_CURVE ( 'NONE', #2654, #51468, #20082, .T. ) ;
#17648=EDGE_CURVE ( 'NONE', #13341, #41874, #19827, .T. ) ;
#17649=AXIS2_PLACEMENT_3D ( 'NONE', #21804, #35181, #39126 ) ;
#17650=ORIENTED_EDGE ( 'NONE', *, *, #28887, .F. ) ;
#17651=CARTESIAN_POINT ( 'NONE',  ( -11.20636620717317378, 0.000000000000000000, 11.32298014792380414 ) ) ;
#17652=AXIS2_PLACEMENT_3D ( 'NONE', #9127, #30728, #48030 ) ;
#17653=VERTEX_POINT ( 'NONE', #6489 ) ;
#17654=CARTESIAN_POINT ( 'NONE',  ( -10.69200559576499643, 0.000000000000000000, 4.937205521938968111 ) ) ;
#17655=VERTEX_POINT ( 'NONE', #54445 ) ;
#17657=CARTESIAN_POINT ( 'NONE',  ( -29.86352658060627618, 0.000000000000000000, 8.481329010720569883 ) ) ;
#17658=CARTESIAN_POINT ( 'NONE',  ( -22.56675936406184135, 4.495856970884013037, 5.304186063099788129 ) ) ;
#17659=ORIENTED_EDGE ( 'NONE', *, *, #11979, .T. ) ;
#17660=DIRECTION ( 'NONE',  ( -0.5449076811759708816, 0.6444004775717707689, 0.5364919789714475140 ) ) ;
#17661=VECTOR ( 'NONE', #40296, 999.9999999999998863 ) ;
#17662=ORIENTED_EDGE ( 'NONE', *, *, #29274, .F. ) ;
#17665=AXIS2_PLACEMENT_3D ( 'NONE', #37874, #16267, #34180 ) ;
#17666=ORIENTED_EDGE ( 'NONE', *, *, #31775, .F. ) ;
#17667=DIRECTION ( 'NONE',  ( 0.000000000000000000, -1.000000000000000000, 0.000000000000000000 ) ) ;
#17668=DIRECTION ( 'NONE',  ( -0.005002170337468016433, -0.7660444431189770143, 0.6427681459581293666 ) ) ;
#17669=VECTOR ( 'NONE', #31432, 999.9999999999998863 ) ;
#17670=LINE ( 'NONE', #48305, #26451 ) ;
#17671=ORIENTED_EDGE ( 'NONE', *, *, #33306, .T. ) ;
#17672=VECTOR ( 'NONE', #22451, 999.9999999999998863 ) ;
#17673=LINE ( 'NONE', #17372, #15660 ) ;
#17674=LINE ( 'NONE', #333, #12855 ) ;
#17675=CARTESIAN_POINT ( 'NONE',  ( -21.17884633731301136, -1.975113310420658852, 5.044887815787086893 ) ) ;
#17676=PLANE ( 'NONE',  #52241 ) ;
#17677=CARTESIAN_POINT ( 'NONE',  ( -15.54256021603320015, 0.000000000000000000, 5.438115467695609162 ) ) ;
#17678=DIRECTION ( 'NONE',  ( -0.005961354470445682716, -0.6427876096865404731, 0.7660212471507180654 ) ) ;
#17679=VECTOR ( 'NONE', #41012, 999.9999999999998863 ) ;
#17680=VECTOR ( 'NONE', #415, 1000.000000000000227 ) ;
#17681=CARTESIAN_POINT ( 'NONE',  ( -9.751235588061692994, 0.000000000000000000, 3.467198532443927839 ) ) ;
#17682=ORIENTED_EDGE ( 'NONE', *, *, #11928, .T. ) ;
#17683=CARTESIAN_POINT ( 'NONE',  ( -16.82862997361721824, -0.1191753592594196748, 4.420113794157683351 ) ) ;
#17684=CARTESIAN_POINT ( 'NONE',  ( -14.97583049326344096, -0.1191753592594192307, 5.173196847745247240 ) ) ;
#17685=CARTESIAN_POINT ( 'NONE',  ( -19.22961988024793101, -0.1191753592594177458, 14.39986392600063603 ) ) ;
#17686=EDGE_LOOP ( 'NONE', ( #26356, #6686, #5238, #4459 ) ) ;
#17687=PLANE ( 'NONE',  #21155 ) ;
#17688=CARTESIAN_POINT ( 'NONE',  ( -16.08055152492125828, 1.743523803501506819, 5.988973023155203634 ) ) ;
#17689=VERTEX_POINT ( 'NONE', #1666 ) ;
#17690=DIRECTION ( 'NONE',  ( 0.7660212471507180654, -0.6427876096865404731, 0.005961354470445141482 ) ) ;
#17691=EDGE_CURVE ( 'NONE', #14368, #26120, #18994, .T. ) ;
#17692=LINE ( 'NONE', #31603, #41142 ) ;
#17693=DIRECTION ( 'NONE',  ( 0.005961354470445682716, -0.6427876096865404731, -0.7660212471507180654 ) ) ;
#17695=AXIS2_PLACEMENT_3D ( 'NONE', #5829, #10670, #27694 ) ;
#17696=ORIENTED_EDGE ( 'NONE', *, *, #29936, .T. ) ;
#17697=ORIENTED_EDGE ( 'NONE', *, *, #54517, .F. ) ;
#17698=DIRECTION ( 'NONE',  ( 0.007781995580012663651, 0.000000000000000000, -0.9999697198139515519 ) ) ;
#17699=FACE_OUTER_BOUND ( 'NONE', #49771, .T. ) ;
#17700=CARTESIAN_POINT ( 'NONE',  ( -11.62990154996301051, 0.000000000000000000, 6.037902808176242253 ) ) ;
#17701=VECTOR ( 'NONE', #14736, 999.9999999999998863 ) ;
#17702=ADVANCED_FACE ( 'NONE', ( #14728 ), #32053, .F. ) ;
#17703=CARTESIAN_POINT ( 'NONE',  ( -13.12015695940438320, -0.1191753592594174960, 5.556970198075047662 ) ) ;
#17704=CARTESIAN_POINT ( 'NONE',  ( -12.60458797795435615, 0.000000000000000000, 11.86609696750642229 ) ) ;
#17705=PLANE ( 'NONE',  #48485 ) ;
#17706=VECTOR ( 'NONE', #25624, 999.9999999999998863 ) ;
#17707=VERTEX_POINT ( 'NONE', #7912 ) ;
#17708=ADVANCED_FACE ( 'NONE', ( #7601 ), #20678, .F. ) ;
#17709=DIRECTION ( 'NONE',  ( -0.6246952433987893460, -0.7422098413412802076, 0.2426528472758542054 ) ) ;
#17710=ADVANCED_FACE ( 'NONE', ( #24629 ), #34305, .F. ) ;
#17712=VECTOR ( 'NONE', #25144, 1000.000000000000114 ) ;
#17714=ORIENTED_EDGE ( 'NONE', *, *, #1624, .T. ) ;
#17715=VECTOR ( 'NONE', #3442, 1000.000000000000000 ) ;
#17716=CARTESIAN_POINT ( 'NONE',  ( -15.36424104572339289, 0.000000000000000000, 8.224833733578753581 ) ) ;
#17717=EDGE_CURVE ( 'NONE', #46531, #23582, #55883, .T. ) ;
#17718=CARTESIAN_POINT ( 'NONE',  ( -9.110551994824897193, -1.000000000000000000, 3.538847790438064411 ) ) ;
#17719=DIRECTION ( 'NONE',  ( 0.5364919789714477361, 0.6444004775717706579, 0.5449076811759711036 ) ) ;
#17720=VECTOR ( 'NONE', #9880, 999.9999999999998863 ) ;
#17721=ORIENTED_EDGE ( 'NONE', *, *, #52374, .T. ) ;
#17722=VECTOR ( 'NONE', #30377, 999.9999999999998863 ) ;
#17724=EDGE_CURVE ( 'NONE', #16052, #28453, #29476, .T. ) ;
#17725=VERTEX_POINT ( 'NONE', #41944 ) ;
#17726=ADVANCED_FACE ( 'NONE', ( #37993 ), #38844, .F. ) ;
#17727=VECTOR ( 'NONE', #51583, 999.9999999999998863 ) ;
#17728=ORIENTED_EDGE ( 'NONE', *, *, #4489, .F. ) ;
#17729=AXIS2_PLACEMENT_3D ( 'NONE', #49234, #10352, #27673 ) ;
#17730=ORIENTED_EDGE ( 'NONE', *, *, #40678, .T. ) ;
#17731=ORIENTED_EDGE ( 'NONE', *, *, #41453, .T. ) ;
#17732=LINE ( 'NONE', #38762, #40232 ) ;
#17733=ORIENTED_EDGE ( 'NONE', *, *, #8388, .T. ) ;
#17734=CARTESIAN_POINT ( 'NONE',  ( 1.086233639165236964, 0.000000000000000000, 2.796443541562362078 ) ) ;
#17735=EDGE_CURVE ( 'NONE', #25817, #9694, #50500, .T. ) ;
#17736=VERTEX_POINT ( 'NONE', #42790 ) ;
#17738=ORIENTED_EDGE ( 'NONE', *, *, #23359, .T. ) ;
#17739=DIRECTION ( 'NONE',  ( -0.6427681459581293666, -0.7660444431189770143, -0.005002170337467561935 ) ) ;
#17740=EDGE_LOOP ( 'NONE', ( #27708, #44173, #148, #14004 ) ) ;
#17741=AXIS2_PLACEMENT_3D ( 'NONE', #34453, #13450, #30500 ) ;
#17742=EDGE_CURVE ( 'NONE', #20003, #16426, #8444, .T. ) ;
#17744=AXIS2_PLACEMENT_3D ( 'NONE', #13389, #35249, #858 ) ;
#17745=LINE ( 'NONE', #34485, #4180 ) ;
#17746=DIRECTION ( 'NONE',  ( 0.007781995580012663651, 0.000000000000000000, -0.9999697198139515519 ) ) ;
#17747=LINE ( 'NONE', #9797, #35087 ) ;
#17748=CARTESIAN_POINT ( 'NONE',  ( -19.37194182085847416, -1.489407457353156827, 4.358521298522645360 ) ) ;
#17749=AXIS2_PLACEMENT_3D ( 'NONE', #17389, #8056, #43272 ) ;
#17750=EDGE_LOOP ( 'NONE', ( #28032, #9883, #44271, #30390 ) ) ;
#17751=VERTEX_POINT ( 'NONE', #33181 ) ;
#17752=DIRECTION ( 'NONE',  ( 0.007781995580012663651, -3.146120232559066537E-19, -0.9999697198139514409 ) ) ;
#17753=CARTESIAN_POINT ( 'NONE',  ( -10.23311680593447193, 0.000000000000000000, 5.679440840222505393 ) ) ;
#17754=VECTOR ( 'NONE', #32675, 1000.000000000000227 ) ;
#17755=CARTESIAN_POINT ( 'NONE',  ( -13.04747015058856618, -5.051250379848164940, 1.788240284305238070 ) ) ;
#17757=AXIS2_PLACEMENT_3D ( 'NONE', #23930, #6344, #15157 ) ;
#17758=DIRECTION ( 'NONE',  ( -0.9999697198139514409, -0.000000000000000000, -0.007781995580013368816 ) ) ;
#17759=CARTESIAN_POINT ( 'NONE',  ( -11.40636015113596180, 0.000000000000000000, 11.32142374880780089 ) ) ;
#17760=DIRECTION ( 'NONE',  ( 0.5449076811759707706, 0.6444004775717708799, -0.5364919789714476250 ) ) ;
#17762=DIRECTION ( 'NONE',  ( 0.000000000000000000, -1.000000000000000000, 0.000000000000000000 ) ) ;
#17763=PLANE ( 'NONE',  #8628 ) ;
#17764=VERTEX_POINT ( 'NONE', #51340 ) ;
#17765=AXIS2_PLACEMENT_3D ( 'NONE', #14895, #36763, #31928 ) ;
#17766=DIRECTION ( 'NONE',  ( 0.9999697198139515519, 0.000000000000000000, 0.007781995580013368816 ) ) ;
#17767=CARTESIAN_POINT ( 'NONE',  ( -12.07442007226712199, 0.000000000000000000, 3.449118973603880978 ) ) ;
#17768=VECTOR ( 'NONE', #47118, 1000.000000000000000 ) ;
#17769=VECTOR ( 'NONE', #50077, 1000.000000000000114 ) ;
#17770=EDGE_CURVE ( 'NONE', #30294, #26568, #24933, .T. ) ;
#17771=LINE ( 'NONE', #17463, #25959 ) ;
#17772=CARTESIAN_POINT ( 'NONE',  ( -12.66701627658442497, -0.1191753592594181482, 7.037824922874117206 ) ) ;
#17773=AXIS2_PLACEMENT_3D ( 'NONE', #9465, #4385, #10025 ) ;
#17774=CARTESIAN_POINT ( 'NONE',  ( -20.54049170961573267, 0.000000000000000000, 4.660556269540326646 ) ) ;
#17775=VERTEX_POINT ( 'NONE', #3623 ) ;
#17776=VECTOR ( 'NONE', #15500, 1000.000000000000227 ) ;
#17777=ORIENTED_EDGE ( 'NONE', *, *, #204, .F. ) ;
#17778=FACE_OUTER_BOUND ( 'NONE', #47424, .T. ) ;
#17779=PLANE ( 'NONE',  #24057 ) ;
#17780=CARTESIAN_POINT ( 'NONE',  ( -20.54126990917373519, -0.1191753592594197858, 4.760553241521720658 ) ) ;
#17782=CARTESIAN_POINT ( 'NONE',  ( -18.64035723371328857, -5.051250379848164940, 3.960707562635710666 ) ) ;
#17783=DIRECTION ( 'NONE',  ( 0.000000000000000000, -1.000000000000000000, 0.000000000000000000 ) ) ;
#17784=FACE_OUTER_BOUND ( 'NONE', #47978, .T. ) ;
#17785=ORIENTED_EDGE ( 'NONE', *, *, #53040, .T. ) ;
#17786=ADVANCED_FACE ( 'NONE', ( #37721 ), #7314, .F. ) ;
#17787=AXIS2_PLACEMENT_3D ( 'NONE', #18529, #24454, #12244 ) ;
#17788=LINE ( 'NONE', #987, #20529 ) ;
#17789=DIRECTION ( 'NONE',  ( 0.9999697198139515519, 0.000000000000000000, 0.007781995580013368816 ) ) ;
#17790=VERTEX_POINT ( 'NONE', #43099 ) ;
#17791=CARTESIAN_POINT ( 'NONE',  ( -10.74029228357944987, 0.000000000000000000, 11.14194120806293320 ) ) ;
#17792=ORIENTED_EDGE ( 'NONE', *, *, #52367, .F. ) ;
#17793=PLANE ( 'NONE',  #51328 ) ;
#17794=VECTOR ( 'NONE', #27373, 1000.000000000000227 ) ;
#17795=CARTESIAN_POINT ( 'NONE',  ( -18.10035294465630074, -4.889348428825659454, 11.73697724819580657 ) ) ;
#17796=EDGE_LOOP ( 'NONE', ( #15475, #37880, #5698 ) ) ;
#17797=ADVANCED_FACE ( 'NONE', ( #28913 ), #12711, .F. ) ;
#17799=ORIENTED_EDGE ( 'NONE', *, *, #23243, .F. ) ;
#17800=EDGE_CURVE ( 'NONE', #7467, #25938, #55577, .T. ) ;
#17801=ORIENTED_EDGE ( 'NONE', *, *, #36617, .F. ) ;
#17802=AXIS2_PLACEMENT_3D ( 'NONE', #46807, #47079, #42265 ) ;
#17803=VERTEX_POINT ( 'NONE', #8173 ) ;
#17804=AXIS2_PLACEMENT_3D ( 'NONE', #16836, #55721, #16255 ) ;
#17805=ORIENTED_EDGE ( 'NONE', *, *, #17022, .T. ) ;
#17807=LINE ( 'NONE', #42768, #25916 ) ;
#17808=DIRECTION ( 'NONE',  ( 0.000000000000000000, -1.000000000000000000, 0.000000000000000000 ) ) ;
#17810=AXIS2_PLACEMENT_3D ( 'NONE', #54465, #50218, #11329 ) ;
#17811=ADVANCED_FACE ( 'NONE', ( #25482 ), #3896, .F. ) ;
#17812=VECTOR ( 'NONE', #25761, 1000.000000000000227 ) ;
#17813=EDGE_LOOP ( 'NONE', ( #50122, #34671, #47693, #23003 ) ) ;
#17814=CARTESIAN_POINT ( 'NONE',  ( -20.61943528392893654, -4.079838673713161334, 4.760441806437299306 ) ) ;
#17815=EDGE_LOOP ( 'NONE', ( #38884, #34750, #45444, #29862 ) ) ;
#17816=VERTEX_POINT ( 'NONE', #30029 ) ;
#17817=AXIS2_PLACEMENT_3D ( 'NONE', #20776, #55143, #42371 ) ;
#17818=EDGE_CURVE ( 'NONE', #29996, #7048, #38554, .T. ) ;
#17819=VECTOR ( 'NONE', #46364, 1000.000000000000227 ) ;
#17820=CARTESIAN_POINT ( 'NONE',  ( -8.875996589204540044, 0.000000000000000000, 10.41778544861944233 ) ) ;
#17821=DIRECTION ( 'NONE',  ( 0.6427681459581294776, -0.7660444431189769032, 0.005002170337467562802 ) ) ;
#17822=FACE_OUTER_BOUND ( 'NONE', #16800, .T. ) ;
#17823=EDGE_LOOP ( 'NONE', ( #9827, #50233, #13075, #2421 ) ) ;
#17824=DIRECTION ( 'NONE',  ( -0.9999697198139514409, -0.000000000000000000, -0.007781995580013368816 ) ) ;
#17825=ORIENTED_EDGE ( 'NONE', *, *, #12944, .T. ) ;
#17826=CARTESIAN_POINT ( 'NONE',  ( -21.70925593905789341, -5.375054281893165253, 5.142441000255496775 ) ) ;
#17827=CARTESIAN_POINT ( 'NONE',  ( -1.148446742091705719, -6.446785546503744690, 3.664469291707747267 ) ) ;
#17828=VECTOR ( 'NONE', #14627, 1000.000000000000227 ) ;
#17829=DIRECTION ( 'NONE',  ( 0.9999697198139515519, 0.000000000000000000, 0.007781995580013368816 ) ) ;
#17830=FACE_OUTER_BOUND ( 'NONE', #35906, .T. ) ;
#17831=DIRECTION ( 'NONE',  ( 0.5449076811759707706, 0.6444004775717708799, -0.5364919789714476250 ) ) ;
#17832=FACE_OUTER_BOUND ( 'NONE', #17074, .T. ) ;
#17833=CARTESIAN_POINT ( 'NONE',  ( -19.22961988024793101, -0.1191753592594177458, 14.39986392600063603 ) ) ;
#17835=LINE ( 'NONE', #52179, #41924 ) ;
#17836=VECTOR ( 'NONE', #21609, 1000.000000000000227 ) ;
#17837=EDGE_CURVE ( 'NONE', #54540, #20884, #33450, .T. ) ;
#17838=DIRECTION ( 'NONE',  ( 0.005002170337468016433, -0.7660444431189770143, -0.6427681459581293666 ) ) ;
#17839=FACE_OUTER_BOUND ( 'NONE', #29934, .T. ) ;
#17840=VECTOR ( 'NONE', #35569, 999.9999999999998863 ) ;
#17841=DIRECTION ( 'NONE',  ( -0.005961354470445682716, -0.6427876096865404731, 0.7660212471507180654 ) ) ;
#17842=EDGE_CURVE ( 'NONE', #41679, #39446, #35696, .T. ) ;
#17844=FACE_OUTER_BOUND ( 'NONE', #36144, .T. ) ;
#17845=CARTESIAN_POINT ( 'NONE',  ( -17.93139508144814442, 0.000000000000000000, 13.85596890686001537 ) ) ;
#17846=VECTOR ( 'NONE', #16625, 1000.000000000000114 ) ;
#17847=DIRECTION ( 'NONE',  ( -0.5449076811759708816, 0.6444004775717707689, 0.5364919789714475140 ) ) ;
#17848=ADVANCED_FACE ( 'NONE', ( #30866 ), #44227, .F. ) ;
#17849=VERTEX_POINT ( 'NONE', #9869 ) ;
#17850=EDGE_CURVE ( 'NONE', #1909, #49895, #22069, .T. ) ;
#17851=CARTESIAN_POINT ( 'NONE',  ( -14.89673009537702697, 0.000000000000000000, 7.859139942088997799 ) ) ;
#17852=CARTESIAN_POINT ( 'NONE',  ( -12.97782006657300258, 4.657758921906509642, 9.566523066637216743 ) ) ;
#17853=PLANE ( 'NONE',  #23681 ) ;
#17854=ADVANCED_FACE ( 'NONE', ( #17830 ), #39945, .F. ) ;
#17855=EDGE_CURVE ( 'NONE', #34917, #44182, #26322, .T. ) ;
#17856=EDGE_CURVE ( 'NONE', #49471, #46628, #22374, .T. ) ;
#17857=VECTOR ( 'NONE', #23940, 1000.000000000000114 ) ;
#17858=LINE ( 'NONE', #25798, #34568 ) ;
#17859=CARTESIAN_POINT ( 'NONE',  ( -2.056461029976381472, 6.659969651376628441, 4.017172877417169552 ) ) ;
#17860=CARTESIAN_POINT ( 'NONE',  ( -27.06552663992790997, 0.000000000000000000, 7.195101427592543786 ) ) ;
#17861=CARTESIAN_POINT ( 'NONE',  ( 2.072287782118878319, 0.000000000000000000, -2.950529333540147015 ) ) ;
#17862=VECTOR ( 'NONE', #45109, 1000.000000000000227 ) ;
#17863=VECTOR ( 'NONE', #28430, 999.9999999999998863 ) ;
#17864=DIRECTION ( 'NONE',  ( -0.005002170337468016433, -0.7660444431189770143, 0.6427681459581293666 ) ) ;
#17865=LINE ( 'NONE', #35730, #35592 ) ;
#17866=VERTEX_POINT ( 'NONE', #182 ) ;
#17867=ADVANCED_FACE ( 'NONE', ( #35160 ), #39690, .F. ) ;
#17868=AXIS2_PLACEMENT_3D ( 'NONE', #46027, #15103, #10576 ) ;
#17869=EDGE_CURVE ( 'NONE', #17442, #47891, #53014, .T. ) ;
#17870=VERTEX_POINT ( 'NONE', #769 ) ;
#17871=EDGE_LOOP ( 'NONE', ( #52931, #33939, #1916, #16372 ) ) ;
#17873=EDGE_CURVE ( 'NONE', #13581, #2493, #44478, .T. ) ;
#17874=ORIENTED_EDGE ( 'NONE', *, *, #43846, .F. ) ;
#17875=CARTESIAN_POINT ( 'NONE',  ( -11.64230387957660007, -1.165603555308156514, 1.366398462294132532 ) ) ;
#17876=DIRECTION ( 'NONE',  ( -0.9999697198139514409, -0.000000000000000000, -0.007781995580013368816 ) ) ;
#17877=ADVANCED_FACE ( 'NONE', ( #22910 ), #17527, .F. ) ;
#17878=ORIENTED_EDGE ( 'NONE', *, *, #50465, .T. ) ;
#17879=VECTOR ( 'NONE', #7495, 1000.000000000000000 ) ;
#17880=ORIENTED_EDGE ( 'NONE', *, *, #41307, .F. ) ;
#17881=VECTOR ( 'NONE', #39638, 1000.000000000000227 ) ;
#17882=DIRECTION ( 'NONE',  ( -0.005961354470445682716, -0.6427876096865404731, 0.7660212471507180654 ) ) ;
#17883=EDGE_LOOP ( 'NONE', ( #40277, #37006, #30604, #53981 ) ) ;
#17884=CARTESIAN_POINT ( 'NONE',  ( -18.27257916373564228, 1.581621852479005552, 6.574722315692204333 ) ) ;
#17885=FACE_OUTER_BOUND ( 'NONE', #48939, .T. ) ;
#17886=EDGE_CURVE ( 'NONE', #46046, #31141, #30618, .T. ) ;
#17887=ORIENTED_EDGE ( 'NONE', *, *, #9094, .T. ) ;
#17888=PLANE ( 'NONE',  #24770 ) ;
#17889=ORIENTED_EDGE ( 'NONE', *, *, #36821, .F. ) ;
#17890=VECTOR ( 'NONE', #30315, 999.9999999999998863 ) ;
#17891=CARTESIAN_POINT ( 'NONE',  ( -18.67062061514484483, -0.1191753592594160666, 9.576427974360404605 ) ) ;
#17892=LINE ( 'NONE', #53620, #35474 ) ;
#17893=DIRECTION ( 'NONE',  ( 0.7660212471507180654, -0.6427876096865404731, 0.005961354470445141482 ) ) ;
#17894=VECTOR ( 'NONE', #20828, 999.9999999999998863 ) ;
#17895=ORIENTED_EDGE ( 'NONE', *, *, #33598, .T. ) ;
#17896=FACE_OUTER_BOUND ( 'NONE', #31112, .T. ) ;
#17897=CARTESIAN_POINT ( 'NONE',  ( -14.00280974873554030, 0.000000000000000000, 12.40921378708904044 ) ) ;
#17898=CARTESIAN_POINT ( 'NONE',  ( -14.93495759592298988, 0.000000000000000000, 12.77129166681078409 ) ) ;
#17899=ORIENTED_EDGE ( 'NONE', *, *, #55593, .T. ) ;
#17901=VERTEX_POINT ( 'NONE', #17239 ) ;
#17902=LINE ( 'NONE', #22446, #19287 ) ;
#17903=LINE ( 'NONE', #43701, #40535 ) ;
#17904=DIRECTION ( 'NONE',  ( -0.005961354470445682716, -0.6427876096865404731, 0.7660212471507180654 ) ) ;
#17906=CARTESIAN_POINT ( 'NONE',  ( -11.67244013076689946, 0.000000000000000000, 11.50401908778467863 ) ) ;
#17907=DIRECTION ( 'NONE',  ( 0.005002170337468016433, -0.7660444431189770143, -0.6427681459581293666 ) ) ;
#17908=PLANE ( 'NONE',  #47017 ) ;
#17909=FACE_OUTER_BOUND ( 'NONE', #17434, .T. ) ;
#17910=DIRECTION ( 'NONE',  ( 0.005002170337468016433, -0.7660444431189770143, -0.6427681459581293666 ) ) ;
#17911=ORIENTED_EDGE ( 'NONE', *, *, #5531, .T. ) ;
#17912=FACE_OUTER_BOUND ( 'NONE', #6209, .T. ) ;
#17913=CARTESIAN_POINT ( 'NONE',  ( -12.60458797795435615, 0.000000000000000000, 11.86609696750642229 ) ) ;
#17914=LINE ( 'NONE', #52535, #35989 ) ;
#17915=EDGE_CURVE ( 'NONE', #30544, #36108, #13820, .T. ) ;
#17916=EDGE_CURVE ( 'NONE', #31662, #29422, #12993, .T. ) ;
#17917=LINE ( 'NONE', #52801, #995 ) ;
#17918=ADVANCED_FACE ( 'NONE', ( #43383 ), #4478, .F. ) ;
#17919=DIRECTION ( 'NONE',  ( 0.007781995580012663651, -3.146120232559066537E-19, -0.9999697198139514409 ) ) ;
#17921=VERTEX_POINT ( 'NONE', #52173 ) ;
#17922=VECTOR ( 'NONE', #33899, 1000.000000000000227 ) ;
#17923=VERTEX_POINT ( 'NONE', #13289 ) ;
#17924=DIRECTION ( 'NONE',  ( -0.6427681459581293666, -0.7660444431189770143, -0.005002170337467561935 ) ) ;
#17925=DIRECTION ( 'NONE',  ( 0.6427681459581294776, -0.7660444431189769032, 0.005002170337467562802 ) ) ;
#17927=VECTOR ( 'NONE', #50051, 1000.000000000000227 ) ;
#17928=ORIENTED_EDGE ( 'NONE', *, *, #51577, .F. ) ;
#17930=ORIENTED_EDGE ( 'NONE', *, *, #16034, .F. ) ;
#17931=LINE ( 'NONE', #35254, #27474 ) ;
#17932=EDGE_CURVE ( 'NONE', #38002, #50731, #47921, .T. ) ;
#17933=ORIENTED_EDGE ( 'NONE', *, *, #26576, .T. ) ;
#17934=ORIENTED_EDGE ( 'NONE', *, *, #42322, .T. ) ;
#17935=EDGE_LOOP ( 'NONE', ( #48636, #52793, #38205, #19238 ) ) ;
#17936=EDGE_CURVE ( 'NONE', #11344, #30222, #43635, .T. ) ;
#17937=FACE_OUTER_BOUND ( 'NONE', #11276, .T. ) ;
#17938=CARTESIAN_POINT ( 'NONE',  ( -28.93137873341882127, 0.000000000000000000, 8.119251130998824451 ) ) ;
#17940=EDGE_CURVE ( 'NONE', #32323, #25140, #3208, .T. ) ;
#17941=CARTESIAN_POINT ( 'NONE',  ( -12.15193928448664629, -0.1191753592594197858, 1.501852324026012209 ) ) ;
#17942=ORIENTED_EDGE ( 'NONE', *, *, #37587, .F. ) ;
#17943=VERTEX_POINT ( 'NONE', #1868 ) ;
#17944=CARTESIAN_POINT ( 'NONE',  ( -16.96389378722000529, 0.000000000000000000, 8.951049005674249770 ) ) ;
#17945=ORIENTED_EDGE ( 'NONE', *, *, #46452, .F. ) ;
#17946=DIRECTION ( 'NONE',  ( 0.005961354470445682716, -0.6427876096865404731, -0.7660212471507180654 ) ) ;
#17947=EDGE_CURVE ( 'NONE', #34394, #24292, #29332, .T. ) ;
#17949=DIRECTION ( 'NONE',  ( -0.5364919789714478471, 0.6444004775717705469, -0.5449076811759709926 ) ) ;
#17950=ORIENTED_EDGE ( 'NONE', *, *, #21508, .F. ) ;
#17951=CARTESIAN_POINT ( 'NONE',  ( -12.10724190330752315, -2.784623065533159636, 5.954836501472268395 ) ) ;
#17952=ORIENTED_EDGE ( 'NONE', *, *, #15636, .T. ) ;
#17953=CARTESIAN_POINT ( 'NONE',  ( 2.072287782118878319, 0.000000000000000000, -2.950529333540147015 ) ) ;
#17954=ORIENTED_EDGE ( 'NONE', *, *, #9197, .F. ) ;
#17955=DIRECTION ( 'NONE',  ( 0.007781995580012663651, 0.000000000000000000, -0.9999697198139515519 ) ) ;
#17956=CARTESIAN_POINT ( 'NONE',  ( -17.31338524499528830, -0.1191753592594166911, 7.001665805194019043 ) ) ;
#17957=DIRECTION ( 'NONE',  ( -0.7660212471507179544, -0.6427876096865405842, -0.005961354470445141482 ) ) ;
#17958=ORIENTED_EDGE ( 'NONE', *, *, #18569, .T. ) ;
#17959=DIRECTION ( 'NONE',  ( -0.9999697198139514409, -0.000000000000000000, -0.007781995580013368816 ) ) ;
#17960=VECTOR ( 'NONE', #55176, 1000.000000000000227 ) ;
#17961=DIRECTION ( 'NONE',  ( 0.7660212471507180654, -0.6427876096865404731, 0.005961354470445141482 ) ) ;
#17963=DIRECTION ( 'NONE',  ( 0.007781995580012663651, 0.000000000000000000, -0.9999697198139515519 ) ) ;
#17964=DIRECTION ( 'NONE',  ( -0.5364919789714478471, 0.6444004775717705469, -0.5449076811759709926 ) ) ;
#17965=DIRECTION ( 'NONE',  ( 0.005961354470445682716, -0.6427876096865404731, -0.7660212471507180654 ) ) ;
#17966=DIRECTION ( 'NONE',  ( 0.007781995580012663651, -3.146120232559066537E-19, -0.9999697198139514409 ) ) ;
#17967=ORIENTED_EDGE ( 'NONE', *, *, #48078, .F. ) ;
#17968=DIRECTION ( 'NONE',  ( 0.007781995580012663651, -3.146120232559066537E-19, -0.9999697198139514409 ) ) ;
#17969=LINE ( 'NONE', #27601, #22269 ) ;
#17970=CARTESIAN_POINT ( 'NONE',  ( -12.15116108492864377, 0.000000000000000000, 1.401855352044617975 ) ) ;
#17971=EDGE_LOOP ( 'NONE', ( #26079, #31342, #31967, #55911 ) ) ;
#17972=DIRECTION ( 'NONE',  ( 0.000000000000000000, -1.000000000000000000, 0.000000000000000000 ) ) ;
#17973=DIRECTION ( 'NONE',  ( 0.5364919789714477361, 0.6444004775717706579, 0.5449076811759711036 ) ) ;
#17974=VERTEX_POINT ( 'NONE', #31990 ) ;
#17975=EDGE_CURVE ( 'NONE', #44387, #41818, #27752, .T. ) ;
#17976=DIRECTION ( 'NONE',  ( -0.6427681459581293666, -0.7660444431189770143, -0.005002170337467561935 ) ) ;
#17977=FACE_OUTER_BOUND ( 'NONE', #9798, .T. ) ;
#17978=EDGE_CURVE ( 'NONE', #29379, #15700, #14665, .T. ) ;
#17979=EDGE_CURVE ( 'NONE', #6764, #6080, #44768, .T. ) ;
#17980=PLANE ( 'NONE',  #35996 ) ;
#17981=CARTESIAN_POINT ( 'NONE',  ( 2.072287782118878319, 0.000000000000000000, -2.950529333540147015 ) ) ;
#17982=ORIENTED_EDGE ( 'NONE', *, *, #13399, .T. ) ;
#17983=ORIENTED_EDGE ( 'NONE', *, *, #31276, .T. ) ;
#17984=CARTESIAN_POINT ( 'NONE',  ( -23.33849165029409889, 0.000000000000000000, 5.946783852668351855 ) ) ;
#17985=LINE ( 'NONE', #25957, #21386 ) ;
#17986=CARTESIAN_POINT ( 'NONE',  ( -27.99923088623136636, 0.000000000000000000, 7.757173251277078130 ) ) ;
#17987=PLANE ( 'NONE',  #54689 ) ;
#17988=FACE_OUTER_BOUND ( 'NONE', #53481, .T. ) ;
#17989=DIRECTION ( 'NONE',  ( 0.9999697198139515519, 0.000000000000000000, 0.007781995580013368816 ) ) ;
#17990=ORIENTED_EDGE ( 'NONE', *, *, #40746, .T. ) ;
#17991=CARTESIAN_POINT ( 'NONE',  ( -12.80458192191714595, 0.000000000000000000, 11.86454056839041726 ) ) ;
#17992=LINE ( 'NONE', #35314, #21525 ) ;
#17993=VERTEX_POINT ( 'NONE', #11463 ) ;
#17994=LINE ( 'NONE', #35317, #20206 ) ;
#17995=PLANE ( 'NONE',  #36865 ) ;
#17996=DIRECTION ( 'NONE',  ( -0.7660212471507179544, -0.6427876096865405842, -0.005961354470445141482 ) ) ;
#17997=ORIENTED_EDGE ( 'NONE', *, *, #11645, .F. ) ;
#18000=EDGE_LOOP ( 'NONE', ( #31694, #35953, #51324, #25354 ) ) ;
#18001=EDGE_CURVE ( 'NONE', #19601, #24549, #40537, .T. ) ;
#18002=EDGE_LOOP ( 'NONE', ( #42098, #30789, #21038, #9809 ) ) ;
#18003=ORIENTED_EDGE ( 'NONE', *, *, #34292, .T. ) ;
#18004=EDGE_CURVE ( 'NONE', #28250, #7109, #6177, .T. ) ;
#18005=VERTEX_POINT ( 'NONE', #7462 ) ;
#18007=ORIENTED_EDGE ( 'NONE', *, *, #35287, .F. ) ;
#18008=CARTESIAN_POINT ( 'NONE',  ( -21.41954753101251541, 3.686347215771511365, 4.884397627102543105 ) ) ;
#18009=ORIENTED_EDGE ( 'NONE', *, *, #10796, .T. ) ;
#18010=CARTESIAN_POINT ( 'NONE',  ( -19.60834386242827776, 0.000000000000000000, 4.298478389818581213 ) ) ;
#18011=EDGE_CURVE ( 'NONE', #1435, #22163, #7763, .T. ) ;
#18012=ORIENTED_EDGE ( 'NONE', *, *, #35250, .F. ) ;
#18013=PLANE ( 'NONE',  #4775 ) ;
#18014=EDGE_LOOP ( 'NONE', ( #6191, #7480, #18646, #23341 ) ) ;
#18015=DIRECTION ( 'NONE',  ( 0.5364919789714477361, 0.6444004775717706579, 0.5449076811759711036 ) ) ;
#18016=CARTESIAN_POINT ( 'NONE',  ( -14.20280369269832832, 0.000000000000000000, 12.40765738797303719 ) ) ;
#18017=CARTESIAN_POINT ( 'NONE',  ( -15.79570695489036858, 0.000000000000000000, 3.958817142012544643 ) ) ;
#18019=DIRECTION ( 'NONE',  ( -0.005002170337468016433, -0.7660444431189770143, 0.6427681459581293666 ) ) ;
#18020=CARTESIAN_POINT ( 'NONE',  ( -24.26908309836554878, 0.000000000000000000, 6.108867788427308376 ) ) ;
#18021=VERTEX_POINT ( 'NONE', #10424 ) ;
#18022=ORIENTED_EDGE ( 'NONE', *, *, #30731, .T. ) ;
#18023=FACE_OUTER_BOUND ( 'NONE', #39228, .T. ) ;
#18024=CARTESIAN_POINT ( 'NONE',  ( 2.072287782118878319, 0.000000000000000000, -2.950529333540147015 ) ) ;
#18025=EDGE_CURVE ( 'NONE', #16374, #37342, #42102, .T. ) ;
#18026=FACE_OUTER_BOUND ( 'NONE', #18000, .T. ) ;
#18027=DIRECTION ( 'NONE',  ( 0.9999697198139515519, 0.000000000000000000, 0.007781995580013368816 ) ) ;
#18028=LINE ( 'NONE', #16924, #41267 ) ;
#18029=DIRECTION ( 'NONE',  ( -0.005961354470445682716, -0.6427876096865404731, 0.7660212471507180654 ) ) ;
#18030=VERTEX_POINT ( 'NONE', #37568 ) ;
#18031=LINE ( 'NONE', #15185, #33837 ) ;
#18032=EDGE_CURVE ( 'NONE', #6272, #32386, #24495, .T. ) ;
#18033=LINE ( 'NONE', #30558, #55800 ) ;
#18034=ORIENTED_EDGE ( 'NONE', *, *, #50894, .T. ) ;
#18035=CARTESIAN_POINT ( 'NONE',  ( -17.23428484710887076, 0.000000000000000000, 9.687608899537771379 ) ) ;
#18036=CARTESIAN_POINT ( 'NONE',  ( -16.99361711142231002, -3.594132820645660420, 9.181413994056926597 ) ) ;
#18037=EDGE_CURVE ( 'NONE', #14582, #19374, #54584, .T. ) ;
#18039=EDGE_CURVE ( 'NONE', #32268, #40689, #28788, .T. ) ;
#18041=FACE_OUTER_BOUND ( 'NONE', #1610, .T. ) ;
#18042=ORIENTED_EDGE ( 'NONE', *, *, #23519, .T. ) ;
#18043=ORIENTED_EDGE ( 'NONE', *, *, #33107, .T. ) ;
#18044=DIRECTION ( 'NONE',  ( 0.5364919789714477361, 0.6444004775717706579, 0.5449076811759711036 ) ) ;
#18046=CARTESIAN_POINT ( 'NONE',  ( -8.926160398992163181, -0.1191753592594191058, 4.013552926324940096 ) ) ;
#18049=CARTESIAN_POINT ( 'NONE',  ( -16.49063472986307843, 0.000000000000000000, 7.846735807668965279 ) ) ;
#18050=CARTESIAN_POINT ( 'NONE',  ( -19.65599895527812890, 3.200641362704007786, 9.769176383365808292 ) ) ;
#18052=DIRECTION ( 'NONE',  ( 0.9999697198139515519, 0.000000000000000000, 0.007781995580013368816 ) ) ;
#18053=EDGE_CURVE ( 'NONE', #51694, #55479, #46945, .T. ) ;
#18054=DIRECTION ( 'NONE',  ( -0.005002170337468016433, -0.7660444431189770143, 0.6427681459581293666 ) ) ;
#18055=DIRECTION ( 'NONE',  ( -0.9999697198139514409, -0.000000000000000000, -0.007781995580013368816 ) ) ;
#18056=VERTEX_POINT ( 'NONE', #3758 ) ;
#18057=DIRECTION ( 'NONE',  ( -0.7660212471507179544, -0.6427876096865405842, -0.005961354470445141482 ) ) ;
#18058=ORIENTED_EDGE ( 'NONE', *, *, #39584, .F. ) ;
#18059=CARTESIAN_POINT ( 'NONE',  ( -17.99516527612767192, -2.622721114510662144, 3.787575893809204342 ) ) ;
#18060=DIRECTION ( 'NONE',  ( 0.5449076811759707706, 0.6444004775717708799, -0.5364919789714476250 ) ) ;
#18061=ORIENTED_EDGE ( 'NONE', *, *, #38030, .T. ) ;
#18062=CARTESIAN_POINT ( 'NONE',  ( -14.40179626436711224, 0.000000000000000000, 3.969664877316573914 ) ) ;
#18063=ORIENTED_EDGE ( 'NONE', *, *, #22890, .F. ) ;
#18064=ORIENTED_EDGE ( 'NONE', *, *, #44136, .T. ) ;
#18065=ORIENTED_EDGE ( 'NONE', *, *, #30357, .T. ) ;
#18066=DIRECTION ( 'NONE',  ( -0.9999697198139514409, -0.000000000000000000, -0.007781995580013368816 ) ) ;
#18067=ORIENTED_EDGE ( 'NONE', *, *, #3784, .T. ) ;
#18068=VERTEX_POINT ( 'NONE', #42949 ) ;
#18069=LINE ( 'NONE', #25460, #50141 ) ;
#18070=PLANE ( 'NONE',  #51228 ) ;
#18071=ORIENTED_EDGE ( 'NONE', *, *, #33660, .F. ) ;
#18072=ORIENTED_EDGE ( 'NONE', *, *, #14279, .F. ) ;
#18073=DIRECTION ( 'NONE',  ( -0.005002170337468016433, -0.7660444431189770143, 0.6427681459581293666 ) ) ;
#18074=EDGE_CURVE ( 'NONE', #29764, #48603, #17377, .T. ) ;
#18075=ORIENTED_EDGE ( 'NONE', *, *, #32208, .F. ) ;
#18076=ORIENTED_EDGE ( 'NONE', *, *, #22942, .T. ) ;
#18077=CARTESIAN_POINT ( 'NONE',  ( -13.07066190154808361, 0.000000000000000000, 12.04713590736729678 ) ) ;
#18078=FACE_OUTER_BOUND ( 'NONE', #38229, .T. ) ;
#18079=LINE ( 'NONE', #18654, #49499 ) ;
#18080=ORIENTED_EDGE ( 'NONE', *, *, #44809, .T. ) ;
#18081=DIRECTION ( 'NONE',  ( 0.000000000000000000, -1.000000000000000000, 0.000000000000000000 ) ) ;
#18082=ORIENTED_EDGE ( 'NONE', *, *, #24523, .T. ) ;
#18083=EDGE_CURVE ( 'NONE', #30276, #32205, #12850, .T. ) ;
#18084=LINE ( 'NONE', #47634, #42042 ) ;
#18085=EDGE_CURVE ( 'NONE', #36877, #31801, #3496, .T. ) ;
#18086=EDGE_CURVE ( 'NONE', #24619, #32474, #52327, .T. ) ;
#18087=CARTESIAN_POINT ( 'NONE',  ( 2.072287782118878319, 0.000000000000000000, -2.950529333540147015 ) ) ;
#18088=CARTESIAN_POINT ( 'NONE',  ( -13.08330893211609869, 0.000000000000000000, 1.763933231766363630 ) ) ;
#18089=DIRECTION ( 'NONE',  ( 0.5449076811759707706, 0.6444004775717708799, -0.5364919789714476250 ) ) ;
#18090=DIRECTION ( 'NONE',  ( 0.000000000000000000, -0.000000000000000000, -1.000000000000000000 ) ) ;
#18092=CARTESIAN_POINT ( 'NONE',  ( -12.75629523410269250, 0.000000000000000000, 5.659804882266454840 ) ) ;
#18093=EDGE_LOOP ( 'NONE', ( #41722, #22806, #6474, #12934 ) ) ;
#18094=DIRECTION ( 'NONE',  ( -0.5364919789714478471, 0.6444004775717705469, -0.5449076811759709926 ) ) ;
#18095=DIRECTION ( 'NONE',  ( -0.5364919789714478471, 0.6444004775717705469, -0.5449076811759709926 ) ) ;
#18097=EDGE_CURVE ( 'NONE', #34435, #21097, #47199, .T. ) ;
#18098=LINE ( 'NONE', #13003, #52586 ) ;
#18100=CARTESIAN_POINT ( 'NONE',  ( -16.81190032086591302, 0.000000000000000000, 3.212244750653343583 ) ) ;
#18101=EDGE_CURVE ( 'NONE', #8803, #15538, #4054, .T. ) ;
#18102=DIRECTION ( 'NONE',  ( 0.007781995580012662783, 0.000000000000000000, -0.9999697198139514409 ) ) ;
#18104=ORIENTED_EDGE ( 'NONE', *, *, #45168, .T. ) ;
#18105=CARTESIAN_POINT ( 'NONE',  ( -14.94916102560700821, 0.000000000000000000, 2.688082935172642962 ) ) ;
#18106=CARTESIAN_POINT ( 'NONE',  ( -19.05103928628325605, 0.000000000000000000, 4.302815462894245435 ) ) ;
#18107=CARTESIAN_POINT ( 'NONE',  ( -13.73672976910459909, 0.000000000000000000, 12.22661844811216270 ) ) ;
#18108=EDGE_CURVE ( 'NONE', #21115, #54376, #43259, .T. ) ;
#18109=LINE ( 'NONE', #17324, #32014 ) ;
#18110=LINE ( 'NONE', #43125, #49955 ) ;
#18111=CARTESIAN_POINT ( 'NONE',  ( -19.96464863903120346, -4.889348428825662118, 12.46113300763930098 ) ) ;
#18113=CARTESIAN_POINT ( 'NONE',  ( -14.94916102560700821, 0.000000000000000000, 2.688082935172642962 ) ) ;
#18114=EDGE_CURVE ( 'NONE', #24756, #16295, #25932, .T. ) ;
#18115=DIRECTION ( 'NONE',  ( 0.000000000000000000, 1.000000000000000000, 0.000000000000000000 ) ) ;
#18116=LINE ( 'NONE', #22406, #38296 ) ;
#18117=ORIENTED_EDGE ( 'NONE', *, *, #9572, .F. ) ;
#18118=ORIENTED_EDGE ( 'NONE', *, *, #19703, .T. ) ;
#18119=VERTEX_POINT ( 'NONE', #8305 ) ;
#18120=ORIENTED_EDGE ( 'NONE', *, *, #27082, .F. ) ;
#18121=ORIENTED_EDGE ( 'NONE', *, *, #15753, .T. ) ;
#18122=CARTESIAN_POINT ( 'NONE',  ( 2.072287782118878319, 0.000000000000000000, -2.950529333540147015 ) ) ;
#18123=CARTESIAN_POINT ( 'NONE',  ( -13.66288791392935664, 1.095915999411505082, 3.987035636642269232 ) ) ;
#18124=ORIENTED_EDGE ( 'NONE', *, *, #37193, .T. ) ;
#18125=ORIENTED_EDGE ( 'NONE', *, *, #55945, .F. ) ;
#18126=ADVANCED_FACE ( 'NONE', ( #21382 ), #56028, .F. ) ;
#18127=VECTOR ( 'NONE', #31693, 1000.000000000000227 ) ;
#18128=PLANE ( 'NONE',  #15783 ) ;
#18129=ORIENTED_EDGE ( 'NONE', *, *, #18404, .T. ) ;
#18130=CARTESIAN_POINT ( 'NONE',  ( -10.27421835998572064, 0.000000000000000000, 10.96090226820206048 ) ) ;
#18131=LINE ( 'NONE', #26657, #54970 ) ;
#18132=ORIENTED_EDGE ( 'NONE', *, *, #26813, .F. ) ;
#18133=DIRECTION ( 'NONE',  ( 0.6427681459581294776, -0.7660444431189769032, 0.005002170337467562802 ) ) ;
#18134=EDGE_CURVE ( 'NONE', #9163, #13086, #26202, .T. ) ;
#18135=EDGE_CURVE ( 'NONE', #48012, #19489, #336, .T. ) ;
#18136=ADVANCED_FACE ( 'NONE', ( #29900 ), #39245, .F. ) ;
#18137=VERTEX_POINT ( 'NONE', #8046 ) ;
#18138=DIRECTION ( 'NONE',  ( 0.9999697198139515519, 0.000000000000000000, 0.007781995580013368816 ) ) ;
#18139=LINE ( 'NONE', #35462, #6628 ) ;
#18140=EDGE_CURVE ( 'NONE', #50938, #9324, #4605, .T. ) ;
#18141=LINE ( 'NONE', #22686, #9173 ) ;
#18142=LINE ( 'NONE', #53898, #18785 ) ;
#18143=EDGE_LOOP ( 'NONE', ( #22445, #44035, #54547, #26575, #25537 ) ) ;
#18144=LINE ( 'NONE', #31210, #49401 ) ;
#18145=DIRECTION ( 'NONE',  ( 0.005961354470445682716, -0.6427876096865404731, -0.7660212471507180654 ) ) ;
#18146=DIRECTION ( 'NONE',  ( 0.005961354470445682716, -0.6427876096865404731, -0.7660212471507180654 ) ) ;
#18147=EDGE_LOOP ( 'NONE', ( #15231, #33732, #38, #42439 ) ) ;
#18148=DIRECTION ( 'NONE',  ( 0.007781995580012663651, -3.146120232559066537E-19, -0.9999697198139514409 ) ) ;
#18149=ORIENTED_EDGE ( 'NONE', *, *, #29832, .F. ) ;
#18150=DIRECTION ( 'NONE',  ( -0.005961354470445682716, -0.6427876096865404731, 0.7660212471507180654 ) ) ;
#18151=CARTESIAN_POINT ( 'NONE',  ( -14.94760462649100496, 0.000000000000000000, 2.488088991209854051 ) ) ;
#18152=DIRECTION ( 'NONE',  ( -0.5449076811759708816, 0.6444004775717707689, 0.5364919789714475140 ) ) ;
#18153=ADVANCED_FACE ( 'NONE', ( #12583 ), #17676, .F. ) ;
#18154=DIRECTION ( 'NONE',  ( 0.9999697198139515519, 0.000000000000000000, 0.007781995580013368816 ) ) ;
#18155=DIRECTION ( 'NONE',  ( 0.005961354470445682716, -0.6427876096865404731, -0.7660212471507180654 ) ) ;
#18156=CARTESIAN_POINT ( 'NONE',  ( -18.67619601524082285, 0.000000000000000000, 3.936400510096834893 ) ) ;
#18157=CARTESIAN_POINT ( 'NONE',  ( -32.10901097986136676, 0.000000000000000000, 16.76339505873265168 ) ) ;
#18158=EDGE_CURVE ( 'NONE', #29543, #30294, #13430, .T. ) ;
#18159=CARTESIAN_POINT ( 'NONE',  ( -15.40103151951671734, 0.000000000000000000, 12.95233060667165681 ) ) ;
#18160=EDGE_CURVE ( 'NONE', #29959, #38766, #42405, .T. ) ;
#18161=FACE_OUTER_BOUND ( 'NONE', #44376, .T. ) ;
#18162=VERTEX_POINT ( 'NONE', #38124 ) ;
#18163=CARTESIAN_POINT ( 'NONE',  ( -8.509919637592204822, -0.1191753592594197858, 10.23596830920056711 ) ) ;
#18164=CARTESIAN_POINT ( 'NONE',  ( -15.03495456790438389, -0.1191753592594197858, 12.77051346725278158 ) ) ;
#18165=CARTESIAN_POINT ( 'NONE',  ( -20.54049170961573267, 0.000000000000000000, 4.660556269540326646 ) ) ;
#18166=CARTESIAN_POINT ( 'NONE',  ( -9.405935838180976560, -0.1191753592594177180, 5.955207195476888593 ) ) ;
#18167=EDGE_CURVE ( 'NONE', #17707, #27553, #25357, .T. ) ;
#18170=PLANE ( 'NONE',  #32889 ) ;
#18171=ORIENTED_EDGE ( 'NONE', *, *, #52909, .F. ) ;
#18173=ORIENTED_EDGE ( 'NONE', *, *, #41247, .T. ) ;
#18175=DIRECTION ( 'NONE',  ( 0.5364919789714477361, 0.6444004775717706579, 0.5449076811759711036 ) ) ;
#18176=ORIENTED_EDGE ( 'NONE', *, *, #23411, .F. ) ;
#18178=ORIENTED_EDGE ( 'NONE', *, *, #7626, .T. ) ;
#18179=DIRECTION ( 'NONE',  ( -0.9999697198139514409, -0.000000000000000000, -0.007781995580013368816 ) ) ;
#18180=ORIENTED_EDGE ( 'NONE', *, *, #27748, .T. ) ;
#18181=VERTEX_POINT ( 'NONE', #19058 ) ;
#18182=ORIENTED_EDGE ( 'NONE', *, *, #14467, .T. ) ;
#18183=LINE ( 'NONE', #30963, #53784 ) ;
#18185=CARTESIAN_POINT ( 'NONE',  ( -18.58296605579292660, -5.536956232915664522, 3.922918320456664887 ) ) ;
#18186=EDGE_CURVE ( 'NONE', #2789, #38090, #31589, .T. ) ;
#18187=DIRECTION ( 'NONE',  ( 0.007781995580012663651, 0.000000000000000000, -0.9999697198139515519 ) ) ;
#18189=EDGE_CURVE ( 'NONE', #50687, #41455, #39816, .T. ) ;
#18190=ORIENTED_EDGE ( 'NONE', *, *, #41391, .T. ) ;
#18191=DIRECTION ( 'NONE',  ( 0.5364919789714477361, 0.6444004775717706579, 0.5449076811759711036 ) ) ;
#18192=ORIENTED_EDGE ( 'NONE', *, *, #37397, .T. ) ;
#18193=LINE ( 'NONE', #44592, #34799 ) ;
#18194=EDGE_LOOP ( 'NONE', ( #27882, #22667, #33574, #50954 ) ) ;
#18195=CARTESIAN_POINT ( 'NONE',  ( -18.21966661063519766, -0.1191753592594176486, 4.039956355595887061 ) ) ;
#18196=DIRECTION ( 'NONE',  ( 0.000000000000000000, -1.000000000000000000, 0.000000000000000000 ) ) ;
#18198=EDGE_CURVE ( 'NONE', #530, #21098, #26752, .T. ) ;
#18200=ORIENTED_EDGE ( 'NONE', *, *, #38717, .T. ) ;
#18201=AXIS2_PLACEMENT_3D ( 'NONE', #46932, #629, #43249 ) ;
#18202=LINE ( 'NONE', #19046, #9571 ) ;
#18203=ORIENTED_EDGE ( 'NONE', *, *, #3852, .T. ) ;
#18205=VECTOR ( 'NONE', #7934, 999.9999999999998863 ) ;
#18206=DIRECTION ( 'NONE',  ( 0.005961354470445682716, -0.6427876096865404731, -0.7660212471507180654 ) ) ;
#18207=ORIENTED_EDGE ( 'NONE', *, *, #21517, .F. ) ;
#18208=DIRECTION ( 'NONE',  ( 0.007781995580012662783, 0.000000000000000000, -0.9999697198139514409 ) ) ;
#18209=CARTESIAN_POINT ( 'NONE',  ( -13.81839363928948750, -4.241740624735661491, 9.010884102239385740 ) ) ;
#18210=LINE ( 'NONE', #39546, #28284 ) ;
#18211=ORIENTED_EDGE ( 'NONE', *, *, #10609, .T. ) ;
#18212=CARTESIAN_POINT ( 'NONE',  ( -14.52843791745405255, -0.1191753592594190225, 7.392670979059843717 ) ) ;
#18213=CARTESIAN_POINT ( 'NONE',  ( -11.40636015113596180, 0.000000000000000000, 11.32142374880780089 ) ) ;
#18214=DIRECTION ( 'NONE',  ( 0.5449076811759707706, 0.6444004775717708799, -0.5364919789714476250 ) ) ;
#18216=DIRECTION ( 'NONE',  ( -0.6427681459581293666, -0.7660444431189770143, -0.005002170337467561935 ) ) ;
#18219=ORIENTED_EDGE ( 'NONE', *, *, #30615, .T. ) ;
#18220=CARTESIAN_POINT ( 'NONE',  ( -15.13495153988577968, 0.000000000000000000, 12.76973526769478084 ) ) ;
#18221=DIRECTION ( 'NONE',  ( -0.005961354470445682716, -0.6427876096865404731, 0.7660212471507180654 ) ) ;
#18222=ADVANCED_FACE ( 'NONE', ( #53433 ), #44350, .F. ) ;
#18223=DIRECTION ( 'NONE',  ( 0.9999697198139515519, 0.000000000000000000, 0.007781995580013368816 ) ) ;
#18224=VERTEX_POINT ( 'NONE', #4893 ) ;
#18225=FACE_OUTER_BOUND ( 'NONE', #46431, .T. ) ;
#18226=DIRECTION ( 'NONE',  ( 0.007781995580012663651, -3.146120232559066537E-19, -0.9999697198139514409 ) ) ;
#18227=EDGE_LOOP ( 'NONE', ( #24599, #16320, #35984, #21441 ) ) ;
#18228=DIRECTION ( 'NONE',  ( 0.007781995580012663651, 0.000000000000000000, -0.9999697198139515519 ) ) ;
#18229=AXIS2_PLACEMENT_3D ( 'NONE', #13841, #51631, #515 ) ;
#18230=EDGE_CURVE ( 'NONE', #32968, #7355, #52582, .T. ) ;
#18231=VECTOR ( 'NONE', #32411, 1000.000000000000114 ) ;
#18233=DIRECTION ( 'NONE',  ( 0.9999697198139515519, 0.000000000000000000, 0.007781995580013368816 ) ) ;
#18234=ADVANCED_FACE ( 'NONE', ( #1172 ), #48895, .F. ) ;
#18235=CARTESIAN_POINT ( 'NONE',  ( -20.32198454194807979, -1.489407457353157049, 7.020052044550838310 ) ) ;
#18237=ORIENTED_EDGE ( 'NONE', *, *, #44046, .T. ) ;
#18238=DIRECTION ( 'NONE',  ( -0.5449076811759708816, 0.6444004775717707689, 0.5364919789714475140 ) ) ;
#18239=DIRECTION ( 'NONE',  ( -0.005002170337468016433, -0.7660444431189770143, 0.6427681459581293666 ) ) ;
#18240=DIRECTION ( 'NONE',  ( 0.9999697198139515519, 0.000000000000000000, 0.007781995580013368816 ) ) ;
#18241=CARTESIAN_POINT ( 'NONE',  ( -14.36410299895545961, 0.2864062442990018553, 2.252299284581917860 ) ) ;
#18243=VECTOR ( 'NONE', #40000, 1000.000000000000227 ) ;
#18244=DIRECTION ( 'NONE',  ( -0.6427681459581293666, -0.7660444431189770143, -0.005002170337467561935 ) ) ;
#18245=ORIENTED_EDGE ( 'NONE', *, *, #33434, .T. ) ;
#18246=DIRECTION ( 'NONE',  ( -0.6427681459581293666, -0.7660444431189770143, -0.005002170337467561935 ) ) ;
#18247=VECTOR ( 'NONE', #32659, 1000.000000000000000 ) ;
#18248=LINE ( 'NONE', #1510, #48723 ) ;
#18249=ORIENTED_EDGE ( 'NONE', *, *, #21749, .T. ) ;
#18250=FACE_OUTER_BOUND ( 'NONE', #2860, .T. ) ;
#18251=CARTESIAN_POINT ( 'NONE',  ( -16.25615214383689278, 0.000000000000000000, 3.416575767691794496 ) ) ;
#18252=CARTESIAN_POINT ( 'NONE',  ( -17.90023334230202323, 0.000000000000000000, 9.851752347948734112 ) ) ;
#18253=VERTEX_POINT ( 'NONE', #5449 ) ;
#18254=CARTESIAN_POINT ( 'NONE',  ( -10.37421533196711465, -0.1191753592594197858, 10.96012406864405975 ) ) ;
#18255=ORIENTED_EDGE ( 'NONE', *, *, #26796, .T. ) ;
#18256=ORIENTED_EDGE ( 'NONE', *, *, #46167, .T. ) ;
#18257=ORIENTED_EDGE ( 'NONE', *, *, #33730, .T. ) ;
#18258=ORIENTED_EDGE ( 'NONE', *, *, #42068, .F. ) ;
#18259=LINE ( 'NONE', #23643, #54719 ) ;
#18261=VERTEX_POINT ( 'NONE', #13966 ) ;
#18262=CARTESIAN_POINT ( 'NONE',  ( -17.55224900710100044, -2.653845599528779520, 12.45560879478165184 ) ) ;
#18263=CARTESIAN_POINT ( 'NONE',  ( -26.13493519185646008, 0.000000000000000000, 7.033017491833586377 ) ) ;
#18265=VECTOR ( 'NONE', #33969, 1000.000000000000227 ) ;
#18266=VECTOR ( 'NONE', #41728, 1000.000000000000227 ) ;
#18267=ORIENTED_EDGE ( 'NONE', *, *, #11682, .F. ) ;
#18268=CARTESIAN_POINT ( 'NONE',  ( -15.52974634762279038, 0.000000000000000000, 3.791560895369574080 ) ) ;
#18269=ORIENTED_EDGE ( 'NONE', *, *, #13393, .T. ) ;
#18270=DIRECTION ( 'NONE',  ( 0.005002170337468016433, -0.7660444431189770143, -0.6427681459581293666 ) ) ;
#18271=ORIENTED_EDGE ( 'NONE', *, *, #20451, .F. ) ;
#18272=ADVANCED_FACE ( 'NONE', ( #9990 ), #22217, .F. ) ;
#18273=ADVANCED_FACE ( 'NONE', ( #5729 ), #642, .F. ) ;
#18274=DIRECTION ( 'NONE',  ( 0.000000000000000000, -1.000000000000000000, 0.000000000000000000 ) ) ;
#18275=CARTESIAN_POINT ( 'NONE',  ( -17.22410628747702077, 0.000000000000000000, 8.379685845801690292 ) ) ;
#18276=VECTOR ( 'NONE', #19701, 1000.000000000000227 ) ;
#18277=CARTESIAN_POINT ( 'NONE',  ( -15.18146849030217993, 1.257817950434004350, 2.538798679945565961 ) ) ;
#18279=PLANE ( 'NONE',  #8782 ) ;
#18280=LINE ( 'NONE', #35084, #51922 ) ;
#18281=ORIENTED_EDGE ( 'NONE', *, *, #46594, .F. ) ;
#18282=VERTEX_POINT ( 'NONE', #36381 ) ;
#18283=CARTESIAN_POINT ( 'NONE',  ( -33.59133976979808978, -0.1191753592594197858, 9.829643557626155825 ) ) ;
#18284=DIRECTION ( 'NONE',  ( 0.007781995580012663651, -3.146120232559066537E-19, -0.9999697198139514409 ) ) ;
#18285=DIRECTION ( 'NONE',  ( -0.5449076811759708816, 0.6444004775717707689, 0.5364919789714475140 ) ) ;
#18286=DIRECTION ( 'NONE',  ( -0.5449076811759708816, 0.6444004775717707689, 0.5364919789714475140 ) ) ;
#18287=ORIENTED_EDGE ( 'NONE', *, *, #38708, .T. ) ;
#18288=DIRECTION ( 'NONE',  ( 0.7660212471507180654, -0.6427876096865404731, 0.005961354470445141482 ) ) ;
#18289=LINE ( 'NONE', #44162, #9642 ) ;
#18290=ORIENTED_EDGE ( 'NONE', *, *, #52139, .F. ) ;
#18293=ORIENTED_EDGE ( 'NONE', *, *, #55348, .T. ) ;
#18294=CARTESIAN_POINT ( 'NONE',  ( -17.19249169891891427, 0.000000000000000000, 4.317279109966281503 ) ) ;
#18295=CARTESIAN_POINT ( 'NONE',  ( -27.06708303904391144, 0.000000000000000000, 7.395095371555332697 ) ) ;
#18296=CARTESIAN_POINT ( 'NONE',  ( -19.65553346665874557, 5.467268677019013978, 4.142373939576459385 ) ) ;
#18297=ADVANCED_FACE ( 'NONE', ( #10269 ), #53694, .F. ) ;
#18298=FACE_OUTER_BOUND ( 'NONE', #42299, .T. ) ;
#18299=DIRECTION ( 'NONE',  ( -0.6427681459581293666, -0.7660444431189770143, -0.005002170337467561935 ) ) ;
#18300=ORIENTED_EDGE ( 'NONE', *, *, #34688, .T. ) ;
#18301=ADVANCED_FACE ( 'NONE', ( #37802 ), #49733, .F. ) ;
#18302=EDGE_LOOP ( 'NONE', ( #34442, #8673, #20649, #33296 ) ) ;
#18303=DIRECTION ( 'NONE',  ( 0.5364919789714477361, 0.6444004775717706579, 0.5449076811759711036 ) ) ;
#18304=DIRECTION ( 'NONE',  ( -0.9999697198139514409, -0.000000000000000000, -0.007781995580013368816 ) ) ;
#18305=LINE ( 'NONE', #44177, #50539 ) ;
#18306=EDGE_CURVE ( 'NONE', #14283, #25334, #23874, .T. ) ;
#18308=AXIS2_PLACEMENT_3D ( 'NONE', #44678, #44988, #4742 ) ;
#18309=PLANE ( 'NONE',  #32781 ) ;
#18310=ADVANCED_FACE ( 'NONE', ( #24433 ), #10578, .F. ) ;
#18312=ORIENTED_EDGE ( 'NONE', *, *, #43315, .F. ) ;
#18313=CARTESIAN_POINT ( 'NONE',  ( -12.13851405436063047, 0.000000000000000000, 11.68505802764555135 ) ) ;
#18314=CARTESIAN_POINT ( 'NONE',  ( -27.06552663992790997, 0.000000000000000000, 7.195101427592543786 ) ) ;
#18315=DIRECTION ( 'NONE',  ( 0.005961354470445682716, -0.6427876096865404731, -0.7660212471507180654 ) ) ;
#18316=DIRECTION ( 'NONE',  ( 0.007781995580012663651, 0.000000000000000000, -0.9999697198139515519 ) ) ;
#18317=VECTOR ( 'NONE', #26978, 999.9999999999998863 ) ;
#18318=VERTEX_POINT ( 'NONE', #49980 ) ;
#18319=LINE ( 'NONE', #44726, #18394 ) ;
#18320=ORIENTED_EDGE ( 'NONE', *, *, #48519, .F. ) ;
#18321=CARTESIAN_POINT ( 'NONE',  ( -29.86352658060627618, 0.000000000000000000, 8.481329010720569883 ) ) ;
#18322=LINE ( 'NONE', #52976, #297 ) ;
#18323=ORIENTED_EDGE ( 'NONE', *, *, #34088, .T. ) ;
#18324=DIRECTION ( 'NONE',  ( -0.5449076811759708816, 0.6444004775717707689, 0.5364919789714475140 ) ) ;
#18325=AXIS2_PLACEMENT_3D ( 'NONE', #26315, #1023, #30609 ) ;
#18327=AXIS2_PLACEMENT_3D ( 'NONE', #53234, #18274, #48686 ) ;
#18328=VERTEX_POINT ( 'NONE', #41742 ) ;
#18329=ORIENTED_EDGE ( 'NONE', *, *, #7074, .T. ) ;
#18330=PLANE ( 'NONE',  #32992 ) ;
#18331=VERTEX_POINT ( 'NONE', #15927 ) ;
#18332=ORIENTED_EDGE ( 'NONE', *, *, #32131, .T. ) ;
#18333=DIRECTION ( 'NONE',  ( -0.5449076811759708816, 0.6444004775717707689, 0.5364919789714475140 ) ) ;
#18334=EDGE_CURVE ( 'NONE', #25263, #1167, #15620, .T. ) ;
#18335=DIRECTION ( 'NONE',  ( 0.5364919789714477361, 0.6444004775717706579, 0.5449076811759711036 ) ) ;
#18336=ORIENTED_EDGE ( 'NONE', *, *, #50414, .F. ) ;
#18337=EDGE_CURVE ( 'NONE', #46010, #54122, #53989, .T. ) ;
#18338=ORIENTED_EDGE ( 'NONE', *, *, #21566, .T. ) ;
#18339=DIRECTION ( 'NONE',  ( 0.9999697198139515519, 0.000000000000000000, 0.007781995580013368816 ) ) ;
#18340=VERTEX_POINT ( 'NONE', #27890 ) ;
#18341=VECTOR ( 'NONE', #33469, 1000.000000000000227 ) ;
#18342=ORIENTED_EDGE ( 'NONE', *, *, #29565, .T. ) ;
#18343=EDGE_CURVE ( 'NONE', #42498, #55547, #50274, .T. ) ;
#18344=EDGE_CURVE ( 'NONE', #15522, #6267, #46280, .T. ) ;
#18345=PLANE ( 'NONE',  #23055 ) ;
#18346=CARTESIAN_POINT ( 'NONE',  ( -9.881852802408157999, -0.1159828484229821904, 7.056820793252878588 ) ) ;
#18347=CARTESIAN_POINT ( 'NONE',  ( -8.926928673813481652, -0.1191753592594179401, 4.112274590956074505 ) ) ;
#18348=CARTESIAN_POINT ( 'NONE',  ( -24.26908309836554878, 0.000000000000000000, 6.108867788427308376 ) ) ;
#18349=AXIS2_PLACEMENT_3D ( 'NONE', #9177, #48656, #26226 ) ;
#18350=EDGE_LOOP ( 'NONE', ( #14463, #50168, #27514, #6834 ) ) ;
#18351=LINE ( 'NONE', #43629, #34616 ) ;
#18352=ORIENTED_EDGE ( 'NONE', *, *, #43492, .F. ) ;
#18353=VECTOR ( 'NONE', #46513, 999.9999999999998863 ) ;
#18354=VECTOR ( 'NONE', #46274, 1000.000000000000227 ) ;
#18355=DIRECTION ( 'NONE',  ( -0.005002170337468016433, -0.7660444431189770143, 0.6427681459581293666 ) ) ;
#18356=ADVANCED_FACE ( 'NONE', ( #11386 ), #45198, .F. ) ;
#18357=LINE ( 'NONE', #768, #36028 ) ;
#18358=VECTOR ( 'NONE', #2181, 1000.000000000000114 ) ;
#18359=VECTOR ( 'NONE', #43644, 999.9999999999998863 ) ;
#18360=CARTESIAN_POINT ( 'NONE',  ( 2.072287782118878319, 0.000000000000000000, -2.950529333540147015 ) ) ;
#18362=DIRECTION ( 'NONE',  ( 0.5364919789714477361, 0.6444004775717706579, 0.5449076811759711036 ) ) ;
#18363=LINE ( 'NONE', #5886, #16682 ) ;
#18364=FACE_OUTER_BOUND ( 'NONE', #7342, .T. ) ;
#18365=ORIENTED_EDGE ( 'NONE', *, *, #1132, .F. ) ;
#18366=DIRECTION ( 'NONE',  ( -0.5364919789714478471, 0.6444004775717705469, -0.5449076811759709926 ) ) ;
#18367=FACE_OUTER_BOUND ( 'NONE', #42605, .T. ) ;
#18368=CARTESIAN_POINT ( 'NONE',  ( -16.99924723426068951, 0.000000000000000000, 13.49389102713827171 ) ) ;
#18369=CARTESIAN_POINT ( 'NONE',  ( -12.72755469904986469, 0.000000000000000000, 1.966707849688810850 ) ) ;
#18370=VECTOR ( 'NONE', #404, 1000.000000000000114 ) ;
#18371=PLANE ( 'NONE',  #25862 ) ;
#18372=DIRECTION ( 'NONE',  ( 0.6427681459581294776, -0.7660444431189769032, 0.005002170337467562802 ) ) ;
#18373=LINE ( 'NONE', #31470, #52221 ) ;
#18375=EDGE_LOOP ( 'NONE', ( #19748, #12986, #28603, #51589 ) ) ;
#18376=DIRECTION ( 'NONE',  ( 0.9999697198139515519, 0.000000000000000000, 0.007781995580013368816 ) ) ;
#18377=DIRECTION ( 'NONE',  ( -0.5449076811759708816, 0.6444004775717707689, 0.5364919789714475140 ) ) ;
#18378=PLANE ( 'NONE',  #21858 ) ;
#18379=DIRECTION ( 'NONE',  ( 0.005961354470445682716, -0.6427876096865404731, -0.7660212471507180654 ) ) ;
#18380=ADVANCED_FACE ( 'NONE', ( #6562 ), #46029, .F. ) ;
#18381=DIRECTION ( 'NONE',  ( -0.9999697198139514409, -0.000000000000000000, -0.007781995580013368816 ) ) ;
#18383=LINE ( 'NONE', #792, #54033 ) ;
#18384=DIRECTION ( 'NONE',  ( 0.000000000000000000, -1.000000000000000000, 0.000000000000000000 ) ) ;
#18386=AXIS2_PLACEMENT_3D ( 'NONE', #6966, #37308, #2102 ) ;
#18387=LINE ( 'NONE', #17563, #1120 ) ;
#18388=EDGE_CURVE ( 'NONE', #26517, #16557, #28985, .T. ) ;
#18389=VECTOR ( 'NONE', #44072, 1000.000000000000114 ) ;
#18390=VECTOR ( 'NONE', #11245, 999.9999999999998863 ) ;
#18391=ORIENTED_EDGE ( 'NONE', *, *, #51392, .T. ) ;
#18392=ADVANCED_FACE ( 'NONE', ( #36966 ), #16204, .F. ) ;
#18393=ADVANCED_FACE ( 'NONE', ( #7389 ), #24707, .F. ) ;
#18394=VECTOR ( 'NONE', #18622, 999.9999999999998863 ) ;
#18395=ORIENTED_EDGE ( 'NONE', *, *, #3150, .F. ) ;
#18398=ORIENTED_EDGE ( 'NONE', *, *, #33878, .F. ) ;
#18399=ORIENTED_EDGE ( 'NONE', *, *, #31867, .F. ) ;
#18400=PLANE ( 'NONE',  #18749 ) ;
#18401=ADVANCED_FACE ( 'NONE', ( #45731 ), #20468, .F. ) ;
#18402=CARTESIAN_POINT ( 'NONE',  ( -10.19678563399013527, -1.000000000000000000, 0.7424042488757021108 ) ) ;
#18404=EDGE_CURVE ( 'NONE', #19686, #20661, #19897, .T. ) ;
#18405=ORIENTED_EDGE ( 'NONE', *, *, #8182, .T. ) ;
#18406=VECTOR ( 'NONE', #2758, 1000.000000000000227 ) ;
#18407=AXIS2_PLACEMENT_3D ( 'NONE', #33155, #33693, #51003 ) ;
#18408=EDGE_CURVE ( 'NONE', #1201, #2866, #1998, .T. ) ;
#18409=CARTESIAN_POINT ( 'NONE',  ( -15.88130887279446490, 0.000000000000000000, 3.050160814894388839 ) ) ;
#18410=ORIENTED_EDGE ( 'NONE', *, *, #41913, .F. ) ;
#18411=DIRECTION ( 'NONE',  ( -0.9999697198139514409, -0.000000000000000000, -0.007781995580013368816 ) ) ;
#18412=CARTESIAN_POINT ( 'NONE',  ( -23.33849165029409889, 0.000000000000000000, 5.946783852668351855 ) ) ;
#18413=ORIENTED_EDGE ( 'NONE', *, *, #41312, .F. ) ;
#18414=FACE_OUTER_BOUND ( 'NONE', #24135, .T. ) ;
#18415=AXIS2_PLACEMENT_3D ( 'NONE', #16598, #3814, #38178 ) ;
#18416=ADVANCED_FACE ( 'NONE', ( #12222 ), #56219, .F. ) ;
#18418=CARTESIAN_POINT ( 'NONE',  ( -17.89604163440746021, 0.000000000000000000, 9.313126885395993426 ) ) ;
#18419=DIRECTION ( 'NONE',  ( 0.005961354470445682716, -0.6427876096865404731, -0.7660212471507180654 ) ) ;
#18420=AXIS2_PLACEMENT_3D ( 'NONE', #30126, #47748, #25885 ) ;
#18421=EDGE_CURVE ( 'NONE', #4104, #1645, #51949, .T. ) ;
#18422=LINE ( 'NONE', #39460, #32756 ) ;
#18423=PLANE ( 'NONE',  #40558 ) ;
#18424=ORIENTED_EDGE ( 'NONE', *, *, #1512, .F. ) ;
#18425=CARTESIAN_POINT ( 'NONE',  ( -19.38307830287650191, 5.143464774974014553, 4.046874141121907797 ) ) ;
#18426=DIRECTION ( 'NONE',  ( 0.9321478471874540261, 0.000000000000000000, -0.3620778797217456546 ) ) ;
#18427=CARTESIAN_POINT ( 'NONE',  ( -21.31926590099137897, 1.905425754524007642, 4.902265555185135959 ) ) ;
#18428=VECTOR ( 'NONE', #54232, 1000.000000000000227 ) ;
#18429=ORIENTED_EDGE ( 'NONE', *, *, #33468, .T. ) ;
#18430=DIRECTION ( 'NONE',  ( 0.007781995580012663651, 0.000000000000000000, -0.9999697198139515519 ) ) ;
#18431=ORIENTED_EDGE ( 'NONE', *, *, #6082, .T. ) ;
#18432=VECTOR ( 'NONE', #19052, 1000.000000000000227 ) ;
#18433=VECTOR ( 'NONE', #50362, 1000.000000000000000 ) ;
#18434=LINE ( 'NONE', #1675, #10171 ) ;
#18435=DIRECTION ( 'NONE',  ( -0.5364919789714478471, 0.6444004775717705469, -0.5449076811759709926 ) ) ;
#18436=CARTESIAN_POINT ( 'NONE',  ( -12.50746586153157303, -4.889348428825662118, 9.564509969865337524 ) ) ;
#18437=FACE_OUTER_BOUND ( 'NONE', #41333, .T. ) ;
#18438=LINE ( 'NONE', #1399, #45871 ) ;
#18439=FACE_OUTER_BOUND ( 'NONE', #19285, .T. ) ;
#18440=CARTESIAN_POINT ( 'NONE',  ( -18.59789860346329959, 0.000000000000000000, 5.783670187693309650 ) ) ;
#18441=VECTOR ( 'NONE', #40636, 1000.000000000000227 ) ;
#18443=VECTOR ( 'NONE', #12470, 1000.000000000000227 ) ;
#18444=LINE ( 'NONE', #35780, #29633 ) ;
#18445=ORIENTED_EDGE ( 'NONE', *, *, #12822, .F. ) ;
#18446=LINE ( 'NONE', #35782, #309 ) ;
#18447=FACE_OUTER_BOUND ( 'NONE', #53370, .T. ) ;
#18448=CARTESIAN_POINT ( 'NONE',  ( -19.32826701083865117, 3.362543313726507499, 9.907582850272294905 ) ) ;
#18449=CARTESIAN_POINT ( 'NONE',  ( -22.40556560354864146, -0.1191753592594197858, 5.484709000965211523 ) ) ;
#18450=DIRECTION ( 'NONE',  ( -0.5449076811759708816, 0.6444004775717707689, 0.5364919789714475140 ) ) ;
#18451=ADVANCED_FACE ( 'NONE', ( #34102 ), #262, .F. ) ;
#18452=FACE_OUTER_BOUND ( 'NONE', #7887, .T. ) ;
#18453=LINE ( 'NONE', #52274, #2070 ) ;
#18454=ORIENTED_EDGE ( 'NONE', *, *, #13387, .T. ) ;
#18455=ORIENTED_EDGE ( 'NONE', *, *, #14409, .F. ) ;
#18456=VECTOR ( 'NONE', #38958, 1000.000000000000000 ) ;
#18457=DIRECTION ( 'NONE',  ( -0.5449076811759708816, 0.6444004775717707689, 0.5364919789714475140 ) ) ;
#18458=CARTESIAN_POINT ( 'NONE',  ( -12.40433439172452701, 0.000000000000000000, 1.599891155051114788 ) ) ;
#18459=VECTOR ( 'NONE', #25480, 999.9999999999998863 ) ;
#18460=ORIENTED_EDGE ( 'NONE', *, *, #12001, .T. ) ;
#18461=DIRECTION ( 'NONE',  ( 0.000000000000000000, 0.000000000000000000, -1.000000000000000000 ) ) ;
#18462=AXIS2_PLACEMENT_3D ( 'NONE', #43638, #4750, #43925 ) ;
#18463=ORIENTED_EDGE ( 'NONE', *, *, #43039, .T. ) ;
#18464=CARTESIAN_POINT ( 'NONE',  ( -13.07066190154808361, 0.000000000000000000, 12.04713590736729678 ) ) ;
#18465=ADVANCED_FACE ( 'NONE', ( #25294 ), #42597, .F. ) ;
#18466=ORIENTED_EDGE ( 'NONE', *, *, #3131, .T. ) ;
#18467=ORIENTED_EDGE ( 'NONE', *, *, #7614, .F. ) ;
#18468=ORIENTED_EDGE ( 'NONE', *, *, #12487, .F. ) ;
#18469=DIRECTION ( 'NONE',  ( -0.6427681459581293666, -0.7660444431189770143, -0.005002170337467561935 ) ) ;
#18470=AXIS2_PLACEMENT_3D ( 'NONE', #52681, #993, #44449 ) ;
#18471=DIRECTION ( 'NONE',  ( 0.005002170337468016433, -0.7660444431189770143, -0.6427681459581293666 ) ) ;
#18472=FACE_OUTER_BOUND ( 'NONE', #19797, .T. ) ;
#18473=AXIS2_PLACEMENT_3D ( 'NONE', #15169, #32728, #28476 ) ;
#18474=LINE ( 'NONE', #25206, #20220 ) ;
#18475=EDGE_CURVE ( 'NONE', #35585, #6991, #4289, .T. ) ;
#18476=ORIENTED_EDGE ( 'NONE', *, *, #41190, .F. ) ;
#18477=ORIENTED_EDGE ( 'NONE', *, *, #48875, .T. ) ;
#18478=EDGE_CURVE ( 'NONE', #48488, #9624, #13069, .T. ) ;
#18479=VECTOR ( 'NONE', #45400, 1000.000000000000227 ) ;
#18481=LINE ( 'NONE', #17651, #3713 ) ;
#18482=EDGE_LOOP ( 'NONE', ( #47054, #51769, #26398, #2044 ) ) ;
#18483=DIRECTION ( 'NONE',  ( 0.005961354470445682716, -0.6427876096865404731, -0.7660212471507180654 ) ) ;
#18484=VERTEX_POINT ( 'NONE', #30397 ) ;
#18485=CARTESIAN_POINT ( 'NONE',  ( -9.908141408373387193, -0.1191753592594197858, 10.77908512878318703 ) ) ;
#18486=CARTESIAN_POINT ( 'NONE',  ( -24.27063949748155380, 0.000000000000000000, 6.308861732390097288 ) ) ;
#18487=EDGE_CURVE ( 'NONE', #21607, #29890, #46569, .T. ) ;
#18488=VERTEX_POINT ( 'NONE', #12520 ) ;
#18489=CARTESIAN_POINT ( 'NONE',  ( -12.02954139919957299, -0.5179957512181571078, 1.537476745106777454 ) ) ;
#18490=ORIENTED_EDGE ( 'NONE', *, *, #46067, .F. ) ;
#18491=EDGE_CURVE ( 'NONE', #51394, #20189, #3430, .T. ) ;
#18492=CARTESIAN_POINT ( 'NONE',  ( -9.342070512798265725, 0.000000000000000000, 10.59882438848031505 ) ) ;
#18493=VECTOR ( 'NONE', #8275, 1000.000000000000114 ) ;
#18495=CARTESIAN_POINT ( 'NONE',  ( -12.80458192191714595, 0.000000000000000000, 11.86454056839041726 ) ) ;
#18496=DIRECTION ( 'NONE',  ( 0.5364919789714477361, 0.6444004775717706579, 0.5449076811759711036 ) ) ;
#18497=LINE ( 'NONE', #2292, #24665 ) ;
#18498=ORIENTED_EDGE ( 'NONE', *, *, #25297, .T. ) ;
#18500=DIRECTION ( 'NONE',  ( 0.5449076811759707706, 0.6444004775717708799, -0.5364919789714476250 ) ) ;
#18501=CARTESIAN_POINT ( 'NONE',  ( -11.14358987946894430, 0.000000000000000000, 3.256356853177110100 ) ) ;
#18502=VECTOR ( 'NONE', #45959, 1000.000000000000227 ) ;
#18504=DIRECTION ( 'NONE',  ( -0.005961354470445682716, -0.6427876096865404731, 0.7660212471507180654 ) ) ;
#18505=LINE ( 'NONE', #13682, #24283 ) ;
#18507=ORIENTED_EDGE ( 'NONE', *, *, #9412, .F. ) ;
#18508=DIRECTION ( 'NONE',  ( 0.007781995580012663651, -3.146120232559066537E-19, -0.9999697198139514409 ) ) ;
#18509=DIRECTION ( 'NONE',  ( 0.005002170337468016433, -0.7660444431189770143, -0.6427681459581293666 ) ) ;
#18510=DIRECTION ( 'NONE',  ( 0.007781995580012662783, 0.000000000000000000, -0.9999697198139514409 ) ) ;
#18511=ORIENTED_EDGE ( 'NONE', *, *, #37623, .T. ) ;
#18512=VECTOR ( 'NONE', #8014, 1000.000000000000000 ) ;
#18513=DIRECTION ( 'NONE',  ( -0.7660212471507179544, -0.6427876096865405842, -0.005961354470445141482 ) ) ;
#18514=DIRECTION ( 'NONE',  ( 0.6427681459581294776, -0.7660444431189769032, 0.005002170337467562802 ) ) ;
#18515=ORIENTED_EDGE ( 'NONE', *, *, #49439, .T. ) ;
#18517=VECTOR ( 'NONE', #14462, 1000.000000000000000 ) ;
#18518=CARTESIAN_POINT ( 'NONE',  ( -15.96710241509184058, -0.1191753592594218814, 13.13259134697452879 ) ) ;
#18519=LINE ( 'NONE', #909, #44796 ) ;
#18520=EDGE_CURVE ( 'NONE', #51971, #36728, #4544, .T. ) ;
#18521=CARTESIAN_POINT ( 'NONE',  ( -16.88915937219315921, -0.03739765774599798642, 3.380268248018597266 ) ) ;
#18522=FACE_OUTER_BOUND ( 'NONE', #55525, .T. ) ;
#18523=ORIENTED_EDGE ( 'NONE', *, *, #54283, .F. ) ;
#18524=VECTOR ( 'NONE', #3382, 1000.000000000000227 ) ;
#18525=VECTOR ( 'NONE', #8395, 1000.000000000000227 ) ;
#18526=VERTEX_POINT ( 'NONE', #50828 ) ;
#18527=EDGE_CURVE ( 'NONE', #36877, #46331, #12781, .T. ) ;
#18528=PLANE ( 'NONE',  #28535 ) ;
#18529=CARTESIAN_POINT ( 'NONE',  ( -23.33693525117809386, 0.000000000000000000, 5.746789908705562944 ) ) ;
#18530=DIRECTION ( 'NONE',  ( -0.6427681459581293666, -0.7660444431189770143, -0.005002170337467561935 ) ) ;
#18531=EDGE_CURVE ( 'NONE', #56226, #31598, #29253, .T. ) ;
#18532=EDGE_CURVE ( 'NONE', #56039, #18526, #47136, .T. ) ;
#18533=EDGE_CURVE ( 'NONE', #5817, #9950, #21306, .T. ) ;
#18534=DIRECTION ( 'NONE',  ( -0.005961354470445682716, -0.6427876096865404731, 0.7660212471507180654 ) ) ;
#18535=DIRECTION ( 'NONE',  ( 0.5449076811759707706, 0.6444004775717708799, -0.5364919789714476250 ) ) ;
#18537=EDGE_LOOP ( 'NONE', ( #13586, #4000, #13810, #33284 ) ) ;
#18538=PLANE ( 'NONE',  #18349 ) ;
#18539=AXIS2_PLACEMENT_3D ( 'NONE', #43625, #22056, #26595 ) ;
#18540=LINE ( 'NONE', #6072, #53274 ) ;
#18541=ORIENTED_EDGE ( 'NONE', *, *, #55015, .T. ) ;
#18542=VECTOR ( 'NONE', #52565, 1000.000000000000227 ) ;
#18543=CARTESIAN_POINT ( 'NONE',  ( -10.94028622754223967, 0.000000000000000000, 11.14038480894692995 ) ) ;
#18544=DIRECTION ( 'NONE',  ( 0.007781995580012663651, 0.000000000000000000, -0.9999697198139515519 ) ) ;
#18545=VECTOR ( 'NONE', #33521, 999.9999999999998863 ) ;
#18546=DIRECTION ( 'NONE',  ( 0.9999697198139515519, 0.000000000000000000, 0.007781995580013368816 ) ) ;
#18548=LINE ( 'NONE', #44963, #39386 ) ;
#18549=EDGE_CURVE ( 'NONE', #34742, #6991, #29566, .T. ) ;
#18550=ORIENTED_EDGE ( 'NONE', *, *, #2115, .F. ) ;
#18551=EDGE_CURVE ( 'NONE', #48671, #55683, #55370, .T. ) ;
#18552=ORIENTED_EDGE ( 'NONE', *, *, #5349, .T. ) ;
#18553=ORIENTED_EDGE ( 'NONE', *, *, #49664, .F. ) ;
#18554=VECTOR ( 'NONE', #18286, 1000.000000000000227 ) ;
#18555=ADVANCED_FACE ( 'NONE', ( #38638 ), #51677, .F. ) ;
#18556=ORIENTED_EDGE ( 'NONE', *, *, #55272, .T. ) ;
#18557=VECTOR ( 'NONE', #20131, 1000.000000000000227 ) ;
#18558=CARTESIAN_POINT ( 'NONE',  ( -13.66676830763716488, 0.000000000000000000, 3.236720895221059102 ) ) ;
#18559=ORIENTED_EDGE ( 'NONE', *, *, #14413, .F. ) ;
#18562=VECTOR ( 'NONE', #37027, 1000.000000000000227 ) ;
#18563=EDGE_CURVE ( 'NONE', #9163, #52307, #53377, .T. ) ;
#18564=EDGE_LOOP ( 'NONE', ( #11269, #26102, #54370, #27921 ) ) ;
#18565=DIRECTION ( 'NONE',  ( -0.5449076811759708816, 0.6444004775717707689, 0.5364919789714475140 ) ) ;
#18566=ORIENTED_EDGE ( 'NONE', *, *, #20093, .T. ) ;
#18567=DIRECTION ( 'NONE',  ( 0.9999697198139515519, 0.000000000000000000, 0.007781995580013368816 ) ) ;
#18569=EDGE_CURVE ( 'NONE', #42656, #21969, #13617, .T. ) ;
#18570=VECTOR ( 'NONE', #55761, 999.9999999999998863 ) ;
#18571=CARTESIAN_POINT ( 'NONE',  ( -22.40478740399063895, 0.000000000000000000, 5.384712028983816623 ) ) ;
#18572=AXIS2_PLACEMENT_3D ( 'NONE', #22526, #52605, #47813 ) ;
#18573=CARTESIAN_POINT ( 'NONE',  ( -12.33850799832341849, 0.000000000000000000, 11.68350162852954632 ) ) ;
#18574=LINE ( 'NONE', #49220, #53144 ) ;
#18576=LINE ( 'NONE', #31366, #11478 ) ;
#18577=CARTESIAN_POINT ( 'NONE',  ( -13.08486533123210194, 0.000000000000000000, 1.963927175729152541 ) ) ;
#18578=ORIENTED_EDGE ( 'NONE', *, *, #17435, .T. ) ;
#18579=ORIENTED_EDGE ( 'NONE', *, *, #7629, .F. ) ;
#18581=PLANE ( 'NONE',  #35742 ) ;
#18582=CARTESIAN_POINT ( 'NONE',  ( -15.84116117370739119, 0.9340140483890051470, 2.805376761212760250 ) ) ;
#18583=VECTOR ( 'NONE', #42812, 999.9999999999998863 ) ;
#18584=DIRECTION ( 'NONE',  ( 0.000000000000000000, 0.000000000000000000, 1.000000000000000000 ) ) ;
#18585=VERTEX_POINT ( 'NONE', #18744 ) ;
#18586=VECTOR ( 'NONE', #44210, 999.9999999999998863 ) ;
#18587=CARTESIAN_POINT ( 'NONE',  ( -13.00081981244401064, 0.000000000000000000, 3.072577446810097701 ) ) ;
#18588=CARTESIAN_POINT ( 'NONE',  ( -12.17737215012490459, 0.4483081953215047322, 2.347176129851082482 ) ) ;
#18589=VERTEX_POINT ( 'NONE', #9667 ) ;
#18590=CARTESIAN_POINT ( 'NONE',  ( -18.32750754357443412, 0.000000000000000000, 5.047110293829786265 ) ) ;
#18591=CARTESIAN_POINT ( 'NONE',  ( -19.60990026154428278, 0.000000000000000000, 4.498472333781370125 ) ) ;
#18592=VECTOR ( 'NONE', #29117, 1000.000000000000227 ) ;
#18593=ORIENTED_EDGE ( 'NONE', *, *, #49383, .F. ) ;
#18595=CARTESIAN_POINT ( 'NONE',  ( -17.49593704190832355, -4.727446477803161073, 11.23649290156757452 ) ) ;
#18596=VECTOR ( 'NONE', #40072, 999.9999999999998863 ) ;
#18597=LINE ( 'NONE', #14062, #51319 ) ;
#18598=DIRECTION ( 'NONE',  ( 0.005961354470445682716, -0.6427876096865404731, -0.7660212471507180654 ) ) ;
#18599=DIRECTION ( 'NONE',  ( 0.9999697198139515519, 0.000000000000000000, 0.007781995580013368816 ) ) ;
#18600=ORIENTED_EDGE ( 'NONE', *, *, #53265, .F. ) ;
#18601=VECTOR ( 'NONE', #46072, 1000.000000000000227 ) ;
#18602=STYLED_ITEM ( 'NONE', ( #9146 ), #3992 ) ;
#18603=ORIENTED_EDGE ( 'NONE', *, *, #18001, .T. ) ;
#18604=VECTOR ( 'NONE', #16780, 1000.000000000000227 ) ;
#18605=LINE ( 'NONE', #43588, #46604 ) ;
#18606=FACE_OUTER_BOUND ( 'NONE', #49591, .T. ) ;
#18607=CARTESIAN_POINT ( 'NONE',  ( -16.89925026227929195, -0.1191753592594197858, 13.49466922669627422 ) ) ;
#18608=AXIS2_PLACEMENT_3D ( 'NONE', #18811, #19059, #18216 ) ;
#18609=EDGE_CURVE ( 'NONE', #48572, #49125, #27238, .T. ) ;
#18610=EDGE_CURVE ( 'NONE', #32587, #16370, #14212, .T. ) ;
#18611=LINE ( 'NONE', #41011, #15539 ) ;
#18612=LINE ( 'NONE', #31098, #20340 ) ;
#18613=ORIENTED_EDGE ( 'NONE', *, *, #36040, .T. ) ;
#18614=ADVANCED_FACE ( 'NONE', ( #22986 ), #34943, .F. ) ;
#18615=CARTESIAN_POINT ( 'NONE',  ( -11.87108423333901719, 3.362543313726507499, 7.010959812498333221 ) ) ;
#18616=LINE ( 'NONE', #48986, #34731 ) ;
#18617=VECTOR ( 'NONE', #48270, 1000.000000000000227 ) ;
#18618=LINE ( 'NONE', #6139, #49566 ) ;
#18619=VECTOR ( 'NONE', #2984, 1000.000000000000227 ) ;
#18620=FACE_OUTER_BOUND ( 'NONE', #21268, .T. ) ;
#18621=VERTEX_POINT ( 'NONE', #5125 ) ;
#18622=DIRECTION ( 'NONE',  ( 0.007781995580012663651, 0.000000000000000000, -0.9999697198139515519 ) ) ;
#18623=ORIENTED_EDGE ( 'NONE', *, *, #45732, .F. ) ;
#18624=DIRECTION ( 'NONE',  ( 0.000000000000000000, -0.000000000000000000, -1.000000000000000000 ) ) ;
#18625=LINE ( 'NONE', #48434, #29341 ) ;
#18626=EDGE_LOOP ( 'NONE', ( #10384, #10798, #36540, #44580 ) ) ;
#18627=CARTESIAN_POINT ( 'NONE',  ( -16.73228525469910721, 0.000000000000000000, 4.890198668954845118 ) ) ;
#18628=EDGE_LOOP ( 'NONE', ( #40827, #29599, #46654, #29590 ) ) ;
#18629=ADVANCED_FACE ( 'NONE', ( #17603 ), #5394, .F. ) ;
#18630=VECTOR ( 'NONE', #37048, 999.9999999999998863 ) ;
#18631=VERTEX_POINT ( 'NONE', #43704 ) ;
#18632=EDGE_LOOP ( 'NONE', ( #44576, #33907, #30658, #42399 ) ) ;
#18633=LINE ( 'NONE', #35983, #37528 ) ;
#18634=ORIENTED_EDGE ( 'NONE', *, *, #32427, .T. ) ;
#18635=VECTOR ( 'NONE', #8854, 999.9999999999998863 ) ;
#18636=ORIENTED_EDGE ( 'NONE', *, *, #24734, .T. ) ;
#18637=DIRECTION ( 'NONE',  ( 0.5364919789714477361, 0.6444004775717706579, 0.5449076811759711036 ) ) ;
#18638=CARTESIAN_POINT ( 'NONE',  ( -20.66063881625015242, 5.467268677019012202, 13.87933419838711124 ) ) ;
#18639=AXIS2_PLACEMENT_3D ( 'NONE', #32814, #2702, #50436 ) ;
#18641=EDGE_CURVE ( 'NONE', #46187, #32158, #35773, .T. ) ;
#18642=ORIENTED_EDGE ( 'NONE', *, *, #28489, .T. ) ;
#18643=CARTESIAN_POINT ( 'NONE',  ( -14.75054148647694241, -4.241740624735661491, 9.372961981961132949 ) ) ;
#18644=ORIENTED_EDGE ( 'NONE', *, *, #54830, .F. ) ;
#18645=VECTOR ( 'NONE', #5584, 999.9999999999998863 ) ;
#18646=ORIENTED_EDGE ( 'NONE', *, *, #52477, .T. ) ;
#18647=EDGE_CURVE ( 'NONE', #28250, #17105, #49094, .T. ) ;
#18648=AXIS2_PLACEMENT_3D ( 'NONE', #52841, #13949, #31275 ) ;
#18649=VECTOR ( 'NONE', #8159, 1000.000000000000227 ) ;
#18650=DIRECTION ( 'NONE',  ( 0.005961354470445682716, -0.6427876096865404731, -0.7660212471507180654 ) ) ;
#18651=EDGE_CURVE ( 'NONE', #26440, #29351, #18438, .T. ) ;
#18652=DIRECTION ( 'NONE',  ( -0.6427681459581293666, -0.7660444431189770143, -0.005002170337467561935 ) ) ;
#18653=CARTESIAN_POINT ( 'NONE',  ( -15.50102849149811135, -0.1191753592594197858, 12.95155240711365430 ) ) ;
#18654=CARTESIAN_POINT ( 'NONE',  ( -12.27024259289907704, 2.229229656569006401, 1.376986556422233665 ) ) ;
#18655=ADVANCED_FACE ( 'NONE', ( #52258 ), #40306, .F. ) ;
#18656=ORIENTED_EDGE ( 'NONE', *, *, #47286, .F. ) ;
#18657=CARTESIAN_POINT ( 'NONE',  ( -18.39746900504187010, 0.000000000000000000, 14.03700784672088808 ) ) ;
#18658=VERTEX_POINT ( 'NONE', #9357 ) ;
#18659=VECTOR ( 'NONE', #5339, 1000.000000000000000 ) ;
#18660=VECTOR ( 'NONE', #16511, 1000.000000000000227 ) ;
#18661=EDGE_CURVE ( 'NONE', #50133, #48446, #837, .T. ) ;
#18662=CARTESIAN_POINT ( 'NONE',  ( -13.07066190154808361, 0.000000000000000000, 12.04713590736729678 ) ) ;
#18663=AXIS2_PLACEMENT_3D ( 'NONE', #41589, #6671, #54628 ) ;
#18665=VECTOR ( 'NONE', #49468, 1000.000000000000114 ) ;
#18666=DIRECTION ( 'NONE',  ( 0.2426528472758542054, 0.7422098413412800966, 0.6246952433987894571 ) ) ;
#18667=DIRECTION ( 'NONE',  ( 0.9999697198139515519, 0.000000000000000000, 0.007781995580013368816 ) ) ;
#18668=CARTESIAN_POINT ( 'NONE',  ( -19.60990026154428278, 0.000000000000000000, 4.498472333781370125 ) ) ;
#18669=DIRECTION ( 'NONE',  ( -0.5364919789714478471, 0.6444004775717705469, -0.5449076811759709926 ) ) ;
#18670=ORIENTED_EDGE ( 'NONE', *, *, #23603, .T. ) ;
#18671=DIRECTION ( 'NONE',  ( 0.007781995580012662783, 0.000000000000000000, -0.9999697198139514409 ) ) ;
#18672=ORIENTED_EDGE ( 'NONE', *, *, #28922, .F. ) ;
#18673=CARTESIAN_POINT ( 'NONE',  ( -22.40634380310664397, 0.000000000000000000, 5.584705972946605534 ) ) ;
#18674=DIRECTION ( 'NONE',  ( -0.5449076811759708816, 0.6444004775717707689, 0.5364919789714475140 ) ) ;
#18675=DIRECTION ( 'NONE',  ( -0.005961354470445682716, -0.6427876096865404731, 0.7660212471507180654 ) ) ;
#18676=PLANE ( 'NONE',  #23156 ) ;
#18677=CARTESIAN_POINT ( 'NONE',  ( -18.79214444041551957, 0.000000000000000000, 5.043494382061776804 ) ) ;
#18678=VECTOR ( 'NONE', #27061, 999.9999999999998863 ) ;
#18679=CARTESIAN_POINT ( 'NONE',  ( -16.06709938707323460, 0.000000000000000000, 13.13181314741652628 ) ) ;
#18680=AXIS2_PLACEMENT_3D ( 'NONE', #36630, #28949, #11341 ) ;
#18681=VERTEX_POINT ( 'NONE', #26982 ) ;
#18682=CARTESIAN_POINT ( 'NONE',  ( -14.56466625899772893, 3.848249166794011522, 2.216563428416727266 ) ) ;
#18683=CARTESIAN_POINT ( 'NONE',  ( 2.072287782118878319, 0.000000000000000000, -2.950529333540147015 ) ) ;
#18684=DIRECTION ( 'NONE',  ( 0.9999697198139515519, 0.000000000000000000, 0.007781995580013368816 ) ) ;
#18685=AXIS2_PLACEMENT_3D ( 'NONE', #29339, #4065, #16012 ) ;
#18686=ADVANCED_FACE ( 'NONE', ( #27522 ), #13895, .F. ) ;
#18687=PLANE ( 'NONE',  #1958 ) ;
#18688=VECTOR ( 'NONE', #17963, 999.9999999999998863 ) ;
#18689=CARTESIAN_POINT ( 'NONE',  ( -9.850454360485084493, -0.1191753592594188005, 3.366423360904528650 ) ) ;
#18690=LINE ( 'NONE', #31172, #35001 ) ;
#18691=EDGE_CURVE ( 'NONE', #51439, #22392, #40014, .T. ) ;
#18693=DIRECTION ( 'NONE',  ( -0.9999697198139514409, -0.000000000000000000, -0.007781995580013368816 ) ) ;
#18694=VECTOR ( 'NONE', #9083, 999.9999999999998863 ) ;
#18695=VECTOR ( 'NONE', #51253, 999.9999999999998863 ) ;
#18696=DIRECTION ( 'NONE',  ( 0.9999697198139515519, 0.000000000000000000, 0.007781995580013368816 ) ) ;
#18697=VECTOR ( 'NONE', #5263, 1000.000000000000227 ) ;
#18698=LINE ( 'NONE', #32579, #19242 ) ;
#18699=AXIS2_PLACEMENT_3D ( 'NONE', #8126, #34257, #25430 ) ;
#18700=ORIENTED_EDGE ( 'NONE', *, *, #30009, .T. ) ;
#18701=AXIS2_PLACEMENT_3D ( 'NONE', #42780, #56146, #3886 ) ;
#18702=EDGE_CURVE ( 'NONE', #41663, #17993, #9937, .T. ) ;
#18703=VECTOR ( 'NONE', #22481, 1000.000000000000227 ) ;
#18704=ORIENTED_EDGE ( 'NONE', *, *, #766, .T. ) ;
#18705=VECTOR ( 'NONE', #18102, 1000.000000000000227 ) ;
#18706=ORIENTED_EDGE ( 'NONE', *, *, #18404, .F. ) ;
#18707=ORIENTED_EDGE ( 'NONE', *, *, #20854, .T. ) ;
#18708=ORIENTED_EDGE ( 'NONE', *, *, #36979, .F. ) ;
#18709=FACE_OUTER_BOUND ( 'NONE', #15613, .T. ) ;
#18710=CARTESIAN_POINT ( 'NONE',  ( -8.312110554741027002, -0.1191753592594199662, 5.594387526948322531 ) ) ;
#18711=ORIENTED_EDGE ( 'NONE', *, *, #7877, .F. ) ;
#18712=EDGE_LOOP ( 'NONE', ( #35012, #50582, #5932, #5842 ) ) ;
#18713=ORIENTED_EDGE ( 'NONE', *, *, #50667, .F. ) ;
#18714=ADVANCED_FACE ( 'NONE', ( #15558 ), #24108, .F. ) ;
#18715=AXIS2_PLACEMENT_3D ( 'NONE', #52969, #43599, #18054 ) ;
#18716=DIRECTION ( 'NONE',  ( 0.9999697198139515519, 0.000000000000000000, 0.007781995580013368816 ) ) ;
#18717=CARTESIAN_POINT ( 'NONE',  ( -22.23691302235923573, 4.657758921906512306, 5.170897022466190762 ) ) ;
#18718=LINE ( 'NONE', #5374, #2338 ) ;
#18719=EDGE_CURVE ( 'NONE', #7643, #30900, #50512, .T. ) ;
#18720=ORIENTED_EDGE ( 'NONE', *, *, #7716, .F. ) ;
#18721=AXIS2_PLACEMENT_3D ( 'NONE', #26144, #47991, #17910 ) ;
#18722=CARTESIAN_POINT ( 'NONE',  ( -22.40634380310664397, 0.000000000000000000, 5.584705972946605534 ) ) ;
#18723=ORIENTED_EDGE ( 'NONE', *, *, #4907, .F. ) ;
#18724=LINE ( 'NONE', #15833, #15540 ) ;
#18725=VECTOR ( 'NONE', #46832, 999.9999999999998863 ) ;
#18726=EDGE_CURVE ( 'NONE', #38932, #18937, #20094, .T. ) ;
#18727=DIRECTION ( 'NONE',  ( 0.000000000000000000, -0.000000000000000000, -1.000000000000000000 ) ) ;
#18728=CARTESIAN_POINT ( 'NONE',  ( -17.43140473756637476, 0.000000000000000000, 9.316742797164003775 ) ) ;
#18729=CARTESIAN_POINT ( 'NONE',  ( -20.64971648638756108, -1.327505506330656670, 6.881645577644349920 ) ) ;
#18730=VECTOR ( 'NONE', #31730, 1000.000000000000227 ) ;
#18731=DIRECTION ( 'NONE',  ( -0.5449076811759708816, 0.6444004775717707689, 0.5364919789714475140 ) ) ;
#18732=CARTESIAN_POINT ( 'NONE',  ( -11.81396882728338582, 0.000000000000000000, 3.989803948808627432 ) ) ;
#18733=CARTESIAN_POINT ( 'NONE',  ( -19.45503627000849889, 0.000000000000000000, 7.556996783084074742 ) ) ;
#18734=VERTEX_POINT ( 'NONE', #1679 ) ;
#18735=CARTESIAN_POINT ( 'NONE',  ( -17.21416647257189325, 0.000000000000000000, 7.102440976733420008 ) ) ;
#18736=ORIENTED_EDGE ( 'NONE', *, *, #24577, .T. ) ;
#18737=VECTOR ( 'NONE', #44469, 1000.000000000000227 ) ;
#18738=EDGE_CURVE ( 'NONE', #41032, #20216, #19838, .T. ) ;
#18739=AXIS2_PLACEMENT_3D ( 'NONE', #25997, #55231, #43319 ) ;
#18740=PLANE ( 'NONE',  #46433 ) ;
#18741=FACE_OUTER_BOUND ( 'NONE', #44089, .T. ) ;
#18742=DIRECTION ( 'NONE',  ( 0.5364919789714477361, 0.6444004775717706579, 0.5449076811759711036 ) ) ;
#18743=FACE_OUTER_BOUND ( 'NONE', #25708, .T. ) ;
#18744=CARTESIAN_POINT ( 'NONE',  ( -11.60403506841546850, 0.000000000000000000, 2.714115478856362174 ) ) ;
#18745=EDGE_CURVE ( 'NONE', #24514, #8995, #45970, .T. ) ;
#18746=CARTESIAN_POINT ( 'NONE',  ( -12.60458797795435615, 0.000000000000000000, 11.86609696750642229 ) ) ;
#18748=EDGE_CURVE ( 'NONE', #17790, #8254, #2769, .T. ) ;
#18749=AXIS2_PLACEMENT_3D ( 'NONE', #49065, #10164, #40270 ) ;
#18750=VECTOR ( 'NONE', #35300, 1000.000000000000227 ) ;
#18751=LINE ( 'NONE', #19570, #26586 ) ;
#18752=FILL_AREA_STYLE ('',( #49099 ) ) ;
#18753=CARTESIAN_POINT ( 'NONE',  ( -13.00501152033857544, 0.000000000000000000, 3.611202909362837055 ) ) ;
#18754=ORIENTED_EDGE ( 'NONE', *, *, #48078, .T. ) ;
#18755=DIRECTION ( 'NONE',  ( -0.005961354470445682716, -0.6427876096865404731, 0.7660212471507180654 ) ) ;
#18756=LINE ( 'NONE', #56042, #3359 ) ;
#18757=EDGE_CURVE ( 'NONE', #44098, #40790, #7327, .T. ) ;
#18758=LINE ( 'NONE', #15045, #28222 ) ;
#18759=DIRECTION ( 'NONE',  ( 0.5364919789714477361, 0.6444004775717706579, 0.5449076811759711036 ) ) ;
#18760=EDGE_CURVE ( 'NONE', #47831, #48336, #36605, .T. ) ;
#18761=CARTESIAN_POINT ( 'NONE',  ( -9.502280557099082259, 0.000000000000000000, 5.485122320679733043 ) ) ;
#18762=CARTESIAN_POINT ( 'NONE',  ( -15.56423498968618269, 0.000000000000000000, 8.223277334462750332 ) ) ;
#18763=ADVANCED_FACE ( 'NONE', ( #54208 ), #50208, .F. ) ;
#18764=CARTESIAN_POINT ( 'NONE',  ( -13.69419118830071014, 0.000000000000000000, 6.760502168503728093 ) ) ;
#18765=AXIS2_PLACEMENT_3D ( 'NONE', #9664, #26979, #26387 ) ;
#18766=ORIENTED_EDGE ( 'NONE', *, *, #35101, .T. ) ;
#18767=ORIENTED_EDGE ( 'NONE', *, *, #14851, .F. ) ;
#18768=LINE ( 'NONE', #48858, #2318 ) ;
#18770=DIRECTION ( 'NONE',  ( 0.5449076811759707706, 0.6444004775717708799, -0.5364919789714476250 ) ) ;
#18771=EDGE_CURVE ( 'NONE', #56039, #23328, #49920, .T. ) ;
#18772=EDGE_LOOP ( 'NONE', ( #36219, #37141, #24336, #54567 ) ) ;
#18773=DIRECTION ( 'NONE',  ( -0.005961354470445682716, -0.6427876096865404731, 0.7660212471507180654 ) ) ;
#18774=AXIS2_PLACEMENT_3D ( 'NONE', #16294, #45847, #37605 ) ;
#18775=ORIENTED_EDGE ( 'NONE', *, *, #23792, .F. ) ;
#18776=DIRECTION ( 'NONE',  ( -0.6427681459581293666, -0.7660444431189770143, -0.005002170337467561935 ) ) ;
#18777=ADVANCED_FACE ( 'NONE', ( #53632 ), #2518, .F. ) ;
#18778=VECTOR ( 'NONE', #13762, 1000.000000000000114 ) ;
#18780=EDGE_LOOP ( 'NONE', ( #20349, #40724, #16087 ) ) ;
#18781=ORIENTED_EDGE ( 'NONE', *, *, #35590, .T. ) ;
#18782=DIRECTION ( 'NONE',  ( 0.9321478471874538041, 0.000000000000000000, -0.3620778797217461542 ) ) ;
#18783=CARTESIAN_POINT ( 'NONE',  ( -15.09959809284509902, 0.000000000000000000, 8.226893246230758905 ) ) ;
#18784=LINE ( 'NONE', #19869, #30280 ) ;
#18785=VECTOR ( 'NONE', #43987, 1000.000000000000227 ) ;
#18786=FACE_OUTER_BOUND ( 'NONE', #27987, .T. ) ;
#18787=ORIENTED_EDGE ( 'NONE', *, *, #29882, .T. ) ;
#18788=ORIENTED_EDGE ( 'NONE', *, *, #36952, .F. ) ;
#18789=VECTOR ( 'NONE', #38652, 999.9999999999998863 ) ;
#18791=ORIENTED_EDGE ( 'NONE', *, *, #53436, .T. ) ;
#18792=CARTESIAN_POINT ( 'NONE',  ( -13.38856572258804611, -5.375054281893163477, 10.70388513002829178 ) ) ;
#18793=ORIENTED_EDGE ( 'NONE', *, *, #15087, .F. ) ;
#18795=CARTESIAN_POINT ( 'NONE',  ( 2.072287782118878319, 0.000000000000000000, -2.950529333540147015 ) ) ;
#18796=EDGE_LOOP ( 'NONE', ( #15356, #55226, #15945, #4436 ) ) ;
#18797=CARTESIAN_POINT ( 'NONE',  ( 2.072287782118878319, 0.000000000000000000, -2.950529333540147015 ) ) ;
#18798=EDGE_CURVE ( 'NONE', #55742, #24350, #28650, .T. ) ;
#18799=ORIENTED_EDGE ( 'NONE', *, *, #33611, .T. ) ;
#18800=LINE ( 'NONE', #23043, #53593 ) ;
#18801=ORIENTED_EDGE ( 'NONE', *, *, #3711, .T. ) ;
#18802=CARTESIAN_POINT ( 'NONE',  ( -14.41197482399896401, 0.000000000000000000, 5.277587931052655001 ) ) ;
#18803=DIRECTION ( 'NONE',  ( -0.7660212471507179544, -0.6427876096865405842, -0.005961354470445141482 ) ) ;
#18804=DIRECTION ( 'NONE',  ( 0.5364919789714477361, 0.6444004775717706579, 0.5449076811759711036 ) ) ;
#18805=ORIENTED_EDGE ( 'NONE', *, *, #42502, .F. ) ;
#18806=EDGE_CURVE ( 'NONE', #46599, #31490, #14740, .T. ) ;
#18807=PLANE ( 'NONE',  #36483 ) ;
#18810=ADVANCED_FACE ( 'NONE', ( #45668 ), #49678, .F. ) ;
#18811=CARTESIAN_POINT ( 'NONE',  ( -16.33317936670417225, 0.000000000000000000, 13.31440848639340224 ) ) ;
#18812=CARTESIAN_POINT ( 'NONE',  ( -9.914677157360957338, -0.6196009389936254497, 1.468675650391051413 ) ) ;
#18813=EDGE_CURVE ( 'NONE', #9942, #19401, #10773, .T. ) ;
#18814=VECTOR ( 'NONE', #9822, 1000.000000000000000 ) ;
#18816=ORIENTED_EDGE ( 'NONE', *, *, #12958, .T. ) ;
#18817=LINE ( 'NONE', #31595, #29834 ) ;
#18818=CARTESIAN_POINT ( 'NONE',  ( -17.22698034098230480, 0.000000000000000000, 8.748995549059454646 ) ) ;
#18820=ORIENTED_EDGE ( 'NONE', *, *, #43869, .F. ) ;
#18821=LINE ( 'NONE', #40675, #54664 ) ;
#18822=CARTESIAN_POINT ( 'NONE',  ( -19.60834386242827776, 0.000000000000000000, 4.298478389818581213 ) ) ;
#18823=EDGE_LOOP ( 'NONE', ( #17046, #27213, #39843, #510 ) ) ;
#18825=DIRECTION ( 'NONE',  ( 0.9999697198139515519, 0.000000000000000000, 0.007781995580013368816 ) ) ;
#18826=CARTESIAN_POINT ( 'NONE',  ( -19.55390298301616525, 4.172053068839008283, 11.32377094424822772 ) ) ;
#18827=ADVANCED_FACE ( 'NONE', ( #1937 ), #19269, .F. ) ;
#18829=ORIENTED_EDGE ( 'NONE', *, *, #11620, .T. ) ;
#18831=DIRECTION ( 'NONE',  ( 0.000000000000000000, -1.000000000000000000, 0.000000000000000000 ) ) ;
#18832=LINE ( 'NONE', #1758, #15122 ) ;
#18833=DIRECTION ( 'NONE',  ( -0.5364919789714478471, 0.6444004775717705469, -0.5449076811759709926 ) ) ;
#18834=EDGE_CURVE ( 'NONE', #50938, #606, #43111, .T. ) ;
#18835=DIRECTION ( 'NONE',  ( -0.7660212471507179544, -0.6427876096865405842, -0.005961354470445141482 ) ) ;
#18836=VERTEX_POINT ( 'NONE', #13005 ) ;
#18838=ORIENTED_EDGE ( 'NONE', *, *, #19930, .F. ) ;
#18839=LINE ( 'NONE', #53460, #12059 ) ;
#18840=ADVANCED_FACE ( 'NONE', ( #47650 ), #12153, .F. ) ;
#18841=CARTESIAN_POINT ( 'NONE',  ( -16.99924723426068951, 0.000000000000000000, 13.49389102713827171 ) ) ;
#18842=VERTEX_POINT ( 'NONE', #34573 ) ;
#18843=FACE_OUTER_BOUND ( 'NONE', #47364, .T. ) ;
#18844=CARTESIAN_POINT ( 'NONE',  ( -12.23078190322307357, -4.565544526780662693, 8.925619156330617088 ) ) ;
#18845=CARTESIAN_POINT ( 'NONE',  ( -17.89316758090218329, 0.000000000000000000, 8.943817182138230848 ) ) ;
#18846=VERTEX_POINT ( 'NONE', #51044 ) ;
#18847=DIRECTION ( 'NONE',  ( 0.5449076811759707706, 0.6444004775717708799, -0.5364919789714476250 ) ) ;
#18848=EDGE_LOOP ( 'NONE', ( #22547, #9525, #5417, #991 ) ) ;
#18849=VERTEX_POINT ( 'NONE', #8770 ) ;
#18850=VECTOR ( 'NONE', #11629, 1000.000000000000227 ) ;
#18851=ORIENTED_EDGE ( 'NONE', *, *, #7019, .T. ) ;
#18852=CARTESIAN_POINT ( 'NONE',  ( -8.875996589204540044, 0.000000000000000000, 10.41778544861944233 ) ) ;
#18853=ORIENTED_EDGE ( 'NONE', *, *, #43659, .T. ) ;
#18854=CARTESIAN_POINT ( 'NONE',  ( 2.072287782118878319, 0.000000000000000000, -2.950529333540147015 ) ) ;
#18855=ORIENTED_EDGE ( 'NONE', *, *, #43055, .F. ) ;
#18856=DIRECTION ( 'NONE',  ( 0.9321478471874541372, 0.000000000000000000, -0.3620778797217453771 ) ) ;
#18857=PLANE ( 'NONE',  #9573 ) ;
#18858=VECTOR ( 'NONE', #8900, 1000.000000000000114 ) ;
#18859=ORIENTED_EDGE ( 'NONE', *, *, #41523, .T. ) ;
#18860=LINE ( 'NONE', #40441, #24026 ) ;
#18861=EDGE_CURVE ( 'NONE', #34678, #34282, #38006, .T. ) ;
#18862=ORIENTED_EDGE ( 'NONE', *, *, #27613, .T. ) ;
#18863=CARTESIAN_POINT ( 'NONE',  ( -16.92653109165133429, 0.000000000000000000, 4.150022863323312272 ) ) ;
#18864=EDGE_CURVE ( 'NONE', #39352, #14416, #16403, .T. ) ;
#18865=DIRECTION ( 'NONE',  ( 0.6427681459581294776, -0.7660444431189769032, 0.005002170337467562802 ) ) ;
#18867=ADVANCED_FACE ( 'NONE', ( #7925 ), #42267, .F. ) ;
#18869=CARTESIAN_POINT ( 'NONE',  ( -13.46545670928509431, 0.000000000000000000, 3.068961535042087796 ) ) ;
#18870=DIRECTION ( 'NONE',  ( -0.005961354470445682716, -0.6427876096865404731, 0.7660212471507180654 ) ) ;
#18872=ORIENTED_EDGE ( 'NONE', *, *, #13023, .F. ) ;
#18873=EDGE_CURVE ( 'NONE', #50295, #8803, #42544, .T. ) ;
#18874=EDGE_CURVE ( 'NONE', #8988, #30987, #47080, .T. ) ;
#18875=ADVANCED_FACE ( 'NONE', ( #3372 ), #20691, .F. ) ;
#18876=ORIENTED_EDGE ( 'NONE', *, *, #44605, .F. ) ;
#18877=DIRECTION ( 'NONE',  ( 0.007781995580012663651, 0.000000000000000000, -0.9999697198139515519 ) ) ;
#18878=CARTESIAN_POINT ( 'NONE',  ( -11.31245753787399089, -1.327505506330657781, 1.233109421660533833 ) ) ;
#18879=PLANE ( 'NONE',  #36056 ) ;
#18880=CARTESIAN_POINT ( 'NONE',  ( -10.88337737921193948, 0.000000000000000000, 3.827720013049670023 ) ) ;
#18881=EDGE_LOOP ( 'NONE', ( #19237, #1064, #48376, #51659 ) ) ;
#18882=CARTESIAN_POINT ( 'NONE',  ( -14.94916102560700821, 0.000000000000000000, 2.688082935172642962 ) ) ;
#18883=DIRECTION ( 'NONE',  ( -0.9999697198139514409, -0.000000000000000000, -0.007781995580013368816 ) ) ;
#18884=EDGE_LOOP ( 'NONE', ( #19263, #16363, #21626, #39090 ) ) ;
#18885=DIRECTION ( 'NONE',  ( 0.000000000000000000, -0.000000000000000000, -1.000000000000000000 ) ) ;
#18886=DIRECTION ( 'NONE',  ( -0.005961354470445682716, -0.6427876096865404731, 0.7660212471507180654 ) ) ;
#18887=ORIENTED_EDGE ( 'NONE', *, *, #32404, .T. ) ;
#18889=CARTESIAN_POINT ( 'NONE',  ( -11.37769377693735962, 0.000000000000000000, 7.637856226733343412 ) ) ;
#18890=EDGE_CURVE ( 'NONE', #48904, #34052, #3062, .T. ) ;
#18891=CARTESIAN_POINT ( 'NONE',  ( -17.46532115785441519, 0.000000000000000000, 13.67492996699914265 ) ) ;
#18892=DIRECTION ( 'NONE',  ( 0.000000000000000000, -1.000000000000000000, 0.000000000000000000 ) ) ;
#18893=EDGE_CURVE ( 'NONE', #23668, #50643, #8186, .T. ) ;
#18894=CARTESIAN_POINT ( 'NONE',  ( -27.99923088623136636, 0.000000000000000000, 7.757173251277078130 ) ) ;
#18895=ORIENTED_EDGE ( 'NONE', *, *, #6002, .T. ) ;
#18896=EDGE_LOOP ( 'NONE', ( #45562, #29844, #30527, #6517 ) ) ;
#18897=EDGE_CURVE ( 'NONE', #25320, #17870, #20392, .T. ) ;
#18898=DIRECTION ( 'NONE',  ( -0.7660212471507179544, -0.6427876096865405842, -0.005961354470445141482 ) ) ;
#18899=DIRECTION ( 'NONE',  ( 0.005961354470445682716, -0.6427876096865404731, -0.7660212471507180654 ) ) ;
#18900=CARTESIAN_POINT ( 'NONE',  ( -14.46888367232926420, 0.000000000000000000, 12.59025272694991315 ) ) ;
#18901=EDGE_CURVE ( 'NONE', #10313, #25745, #47350, .T. ) ;
#18902=VECTOR ( 'NONE', #7209, 1000.000000000000227 ) ;
#18903=DIRECTION ( 'NONE',  ( 0.9999697198139515519, 0.000000000000000000, 0.007781995580013368816 ) ) ;
#18904=CARTESIAN_POINT ( 'NONE',  ( -8.186969886387416295, 7.982592133067664797, 6.398470710204317236 ) ) ;
#18905=ORIENTED_EDGE ( 'NONE', *, *, #18189, .T. ) ;
#18906=DIRECTION ( 'NONE',  ( 0.7660212471507180654, -0.6427876096865404731, 0.005961354470445141482 ) ) ;
#18907=PLANE ( 'NONE',  #3922 ) ;
#18908=LINE ( 'NONE', #6394, #7817 ) ;
#18909=LINE ( 'NONE', #5841, #13337 ) ;
#18910=VERTEX_POINT ( 'NONE', #7615 ) ;
#18911=DIRECTION ( 'NONE',  ( -0.005002170337468016433, -0.7660444431189770143, 0.6427681459581293666 ) ) ;
#18912=VERTEX_POINT ( 'NONE', #42804 ) ;
#18913=LINE ( 'NONE', #45851, #22314 ) ;
#18914=CARTESIAN_POINT ( 'NONE',  ( -21.12007069142898885, 1.095915999411505082, 6.883658674416231804 ) ) ;
#18915=ORIENTED_EDGE ( 'NONE', *, *, #27342, .T. ) ;
#18916=LINE ( 'NONE', #44732, #6393 ) ;
#18918=VERTEX_POINT ( 'NONE', #8459 ) ;
#18919=ORIENTED_EDGE ( 'NONE', *, *, #12533, .T. ) ;
#18920=DIRECTION ( 'NONE',  ( -0.5364919789714478471, 0.6444004775717705469, -0.5449076811759709926 ) ) ;
#18921=VERTEX_POINT ( 'NONE', #38268 ) ;
#18922=VERTEX_POINT ( 'NONE', #37734 ) ;
#18923=CARTESIAN_POINT ( 'NONE',  ( -17.46532115785441519, 0.000000000000000000, 13.67492996699914265 ) ) ;
#18924=CARTESIAN_POINT ( 'NONE',  ( -15.40103151951671734, 0.000000000000000000, 12.95233060667165681 ) ) ;
#18925=EDGE_LOOP ( 'NONE', ( #13797, #55407, #18707, #14994 ) ) ;
#18927=LINE ( 'NONE', #31437, #5015 ) ;
#18928=ORIENTED_EDGE ( 'NONE', *, *, #21951, .T. ) ;
#18929=EDGE_CURVE ( 'NONE', #41830, #38527, #55591, .T. ) ;
#18930=ORIENTED_EDGE ( 'NONE', *, *, #38865, .T. ) ;
#18931=DIRECTION ( 'NONE',  ( 0.000000000000000000, -0.000000000000000000, -1.000000000000000000 ) ) ;
#18932=DIRECTION ( 'NONE',  ( 0.7660212471507180654, -0.6427876096865404731, 0.005961354470445141482 ) ) ;
#18933=DIRECTION ( 'NONE',  ( 0.005002170337468016433, -0.7660444431189770143, -0.6427681459581293666 ) ) ;
#18934=DIRECTION ( 'NONE',  ( -0.005002170337468016433, -0.7660444431189770143, 0.6427681459581293666 ) ) ;
#18935=EDGE_LOOP ( 'NONE', ( #47483, #21170, #37471, #17880 ) ) ;
#18936=CARTESIAN_POINT ( 'NONE',  ( -11.84270936233621008, 0.000000000000000000, 7.682900981386271866 ) ) ;
#18937=VERTEX_POINT ( 'NONE', #17251 ) ;
#18938=EDGE_CURVE ( 'NONE', #55190, #52574, #56167, .T. ) ;
#18939=EDGE_CURVE ( 'NONE', #38452, #165, #12465, .T. ) ;
#18940=ADVANCED_FACE ( 'NONE', ( #55896 ), #34316, .F. ) ;
#18941=AXIS2_PLACEMENT_3D ( 'NONE', #39556, #4898, #38981 ) ;
#18942=DIRECTION ( 'NONE',  ( -0.5449076811759708816, 0.6444004775717707689, 0.5364919789714475140 ) ) ;
#18943=ADVANCED_FACE ( 'NONE', ( #31467 ), #31158, .F. ) ;
#18944=DIRECTION ( 'NONE',  ( 0.007781995580012662783, 0.000000000000000000, -0.9999697198139514409 ) ) ;
#18945=DIRECTION ( 'NONE',  ( -0.9999697198139514409, -0.000000000000000000, -0.007781995580013368816 ) ) ;
#18946=DIRECTION ( 'NONE',  ( 0.5364919789714477361, 0.6444004775717706579, 0.5449076811759711036 ) ) ;
#18947=CARTESIAN_POINT ( 'NONE',  ( -28.93060053386082231, -0.1191753592594197858, 8.019254159017428663 ) ) ;
#18948=CARTESIAN_POINT ( 'NONE',  ( -24.26986129792355129, -0.1191753592594197858, 6.208864760408702388 ) ) ;
#18949=ORIENTED_EDGE ( 'NONE', *, *, #52297, .F. ) ;
#18950=DIRECTION ( 'NONE',  ( -0.9999697198139514409, -0.000000000000000000, -0.007781995580013368816 ) ) ;
#18951=ORIENTED_EDGE ( 'NONE', *, *, #41517, .F. ) ;
#18952=DIRECTION ( 'NONE',  ( -0.005961354470445682716, -0.6427876096865404731, 0.7660212471507180654 ) ) ;
#18953=CARTESIAN_POINT ( 'NONE',  ( -21.47341775636118655, -0.1191753592594197858, 5.122631121243466090 ) ) ;
#18954=PLANE ( 'NONE',  #11806 ) ;
#18955=FACE_OUTER_BOUND ( 'NONE', #27320, .T. ) ;
#18956=ADVANCED_FACE ( 'NONE', ( #35173 ), #18371, .F. ) ;
#18957=CARTESIAN_POINT ( 'NONE',  ( -12.60458797795435615, 0.000000000000000000, 11.86609696750642229 ) ) ;
#18959=ORIENTED_EDGE ( 'NONE', *, *, #33796, .F. ) ;
#18962=FACE_OUTER_BOUND ( 'NONE', #48745, .T. ) ;
#18964=ADVANCED_FACE ( 'NONE', ( #16899 ), #34230, .F. ) ;
#18965=CARTESIAN_POINT ( 'NONE',  ( -14.46888367232926420, 0.000000000000000000, 12.59025272694991315 ) ) ;
#18966=DIRECTION ( 'NONE',  ( -0.7660212471507179544, -0.6427876096865405842, -0.005961354470445141482 ) ) ;
#18967=PLANE ( 'NONE',  #39224 ) ;
#18968=EDGE_CURVE ( 'NONE', #29513, #55994, #12046, .T. ) ;
#18969=CARTESIAN_POINT ( 'NONE',  ( -16.07347840383240012, -3.108426967578160838, 3.025630892186666809 ) ) ;
#18970=LINE ( 'NONE', #2479, #32864 ) ;
#18971=ORIENTED_EDGE ( 'NONE', *, *, #24050, .T. ) ;
#18972=EDGE_LOOP ( 'NONE', ( #29361, #54339, #17033, #30674 ) ) ;
#18973=ORIENTED_EDGE ( 'NONE', *, *, #33967, .F. ) ;
#18975=ORIENTED_EDGE ( 'NONE', *, *, #43848, .T. ) ;
#18976=CARTESIAN_POINT ( 'NONE',  ( -33.59056157024009082, 0.000000000000000000, 9.729646585644761814 ) ) ;
#18977=LINE ( 'NONE', #6750, #53886 ) ;
#18978=VERTEX_POINT ( 'NONE', #25986 ) ;
#18979=EDGE_LOOP ( 'NONE', ( #51227, #11084, #34471, #22869 ) ) ;
#18980=VERTEX_POINT ( 'NONE', #8093 ) ;
#18981=DIRECTION ( 'NONE',  ( 0.5449076811759707706, 0.6444004775717708799, -0.5364919789714476250 ) ) ;
#18982=LINE ( 'NONE', #50181, #11953 ) ;
#18983=DIRECTION ( 'NONE',  ( 0.005002170337468016433, -0.7660444431189770143, -0.6427681459581293666 ) ) ;
#18984=ORIENTED_EDGE ( 'NONE', *, *, #35132, .F. ) ;
#18985=DIRECTION ( 'NONE',  ( 0.5364919789714477361, 0.6444004775717706579, 0.5449076811759711036 ) ) ;
#18986=EDGE_CURVE ( 'NONE', #345, #33161, #4112, .T. ) ;
#18988=LINE ( 'NONE', #36306, #32783 ) ;
#18989=DIRECTION ( 'NONE',  ( 0.007781995580012663651, -3.146120232559066537E-19, -0.9999697198139514409 ) ) ;
#18990=EDGE_CURVE ( 'NONE', #50596, #39497, #42451, .T. ) ;
#18991=EDGE_CURVE ( 'NONE', #34361, #30589, #37912, .T. ) ;
#18992=DIRECTION ( 'NONE',  ( 0.005002170337468016433, -0.7660444431189770143, -0.6427681459581293666 ) ) ;
#18993=DIRECTION ( 'NONE',  ( -0.005002170337468016433, -0.7660444431189770143, 0.6427681459581293666 ) ) ;
#18994=LINE ( 'NONE', #36311, #36762 ) ;
#18995=CARTESIAN_POINT ( 'NONE',  ( 2.072287782118878319, 0.000000000000000000, -2.950529333540147015 ) ) ;
#18996=PLANE ( 'NONE',  #11296 ) ;
#18997=VERTEX_POINT ( 'NONE', #3807 ) ;
#18998=LINE ( 'NONE', #48830, #48256 ) ;
#18999=VERTEX_POINT ( 'NONE', #43555 ) ;
#19001=CARTESIAN_POINT ( 'NONE',  ( -14.00280974873554030, 0.000000000000000000, 12.40921378708904044 ) ) ;
#19002=CARTESIAN_POINT ( 'NONE',  ( -20.54126990917373519, -0.1191753592594197858, 4.760553241521720658 ) ) ;
#19003=CARTESIAN_POINT ( 'NONE',  ( -8.956466202847114033, -0.1191753592594181482, 6.697369211722168814 ) ) ;
#19004=CARTESIAN_POINT ( 'NONE',  ( -14.54398777498582618, 1.581621852479005552, 5.126410796805221715 ) ) ;
#19005=CARTESIAN_POINT ( 'NONE',  ( -17.70545686808230101, 0.9340140483890051470, 3.529532520656252448 ) ) ;
#19006=DIRECTION ( 'NONE',  ( 0.9999697198139515519, 0.000000000000000000, 0.007781995580013368816 ) ) ;
#19007=DIRECTION ( 'NONE',  ( 0.007781995580012663651, -3.146120232559066537E-19, -0.9999697198139514409 ) ) ;
#19008=CARTESIAN_POINT ( 'NONE',  ( -15.42828644624678169, -0.6798977022406558213, 2.852499223360160929 ) ) ;
#19009=SHAPE_REPRESENTATION_RELATIONSHIP ( 'NONE' , 'NONE' ,  #12294, #29299 ) ;
#19010=PLANE ( 'NONE',  #14739 ) ;
#19011=EDGE_LOOP ( 'NONE', ( #9706, #54369, #45052, #48000 ) ) ;
#19012=DIRECTION ( 'NONE',  ( 0.005961354470445682716, -0.6427876096865404731, -0.7660212471507180654 ) ) ;
#19013=LINE ( 'NONE', #19575, #4074 ) ;
#19014=DIRECTION ( 'NONE',  ( 0.005961354470445682716, -0.6427876096865404731, -0.7660212471507180654 ) ) ;
#19015=LINE ( 'NONE', #9371, #55769 ) ;
#19016=CARTESIAN_POINT ( 'NONE',  ( -27.99845268667336384, -0.1191753592594197858, 7.657176279295684118 ) ) ;
#19017=ADVANCED_FACE ( 'NONE', ( #30228 ), #21130, .F. ) ;
#19019=CARTESIAN_POINT ( 'NONE',  ( -18.04694319155812821, 0.7721120973665051013, 5.158534221716275958 ) ) ;
#19020=ORIENTED_EDGE ( 'NONE', *, *, #31442, .F. ) ;
#19021=ORIENTED_EDGE ( 'NONE', *, *, #49041, .T. ) ;
#19022=ADVANCED_FACE ( 'NONE', ( #7824 ), #46701, .F. ) ;
#19023=DIRECTION ( 'NONE',  ( 0.6427681459581294776, -0.7660444431189769032, 0.005002170337467562802 ) ) ;
#19024=LINE ( 'NONE', #26411, #8718 ) ;
#19025=ORIENTED_EDGE ( 'NONE', *, *, #37680, .F. ) ;
#19026=LINE ( 'NONE', #9956, #1372 ) ;
#19027=ADVANCED_FACE ( 'NONE', ( #33923 ), #12629, .F. ) ;
#19029=DIRECTION ( 'NONE',  ( 0.7660212471507180654, -0.6427876096865404731, 0.005961354470445141482 ) ) ;
#19030=ORIENTED_EDGE ( 'NONE', *, *, #55323, .F. ) ;
#19031=ORIENTED_EDGE ( 'NONE', *, *, #46294, .T. ) ;
#19032=EDGE_LOOP ( 'NONE', ( #26189, #47494, #12390, #32789 ) ) ;
#19033=DIRECTION ( 'NONE',  ( 0.005961354470445682716, -0.6427876096865404731, -0.7660212471507180654 ) ) ;
#19034=DIRECTION ( 'NONE',  ( -0.9999697198139514409, -0.000000000000000000, -0.007781995580013368816 ) ) ;
#19035=CARTESIAN_POINT ( 'NONE',  ( -21.47419595591918906, 0.000000000000000000, 5.222628093224860102 ) ) ;
#19036=EDGE_LOOP ( 'NONE', ( #50797, #20017, #39199, #27478 ) ) ;
#19038=PLANE ( 'NONE',  #48143 ) ;
#19039=ORIENTED_EDGE ( 'NONE', *, *, #23325, .F. ) ;
#19040=CARTESIAN_POINT ( 'NONE',  ( -15.40103151951671734, 0.000000000000000000, 12.95233060667165681 ) ) ;
#19041=EDGE_CURVE ( 'NONE', #15321, #29206, #38764, .T. ) ;
#19042=EDGE_LOOP ( 'NONE', ( #31971, #50865, #54481, #2047 ) ) ;
#19043=LINE ( 'NONE', #28699, #48455 ) ;
#19045=ORIENTED_EDGE ( 'NONE', *, *, #45436, .F. ) ;
#19046=CARTESIAN_POINT ( 'NONE',  ( -13.07066190154808361, 0.000000000000000000, 12.04713590736729678 ) ) ;
#19047=EDGE_LOOP ( 'NONE', ( #22841, #28104, #8691, #19478 ) ) ;
#19048=EDGE_CURVE ( 'NONE', #8803, #3951, #35072, .T. ) ;
#19049=PLANE ( 'NONE',  #14608 ) ;
#19050=EDGE_LOOP ( 'NONE', ( #44398, #22107, #4242, #26587 ) ) ;
#19051=DIRECTION ( 'NONE',  ( -0.6427681459581293666, -0.7660444431189770143, -0.005002170337467561935 ) ) ;
#19052=DIRECTION ( 'NONE',  ( 0.007781995580012662783, 0.000000000000000000, -0.9999697198139514409 ) ) ;
#19053=DIRECTION ( 'NONE',  ( -0.6427681459581293666, -0.7660444431189770143, -0.005002170337467561935 ) ) ;
#19054=VERTEX_POINT ( 'NONE', #27088 ) ;
#19055=FACE_OUTER_BOUND ( 'NONE', #12923, .T. ) ;
#19056=CARTESIAN_POINT ( 'NONE',  ( -9.342070512798265725, 0.000000000000000000, 10.59882438848031505 ) ) ;
#19057=CARTESIAN_POINT ( 'NONE',  ( -21.15203641687357461, -2.460819163488157546, 8.936724485154998732 ) ) ;
#19058=CARTESIAN_POINT ( 'NONE',  ( -19.18055499287547860, -0.1191753592594166911, 8.095131267895274263 ) ) ;
#19059=DIRECTION ( 'NONE',  ( 0.7660212471507180654, -0.6427876096865404731, 0.005961354470445141482 ) ) ;
#19060=PLANE ( 'NONE',  #49697 ) ;
#19061=EDGE_CURVE ( 'NONE', #45704, #36899, #40131, .T. ) ;
#19062=VECTOR ( 'NONE', #31731, 1000.000000000000227 ) ;
#19064=ORIENTED_EDGE ( 'NONE', *, *, #54626, .T. ) ;
#19065=DIRECTION ( 'NONE',  ( 0.007781995580012663651, 0.000000000000000000, -0.9999697198139515519 ) ) ;
#19066=LINE ( 'NONE', #44619, #2303 ) ;
#19069=CARTESIAN_POINT ( 'NONE',  ( -15.82157343643791236, 0.000000000000000000, 7.282604471332424723 ) ) ;
#19070=CARTESIAN_POINT ( 'NONE',  ( -14.02358693954004210, -0.1191753592594190225, 2.228863834670655741 ) ) ;
#19071=DIRECTION ( 'NONE',  ( 0.9999697198139515519, 0.000000000000000000, 0.007781995580013368816 ) ) ;
#19072=DIRECTION ( 'NONE',  ( -0.9999697198139514409, -0.000000000000000000, -0.007781995580013368816 ) ) ;
#19073=LINE ( 'NONE', #50000, #41084 ) ;
#19074=VERTEX_POINT ( 'NONE', #10325 ) ;
#19075=VERTEX_POINT ( 'NONE', #53479 ) ;
#19077=CARTESIAN_POINT ( 'NONE',  ( 2.072287782118878319, 0.000000000000000000, -2.950529333540147015 ) ) ;
#19078=DIRECTION ( 'NONE',  ( 0.005961354470445682716, -0.6427876096865404731, -0.7660212471507180654 ) ) ;
#19079=CARTESIAN_POINT ( 'NONE',  ( -19.84220772623944740, 1.257817950434005683, 4.349188078554292680 ) ) ;
#19080=ORIENTED_EDGE ( 'NONE', *, *, #20488, .T. ) ;
#19081=PLANE ( 'NONE',  #43938 ) ;
#19082=EDGE_CURVE ( 'NONE', #19083, #33225, #52376, .T. ) ;
#19083=VERTEX_POINT ( 'NONE', #48369 ) ;
#19084=DIRECTION ( 'NONE',  ( -0.005961354470445682716, -0.6427876096865404731, 0.7660212471507180654 ) ) ;
#19085=DIRECTION ( 'NONE',  ( -0.5364919789714478471, 0.6444004775717705469, -0.5449076811759709926 ) ) ;
#19086=ORIENTED_EDGE ( 'NONE', *, *, #13742, .T. ) ;
#19087=FACE_OUTER_BOUND ( 'NONE', #46100, .T. ) ;
#19088=DIRECTION ( 'NONE',  ( 0.6427681459581294776, -0.7660444431189769032, 0.005002170337467562802 ) ) ;
#19089=DIRECTION ( 'NONE',  ( 0.005961354470445682716, -0.6427876096865404731, -0.7660212471507180654 ) ) ;
#19091=EDGE_LOOP ( 'NONE', ( #4262, #23337, #5521, #23355 ) ) ;
#19092=DIRECTION ( 'NONE',  ( 0.007781995580012663651, -3.146120232559066537E-19, -0.9999697198139514409 ) ) ;
#19093=VERTEX_POINT ( 'NONE', #52627 ) ;
#19094=ADVANCED_FACE ( 'NONE', ( #13475 ), #941, .F. ) ;
#19095=ADVANCED_FACE ( 'NONE', ( #53224 ), #14579, .F. ) ;
#19096=AXIS2_PLACEMENT_3D ( 'NONE', #2012, #10589, #24188 ) ;
#19097=EDGE_LOOP ( 'NONE', ( #45873, #15517, #46640, #15691 ) ) ;
#19098=VERTEX_POINT ( 'NONE', #48090 ) ;
#19099=PLANE ( 'NONE',  #51281 ) ;
#19100=EDGE_LOOP ( 'NONE', ( #9973, #2871, #16865, #38941 ) ) ;
#19101=CARTESIAN_POINT ( 'NONE',  ( -16.81902912537577777, -2.298917212465658277, 6.987928619639786731 ) ) ;
#19102=EDGE_CURVE ( 'NONE', #9089, #26894, #9783, .T. ) ;
#19103=VERTEX_POINT ( 'NONE', #22552 ) ;
#19104=CARTESIAN_POINT ( 'NONE',  ( -13.45970860227452981, 0.000000000000000000, 2.330342128526559087 ) ) ;
#19105=CARTESIAN_POINT ( 'NONE',  ( -9.597601843825197321, -1.410310748667299885, 2.284967082322166387 ) ) ;
#19106=ORIENTED_EDGE ( 'NONE', *, *, #10615, .F. ) ;
#19107=ADVANCED_FACE ( 'NONE', ( #14324 ), #22812, .F. ) ;
#19108=CARTESIAN_POINT ( 'NONE',  ( -27.99767448711536133, 0.000000000000000000, 7.557179307314289218 ) ) ;
#19109=ORIENTED_EDGE ( 'NONE', *, *, #44884, .T. ) ;
#19110=EDGE_CURVE ( 'NONE', #40075, #15737, #10037, .T. ) ;
#19111=DIRECTION ( 'NONE',  ( -0.005002170337468016433, -0.7660444431189770143, 0.6427681459581293666 ) ) ;
#19112=CARTESIAN_POINT ( 'NONE',  ( -9.808144436391993182, 0.000000000000000000, 10.77986332834118777 ) ) ;
#19113=LINE ( 'NONE', #52926, #1449 ) ;
#19115=CARTESIAN_POINT ( 'NONE',  ( -16.33317936670417225, 0.000000000000000000, 13.31440848639340224 ) ) ;
#19116=DIRECTION ( 'NONE',  ( 0.9999697198139515519, 0.000000000000000000, 0.007781995580013368816 ) ) ;
#19117=CARTESIAN_POINT ( 'NONE',  ( -10.47421230394850866, 0.000000000000000000, 10.95934586908605723 ) ) ;
#19118=ORIENTED_EDGE ( 'NONE', *, *, #51759, .F. ) ;
#19119=EDGE_CURVE ( 'NONE', #47218, #47771, #4658, .T. ) ;
#19120=ORIENTED_EDGE ( 'NONE', *, *, #36604, .T. ) ;
#19122=FACE_OUTER_BOUND ( 'NONE', #38067, .T. ) ;
#19123=DIRECTION ( 'NONE',  ( -0.6427681459581293666, -0.7660444431189770143, -0.005002170337467561935 ) ) ;
#19124=DIRECTION ( 'NONE',  ( 0.5449076811759707706, 0.6444004775717708799, -0.5364919789714476250 ) ) ;
#19125=EDGE_CURVE ( 'NONE', #36112, #3699, #21971, .T. ) ;
#19126=FACE_OUTER_BOUND ( 'NONE', #25457, .T. ) ;
#19127=ORIENTED_EDGE ( 'NONE', *, *, #8971, .T. ) ;
#19128=LINE ( 'NONE', #31382, #37618 ) ;
#19129=DIRECTION ( 'NONE',  ( 0.000000000000000000, -1.000000000000000000, 0.000000000000000000 ) ) ;
#19130=ORIENTED_EDGE ( 'NONE', *, *, #11495, .F. ) ;
#19131=PLANE ( 'NONE',  #10251 ) ;
#19132=PLANE ( 'NONE',  #49435 ) ;
#19133=ORIENTED_EDGE ( 'NONE', *, *, #20953, .T. ) ;
#19135=CARTESIAN_POINT ( 'NONE',  ( -10.14379749791080876, 0.000000000000000000, 0.8788190362434851188 ) ) ;
#19136=VECTOR ( 'NONE', #8515, 999.9999999999998863 ) ;
#19137=LINE ( 'NONE', #41569, #47715 ) ;
#19138=CARTESIAN_POINT ( 'NONE',  ( -12.15116108492864377, 0.000000000000000000, 1.401855352044617975 ) ) ;
#19139=VECTOR ( 'NONE', #41078, 1000.000000000000227 ) ;
#19140=CARTESIAN_POINT ( 'NONE',  ( -16.81190032086591302, 0.000000000000000000, 3.212244750653343583 ) ) ;
#19141=VERTEX_POINT ( 'NONE', #40437 ) ;
#19142=ORIENTED_EDGE ( 'NONE', *, *, #40424, .T. ) ;
#19143=CARTESIAN_POINT ( 'NONE',  ( 2.072287782118878319, 0.000000000000000000, -2.950529333540147015 ) ) ;
#19144=FACE_OUTER_BOUND ( 'NONE', #3868, .T. ) ;
#19145=CARTESIAN_POINT ( 'NONE',  ( -13.04105656151796744, 0.000000000000000000, 8.242913292418799998 ) ) ;
#19146=PLANE ( 'NONE',  #11006 ) ;
#19147=DIRECTION ( 'NONE',  ( -0.5364919789714478471, 0.6444004775717705469, -0.5449076811759709926 ) ) ;
#19148=EDGE_CURVE ( 'NONE', #20170, #27352, #39301, .T. ) ;
#19149=ORIENTED_EDGE ( 'NONE', *, *, #54714, .T. ) ;
#19150=FACE_OUTER_BOUND ( 'NONE', #13250, .T. ) ;
#19151=FACE_OUTER_BOUND ( 'NONE', #28678, .T. ) ;
#19153=VERTEX_POINT ( 'NONE', #389 ) ;
#19154=CARTESIAN_POINT ( 'NONE',  ( -14.64844551421497876, -5.213152330870663320, 10.92755654284354883 ) ) ;
#19155=VERTEX_POINT ( 'NONE', #39607 ) ;
#19157=EDGE_CURVE ( 'NONE', #17736, #33305, #48675, .T. ) ;
#19158=EDGE_CURVE ( 'NONE', #6150, #56189, #35598, .T. ) ;
#19159=PLANE ( 'NONE',  #48382 ) ;
#19160=ORIENTED_EDGE ( 'NONE', *, *, #34088, .F. ) ;
#19161=VECTOR ( 'NONE', #39187, 1000.000000000000227 ) ;
#19162=AXIS2_PLACEMENT_3D ( 'NONE', #8751, #17520, #26068 ) ;
#19163=DIRECTION ( 'NONE',  ( 0.007781995580012663651, 0.000000000000000000, -0.9999697198139515519 ) ) ;
#19166=EDGE_LOOP ( 'NONE', ( #53513, #16260, #31066, #50481 ) ) ;
#19167=ORIENTED_EDGE ( 'NONE', *, *, #29686, .F. ) ;
#19169=ORIENTED_EDGE ( 'NONE', *, *, #24229, .F. ) ;
#19170=VERTEX_POINT ( 'NONE', #2884 ) ;
#19171=DIRECTION ( 'NONE',  ( 0.000000000000000000, -0.000000000000000000, -1.000000000000000000 ) ) ;
#19172=DIRECTION ( 'NONE',  ( 0.007781995580012662783, 0.000000000000000000, -0.9999697198139514409 ) ) ;
#19174=ORIENTED_EDGE ( 'NONE', *, *, #8336, .F. ) ;
#19175=CARTESIAN_POINT ( 'NONE',  ( -12.15116108492864377, 0.000000000000000000, 1.401855352044617975 ) ) ;
#19176=EDGE_CURVE ( 'NONE', #47771, #22086, #41792, .T. ) ;
#19178=VERTEX_POINT ( 'NONE', #49511 ) ;
#19179=VECTOR ( 'NONE', #39154, 1000.000000000000227 ) ;
#19180=EDGE_CURVE ( 'NONE', #9180, #21025, #27939, .T. ) ;
#19181=DIRECTION ( 'NONE',  ( -0.9999697198139514409, -0.000000000000000000, -0.007781995580013368816 ) ) ;
#19182=DIRECTION ( 'NONE',  ( -0.6427681459581293666, -0.7660444431189770143, -0.005002170337467561935 ) ) ;
#19183=CARTESIAN_POINT ( 'NONE',  ( -9.741057028429843001, 0.000000000000000000, 2.159275478707846307 ) ) ;
#19184=FACE_OUTER_BOUND ( 'NONE', #38582, .T. ) ;
#19185=EDGE_LOOP ( 'NONE', ( #17095, #32952, #2122, #12748 ) ) ;
#19186=FACE_OUTER_BOUND ( 'NONE', #8664, .T. ) ;
#19188=EDGE_CURVE ( 'NONE', #33148, #39021, #41259, .T. ) ;
#19189=DIRECTION ( 'NONE',  ( -0.005961354470445682716, -0.6427876096865404731, 0.7660212471507180654 ) ) ;
#19190=PLANE ( 'NONE',  #43308 ) ;
#19191=CARTESIAN_POINT ( 'NONE',  ( -17.73140113748535285, 0.000000000000000000, 13.85752530597602039 ) ) ;
#19192=CARTESIAN_POINT ( 'NONE',  ( -20.54204810873173415, 0.000000000000000000, 4.860550213503115558 ) ) ;
#19193=CARTESIAN_POINT ( 'NONE',  ( -11.75708623541733289, -0.1941918491731566832, 1.441976946652226976 ) ) ;
#19194=CARTESIAN_POINT ( 'NONE',  ( -10.47421230394850866, 0.000000000000000000, 10.95934586908605723 ) ) ;
#19195=EDGE_LOOP ( 'NONE', ( #8383, #2272, #2555, #44851 ) ) ;
#19196=CARTESIAN_POINT ( 'NONE',  ( -18.12176549260108160, 0.000000000000000000, 4.310047286430262581 ) ) ;
#19197=VERTEX_POINT ( 'NONE', #19104 ) ;
#19198=AXIS2_PLACEMENT_3D ( 'NONE', #27195, #49877, #10732 ) ;
#19199=VECTOR ( 'NONE', #50345, 999.9999999999998863 ) ;
#19200=CARTESIAN_POINT ( 'NONE',  ( -19.60912206198628027, -0.1191753592594197858, 4.398475361799976113 ) ) ;
#19201=CARTESIAN_POINT ( 'NONE',  ( -22.40478740399063895, 0.000000000000000000, 5.384712028983816623 ) ) ;
#19202=CARTESIAN_POINT ( 'NONE',  ( -15.13495153988577968, 0.000000000000000000, 12.76973526769478084 ) ) ;
#19203=DIRECTION ( 'NONE',  ( -0.9999697198139514409, -0.000000000000000000, -0.007781995580013368816 ) ) ;
#19204=CARTESIAN_POINT ( 'NONE',  ( -14.90379585677687224, 0.000000000000000000, 8.767075107899501063 ) ) ;
#19205=LINE ( 'NONE', #39961, #19359 ) ;
#19206=VECTOR ( 'NONE', #25191, 1000.000000000000000 ) ;
#19207=VERTEX_POINT ( 'NONE', #10628 ) ;
#19208=DIRECTION ( 'NONE',  ( 0.007781995580012663651, 0.000000000000000000, -0.9999697198139515519 ) ) ;
#19209=PLANE ( 'NONE',  #26721 ) ;
#19210=CARTESIAN_POINT ( 'NONE',  ( -18.67775241435682432, 0.000000000000000000, 4.136394454059623804 ) ) ;
#19211=EDGE_CURVE ( 'NONE', #41396, #55875, #15156, .T. ) ;
#19213=AXIS2_PLACEMENT_3D ( 'NONE', #37140, #14721, #6479 ) ;
#19214=CARTESIAN_POINT ( 'NONE',  ( -19.22961988024793101, -0.1191753592594177458, 14.39986392600063603 ) ) ;
#19215=EDGE_CURVE ( 'NONE', #21025, #30222, #50330, .T. ) ;
#19216=DIRECTION ( 'NONE',  ( -0.6427681459581293666, -0.7660444431189770143, -0.005002170337467561935 ) ) ;
#19217=DIRECTION ( 'NONE',  ( -0.7660212471507179544, -0.6427876096865405842, -0.005961354470445141482 ) ) ;
#19218=VECTOR ( 'NONE', #10878, 1000.000000000000227 ) ;
#19219=CARTESIAN_POINT ( 'NONE',  ( -27.06708303904391144, 0.000000000000000000, 7.395095371555332697 ) ) ;
#19220=ADVANCED_FACE ( 'NONE', ( #54563 ), #10872, .F. ) ;
#19221=DIRECTION ( 'NONE',  ( 0.8531650599175527594, 0.4028455766673922356, -0.3313982828793700652 ) ) ;
#19222=ORIENTED_EDGE ( 'NONE', *, *, #16613, .T. ) ;
#19223=EDGE_CURVE ( 'NONE', #883, #3308, #2351, .T. ) ;
#19224=ADVANCED_FACE ( 'NONE', ( #32475 ), #11445, .F. ) ;
#19225=EDGE_CURVE ( 'NONE', #34036, #13341, #41538, .T. ) ;
#19226=VERTEX_POINT ( 'NONE', #50617 ) ;
#19227=EDGE_CURVE ( 'NONE', #26641, #49112, #20214, .T. ) ;
#19228=ORIENTED_EDGE ( 'NONE', *, *, #35542, .F. ) ;
#19229=ORIENTED_EDGE ( 'NONE', *, *, #10474, .F. ) ;
#19230=ORIENTED_EDGE ( 'NONE', *, *, #43039, .F. ) ;
#19231=ORIENTED_EDGE ( 'NONE', *, *, #11071, .F. ) ;
#19232=AXIS2_PLACEMENT_3D ( 'NONE', #56170, #51357, #30879 ) ;
#19233=LINE ( 'NONE', #5621, #47767 ) ;
#19234=DIRECTION ( 'NONE',  ( 0.9999697198139515519, 0.000000000000000000, 0.007781995580013368816 ) ) ;
#19235=VECTOR ( 'NONE', #43288, 1000.000000000000114 ) ;
#19236=VECTOR ( 'NONE', #47409, 1000.000000000000227 ) ;
#19237=ORIENTED_EDGE ( 'NONE', *, *, #45793, .T. ) ;
#19238=ORIENTED_EDGE ( 'NONE', *, *, #36471, .T. ) ;
#19239=EDGE_CURVE ( 'NONE', #695, #29014, #50027, .T. ) ;
#19240=ORIENTED_EDGE ( 'NONE', *, *, #39120, .T. ) ;
#19241=EDGE_CURVE ( 'NONE', #27276, #23644, #7180, .T. ) ;
#19242=VECTOR ( 'NONE', #19221, 999.9999999999998863 ) ;
#19243=VECTOR ( 'NONE', #24704, 999.9999999999998863 ) ;
#19244=DIRECTION ( 'NONE',  ( 0.6427681459581294776, -0.7660444431189769032, 0.005002170337467562802 ) ) ;
#19245=EDGE_CURVE ( 'NONE', #26740, #9909, #33314, .T. ) ;
#19246=LINE ( 'NONE', #2746, #35563 ) ;
#19247=CARTESIAN_POINT ( 'NONE',  ( -13.57512723388990850, 4.333955019861511992, 1.816696306515934278 ) ) ;
#19249=DIRECTION ( 'NONE',  ( 0.9999697198139515519, 0.000000000000000000, 0.007781995580013368816 ) ) ;
#19250=ORIENTED_EDGE ( 'NONE', *, *, #45178, .F. ) ;
#19251=ADVANCED_FACE ( 'NONE', ( #54870 ), #6912, .F. ) ;
#19252=CARTESIAN_POINT ( 'NONE',  ( -26.13337879274045505, 0.000000000000000000, 6.833023547870798353 ) ) ;
#19253=PLANE ( 'NONE',  #15735 ) ;
#19254=ADVANCED_FACE ( 'NONE', ( #15983 ), #37262, .F. ) ;
#19255=CARTESIAN_POINT ( 'NONE',  ( -22.40478740399063895, 0.000000000000000000, 5.384712028983816623 ) ) ;
#19256=DIRECTION ( 'NONE',  ( -0.005002170337468016433, -0.7660444431189770143, 0.6427681459581293666 ) ) ;
#19257=DIRECTION ( 'NONE',  ( 0.007781995580012662783, 0.000000000000000000, -0.9999697198139514409 ) ) ;
#19258=LINE ( 'NONE', #24630, #43774 ) ;
#19259=FACE_OUTER_BOUND ( 'NONE', #25047, .T. ) ;
#19260=DIRECTION ( 'NONE',  ( -0.9999697198139514409, -0.000000000000000000, -0.007781995580013368816 ) ) ;
#19262=CARTESIAN_POINT ( 'NONE',  ( -21.76664711697825894, -4.889348428825664783, 5.180230242434543442 ) ) ;
#19263=ORIENTED_EDGE ( 'NONE', *, *, #7547, .T. ) ;
#19264=DIRECTION ( 'NONE',  ( 0.7660212471507180654, -0.6427876096865404731, 0.005961354470445141482 ) ) ;
#19265=FACE_OUTER_BOUND ( 'NONE', #47043, .T. ) ;
#19266=CARTESIAN_POINT ( 'NONE',  ( -11.63277560346829453, 0.000000000000000000, 6.407212511434006608 ) ) ;
#19267=CARTESIAN_POINT ( 'NONE',  ( -22.40478740399063895, 0.000000000000000000, 5.384712028983816623 ) ) ;
#19268=VECTOR ( 'NONE', #49683, 999.9999999999998863 ) ;
#19269=PLANE ( 'NONE',  #49532 ) ;
#19270=LINE ( 'NONE', #49679, #52167 ) ;
#19271=DIRECTION ( 'NONE',  ( -0.5364919789714478471, 0.6444004775717705469, -0.5449076811759709926 ) ) ;
#19272=LINE ( 'NONE', #40862, #2083 ) ;
#19273=CARTESIAN_POINT ( 'NONE',  ( -13.93428531402074633, 0.000000000000000000, 3.603971085826818133 ) ) ;
#19274=VECTOR ( 'NONE', #2329, 1000.000000000000227 ) ;
#19275=CARTESIAN_POINT ( 'NONE',  ( -14.00280974873554030, 0.000000000000000000, 12.40921378708904044 ) ) ;
#19276=LINE ( 'NONE', #6248, #14045 ) ;
#19279=CIRCLE ( 'NONE', #27436, 1.000000000000000222 ) ;
#19281=CARTESIAN_POINT ( 'NONE',  ( -18.81226281495249708, 0.000000000000000000, 7.628662304866128174 ) ) ;
#19282=LINE ( 'NONE', #28095, #18479 ) ;
#19283=DIRECTION ( 'NONE',  ( 0.005961354470445682716, -0.6427876096865404731, -0.7660212471507180654 ) ) ;
#19284=CARTESIAN_POINT ( 'NONE',  ( -17.74404816805336793, 0.000000000000000000, 3.574322630375089460 ) ) ;
#19285=EDGE_LOOP ( 'NONE', ( #16172, #19427, #37388, #25434 ) ) ;
#19286=AXIS2_PLACEMENT_3D ( 'NONE', #48992, #2108, #14630 ) ;
#19287=VECTOR ( 'NONE', #7324, 999.9999999999998863 ) ;
#19288=VERTEX_POINT ( 'NONE', #40964 ) ;
#19289=DIRECTION ( 'NONE',  ( -0.5449076811759708816, 0.6444004775717707689, 0.5364919789714475140 ) ) ;
#19290=DIRECTION ( 'NONE',  ( 0.5449076811759707706, 0.6444004775717708799, -0.5364919789714476250 ) ) ;
#19291=EDGE_CURVE ( 'NONE', #51712, #47765, #2050, .T. ) ;
#19292=ADVANCED_FACE ( 'NONE', ( #44670 ), #14583, .F. ) ;
#19293=ORIENTED_EDGE ( 'NONE', *, *, #44682, .T. ) ;
#19294=PLANE ( 'NONE',  #9542 ) ;
#19295=AXIS2_PLACEMENT_3D ( 'NONE', #19828, #15296, #15021 ) ;
#19296=ORIENTED_EDGE ( 'NONE', *, *, #6060, .T. ) ;
#19297=CARTESIAN_POINT ( 'NONE',  ( -12.80458192191714595, 0.000000000000000000, 11.86454056839041726 ) ) ;
#19298=EDGE_CURVE ( 'NONE', #36530, #50929, #19389, .T. ) ;
#19299=VECTOR ( 'NONE', #22045, 1000.000000000000227 ) ;
#19300=ORIENTED_EDGE ( 'NONE', *, *, #6742, .F. ) ;
#19302=ORIENTED_EDGE ( 'NONE', *, *, #30894, .T. ) ;
#19304=DIRECTION ( 'NONE',  ( 0.007781995580012663651, 0.000000000000000000, -0.9999697198139515519 ) ) ;
#19305=CARTESIAN_POINT ( 'NONE',  ( -13.53223678178913936, 2.067327705546508021, 1.872353476777575798 ) ) ;
#19306=VECTOR ( 'NONE', #25471, 1000.000000000000227 ) ;
#19307=ORIENTED_EDGE ( 'NONE', *, *, #53485, .T. ) ;
#19308=ORIENTED_EDGE ( 'NONE', *, *, #1486, .T. ) ;
#19309=VECTOR ( 'NONE', #46585, 999.9999999999998863 ) ;
#19310=CARTESIAN_POINT ( 'NONE',  ( -20.49857661154221589, 0.1903768112243051092, 4.870464582990948088 ) ) ;
#19311=ORIENTED_EDGE ( 'NONE', *, *, #37806, .F. ) ;
#19312=VECTOR ( 'NONE', #48010, 1000.000000000000000 ) ;
#19314=ORIENTED_EDGE ( 'NONE', *, *, #35156, .F. ) ;
#19315=LINE ( 'NONE', #15345, #25805 ) ;
#19317=AXIS2_PLACEMENT_3D ( 'NONE', #7031, #24332, #17204 ) ;
#19318=VECTOR ( 'NONE', #8964, 999.9999999999998863 ) ;
#19319=ORIENTED_EDGE ( 'NONE', *, *, #4194, .T. ) ;
#19320=CARTESIAN_POINT ( 'NONE',  ( 2.072287782118878319, 0.000000000000000000, -2.950529333540147015 ) ) ;
#19321=EDGE_CURVE ( 'NONE', #50536, #25204, #27652, .T. ) ;
#19322=VECTOR ( 'NONE', #38034, 999.9999999999998863 ) ;
#19323=CARTESIAN_POINT ( 'NONE',  ( -17.27030106973081303, -3.917936722690659401, 9.820304807591645258 ) ) ;
#19324=VECTOR ( 'NONE', #35295, 1000.000000000000227 ) ;
#19325=ORIENTED_EDGE ( 'NONE', *, *, #16683, .F. ) ;
#19326=ADVANCED_FACE ( 'NONE', ( #49516 ), #9790, .F. ) ;
#19327=PLANE ( 'NONE',  #41245 ) ;
#19328=CARTESIAN_POINT ( 'NONE',  ( -16.63391944153825008, 2.391131607591507446, 7.266754650224643619 ) ) ;
#19329=DIRECTION ( 'NONE',  ( 0.007781995580012663651, -3.146120232559066537E-19, -0.9999697198139514409 ) ) ;
#19330=ADVANCED_FACE ( 'NONE', ( #27944 ), #1783, .F. ) ;
#19331=ORIENTED_EDGE ( 'NONE', *, *, #9046, .F. ) ;
#19332=LINE ( 'NONE', #11665, #39193 ) ;
#19333=FACE_OUTER_BOUND ( 'NONE', #4610, .T. ) ;
#19334=EDGE_CURVE ( 'NONE', #44511, #7820, #23397, .T. ) ;
#19335=LINE ( 'NONE', #49457, #5878 ) ;
#19336=DIRECTION ( 'NONE',  ( 0.5449076811759707706, 0.6444004775717708799, -0.5364919789714476250 ) ) ;
#19337=AXIS2_PLACEMENT_3D ( 'NONE', #17223, #9259, #30598 ) ;
#19338=DIRECTION ( 'NONE',  ( -0.005961354470445682716, -0.6427876096865404731, 0.7660212471507180654 ) ) ;
#19339=CARTESIAN_POINT ( 'NONE',  ( -20.54204810873173415, 0.000000000000000000, 4.860550213503115558 ) ) ;
#19341=ORIENTED_EDGE ( 'NONE', *, *, #42694, .T. ) ;
#19342=CARTESIAN_POINT ( 'NONE',  ( -14.53990499995960306, -0.1191753592594190225, 8.866166454900344718 ) ) ;
#19343=CARTESIAN_POINT ( 'NONE',  ( -24.26986129792355129, -0.1191753592594197858, 6.208864760408702388 ) ) ;
#19345=ORIENTED_EDGE ( 'NONE', *, *, #50994, .F. ) ;
#19346=CARTESIAN_POINT ( 'NONE',  ( -30.79567442779373110, 0.000000000000000000, 8.843406890442315316 ) ) ;
#19347=LINE ( 'NONE', #40676, #8205 ) ;
#19348=AXIS2_PLACEMENT_3D ( 'NONE', #2359, #19692, #45247 ) ;
#19349=FACE_OUTER_BOUND ( 'NONE', #20421, .T. ) ;
#19350=VECTOR ( 'NONE', #29005, 999.9999999999998863 ) ;
#19351=LINE ( 'NONE', #18826, #26048 ) ;
#19353=ORIENTED_EDGE ( 'NONE', *, *, #28804, .F. ) ;
#19354=EDGE_LOOP ( 'NONE', ( #9099, #9474, #11951, #32787 ) ) ;
#19355=CARTESIAN_POINT ( 'NONE',  ( -18.78077679739165973, 4.981562823951513508, 3.818085302033760620 ) ) ;
#19356=VECTOR ( 'NONE', #20582, 999.9999999999998863 ) ;
#19358=DIRECTION ( 'NONE',  ( 0.5364919789714477361, 0.6444004775717706579, 0.5449076811759711036 ) ) ;
#19359=VECTOR ( 'NONE', #1046, 999.9999999999998863 ) ;
#19360=EDGE_CURVE ( 'NONE', #28890, #1495, #18860, .T. ) ;
#19361=EDGE_LOOP ( 'NONE', ( #53813, #26114, #35235, #19936 ) ) ;
#19363=EDGE_LOOP ( 'NONE', ( #27387, #3327, #6591, #2740 ) ) ;
#19365=EDGE_CURVE ( 'NONE', #17633, #24207, #23932, .T. ) ;
#19366=ADVANCED_FACE ( 'NONE', ( #41263 ), #6346, .F. ) ;
#19367=VECTOR ( 'NONE', #18920, 1000.000000000000000 ) ;
#19368=ORIENTED_EDGE ( 'NONE', *, *, #17873, .T. ) ;
#19369=AXIS2_PLACEMENT_3D ( 'NONE', #40554, #10445, #40248 ) ;
#19370=VERTEX_POINT ( 'NONE', #31642 ) ;
#19371=CARTESIAN_POINT ( 'NONE',  ( -14.60334660744590174, 0.000000000000000000, 4.168102422163359577 ) ) ;
#19372=DIRECTION ( 'NONE',  ( -0.005961354470445682716, -0.6427876096865404731, 0.7660212471507180654 ) ) ;
#19373=CARTESIAN_POINT ( 'NONE',  ( -12.88979734264706067, -3.756034771668162797, 1.768318970208784924 ) ) ;
#19374=VERTEX_POINT ( 'NONE', #1531 ) ;
#19375=LINE ( 'NONE', #37250, #7508 ) ;
#19376=ORIENTED_EDGE ( 'NONE', *, *, #31549, .T. ) ;
#19377=ADVANCED_FACE ( 'NONE', ( #54046 ), #36730, .F. ) ;
#19378=VERTEX_POINT ( 'NONE', #32479 ) ;
#19379=EDGE_LOOP ( 'NONE', ( #27859, #41110, #24400, #43619, #7884 ) ) ;
#19380=DIRECTION ( 'NONE',  ( 0.6427681459581294776, -0.7660444431189769032, 0.005002170337467562802 ) ) ;
#19381=VECTOR ( 'NONE', #10870, 999.9999999999998863 ) ;
#19382=ORIENTED_EDGE ( 'NONE', *, *, #3078, .F. ) ;
#19383=DIRECTION ( 'NONE',  ( 0.005961354470445682716, -0.6427876096865404731, -0.7660212471507180654 ) ) ;
#19384=EDGE_LOOP ( 'NONE', ( #52690, #43734, #49584, #9435 ) ) ;
#19385=VECTOR ( 'NONE', #44765, 1000.000000000000227 ) ;
#19386=CARTESIAN_POINT ( 'NONE',  ( -10.00813838035478298, 0.000000000000000000, 10.77830692922518452 ) ) ;
#19387=LINE ( 'NONE', #19942, #29512 ) ;
#19388=ORIENTED_EDGE ( 'NONE', *, *, #30289, .F. ) ;
#19389=LINE ( 'NONE', #40712, #20413 ) ;
#19390=VECTOR ( 'NONE', #55094, 1000.000000000000000 ) ;
#19391=VERTEX_POINT ( 'NONE', #32192 ) ;
#19392=FACE_OUTER_BOUND ( 'NONE', #1804, .T. ) ;
#19393=CARTESIAN_POINT ( 'NONE',  ( -24.26908309836554878, 0.000000000000000000, 6.108867788427308376 ) ) ;
#19394=LINE ( 'NONE', #2629, #40461 ) ;
#19395=CARTESIAN_POINT ( 'NONE',  ( -24.26908309836554878, 0.000000000000000000, 6.108867788427308376 ) ) ;
#19396=FACE_OUTER_BOUND ( 'NONE', #27267, .T. ) ;
#19397=VECTOR ( 'NONE', #23382, 1000.000000000000227 ) ;
#19398=LINE ( 'NONE', #30861, #29167 ) ;
#19399=DIRECTION ( 'NONE',  ( 0.5364919789714477361, 0.6444004775717706579, 0.5449076811759711036 ) ) ;
#19400=ORIENTED_EDGE ( 'NONE', *, *, #43951, .T. ) ;
#19401=VERTEX_POINT ( 'NONE', #35909 ) ;
#19402=CARTESIAN_POINT ( 'NONE',  ( -18.39746900504187010, 0.000000000000000000, 14.03700784672088808 ) ) ;
#19404=CARTESIAN_POINT ( 'NONE',  ( -11.30636317915456779, -0.1191753592594197858, 11.32220194836580340 ) ) ;
#19405=LINE ( 'NONE', #39692, #30325 ) ;
#19406=CARTESIAN_POINT ( 'NONE',  ( -13.73672976910459909, 0.000000000000000000, 12.22661844811216270 ) ) ;
#19407=AXIS2_PLACEMENT_3D ( 'NONE', #37369, #15261, #28038 ) ;
#19408=VECTOR ( 'NONE', #4696, 999.9999999999998863 ) ;
#19409=PLANE ( 'NONE',  #49406 ) ;
#19410=ORIENTED_EDGE ( 'NONE', *, *, #33046, .T. ) ;
#19411=PLANE ( 'NONE',  #39499 ) ;
#19412=CARTESIAN_POINT ( 'NONE',  ( 2.072287782118878319, 0.000000000000000000, -2.950529333540147015 ) ) ;
#19414=CARTESIAN_POINT ( 'NONE',  ( -29.86197018149027116, 0.000000000000000000, 8.281335066757780083 ) ) ;
#19416=EDGE_LOOP ( 'NONE', ( #24743, #23012, #17982, #49313 ) ) ;
#19417=EDGE_CURVE ( 'NONE', #14383, #28433, #45498, .T. ) ;
#19418=DIRECTION ( 'NONE',  ( 0.005002170337468016433, -0.7660444431189770143, -0.6427681459581293666 ) ) ;
#19419=CARTESIAN_POINT ( 'NONE',  ( -15.08654547970796500, 0.000000000000000000, 6.549660489236909910 ) ) ;
#19420=CARTESIAN_POINT ( 'NONE',  ( -16.56378919472086864, -4.727446477803161073, 10.87441502184582909 ) ) ;
#19421=EDGE_CURVE ( 'NONE', #12571, #4309, #14028, .T. ) ;
#19422=EDGE_CURVE ( 'NONE', #3167, #2376, #27094, .T. ) ;
#19423=CARTESIAN_POINT ( 'NONE',  ( -21.74939387271512103, 3.524445264749011208, 5.017686667736141359 ) ) ;
#19424=LINE ( 'NONE', #36766, #52787 ) ;
#19426=ORIENTED_EDGE ( 'NONE', *, *, #26045, .T. ) ;
#19427=ORIENTED_EDGE ( 'NONE', *, *, #43307, .T. ) ;
#19428=DIRECTION ( 'NONE',  ( -0.005002170337468016433, -0.7660444431189770143, 0.6427681459581293666 ) ) ;
#19429=LINE ( 'NONE', #41305, #3212 ) ;
#19430=DIRECTION ( 'NONE',  ( 0.8531650599175527594, 0.4028455766673922356, -0.3313982828793700652 ) ) ;
#19431=ADVANCED_FACE ( 'NONE', ( #22819 ), #40137, .F. ) ;
#19432=VECTOR ( 'NONE', #31655, 1000.000000000000227 ) ;
#19433=CARTESIAN_POINT ( 'NONE',  ( -13.31717279592726833, 1.257817950434005683, 1.814642920502075540 ) ) ;
#19435=DIRECTION ( 'NONE',  ( 0.007781995580012663651, -3.146120232559066537E-19, -0.9999697198139514409 ) ) ;
#19436=ORIENTED_EDGE ( 'NONE', *, *, #41783, .F. ) ;
#19438=EDGE_CURVE ( 'NONE', #20292, #3728, #20792, .T. ) ;
#19439=LINE ( 'NONE', #41584, #21431 ) ;
#19440=LINE ( 'NONE', #45549, #19649 ) ;
#19441=ORIENTED_EDGE ( 'NONE', *, *, #32016, .F. ) ;
#19442=VECTOR ( 'NONE', #38303, 1000.000000000000000 ) ;
#19443=ADVANCED_FACE ( 'NONE', ( #8030 ), #19944, .F. ) ;
#19444=CARTESIAN_POINT ( 'NONE',  ( -13.08486533123210194, 0.000000000000000000, 1.963927175729152541 ) ) ;
#19445=VERTEX_POINT ( 'NONE', #37013 ) ;
#19446=CARTESIAN_POINT ( 'NONE',  ( -25.20278734466900517, 0.000000000000000000, 6.670939612111840944 ) ) ;
#19447=CARTESIAN_POINT ( 'NONE',  ( -8.975993561185934055, -0.1191753592594197858, 10.41700724906143982 ) ) ;
#19448=AXIS2_PLACEMENT_3D ( 'NONE', #51489, #51192, #12584 ) ;
#19449=EDGE_CURVE ( 'NONE', #28956, #18999, #33569, .T. ) ;
#19450=VERTEX_POINT ( 'NONE', #19688 ) ;
#19451=DIRECTION ( 'NONE',  ( -0.005002170337468016433, -0.7660444431189770143, 0.6427681459581293666 ) ) ;
#19452=ORIENTED_EDGE ( 'NONE', *, *, #27797, .F. ) ;
#19453=ADVANCED_FACE ( 'NONE', ( #46928 ), #32723, .F. ) ;
#19454=VECTOR ( 'NONE', #11115, 1000.000000000000114 ) ;
#19455=ORIENTED_EDGE ( 'NONE', *, *, #37314, .T. ) ;
#19456=ORIENTED_EDGE ( 'NONE', *, *, #50697, .T. ) ;
#19457=DIRECTION ( 'NONE',  ( 0.005002170337468016433, -0.7660444431189770143, -0.6427681459581293666 ) ) ;
#19458=AXIS2_PLACEMENT_3D ( 'NONE', #12738, #25806, #43132 ) ;
#19459=EDGE_LOOP ( 'NONE', ( #16735, #9743, #15670, #40894 ) ) ;
#19460=ORIENTED_EDGE ( 'NONE', *, *, #48211, .T. ) ;
#19461=LINE ( 'NONE', #36801, #8442 ) ;
#19462=ORIENTED_EDGE ( 'NONE', *, *, #21354, .F. ) ;
#19463=ORIENTED_EDGE ( 'NONE', *, *, #12440, .T. ) ;
#19464=DIRECTION ( 'NONE',  ( 0.5364919789714477361, 0.6444004775717706579, 0.5449076811759711036 ) ) ;
#19465=ORIENTED_EDGE ( 'NONE', *, *, #33874, .T. ) ;
#19466=ORIENTED_EDGE ( 'NONE', *, *, #27649, .F. ) ;
#19467=ORIENTED_EDGE ( 'NONE', *, *, #12255, .F. ) ;
#19468=AXIS2_PLACEMENT_3D ( 'NONE', #18683, #50148, #15503 ) ;
#19469=CARTESIAN_POINT ( 'NONE',  ( -10.37421533196711465, -0.1191753592594197858, 10.96012406864405975 ) ) ;
#19470=VECTOR ( 'NONE', #38961, 999.9999999999998863 ) ;
#19471=CARTESIAN_POINT ( 'NONE',  ( -18.65135909430610539, 0.9340140483890049250, 5.659018568344508893 ) ) ;
#19473=FACE_OUTER_BOUND ( 'NONE', #31409, .T. ) ;
#19474=ORIENTED_EDGE ( 'NONE', *, *, #314, .F. ) ;
#19475=LINE ( 'NONE', #1611, #36492 ) ;
#19476=AXIS2_PLACEMENT_3D ( 'NONE', #35016, #43504, #20805 ) ;
#19477=EDGE_LOOP ( 'NONE', ( #23387, #30662, #49194, #21632 ) ) ;
#19478=ORIENTED_EDGE ( 'NONE', *, *, #50317, .T. ) ;
#19479=ADVANCED_FACE ( 'NONE', ( #37266 ), #45791, .F. ) ;
#19481=VECTOR ( 'NONE', #23867, 999.9999999999998863 ) ;
#19483=VECTOR ( 'NONE', #33011, 1000.000000000000114 ) ;
#19484=VECTOR ( 'NONE', #41559, 999.9999999999998863 ) ;
#19485=CARTESIAN_POINT ( 'NONE',  ( -13.26502572267249391, -3.594132820645661308, 7.733102475169945755 ) ) ;
#19486=DIRECTION ( 'NONE',  ( -0.6427681459581293666, -0.7660444431189770143, -0.005002170337467561935 ) ) ;
#19487=VECTOR ( 'NONE', #47900, 1000.000000000000227 ) ;
#19488=LINE ( 'NONE', #41882, #35874 ) ;
#19489=VERTEX_POINT ( 'NONE', #16522 ) ;
#19490=CARTESIAN_POINT ( 'NONE',  ( -15.40103151951671734, 0.000000000000000000, 12.95233060667165681 ) ) ;
#19491=EDGE_LOOP ( 'NONE', ( #36657, #54653, #17114, #15146 ) ) ;
#19492=VECTOR ( 'NONE', #13141, 1000.000000000000227 ) ;
#19493=DIRECTION ( 'NONE',  ( -0.5449076811759708816, 0.6444004775717707689, 0.5364919789714475140 ) ) ;
#19494=LINE ( 'NONE', #36839, #6934 ) ;
#19495=LINE ( 'NONE', #54152, #8171 ) ;
#19497=ADVANCED_FACE ( 'NONE', ( #46077 ), #46629, .F. ) ;
#19498=LINE ( 'NONE', #32569, #2344 ) ;
#19499=AXIS2_PLACEMENT_3D ( 'NONE', #1762, #36699, #28439 ) ;
#19500=AXIS2_PLACEMENT_3D ( 'NONE', #9217, #13216, #26532 ) ;
#19501=EDGE_LOOP ( 'NONE', ( #17954, #41601, #35982, #6984 ) ) ;
#19502=DIRECTION ( 'NONE',  ( 0.9999697198139515519, 0.000000000000000000, 0.007781995580013368816 ) ) ;
#19503=DIRECTION ( 'NONE',  ( 0.9999697198139515519, 0.000000000000000000, 0.007781995580013368816 ) ) ;
#19504=LINE ( 'NONE', #19210, #9776 ) ;
#19505=FACE_OUTER_BOUND ( 'NONE', #6429, .T. ) ;
#19506=ADVANCED_FACE ( 'NONE', ( #50877 ), #29623, .F. ) ;
#19507=LINE ( 'NONE', #24330, #41180 ) ;
#19508=CARTESIAN_POINT ( 'NONE',  ( -19.53160284976675598, 0.000000000000000000, 6.345742011377845770 ) ) ;
#19509=CARTESIAN_POINT ( 'NONE',  ( -16.94509306707230678, 0.000000000000000000, 6.535196842164872955 ) ) ;
#19510=ADVANCED_FACE ( 'NONE', ( #42644 ), #25342, .F. ) ;
#19511=VECTOR ( 'NONE', #45283, 1000.000000000000000 ) ;
#19512=CARTESIAN_POINT ( 'NONE',  ( -21.36215635309214989, 4.172053068839010947, 4.846608384923496438 ) ) ;
#19513=VECTOR ( 'NONE', #28615, 1000.000000000000227 ) ;
#19514=DIRECTION ( 'NONE',  ( 0.9999697198139515519, 0.000000000000000000, 0.007781995580013368816 ) ) ;
#19515=VECTOR ( 'NONE', #23806, 1000.000000000000227 ) ;
#19516=ADVANCED_FACE ( 'NONE', ( #7183 ), #2890, .F. ) ;
#19517=ORIENTED_EDGE ( 'NONE', *, *, #22087, .F. ) ;
#19518=VECTOR ( 'NONE', #32605, 1000.000000000000227 ) ;
#19519=EDGE_CURVE ( 'NONE', #22811, #19054, #37854, .T. ) ;
#19520=ORIENTED_EDGE ( 'NONE', *, *, #1067, .F. ) ;
#19521=ORIENTED_EDGE ( 'NONE', *, *, #50258, .T. ) ;
#19522=VECTOR ( 'NONE', #54875, 999.9999999999998863 ) ;
#19523=VECTOR ( 'NONE', #15820, 999.9999999999998863 ) ;
#19524=EDGE_LOOP ( 'NONE', ( #38049, #49960, #32034, #51627 ) ) ;
#19525=VECTOR ( 'NONE', #28997, 999.9999999999998863 ) ;
#19526=EDGE_LOOP ( 'NONE', ( #21972, #51590, #19714, #15061 ) ) ;
#19527=LINE ( 'NONE', #49349, #26939 ) ;
#19528=DIRECTION ( 'NONE',  ( 0.9999697198139515519, 0.000000000000000000, 0.007781995580013368816 ) ) ;
#19529=VECTOR ( 'NONE', #54677, 999.9999999999998863 ) ;
#19530=VECTOR ( 'NONE', #32471, 1000.000000000000114 ) ;
#19532=LINE ( 'NONE', #12433, #47612 ) ;
#19533=EDGE_LOOP ( 'NONE', ( #860, #35595, #48396, #42291 ) ) ;
#19534=ORIENTED_EDGE ( 'NONE', *, *, #35962, .F. ) ;
#19535=AXIS2_PLACEMENT_3D ( 'NONE', #19992, #49828, #2671 ) ;
#19536=AXIS2_PLACEMENT_3D ( 'NONE', #22225, #30178, #16546 ) ;
#19538=PLANE ( 'NONE',  #29189 ) ;
#19539=CARTESIAN_POINT ( 'NONE',  ( -20.40437129806706196, -3.270328918600661439, 4.702731250161795273 ) ) ;
#19540=ORIENTED_EDGE ( 'NONE', *, *, #19048, .F. ) ;
#19541=DIRECTION ( 'NONE',  ( -0.9999697198139514409, -0.000000000000000000, -0.007781995580013368816 ) ) ;
#19542=EDGE_CURVE ( 'NONE', #34361, #30915, #11977, .T. ) ;
#19543=LINE ( 'NONE', #54190, #31859 ) ;
#19545=PLANE ( 'NONE',  #46580 ) ;
#19546=VECTOR ( 'NONE', #1425, 1000.000000000000000 ) ;
#19547=DIRECTION ( 'NONE',  ( -0.005961354470445682716, -0.6427876096865404731, 0.7660212471507180654 ) ) ;
#19548=CARTESIAN_POINT ( 'NONE',  ( -12.22842013625588820, -0.03739765774599676518, 1.569878849409872545 ) ) ;
#19549=EDGE_CURVE ( 'NONE', #52700, #45157, #24481, .T. ) ;
#19550=CARTESIAN_POINT ( 'NONE',  ( -10.43885885690782800, 0.000000000000000000, 6.416503847622031742 ) ) ;
#19551=DIRECTION ( 'NONE',  ( 0.6427681459581294776, -0.7660444431189769032, 0.005002170337467562802 ) ) ;
#19552=LINE ( 'NONE', #24364, #27609 ) ;
#19553=VECTOR ( 'NONE', #42616, 1000.000000000000114 ) ;
#19554=EDGE_CURVE ( 'NONE', #29102, #38297, #41795, .T. ) ;
#19555=PLANE ( 'NONE',  #39274 ) ;
#19556=ORIENTED_EDGE ( 'NONE', *, *, #17277, .T. ) ;
#19557=PLANE ( 'NONE',  #22940 ) ;
#19558=VERTEX_POINT ( 'NONE', #21063 ) ;
#19559=VECTOR ( 'NONE', #28498, 1000.000000000000227 ) ;
#19560=EDGE_CURVE ( 'NONE', #29459, #19401, #21653, .T. ) ;
#19562=ADVANCED_FACE ( 'NONE', ( #12569 ), #26441, .F. ) ;
#19563=CARTESIAN_POINT ( 'NONE',  ( -31.72704407542318350, -0.1191753592594197858, 9.105487798182664960 ) ) ;
#19564=LINE ( 'NONE', #37156, #55898 ) ;
#19565=PLANE ( 'NONE',  #22242 ) ;
#19566=PLANE ( 'NONE',  #22346 ) ;
#19567=AXIS2_PLACEMENT_3D ( 'NONE', #2299, #37213, #11668 ) ;
#19568=DIRECTION ( 'NONE',  ( 0.6246952433987894571, -0.7422098413412800966, -0.2426528472758541777 ) ) ;
#19569=CARTESIAN_POINT ( 'NONE',  ( -12.33850799832341849, 0.000000000000000000, 11.68350162852954632 ) ) ;
#19570=CARTESIAN_POINT ( 'NONE',  ( -10.74029228357944987, 0.000000000000000000, 11.14194120806293320 ) ) ;
#19571=VECTOR ( 'NONE', #55166, 1000.000000000000114 ) ;
#19573=PLANE ( 'NONE',  #43749 ) ;
#19574=CARTESIAN_POINT ( 'NONE',  ( -22.40478740399063895, 0.000000000000000000, 5.384712028983816623 ) ) ;
#19575=CARTESIAN_POINT ( 'NONE',  ( -14.66887761629205222, 0.000000000000000000, 12.58869632783390990 ) ) ;
#19576=CARTESIAN_POINT ( 'NONE',  ( -25.20123094555300369, 0.000000000000000000, 6.470945668149052032 ) ) ;
#19577=DIRECTION ( 'NONE',  ( -0.9999697198139514409, -0.000000000000000000, -0.007781995580013368816 ) ) ;
#19578=AXIS2_PLACEMENT_3D ( 'NONE', #50712, #25177, #46738 ) ;
#19579=VECTOR ( 'NONE', #11292, 999.9999999999998863 ) ;
#19580=FACE_OUTER_BOUND ( 'NONE', #50022, .T. ) ;
#19581=EDGE_CURVE ( 'NONE', #31672, #49287, #52314, .T. ) ;
#19582=VECTOR ( 'NONE', #47943, 999.9999999999998863 ) ;
#19583=LINE ( 'NONE', #24654, #49338 ) ;
#19584=PLANE ( 'NONE',  #52217 ) ;
#19585=CARTESIAN_POINT ( 'NONE',  ( -20.10223246962251764, 1.178764073316398875, 5.890828872904841695 ) ) ;
#19586=EDGE_LOOP ( 'NONE', ( #18182, #15063, #18342, #20060 ) ) ;
#19587=VECTOR ( 'NONE', #451, 1000.000000000000114 ) ;
#19588=EDGE_CURVE ( 'NONE', #49949, #19711, #51723, .T. ) ;
#19589=VECTOR ( 'NONE', #43937, 1000.000000000000114 ) ;
#19590=CARTESIAN_POINT ( 'NONE',  ( -22.40478740399063895, 0.000000000000000000, 5.384712028983816623 ) ) ;
#19591=EDGE_LOOP ( 'NONE', ( #16239, #23943, #2113, #43606 ) ) ;
#19592=ADVANCED_FACE ( 'NONE', ( #43760 ), #34419, .F. ) ;
#19593=DIRECTION ( 'NONE',  ( -0.005961354470445682716, -0.6427876096865404731, 0.7660212471507180654 ) ) ;
#19594=CARTESIAN_POINT ( 'NONE',  ( -9.859076521000934790, -0.1191753592594181482, 4.474352470677822602 ) ) ;
#19595=EDGE_CURVE ( 'NONE', #31964, #26839, #38391, .T. ) ;
#19596=ORIENTED_EDGE ( 'NONE', *, *, #54835, .T. ) ;
#19597=DIRECTION ( 'NONE',  ( -0.5364919789714478471, 0.6444004775717705469, -0.5449076811759709926 ) ) ;
#19598=ORIENTED_EDGE ( 'NONE', *, *, #28868, .T. ) ;
#19599=FACE_OUTER_BOUND ( 'NONE', #17509, .T. ) ;
#19600=VECTOR ( 'NONE', #55469, 1000.000000000000227 ) ;
#19601=VERTEX_POINT ( 'NONE', #16827 ) ;
#19602=ORIENTED_EDGE ( 'NONE', *, *, #21587, .T. ) ;
#19604=LINE ( 'NONE', #10804, #54701 ) ;
#19605=CARTESIAN_POINT ( 'NONE',  ( -16.31417959753190416, 4.819660872929012463, 2.865140703502121688 ) ) ;
#19606=VECTOR ( 'NONE', #4363, 999.9999999999998863 ) ;
#19607=CARTESIAN_POINT ( 'NONE',  ( -17.49802427868480947, 2.481410104826615282, 12.59520711516599256 ) ) ;
#19608=ORIENTED_EDGE ( 'NONE', *, *, #48918, .F. ) ;
#19609=AXIS2_PLACEMENT_3D ( 'NONE', #45140, #24374, #54457 ) ;
#19610=ORIENTED_EDGE ( 'NONE', *, *, #49518, .F. ) ;
#19611=AXIS2_PLACEMENT_3D ( 'NONE', #36070, #40602, #36601 ) ;
#19612=VECTOR ( 'NONE', #18208, 1000.000000000000227 ) ;
#19613=LINE ( 'NONE', #19310, #39079 ) ;
#19614=ORIENTED_EDGE ( 'NONE', *, *, #12019, .T. ) ;
#19615=DIRECTION ( 'NONE',  ( -0.7660212471507179544, -0.6427876096865405842, -0.005961354470445141482 ) ) ;
#19616=ORIENTED_EDGE ( 'NONE', *, *, #51653, .T. ) ;
#19617=FACE_OUTER_BOUND ( 'NONE', #4335, .T. ) ;
#19618=LINE ( 'NONE', #45184, #41238 ) ;
#19619=AXIS2_PLACEMENT_3D ( 'NONE', #14943, #49298, #18933 ) ;
#19620=ORIENTED_EDGE ( 'NONE', *, *, #51028, .T. ) ;
#19622=PLANE ( 'NONE',  #45828 ) ;
#19623=CARTESIAN_POINT ( 'NONE',  ( -12.15271748404464880, 0.000000000000000000, 1.601849296007406664 ) ) ;
#19624=AXIS2_PLACEMENT_3D ( 'NONE', #24802, #11180, #42122 ) ;
#19625=EDGE_LOOP ( 'NONE', ( #40332, #24066, #48606, #6371 ) ) ;
#19627=CARTESIAN_POINT ( 'NONE',  ( -19.80206979258221622, -3.108426967578159950, 4.473942411073648984 ) ) ;
#19628=DIRECTION ( 'NONE',  ( 0.6427681459581294776, -0.7660444431189769032, 0.005002170337467562802 ) ) ;
#19629=ORIENTED_EDGE ( 'NONE', *, *, #27866, .T. ) ;
#19630=EDGE_CURVE ( 'NONE', #18585, #13470, #52009, .T. ) ;
#19631=ADVANCED_FACE ( 'NONE', ( #30734 ), #52570, .F. ) ;
#19632=DIRECTION ( 'NONE',  ( 0.9999697198139515519, 0.000000000000000000, 0.007781995580013368816 ) ) ;
#19633=PLANE ( 'NONE',  #17868 ) ;
#19634=PLANE ( 'NONE',  #420 ) ;
#19635=DIRECTION ( 'NONE',  ( 0.005961354470445682716, -0.6427876096865404731, -0.7660212471507180654 ) ) ;
#19636=EDGE_CURVE ( 'NONE', #33095, #39543, #625, .T. ) ;
#19638=LINE ( 'NONE', #37215, #44234 ) ;
#19639=VECTOR ( 'NONE', #29837, 999.9999999999998863 ) ;
#19641=ORIENTED_EDGE ( 'NONE', *, *, #20055, .F. ) ;
#19642=LINE ( 'NONE', #7394, #55233 ) ;
#19643=CARTESIAN_POINT ( 'NONE',  ( -9.542064456761055524, 0.000000000000000000, 10.59726798936431180 ) ) ;
#19646=LINE ( 'NONE', #37506, #35685 ) ;
#19647=LINE ( 'NONE', #32686, #21820 ) ;
#19648=VECTOR ( 'NONE', #22226, 1000.000000000000227 ) ;
#19649=VECTOR ( 'NONE', #6668, 1000.000000000000227 ) ;
#19651=CARTESIAN_POINT ( 'NONE',  ( -14.59604210131933577, 0.000000000000000000, 3.229489071685041068 ) ) ;
#19652=EDGE_CURVE ( 'NONE', #49950, #33592, #3740, .T. ) ;
#19653=DIRECTION ( 'NONE',  ( 0.007781995580012663651, -3.146120232559066537E-19, -0.9999697198139514409 ) ) ;
#19654=ORIENTED_EDGE ( 'NONE', *, *, #21246, .F. ) ;
#19655=VECTOR ( 'NONE', #15849, 999.9999999999998863 ) ;
#19656=ORIENTED_EDGE ( 'NONE', *, *, #7075, .T. ) ;
#19657=EDGE_CURVE ( 'NONE', #15538, #26566, #13664, .T. ) ;
#19658=DIRECTION ( 'NONE',  ( 0.000000000000000000, -0.000000000000000000, -1.000000000000000000 ) ) ;
#19659=LINE ( 'NONE', #14553, #39307 ) ;
#19660=EDGE_CURVE ( 'NONE', #36681, #25334, #48297, .T. ) ;
#19661=VECTOR ( 'NONE', #50754, 1000.000000000000000 ) ;
#19662=ORIENTED_EDGE ( 'NONE', *, *, #44341, .F. ) ;
#19663=CARTESIAN_POINT ( 'NONE',  ( -17.46532115785441519, 0.000000000000000000, 13.67492996699914265 ) ) ;
#19664=ORIENTED_EDGE ( 'NONE', *, *, #36764, .F. ) ;
#19665=FACE_OUTER_BOUND ( 'NONE', #16650, .T. ) ;
#19666=EDGE_CURVE ( 'NONE', #46158, #48080, #56015, .T. ) ;
#19667=VECTOR ( 'NONE', #21825, 1000.000000000000114 ) ;
#19668=VECTOR ( 'NONE', #8252, 1000.000000000000227 ) ;
#19669=VERTEX_POINT ( 'NONE', #4592 ) ;
#19670=ORIENTED_EDGE ( 'NONE', *, *, #23312, .F. ) ;
#19671=CARTESIAN_POINT ( 'NONE',  ( -20.81378277464309434, 4.010151117816509903, 11.54744235706348654 ) ) ;
#19672=DIRECTION ( 'NONE',  ( 0.9999697198139515519, 0.000000000000000000, 0.007781995580013368816 ) ) ;
#19673=CARTESIAN_POINT ( 'NONE',  ( -17.74404816805336793, 0.000000000000000000, 3.574322630375089460 ) ) ;
#19674=VERTEX_POINT ( 'NONE', #34161 ) ;
#19675=DIRECTION ( 'NONE',  ( -0.5364919789714478471, 0.6444004775717705469, -0.5449076811759709926 ) ) ;
#19677=VECTOR ( 'NONE', #29620, 1000.000000000000227 ) ;
#19678=ORIENTED_EDGE ( 'NONE', *, *, #41735, .T. ) ;
#19679=EDGE_LOOP ( 'NONE', ( #15493, #14109, #31556, #21822 ) ) ;
#19680=DIRECTION ( 'NONE',  ( -0.5364919789714478471, 0.6444004775717705469, -0.5449076811759709926 ) ) ;
#19681=ORIENTED_EDGE ( 'NONE', *, *, #42598, .T. ) ;
#19682=PLANE ( 'NONE',  #21209 ) ;
#19683=ORIENTED_EDGE ( 'NONE', *, *, #10970, .T. ) ;
#19684=DIRECTION ( 'NONE',  ( 0.8531650599175529814, -0.4028455766673920135, -0.3313982828793697877 ) ) ;
#19686=VERTEX_POINT ( 'NONE', #8290 ) ;
#19687=AXIS2_PLACEMENT_3D ( 'NONE', #18841, #48927, #40413 ) ;
#19688=CARTESIAN_POINT ( 'NONE',  ( -13.02381224048627040, 0.000000000000000000, 6.027055072872212982 ) ) ;
#19689=ORIENTED_EDGE ( 'NONE', *, *, #22681, .F. ) ;
#19690=VECTOR ( 'NONE', #20254, 1000.000000000000000 ) ;
#19691=DIRECTION ( 'NONE',  ( 0.005002170337468016433, -0.7660444431189770143, -0.6427681459581293666 ) ) ;
#19692=DIRECTION ( 'NONE',  ( 0.005961354470445682716, -0.6427876096865404731, -0.7660212471507180654 ) ) ;
#19693=CARTESIAN_POINT ( 'NONE',  ( -21.41819867739107153, 4.172053068839010059, 12.04792670369172036 ) ) ;
#19694=CARTESIAN_POINT ( 'NONE',  ( -14.20280369269832832, 0.000000000000000000, 12.40765738797303719 ) ) ;
#19695=FACE_OUTER_BOUND ( 'NONE', #29558, .T. ) ;
#19696=LINE ( 'NONE', #15172, #16538 ) ;
#19697=ORIENTED_EDGE ( 'NONE', *, *, #23519, .F. ) ;
#19698=EDGE_CURVE ( 'NONE', #485, #55742, #51472, .T. ) ;
#19699=ORIENTED_EDGE ( 'NONE', *, *, #22697, .F. ) ;
#19700=AXIS2_PLACEMENT_3D ( 'NONE', #3290, #52098, #42470 ) ;
#19701=DIRECTION ( 'NONE',  ( 0.007781995580012662783, 0.000000000000000000, -0.9999697198139514409 ) ) ;
#19702=LINE ( 'NONE', #36744, #6715 ) ;
#19703=EDGE_CURVE ( 'NONE', #48176, #38162, #43245, .T. ) ;
#19704=ADVANCED_FACE ( 'NONE', ( #17106 ), #4339, .F. ) ;
#19705=CARTESIAN_POINT ( 'NONE',  ( -14.94916102560700821, 0.000000000000000000, 2.688082935172642962 ) ) ;
#19706=CARTESIAN_POINT ( 'NONE',  ( -10.88050332570665546, 0.000000000000000000, 3.458410309791905224 ) ) ;
#19708=ORIENTED_EDGE ( 'NONE', *, *, #30663, .F. ) ;
#19709=DIRECTION ( 'NONE',  ( 0.007781995580012662783, 0.000000000000000000, -0.9999697198139514409 ) ) ;
#19710=LINE ( 'NONE', #14601, #55891 ) ;
#19711=VERTEX_POINT ( 'NONE', #36369 ) ;
#19712=DIRECTION ( 'NONE',  ( -0.005002170337468016433, -0.7660444431189770143, 0.6427681459581293666 ) ) ;
#19713=LINE ( 'NONE', #54338, #29544 ) ;
#19714=ORIENTED_EDGE ( 'NONE', *, *, #24405, .T. ) ;
#19715=FACE_OUTER_BOUND ( 'NONE', #48189, .T. ) ;
#19717=CARTESIAN_POINT ( 'NONE',  ( -18.13558483980604308, 2.553033558614008047, 3.644953633207256072 ) ) ;
#19718=CARTESIAN_POINT ( 'NONE',  ( -21.47419595591918906, 0.000000000000000000, 5.222628093224860102 ) ) ;
#19720=ORIENTED_EDGE ( 'NONE', *, *, #14649, .T. ) ;
#19721=EDGE_LOOP ( 'NONE', ( #25487, #1519, #51273, #162 ) ) ;
#19722=CARTESIAN_POINT ( 'NONE',  ( -11.14802033209023158, 0.000000000000000000, 3.825660500397664254 ) ) ;
#19723=CARTESIAN_POINT ( 'NONE',  ( -14.59029399430876950, 0.000000000000000000, 2.490869665169511915 ) ) ;
#19724=LINE ( 'NONE', #41834, #40579 ) ;
#19725=CARTESIAN_POINT ( 'NONE',  ( -16.40688773272033885, -0.1159828484229834950, 9.591365951305096615 ) ) ;
#19726=CARTESIAN_POINT ( 'NONE',  ( -16.01007116637957495, 0.000000000000000000, 5.803809259185364056 ) ) ;
#19727=DIRECTION ( 'NONE',  ( -0.5364919789714478471, 0.6444004775717705469, -0.5449076811759709926 ) ) ;
#19728=EDGE_LOOP ( 'NONE', ( #37380, #35376, #37066, #41573 ) ) ;
#19729=CARTESIAN_POINT ( 'NONE',  ( -12.80458192191714595, 0.000000000000000000, 11.86454056839041726 ) ) ;
#19730=EDGE_CURVE ( 'NONE', #14403, #29996, #5439, .T. ) ;
#19731=CARTESIAN_POINT ( 'NONE',  ( -14.39604815735654597, 0.000000000000000000, 3.231045470801043429 ) ) ;
#19732=AXIS2_PLACEMENT_3D ( 'NONE', #21747, #39062, #5539 ) ;
#19733=CARTESIAN_POINT ( 'NONE',  ( -12.60458797795435615, 0.000000000000000000, 11.86609696750642229 ) ) ;
#19734=EDGE_LOOP ( 'NONE', ( #15675, #7040, #27848, #10354 ) ) ;
#19735=EDGE_CURVE ( 'NONE', #35539, #34834, #10253, .T. ) ;
#19736=FACE_OUTER_BOUND ( 'NONE', #42310, .T. ) ;
#19737=DIRECTION ( 'NONE',  ( -0.005961354470445682716, -0.6427876096865404731, 0.7660212471507180654 ) ) ;
#19739=DIRECTION ( 'NONE',  ( -0.5364919789714478471, 0.6444004775717705469, -0.5449076811759709926 ) ) ;
#19740=VERTEX_POINT ( 'NONE', #31831 ) ;
#19741=AXIS2_PLACEMENT_3D ( 'NONE', #38065, #55115, #42600 ) ;
#19742=LINE ( 'NONE', #23992, #12326 ) ;
#19743=EDGE_CURVE ( 'NONE', #14535, #18621, #36661, .T. ) ;
#19744=EDGE_LOOP ( 'NONE', ( #42095, #20573, #48976, #51803 ) ) ;
#19745=EDGE_LOOP ( 'NONE', ( #40889, #35179, #7787, #39645 ) ) ;
#19746=ORIENTED_EDGE ( 'NONE', *, *, #31356, .T. ) ;
#19747=ORIENTED_EDGE ( 'NONE', *, *, #38868, .F. ) ;
#19748=ORIENTED_EDGE ( 'NONE', *, *, #26064, .T. ) ;
#19749=FACE_OUTER_BOUND ( 'NONE', #21846, .T. ) ;
#19750=ORIENTED_EDGE ( 'NONE', *, *, #44421, .F. ) ;
#19751=VERTEX_POINT ( 'NONE', #35830 ) ;
#19752=CARTESIAN_POINT ( 'NONE',  ( -25.20123094555300369, 0.000000000000000000, 6.470945668149052032 ) ) ;
#19753=ORIENTED_EDGE ( 'NONE', *, *, #18986, .F. ) ;
#19754=ORIENTED_EDGE ( 'NONE', *, *, #18726, .T. ) ;
#19755=EDGE_CURVE ( 'NONE', #20189, #30522, #44060, .T. ) ;
#19756=EDGE_LOOP ( 'NONE', ( #45414, #5442, #39823, #20653 ) ) ;
#19757=CARTESIAN_POINT ( 'NONE',  ( -23.33693525117809386, 0.000000000000000000, 5.746789908705562944 ) ) ;
#19758=DIRECTION ( 'NONE',  ( 0.005002170337468016433, -0.7660444431189770143, -0.6427681459581293666 ) ) ;
#19760=FACE_OUTER_BOUND ( 'NONE', #23100, .T. ) ;
#19761=EDGE_CURVE ( 'NONE', #34418, #25320, #5715, .T. ) ;
#19762=VERTEX_POINT ( 'NONE', #23587 ) ;
#19763=CARTESIAN_POINT ( 'NONE',  ( -16.76964795026778532, 0.000000000000000000, 9.691224811305781728 ) ) ;
#19764=ORIENTED_EDGE ( 'NONE', *, *, #18938, .T. ) ;
#19765=EDGE_LOOP ( 'NONE', ( #40586, #48157, #21548, #4588 ) ) ;
#19767=LINE ( 'NONE', #37090, #11349 ) ;
#19768=DIRECTION ( 'NONE',  ( 0.007781995580012663651, -3.146120232559066537E-19, -0.9999697198139514409 ) ) ;
#19769=ADVANCED_FACE ( 'NONE', ( #5179 ), #48884, .F. ) ;
#19770=EDGE_CURVE ( 'NONE', #8057, #7579, #10562, .T. ) ;
#19771=LINE ( 'NONE', #41059, #15175 ) ;
#19772=DIRECTION ( 'NONE',  ( 0.000000000000000000, -1.000000000000000000, 0.000000000000000000 ) ) ;
#19774=LINE ( 'NONE', #23482, #43123 ) ;
#19775=ORIENTED_EDGE ( 'NONE', *, *, #10615, .T. ) ;
#19776=FACE_OUTER_BOUND ( 'NONE', #9194, .T. ) ;
#19777=ORIENTED_EDGE ( 'NONE', *, *, #30639, .F. ) ;
#19779=CARTESIAN_POINT ( 'NONE',  ( -8.949704955220703084, -0.1159828484229828427, 6.694742913531133155 ) ) ;
#19780=LINE ( 'NONE', #23489, #44142 ) ;
#19782=CARTESIAN_POINT ( 'NONE',  ( -30.79567442779373110, 0.000000000000000000, 8.843406890442315316 ) ) ;
#19783=DIRECTION ( 'NONE',  ( 0.007781995580012663651, 0.000000000000000000, -0.9999697198139515519 ) ) ;
#19784=LINE ( 'NONE', #49620, #26851 ) ;
#19785=EDGE_CURVE ( 'NONE', #33865, #51703, #36117, .T. ) ;
#19786=ORIENTED_EDGE ( 'NONE', *, *, #32921, .T. ) ;
#19787=CARTESIAN_POINT ( 'NONE',  ( -29.86352658060627618, 0.000000000000000000, 8.481329010720569883 ) ) ;
#19788=DIRECTION ( 'NONE',  ( 0.007781995580012663651, -3.146120232559066537E-19, -0.9999697198139514409 ) ) ;
#19789=DIRECTION ( 'NONE',  ( -0.7660212471507179544, -0.6427876096865405842, -0.005961354470445141482 ) ) ;
#19790=DIRECTION ( 'NONE',  ( 0.007781995580012663651, -3.146120232559066537E-19, -0.9999697198139514409 ) ) ;
#19791=CARTESIAN_POINT ( 'NONE',  ( -20.06177075545399191, 0.000000000000000000, 14.76272000528038220 ) ) ;
#19792=PLANE ( 'NONE',  #20006 ) ;
#19793=DIRECTION ( 'NONE',  ( -0.5449076811759708816, 0.6444004775717707689, 0.5364919789714475140 ) ) ;
#19794=LINE ( 'NONE', #36860, #43217 ) ;
#19795=CARTESIAN_POINT ( 'NONE',  ( -19.93268291358662481, 3.524445264749008100, 10.40806719690053050 ) ) ;
#19796=ORIENTED_EDGE ( 'NONE', *, *, #40614, .T. ) ;
#19797=EDGE_LOOP ( 'NONE', ( #23323, #8501, #49517, #27484 ) ) ;
#19798=EDGE_CURVE ( 'NONE', #28974, #55568, #18202, .T. ) ;
#19799=ORIENTED_EDGE ( 'NONE', *, *, #56074, .T. ) ;
#19800=ORIENTED_EDGE ( 'NONE', *, *, #471, .T. ) ;
#19801=EDGE_CURVE ( 'NONE', #54647, #52427, #49442, .T. ) ;
#19802=EDGE_LOOP ( 'NONE', ( #34725, #4019, #25454, #24657 ) ) ;
#19803=ORIENTED_EDGE ( 'NONE', *, *, #48286, .F. ) ;
#19804=FACE_OUTER_BOUND ( 'NONE', #12568, .T. ) ;
#19805=CARTESIAN_POINT ( 'NONE',  ( -16.50085385711260599, 0.6102101463440035012, 3.071954842479957204 ) ) ;
#19806=CARTESIAN_POINT ( 'NONE',  ( -14.46888367232926420, 0.000000000000000000, 12.59025272694991315 ) ) ;
#19807=EDGE_CURVE ( 'NONE', #23468, #35736, #1985, .T. ) ;
#19809=EDGE_LOOP ( 'NONE', ( #5411, #38326, #3458, #52462 ) ) ;
#19810=CARTESIAN_POINT ( 'NONE',  ( -10.23024275242918968, 0.000000000000000000, 5.310131136964741039 ) ) ;
#19811=VERTEX_POINT ( 'NONE', #53421 ) ;
#19812=ADVANCED_FACE ( 'NONE', ( #14262 ), #6019, .F. ) ;
#19813=EDGE_LOOP ( 'NONE', ( #54045, #12446, #21694, #5112 ) ) ;
#19814=EDGE_CURVE ( 'NONE', #41874, #21510, #23334, .T. ) ;
#19816=LINE ( 'NONE', #7303, #9253 ) ;
#19817=PLANE ( 'NONE',  #3285 ) ;
#19818=EDGE_CURVE ( 'NONE', #42377, #5037, #15093, .T. ) ;
#19820=PLANE ( 'NONE',  #19213 ) ;
#19821=CARTESIAN_POINT ( 'NONE',  ( -11.81109477377810180, 0.000000000000000000, 3.620494245550860857 ) ) ;
#19822=ADVANCED_FACE ( 'NONE', ( #39805 ), #35529, .F. ) ;
#19823=CARTESIAN_POINT ( 'NONE',  ( -20.13191613428482185, -2.946525016555661125, 4.607231451707245462 ) ) ;
#19824=ADVANCED_FACE ( 'NONE', ( #48605 ), #11371, .F. ) ;
#19825=DIRECTION ( 'NONE',  ( 0.005002170337468016433, -0.7660444431189770143, -0.6427681459581293666 ) ) ;
#19826=LINE ( 'NONE', #28334, #20600 ) ;
#19827=LINE ( 'NONE', #53901, #15910 ) ;
#19828=CARTESIAN_POINT ( 'NONE',  ( -11.40636015113596180, 0.000000000000000000, 11.32142374880780089 ) ) ;
#19829=LINE ( 'NONE', #23533, #49332 ) ;
#19830=LINE ( 'NONE', #50761, #36558 ) ;
#19831=ORIENTED_EDGE ( 'NONE', *, *, #17496, .F. ) ;
#19833=ORIENTED_EDGE ( 'NONE', *, *, #2873, .T. ) ;
#19834=EDGE_CURVE ( 'NONE', #43196, #41770, #50559, .T. ) ;
#19835=LINE ( 'NONE', #37419, #22014 ) ;
#19836=LINE ( 'NONE', #53913, #32317 ) ;
#19837=FACE_OUTER_BOUND ( 'NONE', #24020, .T. ) ;
#19838=LINE ( 'NONE', #37158, #29593 ) ;
#19839=DIRECTION ( 'NONE',  ( 0.7660212471507180654, -0.6427876096865404731, 0.005961354470445141482 ) ) ;
#19841=DIRECTION ( 'NONE',  ( 0.5364919789714477361, 0.6444004775717706579, 0.5449076811759711036 ) ) ;
#19843=ORIENTED_EDGE ( 'NONE', *, *, #51181, .T. ) ;
#19844=CARTESIAN_POINT ( 'NONE',  ( -17.16820509746884582, -4.889348428825661230, 11.37489936847406291 ) ) ;
#19845=DIRECTION ( 'NONE',  ( -0.5364919789714478471, 0.6444004775717705469, -0.5449076811759709926 ) ) ;
#19846=CARTESIAN_POINT ( 'NONE',  ( -13.73672976910459909, 0.000000000000000000, 12.22661844811216270 ) ) ;
#19847=DIRECTION ( 'NONE',  ( 0.000000000000000000, -1.000000000000000000, 0.000000000000000000 ) ) ;
#19848=PLANE ( 'NONE',  #17810 ) ;
#19850=CARTESIAN_POINT ( 'NONE',  ( -20.54049170961573267, 0.000000000000000000, 4.660556269540326646 ) ) ;
#19851=CARTESIAN_POINT ( 'NONE',  ( -26.13337879274045505, 0.000000000000000000, 6.833023547870798353 ) ) ;
#19852=DIRECTION ( 'NONE',  ( -0.3620778797217456546, 0.000000000000000000, -0.9321478471874540261 ) ) ;
#19853=CARTESIAN_POINT ( 'NONE',  ( -16.06709938707323460, 0.000000000000000000, 13.13181314741652628 ) ) ;
#19854=ORIENTED_EDGE ( 'NONE', *, *, #1517, .T. ) ;
#19855=LINE ( 'NONE', #38020, #53031 ) ;
#19856=ORIENTED_EDGE ( 'NONE', *, *, #39360, .F. ) ;
#19857=LINE ( 'NONE', #24661, #11409 ) ;
#19858=CARTESIAN_POINT ( 'NONE',  ( -13.10578669187797018, -0.1191753592594188005, 3.710421681786226777 ) ) ;
#19859=EDGE_LOOP ( 'NONE', ( #23925, #11976, #49425, #6206 ) ) ;
#19860=EDGE_CURVE ( 'NONE', #47452, #45757, #15605, .T. ) ;
#19861=ADVANCED_FACE ( 'NONE', ( #28125 ), #19622, .F. ) ;
#19862=EDGE_LOOP ( 'NONE', ( #33623, #14386, #17268, #30756 ) ) ;
#19863=DIRECTION ( 'NONE',  ( -0.7660212471507179544, -0.6427876096865405842, -0.005961354470445141482 ) ) ;
#19864=ORIENTED_EDGE ( 'NONE', *, *, #2651, .T. ) ;
#19865=ORIENTED_EDGE ( 'NONE', *, *, #47186, .F. ) ;
#19866=ORIENTED_EDGE ( 'NONE', *, *, #40791, .T. ) ;
#19867=CARTESIAN_POINT ( 'NONE',  ( -11.88300507327610411, 2.876837460659008361, 1.205908273609587189 ) ) ;
#19868=PLANE ( 'NONE',  #33253 ) ;
#19869=CARTESIAN_POINT ( 'NONE',  ( -8.409922665610809034, 0.000000000000000000, 10.23674650875856962 ) ) ;
#19871=ADVANCED_FACE ( 'NONE', ( #55358 ), #7374, .F. ) ;
#19872=ORIENTED_EDGE ( 'NONE', *, *, #22094, .T. ) ;
#19873=VERTEX_POINT ( 'NONE', #16452 ) ;
#19874=EDGE_CURVE ( 'NONE', #17790, #41029, #33781, .T. ) ;
#19876=CARTESIAN_POINT ( 'NONE',  ( -12.23851102634202448, -0.1191753592594197858, 11.68427982808754884 ) ) ;
#19877=ORIENTED_EDGE ( 'NONE', *, *, #782, .T. ) ;
#19878=PLANE ( 'NONE',  #27330 ) ;
#19879=ORIENTED_EDGE ( 'NONE', *, *, #22536, .F. ) ;
#19880=DIRECTION ( 'NONE',  ( 0.7660212471507180654, -0.6427876096865404731, 0.005961354470445141482 ) ) ;
#19881=PLANE ( 'NONE',  #28508 ) ;
#19882=VERTEX_POINT ( 'NONE', #24422 ) ;
#19883=DIRECTION ( 'NONE',  ( -0.7660212471507179544, -0.6427876096865405842, -0.005961354470445141482 ) ) ;
#19884=ADVANCED_FACE ( 'NONE', ( #24693 ), #28971, .F. ) ;
#19885=ADVANCED_FACE ( 'NONE', ( #28401 ), #42017, .F. ) ;
#19886=FACE_OUTER_BOUND ( 'NONE', #34342, .T. ) ;
#19887=ORIENTED_EDGE ( 'NONE', *, *, #19188, .F. ) ;
#19888=DIRECTION ( 'NONE',  ( 0.007781995580012663651, 0.000000000000000000, -0.9999697198139515519 ) ) ;
#19889=DIRECTION ( 'NONE',  ( -0.5449076811759708816, 0.6444004775717707689, 0.5364919789714475140 ) ) ;
#19890=ADVANCED_FACE ( 'NONE', ( #51099 ), #54799, .F. ) ;
#19891=CARTESIAN_POINT ( 'NONE',  ( -18.39746900504187010, 0.000000000000000000, 14.03700784672088808 ) ) ;
#19892=EDGE_LOOP ( 'NONE', ( #23460, #16930, #2640, #10061 ) ) ;
#19893=EDGE_CURVE ( 'NONE', #2943, #32088, #41189, .T. ) ;
#19894=DIRECTION ( 'NONE',  ( 0.5449076811759707706, 0.6444004775717708799, -0.5364919789714476250 ) ) ;
#19895=LINE ( 'NONE', #54515, #42341 ) ;
#19896=LINE ( 'NONE', #28984, #48500 ) ;
#19897=LINE ( 'NONE', #55112, #47702 ) ;
#19898=FACE_OUTER_BOUND ( 'NONE', #50336, .T. ) ;
#19899=FACE_OUTER_BOUND ( 'NONE', #36099, .T. ) ;
#19900=FACE_OUTER_BOUND ( 'NONE', #53140, .T. ) ;
#19902=PLANE ( 'NONE',  #7170 ) ;
#19903=CARTESIAN_POINT ( 'NONE',  ( -10.94028622754223967, 0.000000000000000000, 11.14038480894692995 ) ) ;
#19905=ORIENTED_EDGE ( 'NONE', *, *, #35705, .T. ) ;
#19906=DIRECTION ( 'NONE',  ( -0.5449076811759708816, 0.6444004775717707689, 0.5364919789714475140 ) ) ;
#19907=PLANE ( 'NONE',  #32 ) ;
#19908=DIRECTION ( 'NONE',  ( -0.005002170337468016433, -0.7660444431189770143, 0.6427681459581293666 ) ) ;
#19909=CARTESIAN_POINT ( 'NONE',  ( -11.77243710274829525, -0.1191753592594197858, 11.50324088822667612 ) ) ;
#19910=DIRECTION ( 'NONE',  ( 0.6427681459581294776, -0.7660444431189769032, 0.005002170337467562802 ) ) ;
#19911=EDGE_LOOP ( 'NONE', ( #29919, #8741, #6165, #53301 ) ) ;
#19912=ORIENTED_EDGE ( 'NONE', *, *, #50106, .F. ) ;
#19913=DIRECTION ( 'NONE',  ( 0.9999697198139515519, 0.000000000000000000, 0.007781995580013368816 ) ) ;
#19914=EDGE_CURVE ( 'NONE', #15067, #24549, #6548, .T. ) ;
#19917=LINE ( 'NONE', #10086, #46507 ) ;
#19918=VERTEX_POINT ( 'NONE', #15350 ) ;
#19919=CARTESIAN_POINT ( 'NONE',  ( -13.73672976910459909, 0.000000000000000000, 12.22661844811216270 ) ) ;
#19920=EDGE_CURVE ( 'NONE', #12052, #11173, #49967, .T. ) ;
#19921=ORIENTED_EDGE ( 'NONE', *, *, #31766, .T. ) ;
#19922=CARTESIAN_POINT ( 'NONE',  ( -14.16014573953108169, 0.000000000000000000, 6.926202016030694963 ) ) ;
#19923=ORIENTED_EDGE ( 'NONE', *, *, #39728, .F. ) ;
#19925=DIRECTION ( 'NONE',  ( 0.9999697198139515519, 0.000000000000000000, 0.007781995580013368816 ) ) ;
#19926=CARTESIAN_POINT ( 'NONE',  ( -19.79569077582305070, 0.000000000000000000, 14.58012466630350445 ) ) ;
#19927=LINE ( 'NONE', #32998, #346 ) ;
#19928=ADVANCED_FACE ( 'NONE', ( #45717 ), #41482, .F. ) ;
#19929=EDGE_CURVE ( 'NONE', #12677, #52731, #25280, .T. ) ;
#19930=EDGE_CURVE ( 'NONE', #6528, #52808, #9069, .T. ) ;
#19931=ORIENTED_EDGE ( 'NONE', *, *, #19874, .T. ) ;
#19932=CARTESIAN_POINT ( 'NONE',  ( -14.01545677930355183, 0.000000000000000000, 2.126011111488108174 ) ) ;
#19933=ORIENTED_EDGE ( 'NONE', *, *, #5793, .F. ) ;
#19934=EDGE_CURVE ( 'NONE', #5501, #47873, #55948, .T. ) ;
#19935=ORIENTED_EDGE ( 'NONE', *, *, #42608, .F. ) ;
#19936=ORIENTED_EDGE ( 'NONE', *, *, #39397, .F. ) ;
#19937=LINE ( 'NONE', #23923, #41310 ) ;
#19938=VERTEX_POINT ( 'NONE', #26123 ) ;
#19939=CARTESIAN_POINT ( 'NONE',  ( -17.31913335200585280, -0.1191753592594158168, 7.740285211709545976 ) ) ;
#19940=ORIENTED_EDGE ( 'NONE', *, *, #23171, .T. ) ;
#19941=DIRECTION ( 'NONE',  ( 0.6427681459581294776, -0.7660444431189769032, 0.005002170337467562802 ) ) ;
#19942=CARTESIAN_POINT ( 'NONE',  ( -18.39353927776868503, 5.629170628041515023, 3.647007019221114810 ) ) ;
#19943=ORIENTED_EDGE ( 'NONE', *, *, #56180, .T. ) ;
#19944=PLANE ( 'NONE',  #25001 ) ;
#19945=ORIENTED_EDGE ( 'NONE', *, *, #28749, .F. ) ;
#19946=ADVANCED_FACE ( 'NONE', ( #55645 ), #39159, .F. ) ;
#19947=AXIS2_PLACEMENT_3D ( 'NONE', #10687, #14923, #35382 ) ;
#19948=ADVANCED_FACE ( 'NONE', ( #3964 ), #12766, .F. ) ;
#19949=PLANE ( 'NONE',  #1056 ) ;
#19950=CARTESIAN_POINT ( 'NONE',  ( -9.310908773652148085, 0.000000000000000000, 6.594607829569027579 ) ) ;
#19951=FACE_OUTER_BOUND ( 'NONE', #43368, .T. ) ;
#19952=PLANE ( 'NONE',  #32943 ) ;
#19953=EDGE_CURVE ( 'NONE', #38023, #48125, #17044, .T. ) ;
#19954=CARTESIAN_POINT ( 'NONE',  ( -23.33771345073609638, -0.1191753592594197858, 5.846786880686956955 ) ) ;
#19956=ORIENTED_EDGE ( 'NONE', *, *, #7298, .F. ) ;
#19957=EDGE_CURVE ( 'NONE', #47084, #31029, #17588, .T. ) ;
#19958=ORIENTED_EDGE ( 'NONE', *, *, #14936, .T. ) ;
#19959=CARTESIAN_POINT ( 'NONE',  ( -17.77514808833108262, -0.1191753592594194527, 6.628740190168248780 ) ) ;
#19960=DIRECTION ( 'NONE',  ( 0.9999697198139515519, 0.000000000000000000, 0.007781995580013368816 ) ) ;
#19961=LINE ( 'NONE', #7199, #37564 ) ;
#19962=EDGE_CURVE ( 'NONE', #29543, #678, #47968, .T. ) ;
#19963=DIRECTION ( 'NONE',  ( 0.005961354470445682716, -0.6427876096865404731, -0.7660212471507180654 ) ) ;
#19964=LINE ( 'NONE', #7201, #40366 ) ;
#19965=ORIENTED_EDGE ( 'NONE', *, *, #14690, .T. ) ;
#19966=DIRECTION ( 'NONE',  ( 0.000000000000000000, -1.000000000000000000, 0.000000000000000000 ) ) ;
#19967=FACE_OUTER_BOUND ( 'NONE', #3630, .T. ) ;
#19968=ORIENTED_EDGE ( 'NONE', *, *, #37925, .T. ) ;
#19969=LINE ( 'NONE', #1805, #22048 ) ;
#19970=DIRECTION ( 'NONE',  ( 0.007781995580012662783, 0.000000000000000000, -0.9999697198139514409 ) ) ;
#19971=ORIENTED_EDGE ( 'NONE', *, *, #17850, .F. ) ;
#19972=DIRECTION ( 'NONE',  ( -0.9999697198139514409, -0.000000000000000000, -0.007781995580013368816 ) ) ;
#19973=CARTESIAN_POINT ( 'NONE',  ( -14.93495759592298988, 0.000000000000000000, 12.77129166681078409 ) ) ;
#19974=FACE_OUTER_BOUND ( 'NONE', #9468, .T. ) ;
#19975=DIRECTION ( 'NONE',  ( 0.005002170337468016433, -0.7660444431189770143, -0.6427681459581293666 ) ) ;
#19976=DIRECTION ( 'NONE',  ( -0.9999697198139514409, -0.000000000000000000, -0.007781995580013368816 ) ) ;
#19977=EDGE_LOOP ( 'NONE', ( #27638, #20803, #4153, #30842 ) ) ;
#19978=ORIENTED_EDGE ( 'NONE', *, *, #14206, .T. ) ;
#19979=DIRECTION ( 'NONE',  ( -0.5449076811759708816, 0.6444004775717707689, 0.5364919789714475140 ) ) ;
#19980=DIRECTION ( 'NONE',  ( 0.9999697198139515519, 0.000000000000000000, 0.007781995580013368816 ) ) ;
#19981=DIRECTION ( 'NONE',  ( 0.007781995580012663651, 0.000000000000000000, -0.9999697198139515519 ) ) ;
#19982=CARTESIAN_POINT ( 'NONE',  ( -18.35049997161669566, 0.000000000000000000, 8.001587919891903766 ) ) ;
#19983=CARTESIAN_POINT ( 'NONE',  ( -18.70154782850797659, -0.1191753592594164690, 6.252198663374462839 ) ) ;
#19984=LINE ( 'NONE', #32769, #32194 ) ;
#19986=DIRECTION ( 'NONE',  ( -0.005961354470445682716, -0.6427876096865404731, 0.7660212471507180654 ) ) ;
#19987=VECTOR ( 'NONE', #17067, 1000.000000000000227 ) ;
#19988=CARTESIAN_POINT ( 'NONE',  ( -19.60990026154428278, 0.000000000000000000, 4.498472333781370125 ) ) ;
#19989=FACE_OUTER_BOUND ( 'NONE', #220, .T. ) ;
#19990=ORIENTED_EDGE ( 'NONE', *, *, #50231, .F. ) ;
#19992=CARTESIAN_POINT ( 'NONE',  ( -12.15271748404464880, 0.000000000000000000, 1.601849296007406664 ) ) ;
#19993=CARTESIAN_POINT ( 'NONE',  ( -16.64402593923450979, 4.657758921906512306, 2.998429744135719943 ) ) ;
#19994=EDGE_CURVE ( 'NONE', #23668, #8314, #13054, .T. ) ;
#19995=ORIENTED_EDGE ( 'NONE', *, *, #36619, .F. ) ;
#19996=DIRECTION ( 'NONE',  ( 0.007781995580012662783, 0.000000000000000000, -0.9999697198139514409 ) ) ;
#19997=ORIENTED_EDGE ( 'NONE', *, *, #50487, .T. ) ;
#19998=ADVANCED_FACE ( 'NONE', ( #34358 ), #20994, .F. ) ;
#19999=EDGE_CURVE ( 'NONE', #35810, #3699, #51662, .T. ) ;
#20000=VERTEX_POINT ( 'NONE', #17891 ) ;
#20001=EDGE_LOOP ( 'NONE', ( #7593, #34366, #14298, #8148, #3451 ) ) ;
#20002=ORIENTED_EDGE ( 'NONE', *, *, #9836, .T. ) ;
#20003=VERTEX_POINT ( 'NONE', #12506 ) ;
#20004=CARTESIAN_POINT ( 'NONE',  ( -18.29747203306047609, -0.1191753592594177458, 14.03778604627889059 ) ) ;
#20005=ORIENTED_EDGE ( 'NONE', *, *, #42701, .T. ) ;
#20006=AXIS2_PLACEMENT_3D ( 'NONE', #24590, #32576, #45915 ) ;
#20008=DIRECTION ( 'NONE',  ( 0.9999697198139515519, 0.000000000000000000, 0.007781995580013368816 ) ) ;
#20009=ORIENTED_EDGE ( 'NONE', *, *, #46120, .F. ) ;
#20010=EDGE_LOOP ( 'NONE', ( #52842, #17034, #31832, #39819 ) ) ;
#20011=CARTESIAN_POINT ( 'NONE',  ( -12.08693257711994384, -0.03228989815065527735, 1.575265987285825675 ) ) ;
#20012=LINE ( 'NONE', #24014, #39384 ) ;
#20013=CARTESIAN_POINT ( 'NONE',  ( -22.40478740399063895, 0.000000000000000000, 5.384712028983816623 ) ) ;
#20014=DIRECTION ( 'NONE',  ( -0.5449076811759708816, 0.6444004775717707689, 0.5364919789714475140 ) ) ;
#20015=CARTESIAN_POINT ( 'NONE',  ( -12.80458192191714595, 0.000000000000000000, 11.86454056839041726 ) ) ;
#20016=EDGE_LOOP ( 'NONE', ( #29216, #45049, #9955, #5814 ) ) ;
#20017=ORIENTED_EDGE ( 'NONE', *, *, #30411, .F. ) ;
#20018=VECTOR ( 'NONE', #29826, 999.9999999999998863 ) ;
#20020=DIRECTION ( 'NONE',  ( 0.007781995580012663651, -3.146120232559066537E-19, -0.9999697198139514409 ) ) ;
#20021=ADVANCED_FACE ( 'NONE', ( #16747 ), #12207, .F. ) ;
#20022=AXIS2_PLACEMENT_3D ( 'NONE', #5670, #37166, #1947 ) ;
#20023=CARTESIAN_POINT ( 'NONE',  ( 2.072287782118878319, 0.000000000000000000, -2.950529333540147015 ) ) ;
#20024=CARTESIAN_POINT ( 'NONE',  ( 2.072287782118878319, 0.000000000000000000, -2.950529333540147015 ) ) ;
#20025=EDGE_CURVE ( 'NONE', #156, #21894, #21837, .T. ) ;
#20026=PLANE ( 'NONE',  #28580 ) ;
#20027=CARTESIAN_POINT ( 'NONE',  ( -19.45503627000849889, 0.000000000000000000, 7.556996783084074742 ) ) ;
#20028=ORIENTED_EDGE ( 'NONE', *, *, #5021, .F. ) ;
#20029=PLANE ( 'NONE',  #4778 ) ;
#20030=ORIENTED_EDGE ( 'NONE', *, *, #42046, .F. ) ;
#20032=FACE_OUTER_BOUND ( 'NONE', #45426, .T. ) ;
#20033=LINE ( 'NONE', #11545, #55042 ) ;
#20034=DIRECTION ( 'NONE',  ( -0.5449076811759708816, 0.6444004775717707689, 0.5364919789714475140 ) ) ;
#20035=EDGE_CURVE ( 'NONE', #15181, #21588, #38316, .T. ) ;
#20036=FACE_OUTER_BOUND ( 'NONE', #8439, .T. ) ;
#20037=DIRECTION ( 'NONE',  ( 0.007781995580012662783, 0.000000000000000000, -0.9999697198139514409 ) ) ;
#20039=VERTEX_POINT ( 'NONE', #8226 ) ;
#20040=DIRECTION ( 'NONE',  ( -0.3620778797217455991, 0.000000000000000000, -0.9321478471874540261 ) ) ;
#20041=CARTESIAN_POINT ( 'NONE',  ( -1.905187828007888884, 6.291258001618519557, 3.958413228513044668 ) ) ;
#20042=LINE ( 'NONE', #54409, #16086 ) ;
#20043=AXIS2_PLACEMENT_3D ( 'NONE', #34645, #56234, #51966 ) ;
#20044=VECTOR ( 'NONE', #7597, 999.9999999999998863 ) ;
#20045=CARTESIAN_POINT ( 'NONE',  ( 0.000000000000000000, 0.000000000000000000, 0.000000000000000000 ) ) ;
#20046=CARTESIAN_POINT ( 'NONE',  ( -16.02024972601142494, 0.000000000000000000, 7.111732312921445143 ) ) ;
#20047=DIRECTION ( 'NONE',  ( -0.7660212471507179544, -0.6427876096865405842, -0.005961354470445141482 ) ) ;
#20048=CARTESIAN_POINT ( 'NONE',  ( -13.61044419115797410, -0.1159828484229804557, 8.505132312139858541 ) ) ;
#20050=LINE ( 'NONE', #55541, #26505 ) ;
#20051=EDGE_CURVE ( 'NONE', #39913, #15552, #25541, .T. ) ;
#20052=ADVANCED_FACE ( 'NONE', ( #43169 ), #17292, .F. ) ;
#20053=ORIENTED_EDGE ( 'NONE', *, *, #11027, .F. ) ;
#20054=EDGE_CURVE ( 'NONE', #42137, #2673, #47701, .T. ) ;
#20055=EDGE_CURVE ( 'NONE', #45226, #33224, #816, .T. ) ;
#20056=AXIS2_PLACEMENT_3D ( 'NONE', #1148, #17946, #6011 ) ;
#20057=ORIENTED_EDGE ( 'NONE', *, *, #18198, .F. ) ;
#20059=ORIENTED_EDGE ( 'NONE', *, *, #19291, .T. ) ;
#20060=ORIENTED_EDGE ( 'NONE', *, *, #13424, .F. ) ;
#20061=CARTESIAN_POINT ( 'NONE',  ( -16.34593356761463667, -3.432230869623162928, 3.121130690641215732 ) ) ;
#20062=CARTESIAN_POINT ( 'NONE',  ( -31.72626587586518099, 0.000000000000000000, 9.005490826201270949 ) ) ;
#20063=DIRECTION ( 'NONE',  ( -0.005961354470445682716, -0.6427876096865404731, 0.7660212471507180654 ) ) ;
#20064=EDGE_LOOP ( 'NONE', ( #1592, #11366, #8408, #9658 ) ) ;
#20065=ORIENTED_EDGE ( 'NONE', *, *, #44506, .T. ) ;
#20066=ORIENTED_EDGE ( 'NONE', *, *, #21152, .T. ) ;
#20067=CARTESIAN_POINT ( 'NONE',  ( -15.51131483200478201, 1.095915999411505526, 2.672087720579162884 ) ) ;
#20068=ORIENTED_EDGE ( 'NONE', *, *, #53108, .F. ) ;
#20069=EDGE_CURVE ( 'NONE', #32592, #3505, #44824, .T. ) ;
#20071=CARTESIAN_POINT ( 'NONE',  ( -16.53317331066696383, 0.000000000000000000, 13.31285208727739899 ) ) ;
#20072=DIRECTION ( 'NONE',  ( 0.7660212471507180654, -0.6427876096865404731, 0.005961354470445141482 ) ) ;
#20073=VERTEX_POINT ( 'NONE', #22434 ) ;
#20076=VECTOR ( 'NONE', #52168, 1000.000000000000227 ) ;
#20077=CARTESIAN_POINT ( 'NONE',  ( -19.69569380384165669, -0.1191753592594177458, 14.58090286586150697 ) ) ;
#20078=FACE_OUTER_BOUND ( 'NONE', #52987, .T. ) ;
#20079=CARTESIAN_POINT ( 'NONE',  ( 2.072287782118878319, 0.000000000000000000, -2.950529333540147015 ) ) ;
#20080=DIRECTION ( 'NONE',  ( 0.6427681459581294776, -0.7660444431189769032, 0.005002170337467562802 ) ) ;
#20082=LINE ( 'NONE', #24362, #25903 ) ;
#20083=CARTESIAN_POINT ( 'NONE',  ( -16.06709938707323460, 0.000000000000000000, 13.13181314741652628 ) ) ;
#20084=CARTESIAN_POINT ( 'NONE',  ( -17.46532115785441519, 0.000000000000000000, 13.67492996699914265 ) ) ;
#20085=DIRECTION ( 'NONE',  ( 0.7660212471507180654, -0.6427876096865404731, 0.005961354470445141482 ) ) ;
#20086=PLANE ( 'NONE',  #9351 ) ;
#20088=DIRECTION ( 'NONE',  ( 0.6427681459581294776, -0.7660444431189769032, 0.005002170337467562802 ) ) ;
#20089=ORIENTED_EDGE ( 'NONE', *, *, #19929, .T. ) ;
#20090=FACE_OUTER_BOUND ( 'NONE', #24764, .T. ) ;
#20091=CARTESIAN_POINT ( 'NONE',  ( -18.54926312204414174, 1.905425754524005200, 7.213613129226924769 ) ) ;
#20092=DIRECTION ( 'NONE',  ( 0.000000000000000000, -0.000000000000000000, -1.000000000000000000 ) ) ;
#20093=EDGE_CURVE ( 'NONE', #23151, #50536, #5943, .T. ) ;
#20094=LINE ( 'NONE', #32890, #5106 ) ;
#20095=PLANE ( 'NONE',  #44913 ) ;
#20096=VECTOR ( 'NONE', #54049, 999.9999999999998863 ) ;
#20097=DIRECTION ( 'NONE',  ( 0.007781995580012663651, -3.146120232559066537E-19, -0.9999697198139514409 ) ) ;
#20098=ORIENTED_EDGE ( 'NONE', *, *, #54706, .T. ) ;
#20099=DIRECTION ( 'NONE',  ( 0.9999697198139515519, 0.000000000000000000, 0.007781995580013368816 ) ) ;
#20100=LINE ( 'NONE', #32622, #48394 ) ;
#20101=DIRECTION ( 'NONE',  ( 0.5364919789714477361, 0.6444004775717706579, 0.5449076811759711036 ) ) ;
#20102=LINE ( 'NONE', #33208, #52703 ) ;
#20103=CARTESIAN_POINT ( 'NONE',  ( -11.22505254250097906, -0.1166911823299084244, 1.141818036232515876 ) ) ;
#20104=ADVANCED_FACE ( 'NONE', ( #48225 ), #14190, .F. ) ;
#20105=CARTESIAN_POINT ( 'NONE',  ( 2.072287782118878319, 0.000000000000000000, -2.950529333540147015 ) ) ;
#20106=LINE ( 'NONE', #6255, #42971 ) ;
#20107=EDGE_CURVE ( 'NONE', #15058, #38157, #5639, .T. ) ;
#20108=DIRECTION ( 'NONE',  ( 0.005002170337468016433, -0.7660444431189770143, -0.6427681459581293666 ) ) ;
#20109=EDGE_CURVE ( 'NONE', #36639, #3399, #22965, .T. ) ;
#20110=LINE ( 'NONE', #51060, #22902 ) ;
#20111=ORIENTED_EDGE ( 'NONE', *, *, #34582, .T. ) ;
#20112=PLANE ( 'NONE',  #25829 ) ;
#20113=FACE_OUTER_BOUND ( 'NONE', #23396, .T. ) ;
#20114=ORIENTED_EDGE ( 'NONE', *, *, #7771, .T. ) ;
#20115=CARTESIAN_POINT ( 'NONE',  ( -12.70458494993575194, -0.1191753592594197858, 11.86531876794841978 ) ) ;
#20116=FACE_OUTER_BOUND ( 'NONE', #248, .T. ) ;
#20117=EDGE_CURVE ( 'NONE', #1131, #46770, #22683, .T. ) ;
#20118=VECTOR ( 'NONE', #29359, 999.9999999999998863 ) ;
#20119=VECTOR ( 'NONE', #11919, 1000.000000000000227 ) ;
#20120=ORIENTED_EDGE ( 'NONE', *, *, #29785, .T. ) ;
#20121=EDGE_CURVE ( 'NONE', #5026, #18137, #45124, .T. ) ;
#20122=VERTEX_POINT ( 'NONE', #49367 ) ;
#20123=DIRECTION ( 'NONE',  ( 0.5364919789714477361, 0.6444004775717706579, 0.5449076811759711036 ) ) ;
#20124=EDGE_CURVE ( 'NONE', #4731, #27276, #18988, .T. ) ;
#20125=ORIENTED_EDGE ( 'NONE', *, *, #56174, .T. ) ;
#20126=VERTEX_POINT ( 'NONE', #6225 ) ;
#20127=AXIS2_PLACEMENT_3D ( 'NONE', #53430, #48620, #31587 ) ;
#20128=ORIENTED_EDGE ( 'NONE', *, *, #32052, .F. ) ;
#20129=CARTESIAN_POINT ( 'NONE',  ( -19.60990026154428278, 0.000000000000000000, 4.498472333781370125 ) ) ;
#20130=CARTESIAN_POINT ( 'NONE',  ( -11.40636015113596180, 0.000000000000000000, 11.32142374880780089 ) ) ;
#20131=DIRECTION ( 'NONE',  ( 0.007781995580012662783, 0.000000000000000000, -0.9999697198139514409 ) ) ;
#20132=ADVANCED_FACE ( 'NONE', ( #52507 ), #53074, .F. ) ;
#20133=ORIENTED_EDGE ( 'NONE', *, *, #37680, .T. ) ;
#20134=VECTOR ( 'NONE', #19541, 1000.000000000000227 ) ;
#20135=VERTEX_POINT ( 'NONE', #18418 ) ;
#20136=ADVANCED_FACE ( 'NONE', ( #10483 ), #31773, .F. ) ;
#20138=CARTESIAN_POINT ( 'NONE',  ( -16.11361633748963129, 1.257817950434005683, 2.900876559667310950 ) ) ;
#20139=ORIENTED_EDGE ( 'NONE', *, *, #46040, .F. ) ;
#20140=DIRECTION ( 'NONE',  ( -0.7660212471507179544, -0.6427876096865405842, -0.005961354470445141482 ) ) ;
#20141=ORIENTED_EDGE ( 'NONE', *, *, #26754, .T. ) ;
#20142=LINE ( 'NONE', #53416, #23966 ) ;
#20143=CARTESIAN_POINT ( 'NONE',  ( -9.942607371508632497, 0.000000000000000000, 2.357713023554631970 ) ) ;
#20144=ORIENTED_EDGE ( 'NONE', *, *, #35136, .T. ) ;
#20145=CARTESIAN_POINT ( 'NONE',  ( -20.71168680238113424, 4.981562823951510843, 13.10203691794590419 ) ) ;
#20146=VECTOR ( 'NONE', #49552, 1000.000000000000227 ) ;
#20147=LINE ( 'NONE', #19323, #47224 ) ;
#20148=ORIENTED_EDGE ( 'NONE', *, *, #49035, .F. ) ;
#20149=DIRECTION ( 'NONE',  ( 0.5449076811759707706, 0.6444004775717708799, -0.5364919789714476250 ) ) ;
#20151=VECTOR ( 'NONE', #40412, 999.9999999999998863 ) ;
#20152=FACE_OUTER_BOUND ( 'NONE', #34001, .T. ) ;
#20153=ORIENTED_EDGE ( 'NONE', *, *, #34491, .T. ) ;
#20154=VECTOR ( 'NONE', #27539, 1000.000000000000000 ) ;
#20156=LINE ( 'NONE', #41491, #22866 ) ;
#20157=CARTESIAN_POINT ( 'NONE',  ( -3.486932065698848504, -6.851436116247921149, -1.863930744634968883 ) ) ;
#20158=CARTESIAN_POINT ( 'NONE',  ( -23.33693525117809386, 0.000000000000000000, 5.746789908705562944 ) ) ;
#20159=EDGE_CURVE ( 'NONE', #428, #11699, #43981, .T. ) ;
#20160=DIRECTION ( 'NONE',  ( 0.9999697198139515519, 0.000000000000000000, 0.007781995580013368816 ) ) ;
#20161=CARTESIAN_POINT ( 'NONE',  ( -12.52600435597107342, 0.000000000000000000, 1.768270304842026963 ) ) ;
#20162=LINE ( 'NONE', #3693, #51484 ) ;
#20163=VECTOR ( 'NONE', #47887, 1000.000000000000114 ) ;
#20165=VECTOR ( 'NONE', #11249, 1000.000000000000227 ) ;
#20166=ORIENTED_EDGE ( 'NONE', *, *, #11402, .F. ) ;
#20167=DIRECTION ( 'NONE',  ( -0.005961354470445682716, -0.6427876096865404731, 0.7660212471507180654 ) ) ;
#20168=CARTESIAN_POINT ( 'NONE',  ( -12.54480507611877194, 0.000000000000000000, 4.184122468351399782 ) ) ;
#20169=DIRECTION ( 'NONE',  ( 0.007781995580012663651, 0.000000000000000000, -0.9999697198139515519 ) ) ;
#20170=VERTEX_POINT ( 'NONE', #49079 ) ;
#20171=LINE ( 'NONE', #37222, #12069 ) ;
#20172=CARTESIAN_POINT ( 'NONE',  ( -13.10866074538325243, -0.1191753592594186895, 4.079731385043992020 ) ) ;
#20173=CARTESIAN_POINT ( 'NONE',  ( -25.20123094555300369, 0.000000000000000000, 6.470945668149052032 ) ) ;
#20174=AXIS2_PLACEMENT_3D ( 'NONE', #20015, #33938, #12641 ) ;
#20175=AXIS2_PLACEMENT_3D ( 'NONE', #37536, #54856, #29019 ) ;
#20176=DIRECTION ( 'NONE',  ( -0.005961354470445682716, -0.6427876096865404731, 0.7660212471507180654 ) ) ;
#20177=ADVANCED_FACE ( 'NONE', ( #40842 ), #30917, .F. ) ;
#20179=ORIENTED_EDGE ( 'NONE', *, *, #11641, .T. ) ;
#20180=ORIENTED_EDGE ( 'NONE', *, *, #43279, .T. ) ;
#20181=DIRECTION ( 'NONE',  ( -0.5364919789714478471, 0.6444004775717705469, -0.5449076811759709926 ) ) ;
#20182=AXIS2_PLACEMENT_3D ( 'NONE', #39986, #53885, #27802 ) ;
#20183=CARTESIAN_POINT ( 'NONE',  ( -10.90924386075947972, 0.000000000000000000, 7.151507342369550990 ) ) ;
#20184=CARTESIAN_POINT ( 'NONE',  ( 2.072287782118878319, 0.000000000000000000, -2.950529333540147015 ) ) ;
#20185=ORIENTED_EDGE ( 'NONE', *, *, #37145, .T. ) ;
#20186=EDGE_CURVE ( 'NONE', #28807, #11287, #5105, .T. ) ;
#20188=VECTOR ( 'NONE', #54473, 1000.000000000000227 ) ;
#20189=VERTEX_POINT ( 'NONE', #9646 ) ;
#20190=PLANE ( 'NONE',  #10246 ) ;
#20191=ADVANCED_FACE ( 'NONE', ( #26966 ), #44279, .F. ) ;
#20192=ORIENTED_EDGE ( 'NONE', *, *, #11210, .F. ) ;
#20193=ORIENTED_EDGE ( 'NONE', *, *, #54532, .F. ) ;
#20194=CARTESIAN_POINT ( 'NONE',  ( -14.96058358053937454, -0.1134144341942091572, 2.592825150574666448 ) ) ;
#20195=VECTOR ( 'NONE', #30428, 999.9999999999998863 ) ;
#20196=CARTESIAN_POINT ( 'NONE',  ( -12.80458192191714595, 0.000000000000000000, 11.86454056839041726 ) ) ;
#20197=CARTESIAN_POINT ( 'NONE',  ( -21.47419595591918906, 0.000000000000000000, 5.222628093224860102 ) ) ;
#20198=ORIENTED_EDGE ( 'NONE', *, *, #40271, .F. ) ;
#20199=VECTOR ( 'NONE', #54448, 1000.000000000000227 ) ;
#20200=EDGE_CURVE ( 'NONE', #29054, #12905, #18724, .T. ) ;
#20202=CARTESIAN_POINT ( 'NONE',  ( -15.54411661514920695, 0.000000000000000000, 5.638109411658397185 ) ) ;
#20203=ORIENTED_EDGE ( 'NONE', *, *, #1843, .F. ) ;
#20204=ORIENTED_EDGE ( 'NONE', *, *, #41803, .T. ) ;
#20205=EDGE_CURVE ( 'NONE', #37323, #42326, #49904, .T. ) ;
#20206=VECTOR ( 'NONE', #47825, 999.9999999999998863 ) ;
#20207=ORIENTED_EDGE ( 'NONE', *, *, #52309, .F. ) ;
#20208=LINE ( 'NONE', #14575, #53112 ) ;
#20209=VECTOR ( 'NONE', #24445, 999.9999999999998863 ) ;
#20210=PLANE ( 'NONE',  #45784 ) ;
#20211=ORIENTED_EDGE ( 'NONE', *, *, #28097, .F. ) ;
#20212=LINE ( 'NONE', #11968, #17568 ) ;
#20213=ORIENTED_EDGE ( 'NONE', *, *, #33762, .T. ) ;
#20214=LINE ( 'NONE', #49780, #29461 ) ;
#20215=CARTESIAN_POINT ( 'NONE',  ( -17.46532115785441519, 0.000000000000000000, 13.67492996699914265 ) ) ;
#20216=VERTEX_POINT ( 'NONE', #6483 ) ;
#20217=CARTESIAN_POINT ( 'NONE',  ( -15.72637881786665837, 1.905425754524006532, 2.729798276854666028 ) ) ;
#20218=VECTOR ( 'NONE', #30317, 1000.000000000000227 ) ;
#20219=EDGE_LOOP ( 'NONE', ( #31014, #9806, #49123, #31996 ) ) ;
#20220=VECTOR ( 'NONE', #33432, 999.9999999999998863 ) ;
#20221=DIRECTION ( 'NONE',  ( -0.5364919789714478471, 0.6444004775717705469, -0.5449076811759709926 ) ) ;
#20222=LINE ( 'NONE', #6920, #20228 ) ;
#20223=DIRECTION ( 'NONE',  ( -0.6427681459581293666, -0.7660444431189770143, -0.005002170337467561935 ) ) ;
#20224=CARTESIAN_POINT ( 'NONE',  ( -16.76389984325721727, 0.000000000000000000, 8.952605404790253019 ) ) ;
#20225=DIRECTION ( 'NONE',  ( 0.007781995580012662783, 0.000000000000000000, -0.9999697198139514409 ) ) ;
#20226=ORIENTED_EDGE ( 'NONE', *, *, #27877, .F. ) ;
#20227=ADVANCED_FACE ( 'NONE', ( #50494 ), #46479, .F. ) ;
#20228=VECTOR ( 'NONE', #24774, 999.9999999999998863 ) ;
#20229=EDGE_LOOP ( 'NONE', ( #56093, #49793, #41533, #42548 ) ) ;
#20230=LINE ( 'NONE', #42403, #28251 ) ;
#20232=EDGE_CURVE ( 'NONE', #39606, #2632, #6768, .T. ) ;
#20233=VECTOR ( 'NONE', #9454, 999.9999999999998863 ) ;
#20235=CARTESIAN_POINT ( 'NONE',  ( -24.26986129792355129, -0.1191753592594197858, 6.208864760408702388 ) ) ;
#20236=LINE ( 'NONE', #19406, #32443 ) ;
#20237=DIRECTION ( 'NONE',  ( 0.5449076811759707706, 0.6444004775717708799, -0.5364919789714476250 ) ) ;
#20238=VERTEX_POINT ( 'NONE', #50188 ) ;
#20239=EDGE_CURVE ( 'NONE', #36106, #55458, #23789, .T. ) ;
#20240=CARTESIAN_POINT ( 'NONE',  ( -28.92982233430281980, 0.000000000000000000, 7.919257187036034651 ) ) ;
#20241=PLANE ( 'NONE',  #12361 ) ;
#20242=ORIENTED_EDGE ( 'NONE', *, *, #49469, .F. ) ;
#20243=VECTOR ( 'NONE', #19739, 1000.000000000000000 ) ;
#20244=LINE ( 'NONE', #24504, #13889 ) ;
#20245=DIRECTION ( 'NONE',  ( -0.005961354470445682716, -0.6427876096865404731, 0.7660212471507180654 ) ) ;
#20246=VERTEX_POINT ( 'NONE', #3044 ) ;
#20247=EDGE_CURVE ( 'NONE', #10472, #45226, #45950, .T. ) ;
#20248=EDGE_CURVE ( 'NONE', #52686, #46703, #24088, .T. ) ;
#20249=EDGE_CURVE ( 'NONE', #52604, #4570, #33176, .T. ) ;
#20250=AXIS2_PLACEMENT_3D ( 'NONE', #3199, #33576, #20533 ) ;
#20251=VECTOR ( 'NONE', #28796, 999.9999999999998863 ) ;
#20252=DIRECTION ( 'NONE',  ( -0.005961354470445682716, -0.6427876096865404731, 0.7660212471507180654 ) ) ;
#20254=DIRECTION ( 'NONE',  ( -0.5364919789714478471, 0.6444004775717705469, -0.5449076811759709926 ) ) ;
#20255=DIRECTION ( 'NONE',  ( -0.9999697198139514409, -0.000000000000000000, -0.007781995580013368816 ) ) ;
#20256=DIRECTION ( 'NONE',  ( -0.005961354470445682716, -0.6427876096865404731, 0.7660212471507180654 ) ) ;
#20258=ORIENTED_EDGE ( 'NONE', *, *, #27144, .F. ) ;
#20259=AXIS2_PLACEMENT_3D ( 'NONE', #37187, #54489, #32925 ) ;
#20260=VECTOR ( 'NONE', #51686, 1000.000000000000227 ) ;
#20261=VERTEX_POINT ( 'NONE', #19821 ) ;
#20262=DIRECTION ( 'NONE',  ( 0.9999697198139515519, 0.000000000000000000, 0.007781995580013368816 ) ) ;
#20263=DIRECTION ( 'NONE',  ( 0.000000000000000000, -0.000000000000000000, -1.000000000000000000 ) ) ;
#20264=CARTESIAN_POINT ( 'NONE',  ( -18.66354898467281132, 0.000000000000000000, 14.21960318569776582 ) ) ;
#20265=CARTESIAN_POINT ( 'NONE',  ( -17.93139508144814442, 0.000000000000000000, 13.85596890686001537 ) ) ;
#20266=DIRECTION ( 'NONE',  ( 0.000000000000000000, -0.000000000000000000, -1.000000000000000000 ) ) ;
#20267=ADVANCED_FACE ( 'NONE', ( #36584 ), #28064, .F. ) ;
#20268=DIRECTION ( 'NONE',  ( 0.005002170337468016433, -0.7660444431189770143, -0.6427681459581293666 ) ) ;
#20269=ORIENTED_EDGE ( 'NONE', *, *, #28418, .T. ) ;
#20270=DIRECTION ( 'NONE',  ( 0.000000000000000000, -0.000000000000000000, -1.000000000000000000 ) ) ;
#20271=EDGE_CURVE ( 'NONE', #547, #6826, #11297, .T. ) ;
#20272=CARTESIAN_POINT ( 'NONE',  ( -16.06709938707323460, 0.000000000000000000, 13.13181314741652628 ) ) ;
#20273=PLANE ( 'NONE',  #18774 ) ;
#20274=ORIENTED_EDGE ( 'NONE', *, *, #46702, .F. ) ;
#20275=VECTOR ( 'NONE', #4033, 1000.000000000000000 ) ;
#20276=EDGE_CURVE ( 'NONE', #27953, #47622, #19543, .T. ) ;
#20278=CARTESIAN_POINT ( 'NONE',  ( -13.27065584551087163, 0.000000000000000000, 12.04557950825129176 ) ) ;
#20279=AXIS2_PLACEMENT_3D ( 'NONE', #32874, #37407, #54727 ) ;
#20280=CARTESIAN_POINT ( 'NONE',  ( -14.66887761629205222, 0.000000000000000000, 12.58869632783390990 ) ) ;
#20281=ORIENTED_EDGE ( 'NONE', *, *, #37400, .F. ) ;
#20282=EDGE_CURVE ( 'NONE', #35036, #15384, #41413, .T. ) ;
#20283=PLANE ( 'NONE',  #7789 ) ;
#20284=VECTOR ( 'NONE', #55580, 999.9999999999998863 ) ;
#20285=VERTEX_POINT ( 'NONE', #24357 ) ;
#20286=EDGE_CURVE ( 'NONE', #18631, #31141, #32601, .T. ) ;
#20287=VERTEX_POINT ( 'NONE', #3354 ) ;
#20288=ORIENTED_EDGE ( 'NONE', *, *, #19581, .F. ) ;
#20289=ORIENTED_EDGE ( 'NONE', *, *, #25722, .F. ) ;
#20290=VECTOR ( 'NONE', #54491, 1000.000000000000000 ) ;
#20291=CARTESIAN_POINT ( 'NONE',  ( 1.710209902397132220, 0.000000000000000000, -3.882677180727601041 ) ) ;
#20292=VERTEX_POINT ( 'NONE', #54441 ) ;
#20293=VECTOR ( 'NONE', #43177, 1000.000000000000114 ) ;
#20294=VERTEX_POINT ( 'NONE', #15541 ) ;
#20295=PLANE ( 'NONE',  #463 ) ;
#20296=ORIENTED_EDGE ( 'NONE', *, *, #10970, .F. ) ;
#20297=ORIENTED_EDGE ( 'NONE', *, *, #25329, .F. ) ;
#20298=AXIS2_PLACEMENT_3D ( 'NONE', #41449, #15572, #46233 ) ;
#20299=AXIS2_PLACEMENT_3D ( 'NONE', #1265, #35643, #27389 ) ;
#20300=DIRECTION ( 'NONE',  ( 0.000000000000000000, -1.000000000000000000, 0.000000000000000000 ) ) ;
#20301=DIRECTION ( 'NONE',  ( 0.005002170337468016433, -0.7660444431189770143, -0.6427681459581293666 ) ) ;
#20302=CARTESIAN_POINT ( 'NONE',  ( -12.13851405436063047, 0.000000000000000000, 11.68505802764555135 ) ) ;
#20303=DIRECTION ( 'NONE',  ( -0.5364919789714478471, 0.6444004775717705469, -0.5449076811759709926 ) ) ;
#20304=CARTESIAN_POINT ( 'NONE',  ( -12.75916928760797653, 0.000000000000000000, 6.029114585524220082 ) ) ;
#20305=EDGE_LOOP ( 'NONE', ( #27861, #28608, #19654, #38462 ) ) ;
#20306=VERTEX_POINT ( 'NONE', #32872 ) ;
#20307=LINE ( 'NONE', #55235, #30335 ) ;
#20308=CARTESIAN_POINT ( 'NONE',  ( -16.39273361182896238, -0.1191753592594177180, 8.116826738503332805 ) ) ;
#20309=DIRECTION ( 'NONE',  ( -0.005002170337468016433, -0.7660444431189770143, 0.6427681459581293666 ) ) ;
#20310=DIRECTION ( 'NONE',  ( 0.007781995580012663651, 0.000000000000000000, -0.9999697198139515519 ) ) ;
#20311=VECTOR ( 'NONE', #47829, 999.9999999999998863 ) ;
#20312=DIRECTION ( 'NONE',  ( -0.7660212471507179544, -0.6427876096865405842, -0.005961354470445141482 ) ) ;
#20313=CARTESIAN_POINT ( 'NONE',  ( -10.39862210783386942, 0.000000000000000000, 1.246168002013329446 ) ) ;
#20314=VERTEX_POINT ( 'NONE', #53893 ) ;
#20316=VECTOR ( 'NONE', #51486, 999.9999999999998863 ) ;
#20317=ORIENTED_EDGE ( 'NONE', *, *, #15158, .F. ) ;
#20318=EDGE_CURVE ( 'NONE', #40480, #20696, #41666, .T. ) ;
#20319=EDGE_CURVE ( 'NONE', #12432, #14535, #2752, .T. ) ;
#20320=CARTESIAN_POINT ( 'NONE',  ( -15.00578141713185332, -1.813211359398156919, 5.486475579755086152 ) ) ;
#20321=CARTESIAN_POINT ( 'NONE',  ( -11.40636015113596180, 0.000000000000000000, 11.32142374880780089 ) ) ;
#20322=CARTESIAN_POINT ( 'NONE',  ( -16.33317936670417225, 0.000000000000000000, 13.31440848639340224 ) ) ;
#20323=LINE ( 'NONE', #10968, #26355 ) ;
#20324=AXIS2_PLACEMENT_3D ( 'NONE', #27162, #5572, #5871 ) ;
#20325=LINE ( 'NONE', #21473, #2336 ) ;
#20326=ADVANCED_FACE ( 'NONE', ( #24927 ), #15014, .F. ) ;
#20327=LINE ( 'NONE', #33408, #49505 ) ;
#20328=ORIENTED_EDGE ( 'NONE', *, *, #50151, .F. ) ;
#20329=EDGE_LOOP ( 'NONE', ( #28614, #24143, #32553, #1277 ) ) ;
#20330=VECTOR ( 'NONE', #54711, 999.9999999999998863 ) ;
#20331=CARTESIAN_POINT ( 'NONE',  ( -23.33693525117809386, 0.000000000000000000, 5.746789908705562944 ) ) ;
#20332=LINE ( 'NONE', #37673, #459 ) ;
#20333=CARTESIAN_POINT ( 'NONE',  ( -11.40636015113596180, 0.000000000000000000, 11.32142374880780089 ) ) ;
#20334=VECTOR ( 'NONE', #24631, 1000.000000000000227 ) ;
#20335=DIRECTION ( 'NONE',  ( 0.000000000000000000, -1.000000000000000000, 0.000000000000000000 ) ) ;
#20336=CARTESIAN_POINT ( 'NONE',  ( -13.60203817727716391, -0.1191753592594181482, 7.769212505853626105 ) ) ;
#20337=FACE_OUTER_BOUND ( 'NONE', #34687, .T. ) ;
#20338=CARTESIAN_POINT ( 'NONE',  ( -13.96589990257885638, 0.000000000000000000, 7.666377821662226033 ) ) ;
#20339=EDGE_CURVE ( 'NONE', #42669, #42711, #45370, .T. ) ;
#20340=VECTOR ( 'NONE', #27130, 999.9999999999998863 ) ;
#20341=VECTOR ( 'NONE', #2787, 999.9999999999998863 ) ;
#20342=DIRECTION ( 'NONE',  ( 0.5364919789714477361, 0.6444004775717706579, 0.5449076811759711036 ) ) ;
#20343=EDGE_CURVE ( 'NONE', #41698, #3615, #30612, .T. ) ;
#20344=FACE_OUTER_BOUND ( 'NONE', #45782, .T. ) ;
#20346=ADVANCED_FACE ( 'NONE', ( #43379 ), #8168, .F. ) ;
#20347=EDGE_CURVE ( 'NONE', #23998, #42364, #51870, .T. ) ;
#20348=AXIS2_PLACEMENT_3D ( 'NONE', #48161, #9010, #17821 ) ;
#20349=ORIENTED_EDGE ( 'NONE', *, *, #32462, .F. ) ;
#20350=VERTEX_POINT ( 'NONE', #47916 ) ;
#20351=ORIENTED_EDGE ( 'NONE', *, *, #52270, .T. ) ;
#20352=EDGE_CURVE ( 'NONE', #55206, #22415, #16980, .T. ) ;
#20353=AXIS2_PLACEMENT_3D ( 'NONE', #18486, #30977, #39222 ) ;
#20356=CARTESIAN_POINT ( 'NONE',  ( -18.29747203306047609, -0.1191753592594177458, 14.03778604627889059 ) ) ;
#20357=EDGE_CURVE ( 'NONE', #44507, #42836, #47065, .T. ) ;
#20358=DIRECTION ( 'NONE',  ( 0.9999697198139515519, 0.000000000000000000, 0.007781995580013368816 ) ) ;
#20359=VECTOR ( 'NONE', #16467, 1000.000000000000227 ) ;
#20360=ORIENTED_EDGE ( 'NONE', *, *, #3610, .F. ) ;
#20361=VERTEX_POINT ( 'NONE', #21783 ) ;
#20362=EDGE_CURVE ( 'NONE', #54876, #46454, #37990, .T. ) ;
#20363=ORIENTED_EDGE ( 'NONE', *, *, #45910, .F. ) ;
#20364=DIRECTION ( 'NONE',  ( 0.007781995580012663651, -3.146120232559066537E-19, -0.9999697198139514409 ) ) ;
#20365=VERTEX_POINT ( 'NONE', #39101 ) ;
#20366=VECTOR ( 'NONE', #183, 999.9999999999998863 ) ;
#20368=VECTOR ( 'NONE', #25908, 1000.000000000000227 ) ;
#20369=DIRECTION ( 'NONE',  ( 0.005961354470445682716, -0.6427876096865404731, -0.7660212471507180654 ) ) ;
#20370=LINE ( 'NONE', #41935, #45886 ) ;
#20371=ORIENTED_EDGE ( 'NONE', *, *, #45500, .F. ) ;
#20372=CARTESIAN_POINT ( 'NONE',  ( -12.99219765192816212, 0.000000000000000000, 1.964648337036805081 ) ) ;
#20373=VERTEX_POINT ( 'NONE', #46791 ) ;
#20374=AXIS2_PLACEMENT_3D ( 'NONE', #30687, #3431, #33798 ) ;
#20375=CARTESIAN_POINT ( 'NONE',  ( -13.19253370888792709, -1.327505506330656893, 3.985022539870387348 ) ) ;
#20376=DIRECTION ( 'NONE',  ( 0.007781995580012663651, -3.146120232559066537E-19, -0.9999697198139514409 ) ) ;
#20377=VECTOR ( 'NONE', #1821, 1000.000000000000114 ) ;
#20378=DIRECTION ( 'NONE',  ( -0.7660212471507179544, -0.6427876096865405842, -0.005961354470445141482 ) ) ;
#20379=AXIS2_PLACEMENT_3D ( 'NONE', #54071, #23669, #48703 ) ;
#20380=DIRECTION ( 'NONE',  ( 0.007781995580012663651, -3.146120232559066537E-19, -0.9999697198139514409 ) ) ;
#20381=LINE ( 'NONE', #3624, #22954 ) ;
#20382=DIRECTION ( 'NONE',  ( 0.6427681459581294776, -0.7660444431189769032, 0.005002170337467562802 ) ) ;
#20383=DIRECTION ( 'NONE',  ( 0.007781995580012663651, 0.000000000000000000, -0.9999697198139515519 ) ) ;
#20384=LINE ( 'NONE', #2510, #4816 ) ;
#20385=ORIENTED_EDGE ( 'NONE', *, *, #20724, .T. ) ;
#20387=ORIENTED_EDGE ( 'NONE', *, *, #45732, .T. ) ;
#20388=ADVANCED_FACE ( 'NONE', ( #51606 ), #34301, .F. ) ;
#20389=DIRECTION ( 'NONE',  ( 0.007781995580012662783, 0.000000000000000000, -0.9999697198139514409 ) ) ;
#20390=DIRECTION ( 'NONE',  ( 0.9999697198139515519, 0.000000000000000000, 0.007781995580013368816 ) ) ;
#20391=DIRECTION ( 'NONE',  ( 0.5449076811759707706, 0.6444004775717708799, -0.5364919789714476250 ) ) ;
#20392=LINE ( 'NONE', #38856, #53053 ) ;
#20393=DIRECTION ( 'NONE',  ( 0.9999697198139515519, 0.000000000000000000, 0.007781995580013368816 ) ) ;
#20394=ADVANCED_FACE ( 'NONE', ( #34013 ), #38547, .F. ) ;
#20395=EDGE_CURVE ( 'NONE', #1256, #34545, #26317, .T. ) ;
#20396=VECTOR ( 'NONE', #3071, 1000.000000000000227 ) ;
#20397=DIRECTION ( 'NONE',  ( -0.9999697198139514409, -0.000000000000000000, -0.007781995580013368816 ) ) ;
#20398=ORIENTED_EDGE ( 'NONE', *, *, #38700, .T. ) ;
#20399=CARTESIAN_POINT ( 'NONE',  ( -18.76354595665420177, -0.1191753592594177458, 14.21882498613976331 ) ) ;
#20400=CARTESIAN_POINT ( 'NONE',  ( -16.94664946618831181, 0.000000000000000000, 6.735190786127661866 ) ) ;
#20401=LINE ( 'NONE', #8467, #30382 ) ;
#20402=LINE ( 'NONE', #51054, #29110 ) ;
#20403=VECTOR ( 'NONE', #40304, 1000.000000000000227 ) ;
#20404=LINE ( 'NONE', #28661, #4236 ) ;
#20405=CARTESIAN_POINT ( 'NONE',  ( 2.072287782118878319, 0.000000000000000000, -2.950529333540147015 ) ) ;
#20406=AXIS2_PLACEMENT_3D ( 'NONE', #45440, #54257, #19051 ) ;
#20407=CARTESIAN_POINT ( 'NONE',  ( -15.80720316891149757, 0.000000000000000000, 5.436055955043602061 ) ) ;
#20408=CARTESIAN_POINT ( 'NONE',  ( -14.79423097067920168, 1.905425754524006532, 2.367720397132919707 ) ) ;
#20409=DIRECTION ( 'NONE',  ( 0.5449076811759707706, 0.6444004775717708799, -0.5364919789714476250 ) ) ;
#20410=EDGE_CURVE ( 'NONE', #40212, #940, #51336, .T. ) ;
#20411=ORIENTED_EDGE ( 'NONE', *, *, #55186, .T. ) ;
#20412=CARTESIAN_POINT ( 'NONE',  ( -16.36111902327085232, -0.1191753592594190780, 4.054420002667924905 ) ) ;
#20413=VECTOR ( 'NONE', #18567, 999.9999999999998863 ) ;
#20414=CARTESIAN_POINT ( 'NONE',  ( 2.072287782118878319, 0.000000000000000000, -2.950529333540147015 ) ) ;
#20415=AXIS2_PLACEMENT_3D ( 'NONE', #55441, #29904, #20548 ) ;
#20416=ORIENTED_EDGE ( 'NONE', *, *, #54945, .T. ) ;
#20418=CARTESIAN_POINT ( 'NONE',  ( -18.29747203306047609, -0.1191753592594177458, 14.03778604627889059 ) ) ;
#20419=FACE_OUTER_BOUND ( 'NONE', #42774, .T. ) ;
#20420=AXIS2_PLACEMENT_3D ( 'NONE', #18746, #19839, #1938 ) ;
#20421=EDGE_LOOP ( 'NONE', ( #5777, #52511, #48845, #35959, #56014, #42692, #1712, #42174, #27998, #27284, #19325, #27420, #6942, #6869, #35203, #22877, #38182, #38616, #29204, #11672, #47463, #53282, #34348, #8724, #27867, #35523, #20634, #10661, #44800, #46924, #42697, #54449, #21760, #18959, #55492, #38613, #6126, #39288, #47321, #33260, #33438, #26976, #45296, #39075, #54280, #22113, #33327, #53664, #10556 ) ) ;
#20422=EDGE_LOOP ( 'NONE', ( #15468, #12611, #40058, #53882 ) ) ;
#20423=CARTESIAN_POINT ( 'NONE',  ( -15.86710544311044302, 0.000000000000000000, 13.13336954653252953 ) ) ;
#20424=EDGE_CURVE ( 'NONE', #40139, #35650, #4206, .T. ) ;
#20425=VECTOR ( 'NONE', #25198, 999.9999999999998863 ) ;
#20426=ORIENTED_EDGE ( 'NONE', *, *, #7163, .F. ) ;
#20427=VECTOR ( 'NONE', #43511, 1000.000000000000227 ) ;
#20428=ORIENTED_EDGE ( 'NONE', *, *, #46989, .T. ) ;
#20430=EDGE_CURVE ( 'NONE', #27953, #52707, #16383, .T. ) ;
#20431=DIRECTION ( 'NONE',  ( 0.000000000000000000, -0.000000000000000000, -1.000000000000000000 ) ) ;
#20432=LINE ( 'NONE', #51389, #36908 ) ;
#20433=CARTESIAN_POINT ( 'NONE',  ( -12.16414003897701690, -0.1134144341942073114, 1.506591511409430817 ) ) ;
#20434=EDGE_LOOP ( 'NONE', ( #9325, #26943, #34352 ) ) ;
#20435=ADVANCED_FACE ( 'NONE', ( #51023 ), #29768, .F. ) ;
#20436=ORIENTED_EDGE ( 'NONE', *, *, #6705, .T. ) ;
#20437=AXIS2_PLACEMENT_3D ( 'NONE', #28874, #37364, #3577 ) ;
#20438=DIRECTION ( 'NONE',  ( 0.000000000000000000, -1.000000000000000000, 0.000000000000000000 ) ) ;
#20439=CARTESIAN_POINT ( 'NONE',  ( -26.13415699229845757, -0.1191753592594197858, 6.933020519852192365 ) ) ;
#20440=VECTOR ( 'NONE', #29387, 1000.000000000000114 ) ;
#20441=ORIENTED_EDGE ( 'NONE', *, *, #9039, .F. ) ;
#20442=CARTESIAN_POINT ( 'NONE',  ( -14.00280974873554030, 0.000000000000000000, 12.40921378708904044 ) ) ;
#20444=AXIS2_PLACEMENT_3D ( 'NONE', #45327, #37653, #32295 ) ;
#20445=FACE_OUTER_BOUND ( 'NONE', #23068, .T. ) ;
#20447=EDGE_CURVE ( 'NONE', #40382, #2633, #12135, .T. ) ;
#20448=EDGE_LOOP ( 'NONE', ( #31883, #33357, #8065, #22340 ) ) ;
#20449=CARTESIAN_POINT ( 'NONE',  ( -18.86354292863559579, 0.000000000000000000, 14.21804678658176080 ) ) ;
#20450=VECTOR ( 'NONE', #51191, 999.9999999999998863 ) ;
#20451=EDGE_CURVE ( 'NONE', #16795, #42240, #38248, .T. ) ;
#20452=CARTESIAN_POINT ( 'NONE',  ( -14.00280974873554030, 0.000000000000000000, 12.40921378708904044 ) ) ;
#20453=VECTOR ( 'NONE', #39227, 999.9999999999998863 ) ;
#20454=AXIS2_PLACEMENT_3D ( 'NONE', #11835, #20916, #3341 ) ;
#20455=ORIENTED_EDGE ( 'NONE', *, *, #43705, .F. ) ;
#20456=CARTESIAN_POINT ( 'NONE',  ( -15.86710544311044302, 0.000000000000000000, 13.13336954653252953 ) ) ;
#20457=LINE ( 'NONE', #27884, #22123 ) ;
#20458=CARTESIAN_POINT ( 'NONE',  ( -15.81869938293262834, 0.000000000000000000, 6.913294768074659480 ) ) ;
#20459=EDGE_CURVE ( 'NONE', #8988, #15552, #30024, .T. ) ;
#20460=VERTEX_POINT ( 'NONE', #25766 ) ;
#20461=VECTOR ( 'NONE', #31669, 999.9999999999998863 ) ;
#20462=VECTOR ( 'NONE', #29303, 1000.000000000000114 ) ;
#20463=ADVANCED_FACE ( 'NONE', ( #17235 ), #10883, .F. ) ;
#20464=DIRECTION ( 'NONE',  ( 0.000000000000000000, -0.000000000000000000, -1.000000000000000000 ) ) ;
#20465=PLANE ( 'NONE',  #31454 ) ;
#20466=DIRECTION ( 'NONE',  ( -0.8531650599175527594, 0.4028455766673922356, 0.3313982828793700652 ) ) ;
#20467=AXIS2_PLACEMENT_3D ( 'NONE', #41450, #11625, #2531 ) ;
#20468=PLANE ( 'NONE',  #34087 ) ;
#20469=LINE ( 'NONE', #15622, #7699 ) ;
#20470=EDGE_CURVE ( 'NONE', #33290, #1300, #15171, .T. ) ;
#20471=CARTESIAN_POINT ( 'NONE',  ( -11.69969505749696559, -0.6798977022406572646, 1.404187704473179865 ) ) ;
#20472=AXIS2_PLACEMENT_3D ( 'NONE', #48139, #39914, #44728 ) ;
#20473=VECTOR ( 'NONE', #25178, 1000.000000000000227 ) ;
#20474=PLANE ( 'NONE',  #34004 ) ;
#20476=LINE ( 'NONE', #24440, #43442 ) ;
#20477=CARTESIAN_POINT ( 'NONE',  ( -14.28874784433092060, 4.010151117816508126, 9.012897199011266736 ) ) ;
#20478=DIRECTION ( 'NONE',  ( 0.007781995580012663651, 0.000000000000000000, -0.9999697198139515519 ) ) ;
#20479=EDGE_LOOP ( 'NONE', ( #51287, #47398, #38098, #14926 ) ) ;
#20480=DIRECTION ( 'NONE',  ( 0.000000000000000000, -1.000000000000000000, 0.000000000000000000 ) ) ;
#20481=DIRECTION ( 'NONE',  ( -0.5364919789714478471, 0.6444004775717705469, -0.5449076811759709926 ) ) ;
#20482=ADVANCED_FACE ( 'NONE', ( #31907 ), #28479, .F. ) ;
#20483=EDGE_CURVE ( 'NONE', #43341, #32707, #53491, .T. ) ;
#20484=LINE ( 'NONE', #41754, #29514 ) ;
#20485=LINE ( 'NONE', #11683, #53251 ) ;
#20486=CARTESIAN_POINT ( 'NONE',  ( -10.84028925556084388, -0.1191753592594197858, 11.14116300850493246 ) ) ;
#20487=AXIS2_PLACEMENT_3D ( 'NONE', #13388, #25309, #35248 ) ;
#20488=EDGE_CURVE ( 'NONE', #49068, #53142, #49223, .T. ) ;
#20489=ORIENTED_EDGE ( 'NONE', *, *, #18771, .F. ) ;
#20490=EDGE_LOOP ( 'NONE', ( #46132, #31966, #2852, #13221 ) ) ;
#20491=DIRECTION ( 'NONE',  ( 0.6427681459581294776, -0.7660444431189769032, 0.005002170337467562802 ) ) ;
#20492=VECTOR ( 'NONE', #16547, 1000.000000000000227 ) ;
#20493=DIRECTION ( 'NONE',  ( 0.6246952433987894571, -0.7422098413412800966, -0.2426528472758541777 ) ) ;
#20495=PLANE ( 'NONE',  #491 ) ;
#20497=ORIENTED_EDGE ( 'NONE', *, *, #54100, .F. ) ;
#20498=DIRECTION ( 'NONE',  ( 0.007781995580012662783, 0.000000000000000000, -0.9999697198139514409 ) ) ;
#20499=VECTOR ( 'NONE', #39174, 1000.000000000000227 ) ;
#20500=VECTOR ( 'NONE', #54318, 1000.000000000000227 ) ;
#20501=ORIENTED_EDGE ( 'NONE', *, *, #35347, .T. ) ;
#20502=ORIENTED_EDGE ( 'NONE', *, *, #23683, .F. ) ;
#20504=DIRECTION ( 'NONE',  ( -0.6427681459581293666, -0.7660444431189770143, -0.005002170337467561935 ) ) ;
#20505=DIRECTION ( 'NONE',  ( 0.005961354470445682716, -0.6427876096865404731, -0.7660212471507180654 ) ) ;
#20506=DIRECTION ( 'NONE',  ( 0.2426528472758542054, 0.7422098413412800966, 0.6246952433987894571 ) ) ;
#20507=VECTOR ( 'NONE', #44218, 999.9999999999998863 ) ;
#20508=VECTOR ( 'NONE', #52706, 1000.000000000000114 ) ;
#20509=PLANE ( 'NONE',  #37541 ) ;
#20510=ADVANCED_FACE ( 'NONE', ( #52452 ), #1539, .F. ) ;
#20511=ORIENTED_EDGE ( 'NONE', *, *, #19157, .T. ) ;
#20512=AXIS2_PLACEMENT_3D ( 'NONE', #52295, #30717, #48017 ) ;
#20513=ORIENTED_EDGE ( 'NONE', *, *, #49438, .F. ) ;
#20514=VECTOR ( 'NONE', #12663, 1000.000000000000000 ) ;
#20515=ORIENTED_EDGE ( 'NONE', *, *, #39592, .T. ) ;
#20516=FACE_OUTER_BOUND ( 'NONE', #14255, .T. ) ;
#20517=FACE_OUTER_BOUND ( 'NONE', #37693, .T. ) ;
#20518=VERTEX_POINT ( 'NONE', #6626 ) ;
#20519=FACE_OUTER_BOUND ( 'NONE', #15563, .T. ) ;
#20520=ORIENTED_EDGE ( 'NONE', *, *, #24450, .F. ) ;
#20521=PLANE ( 'NONE',  #13329 ) ;
#20522=FACE_OUTER_BOUND ( 'NONE', #42413, .T. ) ;
#20523=EDGE_CURVE ( 'NONE', #14352, #52494, #19398, .T. ) ;
#20524=ORIENTED_EDGE ( 'NONE', *, *, #9104, .T. ) ;
#20525=DIRECTION ( 'NONE',  ( 0.000000000000000000, -1.000000000000000000, 0.000000000000000000 ) ) ;
#20526=ORIENTED_EDGE ( 'NONE', *, *, #23411, .T. ) ;
#20527=ADVANCED_FACE ( 'NONE', ( #32488 ), #54054, .F. ) ;
#20528=EDGE_CURVE ( 'NONE', #40640, #49579, #41272, .T. ) ;
#20529=VECTOR ( 'NONE', #4707, 1000.000000000000114 ) ;
#20530=LINE ( 'NONE', #15991, #49136 ) ;
#20531=DIRECTION ( 'NONE',  ( -0.9999697198139514409, -0.000000000000000000, -0.007781995580013368816 ) ) ;
#20532=LINE ( 'NONE', #37018, #20500 ) ;
#20533=DIRECTION ( 'NONE',  ( 0.6427681459581294776, -0.7660444431189769032, 0.005002170337467562802 ) ) ;
#20534=DIRECTION ( 'NONE',  ( 0.000000000000000000, -0.000000000000000000, -1.000000000000000000 ) ) ;
#20535=PLANE ( 'NONE',  #31897 ) ;
#20536=VECTOR ( 'NONE', #16774, 1000.000000000000227 ) ;
#20537=ORIENTED_EDGE ( 'NONE', *, *, #53113, .T. ) ;
#20538=ORIENTED_EDGE ( 'NONE', *, *, #54058, .F. ) ;
#20539=EDGE_CURVE ( 'NONE', #35388, #36770, #2064, .T. ) ;
#20540=DIRECTION ( 'NONE',  ( -0.5449076811759708816, 0.6444004775717707689, 0.5364919789714475140 ) ) ;
#20541=AXIS2_PLACEMENT_3D ( 'NONE', #37757, #33483, #51376 ) ;
#20542=DIRECTION ( 'NONE',  ( -0.005002170337468016433, -0.7660444431189770143, 0.6427681459581293666 ) ) ;
#20543=CARTESIAN_POINT ( 'NONE',  ( -23.33849165029409889, 0.000000000000000000, 5.946783852668351855 ) ) ;
#20544=DIRECTION ( 'NONE',  ( 0.000000000000000000, 1.000000000000000000, 0.000000000000000000 ) ) ;
#20545=EDGE_CURVE ( 'NONE', #23008, #55560, #2363, .T. ) ;
#20546=CARTESIAN_POINT ( 'NONE',  ( -10.00813838035478298, 0.000000000000000000, 10.77830692922518452 ) ) ;
#20547=VECTOR ( 'NONE', #33659, 1000.000000000000227 ) ;
#20548=DIRECTION ( 'NONE',  ( 0.6427681459581294776, -0.7660444431189769032, 0.005002170337467562802 ) ) ;
#20549=ORIENTED_EDGE ( 'NONE', *, *, #3283, .T. ) ;
#20550=LINE ( 'NONE', #7772, #8703 ) ;
#20551=CARTESIAN_POINT ( 'NONE',  ( -30.79411802867772607, 0.000000000000000000, 8.643412946479525516 ) ) ;
#20552=ORIENTED_EDGE ( 'NONE', *, *, #22495, .F. ) ;
#20553=LINE ( 'NONE', #3219, #36802 ) ;
#20554=ORIENTED_EDGE ( 'NONE', *, *, #52554, .F. ) ;
#20555=EDGE_CURVE ( 'NONE', #15522, #35148, #1791, .T. ) ;
#20556=DIRECTION ( 'NONE',  ( 0.6427681459581294776, -0.7660444431189769032, 0.005002170337467562802 ) ) ;
#20557=LINE ( 'NONE', #19973, #29691 ) ;
#20558=VECTOR ( 'NONE', #699, 999.9999999999998863 ) ;
#20559=DIRECTION ( 'NONE',  ( 0.007781995580012662783, 0.000000000000000000, -0.9999697198139514409 ) ) ;
#20560=DIRECTION ( 'NONE',  ( -0.005961354470445682716, -0.6427876096865404731, 0.7660212471507180654 ) ) ;
#20561=VECTOR ( 'NONE', #5925, 999.9999999999998863 ) ;
#20563=ADVANCED_FACE ( 'NONE', ( #19695 ), #5800, .F. ) ;
#20564=ORIENTED_EDGE ( 'NONE', *, *, #33851, .T. ) ;
#20565=VECTOR ( 'NONE', #8545, 999.9999999999998863 ) ;
#20566=ORIENTED_EDGE ( 'NONE', *, *, #1841, .T. ) ;
#20568=CARTESIAN_POINT ( 'NONE',  ( -20.54049170961573267, 0.000000000000000000, 4.660556269540326646 ) ) ;
#20570=DIRECTION ( 'NONE',  ( 0.005961354470445682716, -0.6427876096865404731, -0.7660212471507180654 ) ) ;
#20572=LINE ( 'NONE', #38742, #442 ) ;
#20573=ORIENTED_EDGE ( 'NONE', *, *, #21878, .F. ) ;
#20574=FACE_OUTER_BOUND ( 'NONE', #21061, .T. ) ;
#20575=VECTOR ( 'NONE', #37309, 1000.000000000000114 ) ;
#20576=LINE ( 'NONE', #37897, #22372 ) ;
#20577=DIRECTION ( 'NONE',  ( 0.000000000000000000, -0.000000000000000000, -1.000000000000000000 ) ) ;
#20578=ORIENTED_EDGE ( 'NONE', *, *, #10311, .T. ) ;
#20580=DIRECTION ( 'NONE',  ( -0.5449076811759708816, 0.6444004775717707689, 0.5364919789714475140 ) ) ;
#20581=ADVANCED_FACE ( 'NONE', ( #40451 ), #49525, .F. ) ;
#20582=DIRECTION ( 'NONE',  ( 0.007781995580012663651, 0.000000000000000000, -0.9999697198139515519 ) ) ;
#20583=ORIENTED_EDGE ( 'NONE', *, *, #33568, .F. ) ;
#20584=LINE ( 'NONE', #29374, #29552 ) ;
#20585=VECTOR ( 'NONE', #39657, 1000.000000000000000 ) ;
#20586=ADVANCED_FACE ( 'NONE', ( #36187 ), #27662, .F. ) ;
#20587=ORIENTED_EDGE ( 'NONE', *, *, #30611, .T. ) ;
#20588=ORIENTED_EDGE ( 'NONE', *, *, #1559, .T. ) ;
#20589=VECTOR ( 'NONE', #11477, 1000.000000000000227 ) ;
#20590=EDGE_CURVE ( 'NONE', #33865, #15187, #23404, .T. ) ;
#20591=VERTEX_POINT ( 'NONE', #10642 ) ;
#20592=ADVANCED_FACE ( 'NONE', ( #46338 ), #29324, .F. ) ;
#20593=EDGE_LOOP ( 'NONE', ( #47952, #4297, #16067, #881 ) ) ;
#20594=PLANE ( 'NONE',  #41109 ) ;
#20595=ORIENTED_EDGE ( 'NONE', *, *, #4873, .F. ) ;
#20598=EDGE_CURVE ( 'NONE', #14819, #10694, #37273, .T. ) ;
#20599=ADVANCED_FACE ( 'NONE', ( #42654 ), #20535, .F. ) ;
#20600=VECTOR ( 'NONE', #32353, 1000.000000000000114 ) ;
#20601=ORIENTED_EDGE ( 'NONE', *, *, #47103, .T. ) ;
#20603=ORIENTED_EDGE ( 'NONE', *, *, #51515, .T. ) ;
#20604=EDGE_LOOP ( 'NONE', ( #27177, #27919, #35892, #51531 ) ) ;
#20605=ADVANCED_FACE ( 'NONE', ( #29039 ), #7455, .F. ) ;
#20606=AXIS2_PLACEMENT_3D ( 'NONE', #30347, #39130, #13318 ) ;
#20607=FACE_OUTER_BOUND ( 'NONE', #11567, .T. ) ;
#20610=PLANE ( 'NONE',  #1500 ) ;
#20611=DIRECTION ( 'NONE',  ( -0.9999697198139514409, -0.000000000000000000, -0.007781995580013368816 ) ) ;
#20612=ORIENTED_EDGE ( 'NONE', *, *, #28542, .T. ) ;
#20613=EDGE_LOOP ( 'NONE', ( #19923, #23386, #42165, #41706 ) ) ;
#20614=ADVANCED_FACE ( 'NONE', ( #37863 ), #41549, .F. ) ;
#20615=LINE ( 'NONE', #28558, #15803 ) ;
#20616=CARTESIAN_POINT ( 'NONE',  ( -17.35017059011151375, 1.553641160433663071, 12.97584759397192045 ) ) ;
#20619=CARTESIAN_POINT ( 'NONE',  ( -13.19925735729079719, 0.000000000000000000, 2.871027103731305541 ) ) ;
#20620=EDGE_CURVE ( 'NONE', #54500, #55411, #15996, .T. ) ;
#20621=DIRECTION ( 'NONE',  ( 0.6427681459581294776, -0.7660444431189769032, 0.005002170337467562802 ) ) ;
#20622=FACE_OUTER_BOUND ( 'NONE', #38758, .T. ) ;
#20623=ORIENTED_EDGE ( 'NONE', *, *, #15867, .T. ) ;
#20624=DIRECTION ( 'NONE',  ( 0.000000000000000000, -0.000000000000000000, -1.000000000000000000 ) ) ;
#20625=CARTESIAN_POINT ( 'NONE',  ( -18.86354292863559579, 0.000000000000000000, 14.21804678658176080 ) ) ;
#20626=ORIENTED_EDGE ( 'NONE', *, *, #13299, .F. ) ;
#20627=ADVANCED_FACE ( 'NONE', ( #54576 ), #21073, .F. ) ;
#20628=FACE_OUTER_BOUND ( 'NONE', #24717, .T. ) ;
#20629=DIRECTION ( 'NONE',  ( 0.7660212471507180654, -0.6427876096865404731, 0.005961354470445141482 ) ) ;
#20630=PLANE ( 'NONE',  #1825 ) ;
#20631=CARTESIAN_POINT ( 'NONE',  ( -16.01450161900085689, 0.000000000000000000, 6.373112906405917322 ) ) ;
#20632=LINE ( 'NONE', #46168, #54933 ) ;
#20633=AXIS2_PLACEMENT_3D ( 'NONE', #16635, #16346, #32833 ) ;
#20634=ORIENTED_EDGE ( 'NONE', *, *, #3742, .F. ) ;
#20635=VERTEX_POINT ( 'NONE', #42094 ) ;
#20636=PLANE ( 'NONE',  #14883 ) ;
#20637=DIRECTION ( 'NONE',  ( -0.5449076811759708816, 0.6444004775717707689, 0.5364919789714475140 ) ) ;
#20639=VECTOR ( 'NONE', #24859, 999.9999999999998863 ) ;
#20640=DIRECTION ( 'NONE',  ( 0.007781995580012663651, -3.146120232559066537E-19, -0.9999697198139514409 ) ) ;
#20641=LINE ( 'NONE', #33675, #36652 ) ;
#20642=LINE ( 'NONE', #34270, #1966 ) ;
#20643=CARTESIAN_POINT ( 'NONE',  ( -6.599926418471779854, -8.445284758064715902, 5.782009131042851635 ) ) ;
#20644=LINE ( 'NONE', #47037, #16892 ) ;
#20645=LINE ( 'NONE', #12416, #28732 ) ;
#20646=DIRECTION ( 'NONE',  ( 0.5364919789714477361, 0.6444004775717706579, 0.5449076811759711036 ) ) ;
#20647=EDGE_LOOP ( 'NONE', ( #9123, #31685, #29139 ) ) ;
#20648=FACE_OUTER_BOUND ( 'NONE', #42720, .T. ) ;
#20649=ORIENTED_EDGE ( 'NONE', *, *, #635, .T. ) ;
#20650=ADVANCED_FACE ( 'NONE', ( #16840 ), #12578, .F. ) ;
#20651=ORIENTED_EDGE ( 'NONE', *, *, #32486, .T. ) ;
#20652=VERTEX_POINT ( 'NONE', #55431 ) ;
#20653=ORIENTED_EDGE ( 'NONE', *, *, #50713, .T. ) ;
#20654=ORIENTED_EDGE ( 'NONE', *, *, #50063, .F. ) ;
#20655=LINE ( 'NONE', #7290, #14217 ) ;
#20656=LINE ( 'NONE', #54427, #13866 ) ;
#20657=CARTESIAN_POINT ( 'NONE',  ( -18.67775241435682432, 0.000000000000000000, 4.136394454059623804 ) ) ;
#20658=EDGE_CURVE ( 'NONE', #8289, #713, #25351, .T. ) ;
#20659=EDGE_CURVE ( 'NONE', #34052, #54291, #16532, .T. ) ;
#20660=EDGE_CURVE ( 'NONE', #32666, #31029, #41805, .T. ) ;
#20661=VERTEX_POINT ( 'NONE', #7190 ) ;
#20662=PLANE ( 'NONE',  #14103 ) ;
#20663=VERTEX_POINT ( 'NONE', #2898 ) ;
#20665=EDGE_CURVE ( 'NONE', #10496, #32467, #51184, .T. ) ;
#20668=LINE ( 'NONE', #37984, #50947 ) ;
#20670=ORIENTED_EDGE ( 'NONE', *, *, #6136, .T. ) ;
#20671=CARTESIAN_POINT ( 'NONE',  ( -22.40478740399063895, 0.000000000000000000, 5.384712028983816623 ) ) ;
#20672=ORIENTED_EDGE ( 'NONE', *, *, #54889, .F. ) ;
#20673=VECTOR ( 'NONE', #49983, 1000.000000000000227 ) ;
#20674=DIRECTION ( 'NONE',  ( -0.5364919789714478471, 0.6444004775717705469, -0.5449076811759709926 ) ) ;
#20675=CARTESIAN_POINT ( 'NONE',  ( -30.79411802867772607, 0.000000000000000000, 8.643412946479525516 ) ) ;
#20676=EDGE_CURVE ( 'NONE', #9163, #37975, #16257, .T. ) ;
#20677=CARTESIAN_POINT ( 'NONE',  ( -17.69029958343410769, 0.000000000000000000, 8.576063877996469742 ) ) ;
#20678=PLANE ( 'NONE',  #34043 ) ;
#20680=CARTESIAN_POINT ( 'NONE',  ( -15.53106400201207116, 0.000000000000000000, 3.960876654664550411 ) ) ;
#20681=ADVANCED_FACE ( 'NONE', ( #33578 ), #55725, .F. ) ;
#20682=LINE ( 'NONE', #42535, #28470 ) ;
#20684=ORIENTED_EDGE ( 'NONE', *, *, #11182, .T. ) ;
#20686=ORIENTED_EDGE ( 'NONE', *, *, #49664, .T. ) ;
#20687=ADVANCED_FACE ( 'NONE', ( #44070 ), #634, .F. ) ;
#20688=FACE_OUTER_BOUND ( 'NONE', #25757, .T. ) ;
#20689=DIRECTION ( 'NONE',  ( 0.9999697198139515519, 0.000000000000000000, 0.007781995580013368816 ) ) ;
#20690=LINE ( 'NONE', #16402, #15957 ) ;
#20691=PLANE ( 'NONE',  #6803 ) ;
#20692=CARTESIAN_POINT ( 'NONE',  ( -12.64297938670245536, 4.333955019861511992, 1.454618426794188402 ) ) ;
#20693=EDGE_CURVE ( 'NONE', #11344, #3168, #17670, .T. ) ;
#20694=DIRECTION ( 'NONE',  ( 0.007781995580012663651, -3.146120232559066537E-19, -0.9999697198139514409 ) ) ;
#20696=VERTEX_POINT ( 'NONE', #21911 ) ;
#20697=LINE ( 'NONE', #16409, #42819 ) ;
#20698=DIRECTION ( 'NONE',  ( 0.000000000000000000, -1.000000000000000000, 0.000000000000000000 ) ) ;
#20699=CARTESIAN_POINT ( 'NONE',  ( -11.79672450625168878, 0.000000000000000000, 1.773945729262041748 ) ) ;
#20700=CARTESIAN_POINT ( 'NONE',  ( -19.60990026154428278, 0.000000000000000000, 4.498472333781370125 ) ) ;
#20702=DIRECTION ( 'NONE',  ( 0.6427681459581294776, -0.7660444431189769032, 0.005002170337467562802 ) ) ;
#20703=CARTESIAN_POINT ( 'NONE',  ( -9.808144436391993182, 0.000000000000000000, 10.77986332834118777 ) ) ;
#20705=ORIENTED_EDGE ( 'NONE', *, *, #15191, .T. ) ;
#20706=DIRECTION ( 'NONE',  ( -0.6427681459581293666, -0.7660444431189770143, -0.005002170337467561935 ) ) ;
#20708=ORIENTED_EDGE ( 'NONE', *, *, #31040, .F. ) ;
#20709=ORIENTED_EDGE ( 'NONE', *, *, #16802, .T. ) ;
#20710=DIRECTION ( 'NONE',  ( -0.9999697198139514409, -0.000000000000000000, -0.007781995580013368816 ) ) ;
#20711=AXIS2_PLACEMENT_3D ( 'NONE', #47018, #12930, #42735 ) ;
#20712=ORIENTED_EDGE ( 'NONE', *, *, #31844, .F. ) ;
#20713=ORIENTED_EDGE ( 'NONE', *, *, #41083, .F. ) ;
#20714=PLANE ( 'NONE',  #8419 ) ;
#20715=EDGE_LOOP ( 'NONE', ( #30555, #15642, #23461, #6752 ) ) ;
#20716=ORIENTED_EDGE ( 'NONE', *, *, #47724, .T. ) ;
#20717=ORIENTED_EDGE ( 'NONE', *, *, #46106, .F. ) ;
#20718=LINE ( 'NONE', #26879, #14882 ) ;
#20719=DIRECTION ( 'NONE',  ( 0.6427681459581294776, -0.7660444431189769032, 0.005002170337467562802 ) ) ;
#20720=PLANE ( 'NONE',  #4047 ) ;
#20721=ADVANCED_FACE ( 'NONE', ( #21659 ), #30469, .F. ) ;
#20722=EDGE_LOOP ( 'NONE', ( #29389, #44315, #33494, #23800 ) ) ;
#20723=ORIENTED_EDGE ( 'NONE', *, *, #37142, .T. ) ;
#20724=EDGE_CURVE ( 'NONE', #22478, #21969, #35279, .T. ) ;
#20725=EDGE_CURVE ( 'NONE', #42368, #45163, #13674, .T. ) ;
#20726=CARTESIAN_POINT ( 'NONE',  ( -20.37261732798432945, 4.657758921906512306, 4.446741263022703450 ) ) ;
#20727=FACE_OUTER_BOUND ( 'NONE', #44166, .T. ) ;
#20728=EDGE_LOOP ( 'NONE', ( #19240, #7179, #24646, #25737 ) ) ;
#20729=DIRECTION ( 'NONE',  ( 0.9999697198139515519, 0.000000000000000000, 0.007781995580013368816 ) ) ;
#20730=ORIENTED_EDGE ( 'NONE', *, *, #8109, .F. ) ;
#20731=CARTESIAN_POINT ( 'NONE',  ( 2.072287782118878319, 0.000000000000000000, -2.950529333540147015 ) ) ;
#20732=DIRECTION ( 'NONE',  ( -0.5449076811759708816, 0.6444004775717707689, 0.5364919789714475140 ) ) ;
#20733=EDGE_LOOP ( 'NONE', ( #4905, #40175, #5212, #36053 ) ) ;
#20734=CARTESIAN_POINT ( 'NONE',  ( -24.26986129792355129, -0.1191753592594197858, 6.208864760408702388 ) ) ;
#20735=CARTESIAN_POINT ( 'NONE',  ( -12.23851102634202448, -0.1191753592594197858, 11.68427982808754884 ) ) ;
#20736=ORIENTED_EDGE ( 'NONE', *, *, #46863, .T. ) ;
#20737=CARTESIAN_POINT ( 'NONE',  ( -11.63121920435228951, 0.000000000000000000, 6.207218567471217696 ) ) ;
#20738=LINE ( 'NONE', #42863, #2055 ) ;
#20739=CARTESIAN_POINT ( 'NONE',  ( 2.072287782118878319, 0.000000000000000000, -2.950529333540147015 ) ) ;
#20740=DIRECTION ( 'NONE',  ( 0.9999697198139515519, 0.000000000000000000, 0.007781995580013368816 ) ) ;
#20741=ORIENTED_EDGE ( 'NONE', *, *, #55093, .F. ) ;
#20742=AXIS2_PLACEMENT_3D ( 'NONE', #3764, #8311, #25939 ) ;
#20743=PLANE ( 'NONE',  #35550 ) ;
#20744=DIRECTION ( 'NONE',  ( -0.9999697198139514409, -0.000000000000000000, -0.007781995580013368816 ) ) ;
#20745=DIRECTION ( 'NONE',  ( -0.005002170337468016433, -0.7660444431189770143, 0.6427681459581293666 ) ) ;
#20746=DIRECTION ( 'NONE',  ( 0.9999697198139515519, 0.000000000000000000, 0.007781995580013368816 ) ) ;
#20747=EDGE_CURVE ( 'NONE', #25299, #3665, #34698, .T. ) ;
#20748=FACE_OUTER_BOUND ( 'NONE', #31735, .T. ) ;
#20749=CARTESIAN_POINT ( 'NONE',  ( -13.53673582514181106, 0.000000000000000000, 12.22817484722816772 ) ) ;
#20751=ORIENTED_EDGE ( 'NONE', *, *, #29487, .F. ) ;
#20752=DIRECTION ( 'NONE',  ( 0.5449076811759707706, 0.6444004775717708799, -0.5364919789714476250 ) ) ;
#20753=EDGE_CURVE ( 'NONE', #47842, #47452, #47194, .T. ) ;
#20754=CARTESIAN_POINT ( 'NONE',  ( -13.23414441016926801, -0.8417996532631562001, 1.995054423283073586 ) ) ;
#20755=ORIENTED_EDGE ( 'NONE', *, *, #49876, .F. ) ;
#20756=DIRECTION ( 'NONE',  ( -0.7660212471507179544, -0.6427876096865405842, -0.005961354470445141482 ) ) ;
#20757=LINE ( 'NONE', #51430, #13667 ) ;
#20758=EDGE_CURVE ( 'NONE', #48862, #41291, #8892, .T. ) ;
#20759=PLANE ( 'NONE',  #53056 ) ;
#20760=CARTESIAN_POINT ( 'NONE',  ( -15.13495153988577968, 0.000000000000000000, 12.76973526769478084 ) ) ;
#20761=DIRECTION ( 'NONE',  ( -0.005961354470445682716, -0.6427876096865404731, 0.7660212471507180654 ) ) ;
#20762=ORIENTED_EDGE ( 'NONE', *, *, #44510, .F. ) ;
#20764=CARTESIAN_POINT ( 'NONE',  ( -19.82770700041984924, 4.010151117816509903, 4.255741666113602939 ) ) ;
#20765=PLANE ( 'NONE',  #27721 ) ;
#20766=LINE ( 'NONE', #3710, #55628 ) ;
#20767=VERTEX_POINT ( 'NONE', #4048 ) ;
#20768=CARTESIAN_POINT ( 'NONE',  ( -17.66730715539184615, 0.000000000000000000, 5.621586251934354017 ) ) ;
#20769=EDGE_LOOP ( 'NONE', ( #31258, #37887, #29806, #46995 ) ) ;
#20770=CARTESIAN_POINT ( 'NONE',  ( -14.56888064431065821, -0.1191753592594197858, 12.58947452739191064 ) ) ;
#20771=ORIENTED_EDGE ( 'NONE', *, *, #48333, .T. ) ;
#20772=EDGE_LOOP ( 'NONE', ( #46841, #8074, #27309, #19167 ) ) ;
#20773=ORIENTED_EDGE ( 'NONE', *, *, #45738, .F. ) ;
#20774=CARTESIAN_POINT ( 'NONE',  ( -13.63673279712320507, -0.1191753592594197858, 12.22739664767016521 ) ) ;
#20775=EDGE_CURVE ( 'NONE', #17655, #30132, #26196, .T. ) ;
#20776=CARTESIAN_POINT ( 'NONE',  ( -17.74560456716937296, 0.000000000000000000, 3.774316574337878372 ) ) ;
#20777=PLANE ( 'NONE',  #1278 ) ;
#20779=CARTESIAN_POINT ( 'NONE',  ( -14.56888064431065821, -0.1191753592594197858, 12.58947452739191064 ) ) ;
#20780=ORIENTED_EDGE ( 'NONE', *, *, #48203, .T. ) ;
#20781=ADVANCED_FACE ( 'NONE', ( #21378 ), #38709, .F. ) ;
#20782=ORIENTED_EDGE ( 'NONE', *, *, #53335, .T. ) ;
#20783=ORIENTED_EDGE ( 'NONE', *, *, #32584, .F. ) ;
#20784=DIRECTION ( 'NONE',  ( 0.007781995580012663651, 0.000000000000000000, -0.9999697198139515519 ) ) ;
#20785=CARTESIAN_POINT ( 'NONE',  ( -24.27063949748155380, 0.000000000000000000, 6.308861732390097288 ) ) ;
#20786=ORIENTED_EDGE ( 'NONE', *, *, #5022, .F. ) ;
#20787=CARTESIAN_POINT ( 'NONE',  ( 1.969897575278193980, 0.000000000000000000, 10.20639235748909890 ) ) ;
#20788=ORIENTED_EDGE ( 'NONE', *, *, #31094, .F. ) ;
#20789=DIRECTION ( 'NONE',  ( 0.9999697198139515519, 0.000000000000000000, 0.007781995580013368816 ) ) ;
#20790=DIRECTION ( 'NONE',  ( 0.000000000000000000, -0.000000000000000000, -1.000000000000000000 ) ) ;
#20791=ORIENTED_EDGE ( 'NONE', *, *, #50697, .F. ) ;
#20792=LINE ( 'NONE', #3480, #19522 ) ;
#20793=EDGE_LOOP ( 'NONE', ( #38166, #23178, #26823 ) ) ;
#20794=EDGE_CURVE ( 'NONE', #12574, #49826, #9138, .T. ) ;
#20795=CARTESIAN_POINT ( 'NONE',  ( -12.33850799832341849, 0.000000000000000000, 11.68350162852954632 ) ) ;
#20797=ORIENTED_EDGE ( 'NONE', *, *, #19807, .F. ) ;
#20798=DIRECTION ( 'NONE',  ( 0.9999697198139515519, 0.000000000000000000, 0.007781995580013368816 ) ) ;
#20799=DIRECTION ( 'NONE',  ( 0.007781995580012663651, -3.146120232559066537E-19, -0.9999697198139514409 ) ) ;
#20800=DIRECTION ( 'NONE',  ( -0.5364919789714478471, 0.6444004775717705469, -0.5449076811759709926 ) ) ;
#20801=DIRECTION ( 'NONE',  ( 0.007781995580012662783, 0.000000000000000000, -0.9999697198139514409 ) ) ;
#20802=ORIENTED_EDGE ( 'NONE', *, *, #37964, .T. ) ;
#20803=ORIENTED_EDGE ( 'NONE', *, *, #39241, .T. ) ;
#20804=LINE ( 'NONE', #37868, #42755 ) ;
#20805=DIRECTION ( 'NONE',  ( -0.005002170337468016433, -0.7660444431189770143, 0.6427681459581293666 ) ) ;
#20806=CARTESIAN_POINT ( 'NONE',  ( -17.11479534437067329, 0.7721120973665037690, 4.796456341994528749 ) ) ;
#20807=FACE_OUTER_BOUND ( 'NONE', #13530, .T. ) ;
#20808=DIRECTION ( 'NONE',  ( 0.9999697198139515519, 0.000000000000000000, 0.007781995580013368816 ) ) ;
#20809=CARTESIAN_POINT ( 'NONE',  ( -13.24198947131226944, 0.000000000000000000, 8.362011986176833389 ) ) ;
#20810=ORIENTED_EDGE ( 'NONE', *, *, #1876, .T. ) ;
#20811=DIRECTION ( 'NONE',  ( 0.5449076811759707706, 0.6444004775717708799, -0.5364919789714476250 ) ) ;
#20812=PLANE ( 'NONE',  #3262 ) ;
#20813=ORIENTED_EDGE ( 'NONE', *, *, #22192, .F. ) ;
#20814=CARTESIAN_POINT ( 'NONE',  ( -29.86352658060627618, 0.000000000000000000, 8.481329010720569883 ) ) ;
#20815=EDGE_LOOP ( 'NONE', ( #24736, #25527, #34208, #14314 ) ) ;
#20816=CARTESIAN_POINT ( 'NONE',  ( -9.292346798231170268, 0.000000000000000000, 4.209433850727466009 ) ) ;
#20817=CARTESIAN_POINT ( 'NONE',  ( -8.975993561185934055, -0.1191753592594197858, 10.41700724906143982 ) ) ;
#20818=EDGE_CURVE ( 'NONE', #39737, #31756, #4884, .T. ) ;
#20819=DIRECTION ( 'NONE',  ( 0.007781995580012663651, 0.000000000000000000, -0.9999697198139515519 ) ) ;
#20820=FACE_OUTER_BOUND ( 'NONE', #6155, .T. ) ;
#20822=EDGE_LOOP ( 'NONE', ( #48302, #24925, #21258, #22271 ) ) ;
#20823=ORIENTED_EDGE ( 'NONE', *, *, #35511, .T. ) ;
#20824=DIRECTION ( 'NONE',  ( 0.005002170337468016433, -0.7660444431189770143, -0.6427681459581293666 ) ) ;
#20825=FACE_OUTER_BOUND ( 'NONE', #32523, .T. ) ;
#20826=LINE ( 'NONE', #23971, #1580 ) ;
#20827=EDGE_CURVE ( 'NONE', #46599, #36877, #18210, .T. ) ;
#20828=DIRECTION ( 'NONE',  ( 0.007781995580012663651, 0.000000000000000000, -0.9999697198139515519 ) ) ;
#20829=LINE ( 'NONE', #52355, #43718 ) ;
#20830=DIRECTION ( 'NONE',  ( 0.8531650599175527594, 0.4028455766673922356, -0.3313982828793700652 ) ) ;
#20831=EDGE_LOOP ( 'NONE', ( #1594, #49528, #36810, #18915, #13186 ) ) ;
#20832=EDGE_CURVE ( 'NONE', #36873, #33080, #26744, .T. ) ;
#20833=DIRECTION ( 'NONE',  ( 0.5449076811759707706, 0.6444004775717708799, -0.5364919789714476250 ) ) ;
#20834=EDGE_CURVE ( 'NONE', #32724, #6604, #30986, .T. ) ;
#20835=FACE_OUTER_BOUND ( 'NONE', #54424, .T. ) ;
#20836=CARTESIAN_POINT ( 'NONE',  ( -10.44017651129710700, 0.000000000000000000, 6.585819606917006297 ) ) ;
#20837=VERTEX_POINT ( 'NONE', #35538 ) ;
#20838=DIRECTION ( 'NONE',  ( 0.7660212471507180654, -0.6427876096865404731, 0.005961354470445141482 ) ) ;
#20839=EDGE_CURVE ( 'NONE', #33297, #46700, #25617, .T. ) ;
#20840=LINE ( 'NONE', #37610, #42241 ) ;
#20841=CARTESIAN_POINT ( 'NONE',  ( -9.808144436391993182, 0.000000000000000000, 10.77986332834118777 ) ) ;
#20842=ORIENTED_EDGE ( 'NONE', *, *, #31578, .F. ) ;
#20844=ADVANCED_FACE ( 'NONE', ( #34427 ), #51733, .F. ) ;
#20845=VERTEX_POINT ( 'NONE', #6555 ) ;
#20846=EDGE_CURVE ( 'NONE', #17974, #8156, #44344, .T. ) ;
#20847=VECTOR ( 'NONE', #21235, 999.9999999999998863 ) ;
#20848=ORIENTED_EDGE ( 'NONE', *, *, #11355, .F. ) ;
#20849=ORIENTED_EDGE ( 'NONE', *, *, #47304, .T. ) ;
#20850=ORIENTED_EDGE ( 'NONE', *, *, #40969, .T. ) ;
#20851=DIRECTION ( 'NONE',  ( -0.7660212471507179544, -0.6427876096865405842, -0.005961354470445141482 ) ) ;
#20852=ORIENTED_EDGE ( 'NONE', *, *, #17574, .F. ) ;
#20853=DIRECTION ( 'NONE',  ( 0.005961354470445682716, -0.6427876096865404731, -0.7660212471507180654 ) ) ;
#20854=EDGE_CURVE ( 'NONE', #34036, #43311, #5724, .T. ) ;
#20855=ORIENTED_EDGE ( 'NONE', *, *, #20424, .F. ) ;
#20856=DIRECTION ( 'NONE',  ( -0.005961354470445682716, -0.6427876096865404731, 0.7660212471507180654 ) ) ;
#20857=EDGE_LOOP ( 'NONE', ( #12937, #47713, #52225, #26363 ) ) ;
#20858=ORIENTED_EDGE ( 'NONE', *, *, #19785, .T. ) ;
#20859=EDGE_CURVE ( 'NONE', #33755, #1256, #31287, .T. ) ;
#20860=LINE ( 'NONE', #4406, #13874 ) ;
#20861=DIRECTION ( 'NONE',  ( 0.000000000000000000, -0.000000000000000000, -1.000000000000000000 ) ) ;
#20862=CARTESIAN_POINT ( 'NONE',  ( -10.94028622754223967, 0.000000000000000000, 11.14038480894692995 ) ) ;
#20863=DIRECTION ( 'NONE',  ( 0.000000000000000000, -0.000000000000000000, -1.000000000000000000 ) ) ;
#20864=ORIENTED_EDGE ( 'NONE', *, *, #55791, .F. ) ;
#20865=ORIENTED_EDGE ( 'NONE', *, *, #15340, .F. ) ;
#20866=CARTESIAN_POINT ( 'NONE',  ( -18.66354898467281132, 0.000000000000000000, 14.21960318569776582 ) ) ;
#20868=FACE_OUTER_BOUND ( 'NONE', #9645, .T. ) ;
#20869=LINE ( 'NONE', #29965, #11288 ) ;
#20870=PLANE ( 'NONE',  #40380 ) ;
#20871=LINE ( 'NONE', #43028, #39562 ) ;
#20872=ORIENTED_EDGE ( 'NONE', *, *, #13124, .T. ) ;
#20873=LINE ( 'NONE', #25170, #41056 ) ;
#20874=LINE ( 'NONE', #42189, #30391 ) ;
#20875=ORIENTED_EDGE ( 'NONE', *, *, #15714, .F. ) ;
#20876=DIRECTION ( 'NONE',  ( 0.005961354470445682716, -0.6427876096865404731, -0.7660212471507180654 ) ) ;
#20877=LINE ( 'NONE', #51280, #20547 ) ;
#20878=LINE ( 'NONE', #46427, #30864 ) ;
#20879=ADVANCED_FACE ( 'NONE', ( #36960 ), #28132, .F. ) ;
#20880=CARTESIAN_POINT ( 'NONE',  ( -13.27065584551087163, 0.000000000000000000, 12.04557950825129176 ) ) ;
#20881=CARTESIAN_POINT ( 'NONE',  ( -16.80850742758478233, 3.686347215771509145, 9.460240024641782597 ) ) ;
#20882=AXIS2_PLACEMENT_3D ( 'NONE', #53571, #22645, #31999 ) ;
#20883=ORIENTED_EDGE ( 'NONE', *, *, #8016, .T. ) ;
#20884=VERTEX_POINT ( 'NONE', #27885 ) ;
#20885=LINE ( 'NONE', #29128, #6736 ) ;
#20887=LINE ( 'NONE', #38209, #4305 ) ;
#20888=EDGE_CURVE ( 'NONE', #22464, #51166, #40371, .T. ) ;
#20889=DIRECTION ( 'NONE',  ( 0.9999697198139515519, 0.000000000000000000, 0.007781995580013368816 ) ) ;
#20890=PLANE ( 'NONE',  #33932 ) ;
#20891=LINE ( 'NONE', #16350, #1047 ) ;
#20892=CARTESIAN_POINT ( 'NONE',  ( -15.81007722241678159, 0.000000000000000000, 5.805365658301368192 ) ) ;
#20893=EDGE_CURVE ( 'NONE', #30294, #55101, #48891, .T. ) ;
#20894=LINE ( 'NONE', #38218, #42298 ) ;
#20897=CARTESIAN_POINT ( 'NONE',  ( -14.01545677930355183, 0.000000000000000000, 2.126011111488108174 ) ) ;
#20898=EDGE_LOOP ( 'NONE', ( #43354, #52489, #230, #499 ) ) ;
#20899=CARTESIAN_POINT ( 'NONE',  ( -24.27063949748155380, 0.000000000000000000, 6.308861732390097288 ) ) ;
#20901=EDGE_CURVE ( 'NONE', #23998, #35256, #48615, .T. ) ;
#20902=EDGE_LOOP ( 'NONE', ( #9252, #10984, #21725, #47211 ) ) ;
#20903=EDGE_CURVE ( 'NONE', #44587, #4593, #18497, .T. ) ;
#20904=VERTEX_POINT ( 'NONE', #10261 ) ;
#20905=ORIENTED_EDGE ( 'NONE', *, *, #42469, .F. ) ;
#20906=ORIENTED_EDGE ( 'NONE', *, *, #30357, .F. ) ;
#20907=EDGE_LOOP ( 'NONE', ( #1253, #7649, #55699, #13950 ) ) ;
#20908=CARTESIAN_POINT ( 'NONE',  ( -17.42565663055581382, 0.000000000000000000, 8.578123390648475066 ) ) ;
#20909=CARTESIAN_POINT ( 'NONE',  ( -18.67619601524082285, 0.000000000000000000, 3.936400510096834893 ) ) ;
#20910=CARTESIAN_POINT ( 'NONE',  ( -13.02886805270398618, 4.172053068839010059, 8.789225786196009693 ) ) ;
#20911=ADVANCED_FACE ( 'NONE', ( #23869 ), #27586, .F. ) ;
#20912=AXIS2_PLACEMENT_3D ( 'NONE', #31835, #49146, #27581 ) ;
#20914=CARTESIAN_POINT ( 'NONE',  ( -20.16176772743538237, -0.1191753592594197858, 14.76194180572237968 ) ) ;
#20915=ORIENTED_EDGE ( 'NONE', *, *, #45591, .T. ) ;
#20916=DIRECTION ( 'NONE',  ( 0.000000000000000000, -1.000000000000000000, 0.000000000000000000 ) ) ;
#20917=ORIENTED_EDGE ( 'NONE', *, *, #16007, .T. ) ;
#20918=VECTOR ( 'NONE', #42348, 1000.000000000000227 ) ;
#20920=LINE ( 'NONE', #7591, #50011 ) ;
#20921=DIRECTION ( 'NONE',  ( 0.9321478471874540261, 0.000000000000000000, -0.3620778797217456546 ) ) ;
#20922=ORIENTED_EDGE ( 'NONE', *, *, #45357, .T. ) ;
#20923=DIRECTION ( 'NONE',  ( 0.000000000000000000, -0.000000000000000000, -1.000000000000000000 ) ) ;
#20924=ORIENTED_EDGE ( 'NONE', *, *, #1866, .F. ) ;
#20925=DIRECTION ( 'NONE',  ( 0.9999697198139515519, 0.000000000000000000, 0.007781995580013368816 ) ) ;
#20926=CARTESIAN_POINT ( 'NONE',  ( -13.63673279712320507, -0.1191753592594197858, 12.22739664767016521 ) ) ;
#20927=CARTESIAN_POINT ( 'NONE',  ( -13.73672976910459909, 0.000000000000000000, 12.22661844811216270 ) ) ;
#20928=CARTESIAN_POINT ( 'NONE',  ( -23.33849165029409889, 0.000000000000000000, 5.946783852668351855 ) ) ;
#20929=DIRECTION ( 'NONE',  ( 0.007781995580012662783, 0.000000000000000000, -0.9999697198139514409 ) ) ;
#20931=PLANE ( 'NONE',  #3996 ) ;
#20932=CARTESIAN_POINT ( 'NONE',  ( -21.47419595591918906, 0.000000000000000000, 5.222628093224860102 ) ) ;
#20933=ORIENTED_EDGE ( 'NONE', *, *, #38878, .T. ) ;
#20934=LINE ( 'NONE', #34867, #42869 ) ;
#20935=ORIENTED_EDGE ( 'NONE', *, *, #4326, .F. ) ;
#20936=EDGE_CURVE ( 'NONE', #5490, #20845, #9727, .T. ) ;
#20937=AXIS2_PLACEMENT_3D ( 'NONE', #10213, #51366, #42553 ) ;
#20938=VECTOR ( 'NONE', #47115, 999.9999999999998863 ) ;
#20939=DIRECTION ( 'NONE',  ( 0.5364919789714477361, 0.6444004775717706579, 0.5449076811759711036 ) ) ;
#20940=CARTESIAN_POINT ( 'NONE',  ( -12.15193928448667116, -0.1191753592594194527, 1.501852324026011987 ) ) ;
#20941=CARTESIAN_POINT ( 'NONE',  ( -20.19028461120871754, -5.698858183938165567, 13.87732110161523202 ) ) ;
#20942=EDGE_CURVE ( 'NONE', #36489, #34036, #40074, .T. ) ;
#20943=DIRECTION ( 'NONE',  ( 0.007781995580012663651, -3.146120232559066537E-19, -0.9999697198139514409 ) ) ;
#20944=FACE_OUTER_BOUND ( 'NONE', #52398, .T. ) ;
#20945=LINE ( 'NONE', #29491, #16514 ) ;
#20947=ORIENTED_EDGE ( 'NONE', *, *, #8469, .T. ) ;
#20948=ADVANCED_FACE ( 'NONE', ( #53686 ), #23594, .F. ) ;
#20950=CARTESIAN_POINT ( 'NONE',  ( -17.93139508144814442, 0.000000000000000000, 13.85596890686001537 ) ) ;
#20951=LINE ( 'NONE', #54757, #6464 ) ;
#20952=EDGE_CURVE ( 'NONE', #13781, #53854, #53980, .T. ) ;
#20953=EDGE_CURVE ( 'NONE', #12359, #15460, #53164, .T. ) ;
#20954=EDGE_CURVE ( 'NONE', #37711, #40517, #32128, .T. ) ;
#20955=VECTOR ( 'NONE', #23267, 999.9999999999998863 ) ;
#20956=CARTESIAN_POINT ( 'NONE',  ( -19.12962290826653700, 0.000000000000000000, 14.40064212555863854 ) ) ;
#20957=PLANE ( 'NONE',  #7617 ) ;
#20958=CARTESIAN_POINT ( 'NONE',  ( 2.072287782118878319, 0.000000000000000000, -2.950529333540147015 ) ) ;
#20959=CARTESIAN_POINT ( 'NONE',  ( -16.74767181305720953, -0.03228989815065406305, 3.385655385894552616 ) ) ;
#20960=ORIENTED_EDGE ( 'NONE', *, *, #42029, .F. ) ;
#20961=AXIS2_PLACEMENT_3D ( 'NONE', #10209, #5973, #23292 ) ;
#20962=CARTESIAN_POINT ( 'NONE',  ( -9.775576553118467515, -0.04422114144963021354, 1.826781837067675607 ) ) ;
#20964=ORIENTED_EDGE ( 'NONE', *, *, #37671, .T. ) ;
#20965=EDGE_LOOP ( 'NONE', ( #44638, #48074, #2492, #50252 ) ) ;
#20966=DIRECTION ( 'NONE',  ( 0.6427681459581294776, -0.7660444431189769032, 0.005002170337467562802 ) ) ;
#20967=EDGE_LOOP ( 'NONE', ( #1777, #54120, #42049, #28758 ) ) ;
#20968=EDGE_CURVE ( 'NONE', #50902, #39023, #9985, .T. ) ;
#20969=LINE ( 'NONE', #20423, #32018 ) ;
#20970=EDGE_CURVE ( 'NONE', #20189, #38808, #44603, .T. ) ;
#20971=ORIENTED_EDGE ( 'NONE', *, *, #22357, .T. ) ;
#20972=ORIENTED_EDGE ( 'NONE', *, *, #6079, .F. ) ;
#20973=VERTEX_POINT ( 'NONE', #36667 ) ;
#20974=EDGE_CURVE ( 'NONE', #20246, #50299, #32425, .T. ) ;
#20975=DIRECTION ( 'NONE',  ( 0.9999697198139515519, 0.000000000000000000, 0.007781995580013368816 ) ) ;
#20976=CARTESIAN_POINT ( 'NONE',  ( -17.93139508144814442, 0.000000000000000000, 13.85596890686001537 ) ) ;
#20977=CARTESIAN_POINT ( 'NONE',  ( -22.31155744454273915, -5.536956232915666298, 5.371229839343643953 ) ) ;
#20978=VECTOR ( 'NONE', #53791, 999.9999999999998863 ) ;
#20979=EDGE_CURVE ( 'NONE', #38944, #49575, #7679, .T. ) ;
#20980=AXIS2_PLACEMENT_3D ( 'NONE', #46269, #42321, #3417 ) ;
#20981=ORIENTED_EDGE ( 'NONE', *, *, #48281, .T. ) ;
#20982=ORIENTED_EDGE ( 'NONE', *, *, #34269, .F. ) ;
#20983=ADVANCED_FACE ( 'NONE', ( #25007 ), #7383, .F. ) ;
#20984=AXIS2_PLACEMENT_3D ( 'NONE', #27105, #14341, #31654 ) ;
#20985=DIRECTION ( 'NONE',  ( -0.5449076811759708816, 0.6444004775717707689, 0.5364919789714475140 ) ) ;
#20986=CARTESIAN_POINT ( 'NONE',  ( -18.39746900504187010, 0.000000000000000000, 14.03700784672088808 ) ) ;
#20987=ORIENTED_EDGE ( 'NONE', *, *, #12885, .F. ) ;
#20988=LINE ( 'NONE', #29541, #47266 ) ;
#20989=LINE ( 'NONE', #38612, #42234 ) ;
#20990=EDGE_LOOP ( 'NONE', ( #151, #3676, #6147, #31369 ) ) ;
#20991=CARTESIAN_POINT ( 'NONE',  ( -17.93139508144814442, 0.000000000000000000, 13.85596890686001537 ) ) ;
#20992=CARTESIAN_POINT ( 'NONE',  ( -15.03495456790438389, -0.1191753592594197858, 12.77051346725278158 ) ) ;
#20993=VERTEX_POINT ( 'NONE', #50268 ) ;
#20994=PLANE ( 'NONE',  #23703 ) ;
#20996=AXIS2_PLACEMENT_3D ( 'NONE', #17286, #7666, #50808 ) ;
#20997=CARTESIAN_POINT ( 'NONE',  ( -13.56399075187187542, -0.6798977022406560433, 2.128343463916670952 ) ) ;
#20998=ORIENTED_EDGE ( 'NONE', *, *, #15867, .F. ) ;
#21000=DIRECTION ( 'NONE',  ( -0.6427681459581293666, -0.7660444431189770143, -0.005002170337467561935 ) ) ;
#21001=CARTESIAN_POINT ( 'NONE',  ( -10.28842178966973897, 0.000000000000000000, 0.8776935365639153552 ) ) ;
#21002=DIRECTION ( 'NONE',  ( 0.7660212471507180654, -0.6427876096865404731, 0.005961354470445141482 ) ) ;
#21003=ORIENTED_EDGE ( 'NONE', *, *, #56052, .T. ) ;
#21004=DIRECTION ( 'NONE',  ( -0.6427681459581293666, -0.7660444431189770143, -0.005002170337467561935 ) ) ;
#21005=DIRECTION ( 'NONE',  ( -0.6427681459581293666, -0.7660444431189770143, -0.005002170337467561935 ) ) ;
#21006=CARTESIAN_POINT ( 'NONE',  ( -24.27063949748155380, 0.000000000000000000, 6.308861732390097288 ) ) ;
#21007=DIRECTION ( 'NONE',  ( -0.005002170337468016433, -0.7660444431189770143, 0.6427681459581293666 ) ) ;
#21008=LINE ( 'NONE', #26392, #14963 ) ;
#21009=LINE ( 'NONE', #38338, #27004 ) ;
#21010=CARTESIAN_POINT ( 'NONE',  ( -25.20278734466900517, 0.000000000000000000, 6.670939612111840944 ) ) ;
#21011=VERTEX_POINT ( 'NONE', #46024 ) ;
#21013=DIRECTION ( 'NONE',  ( -0.7660212471507179544, -0.6427876096865405842, -0.005961354470445141482 ) ) ;
#21014=VERTEX_POINT ( 'NONE', #25288 ) ;
#21015=PLANE ( 'NONE',  #27482 ) ;
#21016=DIRECTION ( 'NONE',  ( -0.005961354470445682716, -0.6427876096865404731, 0.7660212471507180654 ) ) ;
#21017=EDGE_CURVE ( 'NONE', #45314, #48949, #12216, .T. ) ;
#21018=EDGE_CURVE ( 'NONE', #5914, #47750, #32955, .T. ) ;
#21019=VECTOR ( 'NONE', #20889, 999.9999999999998863 ) ;
#21020=VECTOR ( 'NONE', #26447, 1000.000000000000000 ) ;
#21021=DIRECTION ( 'NONE',  ( 0.5364919789714477361, 0.6444004775717706579, 0.5449076811759711036 ) ) ;
#21022=ADVANCED_FACE ( 'NONE', ( #3685 ), #24700, .F. ) ;
#21023=PLANE ( 'NONE',  #11526 ) ;
#21024=LINE ( 'NONE', #16782, #49230 ) ;
#21025=VERTEX_POINT ( 'NONE', #51109 ) ;
#21026=VECTOR ( 'NONE', #38635, 1000.000000000000114 ) ;
#21027=EDGE_LOOP ( 'NONE', ( #47238, #39729, #22502, #48126 ) ) ;
#21028=DIRECTION ( 'NONE',  ( -0.9999697198139514409, -0.000000000000000000, -0.007781995580013368816 ) ) ;
#21029=LINE ( 'NONE', #8002, #39513 ) ;
#21030=ORIENTED_EDGE ( 'NONE', *, *, #34115, .T. ) ;
#21034=AXIS2_PLACEMENT_3D ( 'NONE', #28063, #15011, #28327 ) ;
#21035=ORIENTED_EDGE ( 'NONE', *, *, #7350, .T. ) ;
#21036=FACE_OUTER_BOUND ( 'NONE', #19459, .T. ) ;
#21037=AXIS2_PLACEMENT_3D ( 'NONE', #31059, #20369, #37709 ) ;
#21038=ORIENTED_EDGE ( 'NONE', *, *, #48409, .F. ) ;
#21039=ORIENTED_EDGE ( 'NONE', *, *, #17021, .F. ) ;
#21040=ORIENTED_EDGE ( 'NONE', *, *, #47652, .T. ) ;
#21041=CARTESIAN_POINT ( 'NONE',  ( -12.43266248435915422, 0.000000000000000000, 8.047641899584064618 ) ) ;
#21042=CARTESIAN_POINT ( 'NONE',  ( -18.56568686646327393, 0.000000000000000000, 9.846573634752608939 ) ) ;
#21043=CARTESIAN_POINT ( 'NONE',  ( -15.46633387165207019, -0.1191753592594185784, 8.493368265297117858 ) ) ;
#21044=LINE ( 'NONE', #7726, #34706 ) ;
#21045=ORIENTED_EDGE ( 'NONE', *, *, #13245, .T. ) ;
#21046=ORIENTED_EDGE ( 'NONE', *, *, #38593, .T. ) ;
#21047=EDGE_CURVE ( 'NONE', #30203, #10825, #42330, .T. ) ;
#21048=ORIENTED_EDGE ( 'NONE', *, *, #11715, .F. ) ;
#21049=DIRECTION ( 'NONE',  ( -0.6427681459581293666, -0.7660444431189770143, -0.005002170337467561935 ) ) ;
#21050=EDGE_CURVE ( 'NONE', #9472, #46146, #42024, .T. ) ;
#21051=CARTESIAN_POINT ( 'NONE',  ( -17.26532721389163072, 0.000000000000000000, 13.67648636611514590 ) ) ;
#21052=ORIENTED_EDGE ( 'NONE', *, *, #53929, .F. ) ;
#21053=VECTOR ( 'NONE', #25791, 999.9999999999998863 ) ;
#21054=LINE ( 'NONE', #46923, #5779 ) ;
#21055=EDGE_CURVE ( 'NONE', #55340, #26051, #45724, .T. ) ;
#21056=ORIENTED_EDGE ( 'NONE', *, *, #40344, .T. ) ;
#21057=DIRECTION ( 'NONE',  ( 0.005002170337468016433, -0.7660444431189770143, -0.6427681459581293666 ) ) ;
#21058=DIRECTION ( 'NONE',  ( -0.8531650599175529814, -0.4028455766673920135, 0.3313982828793697877 ) ) ;
#21059=VECTOR ( 'NONE', #44105, 1000.000000000000114 ) ;
#21060=VECTOR ( 'NONE', #17299, 1000.000000000000227 ) ;
#21061=EDGE_LOOP ( 'NONE', ( #12630, #13938, #4341, #41164 ) ) ;
#21062=ADVANCED_FACE ( 'NONE', ( #33517 ), #24172, .F. ) ;
#21063=CARTESIAN_POINT ( 'NONE',  ( -18.35493042423798471, 0.000000000000000000, 8.570891567112456144 ) ) ;
#21064=ORIENTED_EDGE ( 'NONE', *, *, #2853, .F. ) ;
#21065=AXIS2_PLACEMENT_3D ( 'NONE', #20897, #37959, #42216 ) ;
#21066=DIRECTION ( 'NONE',  ( 0.007781995580012663651, 0.000000000000000000, -0.9999697198139515519 ) ) ;
#21067=DIRECTION ( 'NONE',  ( -0.2426528472758542054, 0.7422098413412800966, -0.6246952433987894571 ) ) ;
#21069=ORIENTED_EDGE ( 'NONE', *, *, #24405, .F. ) ;
#21070=PLANE ( 'NONE',  #17804 ) ;
#21071=DIRECTION ( 'NONE',  ( 0.005002170337468016433, -0.7660444431189770143, -0.6427681459581293666 ) ) ;
#21073=PLANE ( 'NONE',  #51829 ) ;
#21074=EDGE_LOOP ( 'NONE', ( #36110, #20166, #28273, #56072 ) ) ;
#21075=DIRECTION ( 'NONE',  ( -0.9999697198139514409, -0.000000000000000000, -0.007781995580013368816 ) ) ;
#21077=AXIS2_PLACEMENT_3D ( 'NONE', #4959, #953, #43320 ) ;
#21078=DIRECTION ( 'NONE',  ( 0.007781995580012662783, 0.000000000000000000, -0.9999697198139514409 ) ) ;
#21079=DIRECTION ( 'NONE',  ( -0.005002170337468016433, -0.7660444431189770143, 0.6427681459581293666 ) ) ;
#21080=CARTESIAN_POINT ( 'NONE',  ( -12.60458797795435615, 0.000000000000000000, 11.86609696750642229 ) ) ;
#21081=FACE_OUTER_BOUND ( 'NONE', #23580, .T. ) ;
#21082=ORIENTED_EDGE ( 'NONE', *, *, #53470, .T. ) ;
#21083=CARTESIAN_POINT ( 'NONE',  ( -21.47263955680318404, 0.000000000000000000, 5.022634149262071190 ) ) ;
#21084=CARTESIAN_POINT ( 'NONE',  ( -17.74404816805336793, 0.000000000000000000, 3.574322630375089460 ) ) ;
#21085=CARTESIAN_POINT ( 'NONE',  ( -15.82312983555391206, 0.000000000000000000, 7.482598415295212746 ) ) ;
#21086=EDGE_LOOP ( 'NONE', ( #2954, #51635, #44202, #35934 ) ) ;
#21087=CARTESIAN_POINT ( 'NONE',  ( -14.53902905116009947, -2.946525016555661125, 2.434764173376773755 ) ) ;
#21088=VERTEX_POINT ( 'NONE', #24427 ) ;
#21089=EDGE_CURVE ( 'NONE', #54842, #44961, #2827, .T. ) ;
#21091=CARTESIAN_POINT ( 'NONE',  ( -21.47263955680318404, 0.000000000000000000, 5.022634149262071190 ) ) ;
#21092=AXIS2_PLACEMENT_3D ( 'NONE', #48411, #9817, #27122 ) ;
#21093=ADVANCED_FACE ( 'NONE', ( #20152 ), #54807, .F. ) ;
#21094=EDGE_CURVE ( 'NONE', #28463, #45380, #41487, .T. ) ;
#21095=CARTESIAN_POINT ( 'NONE',  ( -8.929802727318762123, -0.1191753592594179401, 4.481584294213840636 ) ) ;
#21097=VERTEX_POINT ( 'NONE', #46564 ) ;
#21098=VERTEX_POINT ( 'NONE', #15919 ) ;
#21099=CARTESIAN_POINT ( 'NONE',  ( -10.47421230394850866, 0.000000000000000000, 10.95934586908605723 ) ) ;
#21100=CARTESIAN_POINT ( 'NONE',  ( -10.19575411036579915, 0.000000000000000000, 0.8784146978715680065 ) ) ;
#21101=VECTOR ( 'NONE', #17149, 1000.000000000000000 ) ;
#21102=LINE ( 'NONE', #43801, #33236 ) ;
#21103=AXIS2_PLACEMENT_3D ( 'NONE', #46444, #11563, #54691 ) ;
#21104=DIRECTION ( 'NONE',  ( 0.5364919789714477361, 0.6444004775717706579, 0.5449076811759711036 ) ) ;
#21105=VECTOR ( 'NONE', #33399, 999.9999999999998863 ) ;
#21106=CARTESIAN_POINT ( 'NONE',  ( -12.10160420820394478, 0.000000000000000000, 6.942222062218735168 ) ) ;
#21108=EDGE_LOOP ( 'NONE', ( #22487, #54146, #1424, #5184 ) ) ;
#21109=CARTESIAN_POINT ( 'NONE',  ( -16.81190032086591302, 0.000000000000000000, 3.212244750653343583 ) ) ;
#21110=EDGE_CURVE ( 'NONE', #5924, #27743, #32669, .T. ) ;
#21111=CARTESIAN_POINT ( 'NONE',  ( -16.33317936670417225, 0.000000000000000000, 13.31440848639340224 ) ) ;
#21113=CARTESIAN_POINT ( 'NONE',  ( -15.87975247367846166, 0.000000000000000000, 2.850166870931599927 ) ) ;
#21114=AXIS2_PLACEMENT_3D ( 'NONE', #40545, #14137, #17838 ) ;
#21115=VERTEX_POINT ( 'NONE', #20458 ) ;
#21117=DIRECTION ( 'NONE',  ( -0.7660212471507179544, -0.6427876096865405842, -0.005961354470445141482 ) ) ;
#21118=DIRECTION ( 'NONE',  ( -0.6427681459581293666, -0.7660444431189770143, -0.005002170337467561935 ) ) ;
#21119=VERTEX_POINT ( 'NONE', #37797 ) ;
#21120=DIRECTION ( 'NONE',  ( 0.000000000000000000, 0.000000000000000000, 1.000000000000000000 ) ) ;
#21121=AXIS2_PLACEMENT_3D ( 'NONE', #9344, #9075, #49375 ) ;
#21122=ORIENTED_EDGE ( 'NONE', *, *, #3788, .F. ) ;
#21123=VECTOR ( 'NONE', #18187, 999.9999999999998863 ) ;
#21124=ORIENTED_EDGE ( 'NONE', *, *, #42297, .T. ) ;
#21125=ORIENTED_EDGE ( 'NONE', *, *, #4786, .F. ) ;
#21126=VERTEX_POINT ( 'NONE', #55107 ) ;
#21127=DIRECTION ( 'NONE',  ( 0.7660212471507180654, -0.6427876096865404731, 0.005961354470445141482 ) ) ;
#21128=EDGE_LOOP ( 'NONE', ( #15248, #34567, #50095, #828 ) ) ;
#21129=VECTOR ( 'NONE', #9794, 1000.000000000000114 ) ;
#21130=PLANE ( 'NONE',  #34003 ) ;
#21131=ORIENTED_EDGE ( 'NONE', *, *, #5360, .F. ) ;
#21132=CARTESIAN_POINT ( 'NONE',  ( -14.43496725204122377, 0.000000000000000000, 8.232065557114770726 ) ) ;
#21133=EDGE_CURVE ( 'NONE', #18997, #19093, #38057, .T. ) ;
#21134=VERTEX_POINT ( 'NONE', #55364 ) ;
#21135=VECTOR ( 'NONE', #19653, 1000.000000000000227 ) ;
#21136=ORIENTED_EDGE ( 'NONE', *, *, #24040, .T. ) ;
#21137=CARTESIAN_POINT ( 'NONE',  ( -18.79944894654208909, 0.000000000000000000, 5.982107732540097089 ) ) ;
#21138=LINE ( 'NONE', #3548, #52244 ) ;
#21139=DIRECTION ( 'NONE',  ( 0.5364919789714477361, 0.6444004775717706579, 0.5449076811759711036 ) ) ;
#21140=LINE ( 'NONE', #8104, #54080 ) ;
#21141=AXIS2_PLACEMENT_3D ( 'NONE', #16796, #46908, #8008 ) ;
#21142=DIRECTION ( 'NONE',  ( 0.5449076811759707706, 0.6444004775717708799, -0.5364919789714476250 ) ) ;
#21143=ORIENTED_EDGE ( 'NONE', *, *, #34652, .T. ) ;
#21144=EDGE_CURVE ( 'NONE', #23572, #55568, #16460, .T. ) ;
#21145=AXIS2_PLACEMENT_3D ( 'NONE', #48133, #25730, #39653 ) ;
#21146=VECTOR ( 'NONE', #45267, 1000.000000000000227 ) ;
#21148=FACE_OUTER_BOUND ( 'NONE', #52370, .T. ) ;
#21151=EDGE_CURVE ( 'NONE', #26046, #294, #4282, .T. ) ;
#21152=EDGE_CURVE ( 'NONE', #11770, #27552, #12513, .T. ) ;
#21153=CARTESIAN_POINT ( 'NONE',  ( -5.876231750791062858, 5.744269837952261426, 5.500901545341295495 ) ) ;
#21154=AXIS2_PLACEMENT_3D ( 'NONE', #28381, #6822, #2267 ) ;
#21155=AXIS2_PLACEMENT_3D ( 'NONE', #20321, #13151, #21395 ) ;
#21156=DIRECTION ( 'NONE',  ( 0.000000000000000000, -0.000000000000000000, -1.000000000000000000 ) ) ;
#21157=DIRECTION ( 'NONE',  ( -0.5364919789714478471, 0.6444004775717705469, -0.5449076811759709926 ) ) ;
#21158=PLANE ( 'NONE',  #21437 ) ;
#21159=ORIENTED_EDGE ( 'NONE', *, *, #35731, .F. ) ;
#21160=DIRECTION ( 'NONE',  ( 0.005002170337468016433, -0.7660444431189770143, -0.6427681459581293666 ) ) ;
#21161=EDGE_CURVE ( 'NONE', #13455, #49751, #34625, .T. ) ;
#21162=FACE_OUTER_BOUND ( 'NONE', #54702, .T. ) ;
#21163=ORIENTED_EDGE ( 'NONE', *, *, #15678, .T. ) ;
#21164=DIRECTION ( 'NONE',  ( 0.7660212471507180654, -0.6427876096865404731, 0.005961354470445141482 ) ) ;
#21165=FACE_OUTER_BOUND ( 'NONE', #743, .T. ) ;
#21166=EDGE_CURVE ( 'NONE', #38597, #5370, #9348, .T. ) ;
#21167=LINE ( 'NONE', #33407, #33210 ) ;
#21168=EDGE_CURVE ( 'NONE', #1327, #51910, #9078, .T. ) ;
#21169=DIRECTION ( 'NONE',  ( -0.6427681459581293666, -0.7660444431189770143, -0.005002170337467561935 ) ) ;
#21170=ORIENTED_EDGE ( 'NONE', *, *, #9337, .F. ) ;
#21171=EDGE_LOOP ( 'NONE', ( #51105, #12365, #9778, #27878 ) ) ;
#21172=DIRECTION ( 'NONE',  ( 0.007781995580012662783, 0.000000000000000000, -0.9999697198139514409 ) ) ;
#21173=CARTESIAN_POINT ( 'NONE',  ( -15.15583128246454336, -0.3560938001956568399, 2.756999424905611118 ) ) ;
#21174=PLANE ( 'NONE',  #683 ) ;
#21175=VECTOR ( 'NONE', #8035, 999.9999999999998863 ) ;
#21176=EDGE_CURVE ( 'NONE', #18261, #51932, #21596, .T. ) ;
#21177=FACE_OUTER_BOUND ( 'NONE', #44354, .T. ) ;
#21178=DIRECTION ( 'NONE',  ( 0.000000000000000000, -0.000000000000000000, -1.000000000000000000 ) ) ;
#21179=VECTOR ( 'NONE', #21877, 999.9999999999998863 ) ;
#21180=DIRECTION ( 'NONE',  ( 0.5449076811759707706, 0.6444004775717708799, -0.5364919789714476250 ) ) ;
#21181=CARTESIAN_POINT ( 'NONE',  ( -15.14840367773380336, 1.743523803501505709, 5.626895143433455537 ) ) ;
#21182=ADVANCED_FACE ( 'NONE', ( #56212 ), #55653, .F. ) ;
#21183=PLANE ( 'NONE',  #35963 ) ;
#21185=AXIS2_PLACEMENT_3D ( 'NONE', #4099, #21427, #42148 ) ;
#21186=DIRECTION ( 'NONE',  ( -0.5364919789714478471, 0.6444004775717705469, -0.5449076811759709926 ) ) ;
#21187=VERTEX_POINT ( 'NONE', #43440 ) ;
#21188=DIRECTION ( 'NONE',  ( 0.5364919789714477361, 0.6444004775717706579, 0.5449076811759711036 ) ) ;
#21189=AXIS2_PLACEMENT_3D ( 'NONE', #42652, #17112, #21071 ) ;
#21190=AXIS2_PLACEMENT_3D ( 'NONE', #52472, #30334, #38570 ) ;
#21191=EDGE_LOOP ( 'NONE', ( #6893, #4331, #29365, #40389 ) ) ;
#21192=EDGE_LOOP ( 'NONE', ( #55083, #50001, #7037, #22901 ) ) ;
#21194=ORIENTED_EDGE ( 'NONE', *, *, #3479, .T. ) ;
#21195=ORIENTED_EDGE ( 'NONE', *, *, #48716, .T. ) ;
#21196=VECTOR ( 'NONE', #52795, 1000.000000000000227 ) ;
#21197=ORIENTED_EDGE ( 'NONE', *, *, #22608, .F. ) ;
#21198=ORIENTED_EDGE ( 'NONE', *, *, #49992, .T. ) ;
#21199=CARTESIAN_POINT ( 'NONE',  ( -21.65435634735958104, -3.594132820645660420, 10.99180339266565376 ) ) ;
#21200=DIRECTION ( 'NONE',  ( 0.7660212471507180654, -0.6427876096865404731, 0.005961354470445141482 ) ) ;
#21201=DIRECTION ( 'NONE',  ( 0.9999697198139515519, 0.000000000000000000, 0.007781995580013368816 ) ) ;
#21203=CARTESIAN_POINT ( 'NONE',  ( -24.26986129792355129, -0.1191753592594197858, 6.208864760408702388 ) ) ;
#21204=EDGE_CURVE ( 'NONE', #14373, #51521, #21845, .T. ) ;
#21205=ORIENTED_EDGE ( 'NONE', *, *, #4579, .F. ) ;
#21206=LINE ( 'NONE', #20067, #10510 ) ;
#21207=ORIENTED_EDGE ( 'NONE', *, *, #19893, .T. ) ;
#21208=CARTESIAN_POINT ( 'NONE',  ( -11.23286883698721006, -0.1191753592594199940, 1.878336812569445957 ) ) ;
#21209=AXIS2_PLACEMENT_3D ( 'NONE', #3185, #19383, #29307 ) ;
#21210=LINE ( 'NONE', #4200, #26476 ) ;
#21211=DIRECTION ( 'NONE',  ( -0.3620778797217456546, 0.000000000000000000, -0.9321478471874540261 ) ) ;
#21212=ORIENTED_EDGE ( 'NONE', *, *, #47646, .T. ) ;
#21213=DIRECTION ( 'NONE',  ( -0.005961354470445682716, -0.6427876096865404731, 0.7660212471507180654 ) ) ;
#21214=AXIS2_PLACEMENT_3D ( 'NONE', #41554, #33031, #32738 ) ;
#21215=ORIENTED_EDGE ( 'NONE', *, *, #28039, .T. ) ;
#21216=EDGE_CURVE ( 'NONE', #42837, #37228, #17050, .T. ) ;
#21217=CARTESIAN_POINT ( 'NONE',  ( 2.072287782118878319, 0.000000000000000000, -2.950529333540147015 ) ) ;
#21218=PLANE ( 'NONE',  #43878 ) ;
#21219=VECTOR ( 'NONE', #5586, 999.9999999999998863 ) ;
#21220=EDGE_CURVE ( 'NONE', #2279, #41786, #43994, .T. ) ;
#21221=CARTESIAN_POINT ( 'NONE',  ( -28.93060053386082231, -0.1191753592594197858, 8.019254159017428663 ) ) ;
#21222=DIRECTION ( 'NONE',  ( 0.6427681459581294776, -0.7660444431189769032, 0.005002170337467562802 ) ) ;
#21223=DIRECTION ( 'NONE',  ( -0.005002170337468016433, -0.7660444431189770143, 0.6427681459581293666 ) ) ;
#21224=DIRECTION ( 'NONE',  ( 0.9999697198139515519, 0.000000000000000000, 0.007781995580013368816 ) ) ;
#21225=CARTESIAN_POINT ( 'NONE',  ( -12.19881617777849492, 3.200641362704007786, 6.872553345591845719 ) ) ;
#21226=AXIS2_PLACEMENT_3D ( 'NONE', #870, #21636, #38949 ) ;
#21227=LINE ( 'NONE', #38558, #49485 ) ;
#21228=ORIENTED_EDGE ( 'NONE', *, *, #10419, .F. ) ;
#21229=CARTESIAN_POINT ( 'NONE',  ( -17.74404816805336793, 0.000000000000000000, 3.574322630375089460 ) ) ;
#21230=VERTEX_POINT ( 'NONE', #52250 ) ;
#21231=AXIS2_PLACEMENT_3D ( 'NONE', #28713, #45190, #6849 ) ;
#21232=LINE ( 'NONE', #47647, #47381 ) ;
#21233=FACE_OUTER_BOUND ( 'NONE', #29297, .T. ) ;
#21235=DIRECTION ( 'NONE',  ( 0.007781995580012663651, 0.000000000000000000, -0.9999697198139515519 ) ) ;
#21236=DIRECTION ( 'NONE',  ( 0.5449076811759707706, 0.6444004775717708799, -0.5364919789714476250 ) ) ;
#21237=CARTESIAN_POINT ( 'NONE',  ( 2.072287782118878319, 0.000000000000000000, -2.950529333540147015 ) ) ;
#21238=EDGE_CURVE ( 'NONE', #13281, #34911, #39468, .T. ) ;
#21239=VECTOR ( 'NONE', #53861, 1000.000000000000227 ) ;
#21240=PLANE ( 'NONE',  #19232 ) ;
#21241=VECTOR ( 'NONE', #11554, 999.9999999999998863 ) ;
#21242=VERTEX_POINT ( 'NONE', #5117 ) ;
#21243=LINE ( 'NONE', #47659, #18443 ) ;
#21244=CARTESIAN_POINT ( 'NONE',  ( -15.88053067323646417, -0.1191753592594197858, 2.950163842912994383 ) ) ;
#21245=CARTESIAN_POINT ( 'NONE',  ( -13.27065584551087163, 0.000000000000000000, 12.04557950825129176 ) ) ;
#21246=EDGE_CURVE ( 'NONE', #21762, #41020, #47131, .T. ) ;
#21247=PLANE ( 'NONE',  #2805 ) ;
#21248=CARTESIAN_POINT ( 'NONE',  ( -17.74560456716937296, 0.000000000000000000, 3.774316574337878372 ) ) ;
#21249=DIRECTION ( 'NONE',  ( 0.000000000000000000, -1.000000000000000000, 0.000000000000000000 ) ) ;
#21250=DIRECTION ( 'NONE',  ( 0.005002170337468016433, -0.7660444431189770143, -0.6427681459581293666 ) ) ;
#21251=ORIENTED_EDGE ( 'NONE', *, *, #35218, .T. ) ;
#21252=AXIS2_PLACEMENT_3D ( 'NONE', #6544, #19880, #37199 ) ;
#21253=EDGE_CURVE ( 'NONE', #22669, #48082, #25549, .T. ) ;
#21254=LINE ( 'NONE', #26100, #1294 ) ;
#21255=DIRECTION ( 'NONE',  ( 0.000000000000000000, -0.000000000000000000, -1.000000000000000000 ) ) ;
#21256=VERTEX_POINT ( 'NONE', #17597 ) ;
#21257=AXIS2_PLACEMENT_3D ( 'NONE', #27876, #1718, #41726 ) ;
#21258=ORIENTED_EDGE ( 'NONE', *, *, #30289, .T. ) ;
#21259=DIRECTION ( 'NONE',  ( -0.5449076811759708816, 0.6444004775717707689, 0.5364919789714475140 ) ) ;
#21260=VECTOR ( 'NONE', #15359, 1000.000000000000000 ) ;
#21262=ORIENTED_EDGE ( 'NONE', *, *, #16674, .F. ) ;
#21263=VERTEX_POINT ( 'NONE', #12774 ) ;
#21264=VECTOR ( 'NONE', #8960, 1000.000000000000000 ) ;
#21265=EDGE_LOOP ( 'NONE', ( #6260, #40670, #28460, #43579 ) ) ;
#21266=DIRECTION ( 'NONE',  ( 0.5364919789714477361, 0.6444004775717706579, 0.5449076811759711036 ) ) ;
#21267=AXIS2_PLACEMENT_3D ( 'NONE', #13588, #26647, #52753 ) ;
#21268=EDGE_LOOP ( 'NONE', ( #36288, #45415, #37124, #1368 ) ) ;
#21269=CARTESIAN_POINT ( 'NONE',  ( -19.72716634110825851, 0.000000000000000000, 5.774881965041287479 ) ) ;
#21270=DIRECTION ( 'NONE',  ( -0.5364919789714478471, 0.6444004775717705469, -0.5449076811759709926 ) ) ;
#21271=VECTOR ( 'NONE', #51611, 999.9999999999998863 ) ;
#21272=EDGE_LOOP ( 'NONE', ( #41481, #2090, #15399, #50092 ) ) ;
#21273=EDGE_CURVE ( 'NONE', #5706, #6174, #47712, .T. ) ;
#21274=ORIENTED_EDGE ( 'NONE', *, *, #49981, .F. ) ;
#21276=VECTOR ( 'NONE', #26219, 1000.000000000000227 ) ;
#21277=EDGE_CURVE ( 'NONE', #26788, #15460, #21298, .T. ) ;
#21278=CARTESIAN_POINT ( 'NONE',  ( -13.21518402393321168, 0.000000000000000000, 4.917569563982915781 ) ) ;
#21279=DIRECTION ( 'NONE',  ( 0.5364919789714477361, 0.6444004775717706579, 0.5449076811759711036 ) ) ;
#21280=ORIENTED_EDGE ( 'NONE', *, *, #40021, .T. ) ;
#21281=EDGE_CURVE ( 'NONE', #35085, #21351, #34935, .T. ) ;
#21282=CARTESIAN_POINT ( 'NONE',  ( 2.072287782118878319, 0.000000000000000000, -2.950529333540147015 ) ) ;
#21283=CARTESIAN_POINT ( 'NONE',  ( -17.29039281695302677, -0.1191753592594170658, 4.047188179131904207 ) ) ;
#21284=ORIENTED_EDGE ( 'NONE', *, *, #31045, .T. ) ;
#21285=FACE_OUTER_BOUND ( 'NONE', #44313, .T. ) ;
#21286=EDGE_CURVE ( 'NONE', #44937, #16954, #51669, .T. ) ;
#21287=EDGE_CURVE ( 'NONE', #47771, #48446, #26131, .T. ) ;
#21288=ADVANCED_FACE ( 'NONE', ( #27232 ), #36065, .F. ) ;
#21289=ORIENTED_EDGE ( 'NONE', *, *, #19519, .F. ) ;
#21290=DIRECTION ( 'NONE',  ( 0.000000000000000000, -0.000000000000000000, -1.000000000000000000 ) ) ;
#21291=VECTOR ( 'NONE', #18377, 1000.000000000000227 ) ;
#21292=DIRECTION ( 'NONE',  ( 0.9999697198139515519, 0.000000000000000000, 0.007781995580013368816 ) ) ;
#21293=ORIENTED_EDGE ( 'NONE', *, *, #12054, .T. ) ;
#21294=FACE_OUTER_BOUND ( 'NONE', #24003, .T. ) ;
#21295=CARTESIAN_POINT ( 'NONE',  ( -10.47421230394850866, 0.000000000000000000, 10.95934586908605723 ) ) ;
#21296=LINE ( 'NONE', #51108, #47503 ) ;
#21297=VECTOR ( 'NONE', #43369, 1000.000000000000227 ) ;
#21298=LINE ( 'NONE', #38630, #32858 ) ;
#21299=VERTEX_POINT ( 'NONE', #10190 ) ;
#21300=AXIS2_PLACEMENT_3D ( 'NONE', #6498, #32614, #49382 ) ;
#21301=CARTESIAN_POINT ( 'NONE',  ( -16.89925026227929195, -0.1191753592594197858, 13.49466922669627422 ) ) ;
#21302=DIRECTION ( 'NONE',  ( -0.8531650599175527594, 0.4028455766673922356, 0.3313982828793700652 ) ) ;
#21303=CARTESIAN_POINT ( 'NONE',  ( -14.01545677930355183, 0.000000000000000000, 2.126011111488108174 ) ) ;
#21304=ADVANCED_FACE ( 'NONE', ( #49672 ), #10495, .F. ) ;
#21305=AXIS2_PLACEMENT_3D ( 'NONE', #41421, #2757, #49083 ) ;
#21306=LINE ( 'NONE', #34372, #42222 ) ;
#21307=DIRECTION ( 'NONE',  ( 0.5449076811759707706, 0.6444004775717708799, -0.5364919789714476250 ) ) ;
#21308=LINE ( 'NONE', #34375, #17069 ) ;
#21309=EDGE_CURVE ( 'NONE', #5703, #32241, #23274, .T. ) ;
#21310=CARTESIAN_POINT ( 'NONE',  ( -18.67619601524082285, 0.000000000000000000, 3.936400510096834893 ) ) ;
#21311=VECTOR ( 'NONE', #14022, 1000.000000000000227 ) ;
#21312=CARTESIAN_POINT ( 'NONE',  ( -19.12962290826653700, 0.000000000000000000, 14.40064212555863854 ) ) ;
#21313=VECTOR ( 'NONE', #49799, 1000.000000000000114 ) ;
#21314=ORIENTED_EDGE ( 'NONE', *, *, #47960, .T. ) ;
#21315=ADVANCED_FACE ( 'NONE', ( #22977 ), #14732, .F. ) ;
#21316=AXIS2_PLACEMENT_3D ( 'NONE', #42609, #42888, #34114 ) ;
#21317=DIRECTION ( 'NONE',  ( 0.000000000000000000, -1.000000000000000000, 0.000000000000000000 ) ) ;
#21318=VERTEX_POINT ( 'NONE', #35471 ) ;
#21319=VECTOR ( 'NONE', #37542, 1000.000000000000000 ) ;
#21320=CARTESIAN_POINT ( 'NONE',  ( -13.17065887352947762, -0.1191753592594197858, 12.04635770780929427 ) ) ;
#21321=LINE ( 'NONE', #3993, #9133 ) ;
#21322=VECTOR ( 'NONE', #48314, 999.9999999999998863 ) ;
#21323=ADVANCED_FACE ( 'NONE', ( #26975 ), #5954, .F. ) ;
#21324=DIRECTION ( 'NONE',  ( 0.6427681459581294776, -0.7660444431189769032, 0.005002170337467562802 ) ) ;
#21325=LINE ( 'NONE', #4837, #45059 ) ;
#21327=VERTEX_POINT ( 'NONE', #1671 ) ;
#21329=AXIS2_PLACEMENT_3D ( 'NONE', #42185, #51271, #15774 ) ;
#21330=EDGE_LOOP ( 'NONE', ( #40887, #36798, #14100 ) ) ;
#21331=CARTESIAN_POINT ( 'NONE',  ( -19.45503627000849889, 0.000000000000000000, 7.556996783084074742 ) ) ;
#21332=CARTESIAN_POINT ( 'NONE',  ( -15.40103151951671734, 0.000000000000000000, 12.95233060667165681 ) ) ;
#21333=ORIENTED_EDGE ( 'NONE', *, *, #16732, .F. ) ;
#21334=PLANE ( 'NONE',  #15694 ) ;
#21335=ORIENTED_EDGE ( 'NONE', *, *, #11641, .F. ) ;
#21336=LINE ( 'NONE', #9385, #36782 ) ;
#21337=ORIENTED_EDGE ( 'NONE', *, *, #11569, .F. ) ;
#21338=DIRECTION ( 'NONE',  ( -0.9999697198139514409, -0.000000000000000000, -0.007781995580013368816 ) ) ;
#21339=VECTOR ( 'NONE', #19980, 999.9999999999998863 ) ;
#21340=ORIENTED_EDGE ( 'NONE', *, *, #20318, .F. ) ;
#21341=VERTEX_POINT ( 'NONE', #40007 ) ;
#21342=ORIENTED_EDGE ( 'NONE', *, *, #13506, .T. ) ;
#21343=AXIS2_PLACEMENT_3D ( 'NONE', #49290, #22622, #18073 ) ;
#21344=DIRECTION ( 'NONE',  ( -0.9321478471874540261, 0.000000000000000000, 0.3620778797217457656 ) ) ;
#21345=CARTESIAN_POINT ( 'NONE',  ( -13.07066190154808361, 0.000000000000000000, 12.04713590736729678 ) ) ;
#21346=AXIS2_PLACEMENT_3D ( 'NONE', #48175, #43927, #22378 ) ;
#21347=LINE ( 'NONE', #16506, #51134 ) ;
#21348=DIRECTION ( 'NONE',  ( -0.7660212471507179544, -0.6427876096865405842, -0.005961354470445141482 ) ) ;
#21349=VERTEX_POINT ( 'NONE', #48540 ) ;
#21350=VECTOR ( 'NONE', #26074, 1000.000000000000227 ) ;
#21351=VERTEX_POINT ( 'NONE', #53086 ) ;
#21352=VERTEX_POINT ( 'NONE', #13886 ) ;
#21353=VECTOR ( 'NONE', #11143, 1000.000000000000227 ) ;
#21354=EDGE_CURVE ( 'NONE', #16343, #547, #18998, .T. ) ;
#21355=CARTESIAN_POINT ( 'NONE',  ( 1.969897575278193980, 0.000000000000000000, 10.20639235748909890 ) ) ;
#21356=AXIS2_PLACEMENT_3D ( 'NONE', #47320, #52915, #5785 ) ;
#21357=DIRECTION ( 'NONE',  ( -0.5364919789714478471, 0.6444004775717705469, -0.5449076811759709926 ) ) ;
#21358=ORIENTED_EDGE ( 'NONE', *, *, #22608, .T. ) ;
#21360=EDGE_LOOP ( 'NONE', ( #12050, #25231, #10862, #43873 ) ) ;
#21361=LINE ( 'NONE', #51719, #43248 ) ;
#21362=FACE_OUTER_BOUND ( 'NONE', #20793, .T. ) ;
#21363=VECTOR ( 'NONE', #25238, 999.9999999999998863 ) ;
#21364=EDGE_CURVE ( 'NONE', #13391, #12878, #14464, .T. ) ;
#21365=EDGE_CURVE ( 'NONE', #48176, #14783, #1093, .T. ) ;
#21366=VERTEX_POINT ( 'NONE', #52781 ) ;
#21367=AXIS2_PLACEMENT_3D ( 'NONE', #1776, #23641, #27934 ) ;
#21368=DIRECTION ( 'NONE',  ( 0.5449076811759707706, 0.6444004775717708799, -0.5364919789714476250 ) ) ;
#21369=EDGE_LOOP ( 'NONE', ( #30840, #43667, #51426, #50320, #7839, #24491, #21052, #55924, #44420, #39875, #55330, #12686, #38419, #42308, #48450, #19436, #20797, #9705, #32663, #5853, #36046, #25677, #54638, #16106, #51685, #42957, #5458, #44763, #14521, #2425, #1088, #10158, #24538, #14507, #50578, #20981, #14576, #29972, #18704, #6573, #42783, #31270, #20783, #27623, #41767, #30453, #37209, #42503, #7757, #18129, #31606, #38529, #55354, #31558, #9211, #8082, #38206, #53783, #17196, #14683, #31810, #43297, #16148, #19670, #7050, #10317, #23383, #31771, #30671, #54959, #52578, #1264, #5116, #35658, #49124, #16280, #5154, #3776, #47758, #2022, #4155, #13805, #53906, #9854, #7509, #39294, #14698, #22419, #50610, #26041, #39512, #55026, #54869, #27570, #24295, #23701, #3124, #20198, #2511, #13790, #41552, #49317, #41710, #19664, #6329, #3942, #7511 ) ) ;
#21370=ADVANCED_FACE ( 'NONE', ( #27822 ), #31522, .F. ) ;
#21371=VECTOR ( 'NONE', #26790, 1000.000000000000227 ) ;
#21372=PLANE ( 'NONE',  #39161 ) ;
#21373=AXIS2_PLACEMENT_3D ( 'NONE', #24249, #19966, #50359 ) ;
#21374=CARTESIAN_POINT ( 'NONE',  ( -19.60912206198628027, -0.1191753592594197858, 4.398475361799976113 ) ) ;
#21375=ORIENTED_EDGE ( 'NONE', *, *, #6006, .T. ) ;
#21376=CARTESIAN_POINT ( 'NONE',  ( -24.26986129792355129, -0.1191753592594197858, 6.208864760408702388 ) ) ;
#21377=DIRECTION ( 'NONE',  ( -0.7660212471507179544, -0.6427876096865405842, -0.005961354470445141482 ) ) ;
#21378=FACE_OUTER_BOUND ( 'NONE', #32029, .T. ) ;
#21379=VERTEX_POINT ( 'NONE', #9659 ) ;
#21381=CARTESIAN_POINT ( 'NONE',  ( -15.40103151951671734, 0.000000000000000000, 12.95233060667165681 ) ) ;
#21382=FACE_OUTER_BOUND ( 'NONE', #34244, .T. ) ;
#21383=FACE_OUTER_BOUND ( 'NONE', #12497, .T. ) ;
#21384=DIRECTION ( 'NONE',  ( 0.5449076811759707706, 0.6444004775717708799, -0.5364919789714476250 ) ) ;
#21385=EDGE_CURVE ( 'NONE', #41167, #50834, #40853, .T. ) ;
#21386=VECTOR ( 'NONE', #43285, 999.9999999999998863 ) ;
#21387=LINE ( 'NONE', #48316, #3181 ) ;
#21388=ORIENTED_EDGE ( 'NONE', *, *, #16387, .F. ) ;
#21389=FACE_OUTER_BOUND ( 'NONE', #6653, .T. ) ;
#21390=VECTOR ( 'NONE', #48372, 1000.000000000000000 ) ;
#21391=CARTESIAN_POINT ( 'NONE',  ( -9.908141408373387193, -0.1191753592594197858, 10.77908512878318703 ) ) ;
#21392=EDGE_CURVE ( 'NONE', #8533, #28185, #53371, .T. ) ;
#21393=DIRECTION ( 'NONE',  ( 0.007781995580012663651, -3.146120232559066537E-19, -0.9999697198139514409 ) ) ;
#21395=DIRECTION ( 'NONE',  ( 0.6427681459581294776, -0.7660444431189769032, 0.005002170337467562802 ) ) ;
#21396=DIRECTION ( 'NONE',  ( 0.5364919789714477361, 0.6444004775717706579, 0.5449076811759711036 ) ) ;
#21398=ORIENTED_EDGE ( 'NONE', *, *, #24294, .T. ) ;
#21399=PLANE ( 'NONE',  #6252 ) ;
#21400=CARTESIAN_POINT ( 'NONE',  ( -13.50569345835905111, 0.000000000000000000, 8.239297380650791425 ) ) ;
#21401=EDGE_CURVE ( 'NONE', #41663, #41818, #28074, .T. ) ;
#21402=VECTOR ( 'NONE', #39476, 999.9999999999998863 ) ;
#21403=CARTESIAN_POINT ( 'NONE',  ( -14.93495759592298988, 0.000000000000000000, 12.77129166681078409 ) ) ;
#21404=EDGE_CURVE ( 'NONE', #13581, #9203, #27513, .T. ) ;
#21406=EDGE_LOOP ( 'NONE', ( #51558, #51716, #18003, #17645 ) ) ;
#21407=VECTOR ( 'NONE', #54454, 1000.000000000000227 ) ;
#21408=AXIS2_PLACEMENT_3D ( 'NONE', #1536, #53752, #35915 ) ;
#21411=CARTESIAN_POINT ( 'NONE',  ( -14.52268981044348450, -0.1191753592594179401, 6.654051572544311455 ) ) ;
#21412=CARTESIAN_POINT ( 'NONE',  ( -13.02225584137026893, 0.000000000000000000, 5.827061128909424070 ) ) ;
#21413=VECTOR ( 'NONE', #53015, 999.9999999999998863 ) ;
#21414=VECTOR ( 'NONE', #587, 999.9999999999998863 ) ;
#21415=PLANE ( 'NONE',  #26615 ) ;
#21416=VECTOR ( 'NONE', #35205, 1000.000000000000227 ) ;
#21417=CARTESIAN_POINT ( 'NONE',  ( -17.23519096270132422, -1.165603555308157846, 3.538865740624604683 ) ) ;
#21418=FACE_OUTER_BOUND ( 'NONE', #55014, .T. ) ;
#21419=ORIENTED_EDGE ( 'NONE', *, *, #52302, .F. ) ;
#21420=LINE ( 'NONE', #25656, #3871 ) ;
#21421=AXIS2_PLACEMENT_3D ( 'NONE', #27863, #15070, #10237 ) ;
#21422=VECTOR ( 'NONE', #53998, 1000.000000000000227 ) ;
#21423=LINE ( 'NONE', #25660, #51432 ) ;
#21424=ORIENTED_EDGE ( 'NONE', *, *, #5349, .F. ) ;
#21425=LINE ( 'NONE', #4644, #54663 ) ;
#21426=LINE ( 'NONE', #17155, #41317 ) ;
#21427=DIRECTION ( 'NONE',  ( -0.7660212471507179544, -0.6427876096865405842, -0.005961354470445141482 ) ) ;
#21428=ORIENTED_EDGE ( 'NONE', *, *, #39039, .F. ) ;
#21429=DIRECTION ( 'NONE',  ( 0.000000000000000000, -1.000000000000000000, 0.000000000000000000 ) ) ;
#21430=ORIENTED_EDGE ( 'NONE', *, *, #35440, .T. ) ;
#21431=VECTOR ( 'NONE', #6667, 999.9999999999998863 ) ;
#21432=EDGE_LOOP ( 'NONE', ( #7752, #12288, #12806, #41473 ) ) ;
#21434=ORIENTED_EDGE ( 'NONE', *, *, #37764, .F. ) ;
#21435=ORIENTED_EDGE ( 'NONE', *, *, #40211, .T. ) ;
#21436=PLANE ( 'NONE',  #52954 ) ;
#21437=AXIS2_PLACEMENT_3D ( 'NONE', #55240, #38192, #16619 ) ;
#21438=VERTEX_POINT ( 'NONE', #18735 ) ;
#21439=DIRECTION ( 'NONE',  ( 0.6427681459581294776, -0.7660444431189769032, 0.005002170337467562802 ) ) ;
#21440=EDGE_CURVE ( 'NONE', #5343, #47558, #45379, .T. ) ;
#21441=ORIENTED_EDGE ( 'NONE', *, *, #27498, .F. ) ;
#21442=LINE ( 'NONE', #7516, #15023 ) ;
#21443=AXIS2_PLACEMENT_3D ( 'NONE', #47367, #7636, #15873 ) ;
#21444=ORIENTED_EDGE ( 'NONE', *, *, #39773, .F. ) ;
#21445=LINE ( 'NONE', #35077, #11967 ) ;
#21446=ORIENTED_EDGE ( 'NONE', *, *, #11451, .T. ) ;
#21447=EDGE_CURVE ( 'NONE', #49405, #23911, #7320, .T. ) ;
#21449=AXIS2_PLACEMENT_3D ( 'NONE', #33954, #20629, #7856 ) ;
#21450=DIRECTION ( 'NONE',  ( -0.5449076811759708816, 0.6444004775717707689, 0.5364919789714475140 ) ) ;
#21451=DIRECTION ( 'NONE',  ( 0.000000000000000000, -1.000000000000000000, 0.000000000000000000 ) ) ;
#21452=PLANE ( 'NONE',  #49450 ) ;
#21453=LINE ( 'NONE', #38468, #35990 ) ;
#21454=PLANE ( 'NONE',  #17433 ) ;
#21455=ORIENTED_EDGE ( 'NONE', *, *, #12671, .F. ) ;
#21457=EDGE_LOOP ( 'NONE', ( #53700, #29628, #38588, #30122 ) ) ;
#21458=AXIS2_PLACEMENT_3D ( 'NONE', #7454, #17893, #54885 ) ;
#21459=DIRECTION ( 'NONE',  ( 0.5364919789714477361, 0.6444004775717706579, 0.5449076811759711036 ) ) ;
#21460=DIRECTION ( 'NONE',  ( -0.005961354470445682716, -0.6427876096865404731, 0.7660212471507180654 ) ) ;
#21462=DIRECTION ( 'NONE',  ( 0.6427681459581294776, -0.7660444431189769032, 0.005002170337467562802 ) ) ;
#21463=AXIS2_PLACEMENT_3D ( 'NONE', #40475, #18598, #6379 ) ;
#21464=DIRECTION ( 'NONE',  ( 0.007781995580012663651, 0.000000000000000000, -0.9999697198139515519 ) ) ;
#21465=DIRECTION ( 'NONE',  ( 0.007781995580012662783, 0.000000000000000000, -0.9999697198139514409 ) ) ;
#21466=DIRECTION ( 'NONE',  ( 0.000000000000000000, -1.000000000000000000, 0.000000000000000000 ) ) ;
#21467=ORIENTED_EDGE ( 'NONE', *, *, #1503, .T. ) ;
#21468=DIRECTION ( 'NONE',  ( -0.005961354470445682716, -0.6427876096865404731, 0.7660212471507180654 ) ) ;
#21469=DIRECTION ( 'NONE',  ( 0.005002170337468016433, -0.7660444431189770143, -0.6427681459581293666 ) ) ;
#21470=VERTEX_POINT ( 'NONE', #49914 ) ;
#21471=DIRECTION ( 'NONE',  ( 0.9999697198139515519, 0.000000000000000000, 0.007781995580013368816 ) ) ;
#21472=CARTESIAN_POINT ( 'NONE',  ( -18.70476884740427437, -5.051250379848162275, 12.23746159482404217 ) ) ;
#21473=CARTESIAN_POINT ( 'NONE',  ( -18.66354898467281132, 0.000000000000000000, 14.21960318569776582 ) ) ;
#21474=EDGE_CURVE ( 'NONE', #14373, #33629, #7608, .T. ) ;
#21475=FACE_OUTER_BOUND ( 'NONE', #33094, .T. ) ;
#21476=AXIS2_PLACEMENT_3D ( 'NONE', #8287, #55419, #21057 ) ;
#21477=VERTEX_POINT ( 'NONE', #54450 ) ;
#21479=VERTEX_POINT ( 'NONE', #37727 ) ;
#21480=DIRECTION ( 'NONE',  ( 0.005961354470445682716, -0.6427876096865404731, -0.7660212471507180654 ) ) ;
#21481=LINE ( 'NONE', #22591, #35867 ) ;
#21482=LINE ( 'NONE', #39345, #55081 ) ;
#21483=CARTESIAN_POINT ( 'NONE',  ( -27.99767448711536133, 0.000000000000000000, 7.557179307314289218 ) ) ;
#21484=AXIS2_PLACEMENT_3D ( 'NONE', #37682, #29435, #16099 ) ;
#21485=ADVANCED_FACE ( 'NONE', ( #42259 ), #46213, .F. ) ;
#21486=LINE ( 'NONE', #7870, #48441 ) ;
#21487=DIRECTION ( 'NONE',  ( 0.6246952433987894571, -0.7422098413412800966, -0.2426528472758541777 ) ) ;
#21488=DIRECTION ( 'NONE',  ( 0.007781995580012663651, -3.146120232559066537E-19, -0.9999697198139514409 ) ) ;
#21489=ORIENTED_EDGE ( 'NONE', *, *, #11801, .T. ) ;
#21490=LINE ( 'NONE', #54224, #28681 ) ;
#21491=VECTOR ( 'NONE', #2916, 1000.000000000000227 ) ;
#21492=LINE ( 'NONE', #17208, #36017 ) ;
#21493=ORIENTED_EDGE ( 'NONE', *, *, #11740, .T. ) ;
#21494=CARTESIAN_POINT ( 'NONE',  ( -16.81267852042391198, -0.1191753592594197858, 3.312241722634738039 ) ) ;
#21495=ORIENTED_EDGE ( 'NONE', *, *, #19735, .F. ) ;
#21496=CARTESIAN_POINT ( 'NONE',  ( -11.40636015113596180, 0.000000000000000000, 11.32142374880780089 ) ) ;
#21497=ORIENTED_EDGE ( 'NONE', *, *, #50659, .F. ) ;
#21498=VECTOR ( 'NONE', #51029, 1000.000000000000227 ) ;
#21499=EDGE_LOOP ( 'NONE', ( #42867, #54172, #27406, #45220 ) ) ;
#21501=ORIENTED_EDGE ( 'NONE', *, *, #41555, .F. ) ;
#21502=AXIS2_PLACEMENT_3D ( 'NONE', #1752, #27907, #49747 ) ;
#21503=ORIENTED_EDGE ( 'NONE', *, *, #7256, .T. ) ;
#21505=ORIENTED_EDGE ( 'NONE', *, *, #53064, .T. ) ;
#21506=DIRECTION ( 'NONE',  ( 0.5449076811759707706, 0.6444004775717708799, -0.5364919789714476250 ) ) ;
#21507=CARTESIAN_POINT ( 'NONE',  ( -21.50121238896663911, -5.051250379848161387, 13.32369523398927846 ) ) ;
#21508=EDGE_CURVE ( 'NONE', #41488, #28129, #41132, .T. ) ;
#21509=CARTESIAN_POINT ( 'NONE',  ( -16.81345671998191449, 0.000000000000000000, 3.412238694616132495 ) ) ;
#21510=VERTEX_POINT ( 'NONE', #28340 ) ;
#21511=ADVANCED_FACE ( 'NONE', ( #33456 ), #19557, .F. ) ;
#21512=FACE_OUTER_BOUND ( 'NONE', #19744, .T. ) ;
#21513=ORIENTED_EDGE ( 'NONE', *, *, #42117, .F. ) ;
#21514=CARTESIAN_POINT ( 'NONE',  ( -17.74404816805336793, 0.000000000000000000, 3.574322630375089460 ) ) ;
#21515=ORIENTED_EDGE ( 'NONE', *, *, #32132, .F. ) ;
#21516=ADVANCED_FACE ( 'NONE', ( #3056 ), #24635, .F. ) ;
#21517=EDGE_CURVE ( 'NONE', #15338, #30167, #24939, .T. ) ;
#21518=CARTESIAN_POINT ( 'NONE',  ( 2.072287782118878319, 0.000000000000000000, -2.950529333540147015 ) ) ;
#21520=CARTESIAN_POINT ( 'NONE',  ( -15.90223023344033315, -0.1191753592594212430, 4.796655320951466628 ) ) ;
#21522=DIRECTION ( 'NONE',  ( 0.5364919789714477361, 0.6444004775717706579, 0.5449076811759711036 ) ) ;
#21523=ORIENTED_EDGE ( 'NONE', *, *, #25878, .T. ) ;
#21524=CARTESIAN_POINT ( 'NONE',  ( -13.53673582514181106, 0.000000000000000000, 12.22817484722816772 ) ) ;
#21525=VECTOR ( 'NONE', #5767, 1000.000000000000227 ) ;
#21526=PLANE ( 'NONE',  #49316 ) ;
#21527=EDGE_CURVE ( 'NONE', #33755, #2289, #38001, .T. ) ;
#21528=CARTESIAN_POINT ( 'NONE',  ( -21.22173678941378228, -4.241740624735664156, 4.989230645525445595 ) ) ;
#21529=AXIS2_PLACEMENT_3D ( 'NONE', #7866, #12089, #37674 ) ;
#21530=DIRECTION ( 'NONE',  ( 0.8531650599175527594, 0.4028455766673922356, -0.3313982828793700652 ) ) ;
#21531=CARTESIAN_POINT ( 'NONE',  ( -24.26908309836554878, 0.000000000000000000, 6.108867788427308376 ) ) ;
#21532=LINE ( 'NONE', #29176, #2206 ) ;
#21534=CARTESIAN_POINT ( 'NONE',  ( -11.23781311569048924, 0.4483081953215033444, 1.032776604783083307 ) ) ;
#21535=EDGE_LOOP ( 'NONE', ( #8702, #21628, #51665, #41525 ) ) ;
#21536=PLANE ( 'NONE',  #15661 ) ;
#21537=ORIENTED_EDGE ( 'NONE', *, *, #55936, .T. ) ;
#21538=VECTOR ( 'NONE', #40459, 1000.000000000000227 ) ;
#21539=DIRECTION ( 'NONE',  ( 0.000000000000000000, -0.000000000000000000, -1.000000000000000000 ) ) ;
#21540=LINE ( 'NONE', #53024, #28693 ) ;
#21541=DIRECTION ( 'NONE',  ( 0.000000000000000000, -1.000000000000000000, 0.000000000000000000 ) ) ;
#21542=DIRECTION ( 'NONE',  ( -0.9999697198139514409, -0.000000000000000000, -0.007781995580013368816 ) ) ;
#21543=FACE_OUTER_BOUND ( 'NONE', #801, .T. ) ;
#21544=CARTESIAN_POINT ( 'NONE',  ( -27.06552663992790997, 0.000000000000000000, 7.195101427592543786 ) ) ;
#21546=LINE ( 'NONE', #29787, #32065 ) ;
#21548=ORIENTED_EDGE ( 'NONE', *, *, #29532, .T. ) ;
#21549=CARTESIAN_POINT ( 'NONE',  ( -11.87243407472968926, 0.000000000000000000, 11.50246268866867361 ) ) ;
#21550=CARTESIAN_POINT ( 'NONE',  ( -11.77243710274829525, -0.1191753592594197858, 11.50324088822667612 ) ) ;
#21551=CARTESIAN_POINT ( 'NONE',  ( -15.22435894240294552, 3.524445264749009876, 2.483141509683923775 ) ) ;
#21552=LINE ( 'NONE', #22398, #38172 ) ;
#21553=ADVANCED_FACE ( 'NONE', ( #15300 ), #24099, .F. ) ;
#21554=CARTESIAN_POINT ( 'NONE',  ( -18.67619601524082285, 0.000000000000000000, 3.936400510096834893 ) ) ;
#21555=CARTESIAN_POINT ( 'NONE',  ( -16.28776673239499928, 0.000000000000000000, 7.478982503527205061 ) ) ;
#21556=CARTESIAN_POINT ( 'NONE',  ( -17.99589520542714638, 1.257817950434005461, 5.935831502157483897 ) ) ;
#21557=ORIENTED_EDGE ( 'NONE', *, *, #24391, .F. ) ;
#21560=ORIENTED_EDGE ( 'NONE', *, *, #3618, .F. ) ;
#21561=ORIENTED_EDGE ( 'NONE', *, *, #29786, .F. ) ;
#21562=CARTESIAN_POINT ( 'NONE',  ( -9.974221960066742554, 0.000000000000000000, 6.420119759390041203 ) ) ;
#21563=ADVANCED_FACE ( 'NONE', ( #51036 ), #32610, .F. ) ;
#21564=ORIENTED_EDGE ( 'NONE', *, *, #1732, .T. ) ;
#21566=EDGE_CURVE ( 'NONE', #42380, #35539, #7072, .T. ) ;
#21567=AXIS2_PLACEMENT_3D ( 'NONE', #14152, #36280, #54160 ) ;
#21568=ORIENTED_EDGE ( 'NONE', *, *, #31203, .F. ) ;
#21569=ORIENTED_EDGE ( 'NONE', *, *, #53310, .T. ) ;
#21570=ORIENTED_EDGE ( 'NONE', *, *, #15087, .T. ) ;
#21571=DIRECTION ( 'NONE',  ( 0.005002170337468016433, -0.7660444431189770143, -0.6427681459581293666 ) ) ;
#21572=ORIENTED_EDGE ( 'NONE', *, *, #13722, .T. ) ;
#21573=CARTESIAN_POINT ( 'NONE',  ( -13.53673582514181106, 0.000000000000000000, 12.22817484722816772 ) ) ;
#21574=EDGE_CURVE ( 'NONE', #55289, #6087, #20934, .T. ) ;
#21575=PLANE ( 'NONE',  #55724 ) ;
#21576=CIRCLE ( 'NONE', #41507, 1.000000000000000444 ) ;
#21577=EDGE_CURVE ( 'NONE', #50902, #1435, #56161, .T. ) ;
#21578=ORIENTED_EDGE ( 'NONE', *, *, #25281, .T. ) ;
#21579=EDGE_LOOP ( 'NONE', ( #14439, #1851, #5619, #16692 ) ) ;
#21580=EDGE_CURVE ( 'NONE', #38002, #50681, #17835, .T. ) ;
#21581=DIRECTION ( 'NONE',  ( 0.007781995580012663651, -3.146120232559066537E-19, -0.9999697198139514409 ) ) ;
#21582=ORIENTED_EDGE ( 'NONE', *, *, #23918, .T. ) ;
#21583=LINE ( 'NONE', #25832, #31877 ) ;
#21585=ORIENTED_EDGE ( 'NONE', *, *, #15381, .F. ) ;
#21586=CARTESIAN_POINT ( 'NONE',  ( -19.27721902470766935, 3.848249166794008413, 10.68488013071350551 ) ) ;
#21587=EDGE_CURVE ( 'NONE', #22163, #19674, #17245, .T. ) ;
#21588=VERTEX_POINT ( 'NONE', #34566 ) ;
#21589=CARTESIAN_POINT ( 'NONE',  ( 2.072287782118878319, 0.000000000000000000, -2.950529333540147015 ) ) ;
#21590=EDGE_CURVE ( 'NONE', #37607, #12378, #43641, .T. ) ;
#21591=DIRECTION ( 'NONE',  ( -0.9999697198139514409, -0.000000000000000000, -0.007781995580013368816 ) ) ;
#21592=EDGE_LOOP ( 'NONE', ( #17482, #52223, #17934, #8348 ) ) ;
#21593=CARTESIAN_POINT ( 'NONE',  ( -16.28046222626843331, 0.000000000000000000, 6.540369153048884776 ) ) ;
#21594=DIRECTION ( 'NONE',  ( -0.005961354470445682716, -0.6427876096865404731, 0.7660212471507180654 ) ) ;
#21595=DIRECTION ( 'NONE',  ( 0.000000000000000000, -1.000000000000000000, 0.000000000000000000 ) ) ;
#21596=LINE ( 'NONE', #22138, #40121 ) ;
#21597=ORIENTED_EDGE ( 'NONE', *, *, #2237, .F. ) ;
#21598=CARTESIAN_POINT ( 'NONE',  ( -10.47421230394850866, 0.000000000000000000, 10.95934586908605723 ) ) ;
#21599=DIRECTION ( 'NONE',  ( 0.2426528472758541499, 0.7422098413412800966, 0.6246952433987894571 ) ) ;
#21600=CARTESIAN_POINT ( 'NONE',  ( -20.83174675134727138, 0.7721120973665036580, 4.749055200455086556 ) ) ;
#21601=DIRECTION ( 'NONE',  ( 0.5364919789714477361, 0.6444004775717706579, 0.5449076811759711036 ) ) ;
#21602=CARTESIAN_POINT ( 'NONE',  ( -20.26176469941677993, 0.000000000000000000, 14.76116360616437895 ) ) ;
#21603=DIRECTION ( 'NONE',  ( -0.7660212471507179544, -0.6427876096865405842, -0.005961354470445141482 ) ) ;
#21604=FACE_OUTER_BOUND ( 'NONE', #474, .T. ) ;
#21605=DIRECTION ( 'NONE',  ( -0.005002170337468016433, -0.7660444431189770143, 0.6427681459581293666 ) ) ;
#21606=DIRECTION ( 'NONE',  ( 0.007781995580012663651, 0.000000000000000000, -0.9999697198139515519 ) ) ;
#21607=VERTEX_POINT ( 'NONE', #35166 ) ;
#21609=DIRECTION ( 'NONE',  ( 0.007781995580012663651, -3.146120232559066537E-19, -0.9999697198139514409 ) ) ;
#21610=ORIENTED_EDGE ( 'NONE', *, *, #4327, .T. ) ;
#21611=PLANE ( 'NONE',  #12980 ) ;
#21613=VECTOR ( 'NONE', #36077, 1000.000000000000227 ) ;
#21614=CARTESIAN_POINT ( 'NONE',  ( -13.56754953521377161, -0.1191753592594196748, 3.337496066760455182 ) ) ;
#21615=ADVANCED_FACE ( 'NONE', ( #26328 ), #16693, .F. ) ;
#21616=LINE ( 'NONE', #55976, #38735 ) ;
#21617=LINE ( 'NONE', #3704, #51043 ) ;
#21618=ORIENTED_EDGE ( 'NONE', *, *, #8487, .T. ) ;
#21619=VERTEX_POINT ( 'NONE', #51615 ) ;
#21621=PLANE ( 'NONE',  #28593 ) ;
#21623=EDGE_CURVE ( 'NONE', #16632, #7363, #8763, .T. ) ;
#21624=EDGE_CURVE ( 'NONE', #2289, #17587, #38850, .T. ) ;
#21625=DIRECTION ( 'NONE',  ( 0.000000000000000000, -0.000000000000000000, -1.000000000000000000 ) ) ;
#21626=ORIENTED_EDGE ( 'NONE', *, *, #51527, .F. ) ;
#21627=DIRECTION ( 'NONE',  ( 0.5449076811759707706, 0.6444004775717708799, -0.5364919789714476250 ) ) ;
#21628=ORIENTED_EDGE ( 'NONE', *, *, #16760, .F. ) ;
#21629=CARTESIAN_POINT ( 'NONE',  ( -17.75502971379410511, -0.1191753592594194250, 4.043572267363897410 ) ) ;
#21630=EDGE_CURVE ( 'NONE', #26641, #32939, #39407, .T. ) ;
#21632=ORIENTED_EDGE ( 'NONE', *, *, #8064, .T. ) ;
#21633=ORIENTED_EDGE ( 'NONE', *, *, #30945, .F. ) ;
#21634=CARTESIAN_POINT ( 'NONE',  ( -1.905187828007888884, 6.291258001618519557, 3.958413228513044668 ) ) ;
#21635=DIRECTION ( 'NONE',  ( 0.000000000000000000, -1.000000000000000000, 0.000000000000000000 ) ) ;
#21636=DIRECTION ( 'NONE',  ( 0.005961354470445682716, -0.6427876096865404731, -0.7660212471507180654 ) ) ;
#21637=LINE ( 'NONE', #26175, #11240 ) ;
#21638=ADVANCED_FACE ( 'NONE', ( #51882 ), #13560, .F. ) ;
#21639=EDGE_LOOP ( 'NONE', ( #32957, #46907, #43980, #29992 ) ) ;
#21640=ORIENTED_EDGE ( 'NONE', *, *, #2682, .T. ) ;
#21642=VERTEX_POINT ( 'NONE', #3902 ) ;
#21643=CARTESIAN_POINT ( 'NONE',  ( -17.34997331854206237, -0.1941918491731542684, 3.614444224982700682 ) ) ;
#21644=EDGE_CURVE ( 'NONE', #55726, #55546, #188, .T. ) ;
#21645=VERTEX_POINT ( 'NONE', #25778 ) ;
#21646=DIRECTION ( 'NONE',  ( 0.000000000000000000, -1.000000000000000000, 0.000000000000000000 ) ) ;
#21649=LINE ( 'NONE', #43491, #2231 ) ;
#21650=ADVANCED_FACE ( 'NONE', ( #4218 ), #21536, .F. ) ;
#21651=AXIS2_PLACEMENT_3D ( 'NONE', #9148, #38413, #26462 ) ;
#21652=VERTEX_POINT ( 'NONE', #1874 ) ;
#21653=LINE ( 'NONE', #38697, #27735 ) ;
#21654=EDGE_LOOP ( 'NONE', ( #21493, #33086, #20028, #2265 ) ) ;
#21655=LINE ( 'NONE', #26191, #54467 ) ;
#21656=ORIENTED_EDGE ( 'NONE', *, *, #17398, .F. ) ;
#21657=CARTESIAN_POINT ( 'NONE',  ( -17.19692215154019621, 0.000000000000000000, 4.886582757186834769 ) ) ;
#21658=DIRECTION ( 'NONE',  ( -0.5364919789714478471, 0.6444004775717705469, -0.5449076811759709926 ) ) ;
#21659=FACE_OUTER_BOUND ( 'NONE', #5548, .T. ) ;
#21660=ORIENTED_EDGE ( 'NONE', *, *, #25254, .T. ) ;
#21661=CARTESIAN_POINT ( 'NONE',  ( -23.33849165029409889, 0.000000000000000000, 5.946783852668351855 ) ) ;
#21662=FACE_OUTER_BOUND ( 'NONE', #21192, .T. ) ;
#21663=DIRECTION ( 'NONE',  ( 0.7660212471507180654, -0.6427876096865404731, 0.005961354470445141482 ) ) ;
#21664=DIRECTION ( 'NONE',  ( -0.9999697198139514409, -0.000000000000000000, -0.007781995580013368816 ) ) ;
#21665=CARTESIAN_POINT ( 'NONE',  ( -13.50974395553640761, 2.553033558614007603, 6.318927477965895712 ) ) ;
#21666=CARTESIAN_POINT ( 'NONE',  ( -15.40103151951671734, 0.000000000000000000, 12.95233060667165681 ) ) ;
#21667=PLANE ( 'NONE',  #24027 ) ;
#21668=ORIENTED_EDGE ( 'NONE', *, *, #28923, .F. ) ;
#21669=CARTESIAN_POINT ( 'NONE',  ( -15.83750010308032685, 0.000000000000000000, 9.329146931584036295 ) ) ;
#21671=LINE ( 'NONE', #38984, #54104 ) ;
#21672=ORIENTED_EDGE ( 'NONE', *, *, #36461, .T. ) ;
#21673=LINE ( 'NONE', #9437, #38383 ) ;
#21674=LINE ( 'NONE', #12862, #47662 ) ;
#21675=ORIENTED_EDGE ( 'NONE', *, *, #22066, .T. ) ;
#21676=EDGE_CURVE ( 'NONE', #26864, #4402, #775, .T. ) ;
#21677=DIRECTION ( 'NONE',  ( 0.007781995580012663651, 0.000000000000000000, -0.9999697198139515519 ) ) ;
#21678=FACE_OUTER_BOUND ( 'NONE', #24680, .T. ) ;
#21679=ADVANCED_FACE ( 'NONE', ( #23215 ), #27449, .F. ) ;
#21680=CARTESIAN_POINT ( 'NONE',  ( -11.17388681363777181, 0.000000000000000000, 7.149447829717543890 ) ) ;
#21682=ORIENTED_EDGE ( 'NONE', *, *, #54678, .F. ) ;
#21683=ORIENTED_EDGE ( 'NONE', *, *, #41885, .F. ) ;
#21684=ADVANCED_FACE ( 'NONE', ( #31462 ), #5589, .F. ) ;
#21685=LINE ( 'NONE', #13992, #22177 ) ;
#21686=PLANE ( 'NONE',  #1382 ) ;
#21687=DIRECTION ( 'NONE',  ( 0.6427681459581294776, -0.7660444431189769032, 0.005002170337467562802 ) ) ;
#21688=EDGE_CURVE ( 'NONE', #45145, #27973, #36529, .T. ) ;
#21689=ADVANCED_FACE ( 'NONE', ( #39951 ), #26917, .F. ) ;
#21690=ADVANCED_FACE ( 'NONE', ( #9874 ), #13827, .F. ) ;
#21691=DIRECTION ( 'NONE',  ( 0.005002170337468016433, -0.7660444431189770143, -0.6427681459581293666 ) ) ;
#21692=DIRECTION ( 'NONE',  ( 0.5364919789714477361, 0.6444004775717706579, 0.5449076811759711036 ) ) ;
#21693=CARTESIAN_POINT ( 'NONE',  ( 2.072287782118878319, 0.000000000000000000, -2.950529333540147015 ) ) ;
#21694=ORIENTED_EDGE ( 'NONE', *, *, #32776, .F. ) ;
#21695=EDGE_CURVE ( 'NONE', #28180, #40645, #27176, .T. ) ;
#21696=CARTESIAN_POINT ( 'NONE',  ( -11.87243407472968926, 0.000000000000000000, 11.50246268866867361 ) ) ;
#21697=LINE ( 'NONE', #35055, #34219 ) ;
#21698=ORIENTED_EDGE ( 'NONE', *, *, #26350, .T. ) ;
#21699=CARTESIAN_POINT ( 'NONE',  ( -27.06552663992790997, 0.000000000000000000, 7.195101427592543786 ) ) ;
#21702=ORIENTED_EDGE ( 'NONE', *, *, #40617, .F. ) ;
#21703=CARTESIAN_POINT ( 'NONE',  ( -18.86354292863559579, 0.000000000000000000, 14.21804678658176080 ) ) ;
#21704=ORIENTED_EDGE ( 'NONE', *, *, #50385, .T. ) ;
#21705=EDGE_CURVE ( 'NONE', #3673, #44974, #10130, .T. ) ;
#21706=EDGE_LOOP ( 'NONE', ( #12912, #11255, #3955, #25594 ) ) ;
#21707=VERTEX_POINT ( 'NONE', #19196 ) ;
#21708=EDGE_CURVE ( 'NONE', #32088, #42922, #23484, .T. ) ;
#21709=ORIENTED_EDGE ( 'NONE', *, *, #32964, .T. ) ;
#21710=PLANE ( 'NONE',  #39341 ) ;
#21711=EDGE_LOOP ( 'NONE', ( #46069, #48969, #9190, #40226 ) ) ;
#21713=EDGE_CURVE ( 'NONE', #27123, #2, #36268, .T. ) ;
#21714=ORIENTED_EDGE ( 'NONE', *, *, #44121, .F. ) ;
#21715=LINE ( 'NONE', #51538, #23182 ) ;
#21716=VERTEX_POINT ( 'NONE', #26609 ) ;
#21717=DIRECTION ( 'NONE',  ( 0.5364919789714477361, 0.6444004775717706579, 0.5449076811759711036 ) ) ;
#21718=VERTEX_POINT ( 'NONE', #53567 ) ;
#21719=EDGE_CURVE ( 'NONE', #42734, #21652, #5053, .T. ) ;
#21720=DIRECTION ( 'NONE',  ( 0.6246952433987893460, 0.7422098413412802076, -0.2426528472758539279 ) ) ;
#21721=CARTESIAN_POINT ( 'NONE',  ( -9.844706253474519997, -0.1191753592594185784, 2.627803954389000829 ) ) ;
#21722=LINE ( 'NONE', #47554, #46726 ) ;
#21723=DIRECTION ( 'NONE',  ( -0.5364919789714478471, 0.6444004775717705469, -0.5449076811759709926 ) ) ;
#21724=FACE_OUTER_BOUND ( 'NONE', #54839, .T. ) ;
#21725=ORIENTED_EDGE ( 'NONE', *, *, #289, .T. ) ;
#21727=ORIENTED_EDGE ( 'NONE', *, *, #33743, .T. ) ;
#21728=DIRECTION ( 'NONE',  ( -0.3313982828793700652, 0.4028455766673916250, -0.8531650599175529814 ) ) ;
#21729=DIRECTION ( 'NONE',  ( 0.7660212471507180654, -0.6427876096865404731, 0.005961354470445141482 ) ) ;
#21730=CARTESIAN_POINT ( 'NONE',  ( -19.66652065306912789, -1.813211359398156919, 7.296864978363813314 ) ) ;
#21731=CARTESIAN_POINT ( 'NONE',  ( -10.94028622754223967, 0.000000000000000000, 11.14038480894692995 ) ) ;
#21732=CARTESIAN_POINT ( 'NONE',  ( -17.93139508144814442, 0.000000000000000000, 13.85596890686001537 ) ) ;
#21733=PLANE ( 'NONE',  #35029 ) ;
#21735=CARTESIAN_POINT ( 'NONE',  ( -19.60834386242827776, 0.000000000000000000, 4.298478389818581213 ) ) ;
#21736=CARTESIAN_POINT ( 'NONE',  ( -14.90535225589287549, 0.000000000000000000, 8.967069051862290863 ) ) ;
#21737=VERTEX_POINT ( 'NONE', #31727 ) ;
#21738=LINE ( 'NONE', #33953, #5283 ) ;
#21739=DIRECTION ( 'NONE',  ( 0.5449076811759707706, 0.6444004775717708799, -0.5364919789714476250 ) ) ;
#21741=LINE ( 'NONE', #4433, #29570 ) ;
#21742=CARTESIAN_POINT ( 'NONE',  ( -14.93495759592298988, 0.000000000000000000, 12.77129166681078409 ) ) ;
#21743=VERTEX_POINT ( 'NONE', #44774 ) ;
#21744=ORIENTED_EDGE ( 'NONE', *, *, #23803, .T. ) ;
#21745=CARTESIAN_POINT ( 'NONE',  ( 2.072287782118878319, 0.000000000000000000, -2.950529333540147015 ) ) ;
#21746=FACE_OUTER_BOUND ( 'NONE', #2029, .T. ) ;
#21747=CARTESIAN_POINT ( 'NONE',  ( -9.808144436391993182, 0.000000000000000000, 10.77986332834118777 ) ) ;
#21748=EDGE_CURVE ( 'NONE', #32511, #14988, #9288, .T. ) ;
#21749=EDGE_CURVE ( 'NONE', #25259, #695, #5332, .T. ) ;
#21750=LINE ( 'NONE', #13240, #23744 ) ;
#21751=DIRECTION ( 'NONE',  ( -0.9999697198139514409, -0.000000000000000000, -0.007781995580013368816 ) ) ;
#21752=EDGE_CURVE ( 'NONE', #39181, #9112, #6182, .T. ) ;
#21753=DIRECTION ( 'NONE',  ( 0.5364919789714477361, 0.6444004775717706579, 0.5449076811759711036 ) ) ;
#21754=FACE_OUTER_BOUND ( 'NONE', #46765, .T. ) ;
#21755=ORIENTED_EDGE ( 'NONE', *, *, #51872, .T. ) ;
#21756=CARTESIAN_POINT ( 'NONE',  ( -15.10957658656220737, 4.495856970884013037, 2.407563025325826445 ) ) ;
#21757=PLANE ( 'NONE',  #30575 ) ;
#21758=ORIENTED_EDGE ( 'NONE', *, *, #35861, .T. ) ;
#21759=FACE_OUTER_BOUND ( 'NONE', #2356, .T. ) ;
#21760=ORIENTED_EDGE ( 'NONE', *, *, #14952, .T. ) ;
#21761=LINE ( 'NONE', #39076, #17727 ) ;
#21762=VERTEX_POINT ( 'NONE', #35704 ) ;
#21763=ORIENTED_EDGE ( 'NONE', *, *, #19730, .F. ) ;
#21764=VERTEX_POINT ( 'NONE', #36012 ) ;
#21765=EDGE_LOOP ( 'NONE', ( #46450, #12230, #45432, #13338, #28539 ) ) ;
#21766=ORIENTED_EDGE ( 'NONE', *, *, #43366, .F. ) ;
#21767=VERTEX_POINT ( 'NONE', #53021 ) ;
#21768=CARTESIAN_POINT ( 'NONE',  ( -10.20725032438692992, 0.000000000000000000, 2.355653510902626646 ) ) ;
#21769=CARTESIAN_POINT ( 'NONE',  ( -9.837237150914331707, -0.1191753592594208266, 1.668040315669363949 ) ) ;
#21770=LINE ( 'NONE', #39375, #41255 ) ;
#21771=VERTEX_POINT ( 'NONE', #44483 ) ;
#21772=DIRECTION ( 'NONE',  ( 0.007781995580012662783, 0.000000000000000000, -0.9999697198139514409 ) ) ;
#21773=VERTEX_POINT ( 'NONE', #49030 ) ;
#21774=ORIENTED_EDGE ( 'NONE', *, *, #44760, .T. ) ;
#21775=EDGE_CURVE ( 'NONE', #12727, #19669, #32816, .T. ) ;
#21776=DIRECTION ( 'NONE',  ( -0.9999697198139514409, -0.000000000000000000, -0.007781995580013368816 ) ) ;
#21777=ADVANCED_FACE ( 'NONE', ( #50438 ), #28025, .F. ) ;
#21779=ADVANCED_FACE ( 'NONE', ( #41884 ), #24313, .F. ) ;
#21780=VERTEX_POINT ( 'NONE', #33121 ) ;
#21781=DIRECTION ( 'NONE',  ( 0.5449076811759707706, 0.6444004775717708799, -0.5364919789714476250 ) ) ;
#21782=VERTEX_POINT ( 'NONE', #37351 ) ;
#21783=CARTESIAN_POINT ( 'NONE',  ( -19.15181445782265257, -0.1191753592594170796, 4.402034235317630717 ) ) ;
#21784=ADVANCED_FACE ( 'NONE', ( #24570 ), #20029, .F. ) ;
#21785=CARTESIAN_POINT ( 'NONE',  ( -11.20636620717317378, 0.000000000000000000, 11.32298014792380414 ) ) ;
#21786=VECTOR ( 'NONE', #6719, 999.9999999999998863 ) ;
#21787=DIRECTION ( 'NONE',  ( -0.7660212471507179544, -0.6427876096865405842, -0.005961354470445141482 ) ) ;
#21788=CARTESIAN_POINT ( 'NONE',  ( -17.74404816805336793, 0.000000000000000000, 3.574322630375089460 ) ) ;
#21790=CARTESIAN_POINT ( 'NONE',  ( -19.72872274022425643, 0.000000000000000000, 5.974875909004076391 ) ) ;
#21791=DIRECTION ( 'NONE',  ( 0.5449076811759707706, 0.6444004775717708799, -0.5364919789714476250 ) ) ;
#21793=ORIENTED_EDGE ( 'NONE', *, *, #46284, .F. ) ;
#21795=LINE ( 'NONE', #55586, #12030 ) ;
#21797=LINE ( 'NONE', #9028, #43547 ) ;
#21799=LINE ( 'NONE', #25787, #38590 ) ;
#21800=DIRECTION ( 'NONE',  ( 0.9999697198139515519, 0.000000000000000000, 0.007781995580013368816 ) ) ;
#21801=DIRECTION ( 'NONE',  ( 0.007781995580012663651, -3.146120232559066537E-19, -0.9999697198139514409 ) ) ;
#21804=CARTESIAN_POINT ( 'NONE',  ( 2.072287782118878319, 0.000000000000000000, -2.950529333540147015 ) ) ;
#21805=EDGE_CURVE ( 'NONE', #10121, #41600, #15777, .T. ) ;
#21806=CARTESIAN_POINT ( 'NONE',  ( -14.88655153574517520, 0.000000000000000000, 6.551216888352914047 ) ) ;
#21807=EDGE_CURVE ( 'NONE', #27886, #48080, #28860, .T. ) ;
#21808=DIRECTION ( 'NONE',  ( 0.9999697198139515519, 0.000000000000000000, 0.007781995580013368816 ) ) ;
#21809=DIRECTION ( 'NONE',  ( 0.005961354470445682716, -0.6427876096865404731, -0.7660212471507180654 ) ) ;
#21810=PLANE ( 'NONE',  #20606 ) ;
#21811=EDGE_CURVE ( 'NONE', #45157, #41193, #2704, .T. ) ;
#21812=EDGE_CURVE ( 'NONE', #49751, #46200, #36835, .T. ) ;
#21813=PLANE ( 'NONE',  #30154 ) ;
#21814=DIRECTION ( 'NONE',  ( 0.007781995580012662783, 0.000000000000000000, -0.9999697198139514409 ) ) ;
#21815=FACE_OUTER_BOUND ( 'NONE', #7737, .T. ) ;
#21816=ORIENTED_EDGE ( 'NONE', *, *, #37957, .F. ) ;
#21817=DIRECTION ( 'NONE',  ( 0.9999697198139515519, 0.000000000000000000, 0.007781995580013368816 ) ) ;
#21818=ORIENTED_EDGE ( 'NONE', *, *, #56142, .T. ) ;
#21819=ADVANCED_FACE ( 'NONE', ( #7264 ), #2455, .F. ) ;
#21820=VECTOR ( 'NONE', #6310, 999.9999999999998863 ) ;
#21821=ORIENTED_EDGE ( 'NONE', *, *, #32626, .F. ) ;
#21822=ORIENTED_EDGE ( 'NONE', *, *, #30660, .T. ) ;
#21823=ORIENTED_EDGE ( 'NONE', *, *, #2464, .T. ) ;
#21824=ORIENTED_EDGE ( 'NONE', *, *, #19158, .F. ) ;
#21825=DIRECTION ( 'NONE',  ( 0.5449076811759707706, 0.6444004775717708799, -0.5364919789714476250 ) ) ;
#21826=CARTESIAN_POINT ( 'NONE',  ( -13.93715936752603213, 0.000000000000000000, 3.973280789084581599 ) ) ;
#21827=ORIENTED_EDGE ( 'NONE', *, *, #17303, .T. ) ;
#21828=ORIENTED_EDGE ( 'NONE', *, *, #2563, .T. ) ;
#21829=DIRECTION ( 'NONE',  ( 0.007781995580012663651, 0.000000000000000000, -0.9999697198139515519 ) ) ;
#21830=ORIENTED_EDGE ( 'NONE', *, *, #7959, .T. ) ;
#21832=LINE ( 'NONE', #43161, #41438 ) ;
#21833=ORIENTED_EDGE ( 'NONE', *, *, #18834, .T. ) ;
#21834=DIRECTION ( 'NONE',  ( -0.005961354470445682716, -0.6427876096865404731, 0.7660212471507180654 ) ) ;
#21835=EDGE_LOOP ( 'NONE', ( #22784, #31117, #31301, #19341 ) ) ;
#21836=VECTOR ( 'NONE', #14510, 1000.000000000000227 ) ;
#21837=LINE ( 'NONE', #29824, #3754 ) ;
#21838=ADVANCED_FACE ( 'NONE', ( #19776 ), #32562, .F. ) ;
#21839=CARTESIAN_POINT ( 'NONE',  ( -13.93009360612618508, 0.000000000000000000, 3.065345623274078779 ) ) ;
#21840=ORIENTED_EDGE ( 'NONE', *, *, #15012, .F. ) ;
#21841=CARTESIAN_POINT ( 'NONE',  ( -20.54204810873173415, 0.000000000000000000, 4.860550213503115558 ) ) ;
#21842=CARTESIAN_POINT ( 'NONE',  ( -14.40699345105622697, 2.553033558614008047, 2.196642114320274786 ) ) ;
#21843=CARTESIAN_POINT ( 'NONE',  ( -14.96720833274759244, -0.1191753592594192307, 4.065267737971954176 ) ) ;
#21844=ORIENTED_EDGE ( 'NONE', *, *, #11879, .F. ) ;
#21845=LINE ( 'NONE', #8521, #19236 ) ;
#21846=EDGE_LOOP ( 'NONE', ( #38517, #30804, #19608, #36242, #37056 ) ) ;
#21848=VECTOR ( 'NONE', #39162, 999.9999999999998863 ) ;
#21849=CARTESIAN_POINT ( 'NONE',  ( -15.86710544311044302, 0.000000000000000000, 13.13336954653252953 ) ) ;
#21850=CARTESIAN_POINT ( 'NONE',  ( -29.86352658060627618, 0.000000000000000000, 8.481329010720569883 ) ) ;
#21851=LINE ( 'NONE', #38913, #20359 ) ;
#21852=LINE ( 'NONE', #5393, #51356 ) ;
#21853=CARTESIAN_POINT ( 'NONE',  ( -9.342070512798265725, 0.000000000000000000, 10.59882438848031505 ) ) ;
#21854=EDGE_CURVE ( 'NONE', #36639, #16314, #49613, .T. ) ;
#21856=DIRECTION ( 'NONE',  ( 0.005961354470445682716, -0.6427876096865404731, -0.7660212471507180654 ) ) ;
#21857=ADVANCED_FACE ( 'NONE', ( #23742 ), #41066, .F. ) ;
#21858=AXIS2_PLACEMENT_3D ( 'NONE', #1341, #6727, #6452 ) ;
#21859=DIRECTION ( 'NONE',  ( 0.5364919789714477361, 0.6444004775717706579, 0.5449076811759711036 ) ) ;
#21860=CARTESIAN_POINT ( 'NONE',  ( -19.96228687206401631, 0.2864062442990046309, 5.105392700718557109 ) ) ;
#21862=ORIENTED_EDGE ( 'NONE', *, *, #21566, .F. ) ;
#21863=DIRECTION ( 'NONE',  ( -0.005002170337468016433, -0.7660444431189770143, 0.6427681459581293666 ) ) ;
#21865=CARTESIAN_POINT ( 'NONE',  ( -18.95841281422621094, -0.1191753592594164968, 8.835524169308294873 ) ) ;
#21866=CARTESIAN_POINT ( 'NONE',  ( -11.93265391726099445, -1.489407457353155717, 3.761351127055128973 ) ) ;
#21867=EDGE_CURVE ( 'NONE', #34742, #53438, #45600, .T. ) ;
#21868=DIRECTION ( 'NONE',  ( 0.5364919789714477361, 0.6444004775717706579, 0.5449076811759711036 ) ) ;
#21869=LINE ( 'NONE', #51434, #52304 ) ;
#21870=EDGE_CURVE ( 'NONE', #24071, #10102, #50134, .T. ) ;
#21871=CARTESIAN_POINT ( 'NONE',  ( -13.73672976910459909, 0.000000000000000000, 12.22661844811216270 ) ) ;
#21872=ORIENTED_EDGE ( 'NONE', *, *, #28139, .F. ) ;
#21873=ORIENTED_EDGE ( 'NONE', *, *, #51382, .F. ) ;
#21874=FACE_OUTER_BOUND ( 'NONE', #23141, .T. ) ;
#21875=CARTESIAN_POINT ( 'NONE',  ( -15.87975247367846166, 0.000000000000000000, 2.850166870931599927 ) ) ;
#21877=DIRECTION ( 'NONE',  ( 0.007781995580012663651, 0.000000000000000000, -0.9999697198139515519 ) ) ;
#21878=EDGE_CURVE ( 'NONE', #34403, #31401, #28571, .T. ) ;
#21879=VECTOR ( 'NONE', #21868, 999.9999999999998863 ) ;
#21880=AXIS2_PLACEMENT_3D ( 'NONE', #34086, #38902, #4530 ) ;
#21881=ORIENTED_EDGE ( 'NONE', *, *, #36688, .T. ) ;
#21882=FACE_OUTER_BOUND ( 'NONE', #17185, .T. ) ;
#21883=EDGE_LOOP ( 'NONE', ( #51777, #4075, #32999, #37154 ) ) ;
#21884=CARTESIAN_POINT ( 'NONE',  ( -12.33850799832341849, 0.000000000000000000, 11.68350162852954632 ) ) ;
#21885=EDGE_CURVE ( 'NONE', #1428, #12623, #55512, .T. ) ;
#21886=ORIENTED_EDGE ( 'NONE', *, *, #5751, .F. ) ;
#21887=ORIENTED_EDGE ( 'NONE', *, *, #34669, .F. ) ;
#21888=ORIENTED_EDGE ( 'NONE', *, *, #37856, .T. ) ;
#21889=DIRECTION ( 'NONE',  ( -0.005002170337468016433, -0.7660444431189770143, 0.6427681459581293666 ) ) ;
#21890=CARTESIAN_POINT ( 'NONE',  ( -20.54049170961573267, 0.000000000000000000, 4.660556269540326646 ) ) ;
#21891=CARTESIAN_POINT ( 'NONE',  ( -17.33903557990779021, -0.1159828484229830647, 9.953443831026842048 ) ) ;
#21892=DIRECTION ( 'NONE',  ( -0.8531650599175527594, 0.4028455766673922356, 0.3313982828793700652 ) ) ;
#21893=ORIENTED_EDGE ( 'NONE', *, *, #39223, .F. ) ;
#21894=VERTEX_POINT ( 'NONE', #26267 ) ;
#21895=VECTOR ( 'NONE', #14184, 999.9999999999998863 ) ;
#21896=ORIENTED_EDGE ( 'NONE', *, *, #37981, .F. ) ;
#21897=CARTESIAN_POINT ( 'NONE',  ( -31.72782227498118601, 0.000000000000000000, 9.205484770164058972 ) ) ;
#21898=EDGE_LOOP ( 'NONE', ( #21881, #2597, #169, #12802 ) ) ;
#21899=CARTESIAN_POINT ( 'NONE',  ( -20.98941955928877334, 2.067327705546508021, 4.768976514551538592 ) ) ;
#21900=ORIENTED_EDGE ( 'NONE', *, *, #10574, .T. ) ;
#21901=CARTESIAN_POINT ( 'NONE',  ( -18.19747506107908563, 0.000000000000000000, 14.03856424583689311 ) ) ;
#21902=DIRECTION ( 'NONE',  ( 0.000000000000000000, -0.000000000000000000, -1.000000000000000000 ) ) ;
#21903=VERTEX_POINT ( 'NONE', #3566 ) ;
#21904=DIRECTION ( 'NONE',  ( 0.005961354470445682716, -0.6427876096865404731, -0.7660212471507180654 ) ) ;
#21905=EDGE_CURVE ( 'NONE', #21764, #38457, #47014, .T. ) ;
#21906=ORIENTED_EDGE ( 'NONE', *, *, #45337, .F. ) ;
#21907=PLANE ( 'NONE',  #2865 ) ;
#21908=VERTEX_POINT ( 'NONE', #43577 ) ;
#21910=DIRECTION ( 'NONE',  ( -0.005002170337468016433, -0.7660444431189770143, 0.6427681459581293666 ) ) ;
#21911=CARTESIAN_POINT ( 'NONE',  ( -9.034769606752719895, 0.000000000000000000, 5.119428529189977262 ) ) ;
#21912=ORIENTED_EDGE ( 'NONE', *, *, #12821, .T. ) ;
#21913=AXIS2_PLACEMENT_3D ( 'NONE', #436, #43880, #38502 ) ;
#21914=CARTESIAN_POINT ( 'NONE',  ( -13.16292975041053026, -4.565544526780660917, 9.287697036052362520 ) ) ;
#21915=VECTOR ( 'NONE', #20925, 999.9999999999998863 ) ;
#21916=FACE_OUTER_BOUND ( 'NONE', #1125, .T. ) ;
#21917=DIRECTION ( 'NONE',  ( -0.5449076811759708816, 0.6444004775717707689, 0.5364919789714475140 ) ) ;
#21918=DIRECTION ( 'NONE',  ( 0.000000000000000000, -0.000000000000000000, -1.000000000000000000 ) ) ;
#21919=PLANE ( 'NONE',  #45789 ) ;
#21920=DIRECTION ( 'NONE',  ( 0.9999697198139515519, 0.000000000000000000, 0.007781995580013368816 ) ) ;
#21921=EDGE_CURVE ( 'NONE', #53352, #12064, #20873, .T. ) ;
#21922=SURFACE_SIDE_STYLE ('',( #52027 ) ) ;
#21923=VECTOR ( 'NONE', #16945, 1000.000000000000227 ) ;
#21924=EDGE_LOOP ( 'NONE', ( #37535, #46259, #10999, #14838 ) ) ;
#21925=LINE ( 'NONE', #55738, #28895 ) ;
#21926=FACE_OUTER_BOUND ( 'NONE', #48298, .T. ) ;
#21927=LINE ( 'NONE', #27305, #44130 ) ;
#21928=ORIENTED_EDGE ( 'NONE', *, *, #41738, .T. ) ;
#21929=CARTESIAN_POINT ( 'NONE',  ( -18.19747506107908563, 0.000000000000000000, 14.03856424583689311 ) ) ;
#21930=CARTESIAN_POINT ( 'NONE',  ( -17.36532418587302473, -0.1191753592594177458, 13.67570816655714516 ) ) ;
#21931=ORIENTED_EDGE ( 'NONE', *, *, #54485, .T. ) ;
#21932=LINE ( 'NONE', #52341, #33435 ) ;
#21933=EDGE_CURVE ( 'NONE', #18224, #13159, #38194, .T. ) ;
#21934=LINE ( 'NONE', #1186, #17589 ) ;
#21935=VECTOR ( 'NONE', #7594, 1000.000000000000114 ) ;
#21936=DIRECTION ( 'NONE',  ( -0.005002170337468016433, -0.7660444431189770143, 0.6427681459581293666 ) ) ;
#21937=AXIS2_PLACEMENT_3D ( 'NONE', #16377, #11839, #3345 ) ;
#21938=EDGE_CURVE ( 'NONE', #41541, #39671, #55814, .T. ) ;
#21939=LINE ( 'NONE', #35035, #6633 ) ;
#21940=ORIENTED_EDGE ( 'NONE', *, *, #3982, .F. ) ;
#21941=ORIENTED_EDGE ( 'NONE', *, *, #27597, .F. ) ;
#21942=CARTESIAN_POINT ( 'NONE',  ( -16.35824496976556830, -0.1191753592594197164, 3.685110299410161439 ) ) ;
#21943=DIRECTION ( 'NONE',  ( -0.5449076811759708816, 0.6444004775717707689, 0.5364919789714475140 ) ) ;
#21944=CARTESIAN_POINT ( 'NONE',  ( -23.33849165029409889, 0.000000000000000000, 5.946783852668351855 ) ) ;
#21945=FACE_OUTER_BOUND ( 'NONE', #17686, .T. ) ;
#21946=EDGE_CURVE ( 'NONE', #21366, #40198, #42732, .T. ) ;
#21947=LINE ( 'NONE', #55760, #8344 ) ;
#21948=PLANE ( 'NONE',  #53949 ) ;
#21949=ORIENTED_EDGE ( 'NONE', *, *, #42422, .T. ) ;
#21950=LINE ( 'NONE', #39280, #25598 ) ;
#21951=EDGE_CURVE ( 'NONE', #47914, #26746, #118, .T. ) ;
#21952=DIRECTION ( 'NONE',  ( -0.6427681459581293666, -0.7660444431189770143, -0.005002170337467561935 ) ) ;
#21953=ORIENTED_EDGE ( 'NONE', *, *, #48359, .T. ) ;
#21955=FACE_OUTER_BOUND ( 'NONE', #31933, .T. ) ;
#21956=PLANE ( 'NONE',  #579 ) ;
#21957=LINE ( 'NONE', #30781, #36643 ) ;
#21958=ORIENTED_EDGE ( 'NONE', *, *, #46105, .F. ) ;
#21959=VECTOR ( 'NONE', #14304, 999.9999999999998863 ) ;
#21960=VECTOR ( 'NONE', #6292, 1000.000000000000227 ) ;
#21961=CARTESIAN_POINT ( 'NONE',  ( -19.60990026154428278, 0.000000000000000000, 4.498472333781370125 ) ) ;
#21962=ORIENTED_EDGE ( 'NONE', *, *, #39939, .T. ) ;
#21963=VERTEX_POINT ( 'NONE', #29716 ) ;
#21964=VECTOR ( 'NONE', #11268, 1000.000000000000227 ) ;
#21965=ORIENTED_EDGE ( 'NONE', *, *, #12443, .T. ) ;
#21966=VECTOR ( 'NONE', #53628, 1000.000000000000227 ) ;
#21967=ORIENTED_EDGE ( 'NONE', *, *, #7300, .F. ) ;
#21968=PLANE ( 'NONE',  #13036 ) ;
#21969=VERTEX_POINT ( 'NONE', #16330 ) ;
#21970=EDGE_CURVE ( 'NONE', #52222, #9899, #25424, .T. ) ;
#21971=LINE ( 'NONE', #4944, #12225 ) ;
#21972=ORIENTED_EDGE ( 'NONE', *, *, #32420, .F. ) ;
#21974=VERTEX_POINT ( 'NONE', #3831 ) ;
#21975=LINE ( 'NONE', #694, #41135 ) ;
#21976=VECTOR ( 'NONE', #27433, 1000.000000000000114 ) ;
#21977=ADVANCED_FACE ( 'NONE', ( #8119 ), #51556, .F. ) ;
#21978=ORIENTED_EDGE ( 'NONE', *, *, #29109, .T. ) ;
#21979=EDGE_CURVE ( 'NONE', #20361, #13581, #43330, .T. ) ;
#21980=CARTESIAN_POINT ( 'NONE',  ( -16.73360290908838977, 0.000000000000000000, 5.059514428249818785 ) ) ;
#21982=EDGE_CURVE ( 'NONE', #15779, #41229, #38788, .T. ) ;
#21983=DIRECTION ( 'NONE',  ( 0.9999697198139515519, 0.000000000000000000, 0.007781995580013368816 ) ) ;
#21985=CARTESIAN_POINT ( 'NONE',  ( -19.05009385693719537, 0.000000000000000000, 4.181329822281151465 ) ) ;
#21986=VERTEX_POINT ( 'NONE', #16927 ) ;
#21988=ADVANCED_FACE ( 'NONE', ( #34252 ), #12655, .F. ) ;
#21989=EDGE_CURVE ( 'NONE', #50478, #50472, #13219, .T. ) ;
#21990=EDGE_LOOP ( 'NONE', ( #31191, #24212, #13508, #13881 ) ) ;
#21991=DIRECTION ( 'NONE',  ( 0.9999697198139515519, 0.000000000000000000, 0.007781995580013368816 ) ) ;
#21992=FACE_OUTER_BOUND ( 'NONE', #20822, .T. ) ;
#21993=VECTOR ( 'NONE', #28933, 1000.000000000000000 ) ;
#21994=LINE ( 'NONE', #706, #4312 ) ;
#21995=DIRECTION ( 'NONE',  ( 0.6427681459581294776, -0.7660444431189769032, 0.005002170337467562802 ) ) ;
#21996=DIRECTION ( 'NONE',  ( -0.9321478471874540261, 0.000000000000000000, 0.3620778797217457656 ) ) ;
#21997=PLANE ( 'NONE',  #5999 ) ;
#21998=ORIENTED_EDGE ( 'NONE', *, *, #54975, .F. ) ;
#21999=AXIS2_PLACEMENT_3D ( 'NONE', #2404, #54094, #49823 ) ;
#22002=ORIENTED_EDGE ( 'NONE', *, *, #15401, .T. ) ;
#22003=VECTOR ( 'NONE', #55071, 999.9999999999998863 ) ;
#22004=VECTOR ( 'NONE', #45077, 1000.000000000000114 ) ;
#22005=CARTESIAN_POINT ( 'NONE',  ( -11.40636015113596180, 0.000000000000000000, 11.32142374880780089 ) ) ;
#22006=CARTESIAN_POINT ( 'NONE',  ( -22.15667627784559812, -4.727446477803161073, 13.04688230017630346 ) ) ;
#22007=EDGE_CURVE ( 'NONE', #45145, #28385, #50965, .T. ) ;
#22008=CARTESIAN_POINT ( 'NONE',  ( -15.54543426953848595, 0.000000000000000000, 5.807425170953373517 ) ) ;
#22009=LINE ( 'NONE', #47870, #55013 ) ;
#22010=EDGE_CURVE ( 'NONE', #11344, #30714, #7850, .T. ) ;
#22011=DIRECTION ( 'NONE',  ( -0.6427681459581293666, -0.7660444431189770143, -0.005002170337467561935 ) ) ;
#22012=ORIENTED_EDGE ( 'NONE', *, *, #45164, .T. ) ;
#22013=VECTOR ( 'NONE', #32524, 999.9999999999998863 ) ;
#22014=VECTOR ( 'NONE', #20389, 1000.000000000000227 ) ;
#22016=ADVANCED_FACE ( 'NONE', ( #43030 ), #4142, .F. ) ;
#22017=LINE ( 'NONE', #31403, #13990 ) ;
#22018=CARTESIAN_POINT ( 'NONE',  ( -20.54126990917373519, -0.1191753592594197858, 4.760553241521720658 ) ) ;
#22019=FACE_OUTER_BOUND ( 'NONE', #37485, .T. ) ;
#22021=PLANE ( 'NONE',  #45462 ) ;
#22022=VECTOR ( 'NONE', #22690, 999.9999999999998863 ) ;
#22024=CARTESIAN_POINT ( 'NONE',  ( 2.072287782118878319, 0.000000000000000000, -2.950529333540147015 ) ) ;
#22025=VECTOR ( 'NONE', #2339, 1000.000000000000227 ) ;
#22026=CARTESIAN_POINT ( 'NONE',  ( -26.13493519185646008, 0.000000000000000000, 7.033017491833586377 ) ) ;
#22027=ORIENTED_EDGE ( 'NONE', *, *, #18691, .F. ) ;
#22029=PLANE ( 'NONE',  #45082 ) ;
#22030=EDGE_LOOP ( 'NONE', ( #44668, #1807, #36517, #38167 ) ) ;
#22031=FACE_OUTER_BOUND ( 'NONE', #14180, .T. ) ;
#22032=EDGE_LOOP ( 'NONE', ( #1992, #4584, #50108, #47547 ) ) ;
#22033=LINE ( 'NONE', #18059, #27749 ) ;
#22034=AXIS2_PLACEMENT_3D ( 'NONE', #31976, #40784, #31134 ) ;
#22035=CARTESIAN_POINT ( 'NONE',  ( -19.60990026154428278, 0.000000000000000000, 4.498472333781370125 ) ) ;
#22036=ORIENTED_EDGE ( 'NONE', *, *, #41643, .T. ) ;
#22037=VECTOR ( 'NONE', #852, 1000.000000000000227 ) ;
#22038=ORIENTED_EDGE ( 'NONE', *, *, #4342, .T. ) ;
#22039=ORIENTED_EDGE ( 'NONE', *, *, #44959, .T. ) ;
#22040=ORIENTED_EDGE ( 'NONE', *, *, #4648, .F. ) ;
#22041=ORIENTED_EDGE ( 'NONE', *, *, #47821, .F. ) ;
#22042=EDGE_LOOP ( 'NONE', ( #40824, #2550, #12418, #56129 ) ) ;
#22043=VECTOR ( 'NONE', #46307, 1000.000000000000114 ) ;
#22044=DIRECTION ( 'NONE',  ( -0.7660212471507179544, -0.6427876096865405842, -0.005961354470445141482 ) ) ;
#22045=DIRECTION ( 'NONE',  ( 0.007781995580012663651, -3.146120232559066537E-19, -0.9999697198139514409 ) ) ;
#22046=CARTESIAN_POINT ( 'NONE',  ( -19.60990026154428278, 0.000000000000000000, 4.498472333781370125 ) ) ;
#22047=VECTOR ( 'NONE', #3054, 999.9999999999998863 ) ;
#22048=VECTOR ( 'NONE', #50058, 1000.000000000000227 ) ;
#22049=ORIENTED_EDGE ( 'NONE', *, *, #40054, .T. ) ;
#22050=LINE ( 'NONE', #30851, #4077 ) ;
#22051=EDGE_LOOP ( 'NONE', ( #31057, #41665, #42443, #43068 ) ) ;
#22052=EDGE_LOOP ( 'NONE', ( #54057, #21755, #39601, #27491 ) ) ;
#22054=AXIS2_PLACEMENT_3D ( 'NONE', #28285, #45603, #6717 ) ;
#22055=DIRECTION ( 'NONE',  ( 0.007781995580012663651, 0.000000000000000000, -0.9999697198139515519 ) ) ;
#22056=DIRECTION ( 'NONE',  ( -0.005961354470445682716, -0.6427876096865404731, 0.7660212471507180654 ) ) ;
#22057=LINE ( 'NONE', #35402, #24123 ) ;
#22058=ORIENTED_EDGE ( 'NONE', *, *, #35705, .F. ) ;
#22059=PLANE ( 'NONE',  #50049 ) ;
#22060=EDGE_LOOP ( 'NONE', ( #5562, #11794, #25748, #51037 ) ) ;
#22061=EDGE_CURVE ( 'NONE', #48671, #47896, #27676, .T. ) ;
#22062=EDGE_CURVE ( 'NONE', #45380, #4591, #1556, .T. ) ;
#22063=CARTESIAN_POINT ( 'NONE',  ( -16.99924723426068951, 0.000000000000000000, 13.49389102713827171 ) ) ;
#22064=VECTOR ( 'NONE', #20732, 1000.000000000000227 ) ;
#22065=LINE ( 'NONE', #17236, #23007 ) ;
#22066=EDGE_CURVE ( 'NONE', #7431, #22114, #48706, .T. ) ;
#22067=VECTOR ( 'NONE', #43746, 1000.000000000000227 ) ;
#22068=DIRECTION ( 'NONE',  ( 0.005961354470445682716, -0.6427876096865404731, -0.7660212471507180654 ) ) ;
#22069=LINE ( 'NONE', #18088, #33147 ) ;
#22070=CARTESIAN_POINT ( 'NONE',  ( -28.93137873341882127, 0.000000000000000000, 8.119251130998824451 ) ) ;
#22072=CARTESIAN_POINT ( 'NONE',  ( -20.84574850008768010, -5.375054281893163477, 13.60050816780225347 ) ) ;
#22073=LINE ( 'NONE', #39405, #45817 ) ;
#22074=VERTEX_POINT ( 'NONE', #10355 ) ;
#22076=VECTOR ( 'NONE', #13481, 999.9999999999998863 ) ;
#22078=DIRECTION ( 'NONE',  ( -0.7660212471507179544, -0.6427876096865405842, -0.005961354470445141482 ) ) ;
#22079=DIRECTION ( 'NONE',  ( 0.5449076811759707706, 0.6444004775717708799, -0.5364919789714476250 ) ) ;
#22080=AXIS2_PLACEMENT_3D ( 'NONE', #3238, #20570, #37891 ) ;
#22082=PLANE ( 'NONE',  #25914 ) ;
#22083=ADVANCED_FACE ( 'NONE', ( #6118 ), #9513, .F. ) ;
#22084=CARTESIAN_POINT ( 'NONE',  ( -14.46888367232926420, 0.000000000000000000, 12.59025272694991315 ) ) ;
#22085=PLANE ( 'NONE',  #21190 ) ;
#22086=VERTEX_POINT ( 'NONE', #36201 ) ;
#22087=EDGE_CURVE ( 'NONE', #44387, #38521, #10062, .T. ) ;
#22088=VECTOR ( 'NONE', #6146, 1000.000000000000000 ) ;
#22089=CARTESIAN_POINT ( 'NONE',  ( -26.13337879274045505, 0.000000000000000000, 6.833023547870798353 ) ) ;
#22090=CARTESIAN_POINT ( 'NONE',  ( -17.21129241906660923, 0.000000000000000000, 6.733131273475654766 ) ) ;
#22091=CARTESIAN_POINT ( 'NONE',  ( -11.30636317915456779, -0.1191753592594197858, 11.32220194836580340 ) ) ;
#22092=VECTOR ( 'NONE', #35010, 999.9999999999998863 ) ;
#22093=AXIS2_PLACEMENT_3D ( 'NONE', #32374, #27241, #28085 ) ;
#22094=EDGE_CURVE ( 'NONE', #40769, #5645, #52945, .T. ) ;
#22095=DIRECTION ( 'NONE',  ( 0.7660212471507180654, -0.6427876096865404731, 0.005961354470445141482 ) ) ;
#22096=DIRECTION ( 'NONE',  ( 0.007781995580012662783, 0.000000000000000000, -0.9999697198139514409 ) ) ;
#22097=DIRECTION ( 'NONE',  ( -0.9321478471874540261, 0.000000000000000000, 0.3620778797217457656 ) ) ;
#22098=LINE ( 'NONE', #5074, #41054 ) ;
#22099=AXIS2_PLACEMENT_3D ( 'NONE', #42554, #51058, #25504 ) ;
#22100=VECTOR ( 'NONE', #31794, 1000.000000000000227 ) ;
#22101=LINE ( 'NONE', #8791, #40503 ) ;
#22102=LINE ( 'NONE', #30354, #24710 ) ;
#22104=EDGE_LOOP ( 'NONE', ( #34213, #11506, #34276, #39058 ) ) ;
#22105=ORIENTED_EDGE ( 'NONE', *, *, #36952, .T. ) ;
#22106=ORIENTED_EDGE ( 'NONE', *, *, #37856, .F. ) ;
#22107=ORIENTED_EDGE ( 'NONE', *, *, #1289, .F. ) ;
#22108=VECTOR ( 'NONE', #52076, 1000.000000000000000 ) ;
#22109=ORIENTED_EDGE ( 'NONE', *, *, #55023, .F. ) ;
#22110=CARTESIAN_POINT ( 'NONE',  ( -16.82288186660665374, -0.1191753592594196887, 3.681494387642152422 ) ) ;
#22111=DIRECTION ( 'NONE',  ( -0.9999697198139514409, -0.000000000000000000, -0.007781995580013368816 ) ) ;
#22112=VECTOR ( 'NONE', #31774, 999.9999999999998863 ) ;
#22113=ORIENTED_EDGE ( 'NONE', *, *, #21176, .T. ) ;
#22114=VERTEX_POINT ( 'NONE', #18590 ) ;
#22115=VECTOR ( 'NONE', #6711, 999.9999999999998863 ) ;
#22117=EDGE_LOOP ( 'NONE', ( #43751, #44977, #21163, #26430 ) ) ;
#22118=VECTOR ( 'NONE', #46609, 1000.000000000000000 ) ;
#22119=CARTESIAN_POINT ( 'NONE',  ( -16.53317331066696383, 0.000000000000000000, 13.31285208727739899 ) ) ;
#22120=CARTESIAN_POINT ( 'NONE',  ( 2.072287782118878319, 0.000000000000000000, -2.950529333540147015 ) ) ;
#22121=ORIENTED_EDGE ( 'NONE', *, *, #17648, .T. ) ;
#22122=LINE ( 'NONE', #53072, #39290 ) ;
#22123=VECTOR ( 'NONE', #11378, 1000.000000000000227 ) ;
#22124=EDGE_CURVE ( 'NONE', #30466, #46454, #23138, .T. ) ;
#22125=ORIENTED_EDGE ( 'NONE', *, *, #46750, .T. ) ;
#22126=DIRECTION ( 'NONE',  ( -0.9999697198139514409, -0.000000000000000000, -0.007781995580013368816 ) ) ;
#22127=ADVANCED_FACE ( 'NONE', ( #5522 ), #40467, .F. ) ;
#22128=ADVANCED_FACE ( 'NONE', ( #48967 ), #13498, .F. ) ;
#22129=VECTOR ( 'NONE', #10104, 999.9999999999998863 ) ;
#22130=CARTESIAN_POINT ( 'NONE',  ( -11.59385650878361673, 0.000000000000000000, 1.406192425120281309 ) ) ;
#22131=DIRECTION ( 'NONE',  ( -0.7660212471507179544, -0.6427876096865405842, -0.005961354470445141482 ) ) ;
#22132=VECTOR ( 'NONE', #131, 999.9999999999998863 ) ;
#22133=ORIENTED_EDGE ( 'NONE', *, *, #11573, .F. ) ;
#22134=FACE_OUTER_BOUND ( 'NONE', #19091, .T. ) ;
#22135=DIRECTION ( 'NONE',  ( -0.9999697198139514409, -0.000000000000000000, -0.007781995580013368816 ) ) ;
#22136=PLANE ( 'NONE',  #32985 ) ;
#22137=ORIENTED_EDGE ( 'NONE', *, *, #3582, .T. ) ;
#22138=CARTESIAN_POINT ( 'NONE',  ( 1.086233639165236964, 0.000000000000000000, 2.796443541562362078 ) ) ;
#22139=VERTEX_POINT ( 'NONE', #26837 ) ;
#22140=CARTESIAN_POINT ( 'NONE',  ( -21.47263955680318404, 0.000000000000000000, 5.022634149262071190 ) ) ;
#22141=CARTESIAN_POINT ( 'NONE',  ( -12.15546023705834244, 3.200641362704010007, 1.301408072064137222 ) ) ;
#22142=PLANE ( 'NONE',  #468 ) ;
#22143=LINE ( 'NONE', #52257, #40460 ) ;
#22144=CARTESIAN_POINT ( 'NONE',  ( -16.99924723426068951, 0.000000000000000000, 13.49389102713827171 ) ) ;
#22145=PLANE ( 'NONE',  #46688 ) ;
#22147=ADVANCED_FACE ( 'NONE', ( #35629 ), #39634, .F. ) ;
#22148=VECTOR ( 'NONE', #7249, 1000.000000000000114 ) ;
#22149=PLANE ( 'NONE',  #7528 ) ;
#22150=VECTOR ( 'NONE', #51778, 1000.000000000000114 ) ;
#22152=LINE ( 'NONE', #5133, #11457 ) ;
#22153=ORIENTED_EDGE ( 'NONE', *, *, #17947, .F. ) ;
#22154=FACE_OUTER_BOUND ( 'NONE', #55485, .T. ) ;
#22155=DIRECTION ( 'NONE',  ( -0.005961354470445682716, -0.6427876096865404731, 0.7660212471507180654 ) ) ;
#22156=VECTOR ( 'NONE', #40457, 1000.000000000000227 ) ;
#22157=CARTESIAN_POINT ( 'NONE',  ( -12.51706054884368413, -1.651309408375659871, 1.690687099836828411 ) ) ;
#22158=DIRECTION ( 'NONE',  ( 0.005961354470445682716, -0.6427876096865404731, -0.7660212471507180654 ) ) ;
#22159=EDGE_CURVE ( 'NONE', #2187, #9472, #44164, .T. ) ;
#22160=CARTESIAN_POINT ( 'NONE',  ( -11.20636620717317378, 0.000000000000000000, 11.32298014792380414 ) ) ;
#22161=DIRECTION ( 'NONE',  ( -0.8531650599175527594, 0.4028455766673922356, 0.3313982828793700652 ) ) ;
#22162=ORIENTED_EDGE ( 'NONE', *, *, #55468, .T. ) ;
#22163=VERTEX_POINT ( 'NONE', #35098 ) ;
#22164=ADVANCED_FACE ( 'NONE', ( #31922 ), #967, .F. ) ;
#22165=DIRECTION ( 'NONE',  ( -0.3620778797217455991, 0.000000000000000000, -0.9321478471874540261 ) ) ;
#22167=CARTESIAN_POINT ( 'NONE',  ( -14.14733187112066837, 0.000000000000000000, 5.279647443704662102 ) ) ;
#22168=AXIS2_PLACEMENT_3D ( 'NONE', #11464, #2905, #50352 ) ;
#22169=PLANE ( 'NONE',  #52921 ) ;
#22170=VERTEX_POINT ( 'NONE', #711 ) ;
#22171=LINE ( 'NONE', #26418, #35849 ) ;
#22172=EDGE_CURVE ( 'NONE', #18484, #38141, #18031, .T. ) ;
#22173=ORIENTED_EDGE ( 'NONE', *, *, #41357, .T. ) ;
#22174=CARTESIAN_POINT ( 'NONE',  ( -19.07115766082023356, 0.000000000000000000, 6.887983385698593253 ) ) ;
#22175=VECTOR ( 'NONE', #35119, 1000.000000000000227 ) ;
#22176=ORIENTED_EDGE ( 'NONE', *, *, #2516, .T. ) ;
#22177=VECTOR ( 'NONE', #18238, 1000.000000000000227 ) ;
#22178=ORIENTED_EDGE ( 'NONE', *, *, #13363, .F. ) ;
#22179=ORIENTED_EDGE ( 'NONE', *, *, #28227, .T. ) ;
#22180=LINE ( 'NONE', #42626, #48350 ) ;
#22182=FACE_OUTER_BOUND ( 'NONE', #27434, .T. ) ;
#22184=ORIENTED_EDGE ( 'NONE', *, *, #21401, .T. ) ;
#22185=EDGE_LOOP ( 'NONE', ( #52747, #42113, #39936, #43513 ) ) ;
#22186=EDGE_CURVE ( 'NONE', #47891, #52648, #32503, .T. ) ;
#22187=VECTOR ( 'NONE', #32309, 1000.000000000000227 ) ;
#22188=DIRECTION ( 'NONE',  ( -0.005961354470445682716, -0.6427876096865404731, 0.7660212471507180654 ) ) ;
#22189=VECTOR ( 'NONE', #41480, 1000.000000000000227 ) ;
#22190=ORIENTED_EDGE ( 'NONE', *, *, #16662, .T. ) ;
#22191=PLANE ( 'NONE',  #4676 ) ;
#22192=EDGE_CURVE ( 'NONE', #17429, #12259, #49804, .T. ) ;
#22193=ORIENTED_EDGE ( 'NONE', *, *, #24928, .F. ) ;
#22194=AXIS2_PLACEMENT_3D ( 'NONE', #44610, #5727, #1170 ) ;
#22195=LINE ( 'NONE', #39531, #2449 ) ;
#22196=CARTESIAN_POINT ( 'NONE',  ( -18.67697421479882181, -0.1191753592594197858, 4.036397482078229793 ) ) ;
#22197=ORIENTED_EDGE ( 'NONE', *, *, #54878, .F. ) ;
#22198=EDGE_CURVE ( 'NONE', #3650, #5725, #16014, .T. ) ;
#22199=DIRECTION ( 'NONE',  ( 0.005961354470445682716, -0.6427876096865404731, -0.7660212471507180654 ) ) ;
#22200=AXIS2_PLACEMENT_3D ( 'NONE', #39463, #564, #35215 ) ;
#22201=EDGE_LOOP ( 'NONE', ( #38133, #26654, #14844, #35558 ) ) ;
#22202=EDGE_CURVE ( 'NONE', #46872, #51258, #23672, .T. ) ;
#22203=DIRECTION ( 'NONE',  ( -0.2426528472758541499, 0.7422098413412800966, -0.6246952433987894571 ) ) ;
#22204=AXIS2_PLACEMENT_3D ( 'NONE', #48943, #23107, #13728 ) ;
#22205=MECHANICAL_DESIGN_GEOMETRIC_PRESENTATION_REPRESENTATION('',(#18602),#53937);
#22206=EDGE_LOOP ( 'NONE', ( #16049, #19388, #37192, #54223 ) ) ;
#22207=CARTESIAN_POINT ( 'NONE',  ( -25.20123094555300369, 0.000000000000000000, 6.470945668149052032 ) ) ;
#22208=LINE ( 'NONE', #14269, #31200 ) ;
#22210=CARTESIAN_POINT ( 'NONE',  ( -16.81345671998191449, 0.000000000000000000, 3.412238694616132495 ) ) ;
#22211=ORIENTED_EDGE ( 'NONE', *, *, #15614, .T. ) ;
#22212=VECTOR ( 'NONE', #30935, 1000.000000000000114 ) ;
#22213=ADVANCED_FACE ( 'NONE', ( #33339 ), #19131, .F. ) ;
#22214=LINE ( 'NONE', #27820, #18389 ) ;
#22215=FACE_OUTER_BOUND ( 'NONE', #14038, .T. ) ;
#22216=CARTESIAN_POINT ( 'NONE',  ( -19.25965539076188904, 0.000000000000000000, 5.409188173551533474 ) ) ;
#22217=PLANE ( 'NONE',  #51307 ) ;
#22218=DIRECTION ( 'NONE',  ( -0.6427681459581293666, -0.7660444431189770143, -0.005002170337467561935 ) ) ;
#22219=CARTESIAN_POINT ( 'NONE',  ( 2.072287782118878319, -1.000000000000000000, -2.950529333540147015 ) ) ;
#22220=EDGE_CURVE ( 'NONE', #33548, #17624, #33043, .T. ) ;
#22221=VECTOR ( 'NONE', #983, 1000.000000000000227 ) ;
#22222=VECTOR ( 'NONE', #4970, 999.9999999999998863 ) ;
#22223=EDGE_LOOP ( 'NONE', ( #25337, #41376, #27328, #5970 ) ) ;
#22224=LINE ( 'NONE', #4611, #28016 ) ;
#22225=CARTESIAN_POINT ( 'NONE',  ( -9.808144436391993182, 0.000000000000000000, 10.77986332834118777 ) ) ;
#22226=DIRECTION ( 'NONE',  ( 0.007781995580012663651, -3.146120232559066537E-19, -0.9999697198139514409 ) ) ;
#22227=VERTEX_POINT ( 'NONE', #2644 ) ;
#22228=PLANE ( 'NONE',  #33844 ) ;
#22229=DIRECTION ( 'NONE',  ( 0.6427681459581294776, -0.7660444431189769032, 0.005002170337467562802 ) ) ;
#22230=ORIENTED_EDGE ( 'NONE', *, *, #34646, .T. ) ;
#22231=CARTESIAN_POINT ( 'NONE',  ( -12.21285141497871152, 2.714935509636508204, 1.339197314243185222 ) ) ;
#22232=DIRECTION ( 'NONE',  ( -0.6427681459581293666, -0.7660444431189770143, -0.005002170337467561935 ) ) ;
#22233=DIRECTION ( 'NONE',  ( -0.6427681459581293666, -0.7660444431189770143, -0.005002170337467561935 ) ) ;
#22235=AXIS2_PLACEMENT_3D ( 'NONE', #50657, #11488, #46668 ) ;
#22236=ORIENTED_EDGE ( 'NONE', *, *, #24653, .T. ) ;
#22237=ORIENTED_EDGE ( 'NONE', *, *, #39489, .F. ) ;
#22238=CLOSED_SHELL ( 'NONE', ( #4720, #11070, #50560, #11603, #4554, #43545, #14961, #4754, #42672, #3543, #47158, #25743, #1433, #8404, #46671, #9169, #22666, #37325, #14083, #7259, #30764, #51005, #23889, #27562, #14167, #11358, #28979, #22426, #34042, #42458, #14343, #44129, #10014, #11904, #18875, #55667, #11871, #55142, #53594, #30829, #48666, #22698, #52190, #6132, #13568, #29046, #2041, #34746, #6949, #55215, #43275, #15971, #51580, #50626, #50142, #26417, #22128, #14444, #22642, #16129, #38109, #53099, #10012, #3094, #45843, #4358, #2225, #18153, #1284, #52224, #17786, #44345, #53493, #26470, #7359, #22361, #21838, #29918, #39702, #33671, #4310, #23597, #11281, #24256, #14856, #48945, #22593, #56013, #48096, #27063, #2930, #22684, #39054, #54749, #18956, #9780, #55213, #452, #38361, #34555, #1754, #27020, #6047, #40920, #30369, #46958, #36088, #45361, #32159, #40279, #26908, #27249, #15533, #16352, #41162, #21650, #24118, #22016, #33199, #37715, #51150, #34134, #43022, #40561, #47674, #48972, #5582, #40727, #19998, #38317, #33778, #49639, #9067, #21563, #37131, #123, #16179, #9265, #5941, #28906, #30684, #8188, #17447, #3522, #12645, #18392, #4174, #31569, #40261, #17121, #39518, #32708, #42073, #46217, #55318, #2649, #24613, #5636, #5138, #41716, #44214, #13138, #29804, #39707, #11618, #20191, #31833, #16847, #27310, #36410, #20563, #31644, #6903, #18310, #11299, #22584, #17363, #25451, #37853, #36969, #27252, #34265, #6812, #46785, #10604, #50765, #45767, #43687, #10346, #11637, #6093, #29635, #27813, #45350, #31021, #34359, #19516, #11898, #46620, #51100, #27268, #39680, #33771, #37334, #26745, #2688, #34396, #12586, #6565, #38757, #10550, #56214, #54615, #54203, #53185, #17189, #1589, #13582, #8750, #33458, #52522, #108, #36610, #50334, #13791, #9680, #31947, #34125, #31478, #56003, #49560, #15542, #6359, #25049, #19769, #19095, #8912, #46007, #55633, #41024, #8689, #23239, #1357, #30116, #38314, #46373, #16100, #6694, #12333, #13646, #21315, #54180, #3390, #51264, #27454, #5786, #31313, #11028, #4814, #9301, #31372, #9519, #41055, #55922, #32656, #11234, #23113, #24761, #36264, #25282, #41808, #19453, #32063, #7685, #36597, #43347, #19510, #50822, #35508, #15317, #47448, #49305, #12746, #7192, #9017, #28885, #15835, #35105, #17848, #1681, #3003, #11621, #38477, #16358, #3080, #7310, #24916, #49984, #51070, #6311, #52071, #33777, #27931, #22147, #1139, #50463, #31058, #17854, #23585, #51565, #49059, #14571, #8470, #39565, #38329, #40693, #20346, #23305, #48886, #28057, #12843, #51086, #36314, #20586, #38794, #51786, #26562, #55022, #39493, #50730, #30863, #7631, #25726, #40955, #16570, #34383, #14353, #32931, #54095, #31962, #30644, #45331, #28259, #3930, #53116, #47377, #9008, #16048, #2347, #7780, #14537, #32810, #42534, #20463, #16228, #30761, #8499, #54979, #34816, #10345, #42374, #3612, #17280, #34486, #32204, #26807, #44503, #11833, #43152, #30448, #56040, #46361, #19812, #29293, #47178, #27015, #14143, #48514, #23175, #22409, #44193, #17068, #34323, #32975, #54253, #47167, #1354, #49712, #51855, #28562, #48476, #38114, #28951, #45927, #21638, #7409, #26008, #38287, #19948, #33724, #18234, #24274, #27684, #2058, #23125, #13561, #21615, #16277, #13854, #55384, #37675, #28207, #40719, #34554, #34329, #42627, #43372, #10994, #47372, #13907, #5699, #28881, #32753, #34596, #32948, #14864, #13894, #14394, #51172, #33737, #27068, #30614, #34973, #43979, #14969, #51714, #13241, #18380, #6673, #38674, #32061, #9070, #12891, #53790, #47703, #7809, #32850, #22083, #53036, #46231, #7150, #54191, #23453, #54397, #13591, #17708, #16250, #15790, #41956, #37918, #48327, #27800, #15698, #36068, #40599, #25452, #42519, #20482, #9486, #15999, #1082, #19631, #3904, #2781, #6198, #5826, #30797, #44434, #41040, #18356, #32532, #3772, #38283, #30564, #53558, #13939, #23018, #53166, #10904, #49067, #41510, #33473, #896, #44281, #11395, #28719, #44753, #24975, #48404, #44052, #28632, #854, #51711, #35483, #9155, #42833, #8170, #49594, #32463, #4315, #31095, #52049, #36491, #10991, #16288, #7099, #9988, #20687, #29811, #3489, #3383, #42763, #15347, #18777, #20844, #48141, #20781, #25088, #32744, #22759, #6350, #32339, #44371, #31743, #20599, #26674, #33925, #43414, #12334, #48773, #51734, #1848, #4558, #9686, #24075, #38043, #51396, #49881, #4405, #22980, #36875, #46998, #24372, #40439, #5043, #17726, #45388, #20983, #29142, #26874, #48254, #35968, #3857, #47183, #37118, #54433, #40750, #16933, #28108, #15164, #17310, #45161, #45745, #53983, #54392, #36535, #20605, #25220, #4056, #30343, #2341, #35498, #6485, #1750, #22892, #31370, #17702, #25419, #24376, #48345, #37639, #55747, #54857, #14558, #39302, #41893, #26232, #49896, #46478, #12406, #46469, #5568, #52838, #41730, #33077, #38569, #51965, #55711, #51753, #34445, #27096, #6542, #19890, #47482, #48015, #42513, #30519, #31216, #9898, #32958, #22794, #1975, #37840, #39177, #52062, #8245, #17710, #25344, #43591, #47516, #50567, #28332, #22585, #45997, #36889, #53235, #19592, #50045, #11578, #18629, #6161, #32855, #44947, #42540, #3126, #26002, #14424, #35530, #28924, #32496, #42699, #33478, #31985, #2170, #49363, #8112, #25621, #27654, #12358, #50975, #29504, #34060, #50549, #50192, #18940, #50146, #631, #3892, #55588, #55984, #37254, #23428, #12817, #55453, #13545, #31719, #21485, #43434, #46404, #52745, #10193, #23345, #487, #5301, #24605, #44986, #24953, #9536, #9234, #7064, #21288, #7660, #24126, #15444, #34294, #48602, #33663, #955, #28715, #40562, #35175, #814, #48637, #13917, #25219, #55985, #4321, #47478, #13997, #39723, #44426, #53619, #21093, #5009, #28556, #24812, #40681, #33414, #27699, #53303, #6486, #195, #41930, #18222, #8493, #18810, #36168, #43422, #32714, #29073, #32012, #15283, #16913, #27203, #45084, #48643, #54182, #48751, #26469, #39724, #30187, #32468, #21857, #1397, #54557, #48852, #15986, #33319, #41093, #3351, #13457, #38930, #29377, #38469, #856, #44181, #28328, #36115, #35583, #29808, #13327, #25257, #14214, #55822, #19431, #20388, #22432, #18827, #10473, #15230, #39010, #50843, #2655, #11812, #32782, #15570, #48349, #37073, #3211, #52702, #49093, #41424, #31812, #51137, #12191, #10916, #44766, #52885, #53547, #28003, #15606, #34702, #19562, #11141, #54907, #13689, #776, #52879, #1508, #11218, #8981, #30919, #1138, #24407, #38137, #6757, #34924, #32687, #47594, #45702, #37562, #50102, #25382, #50466, #5126, #8661, #36909, #45153, #39524, #29725, #10689, #28134, #17877, #40820, #29327, #47871, #48201, #52530, #5342, #21304, #7036, #25724, #43159, #6226, #34385, #52746, #6586, #33555, #4824, #54710, #50144, #37458, #5315, #33385, #15831, #15652, #5738, #14331, #21977, #28981, #24189, #14057, #24620, #9350, #18401, #8975, #40141, #54578, #7712, #41776, #7247, #16170, #13306, #46903, #4340, #53189, #35211, #6253, #221, #49817, #21988, #36414, #53000, #16973, #41705, #54877, #51193, #28623, #8033, #24122, #31875, #43655, #42771, #27264, #38939, #14392, #5933, #4229, #4503, #56070, #50221, #16488, #3352, #8544, #55629, #44474, #5222, #49607, #7312, #28819, #47664, #26402, #56152, #35975, #39072, #3534, #26365, #51233, #16061, #35282, #42798, #14273, #17031, #13256, #22291, #9186, #36827, #28703, #42929, #34367, #4621, #19871, #44869, #56231, #7421, #20510, #49110, #12331, #10571, #53590, #21679, #35699, #19704, #7644, #32846, #15382, #1168, #12767, #19885, #1332, #3419, #2967, #31006, #40069, #47905, #20614, #49928, #51495, #13093, #6418, #382, #35844, #31020, #51844, #7131, #42574, #54954, #17918, #4420, #33358, #43203, #32892, #4010, #6889, #47139, #11796, #18273, #13539, #9769, #11503, #11859, #32089, #6388, #20581, #43936, #49653, #13651, #9499, #10933, #41277, #47536, #4583, #15395, #13541, #47716, #28531, #36257, #4710, #45258, #48242, #17525, #43037, #49660, #52961, #28450, #5491, #7198, #50887, #6629, #48735, #26983, #19884, #22407, #5599, #1245, #50228, #2177, #38153, #16397, #9233, #26323, #6016, #52454, #32153, #6057, #5054, #17797, #30159, #10684, #29902, #4413, #2663, #30491, #28598, #43031, #4965, #43660, #43520, #27558, #7798, #46160, #36723, #40725, #52696, #42134, #46613, #35383, #178, #15724, #14478, #16696, #25542, #5834, #40659, #44785, #35733, #32885, #15090, #18840, #4612, #32464, #41495, #6446, #46222, #23650, #54472, #17530, #28271, #23010, #9826, #32092, #38890, #17006, #6243, #40084, #43109, #44410, #36211, #50623, #43467, #1315, #49555, #36370, #46542, #25583, #47005, #29041, #35361, #2562, #39796, #11020, #38989, #51111, #3045, #54817, #54808, #32096, #49641, #37527, #2549, #15397, #44733, #35941, #47506, #47324, #19022, #31469, #43804, #23962, #35820, #41382, #18465, #19861, #28676, #45103, #56220, #53245, #7501, #27400, #25849, #32163, #46098, #5930, #23098, #10537, #31450, #46353, #1836, #40216, #37750, #51585, #31138, #603, #31016, #24679, #55500, #15038, #42349, #39941, #43095, #33806, #38542, #6347, #45747, #36047, #48607, #75, #53653, #49647, #7767, #1542, #27579, #35802, #55148, #15016, #53414, #52455, #50071, #5462, #41448, #30914, #13172, #24193, #37495, #42994, #36298, #33360, #35860, #48765, #9389, #33499, #24623, #27935, #36840, #26428, #32739, #14619, #30102, #35319, #12236, #31236, #45664, #10101, #4417, #7573, #16809, #14684, #40029, #10856, #60, #1738, #453, #15229, #19946, #4686, #44543, #30046, #16104, #43165, #29317, #10921, #11775, #9804, #12507, #12570, #46267, #17253, #42810, #45602, #13602, #5140, #7158, #32021, #36637, #34126, #33029, #1999, #8115, #17443, #51383, #6269, #1211, #20592, #56117, #43092, #40206, #50785, #47226, #44882, #25315, #29151, #7762, #48021, #23539, #52992, #10740, #16338, #10788, #6195, #14039, #3751, #25160, #43874, #22330, #5310, #10841, #40792, #14585, #19443, #12833, #8414, #19017, #1724, #50234, #24011, #26115, #53608, #4098, #1215, #32653, #12134, #23486, #48740, #31679, #16887, #28093, #13128, #16227, #1021, #29443, #19326, #30212, #54109, #35893, #604, #54456, #46043, #40392, #26766, #18964, #26158, #40653, #43790, #20721, #22862, #14560, #22804, #33983, #35241, #27880, #4912, #55881, #34514, #15796, #17867, #46587, #47786, #18614, #52567, #29500, #18126, #6518, #2390, #49063, #12580, #51988, #36129, #23508, #12959, #53172, #36553, #10457, #47254, #40403, #30204, #39959, #34613, #31324, #9271, #54589, #25112, #21690, #6888, #35621, #36076, #28255, #32595, #34751, #25336, #53420, #830, #38982, #35964, #50707, #22164, #45874, #20435, #200, #28629, #39069, #22546, #33711, #1976, #38752, #21777, #22436, #44780, #54296, #12628, #2118, #16348, #52825, #50117, #51487, #32243, #37425, #34222, #20911, #20132, #24594, #45381, #35089, #37963, #37930, #49045, #34901, #24437, #55523, #17578, #38367, #35115, #5273, #45982, #33089, #48079, #50752, #44211, #9582, #1351, #2471, #17348, #41969, #19254, #14340, #48926, #44566, #28142, #34461, #17325, #3907, #4895, #50847, #39048, #5095, #52508, #14609, #42221, #55740, #37302, #25653, #40962, #55827, #3936, #39831, #13644, #23384, #37627, #48115, #25031, #53340, #20394, #37983, #33124, #19094, #31869, #1832, #15785, #26421, #18763, #41583, #53910, #42630, #25781, #10030, #47124, #53530, #50067, #33970, #39267, #13369, #32942, #15876, #20627, #44629, #42116, #5642, #18301, #44425, #13600, #51156, #53389, #29523, #43983, #11997, #24215, #22337, #48101, #829, #8846, #11497, #18555, #31912, #26926, #9644, #54132, #34674, #13431, #38493, #18272, #52693, #6257, #40688, #1127, #20052, #1560, #8806, #18451, #12320, #43410, #8503, #24064, #48935, #25087, #15469, #21784, #24314, #29825, #10616, #2528, #27383, #2952, #28620, #8273, #27423, #29612, #54103, #42745, #9164, #10433, #34709, #51101, #54671, #50012, #7702, #15770, #5217, #17081, #27696, #55341, #6433, #1027, #49702, #27916, #55869, #50676, #39952, #49756, #35537, #38777, #23307, #17092, #32531, #8586, #38082, #26253, #51501, #50921, #12108, #21553, #55408, #16842, #31010, #43810, #13816, #14896, #56051, #50410, #27146, #23487, #47291, #55201, #50952, #24004, #29897, #37490, #28223, #52038, #48044, #47297, #19479, #45634, #52664, #22989, #15513, #14753, #36494, #8452, #47857, #55749, #42646, #4001, #2220, #22213, #2725, #28462, #37640, #20326, #50052, #39230, #24432, #12975, #23712, #21182, #4128, #15989, #3866, #47645, #46459, #17418, #35230, #33856, #51234, #2660, #55320, #12660, #41325, #48269, #42967, #38881, #6728, #28939, #40334, #48146, #34634, #6302, #51309, #10772, #24836, #27500, #14419, #25029, #43548, #38263, #38928, #50312, #44646, #794, #15115, #12643, #859, #53399, #24511, #37952, #55270, #6411, #14056, #33474, #47608, #25971, #43262, #11648, #29006, #10486, #23811, #26697, #36204, #55640, #23023, #15560, #9523, #16333, #15260, #53660, #8679, #32399, #32527, #40981, #5364, #20879, #8815, #1419, #12181, #48260, #4889, #7572, #4509, #16923, #30854, #22531, #24509, #42737, #18867, #17085, #14179, #23042, #40632, #30819, #55417, #16886, #35517, #4943, #9693, #42715, #52344, #43155, #1565, #6449, #23094, #13786, #39229, #665, #24691, #35577, #50558, #21511, #55257, #33765, #24729, #37498, #28516, #4352, #45517, #26890, #3466, #43517, #28748, #43202, #8699, #54421, #16483, #6428, #14581, #32338, #41630, #23024, #17426, #34848, #20681, #21779, #39597, #37128, #36336, #6512, #14202, #10645, #12808, #23211, #27119, #39007, #39859, #36404, #6525, #55786, #13673, #20948, #35882, #39142, #54480, #18136, #11784, #22924, #13792, #40484, #30078, #412, #18714, #18686, #3239, #45639, #55932, #7224, #32003, #25799, #2929, #37178, #22400, #23675, #19251, #4431, #10095, #29994, #3834, #48552, #26841, #25814, #14081, #14043, #35799, #9118, #31615, #51046, #8781, #11129, #53394, #2796, #41431, #53939, #29517, #50533, #53956, #48822, #41854, #17374, #33415, #10181, #3588, #55313, #41914, #43458, #5163, #21819, #28393, #37203, #37120, #36759, #25407, #39378, #30487, #49265, #7130, #43708, #22833, #4780, #44217, #38618, #22798, #52199, #39792, #41107, #18655, #31710, #19027, #20527, #13552, #46011, #21689, #32273, #25810, #42890, #11564, #6480, #21370, #40620, #15765, #36686, #1910, #20177, #26477, #20021, #32697, #14655, #49000, #48590, #15110, #40557, #22917, #8431, #9799, #30754, #50456, #12008, #5040, #27202, #53894, #34898, #36308, #53199, #19822, #36126, #5831, #29895, #30543, #25446, #45042, #17272, #19377, #47824, #21062, #32405, #28399, #53466, #12354, #39190, #3939, #8085, #30668, #41420, #12085, #36243, #19824, #5431, #48196, #56181, #6767, #17486, #40405, #49107, #41976, #4640, #27207, #6287, #36119, #1672, #19107, #43005, #52585, #11217, #26341, #22277, #49976, #28440, #34507, #16096, #13550, #742, #43592, #55626, #11313, #5868, #19366, #56144, #51663, #32209, #53606, #54302, #7731, #10863, #34659, #14623, #26332, #15195, #42231, #16191, #19220, #8615, #48677, #23377, #32450, #25187, #55227, #23364, #43192, #43268, #50714, #54631, #6760, #50538, #13285, #8279, #8541, #27575, #15531, #31938, #41316, #54699, #12530, #10436, #48752, #28166, #8886, #34434, #8708, #23699, #26024, #19506, #30007, #33374, #2273, #6741, #43621, #21516, #23373, #54947, #44992, #48354, #7032, #16384, #15407, #19497, #29973, #2585, #19330, #25534, #19928, #30749, #53722, #24302, #50452, #34823, #51019, #31689, #51646, #22127, #53900, #10315, #13228, #23978, #33299, #14058, #1730, #34763, #18943, #48698, #7235, #20136, #41330, #55413, #42001, #15224, #16807, #45569, #17096, #50593, #24322, #34511, #28302, #51559, #17510, #17254, #54941, #19292, #43424, #32227, #16415, #6061, #22874, #14265, #53836, #27134, #3594, #49009, #45104, #2460, #36651, #23907, #2354, #7971, #2097, #18297, #39894, #11558, #49324, #18416, #11817, #5006, #2576, #7446, #9649, #1695, #51431, #16197, #3009, #28675, #6166, #18393, #23048, #32893, #38514, #55559, #9920, #47004, #20104, #35184, #26486, #17217, #41974, #3781, #20227, #21323, #50767, #15930, #49752, #8772, #21022, #19224, #35939, #51368, #20650, #20267, #597, #36539, #5664, #11900, #26174, #45139, #1971, #49722, #51238, #44764, #8347, #55052, #47604, #17811, #47366, #24883, #53477, #14173, #14626, #35789, #2875, #30798, #52293, #45272, #29655, #21684, #12664, #926, #43918, #42680, #33240, #24260, #47196, #42101, #39382, #26565, #31574, #38122, #24333, #50399, #2159, #3746, #30557, #50609, #47678, #32839, #2807, #47003, #16998, #52759, #45303, #35515, #27161, #50829, #47793, #790 ) ) ;
#22239=FACE_OUTER_BOUND ( 'NONE', #25635, .T. ) ;
#22240=CARTESIAN_POINT ( 'NONE',  ( -18.62826334475414924, 0.000000000000000000, 9.685474233794316490 ) ) ;
#22241=DIRECTION ( 'NONE',  ( 0.000000000000000000, -0.000000000000000000, -1.000000000000000000 ) ) ;
#22242=AXIS2_PLACEMENT_3D ( 'NONE', #37936, #46421, #54206 ) ;
#22243=DIRECTION ( 'NONE',  ( -0.005961354470445682716, -0.6427876096865404731, 0.7660212471507180654 ) ) ;
#22244=CARTESIAN_POINT ( 'NONE',  ( -21.27557641678912148, -4.241740624735661491, 11.90750714001334920 ) ) ;
#22245=DIRECTION ( 'NONE',  ( 0.000000000000000000, -0.000000000000000000, -1.000000000000000000 ) ) ;
#22246=EDGE_CURVE ( 'NONE', #51326, #40968, #54337, .T. ) ;
#22247=VECTOR ( 'NONE', #51875, 999.9999999999998863 ) ;
#22248=ORIENTED_EDGE ( 'NONE', *, *, #27155, .T. ) ;
#22249=DIRECTION ( 'NONE',  ( -0.5449076811759708816, 0.6444004775717707689, 0.5364919789714475140 ) ) ;
#22250=DIRECTION ( 'NONE',  ( 0.007781995580012662783, 0.000000000000000000, -0.9999697198139514409 ) ) ;
#22251=VECTOR ( 'NONE', #33463, 1000.000000000000000 ) ;
#22252=VECTOR ( 'NONE', #24766, 1000.000000000000227 ) ;
#22253=ORIENTED_EDGE ( 'NONE', *, *, #51364, .F. ) ;
#22254=VECTOR ( 'NONE', #17174, 1000.000000000000114 ) ;
#22256=DIRECTION ( 'NONE',  ( -0.9999697198139514409, -0.000000000000000000, -0.007781995580013368816 ) ) ;
#22257=DIRECTION ( 'NONE',  ( -0.5449076811759708816, 0.6444004775717707689, 0.5364919789714475140 ) ) ;
#22258=VECTOR ( 'NONE', #28288, 1000.000000000000227 ) ;
#22259=EDGE_CURVE ( 'NONE', #53756, #26056, #45524, .T. ) ;
#22260=EDGE_LOOP ( 'NONE', ( #44134, #37014, #25577, #28000 ) ) ;
#22261=VECTOR ( 'NONE', #25332, 1000.000000000000227 ) ;
#22262=DIRECTION ( 'NONE',  ( 0.7660212471507180654, -0.6427876096865404731, 0.005961354470445141482 ) ) ;
#22263=EDGE_LOOP ( 'NONE', ( #30134, #24742, #12621, #4316 ) ) ;
#22264=EDGE_CURVE ( 'NONE', #7467, #5490, #46097, .T. ) ;
#22266=EDGE_CURVE ( 'NONE', #47757, #3399, #20244, .T. ) ;
#22267=VECTOR ( 'NONE', #39781, 999.9999999999998863 ) ;
#22269=VECTOR ( 'NONE', #9997, 999.9999999999998863 ) ;
#22270=ORIENTED_EDGE ( 'NONE', *, *, #52180, .F. ) ;
#22271=ORIENTED_EDGE ( 'NONE', *, *, #41610, .F. ) ;
#22272=CARTESIAN_POINT ( 'NONE',  ( -23.33849165029409889, 0.000000000000000000, 5.946783852668351855 ) ) ;
#22273=ORIENTED_EDGE ( 'NONE', *, *, #51327, .F. ) ;
#22274=DIRECTION ( 'NONE',  ( 0.9999697198139515519, 0.000000000000000000, 0.007781995580013368816 ) ) ;
#22275=VERTEX_POINT ( 'NONE', #41822 ) ;
#22276=LINE ( 'NONE', #35601, #21390 ) ;
#22277=ADVANCED_FACE ( 'NONE', ( #36754 ), #53770, .F. ) ;
#22279=DIRECTION ( 'NONE',  ( -0.7660212471507179544, -0.6427876096865405842, -0.005961354470445141482 ) ) ;
#22280=ORIENTED_EDGE ( 'NONE', *, *, #40716, .T. ) ;
#22281=EDGE_CURVE ( 'NONE', #9065, #44931, #14889, .T. ) ;
#22283=LINE ( 'NONE', #44983, #34759 ) ;
#22284=VECTOR ( 'NONE', #46400, 1000.000000000000114 ) ;
#22285=LINE ( 'NONE', #10045, #25954 ) ;
#22286=LINE ( 'NONE', #26252, #5033 ) ;
#22288=CARTESIAN_POINT ( 'NONE',  ( -12.50255982302408775, -4.403642575758163424, 1.597240687396138892 ) ) ;
#22289=VECTOR ( 'NONE', #33340, 999.9999999999998863 ) ;
#22290=ORIENTED_EDGE ( 'NONE', *, *, #45867, .F. ) ;
#22291=ADVANCED_FACE ( 'NONE', ( #37579 ), #54903, .F. ) ;
#22292=EDGE_LOOP ( 'NONE', ( #44527, #40171, #38813, #43651 ) ) ;
#22293=CARTESIAN_POINT ( 'NONE',  ( -19.59569683186026268, 0.000000000000000000, 14.58168106541950948 ) ) ;
#22294=FACE_OUTER_BOUND ( 'NONE', #51463, .T. ) ;
#22295=AXIS2_PLACEMENT_3D ( 'NONE', #40080, #26455, #13680 ) ;
#22296=LINE ( 'NONE', #31070, #14293 ) ;
#22297=EDGE_CURVE ( 'NONE', #19093, #33398, #19969, .T. ) ;
#22298=VECTOR ( 'NONE', #55161, 1000.000000000000227 ) ;
#22299=VECTOR ( 'NONE', #52067, 999.9999999999998863 ) ;
#22300=DIRECTION ( 'NONE',  ( -0.2426528472758542054, 0.7422098413412800966, -0.6246952433987894571 ) ) ;
#22301=LINE ( 'NONE', #17759, #8605 ) ;
#22303=ORIENTED_EDGE ( 'NONE', *, *, #41088, .F. ) ;
#22304=DIRECTION ( 'NONE',  ( 0.9999697198139515519, 0.000000000000000000, 0.007781995580013368816 ) ) ;
#22306=ORIENTED_EDGE ( 'NONE', *, *, #34753, .F. ) ;
#22307=AXIS2_PLACEMENT_3D ( 'NONE', #44424, #124, #52406 ) ;
#22309=LINE ( 'NONE', #17462, #17881 ) ;
#22310=AXIS2_PLACEMENT_3D ( 'NONE', #22120, #39454, #39739 ) ;
#22312=DIRECTION ( 'NONE',  ( -0.005002170337468016433, -0.7660444431189770143, 0.6427681459581293666 ) ) ;
#22313=PLANE ( 'NONE',  #51329 ) ;
#22314=VECTOR ( 'NONE', #32252, 1000.000000000000000 ) ;
#22315=CARTESIAN_POINT ( 'NONE',  ( -14.20280369269832832, 0.000000000000000000, 12.40765738797303719 ) ) ;
#22316=ORIENTED_EDGE ( 'NONE', *, *, #29521, .F. ) ;
#22317=VECTOR ( 'NONE', #37943, 1000.000000000000000 ) ;
#22318=ORIENTED_EDGE ( 'NONE', *, *, #15337, .T. ) ;
#22319=CARTESIAN_POINT ( 'NONE',  ( -20.54204810873173415, 0.000000000000000000, 4.860550213503115558 ) ) ;
#22320=PLANE ( 'NONE',  #43985 ) ;
#22321=FACE_OUTER_BOUND ( 'NONE', #23029, .T. ) ;
#22322=CARTESIAN_POINT ( 'NONE',  ( -20.54049170961573267, 0.000000000000000000, 4.660556269540326646 ) ) ;
#22323=FACE_OUTER_BOUND ( 'NONE', #53006, .T. ) ;
#22324=EDGE_CURVE ( 'NONE', #53756, #51780, #41288, .T. ) ;
#22325=CARTESIAN_POINT ( 'NONE',  ( -18.67619601524082285, 0.000000000000000000, 3.936400510096834893 ) ) ;
#22326=LINE ( 'NONE', #51833, #45623 ) ;
#22327=VECTOR ( 'NONE', #10378, 1000.000000000000227 ) ;
#22329=DIRECTION ( 'NONE',  ( 0.005002170337468016433, -0.7660444431189770143, -0.6427681459581293666 ) ) ;
#22330=ADVANCED_FACE ( 'NONE', ( #32218 ), #49541, .F. ) ;
#22331=ORIENTED_EDGE ( 'NONE', *, *, #48838, .F. ) ;
#22332=DIRECTION ( 'NONE',  ( -0.7660212471507179544, -0.6427876096865405842, -0.005961354470445141482 ) ) ;
#22333=ORIENTED_EDGE ( 'NONE', *, *, #54005, .T. ) ;
#22335=VECTOR ( 'NONE', #1803, 999.9999999999998863 ) ;
#22336=EDGE_CURVE ( 'NONE', #17295, #47436, #28497, .T. ) ;
#22337=ADVANCED_FACE ( 'NONE', ( #40995 ), #55966, .F. ) ;
#22338=DIRECTION ( 'NONE',  ( 0.9999697198139515519, 0.000000000000000000, 0.007781995580013368816 ) ) ;
#22339=EDGE_CURVE ( 'NONE', #34418, #47950, #56224, .T. ) ;
#22340=ORIENTED_EDGE ( 'NONE', *, *, #6360, .F. ) ;
#22341=FACE_OUTER_BOUND ( 'NONE', #27805, .T. ) ;
#22342=VECTOR ( 'NONE', #37423, 1000.000000000000000 ) ;
#22343=ORIENTED_EDGE ( 'NONE', *, *, #7920, .T. ) ;
#22344=EDGE_CURVE ( 'NONE', #37937, #10254, #12786, .T. ) ;
#22345=EDGE_LOOP ( 'NONE', ( #42143, #28746, #49189, #9420 ) ) ;
#22346=AXIS2_PLACEMENT_3D ( 'NONE', #19267, #28080, #36603 ) ;
#22347=ORIENTED_EDGE ( 'NONE', *, *, #48544, .T. ) ;
#22348=VECTOR ( 'NONE', #33021, 1000.000000000000227 ) ;
#22350=ORIENTED_EDGE ( 'NONE', *, *, #56233, .T. ) ;
#22351=CARTESIAN_POINT ( 'NONE',  ( -12.42791540084058255, 3.524445264749011208, 1.396907870518687256 ) ) ;
#22352=LINE ( 'NONE', #55859, #3142 ) ;
#22354=VECTOR ( 'NONE', #51480, 1000.000000000000114 ) ;
#22355=ORIENTED_EDGE ( 'NONE', *, *, #7998, .T. ) ;
#22357=EDGE_CURVE ( 'NONE', #30292, #11776, #3985, .T. ) ;
#22358=EDGE_LOOP ( 'NONE', ( #52762, #37360, #3031, #13052 ) ) ;
#22359=EDGE_LOOP ( 'NONE', ( #26409, #45308, #34064, #21793 ) ) ;
#22360=AXIS2_PLACEMENT_3D ( 'NONE', #20196, #16505, #33551 ) ;
#22361=ADVANCED_FACE ( 'NONE', ( #26395 ), #43450, .F. ) ;
#22362=AXIS2_PLACEMENT_3D ( 'NONE', #56044, #17137, #51757 ) ;
#22363=FACE_OUTER_BOUND ( 'NONE', #39708, .T. ) ;
#22364=FACE_OUTER_BOUND ( 'NONE', #52138, .T. ) ;
#22365=EDGE_CURVE ( 'NONE', #12432, #50295, #5131, .T. ) ;
#22366=DIRECTION ( 'NONE',  ( -0.7660212471507179544, -0.6427876096865405842, -0.005961354470445141482 ) ) ;
#22367=ORIENTED_EDGE ( 'NONE', *, *, #28403, .T. ) ;
#22368=CARTESIAN_POINT ( 'NONE',  ( -17.74482636761137044, -0.1191753592594197858, 3.674319602356483916 ) ) ;
#22369=ORIENTED_EDGE ( 'NONE', *, *, #47036, .T. ) ;
#22370=EDGE_CURVE ( 'NONE', #9163, #43762, #4827, .T. ) ;
#22371=CARTESIAN_POINT ( 'NONE',  ( -16.49482643775764146, 0.000000000000000000, 8.385361270221707741 ) ) ;
#22372=VECTOR ( 'NONE', #3525, 1000.000000000000114 ) ;
#22373=FACE_OUTER_BOUND ( 'NONE', #16193, .T. ) ;
#22374=LINE ( 'NONE', #1029, #37688 ) ;
#22375=LINE ( 'NONE', #1030, #25818 ) ;
#22377=CARTESIAN_POINT ( 'NONE',  ( -18.67775241435682432, 0.000000000000000000, 4.136394454059623804 ) ) ;
#22378=DIRECTION ( 'NONE',  ( 0.005002170337468016433, -0.7660444431189770143, -0.6427681459581293666 ) ) ;
#22379=ORIENTED_EDGE ( 'NONE', *, *, #52558, .T. ) ;
#22380=CARTESIAN_POINT ( 'NONE',  ( -16.06709938707323460, 0.000000000000000000, 13.13181314741652628 ) ) ;
#22382=AXIS2_PLACEMENT_3D ( 'NONE', #51960, #6245, #44555 ) ;
#22383=FACE_OUTER_BOUND ( 'NONE', #51020, .T. ) ;
#22384=PLANE ( 'NONE',  #42311 ) ;
#22385=AXIS2_PLACEMENT_3D ( 'NONE', #4376, #4919, #21687 ) ;
#22386=DIRECTION ( 'NONE',  ( 0.005961354470445682716, -0.6427876096865404731, -0.7660212471507180654 ) ) ;
#22388=DIRECTION ( 'NONE',  ( 0.007781995580012663651, -3.146120232559066537E-19, -0.9999697198139514409 ) ) ;
#22389=CARTESIAN_POINT ( 'NONE',  ( -20.34342856960166657, -4.241740624735661491, 11.54542926029160377 ) ) ;
#22390=AXIS2_PLACEMENT_3D ( 'NONE', #51350, #7078, #55893 ) ;
#22391=DIRECTION ( 'NONE',  ( 0.007781995580012663651, -3.146120232559066537E-19, -0.9999697198139514409 ) ) ;
#22392=VERTEX_POINT ( 'NONE', #4293 ) ;
#22393=DIRECTION ( 'NONE',  ( -0.8531650599175529814, -0.4028455766673920135, 0.3313982828793697877 ) ) ;
#22394=DIRECTION ( 'NONE',  ( 0.6427681459581294776, -0.7660444431189769032, 0.005002170337467562802 ) ) ;
#22395=FACE_OUTER_BOUND ( 'NONE', #46453, .T. ) ;
#22396=EDGE_CURVE ( 'NONE', #4104, #46046, #17313, .T. ) ;
#22397=VECTOR ( 'NONE', #7910, 999.9999999999998863 ) ;
#22398=CARTESIAN_POINT ( 'NONE',  ( -9.075990533167328067, 0.000000000000000000, 10.41622904950343909 ) ) ;
#22399=CARTESIAN_POINT ( 'NONE',  ( -14.41329247838824124, 0.000000000000000000, 5.446903690347632221 ) ) ;
#22400=ADVANCED_FACE ( 'NONE', ( #17909 ), #22149, .F. ) ;
#22402=CARTESIAN_POINT ( 'NONE',  ( -14.62921308899344730, 0.000000000000000000, 7.491889751483238769 ) ) ;
#22403=VECTOR ( 'NONE', #29220, 1000.000000000000227 ) ;
#22404=VECTOR ( 'NONE', #19072, 1000.000000000000227 ) ;
#22405=LINE ( 'NONE', #30351, #4343 ) ;
#22406=CARTESIAN_POINT ( 'NONE',  ( -12.23010465924184764, -4.079838673713163111, 1.501740888941589303 ) ) ;
#22407=ADVANCED_FACE ( 'NONE', ( #47421 ), #48246, .F. ) ;
#22408=EDGE_CURVE ( 'NONE', #32474, #13470, #31227, .T. ) ;
#22409=ADVANCED_FACE ( 'NONE', ( #13072 ), #30400, .F. ) ;
#22410=ORIENTED_EDGE ( 'NONE', *, *, #11737, .T. ) ;
#22411=EDGE_CURVE ( 'NONE', #37913, #34403, #8530, .T. ) ;
#22413=ORIENTED_EDGE ( 'NONE', *, *, #32629, .F. ) ;
#22414=VERTEX_POINT ( 'NONE', #8838 ) ;
#22415=VERTEX_POINT ( 'NONE', #38919 ) ;
#22416=ORIENTED_EDGE ( 'NONE', *, *, #38336, .F. ) ;
#22417=FACE_OUTER_BOUND ( 'NONE', #24272, .T. ) ;
#22418=DIRECTION ( 'NONE',  ( 0.000000000000000000, -0.000000000000000000, -1.000000000000000000 ) ) ;
#22419=ORIENTED_EDGE ( 'NONE', *, *, #56180, .F. ) ;
#22420=AXIS2_PLACEMENT_3D ( 'NONE', #42141, #11196, #20577 ) ;
#22421=ORIENTED_EDGE ( 'NONE', *, *, #43336, .F. ) ;
#22422=EDGE_CURVE ( 'NONE', #39021, #49471, #26142, .T. ) ;
#22423=AXIS2_PLACEMENT_3D ( 'NONE', #23677, #22846, #39891 ) ;
#22424=CARTESIAN_POINT ( 'NONE',  ( -19.25813676402126617, -5.698858183938163791, 13.51524322189348659 ) ) ;
#22425=ORIENTED_EDGE ( 'NONE', *, *, #39586, .T. ) ;
#22426=ADVANCED_FACE ( 'NONE', ( #39179 ), #39761, .F. ) ;
#22427=CARTESIAN_POINT ( 'NONE',  ( -16.45426279964252458, 0.000000000000000000, 3.173020884834126587 ) ) ;
#22428=DIRECTION ( 'NONE',  ( 0.7660212471507180654, -0.6427876096865404731, 0.005961354470445141482 ) ) ;
#22429=ORIENTED_EDGE ( 'NONE', *, *, #20430, .F. ) ;
#22430=PLANE ( 'NONE',  #31009 ) ;
#22432=ADVANCED_FACE ( 'NONE', ( #35484 ), #52791, .F. ) ;
#22433=VECTOR ( 'NONE', #49231, 1000.000000000000227 ) ;
#22434=CARTESIAN_POINT ( 'NONE',  ( -15.62813556599864562, 0.000000000000000000, 2.852125011887896910 ) ) ;
#22435=DIRECTION ( 'NONE',  ( 0.005002170337468016433, -0.7660444431189770143, -0.6427681459581293666 ) ) ;
#22436=ADVANCED_FACE ( 'NONE', ( #23549 ), #40609, .F. ) ;
#22437=FACE_OUTER_BOUND ( 'NONE', #7951, .T. ) ;
#22438=CARTESIAN_POINT ( 'NONE',  ( -19.12492725574397312, -0.04999193034575387384, 8.406842698057740648 ) ) ;
#22439=EDGE_LOOP ( 'NONE', ( #29508, #53309, #19463, #43959 ) ) ;
#22440=CARTESIAN_POINT ( 'NONE',  ( -22.40478740399063895, 0.000000000000000000, 5.384712028983816623 ) ) ;
#22441=LINE ( 'NONE', #26972, #11144 ) ;
#22442=CARTESIAN_POINT ( 'NONE',  ( -17.46532115785441519, 0.000000000000000000, 13.67492996699914265 ) ) ;
#22443=ORIENTED_EDGE ( 'NONE', *, *, #52407, .T. ) ;
#22444=CARTESIAN_POINT ( 'NONE',  ( -25.20123094555300369, 0.000000000000000000, 6.470945668149052032 ) ) ;
#22445=ORIENTED_EDGE ( 'NONE', *, *, #52527, .T. ) ;
#22446=CARTESIAN_POINT ( 'NONE',  ( -28.92982233430281980, 0.000000000000000000, 7.919257187036034651 ) ) ;
#22447=DIRECTION ( 'NONE',  ( -0.5449076811759708816, 0.6444004775717707689, 0.5364919789714475140 ) ) ;
#22448=DIRECTION ( 'NONE',  ( -0.9999697198139514409, -0.000000000000000000, -0.007781995580013368816 ) ) ;
#22449=DIRECTION ( 'NONE',  ( 0.000000000000000000, -0.000000000000000000, -1.000000000000000000 ) ) ;
#22450=CARTESIAN_POINT ( 'NONE',  ( -27.99767448711536133, 0.000000000000000000, 7.557179307314289218 ) ) ;
#22451=DIRECTION ( 'NONE',  ( 0.007781995580012663651, 0.000000000000000000, -0.9999697198139515519 ) ) ;
#22452=CARTESIAN_POINT ( 'NONE',  ( 2.072287782118878319, 0.000000000000000000, -2.950529333540147015 ) ) ;
#22453=DIRECTION ( 'NONE',  ( 0.5449076811759707706, 0.6444004775717708799, -0.5364919789714476250 ) ) ;
#22454=( NAMED_UNIT ( * ) SI_UNIT ( $, .STERADIAN. ) SOLID_ANGLE_UNIT ( ) );
#22457=DIRECTION ( 'NONE',  ( 0.6246952433987893460, 0.7422098413412802076, -0.2426528472758539279 ) ) ;
#22458=DIRECTION ( 'NONE',  ( 0.005961354470445682716, -0.6427876096865404731, -0.7660212471507180654 ) ) ;
#22459=PLANE ( 'NONE',  #32678 ) ;
#22460=PLANE ( 'NONE',  #48650 ) ;
#22461=DIRECTION ( 'NONE',  ( -0.005002170337468016433, -0.7660444431189770143, 0.6427681459581293666 ) ) ;
#22462=CARTESIAN_POINT ( 'NONE',  ( 2.072287782118878319, 0.000000000000000000, -2.950529333540147015 ) ) ;
#22463=CARTESIAN_POINT ( 'NONE',  ( -21.47419595591918906, 0.000000000000000000, 5.222628093224860102 ) ) ;
#22464=VERTEX_POINT ( 'NONE', #53100 ) ;
#22465=AXIS2_PLACEMENT_3D ( 'NONE', #10079, #35956, #1572 ) ;
#22466=ORIENTED_EDGE ( 'NONE', *, *, #208, .T. ) ;
#22468=CARTESIAN_POINT ( 'NONE',  ( -27.06708303904391144, 0.000000000000000000, 7.395095371555332697 ) ) ;
#22469=EDGE_CURVE ( 'NONE', #49361, #5782, #48554, .T. ) ;
#22470=VECTOR ( 'NONE', #11996, 999.9999999999998863 ) ;
#22471=ORIENTED_EDGE ( 'NONE', *, *, #22957, .F. ) ;
#22473=EDGE_LOOP ( 'NONE', ( #1485, #55707, #39660, #17728 ) ) ;
#22474=FACE_OUTER_BOUND ( 'NONE', #33485, .T. ) ;
#22475=EDGE_CURVE ( 'NONE', #11984, #36837, #18751, .T. ) ;
#22476=EDGE_CURVE ( 'NONE', #25453, #52834, #19272, .T. ) ;
#22477=ORIENTED_EDGE ( 'NONE', *, *, #20117, .T. ) ;
#22478=VERTEX_POINT ( 'NONE', #9672 ) ;
#22479=ORIENTED_EDGE ( 'NONE', *, *, #30136, .T. ) ;
#22480=CARTESIAN_POINT ( 'NONE',  ( -17.84275124703420090, 2.714935509636508204, 8.267723343481110376 ) ) ;
#22481=DIRECTION ( 'NONE',  ( -0.9999697198139514409, -0.000000000000000000, -0.007781995580013368816 ) ) ;
#22482=LINE ( 'NONE', #27271, #23941 ) ;
#22483=DIRECTION ( 'NONE',  ( -0.9999697198139514409, -0.000000000000000000, -0.007781995580013368816 ) ) ;
#22484=ORIENTED_EDGE ( 'NONE', *, *, #33185, .T. ) ;
#22485=ORIENTED_EDGE ( 'NONE', *, *, #17522, .F. ) ;
#22486=CARTESIAN_POINT ( 'NONE',  ( -12.90532805278843398, 2.391131607591506114, 5.818443131337661001 ) ) ;
#22487=ORIENTED_EDGE ( 'NONE', *, *, #11359, .F. ) ;
#22488=DIRECTION ( 'NONE',  ( 0.007781995580012663651, -3.146120232559066537E-19, -0.9999697198139514409 ) ) ;
#22489=ORIENTED_EDGE ( 'NONE', *, *, #47669, .F. ) ;
#22490=DIRECTION ( 'NONE',  ( 0.000000000000000000, -1.000000000000000000, 0.000000000000000000 ) ) ;
#22491=LINE ( 'NONE', #39802, #14005 ) ;
#22492=ORIENTED_EDGE ( 'NONE', *, *, #24731, .T. ) ;
#22493=CARTESIAN_POINT ( 'NONE',  ( -3.638205267667341758, -7.220147766006030032, -1.805171095730843112 ) ) ;
#22494=ORIENTED_EDGE ( 'NONE', *, *, #12549, .T. ) ;
#22495=EDGE_CURVE ( 'NONE', #10709, #4830, #53636, .T. ) ;
#22496=PLANE ( 'NONE',  #7337 ) ;
#22497=EDGE_LOOP ( 'NONE', ( #40455, #32248, #47389, #35356 ) ) ;
#22498=EDGE_CURVE ( 'NONE', #7889, #53576, #26986, .T. ) ;
#22499=FACE_OUTER_BOUND ( 'NONE', #41031, .T. ) ;
#22500=LINE ( 'NONE', #10260, #13051 ) ;
#22501=DIRECTION ( 'NONE',  ( -0.005961354470445682716, -0.6427876096865404731, 0.7660212471507180654 ) ) ;
#22502=ORIENTED_EDGE ( 'NONE', *, *, #34113, .T. ) ;
#22503=DIRECTION ( 'NONE',  ( 0.000000000000000000, -1.000000000000000000, 0.000000000000000000 ) ) ;
#22504=AXIS2_PLACEMENT_3D ( 'NONE', #42875, #42032, #28988 ) ;
#22505=CARTESIAN_POINT ( 'NONE',  ( -17.46532115785441519, 0.000000000000000000, 13.67492996699914265 ) ) ;
#22506=EDGE_CURVE ( 'NONE', #29959, #51712, #31791, .T. ) ;
#22508=CARTESIAN_POINT ( 'NONE',  ( -8.875996589204540044, 0.000000000000000000, 10.41778544861944233 ) ) ;
#22509=CARTESIAN_POINT ( 'NONE',  ( -19.69569380384165669, -0.1191753592594177458, 14.58090286586150697 ) ) ;
#22510=DIRECTION ( 'NONE',  ( 0.000000000000000000, -0.000000000000000000, -1.000000000000000000 ) ) ;
#22511=CARTESIAN_POINT ( 'NONE',  ( -14.00280974873554030, 0.000000000000000000, 12.40921378708904044 ) ) ;
#22512=ORIENTED_EDGE ( 'NONE', *, *, #17358, .F. ) ;
#22513=DIRECTION ( 'NONE',  ( 0.000000000000000000, -1.000000000000000000, 0.000000000000000000 ) ) ;
#22514=CARTESIAN_POINT ( 'NONE',  ( -10.37421533196711465, -0.1191753592594197858, 10.96012406864405975 ) ) ;
#22515=DIRECTION ( 'NONE',  ( 0.5449076811759707706, 0.6444004775717708799, -0.5364919789714476250 ) ) ;
#22516=ORIENTED_EDGE ( 'NONE', *, *, #11237, .F. ) ;
#22517=FACE_OUTER_BOUND ( 'NONE', #46047, .T. ) ;
#22518=LINE ( 'NONE', #27308, #36341 ) ;
#22519=ORIENTED_EDGE ( 'NONE', *, *, #16463, .T. ) ;
#22520=LINE ( 'NONE', #22231, #39803 ) ;
#22521=DIRECTION ( 'NONE',  ( 0.000000000000000000, -0.000000000000000000, -1.000000000000000000 ) ) ;
#22522=CARTESIAN_POINT ( 'NONE',  ( -7.594507926423646360, 5.304312555146883490, -0.2684087864660597567 ) ) ;
#22523=CARTESIAN_POINT ( 'NONE',  ( -21.47341775636118655, -0.1191753592594197858, 5.122631121243466090 ) ) ;
#22524=EDGE_LOOP ( 'NONE', ( #44430, #52941, #255, #53627 ) ) ;
#22525=EDGE_LOOP ( 'NONE', ( #22236, #32830, #28432, #38097 ) ) ;
#22526=CARTESIAN_POINT ( 'NONE',  ( 2.072287782118878319, 0.000000000000000000, -2.950529333540147015 ) ) ;
#22527=CARTESIAN_POINT ( 'NONE',  ( -10.27421835998572064, 0.000000000000000000, 10.96090226820206048 ) ) ;
#22530=FACE_OUTER_BOUND ( 'NONE', #15653, .T. ) ;
#22531=ADVANCED_FACE ( 'NONE', ( #14476 ), #49681, .F. ) ;
#22532=LINE ( 'NONE', #13706, #28283 ) ;
#22533=FACE_OUTER_BOUND ( 'NONE', #52166, .T. ) ;
#22534=ORIENTED_EDGE ( 'NONE', *, *, #32406, .T. ) ;
#22535=PLANE ( 'NONE',  #43752 ) ;
#22536=EDGE_CURVE ( 'NONE', #49583, #47620, #10508, .T. ) ;
#22538=ORIENTED_EDGE ( 'NONE', *, *, #12472, .F. ) ;
#22539=CARTESIAN_POINT ( 'NONE',  ( -15.80588551452221857, 0.000000000000000000, 5.266740195748627507 ) ) ;
#22540=DIRECTION ( 'NONE',  ( 0.5364919789714477361, 0.6444004775717706579, 0.5449076811759711036 ) ) ;
#22541=LINE ( 'NONE', #36164, #45698 ) ;
#22542=EDGE_LOOP ( 'NONE', ( #32142, #6682, #11233, #10658 ) ) ;
#22543=VECTOR ( 'NONE', #19007, 1000.000000000000227 ) ;
#22544=CARTESIAN_POINT ( 'NONE',  ( -19.60912206198628027, -0.1191753592594197858, 4.398475361799976113 ) ) ;
#22545=EDGE_LOOP ( 'NONE', ( #25330, #41426, #35448, #26424 ) ) ;
#22546=ADVANCED_FACE ( 'NONE', ( #10203 ), #1105, .F. ) ;
#22547=ORIENTED_EDGE ( 'NONE', *, *, #25582, .T. ) ;
#22548=ORIENTED_EDGE ( 'NONE', *, *, #35772, .F. ) ;
#22549=ORIENTED_EDGE ( 'NONE', *, *, #49046, .F. ) ;
#22550=DIRECTION ( 'NONE',  ( 0.5449076811759707706, 0.6444004775717708799, -0.5364919789714476250 ) ) ;
#22551=EDGE_LOOP ( 'NONE', ( #51616, #5858, #10429, #46983 ) ) ;
#22552=CARTESIAN_POINT ( 'NONE',  ( -18.69292566799212807, -0.1191753592594172323, 5.144269553601169775 ) ) ;
#22553=FACE_OUTER_BOUND ( 'NONE', #53639, .T. ) ;
#22554=ORIENTED_EDGE ( 'NONE', *, *, #31867, .T. ) ;
#22555=LINE ( 'NONE', #944, #5952 ) ;
#22556=ORIENTED_EDGE ( 'NONE', *, *, #4221, .T. ) ;
#22557=CARTESIAN_POINT ( 'NONE',  ( -15.13495153988577968, 0.000000000000000000, 12.76973526769478084 ) ) ;
#22558=EDGE_LOOP ( 'NONE', ( #45056, #913, #15194, #47700 ) ) ;
#22559=CARTESIAN_POINT ( 'NONE',  ( -17.83139810946674686, -0.1191753592594197858, 13.85674710641801788 ) ) ;
#22560=CARTESIAN_POINT ( 'NONE',  ( -9.490784343077956819, 0.000000000000000000, 4.007883507648673849 ) ) ;
#22561=PLANE ( 'NONE',  #21408 ) ;
#22562=CARTESIAN_POINT ( 'NONE',  ( -10.19994581826036040, 0.000000000000000000, 1.417040160424308359 ) ) ;
#22563=DIRECTION ( 'NONE',  ( -0.005002170337468016433, -0.7660444431189770143, 0.6427681459581293666 ) ) ;
#22564=LINE ( 'NONE', #43015, #37406 ) ;
#22565=VERTEX_POINT ( 'NONE', #27834 ) ;
#22566=EDGE_LOOP ( 'NONE', ( #34912, #29553, #13233, #26801 ) ) ;
#22567=DIRECTION ( 'NONE',  ( 0.9999697198139515519, 0.000000000000000000, 0.007781995580013368816 ) ) ;
#22568=EDGE_CURVE ( 'NONE', #34236, #42663, #36911, .T. ) ;
#22569=CARTESIAN_POINT ( 'NONE',  ( -21.47263955680318404, 0.000000000000000000, 5.022634149262071190 ) ) ;
#22570=CARTESIAN_POINT ( 'NONE',  ( -14.94760462649100496, 0.000000000000000000, 2.488088991209854051 ) ) ;
#22571=CARTESIAN_POINT ( 'NONE',  ( -13.46102625666381059, 0.000000000000000000, 2.499657887821534086 ) ) ;
#22572=ORIENTED_EDGE ( 'NONE', *, *, #49047, .T. ) ;
#22573=DIRECTION ( 'NONE',  ( 0.6246952433987894571, -0.7422098413412800966, -0.2426528472758541777 ) ) ;
#22574=DIRECTION ( 'NONE',  ( 0.007781995580012663651, -3.146120232559066537E-19, -0.9999697198139514409 ) ) ;
#22576=DIRECTION ( 'NONE',  ( 0.007781995580012663651, -3.146120232559066537E-19, -0.9999697198139514409 ) ) ;
#22577=DIRECTION ( 'NONE',  ( 0.9999697198139515519, 0.000000000000000000, 0.007781995580013368816 ) ) ;
#22578=ORIENTED_EDGE ( 'NONE', *, *, #42529, .T. ) ;
#22579=EDGE_CURVE ( 'NONE', #4939, #10700, #14219, .T. ) ;
#22580=AXIS2_PLACEMENT_3D ( 'NONE', #40671, #1478, #23608 ) ;
#22582=PLANE ( 'NONE',  #37820 ) ;
#22583=CARTESIAN_POINT ( 'NONE',  ( -14.12565709746768761, 0.000000000000000000, 2.494485576937521820 ) ) ;
#22584=ADVANCED_FACE ( 'NONE', ( #32074 ), #45143, .F. ) ;
#22585=ADVANCED_FACE ( 'NONE', ( #27527 ), #5662, .F. ) ;
#22586=PLANE ( 'NONE',  #34106 ) ;
#22587=CARTESIAN_POINT ( 'NONE',  ( -18.18100488926467762, -1.165603555308155626, 5.657005471572626121 ) ) ;
#22588=EDGE_LOOP ( 'NONE', ( #36349, #12483, #50876, #54705 ) ) ;
#22589=EDGE_LOOP ( 'NONE', ( #36171, #39462, #39663, #20148 ) ) ;
#22590=CARTESIAN_POINT ( 'NONE',  ( -20.56204410600856747, -4.565544526780663581, 4.722652564258249974 ) ) ;
#22591=CARTESIAN_POINT ( 'NONE',  ( -14.10280672071693431, -0.1191753592594197858, 12.40843558753103792 ) ) ;
#22592=FACE_OUTER_BOUND ( 'NONE', #54513, .T. ) ;
#22593=ADVANCED_FACE ( 'NONE', ( #22991 ), #44848, .F. ) ;
#22594=DIRECTION ( 'NONE',  ( 0.9999697198139515519, 0.000000000000000000, 0.007781995580013368816 ) ) ;
#22595=EDGE_CURVE ( 'NONE', #40269, #14453, #25239, .T. ) ;
#22596=CARTESIAN_POINT ( 'NONE',  ( -11.77243710274829525, -0.1191753592594197858, 11.50324088822667612 ) ) ;
#22598=PLANE ( 'NONE',  #30997 ) ;
#22599=DIRECTION ( 'NONE',  ( 0.6427681459581294776, -0.7660444431189769032, 0.005002170337467562802 ) ) ;
#22600=EDGE_CURVE ( 'NONE', #14438, #49029, #51047, .T. ) ;
#22601=CARTESIAN_POINT ( 'NONE',  ( -15.95869604799166375, -4.079838673713163111, 2.950052407828571255 ) ) ;
#22602=CARTESIAN_POINT ( 'NONE',  ( 2.072287782118878319, 0.000000000000000000, -2.950529333540147015 ) ) ;
#22603=ORIENTED_EDGE ( 'NONE', *, *, #10484, .F. ) ;
#22604=CARTESIAN_POINT ( 'NONE',  ( -14.20280369269832832, 0.000000000000000000, 12.40765738797303719 ) ) ;
#22605=ORIENTED_EDGE ( 'NONE', *, *, #30015, .T. ) ;
#22606=FACE_OUTER_BOUND ( 'NONE', #20715, .T. ) ;
#22607=DIRECTION ( 'NONE',  ( 0.007781995580012662783, 0.000000000000000000, -0.9999697198139514409 ) ) ;
#22608=EDGE_CURVE ( 'NONE', #54876, #35486, #32894, .T. ) ;
#22609=ORIENTED_EDGE ( 'NONE', *, *, #14564, .T. ) ;
#22610=CARTESIAN_POINT ( 'NONE',  ( -12.80458192191714595, 0.000000000000000000, 11.86454056839041726 ) ) ;
#22611=EDGE_LOOP ( 'NONE', ( #44174, #32542, #5866, #46586 ) ) ;
#22612=EDGE_CURVE ( 'NONE', #26046, #50963, #2771, .T. ) ;
#22613=VERTEX_POINT ( 'NONE', #37737 ) ;
#22614=ORIENTED_EDGE ( 'NONE', *, *, #35409, .T. ) ;
#22615=DIRECTION ( 'NONE',  ( 0.7660212471507180654, -0.6427876096865404731, 0.005961354470445141482 ) ) ;
#22616=ORIENTED_EDGE ( 'NONE', *, *, #24669, .F. ) ;
#22617=ORIENTED_EDGE ( 'NONE', *, *, #19814, .F. ) ;
#22619=LINE ( 'NONE', #54865, #39439 ) ;
#22620=ORIENTED_EDGE ( 'NONE', *, *, #35399, .T. ) ;
#22621=ORIENTED_EDGE ( 'NONE', *, *, #13636, .F. ) ;
#22622=DIRECTION ( 'NONE',  ( 0.005961354470445682716, -0.6427876096865404731, -0.7660212471507180654 ) ) ;
#22623=ORIENTED_EDGE ( 'NONE', *, *, #23993, .T. ) ;
#22624=VERTEX_POINT ( 'NONE', #46812 ) ;
#22625=FACE_OUTER_BOUND ( 'NONE', #43474, .T. ) ;
#22626=CARTESIAN_POINT ( 'NONE',  ( -16.53317331066696383, 0.000000000000000000, 13.31285208727739899 ) ) ;
#22627=DIRECTION ( 'NONE',  ( 0.000000000000000000, -1.000000000000000000, 0.000000000000000000 ) ) ;
#22628=FACE_OUTER_BOUND ( 'NONE', #28493, .T. ) ;
#22629=ORIENTED_EDGE ( 'NONE', *, *, #56058, .T. ) ;
#22630=PLANE ( 'NONE',  #34660 ) ;
#22631=ORIENTED_EDGE ( 'NONE', *, *, #7641, .T. ) ;
#22632=EDGE_CURVE ( 'NONE', #30203, #33225, #3636, .T. ) ;
#22633=CARTESIAN_POINT ( 'NONE',  ( -16.79925329029790149, 0.000000000000000000, 13.49544742625427496 ) ) ;
#22634=PLANE ( 'NONE',  #34232 ) ;
#22635=DIRECTION ( 'NONE',  ( 0.7660212471507180654, -0.6427876096865404731, 0.005961354470445141482 ) ) ;
#22636=CARTESIAN_POINT ( 'NONE',  ( -22.03910228076049904, -5.213152330870665097, 5.275730040889094141 ) ) ;
#22638=DIRECTION ( 'NONE',  ( -0.005961354470445682716, -0.6427876096865404731, 0.7660212471507180654 ) ) ;
#22639=LINE ( 'NONE', #31725, #24101 ) ;
#22640=ORIENTED_EDGE ( 'NONE', *, *, #25658, .T. ) ;
#22641=CARTESIAN_POINT ( 'NONE',  ( -17.74560456716937296, 0.000000000000000000, 3.774316574337878372 ) ) ;
#22642=ADVANCED_FACE ( 'NONE', ( #50773 ), #38272, .F. ) ;
#22644=FACE_OUTER_BOUND ( 'NONE', #50548, .T. ) ;
#22645=DIRECTION ( 'NONE',  ( 0.000000000000000000, -1.000000000000000000, 0.000000000000000000 ) ) ;
#22646=DIRECTION ( 'NONE',  ( 0.005002170337468016433, -0.7660444431189770143, -0.6427681459581293666 ) ) ;
#22647=CARTESIAN_POINT ( 'NONE',  ( -17.26532721389163072, 0.000000000000000000, 13.67648636611514590 ) ) ;
#22648=EDGE_CURVE ( 'NONE', #4507, #9909, #15562, .T. ) ;
#22649=FACE_OUTER_BOUND ( 'NONE', #17871, .T. ) ;
#22651=ORIENTED_EDGE ( 'NONE', *, *, #40840, .T. ) ;
#22652=FACE_OUTER_BOUND ( 'NONE', #11434, .T. ) ;
#22653=DIRECTION ( 'NONE',  ( 0.000000000000000000, -0.000000000000000000, -1.000000000000000000 ) ) ;
#22654=DIRECTION ( 'NONE',  ( 0.000000000000000000, -0.000000000000000000, -1.000000000000000000 ) ) ;
#22655=LINE ( 'NONE', #49049, #30988 ) ;
#22656=EDGE_CURVE ( 'NONE', #50804, #28121, #16406, .T. ) ;
#22657=DIRECTION ( 'NONE',  ( 0.007781995580012662783, 0.000000000000000000, -0.9999697198139514409 ) ) ;
#22659=DIRECTION ( 'NONE',  ( -0.9999697198139514409, -0.000000000000000000, -0.007781995580013368816 ) ) ;
#22662=EDGE_CURVE ( 'NONE', #1435, #16888, #46500, .T. ) ;
#22663=FACE_OUTER_BOUND ( 'NONE', #29619, .T. ) ;
#22665=ORIENTED_EDGE ( 'NONE', *, *, #22246, .F. ) ;
#22666=ADVANCED_FACE ( 'NONE', ( #41440 ), #11610, .F. ) ;
#22667=ORIENTED_EDGE ( 'NONE', *, *, #23780, .T. ) ;
#22668=ORIENTED_EDGE ( 'NONE', *, *, #28916, .T. ) ;
#22669=VERTEX_POINT ( 'NONE', #7618 ) ;
#22671=FACE_OUTER_BOUND ( 'NONE', #50602, .T. ) ;
#22672=CARTESIAN_POINT ( 'NONE',  ( -18.23691093166689114, -0.1191753592594171213, 6.255814575142474077 ) ) ;
#22673=ORIENTED_EDGE ( 'NONE', *, *, #29835, .F. ) ;
#22674=ORIENTED_EDGE ( 'NONE', *, *, #7426, .F. ) ;
#22675=VECTOR ( 'NONE', #22079, 1000.000000000000114 ) ;
#22676=ORIENTED_EDGE ( 'NONE', *, *, #40051, .T. ) ;
#22677=PLANE ( 'NONE',  #7376 ) ;
#22678=LINE ( 'NONE', #14719, #13271 ) ;
#22679=ORIENTED_EDGE ( 'NONE', *, *, #38751, .F. ) ;
#22680=CARTESIAN_POINT ( 'NONE',  ( -27.06708303904391144, 0.000000000000000000, 7.395095371555332697 ) ) ;
#22681=EDGE_CURVE ( 'NONE', #39740, #36296, #20945, .T. ) ;
#22682=ORIENTED_EDGE ( 'NONE', *, *, #50634, .F. ) ;
#22683=LINE ( 'NONE', #31511, #7362 ) ;
#22684=ADVANCED_FACE ( 'NONE', ( #54459 ), #33201, .F. ) ;
#22685=CARTESIAN_POINT ( 'NONE',  ( -16.81190032086591302, 0.000000000000000000, 3.212244750653343583 ) ) ;
#22686=CARTESIAN_POINT ( 'NONE',  ( -21.47341775636118655, -0.1191753592594197858, 5.122631121243466090 ) ) ;
#22687=PLANE ( 'NONE',  #51406 ) ;
#22688=ORIENTED_EDGE ( 'NONE', *, *, #55280, .T. ) ;
#22689=DIRECTION ( 'NONE',  ( 0.000000000000000000, -1.000000000000000000, 0.000000000000000000 ) ) ;
#22690=DIRECTION ( 'NONE',  ( 0.5364919789714477361, 0.6444004775717706579, 0.5449076811759711036 ) ) ;
#22691=LINE ( 'NONE', #18427, #18517 ) ;
#22692=EDGE_CURVE ( 'NONE', #3186, #15388, #24947, .T. ) ;
#22693=ORIENTED_EDGE ( 'NONE', *, *, #51788, .T. ) ;
#22694=CARTESIAN_POINT ( 'NONE',  ( -19.60990026154428278, 0.000000000000000000, 4.498472333781370125 ) ) ;
#22696=EDGE_CURVE ( 'NONE', #34917, #47902, #2521, .T. ) ;
#22697=EDGE_CURVE ( 'NONE', #41830, #7042, #7082, .T. ) ;
#22698=ADVANCED_FACE ( 'NONE', ( #34576 ), #48188, .F. ) ;
#22699=PLANE ( 'NONE',  #12894 ) ;
#22700=CARTESIAN_POINT ( 'NONE',  ( -14.20280369269832832, 0.000000000000000000, 12.40765738797303719 ) ) ;
#22701=LINE ( 'NONE', #5392, #18592 ) ;
#22702=FACE_OUTER_BOUND ( 'NONE', #6627, .T. ) ;
#22703=DIRECTION ( 'NONE',  ( 0.7660212471507180654, -0.6427876096865404731, 0.005961354470445141482 ) ) ;
#22704=CARTESIAN_POINT ( 'NONE',  ( -25.20278734466900517, 0.000000000000000000, 6.670939612111840944 ) ) ;
#22705=CARTESIAN_POINT ( 'NONE',  ( -11.87243407472968926, 0.000000000000000000, 11.50246268866867361 ) ) ;
#22708=CARTESIAN_POINT ( 'NONE',  ( -17.82299174236657180, -4.079838673713163111, 3.674208167272060788 ) ) ;
#22709=ORIENTED_EDGE ( 'NONE', *, *, #42963, .T. ) ;
#22710=DIRECTION ( 'NONE',  ( -0.7660212471507179544, -0.6427876096865405842, -0.005961354470445141482 ) ) ;
#22711=PLANE ( 'NONE',  #13157 ) ;
#22712=DIRECTION ( 'NONE',  ( -0.005002170337468016433, -0.7660444431189770143, 0.6427681459581293666 ) ) ;
#22713=LINE ( 'NONE', #14226, #55904 ) ;
#22714=LINE ( 'NONE', #26403, #39995 ) ;
#22716=PLANE ( 'NONE',  #33294 ) ;
#22717=CARTESIAN_POINT ( 'NONE',  ( -25.20123094555300369, 0.000000000000000000, 6.470945668149052032 ) ) ;
#22719=VECTOR ( 'NONE', #13079, 999.9999999999998863 ) ;
#22720=EDGE_CURVE ( 'NONE', #13435, #16069, #8462, .T. ) ;
#22721=EDGE_LOOP ( 'NONE', ( #31517, #37202, #50346, #10685 ) ) ;
#22722=EDGE_CURVE ( 'NONE', #53290, #8704, #26621, .T. ) ;
#22723=LINE ( 'NONE', #40035, #591 ) ;
#22724=LINE ( 'NONE', #39503, #1388 ) ;
#22725=EDGE_CURVE ( 'NONE', #16370, #52808, #47936, .T. ) ;
#22726=ORIENTED_EDGE ( 'NONE', *, *, #32616, .F. ) ;
#22727=DIRECTION ( 'NONE',  ( 0.005002170337468016433, -0.7660444431189770143, -0.6427681459581293666 ) ) ;
#22728=VERTEX_POINT ( 'NONE', #17545 ) ;
#22729=LINE ( 'NONE', #292, #36555 ) ;
#22730=EDGE_CURVE ( 'NONE', #24292, #37046, #43116, .T. ) ;
#22731=ORIENTED_EDGE ( 'NONE', *, *, #45998, .T. ) ;
#22732=EDGE_LOOP ( 'NONE', ( #37917, #41613, #35389, #40876 ) ) ;
#22734=DIRECTION ( 'NONE',  ( 0.7660212471507180654, -0.6427876096865404731, 0.005961354470445141482 ) ) ;
#22735=LINE ( 'NONE', #26170, #44110 ) ;
#22736=DIRECTION ( 'NONE',  ( 0.9999697198139515519, 0.000000000000000000, 0.007781995580013368816 ) ) ;
#22737=VECTOR ( 'NONE', #8219, 1000.000000000000227 ) ;
#22738=CARTESIAN_POINT ( 'NONE',  ( -16.53317331066696383, 0.000000000000000000, 13.31285208727739899 ) ) ;
#22739=ORIENTED_EDGE ( 'NONE', *, *, #7285, .F. ) ;
#22740=ORIENTED_EDGE ( 'NONE', *, *, #30452, .F. ) ;
#22741=LINE ( 'NONE', #618, #21836 ) ;
#22742=EDGE_LOOP ( 'NONE', ( #54377, #24741, #7816, #14398 ) ) ;
#22743=LINE ( 'NONE', #23034, #50909 ) ;
#22744=VERTEX_POINT ( 'NONE', #13309 ) ;
#22745=DIRECTION ( 'NONE',  ( -0.5364919789714478471, 0.6444004775717705469, -0.5449076811759709926 ) ) ;
#22746=LINE ( 'NONE', #22196, #18542 ) ;
#22747=ORIENTED_EDGE ( 'NONE', *, *, #5427, .F. ) ;
#22748=AXIS2_PLACEMENT_3D ( 'NONE', #54803, #33254, #24696 ) ;
#22749=DIRECTION ( 'NONE',  ( -0.5364919789714478471, 0.6444004775717705469, -0.5449076811759709926 ) ) ;
#22750=ORIENTED_EDGE ( 'NONE', *, *, #44030, .T. ) ;
#22751=AXIS2_PLACEMENT_3D ( 'NONE', #12163, #8193, #25244 ) ;
#22752=DIRECTION ( 'NONE',  ( 0.007781995580012663651, -3.146120232559066537E-19, -0.9999697198139514409 ) ) ;
#22753=EDGE_CURVE ( 'NONE', #15979, #24781, #12725, .T. ) ;
#22754=EDGE_LOOP ( 'NONE', ( #55968, #15173, #18613, #38494 ) ) ;
#22755=DIRECTION ( 'NONE',  ( 0.9999697198139515519, 0.000000000000000000, 0.007781995580013368816 ) ) ;
#22756=DIRECTION ( 'NONE',  ( 0.9999697198139515519, 0.000000000000000000, 0.007781995580013368816 ) ) ;
#22757=DIRECTION ( 'NONE',  ( 0.7660212471507180654, -0.6427876096865404731, 0.005961354470445141482 ) ) ;
#22758=ORIENTED_EDGE ( 'NONE', *, *, #42445, .F. ) ;
#22759=ADVANCED_FACE ( 'NONE', ( #4231 ), #21240, .F. ) ;
#22760=EDGE_CURVE ( 'NONE', #7707, #15806, #42807, .T. ) ;
#22761=FACE_OUTER_BOUND ( 'NONE', #54324, .T. ) ;
#22762=FACE_OUTER_BOUND ( 'NONE', #53131, .T. ) ;
#22764=EDGE_CURVE ( 'NONE', #20837, #31183, #508, .T. ) ;
#22765=CARTESIAN_POINT ( 'NONE',  ( -19.68728743674148163, -4.079838673713161334, 4.398363926715553873 ) ) ;
#22766=DIRECTION ( 'NONE',  ( -0.5364919789714478471, 0.6444004775717705469, -0.5449076811759709926 ) ) ;
#22768=ORIENTED_EDGE ( 'NONE', *, *, #48950, .F. ) ;
#22769=DIRECTION ( 'NONE',  ( 0.000000000000000000, -1.000000000000000000, 0.000000000000000000 ) ) ;
#22770=CARTESIAN_POINT ( 'NONE',  ( -13.76734565315850745, -4.727446477803162850, 9.788181382680596343 ) ) ;
#22771=FACE_OUTER_BOUND ( 'NONE', #19195, .T. ) ;
#22772=ORIENTED_EDGE ( 'NONE', *, *, #8278, .F. ) ;
#22773=CARTESIAN_POINT ( 'NONE',  ( -16.43317633868556626, -0.1191753592594197858, 13.31363028683540151 ) ) ;
#22774=DIRECTION ( 'NONE',  ( 0.007781995580012663651, -3.146120232559066537E-19, -0.9999697198139514409 ) ) ;
#22775=ORIENTED_EDGE ( 'NONE', *, *, #37135, .T. ) ;
#22776=LINE ( 'NONE', #48329, #16199 ) ;
#22777=VECTOR ( 'NONE', #14227, 999.9999999999998863 ) ;
#22778=VECTOR ( 'NONE', #48025, 1000.000000000000114 ) ;
#22779=LINE ( 'NONE', #43791, #38426 ) ;
#22780=CARTESIAN_POINT ( 'NONE',  ( -14.50831954291707504, -0.1191753592594190225, 4.807503056255493235 ) ) ;
#22781=EDGE_CURVE ( 'NONE', #6333, #30167, #17001, .T. ) ;
#22782=DIRECTION ( 'NONE',  ( 0.000000000000000000, -0.000000000000000000, -1.000000000000000000 ) ) ;
#22783=EDGE_LOOP ( 'NONE', ( #51132, #37333, #37076, #38306 ) ) ;
#22784=ORIENTED_EDGE ( 'NONE', *, *, #27866, .F. ) ;
#22785=DIRECTION ( 'NONE',  ( 0.7660212471507180654, -0.6427876096865404731, 0.005961354470445141482 ) ) ;
#22786=PLANE ( 'NONE',  #42251 ) ;
#22788=CARTESIAN_POINT ( 'NONE',  ( -18.81381921406850211, 0.000000000000000000, 7.828656248828915309 ) ) ;
#22789=EDGE_CURVE ( 'NONE', #15659, #22728, #21546, .T. ) ;
#22790=LINE ( 'NONE', #49182, #15581 ) ;
#22791=DIRECTION ( 'NONE',  ( -0.005961354470445682716, -0.6427876096865404731, 0.7660212471507180654 ) ) ;
#22792=ORIENTED_EDGE ( 'NONE', *, *, #15241, .T. ) ;
#22793=DIRECTION ( 'NONE',  ( 0.6427681459581294776, -0.7660444431189769032, 0.005002170337467562802 ) ) ;
#22794=ADVANCED_FACE ( 'NONE', ( #25497 ), #30048, .F. ) ;
#22795=AXIS2_PLACEMENT_3D ( 'NONE', #41723, #19615, #36948 ) ;
#22796=FACE_OUTER_BOUND ( 'NONE', #20016, .T. ) ;
#22797=ORIENTED_EDGE ( 'NONE', *, *, #14949, .F. ) ;
#22798=ADVANCED_FACE ( 'NONE', ( #3915 ), #22085, .F. ) ;
#22799=CARTESIAN_POINT ( 'NONE',  ( -18.67775241435682432, 0.000000000000000000, 4.136394454059623804 ) ) ;
#22800=DIRECTION ( 'NONE',  ( 0.000000000000000000, -0.000000000000000000, -1.000000000000000000 ) ) ;
#22801=LINE ( 'NONE', #13179, #54694 ) ;
#22802=ORIENTED_EDGE ( 'NONE', *, *, #300, .F. ) ;
#22803=LINE ( 'NONE', #4934, #10365 ) ;
#22804=ADVANCED_FACE ( 'NONE', ( #47655 ), #8775, .F. ) ;
#22805=ORIENTED_EDGE ( 'NONE', *, *, #44269, .T. ) ;
#22806=ORIENTED_EDGE ( 'NONE', *, *, #44249, .F. ) ;
#22807=ORIENTED_EDGE ( 'NONE', *, *, #44499, .T. ) ;
#22808=VERTEX_POINT ( 'NONE', #43396 ) ;
#22811=VERTEX_POINT ( 'NONE', #47353 ) ;
#22812=PLANE ( 'NONE',  #476 ) ;
#22813=FACE_OUTER_BOUND ( 'NONE', #44737, .T. ) ;
#22814=VECTOR ( 'NONE', #42748, 1000.000000000000227 ) ;
#22815=VECTOR ( 'NONE', #37143, 1000.000000000000227 ) ;
#22816=ORIENTED_EDGE ( 'NONE', *, *, #19953, .T. ) ;
#22817=DIRECTION ( 'NONE',  ( 0.007781995580012663651, 0.000000000000000000, -0.9999697198139515519 ) ) ;
#22818=VERTEX_POINT ( 'NONE', #4493 ) ;
#22819=FACE_OUTER_BOUND ( 'NONE', #34297, .T. ) ;
#22820=ORIENTED_EDGE ( 'NONE', *, *, #55468, .F. ) ;
#22821=CARTESIAN_POINT ( 'NONE',  ( -18.66354898467281132, 0.000000000000000000, 14.21960318569776582 ) ) ;
#22822=CARTESIAN_POINT ( 'NONE',  ( -19.79569077582305070, 0.000000000000000000, 14.58012466630350445 ) ) ;
#22823=VECTOR ( 'NONE', #12301, 999.9999999999998863 ) ;
#22824=FACE_OUTER_BOUND ( 'NONE', #31696, .T. ) ;
#22825=CARTESIAN_POINT ( 'NONE',  ( -10.32658747134729893, -0.1191753592594177180, 4.840046262167575719 ) ) ;
#22826=DIRECTION ( 'NONE',  ( -0.5449076811759708816, 0.6444004775717707689, 0.5364919789714475140 ) ) ;
#22827=DIRECTION ( 'NONE',  ( 0.9999697198139515519, 0.000000000000000000, 0.007781995580013368816 ) ) ;
#22828=ORIENTED_EDGE ( 'NONE', *, *, #24153, .T. ) ;
#22829=EDGE_CURVE ( 'NONE', #15522, #51817, #26336, .T. ) ;
#22830=VERTEX_POINT ( 'NONE', #13569 ) ;
#22831=DIRECTION ( 'NONE',  ( -0.9999697198139514409, -0.000000000000000000, -0.007781995580013368816 ) ) ;
#22832=DIRECTION ( 'NONE',  ( 0.005961354470445682716, -0.6427876096865404731, -0.7660212471507180654 ) ) ;
#22833=ADVANCED_FACE ( 'NONE', ( #27185 ), #26929, .F. ) ;
#22834=EDGE_CURVE ( 'NONE', #21349, #5026, #10141, .T. ) ;
#22835=VECTOR ( 'NONE', #2202, 999.9999999999998863 ) ;
#22836=DIRECTION ( 'NONE',  ( -0.005961354470445682716, -0.6427876096865404731, 0.7660212471507180654 ) ) ;
#22837=CARTESIAN_POINT ( 'NONE',  ( -15.37403964991131744, 2.553033558614007603, 7.043083237409386577 ) ) ;
#22838=ORIENTED_EDGE ( 'NONE', *, *, #42963, .F. ) ;
#22839=DIRECTION ( 'NONE',  ( 0.9999697198139515519, 0.000000000000000000, 0.007781995580013368816 ) ) ;
#22840=FACE_OUTER_BOUND ( 'NONE', #21706, .T. ) ;
#22841=ORIENTED_EDGE ( 'NONE', *, *, #2406, .T. ) ;
#22842=CARTESIAN_POINT ( 'NONE',  ( -13.08330893211609869, 0.000000000000000000, 1.763933231766363630 ) ) ;
#22843=PLANE ( 'NONE',  #43074 ) ;
#22844=ORIENTED_EDGE ( 'NONE', *, *, #32289, .T. ) ;
#22845=DIRECTION ( 'NONE',  ( 0.6427681459581294776, -0.7660444431189769032, 0.005002170337467562802 ) ) ;
#22846=DIRECTION ( 'NONE',  ( 0.000000000000000000, -1.000000000000000000, 0.000000000000000000 ) ) ;
#22847=FACE_OUTER_BOUND ( 'NONE', #2343, .T. ) ;
#22848=CARTESIAN_POINT ( 'NONE',  ( -16.18500926415040553, -5.375054281893163477, 11.79011876919352630 ) ) ;
#22850=CARTESIAN_POINT ( 'NONE',  ( -11.40636015113596180, 0.000000000000000000, 11.32142374880780089 ) ) ;
#22851=ORIENTED_EDGE ( 'NONE', *, *, #29591, .T. ) ;
#22852=EDGE_LOOP ( 'NONE', ( #33375, #18058, #27364, #40124 ) ) ;
#22853=LINE ( 'NONE', #35112, #25792 ) ;
#22854=CARTESIAN_POINT ( 'NONE',  ( -19.60834386242827776, 0.000000000000000000, 4.298478389818581213 ) ) ;
#22855=CARTESIAN_POINT ( 'NONE',  ( -29.86352658060627618, 0.000000000000000000, 8.481329010720569883 ) ) ;
#22856=AXIS2_PLACEMENT_3D ( 'NONE', #35571, #23371, #5761 ) ;
#22857=VECTOR ( 'NONE', #33864, 1000.000000000000227 ) ;
#22858=FACE_OUTER_BOUND ( 'NONE', #22104, .T. ) ;
#22860=EDGE_LOOP ( 'NONE', ( #34472, #41653, #1793, #25068 ) ) ;
#22861=DIRECTION ( 'NONE',  ( 0.007781995580012662783, 0.000000000000000000, -0.9999697198139514409 ) ) ;
#22862=ADVANCED_FACE ( 'NONE', ( #52729 ), #13836, .F. ) ;
#22863=CARTESIAN_POINT ( 'NONE',  ( -13.46390031016909283, 0.000000000000000000, 2.868967591079298884 ) ) ;
#22864=CARTESIAN_POINT ( 'NONE',  ( -17.79239240936278321, -0.1191753592594190225, 8.844598409714835796 ) ) ;
#22865=CARTESIAN_POINT ( 'NONE',  ( -32.65997012216863737, 0.000000000000000000, 9.567562649885804404 ) ) ;
#22866=VECTOR ( 'NONE', #19894, 1000.000000000000114 ) ;
#22867=ORIENTED_EDGE ( 'NONE', *, *, #12731, .F. ) ;
#22868=PLANE ( 'NONE',  #2981 ) ;
#22869=ORIENTED_EDGE ( 'NONE', *, *, #41848, .F. ) ;
#22870=PLANE ( 'NONE',  #35897 ) ;
#22871=CARTESIAN_POINT ( 'NONE',  ( -21.47263955680318404, 0.000000000000000000, 5.022634149262071190 ) ) ;
#22872=ORIENTED_EDGE ( 'NONE', *, *, #16092, .F. ) ;
#22873=DIRECTION ( 'NONE',  ( 0.007781995580012663651, -3.146120232559066537E-19, -0.9999697198139514409 ) ) ;
#22874=ADVANCED_FACE ( 'NONE', ( #6190 ), #49326, .F. ) ;
#22875=VECTOR ( 'NONE', #11842, 999.9999999999998863 ) ;
#22876=ORIENTED_EDGE ( 'NONE', *, *, #7430, .T. ) ;
#22877=ORIENTED_EDGE ( 'NONE', *, *, #47970, .F. ) ;
#22879=PLANE ( 'NONE',  #43855 ) ;
#22880=ORIENTED_EDGE ( 'NONE', *, *, #24070, .T. ) ;
#22881=ORIENTED_EDGE ( 'NONE', *, *, #959, .T. ) ;
#22882=CARTESIAN_POINT ( 'NONE',  ( -14.16745024565764943, 0.000000000000000000, 7.864815366509013472 ) ) ;
#22883=CARTESIAN_POINT ( 'NONE',  ( -12.26579185571406327, 0.000000000000000000, 2.339633464714584221 ) ) ;
#22884=VERTEX_POINT ( 'NONE', #40809 ) ;
#22885=EDGE_CURVE ( 'NONE', #43913, #8391, #1882, .T. ) ;
#22886=ORIENTED_EDGE ( 'NONE', *, *, #40972, .F. ) ;
#22887=DIRECTION ( 'NONE',  ( 0.007781995580012663651, -3.146120232559066537E-19, -0.9999697198139514409 ) ) ;
#22888=ORIENTED_EDGE ( 'NONE', *, *, #29748, .T. ) ;
#22889=VECTOR ( 'NONE', #20099, 999.9999999999998863 ) ;
#22890=EDGE_CURVE ( 'NONE', #29145, #10401, #19205, .T. ) ;
#22891=ORIENTED_EDGE ( 'NONE', *, *, #50647, .F. ) ;
#22892=ADVANCED_FACE ( 'NONE', ( #34765 ), #25683, .F. ) ;
#22893=FACE_OUTER_BOUND ( 'NONE', #31347, .T. ) ;
#22894=DIRECTION ( 'NONE',  ( 0.007781995580012662783, 0.000000000000000000, -0.9999697198139514409 ) ) ;
#22895=DIRECTION ( 'NONE',  ( 0.9999697198139515519, 0.000000000000000000, 0.007781995580013368816 ) ) ;
#22896=CARTESIAN_POINT ( 'NONE',  ( -27.06552663992790997, 0.000000000000000000, 7.195101427592543786 ) ) ;
#22897=VECTOR ( 'NONE', #54930, 1000.000000000000114 ) ;
#22898=EDGE_CURVE ( 'NONE', #22811, #21349, #21445, .T. ) ;
#22899=VERTEX_POINT ( 'NONE', #51540 ) ;
#22900=CARTESIAN_POINT ( 'NONE',  ( 2.072287782118878319, 0.000000000000000000, -2.950529333540147015 ) ) ;
#22901=ORIENTED_EDGE ( 'NONE', *, *, #47717, .T. ) ;
#22902=VECTOR ( 'NONE', #41697, 999.9999999999998863 ) ;
#22904=EDGE_CURVE ( 'NONE', #48219, #29153, #9485, .T. ) ;
#22905=CARTESIAN_POINT ( 'NONE',  ( -13.76455401191414651, -4.241740624735664156, 2.092607607751481691 ) ) ;
#22906=EDGE_CURVE ( 'NONE', #51591, #19370, #13735, .T. ) ;
#22907=CARTESIAN_POINT ( 'NONE',  ( -17.46532115785441519, 0.000000000000000000, 13.67492996699914265 ) ) ;
#22908=VECTOR ( 'NONE', #15516, 1000.000000000000227 ) ;
#22909=VECTOR ( 'NONE', #43931, 1000.000000000000227 ) ;
#22910=FACE_OUTER_BOUND ( 'NONE', #1585, .T. ) ;
#22911=LINE ( 'NONE', #26075, #30361 ) ;
#22912=DIRECTION ( 'NONE',  ( 0.005961354470445682716, -0.6427876096865404731, -0.7660212471507180654 ) ) ;
#22913=CARTESIAN_POINT ( 'NONE',  ( 2.072287782118878319, 0.000000000000000000, -2.950529333540147015 ) ) ;
#22914=ORIENTED_EDGE ( 'NONE', *, *, #22612, .F. ) ;
#22915=CARTESIAN_POINT ( 'NONE',  ( -19.62661949931887762, 2.364828787826911416, 7.115266020801516156 ) ) ;
#22916=ORIENTED_EDGE ( 'NONE', *, *, #53723, .F. ) ;
#22917=ADVANCED_FACE ( 'NONE', ( #4116 ), #56084, .F. ) ;
#22918=LINE ( 'NONE', #777, #3883 ) ;
#22919=CARTESIAN_POINT ( 'NONE',  ( -31.72782227498118601, 0.000000000000000000, 9.205484770164058972 ) ) ;
#22920=FACE_OUTER_BOUND ( 'NONE', #35811, .T. ) ;
#22921=AXIS2_PLACEMENT_3D ( 'NONE', #51546, #11532, #24556 ) ;
#22922=DIRECTION ( 'NONE',  ( -0.5364919789714478471, 0.6444004775717705469, -0.5449076811759709926 ) ) ;
#22923=LINE ( 'NONE', #14970, #17776 ) ;
#22924=ADVANCED_FACE ( 'NONE', ( #4950 ), #26247, .F. ) ;
#22926=ORIENTED_EDGE ( 'NONE', *, *, #52415, .T. ) ;
#22927=FACE_OUTER_BOUND ( 'NONE', #49894, .T. ) ;
#22928=CARTESIAN_POINT ( 'NONE',  ( -20.58814680246558027, 3.200641362704007786, 10.13125426308755372 ) ) ;
#22929=FACE_OUTER_BOUND ( 'NONE', #6916, .T. ) ;
#22930=AXIS2_PLACEMENT_3D ( 'NONE', #27216, #32038, #44520 ) ;
#22932=CARTESIAN_POINT ( 'NONE',  ( -15.55273877566505369, 0.000000000000000000, 6.746038521431690249 ) ) ;
#22933=VECTOR ( 'NONE', #30119, 1000.000000000000227 ) ;
#22934=CARTESIAN_POINT ( 'NONE',  ( -9.853328413990368517, -0.1191753592594190225, 3.735733064162294781 ) ) ;
#22937=AXIS2_PLACEMENT_3D ( 'NONE', #55080, #19863, #28954 ) ;
#22938=CARTESIAN_POINT ( 'NONE',  ( -16.46608590270481187, 0.000000000000000000, 4.692264237644060643 ) ) ;
#22939=VECTOR ( 'NONE', #21488, 1000.000000000000227 ) ;
#22940=AXIS2_PLACEMENT_3D ( 'NONE', #29180, #50506, #24368 ) ;
#22941=EDGE_LOOP ( 'NONE', ( #54248, #52490, #46064, #52493, #49178 ) ) ;
#22942=EDGE_CURVE ( 'NONE', #2673, #40139, #25991, .T. ) ;
#22943=AXIS2_PLACEMENT_3D ( 'NONE', #48355, #9464, #44114 ) ;
#22944=EDGE_LOOP ( 'NONE', ( #50873, #52506, #22688, #53742, #5525 ) ) ;
#22945=ORIENTED_EDGE ( 'NONE', *, *, #29322, .T. ) ;
#22946=AXIS2_PLACEMENT_3D ( 'NONE', #24718, #25028, #24187 ) ;
#22947=ORIENTED_EDGE ( 'NONE', *, *, #26273, .F. ) ;
#22948=ORIENTED_EDGE ( 'NONE', *, *, #53604, .T. ) ;
#22949=DIRECTION ( 'NONE',  ( -0.7660212471507179544, -0.6427876096865405842, -0.005961354470445141482 ) ) ;
#22950=DIRECTION ( 'NONE',  ( 0.005002170337468016433, -0.7660444431189770143, -0.6427681459581293666 ) ) ;
#22951=EDGE_CURVE ( 'NONE', #15779, #15067, #21975, .T. ) ;
#22953=ORIENTED_EDGE ( 'NONE', *, *, #26249, .F. ) ;
#22954=VECTOR ( 'NONE', #20929, 1000.000000000000227 ) ;
#22955=ORIENTED_EDGE ( 'NONE', *, *, #5, .T. ) ;
#22956=VECTOR ( 'NONE', #28838, 999.9999999999998863 ) ;
#22957=EDGE_CURVE ( 'NONE', #45114, #34742, #39306, .T. ) ;
#22959=DIRECTION ( 'NONE',  ( -0.5449076811759708816, 0.6444004775717707689, 0.5364919789714475140 ) ) ;
#22960=DIRECTION ( 'NONE',  ( 0.005002170337468016433, -0.7660444431189770143, -0.6427681459581293666 ) ) ;
#22961=EDGE_LOOP ( 'NONE', ( #13584, #30362, #12434, #25718 ) ) ;
#22962=LINE ( 'NONE', #48527, #46402 ) ;
#22963=VECTOR ( 'NONE', #40717, 1000.000000000000227 ) ;
#22964=ORIENTED_EDGE ( 'NONE', *, *, #49549, .T. ) ;
#22965=LINE ( 'NONE', #1662, #39113 ) ;
#22966=EDGE_CURVE ( 'NONE', #18488, #53403, #8361, .T. ) ;
#22967=LINE ( 'NONE', #14457, #22112 ) ;
#22968=VECTOR ( 'NONE', #12143, 1000.000000000000227 ) ;
#22969=EDGE_CURVE ( 'NONE', #21477, #29224, #38769, .T. ) ;
#22970=DIRECTION ( 'NONE',  ( -0.5364919789714478471, 0.6444004775717705469, -0.5449076811759709926 ) ) ;
#22971=DIRECTION ( 'NONE',  ( -0.005961354470445682716, -0.6427876096865404731, 0.7660212471507180654 ) ) ;
#22972=DIRECTION ( 'NONE',  ( -0.5449076811759708816, 0.6444004775717707689, 0.5364919789714475140 ) ) ;
#22973=CARTESIAN_POINT ( 'NONE',  ( -13.31992531437080274, -5.375054281893166142, 1.883740082759787882 ) ) ;
#22975=VECTOR ( 'NONE', #35890, 1000.000000000000114 ) ;
#22976=ORIENTED_EDGE ( 'NONE', *, *, #23710, .T. ) ;
#22977=FACE_OUTER_BOUND ( 'NONE', #1598, .T. ) ;
#22978=ORIENTED_EDGE ( 'NONE', *, *, #32427, .F. ) ;
#22979=AXIS2_PLACEMENT_3D ( 'NONE', #30165, #16837, #21910 ) ;
#22980=ADVANCED_FACE ( 'NONE', ( #52084 ), #12633, .F. ) ;
#22981=VECTOR ( 'NONE', #46730, 1000.000000000000114 ) ;
#22982=CARTESIAN_POINT ( 'NONE',  ( -11.99778742911683871, 1.905425754524007642, 1.281486757967683632 ) ) ;
#22983=DIRECTION ( 'NONE',  ( 0.007781995580012663651, -3.146120232559066537E-19, -0.9999697198139514409 ) ) ;
#22985=CARTESIAN_POINT ( 'NONE',  ( -10.00813838035478298, 0.000000000000000000, 10.77830692922518452 ) ) ;
#22986=FACE_OUTER_BOUND ( 'NONE', #49724, .T. ) ;
#22987=LINE ( 'NONE', #1680, #49411 ) ;
#22989=ADVANCED_FACE ( 'NONE', ( #9202 ), #5249, .F. ) ;
#22990=VECTOR ( 'NONE', #2546, 1000.000000000000227 ) ;
#22991=FACE_OUTER_BOUND ( 'NONE', #21592, .T. ) ;
#22992=VECTOR ( 'NONE', #53332, 999.9999999999998863 ) ;
#22993=CARTESIAN_POINT ( 'NONE',  ( -30.79411802867772607, 0.000000000000000000, 8.643412946479525516 ) ) ;
#22994=VERTEX_POINT ( 'NONE', #29950 ) ;
#22995=PLANE ( 'NONE',  #45673 ) ;
#22996=DIRECTION ( 'NONE',  ( 0.007781995580012662783, 0.000000000000000000, -0.9999697198139514409 ) ) ;
#22998=DIRECTION ( 'NONE',  ( 0.6427681459581294776, -0.7660444431189769032, 0.005002170337467562802 ) ) ;
#22999=DIRECTION ( 'NONE',  ( 0.5449076811759707706, 0.6444004775717708799, -0.5364919789714476250 ) ) ;
#23000=DIRECTION ( 'NONE',  ( 0.5364919789714477361, 0.6444004775717706579, 0.5449076811759711036 ) ) ;
#23001=FACE_OUTER_BOUND ( 'NONE', #41045, .T. ) ;
#23002=ORIENTED_EDGE ( 'NONE', *, *, #55489, .F. ) ;
#23003=ORIENTED_EDGE ( 'NONE', *, *, #45150, .F. ) ;
#23004=AXIS2_PLACEMENT_3D ( 'NONE', #5434, #877, #5705 ) ;
#23005=CARTESIAN_POINT ( 'NONE',  ( -23.33693525117809386, 0.000000000000000000, 5.746789908705562944 ) ) ;
#23006=PLANE ( 'NONE',  #41334 ) ;
#23007=VECTOR ( 'NONE', #51607, 1000.000000000000227 ) ;
#23008=VERTEX_POINT ( 'NONE', #17170 ) ;
#23009=DIRECTION ( 'NONE',  ( 0.005002170337468016433, -0.7660444431189770143, -0.6427681459581293666 ) ) ;
#23010=ADVANCED_FACE ( 'NONE', ( #39867 ), #18013, .F. ) ;
#23011=AXIS2_PLACEMENT_3D ( 'NONE', #40799, #23739, #19486 ) ;
#23012=ORIENTED_EDGE ( 'NONE', *, *, #54140, .T. ) ;
#23013=DIRECTION ( 'NONE',  ( -0.5364919789714478471, 0.6444004775717705469, -0.5449076811759709926 ) ) ;
#23014=ORIENTED_EDGE ( 'NONE', *, *, #55147, .T. ) ;
#23016=EDGE_CURVE ( 'NONE', #5857, #44275, #30534, .T. ) ;
#23018=ADVANCED_FACE ( 'NONE', ( #30233 ), #47548, .F. ) ;
#23019=CARTESIAN_POINT ( 'NONE',  ( -27.06552663992790997, 0.000000000000000000, 7.195101427592543786 ) ) ;
#23020=VECTOR ( 'NONE', #43745, 1000.000000000000000 ) ;
#23021=DIRECTION ( 'NONE',  ( 0.000000000000000000, -1.000000000000000000, 0.000000000000000000 ) ) ;
#23022=DIRECTION ( 'NONE',  ( 0.9999697198139515519, 0.000000000000000000, 0.007781995580013368816 ) ) ;
#23023=ADVANCED_FACE ( 'NONE', ( #24526 ), #14911, .F. ) ;
#23024=ADVANCED_FACE ( 'NONE', ( #23441 ), #45026, .F. ) ;
#23026=AXIS2_PLACEMENT_3D ( 'NONE', #52248, #4810, #44287 ) ;
#23027=PLANE ( 'NONE',  #275 ) ;
#23028=ORIENTED_EDGE ( 'NONE', *, *, #39942, .T. ) ;
#23029=EDGE_LOOP ( 'NONE', ( #55988, #47345, #55720, #49162, #51692 ) ) ;
#23030=AXIS2_PLACEMENT_3D ( 'NONE', #12751, #12186, #21571 ) ;
#23031=AXIS2_PLACEMENT_3D ( 'NONE', #45536, #23686, #10912 ) ;
#23032=FACE_OUTER_BOUND ( 'NONE', #45236, .T. ) ;
#23033=VERTEX_POINT ( 'NONE', #45289 ) ;
#23034=CARTESIAN_POINT ( 'NONE',  ( -3.487307141772567842, 4.852350322572148933, -1.863785052350299232 ) ) ;
#23035=ORIENTED_EDGE ( 'NONE', *, *, #37999, .T. ) ;
#23036=DIRECTION ( 'NONE',  ( 0.005002170337468016433, -0.7660444431189770143, -0.6427681459581293666 ) ) ;
#23037=CARTESIAN_POINT ( 'NONE',  ( -11.67244013076689946, 0.000000000000000000, 11.50401908778467863 ) ) ;
#23038=VERTEX_POINT ( 'NONE', #15205 ) ;
#23039=CARTESIAN_POINT ( 'NONE',  ( -17.74560456716937296, 0.000000000000000000, 3.774316574337878372 ) ) ;
#23042=ADVANCED_FACE ( 'NONE', ( #32520 ), #23692, .F. ) ;
#23043=CARTESIAN_POINT ( 'NONE',  ( -9.442067484779661513, -0.1191753592594197858, 10.59804618892231254 ) ) ;
#23044=AXIS2_PLACEMENT_3D ( 'NONE', #43819, #14315, #5485 ) ;
#23045=ORIENTED_EDGE ( 'NONE', *, *, #51653, .F. ) ;
#23046=CARTESIAN_POINT ( 'NONE',  ( -13.94003342103131082, 0.000000000000000000, 4.342590492342347730 ) ) ;
#23047=DIRECTION ( 'NONE',  ( -0.5364919789714478471, 0.6444004775717705469, -0.5449076811759709926 ) ) ;
#23048=ADVANCED_FACE ( 'NONE', ( #33065 ), #40758, .F. ) ;
#23049=CARTESIAN_POINT ( 'NONE',  ( -25.20200914511100265, -0.1191753592594197858, 6.570942640130446932 ) ) ;
#23050=ORIENTED_EDGE ( 'NONE', *, *, #52503, .T. ) ;
#23051=AXIS2_PLACEMENT_3D ( 'NONE', #1244, #26827, #13749 ) ;
#23052=EDGE_CURVE ( 'NONE', #40111, #39737, #46119, .T. ) ;
#23053=CARTESIAN_POINT ( 'NONE',  ( -10.74029228357944987, 0.000000000000000000, 11.14194120806293320 ) ) ;
#23054=CARTESIAN_POINT ( 'NONE',  ( -23.33693525117809386, 0.000000000000000000, 5.746789908705562944 ) ) ;
#23055=AXIS2_PLACEMENT_3D ( 'NONE', #1606, #39932, #18931 ) ;
#23057=CARTESIAN_POINT ( 'NONE',  ( -12.80458192191714595, 0.000000000000000000, 11.86454056839041726 ) ) ;
#23058=CARTESIAN_POINT ( 'NONE',  ( -14.05150990151598656, -1.813211359398158029, 2.281553818646722132 ) ) ;
#23061=DIRECTION ( 'NONE',  ( -0.5449076811759708816, 0.6444004775717707689, 0.5364919789714475140 ) ) ;
#23062=DIRECTION ( 'NONE',  ( 0.5449076811759707706, 0.6444004775717708799, -0.5364919789714476250 ) ) ;
#23064=ORIENTED_EDGE ( 'NONE', *, *, #48838, .T. ) ;
#23065=VECTOR ( 'NONE', #24606, 1000.000000000000227 ) ;
#23066=DIRECTION ( 'NONE',  ( -0.5364919789714478471, 0.6444004775717705469, -0.5449076811759709926 ) ) ;
#23067=DIRECTION ( 'NONE',  ( 0.9999697198139515519, 0.000000000000000000, 0.007781995580013368816 ) ) ;
#23068=EDGE_LOOP ( 'NONE', ( #26599, #44208, #17271, #45243 ) ) ;
#23069=AXIS2_PLACEMENT_3D ( 'NONE', #4606, #47491, #34432 ) ;
#23070=DIRECTION ( 'NONE',  ( -0.5364919789714478471, 0.6444004775717705469, -0.5449076811759709926 ) ) ;
#23071=CARTESIAN_POINT ( 'NONE',  ( -15.40103151951671734, 0.000000000000000000, 12.95233060667165681 ) ) ;
#23073=ORIENTED_EDGE ( 'NONE', *, *, #45403, .F. ) ;
#23074=VECTOR ( 'NONE', #50985, 999.9999999999998863 ) ;
#23075=VECTOR ( 'NONE', #2696, 999.9999999999998863 ) ;
#23076=ORIENTED_EDGE ( 'NONE', *, *, #44348, .F. ) ;
#23079=DIRECTION ( 'NONE',  ( 0.007781995580012662783, 0.000000000000000000, -0.9999697198139514409 ) ) ;
#23081=EDGE_LOOP ( 'NONE', ( #12557, #33987, #3265, #43231, #46934, #39808, #38089, #7445 ) ) ;
#23082=DIRECTION ( 'NONE',  ( -0.6427681459581293666, -0.7660444431189770143, -0.005002170337467561935 ) ) ;
#23083=ORIENTED_EDGE ( 'NONE', *, *, #41030, .T. ) ;
#23084=CARTESIAN_POINT ( 'NONE',  ( -25.20278734466900517, 0.000000000000000000, 6.670939612111840944 ) ) ;
#23085=VECTOR ( 'NONE', #5032, 1000.000000000000227 ) ;
#23087=ORIENTED_EDGE ( 'NONE', *, *, #11682, .T. ) ;
#23088=AXIS2_PLACEMENT_3D ( 'NONE', #34684, #52007, #13120 ) ;
#23089=CARTESIAN_POINT ( 'NONE',  ( -17.86861875374391317, 0.000000000000000000, 5.789345612113324435 ) ) ;
#23090=DIRECTION ( 'NONE',  ( 0.5449076811759707706, 0.6444004775717708799, -0.5364919789714476250 ) ) ;
#23091=VECTOR ( 'NONE', #27297, 1000.000000000000000 ) ;
#23092=DIRECTION ( 'NONE',  ( 0.007781995580012663651, 0.000000000000000000, -0.9999697198139515519 ) ) ;
#23093=EDGE_CURVE ( 'NONE', #28121, #20361, #45546, .T. ) ;
#23094=ADVANCED_FACE ( 'NONE', ( #50083 ), #49565, .F. ) ;
#23095=VERTEX_POINT ( 'NONE', #24273 ) ;
#23096=DIRECTION ( 'NONE',  ( -0.6427681459581293666, -0.7660444431189770143, -0.005002170337467561935 ) ) ;
#23097=VERTEX_POINT ( 'NONE', #10675 ) ;
#23098=ADVANCED_FACE ( 'NONE', ( #19150 ), #36478, .F. ) ;
#23099=ORIENTED_EDGE ( 'NONE', *, *, #12370, .T. ) ;
#23100=EDGE_LOOP ( 'NONE', ( #19030, #4840, #37123, #48237 ) ) ;
#23101=CARTESIAN_POINT ( 'NONE',  ( -25.20200914511100265, -0.1191753592594197858, 6.570942640130446932 ) ) ;
#23102=VECTOR ( 'NONE', #53563, 1000.000000000000227 ) ;
#23103=ORIENTED_EDGE ( 'NONE', *, *, #17610, .F. ) ;
#23104=VECTOR ( 'NONE', #5308, 999.9999999999998863 ) ;
#23105=LINE ( 'NONE', #27937, #42034 ) ;
#23106=ORIENTED_EDGE ( 'NONE', *, *, #35208, .T. ) ;
#23107=DIRECTION ( 'NONE',  ( 0.000000000000000000, -1.000000000000000000, 0.000000000000000000 ) ) ;
#23108=DIRECTION ( 'NONE',  ( -0.005002170337468016433, -0.7660444431189770143, 0.6427681459581293666 ) ) ;
#23109=VECTOR ( 'NONE', #35288, 1000.000000000000227 ) ;
#23110=ORIENTED_EDGE ( 'NONE', *, *, #50301, .T. ) ;
#23111=DIRECTION ( 'NONE',  ( 0.7660212471507180654, -0.6427876096865404731, 0.005961354470445141482 ) ) ;
#23112=ORIENTED_EDGE ( 'NONE', *, *, #28594, .F. ) ;
#23113=ADVANCED_FACE ( 'NONE', ( #41015 ), #28818, .F. ) ;
#23114=VECTOR ( 'NONE', #34207, 1000.000000000000227 ) ;
#23115=DIRECTION ( 'NONE',  ( 0.005961354470445682716, -0.6427876096865404731, -0.7660212471507180654 ) ) ;
#23116=VECTOR ( 'NONE', #43574, 1000.000000000000227 ) ;
#23117=FACE_OUTER_BOUND ( 'NONE', #6914, .T. ) ;
#23118=DIRECTION ( 'NONE',  ( -0.7660212471507179544, -0.6427876096865405842, -0.005961354470445141482 ) ) ;
#23119=DIRECTION ( 'NONE',  ( 0.000000000000000000, -1.000000000000000000, 0.000000000000000000 ) ) ;
#23120=EDGE_CURVE ( 'NONE', #28250, #9132, #54618, .T. ) ;
#23121=CARTESIAN_POINT ( 'NONE',  ( -14.98157860027400723, -0.1191753592594192307, 5.911816254260776837 ) ) ;
#23122=CARTESIAN_POINT ( 'NONE',  ( 2.072287782118878319, 0.000000000000000000, -2.950529333540147015 ) ) ;
#23123=PLANE ( 'NONE',  #24681 ) ;
#23124=EDGE_LOOP ( 'NONE', ( #14644, #36496, #1974 ) ) ;
#23125=ADVANCED_FACE ( 'NONE', ( #28518 ), #53521, .F. ) ;
#23126=ORIENTED_EDGE ( 'NONE', *, *, #5169, .F. ) ;
#23127=CARTESIAN_POINT ( 'NONE',  ( -13.19350925028023092, 0.000000000000000000, 2.132407697215775499 ) ) ;
#23128=DIRECTION ( 'NONE',  ( -0.005002170337468016433, -0.7660444431189770143, 0.6427681459581293666 ) ) ;
#23129=EDGE_CURVE ( 'NONE', #39009, #21187, #42687, .T. ) ;
#23130=LINE ( 'NONE', #8959, #21538 ) ;
#23131=AXIS2_PLACEMENT_3D ( 'NONE', #32378, #36914, #1688 ) ;
#23133=VERTEX_POINT ( 'NONE', #29675 ) ;
#23134=AXIS2_PLACEMENT_3D ( 'NONE', #11221, #33093, #49590 ) ;
#23135=DIRECTION ( 'NONE',  ( 0.007781995580012663651, -3.146120232559066537E-19, -0.9999697198139514409 ) ) ;
#23136=LINE ( 'NONE', #52943, #25041 ) ;
#23137=ORIENTED_EDGE ( 'NONE', *, *, #31764, .F. ) ;
#23138=LINE ( 'NONE', #44418, #27516 ) ;
#23139=CARTESIAN_POINT ( 'NONE',  ( -16.02950353879027645, 2.229229656569005957, 6.766270303596409796 ) ) ;
#23140=VECTOR ( 'NONE', #31923, 1000.000000000000227 ) ;
#23141=EDGE_LOOP ( 'NONE', ( #12014, #49487, #41779, #12869 ) ) ;
#23143=CARTESIAN_POINT ( 'NONE',  ( -30.79489622823572859, -0.1191753592594197858, 8.743409918460921304 ) ) ;
#23144=VECTOR ( 'NONE', #35836, 999.9999999999998863 ) ;
#23145=DIRECTION ( 'NONE',  ( 0.5449076811759707706, 0.6444004775717708799, -0.5364919789714476250 ) ) ;
#23146=DIRECTION ( 'NONE',  ( 0.7660212471507180654, -0.6427876096865404731, 0.005961354470445141482 ) ) ;
#23147=DIRECTION ( 'NONE',  ( -0.9999697198139514409, -0.000000000000000000, -0.007781995580013368816 ) ) ;
#23148=ORIENTED_EDGE ( 'NONE', *, *, #20410, .T. ) ;
#23149=VECTOR ( 'NONE', #5784, 1000.000000000000227 ) ;
#23150=AXIS2_PLACEMENT_3D ( 'NONE', #16009, #8308, #42409 ) ;
#23151=VERTEX_POINT ( 'NONE', #50920 ) ;
#23152=VECTOR ( 'NONE', #21983, 999.9999999999998863 ) ;
#23153=PLANE ( 'NONE',  #15756 ) ;
#23154=PLANE ( 'NONE',  #51251 ) ;
#23155=DIRECTION ( 'NONE',  ( -0.005961354470445682716, -0.6427876096865404731, 0.7660212471507180654 ) ) ;
#23156=AXIS2_PLACEMENT_3D ( 'NONE', #35424, #39958, #52727 ) ;
#23157=DIRECTION ( 'NONE',  ( 0.005002170337468016433, -0.7660444431189770143, -0.6427681459581293666 ) ) ;
#23158=CARTESIAN_POINT ( 'NONE',  ( -23.33849165029409889, 0.000000000000000000, 5.946783852668351855 ) ) ;
#23159=ORIENTED_EDGE ( 'NONE', *, *, #36568, .T. ) ;
#23161=PLANE ( 'NONE',  #6646 ) ;
#23162=VECTOR ( 'NONE', #19597, 1000.000000000000000 ) ;
#23163=DIRECTION ( 'NONE',  ( 0.005002170337468016433, -0.7660444431189770143, -0.6427681459581293666 ) ) ;
#23164=VECTOR ( 'NONE', #23062, 1000.000000000000114 ) ;
#23166=ORIENTED_EDGE ( 'NONE', *, *, #12536, .T. ) ;
#23167=PLANE ( 'NONE',  #19286 ) ;
#23168=ORIENTED_EDGE ( 'NONE', *, *, #37301, .F. ) ;
#23169=DIRECTION ( 'NONE',  ( 0.005002170337468016433, -0.7660444431189770143, -0.6427681459581293666 ) ) ;
#23170=DIRECTION ( 'NONE',  ( -0.5364919789714478471, 0.6444004775717705469, -0.5449076811759709926 ) ) ;
#23171=EDGE_CURVE ( 'NONE', #8281, #29778, #29362, .T. ) ;
#23172=ORIENTED_EDGE ( 'NONE', *, *, #45436, .T. ) ;
#23173=DIRECTION ( 'NONE',  ( -0.7660212471507179544, -0.6427876096865405842, -0.005961354470445141482 ) ) ;
#23174=EDGE_LOOP ( 'NONE', ( #13112, #26238, #13640, #45610 ) ) ;
#23175=ADVANCED_FACE ( 'NONE', ( #56059 ), #16878, .F. ) ;
#23176=EDGE_CURVE ( 'NONE', #50963, #51710, #37896, .T. ) ;
#23177=AXIS2_PLACEMENT_3D ( 'NONE', #12088, #2715, #50719 ) ;
#23178=ORIENTED_EDGE ( 'NONE', *, *, #24800, .F. ) ;
#23179=ORIENTED_EDGE ( 'NONE', *, *, #45591, .F. ) ;
#23180=LINE ( 'NONE', #657, #23908 ) ;
#23181=ORIENTED_EDGE ( 'NONE', *, *, #12478, .T. ) ;
#23182=VECTOR ( 'NONE', #17430, 1000.000000000000227 ) ;
#23183=ORIENTED_EDGE ( 'NONE', *, *, #30669, .T. ) ;
#23184=CARTESIAN_POINT ( 'NONE',  ( -24.27063949748155380, 0.000000000000000000, 6.308861732390097288 ) ) ;
#23185=LINE ( 'NONE', #31969, #14071 ) ;
#23186=VECTOR ( 'NONE', #29652, 999.9999999999998863 ) ;
#23187=EDGE_LOOP ( 'NONE', ( #42940, #33766, #15368, #49971 ) ) ;
#23188=ORIENTED_EDGE ( 'NONE', *, *, #7532, .T. ) ;
#23189=CARTESIAN_POINT ( 'NONE',  ( -27.06708303904391144, 0.000000000000000000, 7.395095371555332697 ) ) ;
#23190=ORIENTED_EDGE ( 'NONE', *, *, #42118, .T. ) ;
#23191=VECTOR ( 'NONE', #7065, 999.9999999999998863 ) ;
#23192=ORIENTED_EDGE ( 'NONE', *, *, #6086, .F. ) ;
#23193=VECTOR ( 'NONE', #5502, 999.9999999999998863 ) ;
#23194=AXIS2_PLACEMENT_3D ( 'NONE', #8531, #47140, #30402 ) ;
#23195=CARTESIAN_POINT ( 'NONE',  ( -16.81619947299561701, 3.200641362704010007, 3.111797470672864829 ) ) ;
#23196=DIRECTION ( 'NONE',  ( 0.000000000000000000, 1.000000000000000000, 0.000000000000000000 ) ) ;
#23197=PLANE ( 'NONE',  #26001 ) ;
#23198=FACE_OUTER_BOUND ( 'NONE', #49941, .T. ) ;
#23199=ORIENTED_EDGE ( 'NONE', *, *, #54367, .T. ) ;
#23200=CARTESIAN_POINT ( 'NONE',  ( -14.20280369269832832, 0.000000000000000000, 12.40765738797303719 ) ) ;
#23201=ORIENTED_EDGE ( 'NONE', *, *, #3131, .F. ) ;
#23202=VECTOR ( 'NONE', #41437, 999.9999999999998863 ) ;
#23203=AXIS2_PLACEMENT_3D ( 'NONE', #16240, #11964, #25066 ) ;
#23204=VECTOR ( 'NONE', #9305, 999.9999999999998863 ) ;
#23205=DIRECTION ( 'NONE',  ( 0.005961354470445682716, -0.6427876096865404731, -0.7660212471507180654 ) ) ;
#23206=EDGE_CURVE ( 'NONE', #34036, #26165, #3787, .T. ) ;
#23207=DIRECTION ( 'NONE',  ( 0.007781995580012662783, 0.000000000000000000, -0.9999697198139514409 ) ) ;
#23208=VECTOR ( 'NONE', #39416, 999.9999999999998863 ) ;
#23210=CARTESIAN_POINT ( 'NONE',  ( -10.87894692659065221, 0.000000000000000000, 3.258416365829116312 ) ) ;
#23211=ADVANCED_FACE ( 'NONE', ( #16036 ), #51222, .F. ) ;
#23212=CARTESIAN_POINT ( 'NONE',  ( -14.94838282604900748, -0.1191753592594197858, 2.588085963191248506 ) ) ;
#23213=LINE ( 'NONE', #31993, #40402 ) ;
#23215=FACE_OUTER_BOUND ( 'NONE', #12393, .T. ) ;
#23216=EDGE_CURVE ( 'NONE', #35486, #26049, #38436, .T. ) ;
#23217=ORIENTED_EDGE ( 'NONE', *, *, #33534, .F. ) ;
#23220=DIRECTION ( 'NONE',  ( 0.5364919789714477361, 0.6444004775717706579, 0.5449076811759711036 ) ) ;
#23222=CARTESIAN_POINT ( 'NONE',  ( -16.28621033327900136, 0.000000000000000000, 7.278988559564416150 ) ) ;
#23223=FACE_OUTER_BOUND ( 'NONE', #37184, .T. ) ;
#23224=AXIS2_PLACEMENT_3D ( 'NONE', #11687, #3157, #46048 ) ;
#23228=FACE_OUTER_BOUND ( 'NONE', #21639, .T. ) ;
#23229=CARTESIAN_POINT ( 'NONE',  ( -16.43317633868556626, -0.1191753592594197858, 13.31363028683540151 ) ) ;
#23230=VECTOR ( 'NONE', #36752, 999.9999999999998863 ) ;
#23232=VECTOR ( 'NONE', #35479, 1000.000000000000114 ) ;
#23233=LINE ( 'NONE', #4770, #6735 ) ;
#23234=LINE ( 'NONE', #36856, #31983 ) ;
#23235=VECTOR ( 'NONE', #18154, 999.9999999999998863 ) ;
#23236=VECTOR ( 'NONE', #26519, 999.9999999999998863 ) ;
#23237=LINE ( 'NONE', #32319, #5153 ) ;
#23238=LINE ( 'NONE', #28305, #222 ) ;
#23239=ADVANCED_FACE ( 'NONE', ( #51770 ), #42981, .F. ) ;
#23240=VECTOR ( 'NONE', #43867, 999.9999999999998863 ) ;
#23241=ORIENTED_EDGE ( 'NONE', *, *, #5581, .T. ) ;
#23242=AXIS2_PLACEMENT_3D ( 'NONE', #482, #22366, #5875 ) ;
#23243=EDGE_CURVE ( 'NONE', #15067, #34449, #51518, .T. ) ;
#23244=AXIS2_PLACEMENT_3D ( 'NONE', #42066, #20505, #13648 ) ;
#23245=ORIENTED_EDGE ( 'NONE', *, *, #30261, .F. ) ;
#23246=VECTOR ( 'NONE', #13567, 999.9999999999998863 ) ;
#23247=ORIENTED_EDGE ( 'NONE', *, *, #2956, .T. ) ;
#23248=VERTEX_POINT ( 'NONE', #37603 ) ;
#23249=VERTEX_POINT ( 'NONE', #3524 ) ;
#23251=PLANE ( 'NONE',  #54782 ) ;
#23252=ORIENTED_EDGE ( 'NONE', *, *, #21624, .T. ) ;
#23253=ORIENTED_EDGE ( 'NONE', *, *, #54210, .F. ) ;
#23254=EDGE_LOOP ( 'NONE', ( #21207, #48528, #50401, #11364 ) ) ;
#23255=AXIS2_PLACEMENT_3D ( 'NONE', #52423, #52675, #48728 ) ;
#23256=EDGE_CURVE ( 'NONE', #12044, #38354, #42432, .T. ) ;
#23258=DIRECTION ( 'NONE',  ( 0.6427681459581294776, -0.7660444431189769032, 0.005002170337467562802 ) ) ;
#23259=CARTESIAN_POINT ( 'NONE',  ( -13.69485363937393529, -2.460819163488158878, 6.040101447381037936 ) ) ;
#23260=ORIENTED_EDGE ( 'NONE', *, *, #4619, .T. ) ;
#23261=VECTOR ( 'NONE', #44357, 1000.000000000000000 ) ;
#23262=LINE ( 'NONE', #53612, #15595 ) ;
#23263=VERTEX_POINT ( 'NONE', #47522 ) ;
#23264=DIRECTION ( 'NONE',  ( 0.007781995580012662783, 0.000000000000000000, -0.9999697198139514409 ) ) ;
#23265=VECTOR ( 'NONE', #2788, 1000.000000000000114 ) ;
#23267=DIRECTION ( 'NONE',  ( 0.9999697198139515519, 0.000000000000000000, 0.007781995580013368816 ) ) ;
#23268=PLANE ( 'NONE',  #52342 ) ;
#23269=VECTOR ( 'NONE', #778, 1000.000000000000227 ) ;
#23271=LINE ( 'NONE', #36062, #34749 ) ;
#23272=FACE_OUTER_BOUND ( 'NONE', #40767, .T. ) ;
#23273=ORIENTED_EDGE ( 'NONE', *, *, #32280, .T. ) ;
#23274=LINE ( 'NONE', #827, #51869 ) ;
#23275=ORIENTED_EDGE ( 'NONE', *, *, #37958, .F. ) ;
#23276=VECTOR ( 'NONE', #24300, 999.9999999999998863 ) ;
#23277=LINE ( 'NONE', #31784, #8352 ) ;
#23278=CARTESIAN_POINT ( 'NONE',  ( -16.05622515956926577, 1.743523803501507485, 2.863087317488263395 ) ) ;
#23279=DIRECTION ( 'NONE',  ( 0.000000000000000000, -0.000000000000000000, -1.000000000000000000 ) ) ;
#23280=DIRECTION ( 'NONE',  ( -0.7660212471507179544, -0.6427876096865405842, -0.005961354470445141482 ) ) ;
#23281=EDGE_CURVE ( 'NONE', #17923, #904, #25965, .T. ) ;
#23282=DIRECTION ( 'NONE',  ( -0.5364919789714478471, 0.6444004775717705469, -0.5449076811759709926 ) ) ;
#23283=CARTESIAN_POINT ( 'NONE',  ( -10.70194541067012395, 0.000000000000000000, 6.214450391007236618 ) ) ;
#23284=PLANE ( 'NONE',  #8028 ) ;
#23285=VECTOR ( 'NONE', #45632, 1000.000000000000227 ) ;
#23286=AXIS2_PLACEMENT_3D ( 'NONE', #50066, #37293, #15713 ) ;
#23287=CARTESIAN_POINT ( 'NONE',  ( -17.10315536259745528, 0.7721120973665037690, 3.300743681568104826 ) ) ;
#23289=VERTEX_POINT ( 'NONE', #29928 ) ;
#23290=DIRECTION ( 'NONE',  ( -0.005002170337468016433, -0.7660444431189770143, 0.6427681459581293666 ) ) ;
#23291=PLANE ( 'NONE',  #43065 ) ;
#23292=DIRECTION ( 'NONE',  ( -0.005002170337468016433, -0.7660444431189770143, 0.6427681459581293666 ) ) ;
#23293=CARTESIAN_POINT ( 'NONE',  ( -16.98837300675671713, 1.743523803501507485, 3.225165197210008383 ) ) ;
#23294=EDGE_CURVE ( 'NONE', #9654, #9899, #8335, .T. ) ;
#23295=DIRECTION ( 'NONE',  ( 0.007781995580012663651, 0.000000000000000000, -0.9999697198139515519 ) ) ;
#23296=EDGE_CURVE ( 'NONE', #43832, #36287, #3245, .T. ) ;
#23298=EDGE_CURVE ( 'NONE', #14383, #37255, #21420, .T. ) ;
#23299=DIRECTION ( 'NONE',  ( -0.5364919789714478471, 0.6444004775717705469, -0.5449076811759709926 ) ) ;
#23300=VECTOR ( 'NONE', #50922, 1000.000000000000000 ) ;
#23301=VERTEX_POINT ( 'NONE', #46379 ) ;
#23302=EDGE_LOOP ( 'NONE', ( #3864, #9274, #33500, #18553 ) ) ;
#23303=CARTESIAN_POINT ( 'NONE',  ( -15.35981059310210739, 0.000000000000000000, 7.655530086358199426 ) ) ;
#23304=PLANE ( 'NONE',  #3215 ) ;
#23305=ADVANCED_FACE ( 'NONE', ( #20574 ), #33610, .F. ) ;
#23306=ORIENTED_EDGE ( 'NONE', *, *, #30891, .F. ) ;
#23307=ADVANCED_FACE ( 'NONE', ( #46973 ), #8075, .F. ) ;
#23308=FACE_OUTER_BOUND ( 'NONE', #20604, .T. ) ;
#23309=VECTOR ( 'NONE', #14696, 1000.000000000000000 ) ;
#23310=ORIENTED_EDGE ( 'NONE', *, *, #8915, .T. ) ;
#23311=DIRECTION ( 'NONE',  ( 0.6427681459581294776, -0.7660444431189769032, 0.005002170337467562802 ) ) ;
#23312=EDGE_CURVE ( 'NONE', #37777, #8995, #35312, .T. ) ;
#23313=VECTOR ( 'NONE', #5402, 999.9999999999998863 ) ;
#23314=ORIENTED_EDGE ( 'NONE', *, *, #47082, .F. ) ;
#23315=ORIENTED_EDGE ( 'NONE', *, *, #13963, .T. ) ;
#23316=ORIENTED_EDGE ( 'NONE', *, *, #25966, .T. ) ;
#23317=CARTESIAN_POINT ( 'NONE',  ( -19.60990026154428278, 0.000000000000000000, 4.498472333781370125 ) ) ;
#23318=DIRECTION ( 'NONE',  ( 0.6427681459581294776, -0.7660444431189769032, 0.005002170337467562802 ) ) ;
#23319=LINE ( 'NONE', #32403, #51183 ) ;
#23320=EDGE_CURVE ( 'NONE', #37770, #36287, #13710, .T. ) ;
#23321=AXIS2_PLACEMENT_3D ( 'NONE', #35760, #22971, #44830 ) ;
#23322=DIRECTION ( 'NONE',  ( 0.005961354470445682716, -0.6427876096865404731, -0.7660212471507180654 ) ) ;
#23323=ORIENTED_EDGE ( 'NONE', *, *, #25143, .T. ) ;
#23324=ORIENTED_EDGE ( 'NONE', *, *, #52960, .F. ) ;
#23325=EDGE_CURVE ( 'NONE', #48176, #20000, #44377, .T. ) ;
#23326=VECTOR ( 'NONE', #14546, 999.9999999999998863 ) ;
#23327=CARTESIAN_POINT ( 'NONE',  ( -23.33849165029409889, 0.000000000000000000, 5.946783852668351855 ) ) ;
#23328=VERTEX_POINT ( 'NONE', #40112 ) ;
#23329=DIRECTION ( 'NONE',  ( 0.7660212471507180654, -0.6427876096865404731, 0.005961354470445141482 ) ) ;
#23330=ORIENTED_EDGE ( 'NONE', *, *, #20483, .T. ) ;
#23331=CARTESIAN_POINT ( 'NONE',  ( -13.57042358871905385, -0.1191753592594186895, 3.706805770018217316 ) ) ;
#23333=ORIENTED_EDGE ( 'NONE', *, *, #5881, .T. ) ;
#23334=LINE ( 'NONE', #40649, #31332 ) ;
#23335=EDGE_LOOP ( 'NONE', ( #38543, #27205, #23188, #47106 ) ) ;
#23336=FACE_OUTER_BOUND ( 'NONE', #39547, .T. ) ;
#23337=ORIENTED_EDGE ( 'NONE', *, *, #51364, .T. ) ;
#23338=LINE ( 'NONE', #36959, #43958 ) ;
#23339=DIRECTION ( 'NONE',  ( 0.5449076811759707706, 0.6444004775717708799, -0.5364919789714476250 ) ) ;
#23340=DIRECTION ( 'NONE',  ( -0.5364919789714478471, 0.6444004775717705469, -0.5449076811759709926 ) ) ;
#23341=ORIENTED_EDGE ( 'NONE', *, *, #32491, .F. ) ;
#23342=CARTESIAN_POINT ( 'NONE',  ( -1.753914626039396296, 5.922546351860411562, 3.899653579608918896 ) ) ;
#23343=DIRECTION ( 'NONE',  ( -0.005002170337468016433, -0.7660444431189770143, 0.6427681459581293666 ) ) ;
#23345=ADVANCED_FACE ( 'NONE', ( #48072 ), #53204, .F. ) ;
#23346=DIRECTION ( 'NONE',  ( 0.000000000000000000, -0.000000000000000000, -1.000000000000000000 ) ) ;
#23347=DIRECTION ( 'NONE',  ( -0.6427681459581293666, -0.7660444431189770143, -0.005002170337467561935 ) ) ;
#23348=PLANE ( 'NONE',  #38803 ) ;
#23349=VECTOR ( 'NONE', #16284, 1000.000000000000227 ) ;
#23351=ORIENTED_EDGE ( 'NONE', *, *, #20555, .T. ) ;
#23352=CARTESIAN_POINT ( 'NONE',  ( -14.46888367232926420, 0.000000000000000000, 12.59025272694991315 ) ) ;
#23353=CARTESIAN_POINT ( 'NONE',  ( -16.01737567250614092, 0.000000000000000000, 6.742422609663679900 ) ) ;
#23355=ORIENTED_EDGE ( 'NONE', *, *, #29506, .F. ) ;
#23356=PLANE ( 'NONE',  #51064 ) ;
#23357=DIRECTION ( 'NONE',  ( -0.005002170337468016433, -0.7660444431189770143, 0.6427681459581293666 ) ) ;
#23358=ORIENTED_EDGE ( 'NONE', *, *, #55538, .F. ) ;
#23359=EDGE_CURVE ( 'NONE', #31029, #41467, #31329, .T. ) ;
#23360=EDGE_CURVE ( 'NONE', #4025, #4723, #26784, .T. ) ;
#23361=VECTOR ( 'NONE', #14044, 999.9999999999998863 ) ;
#23362=DIRECTION ( 'NONE',  ( 0.5364919789714477361, 0.6444004775717706579, 0.5449076811759711036 ) ) ;
#23363=LINE ( 'NONE', #44364, #23326 ) ;
#23364=ADVANCED_FACE ( 'NONE', ( #14000 ), #39006, .F. ) ;
#23365=DIRECTION ( 'NONE',  ( 0.000000000000000000, -0.000000000000000000, -1.000000000000000000 ) ) ;
#23366=ORIENTED_EDGE ( 'NONE', *, *, #28922, .T. ) ;
#23367=EDGE_LOOP ( 'NONE', ( #32715, #37060, #40810, #37978 ) ) ;
#23370=FACE_OUTER_BOUND ( 'NONE', #28672, .T. ) ;
#23371=DIRECTION ( 'NONE',  ( 0.005961354470445682716, -0.6427876096865404731, -0.7660212471507180654 ) ) ;
#23372=EDGE_LOOP ( 'NONE', ( #13529, #15583, #2481, #39863 ) ) ;
#23373=ADVANCED_FACE ( 'NONE', ( #27069 ), #18538, .F. ) ;
#23375=EDGE_LOOP ( 'NONE', ( #231, #23921, #49353, #14323 ) ) ;
#23376=DIRECTION ( 'NONE',  ( 0.005002170337468016433, -0.7660444431189770143, -0.6427681459581293666 ) ) ;
#23377=ADVANCED_FACE ( 'NONE', ( #52358 ), #22535, .F. ) ;
#23378=DIRECTION ( 'NONE',  ( 0.9999697198139515519, 0.000000000000000000, 0.007781995580013368816 ) ) ;
#23379=EDGE_LOOP ( 'NONE', ( #43851, #48598, #55779, #10610 ) ) ;
#23380=CARTESIAN_POINT ( 'NONE',  ( -18.12751359961164965, 0.000000000000000000, 5.048666692945789514 ) ) ;
#23381=CARTESIAN_POINT ( 'NONE',  ( -18.32331583567987110, 0.000000000000000000, 4.508484831277049132 ) ) ;
#23382=DIRECTION ( 'NONE',  ( -0.5449076811759708816, 0.6444004775717707689, 0.5364919789714475140 ) ) ;
#23383=ORIENTED_EDGE ( 'NONE', *, *, #8942, .F. ) ;
#23384=ADVANCED_FACE ( 'NONE', ( #47820 ), #43291, .F. ) ;
#23386=ORIENTED_EDGE ( 'NONE', *, *, #28219, .F. ) ;
#23387=ORIENTED_EDGE ( 'NONE', *, *, #38026, .T. ) ;
#23388=ORIENTED_EDGE ( 'NONE', *, *, #48035, .T. ) ;
#23390=VERTEX_POINT ( 'NONE', #14308 ) ;
#23392=ORIENTED_EDGE ( 'NONE', *, *, #1647, .F. ) ;
#23393=DIRECTION ( 'NONE',  ( 0.5449076811759707706, 0.6444004775717708799, -0.5364919789714476250 ) ) ;
#23394=DIRECTION ( 'NONE',  ( 0.5449076811759707706, 0.6444004775717708799, -0.5364919789714476250 ) ) ;
#23395=VECTOR ( 'NONE', #4896, 999.9999999999998863 ) ;
#23396=EDGE_LOOP ( 'NONE', ( #35326, #3421, #55200, #14375 ) ) ;
#23397=LINE ( 'NONE', #45244, #16768 ) ;
#23398=ORIENTED_EDGE ( 'NONE', *, *, #36259, .F. ) ;
#23399=DIRECTION ( 'NONE',  ( 0.9999697198139515519, 0.000000000000000000, 0.007781995580013368816 ) ) ;
#23400=CARTESIAN_POINT ( 'NONE',  ( -16.93098182883635161, 2.229229656569007734, 3.187375955030960384 ) ) ;
#23401=CARTESIAN_POINT ( 'NONE',  ( -23.33693525117809386, 0.000000000000000000, 5.746789908705562944 ) ) ;
#23402=CARTESIAN_POINT ( 'NONE',  ( -17.22853674009830982, 0.000000000000000000, 8.948989493022244446 ) ) ;
#23403=FACE_OUTER_BOUND ( 'NONE', #13181, .T. ) ;
#23404=LINE ( 'NONE', #10337, #49117 ) ;
#23405=CARTESIAN_POINT ( 'NONE',  ( -18.29747203306047609, -0.1191753592594177458, 14.03778604627889059 ) ) ;
#23406=ORIENTED_EDGE ( 'NONE', *, *, #26105, .T. ) ;
#23407=EDGE_CURVE ( 'NONE', #49493, #13272, #13456, .T. ) ;
#23408=ORIENTED_EDGE ( 'NONE', *, *, #44682, .F. ) ;
#23409=FACE_OUTER_BOUND ( 'NONE', #45644, .T. ) ;
#23410=DIRECTION ( 'NONE',  ( -0.005002170337468016433, -0.7660444431189770143, 0.6427681459581293666 ) ) ;
#23411=EDGE_CURVE ( 'NONE', #2305, #20314, #43537, .T. ) ;
#23412=CARTESIAN_POINT ( 'NONE',  ( -14.66887761629205222, 0.000000000000000000, 12.58869632783390990 ) ) ;
#23413=PLANE ( 'NONE',  #41252 ) ;
#23414=ORIENTED_EDGE ( 'NONE', *, *, #48616, .T. ) ;
#23416=FACE_OUTER_BOUND ( 'NONE', #11312, .T. ) ;
#23417=CARTESIAN_POINT ( 'NONE',  ( -14.94760462649100496, 0.000000000000000000, 2.488088991209854051 ) ) ;
#23418=EDGE_LOOP ( 'NONE', ( #8903, #54271, #35801, #17234, #38761 ) ) ;
#23419=CARTESIAN_POINT ( 'NONE',  ( -20.50190040964466220, 0.9340140483890051470, 4.615766159821488301 ) ) ;
#23420=LINE ( 'NONE', #44165, #45769 ) ;
#23421=EDGE_LOOP ( 'NONE', ( #20786, #48034, #21503, #35670 ) ) ;
#23422=EDGE_CURVE ( 'NONE', #24462, #1004, #21950, .T. ) ;
#23423=EDGE_CURVE ( 'NONE', #36489, #2552, #367, .T. ) ;
#23424=EDGE_CURVE ( 'NONE', #722, #23833, #671, .T. ) ;
#23426=FACE_OUTER_BOUND ( 'NONE', #9256, .T. ) ;
#23427=PLANE ( 'NONE',  #54968 ) ;
#23428=ADVANCED_FACE ( 'NONE', ( #10302 ), #11118, .F. ) ;
#23429=LINE ( 'NONE', #45531, #40523 ) ;
#23430=CARTESIAN_POINT ( 'NONE',  ( -16.69028063513684401, -0.5179957512181557755, 3.347866143715504172 ) ) ;
#23431=ORIENTED_EDGE ( 'NONE', *, *, #13845, .F. ) ;
#23432=ORIENTED_EDGE ( 'NONE', *, *, #11744, .F. ) ;
#23433=CARTESIAN_POINT ( 'NONE',  ( -21.24361069134453928, 2.876837460659007473, 9.854441329274578720 ) ) ;
#23435=CARTESIAN_POINT ( 'NONE',  ( -17.73140113748535285, 0.000000000000000000, 13.85752530597602039 ) ) ;
#23436=AXIS2_PLACEMENT_3D ( 'NONE', #22705, #53098, #14216 ) ;
#23437=CARTESIAN_POINT ( 'NONE',  ( -19.67003419247834373, 2.714935509636508204, 4.235820352017147350 ) ) ;
#23438=EDGE_CURVE ( 'NONE', #24207, #37392, #28165, .T. ) ;
#23439=LINE ( 'NONE', #54616, #49416 ) ;
#23440=ORIENTED_EDGE ( 'NONE', *, *, #51691, .T. ) ;
#23441=FACE_OUTER_BOUND ( 'NONE', #3177, .T. ) ;
#23442=LINE ( 'NONE', #10377, #7527 ) ;
#23444=DIRECTION ( 'NONE',  ( -0.005002170337468016433, -0.7660444431189770143, 0.6427681459581293666 ) ) ;
#23446=ORIENTED_EDGE ( 'NONE', *, *, #28948, .F. ) ;
#23447=EDGE_CURVE ( 'NONE', #40865, #15160, #41232, .T. ) ;
#23448=DIRECTION ( 'NONE',  ( -0.9999697198139514409, -0.000000000000000000, -0.007781995580013368816 ) ) ;
#23449=EDGE_LOOP ( 'NONE', ( #22429, #22347, #39522, #48747 ) ) ;
#23450=CARTESIAN_POINT ( 'NONE',  ( 2.072287782118878319, 0.000000000000000000, -2.950529333540147015 ) ) ;
#23451=FACE_OUTER_BOUND ( 'NONE', #15466, .T. ) ;
#23452=ORIENTED_EDGE ( 'NONE', *, *, #50337, .T. ) ;
#23453=ADVANCED_FACE ( 'NONE', ( #28442 ), #45760, .F. ) ;
#23454=FACE_OUTER_BOUND ( 'NONE', #54984, .T. ) ;
#23455=ORIENTED_EDGE ( 'NONE', *, *, #37989, .T. ) ;
#23456=EDGE_CURVE ( 'NONE', #10838, #25675, #32456, .T. ) ;
#23457=VERTEX_POINT ( 'NONE', #19922 ) ;
#23460=ORIENTED_EDGE ( 'NONE', *, *, #47830, .T. ) ;
#23461=ORIENTED_EDGE ( 'NONE', *, *, #406, .T. ) ;
#23463=DIRECTION ( 'NONE',  ( 0.7660212471507180654, -0.6427876096865404731, 0.005961354470445141482 ) ) ;
#23464=ORIENTED_EDGE ( 'NONE', *, *, #39015, .T. ) ;
#23465=ORIENTED_EDGE ( 'NONE', *, *, #41662, .T. ) ;
#23466=DIRECTION ( 'NONE',  ( 0.9999697198139515519, 0.000000000000000000, 0.007781995580013368816 ) ) ;
#23467=ORIENTED_EDGE ( 'NONE', *, *, #54619, .F. ) ;
#23468=VERTEX_POINT ( 'NONE', #1764 ) ;
#23469=DIRECTION ( 'NONE',  ( -0.6427681459581293666, -0.7660444431189770143, -0.005002170337467561935 ) ) ;
#23470=PLANE ( 'NONE',  #14899 ) ;
#23472=DIRECTION ( 'NONE',  ( -0.005002170337468016433, -0.7660444431189770143, 0.6427681459581293666 ) ) ;
#23473=ORIENTED_EDGE ( 'NONE', *, *, #51142, .F. ) ;
#23474=DIRECTION ( 'NONE',  ( -0.6427681459581293666, -0.7660444431189770143, -0.005002170337467561935 ) ) ;
#23475=ORIENTED_EDGE ( 'NONE', *, *, #48325, .F. ) ;
#23476=VECTOR ( 'NONE', #21677, 999.9999999999998863 ) ;
#23478=CARTESIAN_POINT ( 'NONE',  ( -12.33850799832341849, 0.000000000000000000, 11.68350162852954632 ) ) ;
#23479=DIRECTION ( 'NONE',  ( 0.5449076811759707706, 0.6444004775717708799, -0.5364919789714476250 ) ) ;
#23480=FACE_OUTER_BOUND ( 'NONE', #26580, .T. ) ;
#23481=CARTESIAN_POINT ( 'NONE',  ( -34.64355613791357769, -1.000000000000000000, 10.23836012842048326 ) ) ;
#23482=CARTESIAN_POINT ( 'NONE',  ( -5.572931691540063071, -7.450474849124534948, 5.383089502214839506 ) ) ;
#23483=EDGE_LOOP ( 'NONE', ( #42357, #56020, #52629, #41101 ) ) ;
#23484=LINE ( 'NONE', #48177, #2933 ) ;
#23485=EDGE_LOOP ( 'NONE', ( #53345, #40684, #31436, #17511 ) ) ;
#23486=ADVANCED_FACE ( 'NONE', ( #19665 ), #31874, .F. ) ;
#23487=ADVANCED_FACE ( 'NONE', ( #32167 ), #24205, .F. ) ;
#23488=DIRECTION ( 'NONE',  ( 0.5364919789714477361, 0.6444004775717706579, 0.5449076811759711036 ) ) ;
#23489=CARTESIAN_POINT ( 'NONE',  ( -21.47263955680318404, 0.000000000000000000, 5.022634149262071190 ) ) ;
#23490=LINE ( 'NONE', #19202, #39908 ) ;
#23491=DIRECTION ( 'NONE',  ( -0.7660212471507179544, -0.6427876096865405842, -0.005961354470445141482 ) ) ;
#23493=CARTESIAN_POINT ( 'NONE',  ( -16.06709938707323460, 0.000000000000000000, 13.13181314741652628 ) ) ;
#23494=DIRECTION ( 'NONE',  ( 0.6427681459581294776, -0.7660444431189769032, 0.005002170337467562802 ) ) ;
#23495=ORIENTED_EDGE ( 'NONE', *, *, #18738, .T. ) ;
#23496=CARTESIAN_POINT ( 'NONE',  ( -13.07066190154808361, 0.000000000000000000, 12.04713590736729678 ) ) ;
#23497=CARTESIAN_POINT ( 'NONE',  ( -18.86354292863559579, 0.000000000000000000, 14.21804678658176080 ) ) ;
#23498=CARTESIAN_POINT ( 'NONE',  ( -10.39993976222315020, 0.000000000000000000, 1.415483761308304889 ) ) ;
#23499=CARTESIAN_POINT ( 'NONE',  ( -18.29402319138922905, 4.333955019861509328, 11.10009953143296890 ) ) ;
#23500=DIRECTION ( 'NONE',  ( 0.007781995580012663651, 0.000000000000000000, -0.9999697198139515519 ) ) ;
#23501=LINE ( 'NONE', #49631, #33628 ) ;
#23502=DIRECTION ( 'NONE',  ( -0.7660212471507179544, -0.6427876096865405842, -0.005961354470445141482 ) ) ;
#23503=PLANE ( 'NONE',  #24190 ) ;
#23504=CARTESIAN_POINT ( 'NONE',  ( -9.648497380287073710, 7.293932373027242733, 0.5294304711899612270 ) ) ;
#23505=VERTEX_POINT ( 'NONE', #27626 ) ;
#23506=VECTOR ( 'NONE', #28146, 1000.000000000000227 ) ;
#23507=ORIENTED_EDGE ( 'NONE', *, *, #10719, .T. ) ;
#23508=ADVANCED_FACE ( 'NONE', ( #54020 ), #36409, .F. ) ;
#23509=ORIENTED_EDGE ( 'NONE', *, *, #51446, .T. ) ;
#23510=ORIENTED_EDGE ( 'NONE', *, *, #44063, .F. ) ;
#23511=ORIENTED_EDGE ( 'NONE', *, *, #33013, .T. ) ;
#23512=EDGE_CURVE ( 'NONE', #54767, #3728, #15387, .T. ) ;
#23513=ORIENTED_EDGE ( 'NONE', *, *, #51883, .T. ) ;
#23514=DIRECTION ( 'NONE',  ( -0.005002170337468016433, -0.7660444431189770143, 0.6427681459581293666 ) ) ;
#23515=EDGE_CURVE ( 'NONE', #27231, #18068, #2031, .T. ) ;
#23516=CARTESIAN_POINT ( 'NONE',  ( -19.98373089971760663, 3.038739411681507185, 9.630769916459319901 ) ) ;
#23517=ORIENTED_EDGE ( 'NONE', *, *, #14251, .F. ) ;
#23518=EDGE_LOOP ( 'NONE', ( #17088, #9229, #11640, #18149 ) ) ;
#23519=EDGE_CURVE ( 'NONE', #55275, #28007, #15138, .T. ) ;
#23520=ORIENTED_EDGE ( 'NONE', *, *, #19957, .T. ) ;
#23521=LINE ( 'NONE', #9912, #32136 ) ;
#23522=DIRECTION ( 'NONE',  ( 0.007781995580012663651, -3.146120232559066537E-19, -0.9999697198139514409 ) ) ;
#23523=FACE_OUTER_BOUND ( 'NONE', #15404, .T. ) ;
#23524=ORIENTED_EDGE ( 'NONE', *, *, #38476, .F. ) ;
#23525=FACE_OUTER_BOUND ( 'NONE', #1130, .T. ) ;
#23526=ORIENTED_EDGE ( 'NONE', *, *, #4685, .F. ) ;
#23527=DIRECTION ( 'NONE',  ( 0.5449076811759707706, 0.6444004775717708799, -0.5364919789714476250 ) ) ;
#23528=FACE_OUTER_BOUND ( 'NONE', #15821, .T. ) ;
#23529=DIRECTION ( 'NONE',  ( -0.5364919789714478471, 0.6444004775717705469, -0.5449076811759709926 ) ) ;
#23530=FACE_OUTER_BOUND ( 'NONE', #47062, .T. ) ;
#23531=CARTESIAN_POINT ( 'NONE',  ( -11.87243407472968926, 0.000000000000000000, 11.50246268866867361 ) ) ;
#23532=DIRECTION ( 'NONE',  ( 0.005002170337468016433, -0.7660444431189770143, -0.6427681459581293666 ) ) ;
#23533=CARTESIAN_POINT ( 'NONE',  ( -14.58191950326086506, -5.213152330870665097, 2.379107003115130681 ) ) ;
#23534=CARTESIAN_POINT ( 'NONE',  ( -20.12057211929586842, -0.08555834696032495190, 5.843614541628033621 ) ) ;
#23535=ORIENTED_EDGE ( 'NONE', *, *, #24442, .T. ) ;
#23536=CARTESIAN_POINT ( 'NONE',  ( -22.50936818614147583, 4.981562823951513508, 5.266396820920741462 ) ) ;
#23537=ORIENTED_EDGE ( 'NONE', *, *, #26528, .F. ) ;
#23539=ADVANCED_FACE ( 'NONE', ( #36159 ), #15651, .T. ) ;
#23540=DIRECTION ( 'NONE',  ( -0.9999697198139514409, -0.000000000000000000, -0.007781995580013368816 ) ) ;
#23541=DIRECTION ( 'NONE',  ( 0.5449076811759707706, 0.6444004775717708799, -0.5364919789714476250 ) ) ;
#23542=CARTESIAN_POINT ( 'NONE',  ( -13.27065584551087163, 0.000000000000000000, 12.04557950825129176 ) ) ;
#23543=DIRECTION ( 'NONE',  ( -0.5449076811759708816, 0.6444004775717707689, 0.5364919789714475140 ) ) ;
#23545=FACE_OUTER_BOUND ( 'NONE', #9102, .T. ) ;
#23546=EDGE_CURVE ( 'NONE', #28121, #2600, #18839, .T. ) ;
#23547=EDGE_CURVE ( 'NONE', #16295, #37024, #12254, .T. ) ;
#23548=PLANE ( 'NONE',  #51528 ) ;
#23549=FACE_OUTER_BOUND ( 'NONE', #32884, .T. ) ;
#23551=DIRECTION ( 'NONE',  ( 0.5449076811759707706, 0.6444004775717708799, -0.5364919789714476250 ) ) ;
#23552=ORIENTED_EDGE ( 'NONE', *, *, #17800, .F. ) ;
#23553=FACE_OUTER_BOUND ( 'NONE', #14496, .T. ) ;
#23554=CARTESIAN_POINT ( 'NONE',  ( -14.09271583063079980, -0.03739765774599798642, 2.294034608853361856 ) ) ;
#23555=DIRECTION ( 'NONE',  ( 0.007781995580012663651, 0.000000000000000000, -0.9999697198139515519 ) ) ;
#23556=CARTESIAN_POINT ( 'NONE',  ( -16.03749404704311843, 0.000000000000000000, 9.327590532468031270 ) ) ;
#23557=LINE ( 'NONE', #53388, #35458 ) ;
#23558=LINE ( 'NONE', #54218, #34829 ) ;
#23560=FACE_OUTER_BOUND ( 'NONE', #16835, .T. ) ;
#23561=EDGE_CURVE ( 'NONE', #15806, #23767, #51449, .T. ) ;
#23562=EDGE_LOOP ( 'NONE', ( #39316, #52229, #40183, #51652 ) ) ;
#23563=ORIENTED_EDGE ( 'NONE', *, *, #5913, .F. ) ;
#23564=CARTESIAN_POINT ( 'NONE',  ( -19.45503627000849889, 0.000000000000000000, 7.556996783084074742 ) ) ;
#23565=PLANE ( 'NONE',  #51212 ) ;
#23566=ORIENTED_EDGE ( 'NONE', *, *, #19082, .F. ) ;
#23567=CARTESIAN_POINT ( 'NONE',  ( -25.20278734466900517, 0.000000000000000000, 6.670939612111840944 ) ) ;
#23568=ORIENTED_EDGE ( 'NONE', *, *, #18864, .T. ) ;
#23569=DIRECTION ( 'NONE',  ( 0.5449076811759707706, 0.6444004775717708799, -0.5364919789714476250 ) ) ;
#23570=ORIENTED_EDGE ( 'NONE', *, *, #16603, .F. ) ;
#23571=ORIENTED_EDGE ( 'NONE', *, *, #31453, .T. ) ;
#23572=VERTEX_POINT ( 'NONE', #29863 ) ;
#23573=LINE ( 'NONE', #19867, #3931 ) ;
#23574=DIRECTION ( 'NONE',  ( -0.7660212471507179544, -0.6427876096865405842, -0.005961354470445141482 ) ) ;
#23575=PLANE ( 'NONE',  #12187 ) ;
#23576=ORIENTED_EDGE ( 'NONE', *, *, #11071, .T. ) ;
#23577=EDGE_CURVE ( 'NONE', #31801, #18836, #3717, .T. ) ;
#23578=EDGE_LOOP ( 'NONE', ( #4203, #17160, #43671, #40622 ) ) ;
#23579=DIRECTION ( 'NONE',  ( -0.2426528472758541499, 0.7422098413412800966, -0.6246952433987894571 ) ) ;
#23580=EDGE_LOOP ( 'NONE', ( #38559, #21962, #34764, #25643 ) ) ;
#23581=PLANE ( 'NONE',  #29143 ) ;
#23582=VERTEX_POINT ( 'NONE', #47160 ) ;
#23583=CARTESIAN_POINT ( 'NONE',  ( 2.072287782118878319, 0.000000000000000000, -2.950529333540147015 ) ) ;
#23584=PLANE ( 'NONE',  #14048 ) ;
#23585=ADVANCED_FACE ( 'NONE', ( #21036 ), #41768, .F. ) ;
#23587=CARTESIAN_POINT ( 'NONE',  ( -14.14577547200466690, 0.000000000000000000, 5.079653499741873190 ) ) ;
#23588=EDGE_CURVE ( 'NONE', #34236, #17943, #33828, .T. ) ;
#23589=EDGE_CURVE ( 'NONE', #55206, #46078, #38366, .T. ) ;
#23590=LINE ( 'NONE', #40908, #32709 ) ;
#23591=ORIENTED_EDGE ( 'NONE', *, *, #24294, .F. ) ;
#23592=CARTESIAN_POINT ( 'NONE',  ( 2.072287782118878319, 0.000000000000000000, -2.950529333540147015 ) ) ;
#23593=CARTESIAN_POINT ( 'NONE',  ( -15.49757964982686786, 4.333955019861511104, 10.01386589226773616 ) ) ;
#23594=PLANE ( 'NONE',  #54613 ) ;
#23595=EDGE_CURVE ( 'NONE', #40095, #3791, #37829, .T. ) ;
#23596=VERTEX_POINT ( 'NONE', #15956 ) ;
#23597=ADVANCED_FACE ( 'NONE', ( #51144 ), #17084, .F. ) ;
#23598=CARTESIAN_POINT ( 'NONE',  ( -19.45503627000849889, -1.000000000000000000, 7.556996783084074742 ) ) ;
#23599=DIRECTION ( 'NONE',  ( 0.005002170337468016433, -0.7660444431189770143, -0.6427681459581293666 ) ) ;
#23600=CARTESIAN_POINT ( 'NONE',  ( -3.033112459793370075, -5.745301166973593610, -2.040209691347345533 ) ) ;
#23601=DIRECTION ( 'NONE',  ( 0.6246952433987894571, -0.7422098413412800966, -0.2426528472758541777 ) ) ;
#23602=PLANE ( 'NONE',  #50332 ) ;
#23603=EDGE_CURVE ( 'NONE', #1256, #22414, #4014, .T. ) ;
#23604=LINE ( 'NONE', #18812, #55125 ) ;
#23605=VECTOR ( 'NONE', #26614, 1000.000000000000114 ) ;
#23607=ORIENTED_EDGE ( 'NONE', *, *, #35403, .T. ) ;
#23608=DIRECTION ( 'NONE',  ( -0.6427681459581293666, -0.7660444431189770143, -0.005002170337467561935 ) ) ;
#23609=CARTESIAN_POINT ( 'NONE',  ( -27.99923088623136636, 0.000000000000000000, 7.757173251277078130 ) ) ;
#23611=ORIENTED_EDGE ( 'NONE', *, *, #27529, .T. ) ;
#23612=CARTESIAN_POINT ( 'NONE',  ( -30.79411802867772607, 0.000000000000000000, 8.643412946479525516 ) ) ;
#23613=LINE ( 'NONE', #41506, #6434 ) ;
#23614=EDGE_CURVE ( 'NONE', #27150, #44163, #7416, .T. ) ;
#23616=CARTESIAN_POINT ( 'NONE',  ( -19.35787096931604268, 0.1245042932765045296, 4.604908354090325062 ) ) ;
#23617=DIRECTION ( 'NONE',  ( 0.000000000000000000, -1.000000000000000000, 0.000000000000000000 ) ) ;
#23618=EDGE_CURVE ( 'NONE', #36106, #28751, #24740, .T. ) ;
#23619=EDGE_LOOP ( 'NONE', ( #20351, #2977, #40068, #46214 ) ) ;
#23620=ORIENTED_EDGE ( 'NONE', *, *, #49754, .T. ) ;
#23621=PLANE ( 'NONE',  #14145 ) ;
#23622=DIRECTION ( 'NONE',  ( -0.9999697198139514409, -0.000000000000000000, -0.007781995580013368816 ) ) ;
#23624=ORIENTED_EDGE ( 'NONE', *, *, #11511, .T. ) ;
#23625=CARTESIAN_POINT ( 'NONE',  ( -16.33317936670417225, 0.000000000000000000, 13.31440848639340224 ) ) ;
#23626=ORIENTED_EDGE ( 'NONE', *, *, #41772, .F. ) ;
#23627=DIRECTION ( 'NONE',  ( 0.6427681459581294776, -0.7660444431189769032, 0.005002170337467562802 ) ) ;
#23628=ORIENTED_EDGE ( 'NONE', *, *, #2163, .F. ) ;
#23629=ORIENTED_EDGE ( 'NONE', *, *, #36781, .T. ) ;
#23630=FACE_OUTER_BOUND ( 'NONE', #32544, .T. ) ;
#23631=CARTESIAN_POINT ( 'NONE',  ( -11.34226616904245333, 0.000000000000000000, 3.085484694766132741 ) ) ;
#23632=PLANE ( 'NONE',  #37519 ) ;
#23633=ORIENTED_EDGE ( 'NONE', *, *, #2115, .T. ) ;
#23634=VECTOR ( 'NONE', #8227, 1000.000000000000227 ) ;
#23635=CARTESIAN_POINT ( 'NONE',  ( -9.487910289572674571, 0.000000000000000000, 3.638573804390909938 ) ) ;
#23636=EDGE_CURVE ( 'NONE', #8596, #54373, #42622, .T. ) ;
#23637=EDGE_LOOP ( 'NONE', ( #535, #45253, #35100, #55162 ) ) ;
#23638=VECTOR ( 'NONE', #17973, 999.9999999999998863 ) ;
#23639=ORIENTED_EDGE ( 'NONE', *, *, #48684, .F. ) ;
#23640=ORIENTED_EDGE ( 'NONE', *, *, #20832, .T. ) ;
#23641=DIRECTION ( 'NONE',  ( -0.005961354470445682716, -0.6427876096865404731, 0.7660212471507180654 ) ) ;
#23642=ORIENTED_EDGE ( 'NONE', *, *, #19119, .T. ) ;
#23643=CARTESIAN_POINT ( 'NONE',  ( -18.86354292863559579, 0.000000000000000000, 14.21804678658176080 ) ) ;
#23644=VERTEX_POINT ( 'NONE', #38669 ) ;
#23645=DIRECTION ( 'NONE',  ( -0.6427681459581293666, -0.7660444431189770143, -0.005002170337467561935 ) ) ;
#23646=DIRECTION ( 'NONE',  ( 0.005002170337468016433, -0.7660444431189770143, -0.6427681459581293666 ) ) ;
#23647=ORIENTED_EDGE ( 'NONE', *, *, #49992, .F. ) ;
#23648=DIRECTION ( 'NONE',  ( 0.9999697198139515519, 0.000000000000000000, 0.007781995580013368816 ) ) ;
#23649=EDGE_LOOP ( 'NONE', ( #34072, #54560, #55036, #30815 ) ) ;
#23650=ADVANCED_FACE ( 'NONE', ( #3163 ), #11952, .F. ) ;
#23651=LINE ( 'NONE', #31645, #40987 ) ;
#23652=CARTESIAN_POINT ( 'NONE',  ( -18.16643269429632568, 0.000000000000000000, 10.04968677925951681 ) ) ;
#23653=PLANE ( 'NONE',  #46813 ) ;
#23654=DIRECTION ( 'NONE',  ( 0.5449076811759707706, 0.6444004775717708799, -0.5364919789714476250 ) ) ;
#23655=DIRECTION ( 'NONE',  ( 0.7660212471507180654, -0.6427876096865404731, 0.005961354470445141482 ) ) ;
#23656=CARTESIAN_POINT ( 'NONE',  ( 2.072287782118878319, 0.000000000000000000, -2.950529333540147015 ) ) ;
#23657=DIRECTION ( 'NONE',  ( 0.007781995580012663651, -3.146120232559066537E-19, -0.9999697198139514409 ) ) ;
#23658=EDGE_LOOP ( 'NONE', ( #37259, #22578, #41392, #36498 ) ) ;
#23659=ORIENTED_EDGE ( 'NONE', *, *, #41777, .F. ) ;
#23660=VECTOR ( 'NONE', #54690, 999.9999999999998863 ) ;
#23661=EDGE_CURVE ( 'NONE', #36484, #1451, #33546, .T. ) ;
#23664=CARTESIAN_POINT ( 'NONE',  ( -13.87933636775488289, -3.270328918600661883, 2.168186092109577690 ) ) ;
#23665=EDGE_CURVE ( 'NONE', #7585, #25732, #16226, .T. ) ;
#23666=CARTESIAN_POINT ( 'NONE',  ( -15.33550051067056685, 0.000000000000000000, 4.531736701001109147 ) ) ;
#23667=CARTESIAN_POINT ( 'NONE',  ( -9.110551994824897193, -1.000000000000000000, 3.538847790438064411 ) ) ;
#23668=VERTEX_POINT ( 'NONE', #55398 ) ;
#23669=DIRECTION ( 'NONE',  ( 0.000000000000000000, -1.000000000000000000, 0.000000000000000000 ) ) ;
#23670=DIRECTION ( 'NONE',  ( 0.000000000000000000, -0.000000000000000000, -1.000000000000000000 ) ) ;
#23671=ORIENTED_EDGE ( 'NONE', *, *, #2270, .T. ) ;
#23672=LINE ( 'NONE', #54593, #51992 ) ;
#23673=CARTESIAN_POINT ( 'NONE',  ( 2.072287782118878319, 0.000000000000000000, -2.950529333540147015 ) ) ;
#23674=ORIENTED_EDGE ( 'NONE', *, *, #46449, .T. ) ;
#23675=ADVANCED_FACE ( 'NONE', ( #25317 ), #20190, .F. ) ;
#23677=CARTESIAN_POINT ( 'NONE',  ( 2.072287782118878319, 0.000000000000000000, -2.950529333540147015 ) ) ;
#23678=VECTOR ( 'NONE', #22970, 1000.000000000000000 ) ;
#23679=CARTESIAN_POINT ( 'NONE',  ( -16.16125387310899697, 0.000000000000000000, 9.495953418471051677 ) ) ;
#23680=DIRECTION ( 'NONE',  ( 0.005961354470445682716, -0.6427876096865404731, -0.7660212471507180654 ) ) ;
#23681=AXIS2_PLACEMENT_3D ( 'NONE', #13313, #9036, #34324 ) ;
#23682=DIRECTION ( 'NONE',  ( -0.6427681459581293666, -0.7660444431189770143, -0.005002170337467561935 ) ) ;
#23683=EDGE_CURVE ( 'NONE', #23836, #6448, #50597, .T. ) ;
#23684=ORIENTED_EDGE ( 'NONE', *, *, #48616, .F. ) ;
#23685=ORIENTED_EDGE ( 'NONE', *, *, #54325, .T. ) ;
#23686=DIRECTION ( 'NONE',  ( -0.7660212471507179544, -0.6427876096865405842, -0.005961354470445141482 ) ) ;
#23687=FACE_OUTER_BOUND ( 'NONE', #55654, .T. ) ;
#23688=DIRECTION ( 'NONE',  ( 0.5364919789714477361, 0.6444004775717706579, 0.5449076811759711036 ) ) ;
#23689=LINE ( 'NONE', #19433, #47287 ) ;
#23690=DIRECTION ( 'NONE',  ( 0.000000000000000000, 1.000000000000000000, 0.000000000000000000 ) ) ;
#23691=ORIENTED_EDGE ( 'NONE', *, *, #23216, .T. ) ;
#23692=PLANE ( 'NONE',  #6593 ) ;
#23693=DIRECTION ( 'NONE',  ( 0.6427681459581294776, -0.7660444431189769032, 0.005002170337467562802 ) ) ;
#23694=CARTESIAN_POINT ( 'NONE',  ( -23.33693525117809386, 0.000000000000000000, 5.746789908705562944 ) ) ;
#23695=ORIENTED_EDGE ( 'NONE', *, *, #5917, .T. ) ;
#23696=LINE ( 'NONE', #19444, #22013 ) ;
#23697=EDGE_LOOP ( 'NONE', ( #35520, #35566, #44804, #865 ) ) ;
#23698=CARTESIAN_POINT ( 'NONE',  ( -8.842080168916501393, 0.000000000000000000, 6.059598278784299019 ) ) ;
#23699=ADVANCED_FACE ( 'NONE', ( #34972 ), #26420, .F. ) ;
#23700=DIRECTION ( 'NONE',  ( -0.6427681459581293666, -0.7660444431189770143, -0.005002170337467561935 ) ) ;
#23701=ORIENTED_EDGE ( 'NONE', *, *, #48437, .F. ) ;
#23702=VECTOR ( 'NONE', #24956, 1000.000000000000227 ) ;
#23703=AXIS2_PLACEMENT_3D ( 'NONE', #21589, #39458, #21290 ) ;
#23704=LINE ( 'NONE', #41027, #46768 ) ;
#23705=EDGE_CURVE ( 'NONE', #43196, #32551, #51982, .T. ) ;
#23706=ORIENTED_EDGE ( 'NONE', *, *, #24347, .T. ) ;
#23707=ORIENTED_EDGE ( 'NONE', *, *, #26172, .F. ) ;
#23708=ORIENTED_EDGE ( 'NONE', *, *, #41395, .F. ) ;
#23709=LINE ( 'NONE', #1293, #26633 ) ;
#23710=EDGE_CURVE ( 'NONE', #52765, #11344, #17931, .T. ) ;
#23711=ORIENTED_EDGE ( 'NONE', *, *, #33533, .F. ) ;
#23712=ADVANCED_FACE ( 'NONE', ( #22474 ), #52287, .F. ) ;
#23713=ORIENTED_EDGE ( 'NONE', *, *, #7322, .T. ) ;
#23714=CARTESIAN_POINT ( 'NONE',  ( -18.39746900504187010, 0.000000000000000000, 14.03700784672088808 ) ) ;
#23715=EDGE_LOOP ( 'NONE', ( #26720, #52220, #21046, #18859, #34690 ) ) ;
#23717=EDGE_CURVE ( 'NONE', #43426, #36296, #39783, .T. ) ;
#23718=EDGE_CURVE ( 'NONE', #8121, #16962, #1129, .T. ) ;
#23719=EDGE_LOOP ( 'NONE', ( #10234, #20428, #38243, #49578 ) ) ;
#23720=DIRECTION ( 'NONE',  ( -0.005002170337468016433, -0.7660444431189770143, 0.6427681459581293666 ) ) ;
#23721=ORIENTED_EDGE ( 'NONE', *, *, #2032, .T. ) ;
#23723=AXIS2_PLACEMENT_3D ( 'NONE', #19040, #10247, #31825 ) ;
#23725=LINE ( 'NONE', #19469, #32010 ) ;
#23726=FACE_OUTER_BOUND ( 'NONE', #1899, .T. ) ;
#23727=PLANE ( 'NONE',  #19619 ) ;
#23728=PLANE ( 'NONE',  #6064 ) ;
#23729=VERTEX_POINT ( 'NONE', #863 ) ;
#23730=LINE ( 'NONE', #40789, #7461 ) ;
#23731=ORIENTED_EDGE ( 'NONE', *, *, #44612, .F. ) ;
#23732=ORIENTED_EDGE ( 'NONE', *, *, #26471, .T. ) ;
#23733=EDGE_CURVE ( 'NONE', #37328, #17921, #52547, .T. ) ;
#23734=CARTESIAN_POINT ( 'NONE',  ( -14.20918270945749029, -3.108426967578162170, 2.301475132743175056 ) ) ;
#23735=EDGE_CURVE ( 'NONE', #42842, #19450, #52816, .T. ) ;
#23736=LINE ( 'NONE', #36521, #11559 ) ;
#23737=DIRECTION ( 'NONE',  ( 0.5449076811759707706, 0.6444004775717708799, -0.5364919789714476250 ) ) ;
#23738=EDGE_CURVE ( 'NONE', #48144, #24901, #43738, .T. ) ;
#23739=DIRECTION ( 'NONE',  ( 0.7660212471507180654, -0.6427876096865404731, 0.005961354470445141482 ) ) ;
#23740=CARTESIAN_POINT ( 'NONE',  ( -9.759857748577539738, 0.000000000000000000, 4.575127642217221791 ) ) ;
#23741=ORIENTED_EDGE ( 'NONE', *, *, #13053, .F. ) ;
#23742=FACE_OUTER_BOUND ( 'NONE', #34767, .T. ) ;
#23743=EDGE_LOOP ( 'NONE', ( #7818, #9342, #49760, #31344 ) ) ;
#23744=VECTOR ( 'NONE', #4993, 1000.000000000000114 ) ;
#23745=EDGE_CURVE ( 'NONE', #13391, #51597, #30711, .T. ) ;
#23747=DIRECTION ( 'NONE',  ( 0.9999697198139515519, 0.000000000000000000, 0.007781995580013368816 ) ) ;
#23748=LINE ( 'NONE', #27453, #27816 ) ;
#23749=CARTESIAN_POINT ( 'NONE',  ( -13.08330893211609869, 0.000000000000000000, 1.763933231766363630 ) ) ;
#23750=LINE ( 'NONE', #36842, #45834 ) ;
#23751=DIRECTION ( 'NONE',  ( -0.3620778797217457101, 0.000000000000000000, -0.9321478471874540261 ) ) ;
#23752=AXIS2_PLACEMENT_3D ( 'NONE', #32206, #40729, #48696 ) ;
#23753=ORIENTED_EDGE ( 'NONE', *, *, #21870, .T. ) ;
#23754=DIRECTION ( 'NONE',  ( 0.000000000000000000, -1.000000000000000000, 0.000000000000000000 ) ) ;
#23755=PLANE ( 'NONE',  #9506 ) ;
#23756=FACE_OUTER_BOUND ( 'NONE', #50365, .T. ) ;
#23757=PLANE ( 'NONE',  #27348 ) ;
#23758=VECTOR ( 'NONE', #53308, 1000.000000000000227 ) ;
#23759=CARTESIAN_POINT ( 'NONE',  ( -27.99767448711536133, 0.000000000000000000, 7.557179307314289218 ) ) ;
#23760=DIRECTION ( 'NONE',  ( 0.9999697198139515519, 0.000000000000000000, 0.007781995580013368816 ) ) ;
#23761=DIRECTION ( 'NONE',  ( 0.5449076811759707706, 0.6444004775717708799, -0.5364919789714476250 ) ) ;
#23762=AXIS2_PLACEMENT_3D ( 'NONE', #14031, #5504, #19111 ) ;
#23763=CARTESIAN_POINT ( 'NONE',  ( -17.65712859575999616, 0.000000000000000000, 4.313663198198272930 ) ) ;
#23764=DIRECTION ( 'NONE',  ( 0.007781995580012662783, 0.000000000000000000, -0.9999697198139514409 ) ) ;
#23765=VERTEX_POINT ( 'NONE', #22174 ) ;
#23766=EDGE_LOOP ( 'NONE', ( #13103, #50911, #38798, #14427 ) ) ;
#23767=VERTEX_POINT ( 'NONE', #13924 ) ;
#23768=ORIENTED_EDGE ( 'NONE', *, *, #1798, .T. ) ;
#23769=VERTEX_POINT ( 'NONE', #21629 ) ;
#23770=VECTOR ( 'NONE', #23812, 1000.000000000000227 ) ;
#23771=PLANE ( 'NONE',  #39627 ) ;
#23772=CARTESIAN_POINT ( 'NONE',  ( -23.33849165029409889, 0.000000000000000000, 5.946783852668351855 ) ) ;
#23773=EDGE_CURVE ( 'NONE', #8547, #49068, #9695, .T. ) ;
#23774=EDGE_CURVE ( 'NONE', #25905, #11704, #27008, .T. ) ;
#23775=VECTOR ( 'NONE', #42429, 999.9999999999998863 ) ;
#23776=VECTOR ( 'NONE', #18430, 999.9999999999998863 ) ;
#23777=ORIENTED_EDGE ( 'NONE', *, *, #42269, .F. ) ;
#23779=ORIENTED_EDGE ( 'NONE', *, *, #24663, .T. ) ;
#23780=EDGE_CURVE ( 'NONE', #2943, #43670, #22729, .T. ) ;
#23781=ORIENTED_EDGE ( 'NONE', *, *, #4468, .F. ) ;
#23782=VECTOR ( 'NONE', #39431, 1000.000000000000227 ) ;
#23783=VECTOR ( 'NONE', #15357, 1000.000000000000227 ) ;
#23785=DIRECTION ( 'NONE',  ( 0.007781995580012663651, -3.146120232559066537E-19, -0.9999697198139514409 ) ) ;
#23786=LINE ( 'NONE', #6477, #6018 ) ;
#23788=CARTESIAN_POINT ( 'NONE',  ( -10.93224078895172013, 8.537444759202470479, 1.028080007224975168 ) ) ;
#23789=LINE ( 'NONE', #36886, #40039 ) ;
#23790=VECTOR ( 'NONE', #37086, 1000.000000000000227 ) ;
#23791=PLANE ( 'NONE',  #41161 ) ;
#23792=EDGE_CURVE ( 'NONE', #38808, #10480, #40043, .T. ) ;
#23793=FACE_OUTER_BOUND ( 'NONE', #5953, .T. ) ;
#23794=LINE ( 'NONE', #50498, #42361 ) ;
#23796=PLANE ( 'NONE',  #51025 ) ;
#23797=LINE ( 'NONE', #41128, #20334 ) ;
#23798=EDGE_CURVE ( 'NONE', #23836, #45704, #8558, .T. ) ;
#23799=DIRECTION ( 'NONE',  ( 0.7660212471507180654, -0.6427876096865404731, 0.005961354470445141482 ) ) ;
#23800=ORIENTED_EDGE ( 'NONE', *, *, #38891, .T. ) ;
#23801=DIRECTION ( 'NONE',  ( 0.007781995580012662783, 0.000000000000000000, -0.9999697198139514409 ) ) ;
#23802=ORIENTED_EDGE ( 'NONE', *, *, #46147, .F. ) ;
#23803=EDGE_CURVE ( 'NONE', #25259, #56036, #34662, .T. ) ;
#23804=DIRECTION ( 'NONE',  ( 0.5449076811759707706, 0.6444004775717708799, -0.5364919789714476250 ) ) ;
#23805=DIRECTION ( 'NONE',  ( 0.007781995580012663651, -3.146120232559066537E-19, -0.9999697198139514409 ) ) ;
#23806=DIRECTION ( 'NONE',  ( 0.007781995580012663651, -3.146120232559066537E-19, -0.9999697198139514409 ) ) ;
#23807=LINE ( 'NONE', #36322, #14159 ) ;
#23808=AXIS2_PLACEMENT_3D ( 'NONE', #34797, #38011, #4693 ) ;
#23809=DIRECTION ( 'NONE',  ( 0.6427681459581294776, -0.7660444431189769032, 0.005002170337467562802 ) ) ;
#23810=FACE_OUTER_BOUND ( 'NONE', #34081, .T. ) ;
#23811=ADVANCED_FACE ( 'NONE', ( #8861 ), #26164, .F. ) ;
#23812=DIRECTION ( 'NONE',  ( 0.007781995580012662783, 0.000000000000000000, -0.9999697198139514409 ) ) ;
#23814=LINE ( 'NONE', #53922, #3824 ) ;
#23815=VECTOR ( 'NONE', #20833, 1000.000000000000114 ) ;
#23816=LINE ( 'NONE', #45394, #38427 ) ;
#23817=CARTESIAN_POINT ( 'NONE',  ( -15.06510945078170494, 0.000000000000000000, 3.795176807137583985 ) ) ;
#23818=CARTESIAN_POINT ( 'NONE',  ( -19.06253550030438504, 0.000000000000000000, 5.780054275925301077 ) ) ;
#23820=VECTOR ( 'NONE', #6258, 999.9999999999998863 ) ;
#23821=AXIS2_PLACEMENT_3D ( 'NONE', #45896, #2153, #54147 ) ;
#23822=DIRECTION ( 'NONE',  ( 0.7660212471507180654, -0.6427876096865404731, 0.005961354470445141482 ) ) ;
#23823=CARTESIAN_POINT ( 'NONE',  ( -10.27421835998572064, 0.000000000000000000, 10.96090226820206048 ) ) ;
#23824=DIRECTION ( 'NONE',  ( -0.9999697198139514409, -0.000000000000000000, -0.007781995580013368816 ) ) ;
#23825=FACE_OUTER_BOUND ( 'NONE', #33790, .T. ) ;
#23827=VECTOR ( 'NONE', #23448, 1000.000000000000227 ) ;
#23829=VECTOR ( 'NONE', #12462, 1000.000000000000114 ) ;
#23830=ORIENTED_EDGE ( 'NONE', *, *, #18037, .T. ) ;
#23831=DIRECTION ( 'NONE',  ( 0.000000000000000000, -0.000000000000000000, -1.000000000000000000 ) ) ;
#23832=DIRECTION ( 'NONE',  ( 0.007781995580012663651, -3.146120232559066537E-19, -0.9999697198139514409 ) ) ;
#23833=VERTEX_POINT ( 'NONE', #2542 ) ;
#23834=DIRECTION ( 'NONE',  ( 0.005002170337468016433, -0.7660444431189770143, -0.6427681459581293666 ) ) ;
#23835=AXIS2_PLACEMENT_3D ( 'NONE', #4213, #16389, #8445 ) ;
#23836=VERTEX_POINT ( 'NONE', #10799 ) ;
#23838=VECTOR ( 'NONE', #43365, 1000.000000000000227 ) ;
#23839=ORIENTED_EDGE ( 'NONE', *, *, #52906, .F. ) ;
#23840=VERTEX_POINT ( 'NONE', #44871 ) ;
#23841=EDGE_LOOP ( 'NONE', ( #20441, #53445, #53613, #20502 ) ) ;
#23842=CARTESIAN_POINT ( 'NONE',  ( -9.512459116730939357, 0.000000000000000000, 6.793045374415813242 ) ) ;
#23843=CARTESIAN_POINT ( 'NONE',  ( -16.35395655750867405, -0.1191753592594181482, 3.134058533975019323 ) ) ;
#23844=PLANE ( 'NONE',  #23985 ) ;
#23845=VECTOR ( 'NONE', #12373, 999.9999999999998863 ) ;
#23846=EDGE_CURVE ( 'NONE', #24756, #28463, #5688, .T. ) ;
#23847=VERTEX_POINT ( 'NONE', #6527 ) ;
#23848=ORIENTED_EDGE ( 'NONE', *, *, #40505, .T. ) ;
#23849=VECTOR ( 'NONE', #50291, 999.9999999999998863 ) ;
#23850=EDGE_CURVE ( 'NONE', #45468, #17431, #40886, .T. ) ;
#23851=EDGE_CURVE ( 'NONE', #30589, #26710, #45167, .T. ) ;
#23852=DIRECTION ( 'NONE',  ( 0.9999697198139515519, 0.000000000000000000, 0.007781995580013368816 ) ) ;
#23853=ORIENTED_EDGE ( 'NONE', *, *, #15567, .T. ) ;
#23854=VECTOR ( 'NONE', #36348, 1000.000000000000227 ) ;
#23855=CARTESIAN_POINT ( 'NONE',  ( -16.53317331066696383, 0.000000000000000000, 13.31285208727739899 ) ) ;
#23856=EDGE_LOOP ( 'NONE', ( #15761, #47595, #2609, #5628 ) ) ;
#23857=CARTESIAN_POINT ( 'NONE',  ( -22.40478740399063895, 0.000000000000000000, 5.384712028983816623 ) ) ;
#23858=CARTESIAN_POINT ( 'NONE',  ( -15.88130887279446490, 0.000000000000000000, 3.050160814894388839 ) ) ;
#23859=VECTOR ( 'NONE', #16946, 999.9999999999998863 ) ;
#23860=AXIS2_PLACEMENT_3D ( 'NONE', #54074, #40737, #19712 ) ;
#23861=ORIENTED_EDGE ( 'NONE', *, *, #37641, .T. ) ;
#23862=CARTESIAN_POINT ( 'NONE',  ( -21.69488263569956743, 4.495856970884009485, 12.68681751722644080 ) ) ;
#23863=VECTOR ( 'NONE', #35812, 1000.000000000000227 ) ;
#23864=DIRECTION ( 'NONE',  ( 0.7660212471507180654, -0.6427876096865404731, 0.005961354470445141482 ) ) ;
#23865=VECTOR ( 'NONE', #44929, 999.9999999999998863 ) ;
#23866=ORIENTED_EDGE ( 'NONE', *, *, #26643, .T. ) ;
#23867=DIRECTION ( 'NONE',  ( 0.9999697198139515519, 0.000000000000000000, 0.007781995580013368816 ) ) ;
#23868=DIRECTION ( 'NONE',  ( 0.5449076811759707706, 0.6444004775717708799, -0.5364919789714476250 ) ) ;
#23869=FACE_OUTER_BOUND ( 'NONE', #38655, .T. ) ;
#23872=LINE ( 'NONE', #2574, #28724 ) ;
#23873=DIRECTION ( 'NONE',  ( 0.7660212471507180654, -0.6427876096865404731, 0.005961354470445141482 ) ) ;
#23874=LINE ( 'NONE', #32962, #34986 ) ;
#23875=AXIS2_PLACEMENT_3D ( 'NONE', #46396, #7821, #33625 ) ;
#23877=PLANE ( 'NONE',  #24036 ) ;
#23878=DIRECTION ( 'NONE',  ( 0.005002170337468016433, -0.7660444431189770143, -0.6427681459581293666 ) ) ;
#23880=ORIENTED_EDGE ( 'NONE', *, *, #13184, .F. ) ;
#23881=DIRECTION ( 'NONE',  ( 0.005002170337468016433, -0.7660444431189770143, -0.6427681459581293666 ) ) ;
#23882=EDGE_CURVE ( 'NONE', #48860, #44057, #35805, .T. ) ;
#23884=FACE_OUTER_BOUND ( 'NONE', #46196, .T. ) ;
#23886=EDGE_LOOP ( 'NONE', ( #32472, #23848, #4473, #8486 ) ) ;
#23887=DIRECTION ( 'NONE',  ( 0.005002170337468016433, -0.7660444431189770143, -0.6427681459581293666 ) ) ;
#23888=LINE ( 'NONE', #15119, #46283 ) ;
#23889=ADVANCED_FACE ( 'NONE', ( #31811 ), #40631, .F. ) ;
#23890=VECTOR ( 'NONE', #16132, 1000.000000000000000 ) ;
#23891=EDGE_CURVE ( 'NONE', #21762, #39023, #40333, .T. ) ;
#23892=DIRECTION ( 'NONE',  ( -0.9999697198139514409, -0.000000000000000000, -0.007781995580013368816 ) ) ;
#23893=VECTOR ( 'NONE', #1759, 1000.000000000000227 ) ;
#23894=DIRECTION ( 'NONE',  ( 0.005002170337468016433, -0.7660444431189770143, -0.6427681459581293666 ) ) ;
#23895=LINE ( 'NONE', #41756, #40152 ) ;
#23896=ORIENTED_EDGE ( 'NONE', *, *, #36940, .T. ) ;
#23897=ORIENTED_EDGE ( 'NONE', *, *, #10886, .F. ) ;
#23898=LINE ( 'NONE', #5755, #43154 ) ;
#23899=VECTOR ( 'NONE', #42989, 999.9999999999998863 ) ;
#23900=VECTOR ( 'NONE', #48689, 1000.000000000000227 ) ;
#23901=CARTESIAN_POINT ( 'NONE',  ( -10.27421835998572064, 0.000000000000000000, 10.96090226820206048 ) ) ;
#23902=VECTOR ( 'NONE', #45973, 999.9999999999998863 ) ;
#23904=CARTESIAN_POINT ( 'NONE',  ( -14.83119343108531751, -0.5179957512181563306, 3.292990205337949394 ) ) ;
#23905=EDGE_LOOP ( 'NONE', ( #54543, #24876, #31433, #5480 ) ) ;
#23906=CARTESIAN_POINT ( 'NONE',  ( -14.56888064431065821, -0.1191753592594197858, 12.58947452739191064 ) ) ;
#23907=ADVANCED_FACE ( 'NONE', ( #45413 ), #5991, .F. ) ;
#23908=VECTOR ( 'NONE', #48910, 999.9999999999998863 ) ;
#23909=ORIENTED_EDGE ( 'NONE', *, *, #8971, .F. ) ;
#23910=VECTOR ( 'NONE', #24380, 1000.000000000000000 ) ;
#23911=VERTEX_POINT ( 'NONE', #41463 ) ;
#23912=DIRECTION ( 'NONE',  ( 0.007781995580012663651, -3.146120232559066537E-19, -0.9999697198139514409 ) ) ;
#23913=EDGE_CURVE ( 'NONE', #33489, #56039, #53659, .T. ) ;
#23914=CARTESIAN_POINT ( 'NONE',  ( -10.78835031468310746, -0.1191753592594185784, 4.467120647141804568 ) ) ;
#23915=CARTESIAN_POINT ( 'NONE',  ( -15.82025578204862981, 0.000000000000000000, 7.113288712037448391 ) ) ;
#23916=VERTEX_POINT ( 'NONE', #48863 ) ;
#23917=CARTESIAN_POINT ( 'NONE',  ( -18.82375902897363318, 0.000000000000000000, 9.105901117897188257 ) ) ;
#23918=EDGE_CURVE ( 'NONE', #40865, #7098, #53128, .T. ) ;
#23919=ORIENTED_EDGE ( 'NONE', *, *, #38058, .F. ) ;
#23920=EDGE_CURVE ( 'NONE', #15287, #40042, #1963, .T. ) ;
#23921=ORIENTED_EDGE ( 'NONE', *, *, #33730, .F. ) ;
#23922=ORIENTED_EDGE ( 'NONE', *, *, #26951, .T. ) ;
#23923=CARTESIAN_POINT ( 'NONE',  ( -12.26038586170047040, -1.327505506330656893, 3.622944660148642360 ) ) ;
#23924=AXIS2_PLACEMENT_3D ( 'NONE', #33008, #52004, #48027 ) ;
#23925=ORIENTED_EDGE ( 'NONE', *, *, #55601, .F. ) ;
#23926=CARTESIAN_POINT ( 'NONE',  ( -18.86354292863559579, 0.000000000000000000, 14.21804678658176080 ) ) ;
#23927=VERTEX_POINT ( 'NONE', #32101 ) ;
#23928=AXIS2_PLACEMENT_3D ( 'NONE', #28787, #54581, #46346 ) ;
#23929=CARTESIAN_POINT ( 'NONE',  ( -8.609916609573598834, 0.000000000000000000, 10.23519010964256637 ) ) ;
#23930=CARTESIAN_POINT ( 'NONE',  ( -20.54204810873173415, 0.000000000000000000, 4.860550213503115558 ) ) ;
#23931=ORIENTED_EDGE ( 'NONE', *, *, #53591, .T. ) ;
#23932=LINE ( 'NONE', #19108, #55766 ) ;
#23933=VECTOR ( 'NONE', #15244, 999.9999999999998863 ) ;
#23934=EDGE_LOOP ( 'NONE', ( #55241, #10617, #3545, #50239 ) ) ;
#23936=DIRECTION ( 'NONE',  ( 0.007781995580012663651, -3.146120232559066537E-19, -0.9999697198139514409 ) ) ;
#23937=CARTESIAN_POINT ( 'NONE',  ( -11.87243407472968926, 0.000000000000000000, 11.50246268866867361 ) ) ;
#23938=PLANE ( 'NONE',  #30497 ) ;
#23939=CARTESIAN_POINT ( 'NONE',  ( -14.63496119600401357, 0.000000000000000000, 8.230509157998767478 ) ) ;
#23940=DIRECTION ( 'NONE',  ( 0.2426528472758542054, 0.7422098413412800966, 0.6246952433987894571 ) ) ;
#23941=VECTOR ( 'NONE', #8867, 999.9999999999998863 ) ;
#23942=DIRECTION ( 'NONE',  ( 0.007781995580012662783, 0.000000000000000000, -0.9999697198139514409 ) ) ;
#23943=ORIENTED_EDGE ( 'NONE', *, *, #548, .T. ) ;
#23944=VECTOR ( 'NONE', #31520, 1000.000000000000227 ) ;
#23945=EDGE_LOOP ( 'NONE', ( #31952, #20193, #52375, #41026 ) ) ;
#23947=PLANE ( 'NONE',  #21214 ) ;
#23948=DIRECTION ( 'NONE',  ( 0.007781995580012663651, -3.146120232559066537E-19, -0.9999697198139514409 ) ) ;
#23949=LINE ( 'NONE', #15697, #51444 ) ;
#23950=AXIS2_PLACEMENT_3D ( 'NONE', #8710, #26032, #35369 ) ;
#23951=AXIS2_PLACEMENT_3D ( 'NONE', #55253, #21480, #30267 ) ;
#23952=LINE ( 'NONE', #37029, #42182 ) ;
#23954=LINE ( 'NONE', #2377, #13187 ) ;
#23955=CARTESIAN_POINT ( 'NONE',  ( -17.63356496434233378, 4.172053068839010059, 3.398296866036514263 ) ) ;
#23956=VERTEX_POINT ( 'NONE', #15064 ) ;
#23957=CARTESIAN_POINT ( 'NONE',  ( -13.07066190154808361, 0.000000000000000000, 12.04713590736729678 ) ) ;
#23958=DIRECTION ( 'NONE',  ( -0.5449076811759708816, 0.6444004775717707689, 0.5364919789714475140 ) ) ;
#23959=ORIENTED_EDGE ( 'NONE', *, *, #50814, .F. ) ;
#23961=CARTESIAN_POINT ( 'NONE',  ( -11.84011462117533320, 0.6102101463440047224, 1.261565443871230263 ) ) ;
#23962=ADVANCED_FACE ( 'NONE', ( #19599 ), #45693, .F. ) ;
#23963=DIRECTION ( 'NONE',  ( -0.7660212471507179544, -0.6427876096865405842, -0.005961354470445141482 ) ) ;
#23964=FACE_OUTER_BOUND ( 'NONE', #36807, .T. ) ;
#23965=CARTESIAN_POINT ( 'NONE',  ( -9.908141408373387193, -0.1191753592594197858, 10.77908512878318703 ) ) ;
#23966=VECTOR ( 'NONE', #54249, 999.9999999999998863 ) ;
#23967=EDGE_LOOP ( 'NONE', ( #41789, #24411, #46678, #14948 ) ) ;
#23968=ORIENTED_EDGE ( 'NONE', *, *, #22579, .F. ) ;
#23969=CARTESIAN_POINT ( 'NONE',  ( -19.60834386242827776, 0.000000000000000000, 4.298478389818581213 ) ) ;
#23970=FACE_OUTER_BOUND ( 'NONE', #18626, .T. ) ;
#23971=CARTESIAN_POINT ( 'NONE',  ( -11.89750579909570227, 0.1245042932765041271, 1.299354686050277818 ) ) ;
#23972=VECTOR ( 'NONE', #38475, 999.9999999999998863 ) ;
#23973=EDGE_CURVE ( 'NONE', #29009, #42993, #31555, .T. ) ;
#23974=CARTESIAN_POINT ( 'NONE',  ( -22.24825055231656634, 5.143464774974011888, 13.96459914429588167 ) ) ;
#23975=CARTESIAN_POINT ( 'NONE',  ( -17.50764612648356433, -1.489407457353158160, 3.634365539079154050 ) ) ;
#23976=CARTESIAN_POINT ( 'NONE',  ( -20.54049170961573267, 0.000000000000000000, 4.660556269540326646 ) ) ;
#23977=ORIENTED_EDGE ( 'NONE', *, *, #21018, .F. ) ;
#23978=ADVANCED_FACE ( 'NONE', ( #6815 ), #20714, .F. ) ;
#23979=DIRECTION ( 'NONE',  ( 0.6427681459581294776, -0.7660444431189769032, 0.005002170337467562802 ) ) ;
#23980=EDGE_CURVE ( 'NONE', #32939, #18253, #46838, .T. ) ;
#23981=PLANE ( 'NONE',  #3305 ) ;
#23982=DIRECTION ( 'NONE',  ( -0.005002170337468016433, -0.7660444431189770143, 0.6427681459581293666 ) ) ;
#23983=VECTOR ( 'NONE', #18027, 999.9999999999998863 ) ;
#23984=EDGE_LOOP ( 'NONE', ( #24579, #44284, #55122, #30087 ) ) ;
#23985=AXIS2_PLACEMENT_3D ( 'NONE', #28115, #6000, #24148 ) ;
#23987=EDGE_CURVE ( 'NONE', #1435, #33297, #11636, .T. ) ;
#23988=CARTESIAN_POINT ( 'NONE',  ( -24.27063949748155380, 0.000000000000000000, 6.308861732390097288 ) ) ;
#23989=FACE_OUTER_BOUND ( 'NONE', #30281, .T. ) ;
#23990=VECTOR ( 'NONE', #50197, 1000.000000000000114 ) ;
#23991=ORIENTED_EDGE ( 'NONE', *, *, #31040, .T. ) ;
#23992=CARTESIAN_POINT ( 'NONE',  ( -14.00280974873554030, 0.000000000000000000, 12.40921378708904044 ) ) ;
#23993=EDGE_CURVE ( 'NONE', #6150, #52665, #46245, .T. ) ;
#23994=ORIENTED_EDGE ( 'NONE', *, *, #6360, .T. ) ;
#23995=EDGE_CURVE ( 'NONE', #54772, #9210, #42564, .T. ) ;
#23996=VECTOR ( 'NONE', #32453, 1000.000000000000227 ) ;
#23997=ORIENTED_EDGE ( 'NONE', *, *, #25858, .F. ) ;
#23998=VERTEX_POINT ( 'NONE', #7946 ) ;
#23999=VECTOR ( 'NONE', #11880, 1000.000000000000114 ) ;
#24000=ORIENTED_EDGE ( 'NONE', *, *, #51959, .F. ) ;
#24001=ORIENTED_EDGE ( 'NONE', *, *, #40054, .F. ) ;
#24002=DIRECTION ( 'NONE',  ( -0.005002170337468016433, -0.7660444431189770143, 0.6427681459581293666 ) ) ;
#24003=EDGE_LOOP ( 'NONE', ( #44897, #52313, #30479, #40771 ) ) ;
#24004=ADVANCED_FACE ( 'NONE', ( #3655 ), #28679, .F. ) ;
#24005=ORIENTED_EDGE ( 'NONE', *, *, #46510, .F. ) ;
#24006=LINE ( 'NONE', #14935, #32214 ) ;
#24007=ORIENTED_EDGE ( 'NONE', *, *, #1870, .F. ) ;
#24008=EDGE_LOOP ( 'NONE', ( #50670, #12642, #29378, #17390 ) ) ;
#24009=ORIENTED_EDGE ( 'NONE', *, *, #24577, .F. ) ;
#24010=VECTOR ( 'NONE', #2234, 1000.000000000000227 ) ;
#24011=ADVANCED_FACE ( 'NONE', ( #12180 ), #29213, .F. ) ;
#24012=CARTESIAN_POINT ( 'NONE',  ( -23.33693525117809386, 0.000000000000000000, 5.746789908705562944 ) ) ;
#24013=VECTOR ( 'NONE', #41187, 1000.000000000000227 ) ;
#24014=CARTESIAN_POINT ( 'NONE',  ( -15.88053067323646417, -0.1191753592594197858, 2.950163842912994383 ) ) ;
#24015=DIRECTION ( 'NONE',  ( 0.6427681459581294776, -0.7660444431189769032, 0.005002170337467562802 ) ) ;
#24016=LINE ( 'NONE', #10705, #8737 ) ;
#24017=EDGE_LOOP ( 'NONE', ( #2134, #22807, #47002, #11646 ) ) ;
#24018=CARTESIAN_POINT ( 'NONE',  ( -14.93495759592298988, 0.000000000000000000, 12.77129166681078409 ) ) ;
#24019=AXIS2_PLACEMENT_3D ( 'NONE', #20158, #45448, #46278 ) ;
#24020=EDGE_LOOP ( 'NONE', ( #3334, #15396, #30969, #4681, #27166 ) ) ;
#24021=ORIENTED_EDGE ( 'NONE', *, *, #28542, .F. ) ;
#24022=CARTESIAN_POINT ( 'NONE',  ( -1.086233639165236964, 0.000000000000000000, -2.796443541562362078 ) ) ;
#24023=DIRECTION ( 'NONE',  ( -0.5364919789714478471, 0.6444004775717705469, -0.5449076811759709926 ) ) ;
#24025=DIRECTION ( 'NONE',  ( 0.000000000000000000, -1.000000000000000000, 0.000000000000000000 ) ) ;
#24026=VECTOR ( 'NONE', #6096, 999.9999999999998863 ) ;
#24027=AXIS2_PLACEMENT_3D ( 'NONE', #13969, #35290, #47493 ) ;
#24028=LINE ( 'NONE', #36525, #35936 ) ;
#24029=VECTOR ( 'NONE', #53386, 1000.000000000000227 ) ;
#24030=CARTESIAN_POINT ( 'NONE',  ( -30.79567442779373110, 0.000000000000000000, 8.843406890442315316 ) ) ;
#24031=AXIS2_PLACEMENT_3D ( 'NONE', #41788, #33310, #50613 ) ;
#24032=FACE_OUTER_BOUND ( 'NONE', #29042, .T. ) ;
#24033=VERTEX_POINT ( 'NONE', #42296 ) ;
#24034=CARTESIAN_POINT ( 'NONE',  ( -13.53673582514181106, 0.000000000000000000, 12.22817484722816772 ) ) ;
#24035=VERTEX_POINT ( 'NONE', #41991 ) ;
#24036=AXIS2_PLACEMENT_3D ( 'NONE', #50830, #19338, #33266 ) ;
#24037=CARTESIAN_POINT ( 'NONE',  ( -24.27063949748155380, 0.000000000000000000, 6.308861732390097288 ) ) ;
#24038=DIRECTION ( 'NONE',  ( 0.007781995580012663651, 0.000000000000000000, -0.9999697198139515519 ) ) ;
#24039=DIRECTION ( 'NONE',  ( -0.7660212471507179544, -0.6427876096865405842, -0.005961354470445141482 ) ) ;
#24040=EDGE_CURVE ( 'NONE', #37024, #13654, #32919, .T. ) ;
#24041=CARTESIAN_POINT ( 'NONE',  ( -9.482162182562110075, 0.000000000000000000, 2.899954397875381673 ) ) ;
#24042=LINE ( 'NONE', #5600, #40479 ) ;
#24043=VECTOR ( 'NONE', #149, 999.9999999999998863 ) ;
#24044=VECTOR ( 'NONE', #21991, 999.9999999999998863 ) ;
#24045=ORIENTED_EDGE ( 'NONE', *, *, #49822, .T. ) ;
#24046=CARTESIAN_POINT ( 'NONE',  ( -28.93060053386082231, -0.1191753592594197858, 8.019254159017428663 ) ) ;
#24047=CARTESIAN_POINT ( 'NONE',  ( -16.37867951088334451, 4.819660872929009798, 11.15324105243068686 ) ) ;
#24048=CARTESIAN_POINT ( 'NONE',  ( -20.26041485802610609, 3.362543313726507499, 10.26966072999404034 ) ) ;
#24049=EDGE_CURVE ( 'NONE', #1446, #9065, #46526, .T. ) ;
#24050=EDGE_CURVE ( 'NONE', #17921, #35066, #20969, .T. ) ;
#24051=EDGE_CURVE ( 'NONE', #7585, #48014, #7647, .T. ) ;
#24052=CARTESIAN_POINT ( 'NONE',  ( -9.908141408373387193, -0.1191753592594197858, 10.77908512878318703 ) ) ;
#24053=DIRECTION ( 'NONE',  ( 0.000000000000000000, -0.000000000000000000, -1.000000000000000000 ) ) ;
#24054=CARTESIAN_POINT ( 'NONE',  ( -14.46888367232926420, 0.000000000000000000, 12.59025272694991315 ) ) ;
#24055=DIRECTION ( 'NONE',  ( 0.007781995580012663651, -3.146120232559066537E-19, -0.9999697198139514409 ) ) ;
#24056=EDGE_CURVE ( 'NONE', #52707, #33003, #43605, .T. ) ;
#24057=AXIS2_PLACEMENT_3D ( 'NONE', #39647, #26280, #56112 ) ;
#24059=CARTESIAN_POINT ( 'NONE',  ( -19.60834386242827776, 0.000000000000000000, 4.298478389818581213 ) ) ;
#24060=VECTOR ( 'NONE', #26980, 1000.000000000000227 ) ;
#24061=ORIENTED_EDGE ( 'NONE', *, *, #34840, .T. ) ;
#24062=EDGE_CURVE ( 'NONE', #35444, #34483, #55335, .T. ) ;
#24063=VECTOR ( 'NONE', #18666, 1000.000000000000114 ) ;
#24064=ADVANCED_FACE ( 'NONE', ( #52137 ), #16431, .F. ) ;
#24065=ORIENTED_EDGE ( 'NONE', *, *, #32752, .F. ) ;
#24066=ORIENTED_EDGE ( 'NONE', *, *, #24563, .F. ) ;
#24067=AXIS2_PLACEMENT_3D ( 'NONE', #18797, #14797, #53155 ) ;
#24068=VECTOR ( 'NONE', #42878, 999.9999999999998863 ) ;
#24069=EDGE_LOOP ( 'NONE', ( #50735, #41886, #54804, #25765 ) ) ;
#24070=EDGE_CURVE ( 'NONE', #23847, #33893, #29522, .T. ) ;
#24071=VERTEX_POINT ( 'NONE', #25261 ) ;
#24072=DIRECTION ( 'NONE',  ( -0.005002170337468016433, -0.7660444431189770143, 0.6427681459581293666 ) ) ;
#24073=CARTESIAN_POINT ( 'NONE',  ( -18.67697421479882181, -0.1191753592594197858, 4.036397482078229793 ) ) ;
#24074=VECTOR ( 'NONE', #32001, 999.9999999999998863 ) ;
#24075=ADVANCED_FACE ( 'NONE', ( #38295 ), #37181, .F. ) ;
#24076=VECTOR ( 'NONE', #45119, 999.9999999999998863 ) ;
#24077=ORIENTED_EDGE ( 'NONE', *, *, #15911, .T. ) ;
#24078=DIRECTION ( 'NONE',  ( -0.005002170337468016433, -0.7660444431189770143, 0.6427681459581293666 ) ) ;
#24080=ORIENTED_EDGE ( 'NONE', *, *, #21623, .F. ) ;
#24081=VECTOR ( 'NONE', #4645, 999.9999999999998863 ) ;
#24082=AXIS2_PLACEMENT_3D ( 'NONE', #24441, #42037, #55120 ) ;
#24084=CARTESIAN_POINT ( 'NONE',  ( -16.43317633868556626, -0.1191753592594197858, 13.31363028683540151 ) ) ;
#24085=DIRECTION ( 'NONE',  ( 0.7660212471507180654, -0.6427876096865404731, 0.005961354470445141482 ) ) ;
#24086=ORIENTED_EDGE ( 'NONE', *, *, #28948, .T. ) ;
#24088=LINE ( 'NONE', #41120, #92 ) ;
#24089=LINE ( 'NONE', #38250, #27545 ) ;
#24090=VECTOR ( 'NONE', #52542, 1000.000000000000114 ) ;
#24091=DIRECTION ( 'NONE',  ( -0.005002170337468016433, -0.7660444431189770143, 0.6427681459581293666 ) ) ;
#24092=PLANE ( 'NONE',  #5164 ) ;
#24093=CARTESIAN_POINT ( 'NONE',  ( -19.60834386242827776, 0.000000000000000000, 4.298478389818581213 ) ) ;
#24094=CARTESIAN_POINT ( 'NONE',  ( 2.072287782118878319, 0.000000000000000000, -2.950529333540147015 ) ) ;
#24095=LINE ( 'NONE', #2215, #17629 ) ;
#24096=VECTOR ( 'NONE', #53227, 999.9999999999998863 ) ;
#24097=CARTESIAN_POINT ( 'NONE',  ( -14.39084381659288070, 3.038739411681508518, 7.458302638128849971 ) ) ;
#24098=EDGE_LOOP ( 'NONE', ( #3501, #1659, #23909, #11602 ) ) ;
#24099=PLANE ( 'NONE',  #51909 ) ;
#24100=ORIENTED_EDGE ( 'NONE', *, *, #33107, .F. ) ;
#24101=VECTOR ( 'NONE', #13825, 1000.000000000000114 ) ;
#24102=EDGE_CURVE ( 'NONE', #17210, #17624, #15885, .T. ) ;
#24103=LINE ( 'NONE', #6782, #34694 ) ;
#24104=CARTESIAN_POINT ( 'NONE',  ( -13.38620395562085719, 0.7721120973665037690, 3.348144823107547463 ) ) ;
#24105=DIRECTION ( 'NONE',  ( 0.007781995580012663651, 0.000000000000000000, -0.9999697198139515519 ) ) ;
#24106=AXIS2_PLACEMENT_3D ( 'NONE', #22144, #31528, #52524 ) ;
#24107=EDGE_CURVE ( 'NONE', #45238, #17332, #18625, .T. ) ;
#24108=PLANE ( 'NONE',  #9647 ) ;
#24109=LINE ( 'NONE', #15852, #23202 ) ;
#24110=VECTOR ( 'NONE', #2224, 1000.000000000000227 ) ;
#24111=DIRECTION ( 'NONE',  ( 0.000000000000000000, -1.000000000000000000, 0.000000000000000000 ) ) ;
#24113=PLANE ( 'NONE',  #12010 ) ;
#24114=CARTESIAN_POINT ( 'NONE',  ( 2.072287782118878319, 0.000000000000000000, -2.950529333540147015 ) ) ;
#24115=FACE_OUTER_BOUND ( 'NONE', #18772, .T. ) ;
#24116=VECTOR ( 'NONE', #17831, 1000.000000000000114 ) ;
#24117=FACE_OUTER_BOUND ( 'NONE', #20010, .T. ) ;
#24118=ADVANCED_FACE ( 'NONE', ( #9550 ), #10094, .F. ) ;
#24119=DIRECTION ( 'NONE',  ( 0.7660212471507180654, -0.6427876096865404731, 0.005961354470445141482 ) ) ;
#24121=EDGE_CURVE ( 'NONE', #44182, #40596, #53286, .T. ) ;
#24122=ADVANCED_FACE ( 'NONE', ( #1282 ), #44194, .F. ) ;
#24123=VECTOR ( 'NONE', #1309, 1000.000000000000227 ) ;
#24124=CARTESIAN_POINT ( 'NONE',  ( -31.72782227498118601, 0.000000000000000000, 9.205484770164058972 ) ) ;
#24125=CARTESIAN_POINT ( 'NONE',  ( -20.42408051421004345, -0.5179957512181551094, 5.465457483668419769 ) ) ;
#24126=ADVANCED_FACE ( 'NONE', ( #4715 ), #31956, .F. ) ;
#24127=DIRECTION ( 'NONE',  ( -0.005002170337468016433, -0.7660444431189770143, 0.6427681459581293666 ) ) ;
#24128=DIRECTION ( 'NONE',  ( -0.5364919789714478471, 0.6444004775717705469, -0.5449076811759709926 ) ) ;
#24129=EDGE_LOOP ( 'NONE', ( #6692, #17244, #49031, #6531 ) ) ;
#24130=VECTOR ( 'NONE', #41774, 1000.000000000000227 ) ;
#24131=AXIS2_PLACEMENT_3D ( 'NONE', #13835, #196, #39705 ) ;
#24132=CARTESIAN_POINT ( 'NONE',  ( -13.73672976910459909, 0.000000000000000000, 12.22661844811216270 ) ) ;
#24133=EDGE_LOOP ( 'NONE', ( #34283, #39868, #40266, #8495 ) ) ;
#24134=CARTESIAN_POINT ( 'NONE',  ( -24.27063949748155380, 0.000000000000000000, 6.308861732390097288 ) ) ;
#24135=EDGE_LOOP ( 'NONE', ( #27217, #55434, #20065, #6588 ) ) ;
#24136=ORIENTED_EDGE ( 'NONE', *, *, #37633, .T. ) ;
#24137=CARTESIAN_POINT ( 'NONE',  ( -17.74404816805336793, 0.000000000000000000, 3.574322630375089460 ) ) ;
#24138=EDGE_CURVE ( 'NONE', #37968, #50912, #1587, .T. ) ;
#24139=VECTOR ( 'NONE', #24275, 1000.000000000000227 ) ;
#24140=EDGE_CURVE ( 'NONE', #16305, #21974, #31111, .T. ) ;
#24141=ORIENTED_EDGE ( 'NONE', *, *, #2184, .T. ) ;
#24142=ORIENTED_EDGE ( 'NONE', *, *, #5168, .T. ) ;
#24143=ORIENTED_EDGE ( 'NONE', *, *, #46873, .T. ) ;
#24144=EDGE_CURVE ( 'NONE', #42632, #50731, #44730, .T. ) ;
#24145=DIRECTION ( 'NONE',  ( -0.7660212471507179544, -0.6427876096865405842, -0.005961354470445141482 ) ) ;
#24146=CARTESIAN_POINT ( 'NONE',  ( -15.60102546347950536, 0.000000000000000000, 12.95077420755565356 ) ) ;
#24148=DIRECTION ( 'NONE',  ( -0.6427681459581293666, -0.7660444431189770143, -0.005002170337467561935 ) ) ;
#24149=EDGE_CURVE ( 'NONE', #45990, #30666, #26870, .T. ) ;
#24150=VECTOR ( 'NONE', #6737, 999.9999999999998863 ) ;
#24151=ORIENTED_EDGE ( 'NONE', *, *, #48020, .T. ) ;
#24152=EDGE_LOOP ( 'NONE', ( #7747, #7949, #39776, #41543 ) ) ;
#24153=EDGE_CURVE ( 'NONE', #53959, #2345, #18322, .T. ) ;
#24154=VECTOR ( 'NONE', #29782, 999.9999999999998863 ) ;
#24156=DIRECTION ( 'NONE',  ( -0.5364919789714478471, 0.6444004775717705469, -0.5449076811759709926 ) ) ;
#24157=ORIENTED_EDGE ( 'NONE', *, *, #20893, .T. ) ;
#24158=DIRECTION ( 'NONE',  ( 0.007781995580012663651, -3.146120232559066537E-19, -0.9999697198139514409 ) ) ;
#24160=LINE ( 'NONE', #31827, #34844 ) ;
#24161=DIRECTION ( 'NONE',  ( -0.9999697198139514409, -0.000000000000000000, -0.007781995580013368816 ) ) ;
#24162=VECTOR ( 'NONE', #37434, 999.9999999999998863 ) ;
#24163=EDGE_LOOP ( 'NONE', ( #42464, #18895, #44196, #38085 ) ) ;
#24164=AXIS2_PLACEMENT_3D ( 'NONE', #45581, #11230, #28552 ) ;
#24165=DIRECTION ( 'NONE',  ( 0.005961354470445682716, -0.6427876096865404731, -0.7660212471507180654 ) ) ;
#24167=FACE_OUTER_BOUND ( 'NONE', #38096, .T. ) ;
#24169=ORIENTED_EDGE ( 'NONE', *, *, #30548, .T. ) ;
#24170=CARTESIAN_POINT ( 'NONE',  ( -14.02643832504429611, -0.1191753592594190225, 2.595260748476915236 ) ) ;
#24171=CARTESIAN_POINT ( 'NONE',  ( -20.09634856977056927, -0.6798977022406551551, 5.603863950574907271 ) ) ;
#24172=PLANE ( 'NONE',  #42831 ) ;
#24173=ORIENTED_EDGE ( 'NONE', *, *, #50493, .F. ) ;
#24174=CARTESIAN_POINT ( 'NONE',  ( -16.89925026227929195, -0.1191753592594197858, 13.49466922669627422 ) ) ;
#24175=CARTESIAN_POINT ( 'NONE',  ( -10.00813838035478298, 0.000000000000000000, 10.77830692922518452 ) ) ;
#24176=DIRECTION ( 'NONE',  ( -0.6427681459581293666, -0.7660444431189770143, -0.005002170337467561935 ) ) ;
#24177=CARTESIAN_POINT ( 'NONE',  ( -13.27065584551087163, 0.000000000000000000, 12.04557950825129176 ) ) ;
#24178=DIRECTION ( 'NONE',  ( -0.005961354470445682716, -0.6427876096865404731, 0.7660212471507180654 ) ) ;
#24179=DIRECTION ( 'NONE',  ( 0.005002170337468016433, -0.7660444431189770143, -0.6427681459581293666 ) ) ;
#24180=VECTOR ( 'NONE', #12027, 1000.000000000000227 ) ;
#24181=DIRECTION ( 'NONE',  ( -0.6246952433987893460, -0.7422098413412802076, 0.2426528472758542054 ) ) ;
#24182=ORIENTED_EDGE ( 'NONE', *, *, #45793, .F. ) ;
#24183=FACE_OUTER_BOUND ( 'NONE', #30981, .T. ) ;
#24184=CARTESIAN_POINT ( 'NONE',  ( -9.542064456761055524, 0.000000000000000000, 10.59726798936431180 ) ) ;
#24186=ORIENTED_EDGE ( 'NONE', *, *, #51522, .T. ) ;
#24187=DIRECTION ( 'NONE',  ( -0.005002170337468016433, -0.7660444431189770143, 0.6427681459581293666 ) ) ;
#24188=DIRECTION ( 'NONE',  ( 0.000000000000000000, -0.000000000000000000, -1.000000000000000000 ) ) ;
#24189=ADVANCED_FACE ( 'NONE', ( #9838 ), #27141, .F. ) ;
#24190=AXIS2_PLACEMENT_3D ( 'NONE', #19219, #1348, #49053 ) ;
#24191=CARTESIAN_POINT ( 'NONE',  ( -3.033112459793370075, -5.745301166973593610, -2.040209691347345533 ) ) ;
#24192=EDGE_CURVE ( 'NONE', #19093, #12718, #454, .T. ) ;
#24193=ADVANCED_FACE ( 'NONE', ( #27408 ), #52429, .F. ) ;
#24194=LINE ( 'NONE', #19909, #3331 ) ;
#24196=ORIENTED_EDGE ( 'NONE', *, *, #12178, .T. ) ;
#24197=VECTOR ( 'NONE', #54744, 1000.000000000000227 ) ;
#24198=VERTEX_POINT ( 'NONE', #48140 ) ;
#24199=DIRECTION ( 'NONE',  ( -0.7660212471507179544, -0.6427876096865405842, -0.005961354470445141482 ) ) ;
#24200=DIRECTION ( 'NONE',  ( 0.9999697198139515519, 0.000000000000000000, 0.007781995580013368816 ) ) ;
#24201=VECTOR ( 'NONE', #44767, 1000.000000000000114 ) ;
#24202=ORIENTED_EDGE ( 'NONE', *, *, #42453, .F. ) ;
#24203=LINE ( 'NONE', #2326, #23996 ) ;
#24204=ORIENTED_EDGE ( 'NONE', *, *, #14393, .F. ) ;
#24205=PLANE ( 'NONE',  #31979 ) ;
#24206=AXIS2_PLACEMENT_3D ( 'NONE', #55385, #20176, #54531 ) ;
#24207=VERTEX_POINT ( 'NONE', #35973 ) ;
#24208=ORIENTED_EDGE ( 'NONE', *, *, #10082, .T. ) ;
#24209=DIRECTION ( 'NONE',  ( 0.7660212471507180654, -0.6427876096865404731, 0.005961354470445141482 ) ) ;
#24211=DIRECTION ( 'NONE',  ( 0.9999697198139515519, 0.000000000000000000, 0.007781995580013368816 ) ) ;
#24212=ORIENTED_EDGE ( 'NONE', *, *, #42402, .F. ) ;
#24213=CARTESIAN_POINT ( 'NONE',  ( -22.69879496416571740, -4.889348428825663895, 5.542308122156290651 ) ) ;
#24214=ORIENTED_EDGE ( 'NONE', *, *, #25153, .T. ) ;
#24215=ADVANCED_FACE ( 'NONE', ( #5847 ), #9249, .F. ) ;
#24216=VECTOR ( 'NONE', #22745, 1000.000000000000000 ) ;
#24217=ORIENTED_EDGE ( 'NONE', *, *, #35450, .T. ) ;
#24218=ORIENTED_EDGE ( 'NONE', *, *, #55919, .T. ) ;
#24219=DIRECTION ( 'NONE',  ( 0.9999697198139515519, 0.000000000000000000, 0.007781995580013368816 ) ) ;
#24220=EDGE_CURVE ( 'NONE', #29163, #21607, #31691, .T. ) ;
#24221=ORIENTED_EDGE ( 'NONE', *, *, #1772, .T. ) ;
#24222=PLANE ( 'NONE',  #6710 ) ;
#24223=EDGE_CURVE ( 'NONE', #6114, #51035, #39662, .T. ) ;
#24224=ORIENTED_EDGE ( 'NONE', *, *, #45554, .F. ) ;
#24225=CARTESIAN_POINT ( 'NONE',  ( -12.45405610843340050, 0.7721120973665051013, 2.986066943385802475 ) ) ;
#24226=DIRECTION ( 'NONE',  ( 0.007781995580012663651, 0.000000000000000000, -0.9999697198139515519 ) ) ;
#24227=VERTEX_POINT ( 'NONE', #35380 ) ;
#24228=VECTOR ( 'NONE', #43292, 1000.000000000000227 ) ;
#24229=EDGE_CURVE ( 'NONE', #33221, #22744, #54629, .T. ) ;
#24232=VECTOR ( 'NONE', #29658, 999.9999999999998863 ) ;
#24233=DIRECTION ( 'NONE',  ( 0.000000000000000000, -1.000000000000000000, 0.000000000000000000 ) ) ;
#24234=PLANE ( 'NONE',  #43828 ) ;
#24235=CARTESIAN_POINT ( 'NONE',  ( -13.03530845450740117, 0.000000000000000000, 7.504293885903270400 ) ) ;
#24236=DIRECTION ( 'NONE',  ( 0.6427681459581294776, -0.7660444431189769032, 0.005002170337467562802 ) ) ;
#24237=FACE_OUTER_BOUND ( 'NONE', #54038, .T. ) ;
#24238=DIRECTION ( 'NONE',  ( 0.005961354470445682716, -0.6427876096865404731, -0.7660212471507180654 ) ) ;
#24240=ORIENTED_EDGE ( 'NONE', *, *, #9361, .F. ) ;
#24241=ORIENTED_EDGE ( 'NONE', *, *, #29640, .T. ) ;
#24242=AXIS2_PLACEMENT_3D ( 'NONE', #34782, #13212, #21462 ) ;
#24243=LINE ( 'NONE', #45804, #32790 ) ;
#24244=LINE ( 'NONE', #42100, #16721 ) ;
#24245=DIRECTION ( 'NONE',  ( 0.9999697198139515519, 0.000000000000000000, 0.007781995580013368816 ) ) ;
#24246=LINE ( 'NONE', #32741, #22433 ) ;
#24247=CARTESIAN_POINT ( 'NONE',  ( -17.39823374989226679, 0.000000000000000000, 5.054342117365806075 ) ) ;
#24248=ORIENTED_EDGE ( 'NONE', *, *, #32043, .F. ) ;
#24249=CARTESIAN_POINT ( 'NONE',  ( 2.072287782118878319, 0.000000000000000000, -2.950529333540147015 ) ) ;
#24250=LINE ( 'NONE', #23955, #37729 ) ;
#24251=ORIENTED_EDGE ( 'NONE', *, *, #18719, .F. ) ;
#24252=DIRECTION ( 'NONE',  ( 0.5364919789714477361, 0.6444004775717706579, 0.5449076811759711036 ) ) ;
#24253=EDGE_CURVE ( 'NONE', #10694, #31194, #32526, .T. ) ;
#24254=LINE ( 'NONE', #24794, #3172 ) ;
#24255=ORIENTED_EDGE ( 'NONE', *, *, #18563, .F. ) ;
#24256=ADVANCED_FACE ( 'NONE', ( #45036 ), #28242, .F. ) ;
#24257=DIRECTION ( 'NONE',  ( 0.7660212471507180654, -0.6427876096865404731, 0.005961354470445141482 ) ) ;
#24258=CARTESIAN_POINT ( 'NONE',  ( -16.13159951105223655, 1.257817950434005461, 5.211675742713992143 ) ) ;
#24259=PLANE ( 'NONE',  #12332 ) ;
#24260=ADVANCED_FACE ( 'NONE', ( #11202 ), #28826, .F. ) ;
#24261=EDGE_CURVE ( 'NONE', #16128, #49537, #50395, .T. ) ;
#24262=PLANE ( 'NONE',  #31441 ) ;
#24264=ORIENTED_EDGE ( 'NONE', *, *, #25158, .T. ) ;
#24265=ORIENTED_EDGE ( 'NONE', *, *, #12019, .F. ) ;
#24266=DIRECTION ( 'NONE',  ( 0.007781995580012662783, 0.000000000000000000, -0.9999697198139514409 ) ) ;
#24267=DIRECTION ( 'NONE',  ( 0.9999697198139515519, 0.000000000000000000, 0.007781995580013368816 ) ) ;
#24269=PLANE ( 'NONE',  #3374 ) ;
#24270=DIRECTION ( 'NONE',  ( 0.9999697198139515519, 0.000000000000000000, 0.007781995580013368816 ) ) ;
#24271=LINE ( 'NONE', #40487, #4997 ) ;
#24272=EDGE_LOOP ( 'NONE', ( #41911, #21497, #51123, #46560 ) ) ;
#24273=CARTESIAN_POINT ( 'NONE',  ( -11.26160937204003609, -0.1191753592594181482, 5.571433845147086394 ) ) ;
#24274=ADVANCED_FACE ( 'NONE', ( #15212 ), #40766, .F. ) ;
#24275=DIRECTION ( 'NONE',  ( -0.5449076811759708816, 0.6444004775717707689, 0.5364919789714475140 ) ) ;
#24276=AXIS2_PLACEMENT_3D ( 'NONE', #28584, #45908, #7025 ) ;
#24277=PLANE ( 'NONE',  #26031 ) ;
#24278=EDGE_LOOP ( 'NONE', ( #19021, #18395, #15349, #39295 ) ) ;
#24279=PLANE ( 'NONE',  #51014 ) ;
#24280=CARTESIAN_POINT ( 'NONE',  ( -16.76996837579439870, 0.000000000000000000, 9.732398803345603255 ) ) ;
#24281=DIRECTION ( 'NONE',  ( 0.7660212471507180654, -0.6427876096865404731, 0.005961354470445141482 ) ) ;
#24282=ORIENTED_EDGE ( 'NONE', *, *, #54985, .F. ) ;
#24283=VECTOR ( 'NONE', #48049, 1000.000000000000227 ) ;
#24284=DIRECTION ( 'NONE',  ( -0.5449076811759708816, 0.6444004775717707689, 0.5364919789714475140 ) ) ;
#24285=ORIENTED_EDGE ( 'NONE', *, *, #4133, .T. ) ;
#24286=ORIENTED_EDGE ( 'NONE', *, *, #33568, .T. ) ;
#24287=ORIENTED_EDGE ( 'NONE', *, *, #28489, .F. ) ;
#24288=ORIENTED_EDGE ( 'NONE', *, *, #6842, .T. ) ;
#24289=ORIENTED_EDGE ( 'NONE', *, *, #3977, .F. ) ;
#24290=FACE_OUTER_BOUND ( 'NONE', #56120, .T. ) ;
#24291=ORIENTED_EDGE ( 'NONE', *, *, #36014, .F. ) ;
#24292=VERTEX_POINT ( 'NONE', #41324 ) ;
#24293=DIRECTION ( 'NONE',  ( 0.5449076811759707706, 0.6444004775717708799, -0.5364919789714476250 ) ) ;
#24294=EDGE_CURVE ( 'NONE', #6114, #2679, #36488, .T. ) ;
#24295=ORIENTED_EDGE ( 'NONE', *, *, #31553, .T. ) ;
#24296=ORIENTED_EDGE ( 'NONE', *, *, #52869, .T. ) ;
#24297=LINE ( 'NONE', #28263, #33016 ) ;
#24298=CARTESIAN_POINT ( 'NONE',  ( -15.27194367764935379, 3.524445264749008100, 8.597677798291803342 ) ) ;
#24299=CARTESIAN_POINT ( 'NONE',  ( -15.99282684534787613, 0.000000000000000000, 3.587951039638777484 ) ) ;
#24300=DIRECTION ( 'NONE',  ( 0.9999697198139515519, 0.000000000000000000, 0.007781995580013368816 ) ) ;
#24301=ORIENTED_EDGE ( 'NONE', *, *, #27074, .T. ) ;
#24302=ADVANCED_FACE ( 'NONE', ( #23989 ), #49574, .F. ) ;
#24303=ORIENTED_EDGE ( 'NONE', *, *, #29190, .T. ) ;
#24304=CARTESIAN_POINT ( 'NONE',  ( -11.72337221537584107, -0.1191753592594181482, 5.198508230121311691 ) ) ;
#24305=DIRECTION ( 'NONE',  ( -0.005002170337468016433, -0.7660444431189770143, 0.6427681459581293666 ) ) ;
#24306=EDGE_CURVE ( 'NONE', #33602, #52686, #6974, .T. ) ;
#24307=EDGE_CURVE ( 'NONE', #31801, #14557, #10683, .T. ) ;
#24308=CARTESIAN_POINT ( 'NONE',  ( -31.72626587586518099, 0.000000000000000000, 9.005490826201270949 ) ) ;
#24309=LINE ( 'NONE', #10713, #23102 ) ;
#24310=CARTESIAN_POINT ( 'NONE',  ( -14.13008755008897310, 0.000000000000000000, 3.063789224158076419 ) ) ;
#24311=DIRECTION ( 'NONE',  ( -0.6246952433987894571, 0.7422098413412802076, 0.2426528472758539834 ) ) ;
#24312=VERTEX_POINT ( 'NONE', #37315 ) ;
#24313=PLANE ( 'NONE',  #52839 ) ;
#24314=ADVANCED_FACE ( 'NONE', ( #2414 ), #49829, .F. ) ;
#24315=ORIENTED_EDGE ( 'NONE', *, *, #35065, .F. ) ;
#24316=VECTOR ( 'NONE', #43580, 999.9999999999998863 ) ;
#24317=DIRECTION ( 'NONE',  ( -0.9999697198139514409, -0.000000000000000000, -0.007781995580013368816 ) ) ;
#24318=PLANE ( 'NONE',  #46851 ) ;
#24319=EDGE_CURVE ( 'NONE', #41524, #10050, #41590, .T. ) ;
#24320=CARTESIAN_POINT ( 'NONE',  ( -13.94733792715787857, 0.000000000000000000, 5.281203842820665351 ) ) ;
#24321=CARTESIAN_POINT ( 'NONE',  ( -19.60834386242827776, 0.000000000000000000, 4.298478389818581213 ) ) ;
#24322=ADVANCED_FACE ( 'NONE', ( #23451 ), #19159, .F. ) ;
#24323=LINE ( 'NONE', #41629, #22317 ) ;
#24324=ORIENTED_EDGE ( 'NONE', *, *, #16183, .F. ) ;
#24325=CARTESIAN_POINT ( 'NONE',  ( -18.58640238944216705, 0.000000000000000000, 4.306431374662254008 ) ) ;
#24326=DIRECTION ( 'NONE',  ( 0.7660212471507180654, -0.6427876096865404731, 0.005961354470445141482 ) ) ;
#24327=CARTESIAN_POINT ( 'NONE',  ( -19.42906346370737580, 0.000000000000000000, 7.623862219596294842 ) ) ;
#24328=EDGE_CURVE ( 'NONE', #16476, #25539, #32779, .T. ) ;
#24329=CARTESIAN_POINT ( 'NONE',  ( 2.072287782118878319, 0.000000000000000000, -2.950529333540147015 ) ) ;
#24330=CARTESIAN_POINT ( 'NONE',  ( -1.086233639165236964, 0.000000000000000000, -2.796443541562362078 ) ) ;
#24331=DIRECTION ( 'NONE',  ( 0.000000000000000000, -1.000000000000000000, 0.000000000000000000 ) ) ;
#24332=DIRECTION ( 'NONE',  ( -0.7660212471507179544, -0.6427876096865405842, -0.005961354470445141482 ) ) ;
#24333=ADVANCED_FACE ( 'NONE', ( #2672 ), #24533, .F. ) ;
#24334=PLANE ( 'NONE',  #6978 ) ;
#24335=DIRECTION ( 'NONE',  ( -0.5449076811759708816, 0.6444004775717707689, 0.5364919789714475140 ) ) ;
#24336=ORIENTED_EDGE ( 'NONE', *, *, #29998, .T. ) ;
#24337=ORIENTED_EDGE ( 'NONE', *, *, #7877, .T. ) ;
#24338=VERTEX_POINT ( 'NONE', #32253 ) ;
#24339=ORIENTED_EDGE ( 'NONE', *, *, #48909, .T. ) ;
#24340=ORIENTED_EDGE ( 'NONE', *, *, #15378, .T. ) ;
#24341=DIRECTION ( 'NONE',  ( 0.007781995580012663651, -3.146120232559066537E-19, -0.9999697198139514409 ) ) ;
#24342=DIRECTION ( 'NONE',  ( -0.5364919789714478471, 0.6444004775717705469, -0.5449076811759709926 ) ) ;
#24343=DIRECTION ( 'NONE',  ( 0.7660212471507180654, -0.6427876096865404731, 0.005961354470445141482 ) ) ;
#24344=AXIS2_PLACEMENT_3D ( 'NONE', #25105, #33886, #42417 ) ;
#24345=EDGE_LOOP ( 'NONE', ( #52439, #2256, #21978, #52688 ) ) ;
#24346=CARTESIAN_POINT ( 'NONE',  ( -18.45093045568905410, 5.143464774974012776, 3.684796261400164141 ) ) ;
#24347=EDGE_CURVE ( 'NONE', #41029, #48142, #45298, .T. ) ;
#24348=ORIENTED_EDGE ( 'NONE', *, *, #15690, .T. ) ;
#24349=CARTESIAN_POINT ( 'NONE',  ( -26.13493519185646008, 0.000000000000000000, 7.033017491833586377 ) ) ;
#24350=VERTEX_POINT ( 'NONE', #12618 ) ;
#24352=LINE ( 'NONE', #32342, #22835 ) ;
#24353=LINE ( 'NONE', #19539, #11431 ) ;
#24354=ORIENTED_EDGE ( 'NONE', *, *, #22062, .F. ) ;
#24356=ORIENTED_EDGE ( 'NONE', *, *, #28065, .T. ) ;
#24357=CARTESIAN_POINT ( 'NONE',  ( -10.89487359323307025, 0.000000000000000000, 5.304958826080728329 ) ) ;
#24358=CARTESIAN_POINT ( 'NONE',  ( -16.01581927339013589, 0.000000000000000000, 6.542428665700890988 ) ) ;
#24359=EDGE_CURVE ( 'NONE', #15067, #6267, #52065, .T. ) ;
#24360=PLANE ( 'NONE',  #33571 ) ;
#24361=CARTESIAN_POINT ( 'NONE',  ( -19.86075176232942496, 0.000000000000000000, 6.512506512018135574 ) ) ;
#24362=CARTESIAN_POINT ( 'NONE',  ( -14.01545677930355183, 0.000000000000000000, 2.126011111488108174 ) ) ;
#24363=CARTESIAN_POINT ( 'NONE',  ( -16.45933145549171428, 1.095915999411505082, 5.073269275807504641 ) ) ;
#24364=CARTESIAN_POINT ( 'NONE',  ( -16.43317633868556626, -0.1191753592594197858, 13.31363028683540151 ) ) ;
#24365=FACE_OUTER_BOUND ( 'NONE', #12716, .T. ) ;
#24366=LINE ( 'NONE', #11852, #22047 ) ;
#24367=ORIENTED_EDGE ( 'NONE', *, *, #26195, .F. ) ;
#24368=DIRECTION ( 'NONE',  ( -0.6427681459581293666, -0.7660444431189770143, -0.005002170337467561935 ) ) ;
#24369=ORIENTED_EDGE ( 'NONE', *, *, #31806, .F. ) ;
#24371=LINE ( 'NONE', #50510, #54112 ) ;
#24372=ADVANCED_FACE ( 'NONE', ( #25974 ), #37901, .F. ) ;
#24373=CARTESIAN_POINT ( 'NONE',  ( -18.60031110817512356, 1.419719901456505395, 6.436315848785716831 ) ) ;
#24374=DIRECTION ( 'NONE',  ( 0.005961354470445682716, -0.6427876096865404731, -0.7660212471507180654 ) ) ;
#24375=LINE ( 'NONE', #32369, #28612 ) ;
#24376=ADVANCED_FACE ( 'NONE', ( #29081 ), #7500, .F. ) ;
#24377=CARTESIAN_POINT ( 'NONE',  ( -11.21979143729918960, -0.1191753592594197858, 1.139774444304266554 ) ) ;
#24378=VERTEX_POINT ( 'NONE', #47530 ) ;
#24379=DIRECTION ( 'NONE',  ( -0.6427681459581293666, -0.7660444431189770143, -0.005002170337467561935 ) ) ;
#24380=DIRECTION ( 'NONE',  ( -0.5364919789714478471, 0.6444004775717705469, -0.5449076811759709926 ) ) ;
#24381=CARTESIAN_POINT ( 'NONE',  ( -14.26863008609943329, 0.000000000000000000, 2.324046914494605875 ) ) ;
#24382=DIRECTION ( 'NONE',  ( -0.5449076811759708816, 0.6444004775717707689, 0.5364919789714475140 ) ) ;
#24383=CARTESIAN_POINT ( 'NONE',  ( -12.99351530631744289, 0.000000000000000000, 2.133964096331779636 ) ) ;
#24384=EDGE_CURVE ( 'NONE', #15979, #48336, #33618, .T. ) ;
#24385=COLOUR_RGB ( '', 0.31764706, 0.68627451, 0.89019608) ;
#24386=DIRECTION ( 'NONE',  ( 0.000000000000000000, -0.000000000000000000, -1.000000000000000000 ) ) ;
#24387=DIRECTION ( 'NONE',  ( -0.7660212471507179544, -0.6427876096865405842, -0.005961354470445141482 ) ) ;
#24388=CARTESIAN_POINT ( 'NONE',  ( -23.33693525117809386, 0.000000000000000000, 5.746789908705562944 ) ) ;
#24389=CARTESIAN_POINT ( 'NONE',  ( -9.856202467495650765, -0.1191753592594188005, 4.105042767420058247 ) ) ;
#24391=EDGE_CURVE ( 'NONE', #41524, #32862, #8643, .T. ) ;
#24392=CARTESIAN_POINT ( 'NONE',  ( -16.79925329029790149, 0.000000000000000000, 13.49544742625427496 ) ) ;
#24393=ORIENTED_EDGE ( 'NONE', *, *, #4263, .T. ) ;
#24394=CARTESIAN_POINT ( 'NONE',  ( -32.65997012216863737, 0.000000000000000000, 9.567562649885804404 ) ) ;
#24395=DIRECTION ( 'NONE',  ( 0.5449076811759707706, 0.6444004775717708799, -0.5364919789714476250 ) ) ;
#24396=ORIENTED_EDGE ( 'NONE', *, *, #1288, .F. ) ;
#24397=VERTEX_POINT ( 'NONE', #7812 ) ;
#24398=DIRECTION ( 'NONE',  ( 0.007781995580012663651, -3.146120232559066537E-19, -0.9999697198139514409 ) ) ;
#24399=ORIENTED_EDGE ( 'NONE', *, *, #18563, .T. ) ;
#24400=ORIENTED_EDGE ( 'NONE', *, *, #2448, .T. ) ;
#24401=ORIENTED_EDGE ( 'NONE', *, *, #33475, .T. ) ;
#24402=DIRECTION ( 'NONE',  ( -0.5364919789714478471, 0.6444004775717705469, -0.5449076811759709926 ) ) ;
#24404=CARTESIAN_POINT ( 'NONE',  ( -8.609916609573598834, 0.000000000000000000, 10.23519010964256637 ) ) ;
#24405=EDGE_CURVE ( 'NONE', #45690, #46955, #34745, .T. ) ;
#24406=ORIENTED_EDGE ( 'NONE', *, *, #48440, .T. ) ;
#24407=ADVANCED_FACE ( 'NONE', ( #46979 ), #12034, .F. ) ;
#24408=ORIENTED_EDGE ( 'NONE', *, *, #7588, .T. ) ;
#24410=LINE ( 'NONE', #50251, #17291 ) ;
#24411=ORIENTED_EDGE ( 'NONE', *, *, #47474, .F. ) ;
#24413=FACE_OUTER_BOUND ( 'NONE', #38312, .T. ) ;
#24415=FACE_OUTER_BOUND ( 'NONE', #54288, .T. ) ;
#24416=CARTESIAN_POINT ( 'NONE',  ( -18.22254066414048168, -0.1191753592594167466, 4.409266058853649639 ) ) ;
#24417=EDGE_CURVE ( 'NONE', #3505, #6678, #25132, .T. ) ;
#24418=EDGE_CURVE ( 'NONE', #32474, #17347, #29370, .T. ) ;
#24421=ORIENTED_EDGE ( 'NONE', *, *, #43307, .F. ) ;
#24422=CARTESIAN_POINT ( 'NONE',  ( -9.878549426739102302, -0.06895642802817161798, 1.561684332249249296 ) ) ;
#24423=DIRECTION ( 'NONE',  ( 0.000000000000000000, -0.000000000000000000, -1.000000000000000000 ) ) ;
#24424=VERTEX_POINT ( 'NONE', #16885 ) ;
#24425=PLANE ( 'NONE',  #7686 ) ;
#24426=DIRECTION ( 'NONE',  ( -0.9999697198139514409, -0.000000000000000000, -0.007781995580013368816 ) ) ;
#24427=CARTESIAN_POINT ( 'NONE',  ( -10.76535788664084592, -0.1191753592594202438, 1.512643021079689953 ) ) ;
#24428=EDGE_LOOP ( 'NONE', ( #29302, #55049, #34261, #28506 ) ) ;
#24429=LINE ( 'NONE', #41739, #19243 ) ;
#24430=LINE ( 'NONE', #2297, #38701 ) ;
#24431=CARTESIAN_POINT ( 'NONE',  ( -20.54049170961573267, 0.000000000000000000, 4.660556269540326646 ) ) ;
#24432=ADVANCED_FACE ( 'NONE', ( #8081 ), #38750, .F. ) ;
#24433=FACE_OUTER_BOUND ( 'NONE', #26286, .T. ) ;
#24434=CARTESIAN_POINT ( 'NONE',  ( -20.54204810873173415, 0.000000000000000000, 4.860550213503115558 ) ) ;
#24435=PLANE ( 'NONE',  #32477 ) ;
#24436=EDGE_CURVE ( 'NONE', #30300, #43916, #33912, .T. ) ;
#24437=ADVANCED_FACE ( 'NONE', ( #46687 ), #42696, .F. ) ;
#24439=ORIENTED_EDGE ( 'NONE', *, *, #13362, .T. ) ;
#24440=CARTESIAN_POINT ( 'NONE',  ( -15.23141738930936739, -2.622721114510659035, 6.902663673731017191 ) ) ;
#24441=CARTESIAN_POINT ( 'NONE',  ( 2.072287782118878319, 0.000000000000000000, -2.950529333540147015 ) ) ;
#24442=EDGE_CURVE ( 'NONE', #46093, #2126, #38446, .T. ) ;
#24443=LINE ( 'NONE', #50581, #42305 ) ;
#24444=ORIENTED_EDGE ( 'NONE', *, *, #29156, .F. ) ;
#24445=DIRECTION ( 'NONE',  ( 0.9999697198139515519, 0.000000000000000000, 0.007781995580013368816 ) ) ;
#24446=DIRECTION ( 'NONE',  ( -0.005002170337468016433, -0.7660444431189770143, 0.6427681459581293666 ) ) ;
#24447=EDGE_CURVE ( 'NONE', #12870, #43988, #55474, .T. ) ;
#24448=PLANE ( 'NONE',  #51270 ) ;
#24449=LINE ( 'NONE', #41509, #28750 ) ;
#24450=EDGE_CURVE ( 'NONE', #6826, #40411, #34216, .T. ) ;
#24451=DIRECTION ( 'NONE',  ( 0.000000000000000000, 1.000000000000000000, 0.000000000000000000 ) ) ;
#24452=ORIENTED_EDGE ( 'NONE', *, *, #36270, .T. ) ;
#24453=ORIENTED_EDGE ( 'NONE', *, *, #6811, .F. ) ;
#24454=DIRECTION ( 'NONE',  ( 0.005961354470445682716, -0.6427876096865404731, -0.7660212471507180654 ) ) ;
#24455=DIRECTION ( 'NONE',  ( 0.005961354470445682716, -0.6427876096865404731, -0.7660212471507180654 ) ) ;
#24456=LINE ( 'NONE', #9829, #32020 ) ;
#24458=CARTESIAN_POINT ( 'NONE',  ( -15.50102849149811135, -0.1191753592594197858, 12.95155240711365430 ) ) ;
#24459=ORIENTED_EDGE ( 'NONE', *, *, #5529, .F. ) ;
#24460=CARTESIAN_POINT ( 'NONE',  ( -16.70641145532281868, 4.657758921906509642, 11.01483458552420025 ) ) ;
#24461=EDGE_LOOP ( 'NONE', ( #305, #17327, #14491, #28269 ) ) ;
#24462=VERTEX_POINT ( 'NONE', #35582 ) ;
#24463=DIRECTION ( 'NONE',  ( -0.5364919789714478471, 0.6444004775717705469, -0.5449076811759709926 ) ) ;
#24464=DIRECTION ( 'NONE',  ( 0.9999697198139515519, 0.000000000000000000, 0.007781995580013368816 ) ) ;
#24465=DIRECTION ( 'NONE',  ( 0.5449076811759707706, 0.6444004775717708799, -0.5364919789714476250 ) ) ;
#24466=VERTEX_POINT ( 'NONE', #35320 ) ;
#24467=FACE_OUTER_BOUND ( 'NONE', #15431, .T. ) ;
#24468=ORIENTED_EDGE ( 'NONE', *, *, #54193, .F. ) ;
#24469=VERTEX_POINT ( 'NONE', #18252 ) ;
#24470=EDGE_LOOP ( 'NONE', ( #12424, #43871, #13727, #50423 ) ) ;
#24471=LINE ( 'NONE', #15152, #52215 ) ;
#24472=DIRECTION ( 'NONE',  ( -0.6427681459581293666, -0.7660444431189770143, -0.005002170337467561935 ) ) ;
#24473=EDGE_LOOP ( 'NONE', ( #6981, #22039, #34532, #52532 ) ) ;
#24474=LINE ( 'NONE', #11443, #16671 ) ;
#24475=VERTEX_POINT ( 'NONE', #14010 ) ;
#24476=DIRECTION ( 'NONE',  ( -0.7660212471507179544, -0.6427876096865405842, -0.005961354470445141482 ) ) ;
#24477=PLANE ( 'NONE',  #17757 ) ;
#24478=EDGE_CURVE ( 'NONE', #38023, #5343, #52900, .T. ) ;
#24479=EDGE_CURVE ( 'NONE', #8687, #15659, #22801, .T. ) ;
#24480=ORIENTED_EDGE ( 'NONE', *, *, #27435, .F. ) ;
#24481=LINE ( 'NONE', #11448, #40414 ) ;
#24482=ORIENTED_EDGE ( 'NONE', *, *, #14264, .T. ) ;
#24483=EDGE_CURVE ( 'NONE', #28250, #25448, #52617, .T. ) ;
#24484=VECTOR ( 'NONE', #1921, 999.9999999999998863 ) ;
#24485=CARTESIAN_POINT ( 'NONE',  ( -17.26532721389163072, 0.000000000000000000, 13.67648636611514590 ) ) ;
#24486=DIRECTION ( 'NONE',  ( -0.9999697198139514409, -0.000000000000000000, -0.007781995580013368816 ) ) ;
#24487=DIRECTION ( 'NONE',  ( -0.9999697198139514409, -0.000000000000000000, -0.007781995580013368816 ) ) ;
#24488=CARTESIAN_POINT ( 'NONE',  ( -9.774228016103954531, 0.000000000000000000, 6.421676158506044452 ) ) ;
#24489=LINE ( 'NONE', #12297, #14207 ) ;
#24490=DIRECTION ( 'NONE',  ( 0.7660212471507180654, -0.6427876096865404731, 0.005961354470445141482 ) ) ;
#24491=ORIENTED_EDGE ( 'NONE', *, *, #2873, .F. ) ;
#24492=ORIENTED_EDGE ( 'NONE', *, *, #8095, .F. ) ;
#24493=CARTESIAN_POINT ( 'NONE',  ( -18.51965916356675024, 5.143464774974010112, 12.51628762540889994 ) ) ;
#24494=DIRECTION ( 'NONE',  ( -0.6246952433987893460, -0.7422098413412802076, 0.2426528472758542054 ) ) ;
#24495=LINE ( 'NONE', #20543, #53972 ) ;
#24496=DIRECTION ( 'NONE',  ( -0.5449076811759708816, 0.6444004775717707689, 0.5364919789714475140 ) ) ;
#24497=LINE ( 'NONE', #6933, #690 ) ;
#24498=EDGE_CURVE ( 'NONE', #23038, #22613, #39594, .T. ) ;
#24499=CARTESIAN_POINT ( 'NONE',  ( -17.26532721389163072, 0.000000000000000000, 13.67648636611514590 ) ) ;
#24500=ORIENTED_EDGE ( 'NONE', *, *, #15766, .T. ) ;
#24501=LINE ( 'NONE', #55443, #53120 ) ;
#24503=ORIENTED_EDGE ( 'NONE', *, *, #53089, .F. ) ;
#24504=CARTESIAN_POINT ( 'NONE',  ( -12.60008893460168622, 2.067327705546505801, 1.510275597055831698 ) ) ;
#24505=DIRECTION ( 'NONE',  ( -0.005002170337468016433, -0.7660444431189770143, 0.6427681459581293666 ) ) ;
#24506=VERTEX_POINT ( 'NONE', #53212 ) ;
#24507=DIRECTION ( 'NONE',  ( 0.000000000000000000, -0.000000000000000000, -1.000000000000000000 ) ) ;
#24508=LINE ( 'NONE', #41568, #21491 ) ;
#24509=ADVANCED_FACE ( 'NONE', ( #48077 ), #43817, .F. ) ;
#24510=CARTESIAN_POINT ( 'NONE',  ( -8.479536098004086142, -0.1191753592594181482, 6.331748722270672758 ) ) ;
#24511=ADVANCED_FACE ( 'NONE', ( #14313 ), #26497, .F. ) ;
#24512=LINE ( 'NONE', #8062, #33255 ) ;
#24513=LINE ( 'NONE', #2920, #8374 ) ;
#24514=VERTEX_POINT ( 'NONE', #48357 ) ;
#24515=EDGE_CURVE ( 'NONE', #50834, #56081, #31033, .T. ) ;
#24516=VERTEX_POINT ( 'NONE', #9183 ) ;
#24517=PLANE ( 'NONE',  #23031 ) ;
#24518=CARTESIAN_POINT ( 'NONE',  ( -9.542064456761055524, 0.000000000000000000, 10.59726798936431180 ) ) ;
#24519=CARTESIAN_POINT ( 'NONE',  ( -10.77110599365141042, -0.1191753592594194527, 2.251262427595218885 ) ) ;
#24520=EDGE_CURVE ( 'NONE', #44275, #53402, #5483, .T. ) ;
#24521=CARTESIAN_POINT ( 'NONE',  ( -11.35220598394758262, 0.000000000000000000, 4.362729563834402136 ) ) ;
#24522=DIRECTION ( 'NONE',  ( -0.9999697198139514409, -0.000000000000000000, -0.007781995580013368816 ) ) ;
#24523=EDGE_CURVE ( 'NONE', #6407, #8862, #1515, .T. ) ;
#24524=PLANE ( 'NONE',  #7705 ) ;
#24525=ORIENTED_EDGE ( 'NONE', *, *, #13425, .T. ) ;
#24526=FACE_OUTER_BOUND ( 'NONE', #50082, .T. ) ;
#24527=VECTOR ( 'NONE', #18226, 1000.000000000000227 ) ;
#24528=LINE ( 'NONE', #20272, #19600 ) ;
#24529=CARTESIAN_POINT ( 'NONE',  ( -15.60102546347950536, 0.000000000000000000, 12.95077420755565356 ) ) ;
#24530=ORIENTED_EDGE ( 'NONE', *, *, #34420, .T. ) ;
#24531=FACE_OUTER_BOUND ( 'NONE', #45206, .T. ) ;
#24532=DIRECTION ( 'NONE',  ( 0.005002170337468016433, -0.7660444431189770143, -0.6427681459581293666 ) ) ;
#24533=PLANE ( 'NONE',  #55634 ) ;
#24534=ORIENTED_EDGE ( 'NONE', *, *, #38328, .F. ) ;
#24535=DIRECTION ( 'NONE',  ( 0.007781995580012662783, 0.000000000000000000, -0.9999697198139514409 ) ) ;
#24536=ORIENTED_EDGE ( 'NONE', *, *, #11083, .F. ) ;
#24537=ORIENTED_EDGE ( 'NONE', *, *, #12906, .T. ) ;
#24538=ORIENTED_EDGE ( 'NONE', *, *, #4055, .F. ) ;
#24539=ORIENTED_EDGE ( 'NONE', *, *, #49843, .F. ) ;
#24542=CARTESIAN_POINT ( 'NONE',  ( -10.79409842169367373, -0.1191753592594179401, 5.205740053657330613 ) ) ;
#24543=ORIENTED_EDGE ( 'NONE', *, *, #22898, .F. ) ;
#24544=EDGE_CURVE ( 'NONE', #33009, #24728, #13464, .T. ) ;
#24545=VECTOR ( 'NONE', #50551, 999.9999999999998863 ) ;
#24546=EDGE_LOOP ( 'NONE', ( #33842, #34085, #39319, #33770 ) ) ;
#24547=CARTESIAN_POINT ( 'NONE',  ( -17.74404816805336793, 0.000000000000000000, 3.574322630375089460 ) ) ;
#24548=ORIENTED_EDGE ( 'NONE', *, *, #47907, .T. ) ;
#24549=VERTEX_POINT ( 'NONE', #18845 ) ;
#24550=EDGE_CURVE ( 'NONE', #11444, #25938, #22541, .T. ) ;
#24551=EDGE_CURVE ( 'NONE', #38228, #55983, #26791, .T. ) ;
#24552=LINE ( 'NONE', #37336, #14909 ) ;
#24553=DIRECTION ( 'NONE',  ( 0.5449076811759707706, 0.6444004775717708799, -0.5364919789714476250 ) ) ;
#24555=CARTESIAN_POINT ( 'NONE',  ( -18.67697421479882181, -0.1191753592594197858, 4.036397482078229793 ) ) ;
#24556=DIRECTION ( 'NONE',  ( 0.000000000000000000, -0.000000000000000000, -1.000000000000000000 ) ) ;
#24557=ORIENTED_EDGE ( 'NONE', *, *, #46627, .T. ) ;
#24559=AXIS2_PLACEMENT_3D ( 'NONE', #20452, #23864, #41192 ) ;
#24560=DIRECTION ( 'NONE',  ( -0.9321478471874540261, 0.000000000000000000, 0.3620778797217457656 ) ) ;
#24561=CARTESIAN_POINT ( 'NONE',  ( 2.072287782118878319, 0.000000000000000000, -2.950529333540147015 ) ) ;
#24563=EDGE_CURVE ( 'NONE', #31490, #54764, #47827, .T. ) ;
#24564=VECTOR ( 'NONE', #31738, 1000.000000000000000 ) ;
#24565=DIRECTION ( 'NONE',  ( 0.9999697198139515519, 0.000000000000000000, 0.007781995580013368816 ) ) ;
#24566=CARTESIAN_POINT ( 'NONE',  ( -16.72210669506725722, 0.000000000000000000, 3.582275615218761367 ) ) ;
#24567=CARTESIAN_POINT ( 'NONE',  ( -10.27421835998572064, 0.000000000000000000, 10.96090226820206048 ) ) ;
#24568=LINE ( 'NONE', #54981, #52198 ) ;
#24569=ORIENTED_EDGE ( 'NONE', *, *, #3652, .T. ) ;
#24570=FACE_OUTER_BOUND ( 'NONE', #38743, .T. ) ;
#24571=VERTEX_POINT ( 'NONE', #4646 ) ;
#24572=DIRECTION ( 'NONE',  ( 0.5449076811759707706, 0.6444004775717708799, -0.5364919789714476250 ) ) ;
#24574=CARTESIAN_POINT ( 'NONE',  ( -15.13495153988577968, 0.000000000000000000, 12.76973526769478084 ) ) ;
#24575=LINE ( 'NONE', #19782, #21786 ) ;
#24576=FACE_OUTER_BOUND ( 'NONE', #36203, .T. ) ;
#24577=EDGE_CURVE ( 'NONE', #7363, #1451, #21957, .T. ) ;
#24578=CARTESIAN_POINT ( 'NONE',  ( -9.492340742193960068, 0.000000000000000000, 4.207877451611462760 ) ) ;
#24579=ORIENTED_EDGE ( 'NONE', *, *, #38088, .F. ) ;
#24580=EDGE_CURVE ( 'NONE', #20518, #51745, #375, .T. ) ;
#24581=ORIENTED_EDGE ( 'NONE', *, *, #47901, .T. ) ;
#24582=DIRECTION ( 'NONE',  ( -0.5364919789714478471, 0.6444004775717705469, -0.5449076811759709926 ) ) ;
#24583=FACE_OUTER_BOUND ( 'NONE', #5440, .T. ) ;
#24584=DIRECTION ( 'NONE',  ( 0.5449076811759707706, 0.6444004775717708799, -0.5364919789714476250 ) ) ;
#24585=VECTOR ( 'NONE', #31170, 1000.000000000000000 ) ;
#24586=AXIS2_PLACEMENT_3D ( 'NONE', #13599, #10179, #40588 ) ;
#24587=DIRECTION ( 'NONE',  ( -0.9999697198139514409, -0.000000000000000000, -0.007781995580013368816 ) ) ;
#24588=EDGE_CURVE ( 'NONE', #23847, #18842, #35059, .T. ) ;
#24589=LINE ( 'NONE', #12943, #37572 ) ;
#24590=CARTESIAN_POINT ( 'NONE',  ( -26.13337879274045505, 0.000000000000000000, 6.833023547870798353 ) ) ;
#24591=FACE_OUTER_BOUND ( 'NONE', #6204, .T. ) ;
#24592=CARTESIAN_POINT ( 'NONE',  ( -22.40478740399063895, 0.000000000000000000, 5.384712028983816623 ) ) ;
#24593=PLANE ( 'NONE',  #53697 ) ;
#24594=ADVANCED_FACE ( 'NONE', ( #32175 ), #27926, .F. ) ;
#24595=ORIENTED_EDGE ( 'NONE', *, *, #53482, .T. ) ;
#24596=EDGE_CURVE ( 'NONE', #32862, #33548, #11124, .T. ) ;
#24597=EDGE_CURVE ( 'NONE', #14051, #11826, #19927, .T. ) ;
#24598=VECTOR ( 'NONE', #49359, 999.9999999999998863 ) ;
#24599=ORIENTED_EDGE ( 'NONE', *, *, #13460, .F. ) ;
#24600=EDGE_LOOP ( 'NONE', ( #52115, #4111, #47967, #20274 ) ) ;
#24601=VERTEX_POINT ( 'NONE', #49766 ) ;
#24602=ORIENTED_EDGE ( 'NONE', *, *, #21695, .T. ) ;
#24603=PLANE ( 'NONE',  #16023 ) ;
#24604=CARTESIAN_POINT ( 'NONE',  ( -21.47419595591918906, 0.000000000000000000, 5.222628093224860102 ) ) ;
#24605=ADVANCED_FACE ( 'NONE', ( #1769 ), #49193, .F. ) ;
#24606=DIRECTION ( 'NONE',  ( -0.5449076811759708816, 0.6444004775717707689, 0.5364919789714475140 ) ) ;
#24608=EDGE_CURVE ( 'NONE', #32882, #370, #36416, .T. ) ;
#24609=EDGE_LOOP ( 'NONE', ( #19864, #11048, #24503, #7208 ) ) ;
#24610=EDGE_LOOP ( 'NONE', ( #35663, #19877, #51547 ) ) ;
#24611=DIRECTION ( 'NONE',  ( -0.2426528472758541499, 0.7422098413412800966, -0.6246952433987894571 ) ) ;
#24612=ORIENTED_EDGE ( 'NONE', *, *, #50414, .T. ) ;
#24613=ADVANCED_FACE ( 'NONE', ( #10613 ), #53728, .F. ) ;
#24615=LINE ( 'NONE', #41114, #15561 ) ;
#24616=CARTESIAN_POINT ( 'NONE',  ( -27.06552663992790997, 0.000000000000000000, 7.195101427592543786 ) ) ;
#24618=DIRECTION ( 'NONE',  ( 0.005961354470445682716, -0.6427876096865404731, -0.7660212471507180654 ) ) ;
#24619=VERTEX_POINT ( 'NONE', #45482 ) ;
#24620=ADVANCED_FACE ( 'NONE', ( #11428 ), #10312, .F. ) ;
#24621=VECTOR ( 'NONE', #45912, 999.9999999999998863 ) ;
#24622=VECTOR ( 'NONE', #23942, 1000.000000000000227 ) ;
#24623=ADVANCED_FACE ( 'NONE', ( #2870 ), #23632, .F. ) ;
#24624=CARTESIAN_POINT ( 'NONE',  ( -17.46532115785441519, 0.000000000000000000, 13.67492996699914265 ) ) ;
#24625=DIRECTION ( 'NONE',  ( 0.007781995580012663651, -3.146120232559066537E-19, -0.9999697198139514409 ) ) ;
#24626=EDGE_CURVE ( 'NONE', #24462, #9004, #6332, .T. ) ;
#24627=CARTESIAN_POINT ( 'NONE',  ( -22.40478740399063895, 0.000000000000000000, 5.384712028983816623 ) ) ;
#24628=VECTOR ( 'NONE', #8303, 1000.000000000000000 ) ;
#24629=FACE_OUTER_BOUND ( 'NONE', #29525, .T. ) ;
#24630=CARTESIAN_POINT ( 'NONE',  ( -13.17065887352947762, -0.1191753592594197858, 12.04635770780929427 ) ) ;
#24631=DIRECTION ( 'NONE',  ( 0.007781995580012662783, 0.000000000000000000, -0.9999697198139514409 ) ) ;
#24632=DIRECTION ( 'NONE',  ( 0.9999697198139515519, 0.000000000000000000, 0.007781995580013368816 ) ) ;
#24633=LINE ( 'NONE', #32358, #51943 ) ;
#24634=ORIENTED_EDGE ( 'NONE', *, *, #5590, .T. ) ;
#24635=PLANE ( 'NONE',  #16565 ) ;
#24636=VERTEX_POINT ( 'NONE', #23915 ) ;
#24637=DIRECTION ( 'NONE',  ( -0.005002170337468016433, -0.7660444431189770143, 0.6427681459581293666 ) ) ;
#24638=DIRECTION ( 'NONE',  ( -0.5449076811759708816, 0.6444004775717707689, 0.5364919789714475140 ) ) ;
#24639=DIRECTION ( 'NONE',  ( 0.9999697198139515519, 0.000000000000000000, 0.007781995580013368816 ) ) ;
#24640=VECTOR ( 'NONE', #14121, 1000.000000000000227 ) ;
#24641=DIRECTION ( 'NONE',  ( 0.6427681459581294776, -0.7660444431189769032, 0.005002170337467562802 ) ) ;
#24642=CARTESIAN_POINT ( 'NONE',  ( -20.54204810873173415, 0.000000000000000000, 4.860550213503115558 ) ) ;
#24643=VECTOR ( 'NONE', #11718, 999.9999999999998863 ) ;
#24644=CARTESIAN_POINT ( 'NONE',  ( -14.94760462649100496, 0.000000000000000000, 2.488088991209854051 ) ) ;
#24646=ORIENTED_EDGE ( 'NONE', *, *, #55641, .F. ) ;
#24647=DIRECTION ( 'NONE',  ( 0.007781995580012663651, -3.146120232559066537E-19, -0.9999697198139514409 ) ) ;
#24648=LINE ( 'NONE', #50776, #42972 ) ;
#24649=DIRECTION ( 'NONE',  ( -0.7660212471507179544, -0.6427876096865405842, -0.005961354470445141482 ) ) ;
#24650=PLANE ( 'NONE',  #8242 ) ;
#24652=DIRECTION ( 'NONE',  ( 0.007781995580012663651, -3.146120232559066537E-19, -0.9999697198139514409 ) ) ;
#24653=EDGE_CURVE ( 'NONE', #14368, #41698, #36709, .T. ) ;
#24654=CARTESIAN_POINT ( 'NONE',  ( -12.60458797795435615, 0.000000000000000000, 11.86609696750642229 ) ) ;
#24655=PLANE ( 'NONE',  #15140 ) ;
#24656=LINE ( 'NONE', #30057, #12020 ) ;
#24657=ORIENTED_EDGE ( 'NONE', *, *, #26294, .F. ) ;
#24658=DIRECTION ( 'NONE',  ( 0.007781995580012662783, 0.000000000000000000, -0.9999697198139514409 ) ) ;
#24659=DIRECTION ( 'NONE',  ( -0.6427681459581293666, -0.7660444431189770143, -0.005002170337467561935 ) ) ;
#24660=ORIENTED_EDGE ( 'NONE', *, *, #22339, .F. ) ;
#24661=CARTESIAN_POINT ( 'NONE',  ( -20.54049170961573267, 0.000000000000000000, 4.660556269540326646 ) ) ;
#24662=CARTESIAN_POINT ( 'NONE',  ( -16.81345671998191449, 0.000000000000000000, 3.412238694616132495 ) ) ;
#24663=EDGE_CURVE ( 'NONE', #39497, #3767, #50311, .T. ) ;
#24664=VECTOR ( 'NONE', #15201, 1000.000000000000114 ) ;
#24665=VECTOR ( 'NONE', #45191, 999.9999999999998863 ) ;
#24666=EDGE_LOOP ( 'NONE', ( #4713, #48756, #11956, #4574 ) ) ;
#24667=ORIENTED_EDGE ( 'NONE', *, *, #33235, .T. ) ;
#24668=DIRECTION ( 'NONE',  ( -0.5449076811759708816, 0.6444004775717707689, 0.5364919789714475140 ) ) ;
#24669=EDGE_CURVE ( 'NONE', #23840, #8533, #54028, .T. ) ;
#24671=VECTOR ( 'NONE', #23764, 1000.000000000000227 ) ;
#24672=ORIENTED_EDGE ( 'NONE', *, *, #27842, .F. ) ;
#24673=ORIENTED_EDGE ( 'NONE', *, *, #5023, .T. ) ;
#24674=AXIS2_PLACEMENT_3D ( 'NONE', #23598, #44915, #10265 ) ;
#24675=ORIENTED_EDGE ( 'NONE', *, *, #23987, .F. ) ;
#24676=CARTESIAN_POINT ( 'NONE',  ( -15.60102546347950536, 0.000000000000000000, 12.95077420755565356 ) ) ;
#24677=FACE_OUTER_BOUND ( 'NONE', #4650, .T. ) ;
#24678=DIRECTION ( 'NONE',  ( 0.9999697198139515519, 0.000000000000000000, 0.007781995580013368816 ) ) ;
#24679=ADVANCED_FACE ( 'NONE', ( #41775 ), #6897, .F. ) ;
#24680=EDGE_LOOP ( 'NONE', ( #25550, #3943, #55828, #33444 ) ) ;
#24681=AXIS2_PLACEMENT_3D ( 'NONE', #40452, #28195, #5801 ) ;
#24682=ORIENTED_EDGE ( 'NONE', *, *, #19703, .F. ) ;
#24683=EDGE_CURVE ( 'NONE', #18658, #43254, #31882, .T. ) ;
#24684=CARTESIAN_POINT ( 'NONE',  ( -9.303843012252302813, 0.000000000000000000, 5.686672663758525204 ) ) ;
#24685=DIRECTION ( 'NONE',  ( -0.5364919789714478471, 0.6444004775717705469, -0.5449076811759709926 ) ) ;
#24687=FACE_OUTER_BOUND ( 'NONE', #30141, .T. ) ;
#24689=DIRECTION ( 'NONE',  ( -0.005961354470445682716, -0.6427876096865404731, 0.7660212471507180654 ) ) ;
#24690=CARTESIAN_POINT ( 'NONE',  ( -19.79569077582305070, 0.000000000000000000, 14.58012466630350445 ) ) ;
#24691=ADVANCED_FACE ( 'NONE', ( #14847 ), #40698, .F. ) ;
#24692=ORIENTED_EDGE ( 'NONE', *, *, #40521, .F. ) ;
#24693=FACE_OUTER_BOUND ( 'NONE', #45025, .T. ) ;
#24694=AXIS2_PLACEMENT_3D ( 'NONE', #22315, #10362, #5823 ) ;
#24695=EDGE_CURVE ( 'NONE', #23151, #52744, #12264, .T. ) ;
#24696=DIRECTION ( 'NONE',  ( -0.005002170337468016433, -0.7660444431189770143, 0.6427681459581293666 ) ) ;
#24697=ORIENTED_EDGE ( 'NONE', *, *, #22408, .T. ) ;
#24699=VECTOR ( 'NONE', #7492, 1000.000000000000000 ) ;
#24700=PLANE ( 'NONE',  #36473 ) ;
#24702=VECTOR ( 'NONE', #30348, 1000.000000000000114 ) ;
#24703=VECTOR ( 'NONE', #48474, 1000.000000000000114 ) ;
#24704=DIRECTION ( 'NONE',  ( 0.007781995580012663651, 0.000000000000000000, -0.9999697198139515519 ) ) ;
#24705=CARTESIAN_POINT ( 'NONE',  ( -28.93137873341882127, 0.000000000000000000, 8.119251130998824451 ) ) ;
#24706=DIRECTION ( 'NONE',  ( -0.6427681459581293666, -0.7660444431189770143, -0.005002170337467561935 ) ) ;
#24707=PLANE ( 'NONE',  #32271 ) ;
#24708=CARTESIAN_POINT ( 'NONE',  ( -28.93137873341882127, 0.000000000000000000, 8.119251130998824451 ) ) ;
#24709=DIRECTION ( 'NONE',  ( 0.007781995580012663651, -3.146120232559066537E-19, -0.9999697198139514409 ) ) ;
#24710=VECTOR ( 'NONE', #9045, 999.9999999999998863 ) ;
#24711=DIRECTION ( 'NONE',  ( 0.9999697198139515519, 0.000000000000000000, 0.007781995580013368816 ) ) ;
#24712=AXIS2_PLACEMENT_3D ( 'NONE', #25234, #3369, #21539 ) ;
#24713=ORIENTED_EDGE ( 'NONE', *, *, #3961, .F. ) ;
#24714=CARTESIAN_POINT ( 'NONE',  ( -21.47419595591918906, 0.000000000000000000, 5.222628093224860102 ) ) ;
#24715=LINE ( 'NONE', #11396, #41319 ) ;
#24717=EDGE_LOOP ( 'NONE', ( #40903, #21965, #1960, #50790 ) ) ;
#24718=CARTESIAN_POINT ( 'NONE',  ( -18.67619601524082285, 0.000000000000000000, 3.936400510096834893 ) ) ;
#24719=CARTESIAN_POINT ( 'NONE',  ( -26.13337879274045505, 0.000000000000000000, 6.833023547870798353 ) ) ;
#24720=CARTESIAN_POINT ( 'NONE',  ( -15.13495153988577968, 0.000000000000000000, 12.76973526769478084 ) ) ;
#24721=VECTOR ( 'NONE', #32356, 1000.000000000000227 ) ;
#24722=EDGE_CURVE ( 'NONE', #9919, #51258, #37534, .T. ) ;
#24723=AXIS2_PLACEMENT_3D ( 'NONE', #48665, #10864, #54032 ) ;
#24724=DIRECTION ( 'NONE',  ( -0.5449076811759708816, 0.6444004775717707689, 0.5364919789714475140 ) ) ;
#24727=EDGE_CURVE ( 'NONE', #23468, #18912, #4023, .T. ) ;
#24728=VERTEX_POINT ( 'NONE', #21043 ) ;
#24729=ADVANCED_FACE ( 'NONE', ( #34141 ), #29869, .F. ) ;
#24730=DIRECTION ( 'NONE',  ( 0.9999697198139515519, 0.000000000000000000, 0.007781995580013368816 ) ) ;
#24731=EDGE_CURVE ( 'NONE', #5706, #45380, #38677, .T. ) ;
#24732=VECTOR ( 'NONE', #2138, 1000.000000000000114 ) ;
#24733=EDGE_CURVE ( 'NONE', #3673, #22994, #21347, .T. ) ;
#24734=EDGE_CURVE ( 'NONE', #5052, #43426, #25057, .T. ) ;
#24736=ORIENTED_EDGE ( 'NONE', *, *, #8488, .F. ) ;
#24737=DIRECTION ( 'NONE',  ( 0.005002170337468016433, -0.7660444431189770143, -0.6427681459581293666 ) ) ;
#24738=AXIS2_PLACEMENT_3D ( 'NONE', #46045, #44934, #19910 ) ;
#24739=VERTEX_POINT ( 'NONE', #33835 ) ;
#24740=LINE ( 'NONE', #46054, #9346 ) ;
#24741=ORIENTED_EDGE ( 'NONE', *, *, #35662, .T. ) ;
#24742=ORIENTED_EDGE ( 'NONE', *, *, #5545, .F. ) ;
#24743=ORIENTED_EDGE ( 'NONE', *, *, #52743, .T. ) ;
#24744=CARTESIAN_POINT ( 'NONE',  ( -14.93495759592298988, 0.000000000000000000, 12.77129166681078409 ) ) ;
#24745=VECTOR ( 'NONE', #20498, 1000.000000000000227 ) ;
#24746=PLANE ( 'NONE',  #23244 ) ;
#24747=DIRECTION ( 'NONE',  ( -0.5364919789714478471, 0.6444004775717705469, -0.5449076811759709926 ) ) ;
#24748=AXIS2_PLACEMENT_3D ( 'NONE', #46211, #41130, #55048 ) ;
#24749=VECTOR ( 'NONE', #42877, 1000.000000000000227 ) ;
#24750=CARTESIAN_POINT ( 'NONE',  ( -12.33850799832341849, 0.000000000000000000, 11.68350162852954632 ) ) ;
#24751=EDGE_CURVE ( 'NONE', #20238, #31826, #29604, .T. ) ;
#24752=ORIENTED_EDGE ( 'NONE', *, *, #1067, .T. ) ;
#24753=EDGE_CURVE ( 'NONE', #28378, #54423, #17091, .T. ) ;
#24754=EDGE_LOOP ( 'NONE', ( #52083, #16961, #45478, #25216 ) ) ;
#24755=VECTOR ( 'NONE', #38442, 999.9999999999998863 ) ;
#24756=VERTEX_POINT ( 'NONE', #12555 ) ;
#24757=LINE ( 'NONE', #3180, #46736 ) ;
#24758=VECTOR ( 'NONE', #13690, 999.9999999999998863 ) ;
#24760=CARTESIAN_POINT ( 'NONE',  ( -22.40634380310664397, 0.000000000000000000, 5.584705972946605534 ) ) ;
#24761=ADVANCED_FACE ( 'NONE', ( #43226 ), #47166, .F. ) ;
#24762=ORIENTED_EDGE ( 'NONE', *, *, #29334, .T. ) ;
#24763=FACE_BOUND ( 'NONE', #50540, .T. ) ;
#24764=EDGE_LOOP ( 'NONE', ( #40469, #24856, #16054, #21197 ) ) ;
#24766=DIRECTION ( 'NONE',  ( 0.007781995580012662783, 0.000000000000000000, -0.9999697198139514409 ) ) ;
#24767=EDGE_CURVE ( 'NONE', #33148, #28250, #51708, .T. ) ;
#24768=VERTEX_POINT ( 'NONE', #37836 ) ;
#24769=CARTESIAN_POINT ( 'NONE',  ( 2.072287782118878319, 0.000000000000000000, -2.950529333540147015 ) ) ;
#24770=AXIS2_PLACEMENT_3D ( 'NONE', #5103, #27221, #52766 ) ;
#24771=ORIENTED_EDGE ( 'NONE', *, *, #9383, .F. ) ;
#24772=VECTOR ( 'NONE', #15814, 1000.000000000000227 ) ;
#24773=CARTESIAN_POINT ( 'NONE',  ( -14.20280369269832832, 0.000000000000000000, 12.40765738797303719 ) ) ;
#24774=DIRECTION ( 'NONE',  ( -0.8531650599175527594, 0.4028455766673922356, 0.3313982828793700652 ) ) ;
#24775=LINE ( 'NONE', #42090, #12372 ) ;
#24776=FACE_OUTER_BOUND ( 'NONE', #37619, .T. ) ;
#24777=CARTESIAN_POINT ( 'NONE',  ( -19.71756863920010616, -1.327505506330655782, 6.519567697922603600 ) ) ;
#24778=DIRECTION ( 'NONE',  ( 0.005961354470445682716, -0.6427876096865404731, -0.7660212471507180654 ) ) ;
#24779=VERTEX_POINT ( 'NONE', #16234 ) ;
#24780=VECTOR ( 'NONE', #51797, 999.9999999999998863 ) ;
#24781=VERTEX_POINT ( 'NONE', #8272 ) ;
#24783=PLANE ( 'NONE',  #52959 ) ;
#24784=VECTOR ( 'NONE', #52050, 1000.000000000000227 ) ;
#24785=CARTESIAN_POINT ( 'NONE',  ( -18.80686481966623802, -4.079838673713161334, 10.68286703394162629 ) ) ;
#24786=DIRECTION ( 'NONE',  ( 0.007781995580012662783, 0.000000000000000000, -0.9999697198139514409 ) ) ;
#24787=DIRECTION ( 'NONE',  ( 0.000000000000000000, -0.000000000000000000, -1.000000000000000000 ) ) ;
#24788=CARTESIAN_POINT ( 'NONE',  ( -10.47421230394850866, 0.000000000000000000, 10.95934586908605723 ) ) ;
#24789=ORIENTED_EDGE ( 'NONE', *, *, #45270, .T. ) ;
#24790=CARTESIAN_POINT ( 'NONE',  ( -16.00432305936900690, 0.000000000000000000, 5.065189852669833570 ) ) ;
#24791=LINE ( 'NONE', #9150, #8723 ) ;
#24792=ORIENTED_EDGE ( 'NONE', *, *, #17873, .F. ) ;
#24793=AXIS2_PLACEMENT_3D ( 'NONE', #26571, #43892, #14378 ) ;
#24794=CARTESIAN_POINT ( 'NONE',  ( -11.77243710274829525, -0.1191753592594197858, 11.50324088822667612 ) ) ;
#24795=EDGE_LOOP ( 'NONE', ( #2277, #53105, #34463, #9999, #2936 ) ) ;
#24796=VECTOR ( 'NONE', #30740, 1000.000000000000000 ) ;
#24798=CARTESIAN_POINT ( 'NONE',  ( -16.81267852042391198, -0.1191753592594197858, 3.312241722634738039 ) ) ;
#24799=CARTESIAN_POINT ( 'NONE',  ( -14.20280369269832832, 0.000000000000000000, 12.40765738797303719 ) ) ;
#24800=EDGE_CURVE ( 'NONE', #41133, #43762, #33301, .T. ) ;
#24801=DIRECTION ( 'NONE',  ( 0.5449076811759707706, 0.6444004775717708799, -0.5364919789714476250 ) ) ;
#24802=CARTESIAN_POINT ( 'NONE',  ( 2.072287782118878319, 0.000000000000000000, -2.950529333540147015 ) ) ;
#24804=ORIENTED_EDGE ( 'NONE', *, *, #20620, .F. ) ;
#24805=VECTOR ( 'NONE', #38947, 1000.000000000000227 ) ;
#24806=EDGE_CURVE ( 'NONE', #9324, #55008, #8567, .T. ) ;
#24807=VECTOR ( 'NONE', #9034, 1000.000000000000227 ) ;
#24808=ORIENTED_EDGE ( 'NONE', *, *, #4604, .T. ) ;
#24809=LINE ( 'NONE', #29355, #29434 ) ;
#24810=DIRECTION ( 'NONE',  ( 0.005961354470445682716, -0.6427876096865404731, -0.7660212471507180654 ) ) ;
#24811=LINE ( 'NONE', #6959, #45116 ) ;
#24812=ADVANCED_FACE ( 'NONE', ( #15964 ), #20777, .F. ) ;
#24813=EDGE_CURVE ( 'NONE', #27552, #25905, #29017, .T. ) ;
#24814=EDGE_CURVE ( 'NONE', #10480, #7041, #11959, .T. ) ;
#24815=CARTESIAN_POINT ( 'NONE',  ( -16.79925329029790149, 0.000000000000000000, 13.49544742625427496 ) ) ;
#24816=FACE_OUTER_BOUND ( 'NONE', #48324, .T. ) ;
#24817=LINE ( 'NONE', #33063, #9488 ) ;
#24818=ORIENTED_EDGE ( 'NONE', *, *, #46781, .T. ) ;
#24819=EDGE_CURVE ( 'NONE', #23263, #53826, #16806, .T. ) ;
#24820=DIRECTION ( 'NONE',  ( -0.5449076811759708816, 0.6444004775717707689, 0.5364919789714475140 ) ) ;
#24821=DIRECTION ( 'NONE',  ( -0.9999697198139514409, -0.000000000000000000, -0.007781995580013368816 ) ) ;
#24822=CARTESIAN_POINT ( 'NONE',  ( -14.01623497886158454, -0.1191753592594203132, 2.226008083469503518 ) ) ;
#24823=ORIENTED_EDGE ( 'NONE', *, *, #22475, .F. ) ;
#24824=VECTOR ( 'NONE', #56076, 999.9999999999998863 ) ;
#24825=CARTESIAN_POINT ( 'NONE',  ( -12.26291780220878103, 0.000000000000000000, 1.970323761456820755 ) ) ;
#24827=AXIS2_PLACEMENT_3D ( 'NONE', #56153, #4208, #26600 ) ;
#24828=DIRECTION ( 'NONE',  ( -0.005961354470445682716, -0.6427876096865404731, 0.7660212471507180654 ) ) ;
#24829=ORIENTED_EDGE ( 'NONE', *, *, #27536, .T. ) ;
#24830=DIRECTION ( 'NONE',  ( 0.005002170337468016433, -0.7660444431189770143, -0.6427681459581293666 ) ) ;
#24831=AXIS2_PLACEMENT_3D ( 'NONE', #9871, #22912, #45597 ) ;
#24832=EDGE_LOOP ( 'NONE', ( #47253, #10092, #8623, #15961 ) ) ;
#24834=VERTEX_POINT ( 'NONE', #13932 ) ;
#24835=EDGE_LOOP ( 'NONE', ( #32272, #5929, #40203, #13945 ) ) ;
#24836=ADVANCED_FACE ( 'NONE', ( #18472 ), #13405, .F. ) ;
#24837=ORIENTED_EDGE ( 'NONE', *, *, #15351, .F. ) ;
#24838=VECTOR ( 'NONE', #3173, 1000.000000000000227 ) ;
#24839=CARTESIAN_POINT ( 'NONE',  ( -17.95536891708715999, -0.3560938001956550081, 4.240817377596695970 ) ) ;
#24840=ORIENTED_EDGE ( 'NONE', *, *, #34617, .F. ) ;
#24841=VECTOR ( 'NONE', #6231, 1000.000000000000227 ) ;
#24842=EDGE_CURVE ( 'NONE', #55136, #26740, #30718, .T. ) ;
#24843=ORIENTED_EDGE ( 'NONE', *, *, #33495, .T. ) ;
#24845=ORIENTED_EDGE ( 'NONE', *, *, #11083, .T. ) ;
#24846=ORIENTED_EDGE ( 'NONE', *, *, #6264, .T. ) ;
#24848=VECTOR ( 'NONE', #49934, 1000.000000000000114 ) ;
#24849=AXIS2_PLACEMENT_3D ( 'NONE', #49255, #10669, #19428 ) ;
#24850=CARTESIAN_POINT ( 'NONE',  ( -16.75946939063593177, 0.000000000000000000, 8.383301757569700641 ) ) ;
#24851=CARTESIAN_POINT ( 'NONE',  ( -15.63164134753341372, -4.727446477803162850, 10.51233714212408543 ) ) ;
#24852=DIRECTION ( 'NONE',  ( 0.007781995580012662783, 0.000000000000000000, -0.9999697198139514409 ) ) ;
#24853=DIRECTION ( 'NONE',  ( -0.5364919789714478471, 0.6444004775717705469, -0.5449076811759709926 ) ) ;
#24854=CARTESIAN_POINT ( 'NONE',  ( -13.92721955262090106, 0.000000000000000000, 2.696035920016314424 ) ) ;
#24855=ORIENTED_EDGE ( 'NONE', *, *, #1417, .T. ) ;
#24856=ORIENTED_EDGE ( 'NONE', *, *, #55021, .T. ) ;
#24857=FACE_OUTER_BOUND ( 'NONE', #41915, .T. ) ;
#24858=CARTESIAN_POINT ( 'NONE',  ( -6.086429055005921462, -7.947879803594625869, 5.582549316628845126 ) ) ;
#24859=DIRECTION ( 'NONE',  ( 0.9999697198139515519, 0.000000000000000000, 0.007781995580013368816 ) ) ;
#24861=FACE_OUTER_BOUND ( 'NONE', #592, .T. ) ;
#24864=DIRECTION ( 'NONE',  ( -0.6427681459581293666, -0.7660444431189770143, -0.005002170337467561935 ) ) ;
#24865=ORIENTED_EDGE ( 'NONE', *, *, #19761, .F. ) ;
#24866=DIRECTION ( 'NONE',  ( -0.7660212471507179544, -0.6427876096865405842, -0.005961354470445141482 ) ) ;
#24867=LINE ( 'NONE', #25171, #25848 ) ;
#24868=VECTOR ( 'NONE', #5806, 1000.000000000000114 ) ;
#24869=EDGE_LOOP ( 'NONE', ( #6046, #7510, #47309 ) ) ;
#24870=DIRECTION ( 'NONE',  ( 0.9999697198139515519, 0.000000000000000000, 0.007781995580013368816 ) ) ;
#24871=FACE_OUTER_BOUND ( 'NONE', #37740, .T. ) ;
#24872=DIRECTION ( 'NONE',  ( -0.005002170337468016433, -0.7660444431189770143, 0.6427681459581293666 ) ) ;
#24874=DIRECTION ( 'NONE',  ( 0.9999697198139515519, 0.000000000000000000, 0.007781995580013368816 ) ) ;
#24875=CARTESIAN_POINT ( 'NONE',  ( -17.73140113748535285, 0.000000000000000000, 13.85752530597602039 ) ) ;
#24876=ORIENTED_EDGE ( 'NONE', *, *, #51818, .T. ) ;
#24877=ORIENTED_EDGE ( 'NONE', *, *, #30823, .F. ) ;
#24878=AXIS2_PLACEMENT_3D ( 'NONE', #541, #49066, #14708 ) ;
#24879=LINE ( 'NONE', #33668, #11266 ) ;
#24880=LINE ( 'NONE', #3311, #48531 ) ;
#24881=CARTESIAN_POINT ( 'NONE',  ( -14.49394927539066025, -0.1191753592594189670, 2.960954539966670573 ) ) ;
#24882=VECTOR ( 'NONE', #28915, 1000.000000000000227 ) ;
#24883=ADVANCED_FACE ( 'NONE', ( #22182 ), #1137, .F. ) ;
#24885=CARTESIAN_POINT ( 'NONE',  ( 2.072287782118878319, 0.000000000000000000, -2.950529333540147015 ) ) ;
#24886=CARTESIAN_POINT ( 'NONE',  ( -22.36894862246310822, -5.051250379848164052, 5.409019081522692396 ) ) ;
#24887=EDGE_CURVE ( 'NONE', #35148, #23097, #22482, .T. ) ;
#24889=EDGE_CURVE ( 'NONE', #9162, #28180, #39517, .T. ) ;
#24890=LINE ( 'NONE', #37954, #10211 ) ;
#24891=VECTOR ( 'NONE', #16155, 999.9999999999998863 ) ;
#24892=DIRECTION ( 'NONE',  ( 0.5364919789714477361, 0.6444004775717706579, 0.5449076811759711036 ) ) ;
#24893=VECTOR ( 'NONE', #48647, 1000.000000000000227 ) ;
#24894=LINE ( 'NONE', #736, #639 ) ;
#24896=CARTESIAN_POINT ( 'NONE',  ( -22.40478740399063895, 0.000000000000000000, 5.384712028983816623 ) ) ;
#24897=ORIENTED_EDGE ( 'NONE', *, *, #30439, .F. ) ;
#24898=DIRECTION ( 'NONE',  ( -0.6427681459581293666, -0.7660444431189770143, -0.005002170337467561935 ) ) ;
#24899=ORIENTED_EDGE ( 'NONE', *, *, #12784, .T. ) ;
#24900=AXIS2_PLACEMENT_3D ( 'NONE', #53924, #32899, #50216 ) ;
#24901=VERTEX_POINT ( 'NONE', #35261 ) ;
#24902=VERTEX_POINT ( 'NONE', #30965 ) ;
#24903=EDGE_LOOP ( 'NONE', ( #38453, #9969, #24393, #28117 ) ) ;
#24904=VECTOR ( 'NONE', #49437, 999.9999999999998863 ) ;
#24905=ORIENTED_EDGE ( 'NONE', *, *, #37641, .F. ) ;
#24906=CARTESIAN_POINT ( 'NONE',  ( -17.46532115785441519, 0.000000000000000000, 13.67492996699914265 ) ) ;
#24907=LINE ( 'NONE', #24604, #36577 ) ;
#24908=CARTESIAN_POINT ( 'NONE',  ( -7.159975159455704841, 6.987782224127484731, 5.999551081376306882 ) ) ;
#24909=VECTOR ( 'NONE', #55111, 1000.000000000000114 ) ;
#24910=ORIENTED_EDGE ( 'NONE', *, *, #20660, .F. ) ;
#24912=EDGE_LOOP ( 'NONE', ( #24151, #2353, #32770, #56092 ) ) ;
#24913=VECTOR ( 'NONE', #17955, 999.9999999999998863 ) ;
#24915=VERTEX_POINT ( 'NONE', #26427 ) ;
#24916=ADVANCED_FACE ( 'NONE', ( #48587 ), #44585, .F. ) ;
#24917=VECTOR ( 'NONE', #12587, 1000.000000000000227 ) ;
#24919=EDGE_CURVE ( 'NONE', #14383, #40367, #27014, .T. ) ;
#24920=VECTOR ( 'NONE', #29876, 999.9999999999998863 ) ;
#24921=FACE_OUTER_BOUND ( 'NONE', #41096, .T. ) ;
#24922=CARTESIAN_POINT ( 'NONE',  ( -19.45503627000849889, -1.000000000000000000, 7.556996783084074742 ) ) ;
#24923=ORIENTED_EDGE ( 'NONE', *, *, #2728, .T. ) ;
#24924=FACE_OUTER_BOUND ( 'NONE', #28308, .T. ) ;
#24925=ORIENTED_EDGE ( 'NONE', *, *, #53471, .T. ) ;
#24926=AXIS2_PLACEMENT_3D ( 'NONE', #53378, #26984, #10201 ) ;
#24927=FACE_OUTER_BOUND ( 'NONE', #6462, .T. ) ;
#24928=EDGE_CURVE ( 'NONE', #17689, #25841, #4858, .T. ) ;
#24929=CARTESIAN_POINT ( 'NONE',  ( -13.67119876025844860, 0.000000000000000000, 3.806024542441613701 ) ) ;
#24930=VECTOR ( 'NONE', #19147, 1000.000000000000000 ) ;
#24931=DIRECTION ( 'NONE',  ( -0.5449076811759708816, 0.6444004775717707689, 0.5364919789714475140 ) ) ;
#24932=VECTOR ( 'NONE', #52096, 1000.000000000000114 ) ;
#24933=LINE ( 'NONE', #51030, #32224 ) ;
#24936=LINE ( 'NONE', #15843, #20284 ) ;
#24937=DIRECTION ( 'NONE',  ( -0.6246952433987893460, -0.7422098413412802076, 0.2426528472758542054 ) ) ;
#24938=ORIENTED_EDGE ( 'NONE', *, *, #365, .F. ) ;
#24939=LINE ( 'NONE', #3366, #54657 ) ;
#24940=VERTEX_POINT ( 'NONE', #21891 ) ;
#24941=LINE ( 'NONE', #42263, #23829 ) ;
#24942=CARTESIAN_POINT ( 'NONE',  ( -11.36984871579436174, -0.8417996532631562001, 1.270898663839582943 ) ) ;
#24943=FACE_OUTER_BOUND ( 'NONE', #17099, .T. ) ;
#24944=CARTESIAN_POINT ( 'NONE',  ( -11.78272344325496945, 1.095915999411504194, 1.223776201692182930 ) ) ;
#24945=CARTESIAN_POINT ( 'NONE',  ( -9.977096013572023026, 0.000000000000000000, 6.789429462647804669 ) ) ;
#24947=LINE ( 'NONE', #50515, #23902 ) ;
#24948=VECTOR ( 'NONE', #34839, 999.9999999999998863 ) ;
#24949=ORIENTED_EDGE ( 'NONE', *, *, #2442, .F. ) ;
#24950=DIRECTION ( 'NONE',  ( -0.7660212471507179544, -0.6427876096865405842, -0.005961354470445141482 ) ) ;
#24952=CARTESIAN_POINT ( 'NONE',  ( -11.33939211553717286, 0.000000000000000000, 2.716174991508366610 ) ) ;
#24953=ADVANCED_FACE ( 'NONE', ( #4578 ), #39791, .F. ) ;
#24954=DIRECTION ( 'NONE',  ( 0.005002170337468016433, -0.7660444431189770143, -0.6427681459581293666 ) ) ;
#24955=VECTOR ( 'NONE', #14470, 1000.000000000000114 ) ;
#24956=DIRECTION ( 'NONE',  ( -0.5449076811759708816, 0.6444004775717707689, 0.5364919789714475140 ) ) ;
#24957=VECTOR ( 'NONE', #48770, 999.9999999999998863 ) ;
#24958=CARTESIAN_POINT ( 'NONE',  ( -26.13337879274045505, 0.000000000000000000, 6.833023547870798353 ) ) ;
#24959=DIRECTION ( 'NONE',  ( 0.9999697198139515519, 0.000000000000000000, 0.007781995580013368816 ) ) ;
#24960=EDGE_CURVE ( 'NONE', #873, #44414, #44324, .T. ) ;
#24961=ORIENTED_EDGE ( 'NONE', *, *, #39238, .F. ) ;
#24962=LINE ( 'NONE', #45684, #399 ) ;
#24964=CARTESIAN_POINT ( 'NONE',  ( -18.36790206993104846, -4.727446477803164626, 3.865207764181160854 ) ) ;
#24965=VECTOR ( 'NONE', #20364, 1000.000000000000227 ) ;
#24966=ORIENTED_EDGE ( 'NONE', *, *, #23973, .F. ) ;
#24967=VECTOR ( 'NONE', #402, 1000.000000000000227 ) ;
#24968=EDGE_LOOP ( 'NONE', ( #43230, #30759, #5012, #25815 ) ) ;
#24969=LINE ( 'NONE', #29801, #12887 ) ;
#24970=AXIS2_PLACEMENT_3D ( 'NONE', #16701, #38269, #46810 ) ;
#24971=ORIENTED_EDGE ( 'NONE', *, *, #20747, .T. ) ;
#24974=CARTESIAN_POINT ( 'NONE',  ( -17.17779978478095515, -1.651309408375659871, 3.501076498445555352 ) ) ;
#24975=ADVANCED_FACE ( 'NONE', ( #16 ), #17345, .F. ) ;
#24976=AXIS2_PLACEMENT_3D ( 'NONE', #1701, #32642, #49119 ) ;
#24977=EDGE_LOOP ( 'NONE', ( #14915, #6669, #52934 ) ) ;
#24978=VECTOR ( 'NONE', #41285, 1000.000000000000227 ) ;
#24979=EDGE_LOOP ( 'NONE', ( #28851, #53960, #32913, #1157 ) ) ;
#24980=EDGE_LOOP ( 'NONE', ( #15153, #15267, #36342, #24169, #29397 ) ) ;
#24981=CARTESIAN_POINT ( 'NONE',  ( -14.16170213864708138, 0.000000000000000000, 7.126195959993483875 ) ) ;
#24982=PLANE ( 'NONE',  #54974 ) ;
#24983=PLANE ( 'NONE',  #33070 ) ;
#24984=EDGE_LOOP ( 'NONE', ( #31973, #11510, #54569, #53229, #16281 ) ) ;
#24986=AXIS2_PLACEMENT_3D ( 'NONE', #54840, #50591, #50296 ) ;
#24987=CARTESIAN_POINT ( 'NONE',  ( -25.20123094555300369, 0.000000000000000000, 6.470945668149052032 ) ) ;
#24988=LINE ( 'NONE', #42313, #53581 ) ;
#24989=VECTOR ( 'NONE', #18770, 1000.000000000000114 ) ;
#24990=ORIENTED_EDGE ( 'NONE', *, *, #50480, .T. ) ;
#24991=FACE_OUTER_BOUND ( 'NONE', #53687, .T. ) ;
#24992=ORIENTED_EDGE ( 'NONE', *, *, #5881, .F. ) ;
#24993=VECTOR ( 'NONE', #44481, 1000.000000000000227 ) ;
#24994=DIRECTION ( 'NONE',  ( -0.5449076811759708816, 0.6444004775717707689, 0.5364919789714475140 ) ) ;
#24995=LINE ( 'NONE', #3414, #4835 ) ;
#24996=EDGE_LOOP ( 'NONE', ( #45535, #18075, #48913, #47451 ) ) ;
#24997=DIRECTION ( 'NONE',  ( -0.005961354470445682716, -0.6427876096865404731, 0.7660212471507180654 ) ) ;
#24998=EDGE_CURVE ( 'NONE', #13188, #6357, #13107, .T. ) ;
#24999=VECTOR ( 'NONE', #16765, 1000.000000000000227 ) ;
#25000=CARTESIAN_POINT ( 'NONE',  ( -23.33693525117809386, 0.000000000000000000, 5.746789908705562944 ) ) ;
#25001=AXIS2_PLACEMENT_3D ( 'NONE', #50621, #38107, #2624 ) ;
#25002=AXIS2_PLACEMENT_3D ( 'NONE', #20215, #54564, #49781 ) ;
#25003=ORIENTED_EDGE ( 'NONE', *, *, #31474, .T. ) ;
#25004=CARTESIAN_POINT ( 'NONE',  ( -14.94760462649100496, 0.000000000000000000, 2.488088991209854051 ) ) ;
#25005=LINE ( 'NONE', #43438, #51967 ) ;
#25006=CARTESIAN_POINT ( 'NONE',  ( -18.91281239749552867, -5.375054281893166142, 4.056207361090260477 ) ) ;
#25007=FACE_OUTER_BOUND ( 'NONE', #44463, .T. ) ;
#25008=ORIENTED_EDGE ( 'NONE', *, *, #34926, .F. ) ;
#25009=AXIS2_PLACEMENT_3D ( 'NONE', #10069, #9521, #26274 ) ;
#25010=EDGE_CURVE ( 'NONE', #32117, #22899, #17642, .T. ) ;
#25011=AXIS2_PLACEMENT_3D ( 'NONE', #1658, #30911, #18983 ) ;
#25012=DIRECTION ( 'NONE',  ( 0.007781995580012663651, -3.146120232559066537E-19, -0.9999697198139514409 ) ) ;
#25013=LINE ( 'NONE', #42595, #19639 ) ;
#25014=FACE_OUTER_BOUND ( 'NONE', #10992, .T. ) ;
#25015=AXIS2_PLACEMENT_3D ( 'NONE', #14433, #39718, #36031 ) ;
#25016=DIRECTION ( 'NONE',  ( 0.007781995580012663651, -3.146120232559066537E-19, -0.9999697198139514409 ) ) ;
#25017=EDGE_CURVE ( 'NONE', #22830, #36235, #18784, .T. ) ;
#25018=CARTESIAN_POINT ( 'NONE',  ( -23.33849165029409889, 0.000000000000000000, 5.946783852668351855 ) ) ;
#25019=DIRECTION ( 'NONE',  ( 0.9999697198139515519, 0.000000000000000000, 0.007781995580013368816 ) ) ;
#25021=VECTOR ( 'NONE', #38512, 1000.000000000000227 ) ;
#25022=AXIS2_PLACEMENT_3D ( 'NONE', #31160, #8773, #25789 ) ;
#25024=ORIENTED_EDGE ( 'NONE', *, *, #2240, .F. ) ;
#25025=DIRECTION ( 'NONE',  ( 0.005002170337468016433, -0.7660444431189770143, -0.6427681459581293666 ) ) ;
#25026=CARTESIAN_POINT ( 'NONE',  ( 2.072287782118878319, 0.000000000000000000, -2.950529333540147015 ) ) ;
#25027=ORIENTED_EDGE ( 'NONE', *, *, #36360, .T. ) ;
#25028=DIRECTION ( 'NONE',  ( 0.005961354470445682716, -0.6427876096865404731, -0.7660212471507180654 ) ) ;
#25029=ADVANCED_FACE ( 'NONE', ( #45174 ), #10238, .F. ) ;
#25030=CARTESIAN_POINT ( 'NONE',  ( -12.02422819173196089, 1.905425754524007198, 4.679067971174708518 ) ) ;
#25031=ADVANCED_FACE ( 'NONE', ( #2269 ), #40892, .F. ) ;
#25032=DIRECTION ( 'NONE',  ( 0.005961354470445682716, -0.6427876096865404731, -0.7660212471507180654 ) ) ;
#25033=PLANE ( 'NONE',  #51410 ) ;
#25034=EDGE_CURVE ( 'NONE', #40075, #21894, #10543, .T. ) ;
#25035=DIRECTION ( 'NONE',  ( -0.7660212471507179544, -0.6427876096865405842, -0.005961354470445141482 ) ) ;
#25036=AXIS2_PLACEMENT_3D ( 'NONE', #43352, #14084, #31413 ) ;
#25037=EDGE_LOOP ( 'NONE', ( #48946, #12856, #17232, #17565 ) ) ;
#25038=EDGE_LOOP ( 'NONE', ( #4163, #25927, #41843, #35258 ) ) ;
#25039=LINE ( 'NONE', #37232, #54943 ) ;
#25040=CARTESIAN_POINT ( 'NONE',  ( -13.66427238189300830, -2.460819163488160655, 2.110475535834075433 ) ) ;
#25041=VECTOR ( 'NONE', #9511, 1000.000000000000227 ) ;
#25042=DIRECTION ( 'NONE',  ( 0.9999697198139515519, 0.000000000000000000, 0.007781995580013368816 ) ) ;
#25043=EDGE_CURVE ( 'NONE', #23769, #16052, #53667, .T. ) ;
#25044=VERTEX_POINT ( 'NONE', #54238 ) ;
#25045=FACE_OUTER_BOUND ( 'NONE', #2923, .T. ) ;
#25046=VECTOR ( 'NONE', #28081, 1000.000000000000227 ) ;
#25047=EDGE_LOOP ( 'NONE', ( #27895, #2678, #27302, #7364, #47310 ) ) ;
#25048=DIRECTION ( 'NONE',  ( 0.007781995580012663651, -3.146120232559066537E-19, -0.9999697198139514409 ) ) ;
#25049=ADVANCED_FACE ( 'NONE', ( #1970 ), #31818, .F. ) ;
#25050=AXIS2_PLACEMENT_3D ( 'NONE', #49384, #23280, #31787 ) ;
#25051=AXIS2_PLACEMENT_3D ( 'NONE', #51179, #51731, #55428 ) ;
#25052=ORIENTED_EDGE ( 'NONE', *, *, #27459, .T. ) ;
#25053=ORIENTED_EDGE ( 'NONE', *, *, #17379, .F. ) ;
#25054=ORIENTED_EDGE ( 'NONE', *, *, #32580, .F. ) ;
#25055=PLANE ( 'NONE',  #52894 ) ;
#25056=FACE_OUTER_BOUND ( 'NONE', #19721, .T. ) ;
#25057=LINE ( 'NONE', #55697, #28478 ) ;
#25058=AXIS2_PLACEMENT_3D ( 'NONE', #7834, #2437, #42461 ) ;
#25059=VECTOR ( 'NONE', #39097, 1000.000000000000000 ) ;
#25061=ORIENTED_EDGE ( 'NONE', *, *, #11613, .F. ) ;
#25062=AXIS2_PLACEMENT_3D ( 'NONE', #17938, #12815, #18471 ) ;
#25063=ORIENTED_EDGE ( 'NONE', *, *, #50599, .F. ) ;
#25064=VECTOR ( 'NONE', #47808, 1000.000000000000227 ) ;
#25065=EDGE_LOOP ( 'NONE', ( #37265, #54946, #14169, #26731 ) ) ;
#25066=DIRECTION ( 'NONE',  ( 0.6427681459581294776, -0.7660444431189769032, 0.005002170337467562802 ) ) ;
#25067=DIRECTION ( 'NONE',  ( -0.005002170337468016433, -0.7660444431189770143, 0.6427681459581293666 ) ) ;
#25068=ORIENTED_EDGE ( 'NONE', *, *, #52470, .F. ) ;
#25069=FACE_OUTER_BOUND ( 'NONE', #26858, .T. ) ;
#25070=ORIENTED_EDGE ( 'NONE', *, *, #7853, .F. ) ;
#25071=DIRECTION ( 'NONE',  ( 0.6427681459581294776, -0.7660444431189769032, 0.005002170337467562802 ) ) ;
#25072=CARTESIAN_POINT ( 'NONE',  ( -1.300095020133916979, 4.816411402586080470, 3.723374632896542025 ) ) ;
#25073=ORIENTED_EDGE ( 'NONE', *, *, #48608, .T. ) ;
#25074=DIRECTION ( 'NONE',  ( 0.000000000000000000, -0.000000000000000000, -1.000000000000000000 ) ) ;
#25075=EDGE_CURVE ( 'NONE', #30608, #20261, #41470, .T. ) ;
#25076=ORIENTED_EDGE ( 'NONE', *, *, #44256, .F. ) ;
#25077=VECTOR ( 'NONE', #5840, 1000.000000000000227 ) ;
#25078=DIRECTION ( 'NONE',  ( -0.5449076811759708816, 0.6444004775717707689, 0.5364919789714475140 ) ) ;
#25079=CARTESIAN_POINT ( 'NONE',  ( -14.44189180272386430, 2.553033558614007603, 6.681005357687642032 ) ) ;
#25080=ORIENTED_EDGE ( 'NONE', *, *, #42982, .F. ) ;
#25082=LINE ( 'NONE', #34168, #53822 ) ;
#25083=LINE ( 'NONE', #560, #34143 ) ;
#25086=ORIENTED_EDGE ( 'NONE', *, *, #56086, .F. ) ;
#25087=ADVANCED_FACE ( 'NONE', ( #15593 ), #27557, .F. ) ;
#25088=ADVANCED_FACE ( 'NONE', ( #49708 ), #23575, .F. ) ;
#25089=EDGE_LOOP ( 'NONE', ( #24217, #16231, #2798, #53132 ) ) ;
#25091=VECTOR ( 'NONE', #25510, 1000.000000000000227 ) ;
#25092=LINE ( 'NONE', #46644, #20316 ) ;
#25093=DIRECTION ( 'NONE',  ( -0.6246952433987894571, 0.7422098413412802076, 0.2426528472758539834 ) ) ;
#25094=CARTESIAN_POINT ( 'NONE',  ( -27.99767448711536133, 0.000000000000000000, 7.557179307314289218 ) ) ;
#25095=DIRECTION ( 'NONE',  ( -0.7660212471507179544, -0.6427876096865405842, -0.005961354470445141482 ) ) ;
#25096=EDGE_CURVE ( 'NONE', #17177, #940, #36645, .T. ) ;
#25097=VECTOR ( 'NONE', #7923, 999.9999999999998863 ) ;
#25098=PLANE ( 'NONE',  #50323 ) ;
#25099=ORIENTED_EDGE ( 'NONE', *, *, #1559, .F. ) ;
#25100=DIRECTION ( 'NONE',  ( 0.007781995580012663651, -3.146120232559066537E-19, -0.9999697198139514409 ) ) ;
#25101=DIRECTION ( 'NONE',  ( 0.7660212471507180654, -0.6427876096865404731, 0.005961354470445141482 ) ) ;
#25102=VERTEX_POINT ( 'NONE', #44881 ) ;
#25103=CARTESIAN_POINT ( 'NONE',  ( -19.17512305244570214, 4.819660872929010687, 12.23947469159592494 ) ) ;
#25104=ORIENTED_EDGE ( 'NONE', *, *, #20659, .T. ) ;
#25105=CARTESIAN_POINT ( 'NONE',  ( -27.06708303904391144, 0.000000000000000000, 7.395095371555332697 ) ) ;
#25106=CARTESIAN_POINT ( 'NONE',  ( -19.60912206198628027, -0.1191753592594197858, 4.398475361799976113 ) ) ;
#25107=AXIS2_PLACEMENT_3D ( 'NONE', #50040, #11152, #11455 ) ;
#25108=EDGE_CURVE ( 'NONE', #9654, #17188, #28688, .T. ) ;
#25109=PLANE ( 'NONE',  #41353 ) ;
#25110=CARTESIAN_POINT ( 'NONE',  ( 2.072287782118878319, 0.000000000000000000, -2.950529333540147015 ) ) ;
#25111=VECTOR ( 'NONE', #16659, 1000.000000000000227 ) ;
#25112=ADVANCED_FACE ( 'NONE', ( #36104 ), #23844, .F. ) ;
#25115=VECTOR ( 'NONE', #28666, 999.9999999999998863 ) ;
#25116=VERTEX_POINT ( 'NONE', #53958 ) ;
#25117=DIRECTION ( 'NONE',  ( -0.5364919789714478471, 0.6444004775717705469, -0.5449076811759709926 ) ) ;
#25118=LINE ( 'NONE', #38143, #53961 ) ;
#25119=DIRECTION ( 'NONE',  ( 0.007781995580012662783, 0.000000000000000000, -0.9999697198139514409 ) ) ;
#25120=LINE ( 'NONE', #24815, #33163 ) ;
#25121=EDGE_CURVE ( 'NONE', #42656, #11634, #11354, .T. ) ;
#25122=CARTESIAN_POINT ( 'NONE',  ( -26.13337879274045505, 0.000000000000000000, 6.833023547870798353 ) ) ;
#25123=CARTESIAN_POINT ( 'NONE',  ( -15.82600388905919608, 0.000000000000000000, 7.851908118552977989 ) ) ;
#25124=EDGE_LOOP ( 'NONE', ( #12357, #46022, #18257, #26364 ) ) ;
#25125=CARTESIAN_POINT ( 'NONE',  ( -21.49419195319602238, -4.565544526780663581, 5.084730443979996295 ) ) ;
#25126=VECTOR ( 'NONE', #40010, 999.9999999999998863 ) ;
#25127=CARTESIAN_POINT ( 'NONE',  ( -8.024318355659660895, -0.1191753592594181205, 6.335291332000426046 ) ) ;
#25128=CARTESIAN_POINT ( 'NONE',  ( -23.33849165029409889, 0.000000000000000000, 5.946783852668351855 ) ) ;
#25129=ORIENTED_EDGE ( 'NONE', *, *, #23603, .F. ) ;
#25130=LINE ( 'NONE', #15455, #1159 ) ;
#25131=CARTESIAN_POINT ( 'NONE',  ( 2.072287782118878319, 0.000000000000000000, -2.950529333540147015 ) ) ;
#25132=LINE ( 'NONE', #4386, #6684 ) ;
#25133=ORIENTED_EDGE ( 'NONE', *, *, #51842, .F. ) ;
#25134=DIRECTION ( 'NONE',  ( -0.005002170337468016433, -0.7660444431189770143, 0.6427681459581293666 ) ) ;
#25135=VECTOR ( 'NONE', #18696, 999.9999999999998863 ) ;
#25136=ORIENTED_EDGE ( 'NONE', *, *, #41198, .T. ) ;
#25137=EDGE_LOOP ( 'NONE', ( #48373, #16173, #21505, #45108 ) ) ;
#25138=VECTOR ( 'NONE', #1810, 1000.000000000000000 ) ;
#25139=VERTEX_POINT ( 'NONE', #40342 ) ;
#25140=VERTEX_POINT ( 'NONE', #1442 ) ;
#25141=DIRECTION ( 'NONE',  ( 0.9999697198139515519, 0.000000000000000000, 0.007781995580013368816 ) ) ;
#25143=EDGE_CURVE ( 'NONE', #46034, #6528, #23319, .T. ) ;
#25144=DIRECTION ( 'NONE',  ( -0.6246952433987894571, 0.7422098413412802076, 0.2426528472758539834 ) ) ;
#25145=AXIS2_PLACEMENT_3D ( 'NONE', #11594, #2756, #20080 ) ;
#25146=VERTEX_POINT ( 'NONE', #45419 ) ;
#25147=CARTESIAN_POINT ( 'NONE',  ( -21.47419595591918906, 0.000000000000000000, 5.222628093224860102 ) ) ;
#25148=ORIENTED_EDGE ( 'NONE', *, *, #40097, .F. ) ;
#25149=EDGE_CURVE ( 'NONE', #15196, #31624, #6534, .T. ) ;
#25150=ORIENTED_EDGE ( 'NONE', *, *, #18306, .T. ) ;
#25151=DIRECTION ( 'NONE',  ( 0.007781995580012662783, 0.000000000000000000, -0.9999697198139514409 ) ) ;
#25152=CARTESIAN_POINT ( 'NONE',  ( -16.05094756644385967, 4.981562823951511731, 11.29164751933717525 ) ) ;
#25153=EDGE_CURVE ( 'NONE', #38932, #26788, #54784, .T. ) ;
#25155=CARTESIAN_POINT ( 'NONE',  ( -26.13493519185646008, 0.000000000000000000, 7.033017491833586377 ) ) ;
#25156=CARTESIAN_POINT ( 'NONE',  ( -27.06708303904391144, 0.000000000000000000, 7.395095371555332697 ) ) ;
#25157=ORIENTED_EDGE ( 'NONE', *, *, #1345, .F. ) ;
#25158=EDGE_CURVE ( 'NONE', #23927, #38022, #37464, .T. ) ;
#25159=EDGE_CURVE ( 'NONE', #8086, #4449, #34347, .T. ) ;
#25160=ADVANCED_FACE ( 'NONE', ( #38036 ), #51079, .F. ) ;
#25161=EDGE_LOOP ( 'NONE', ( #19456, #10529, #47992, #7379 ) ) ;
#25162=CARTESIAN_POINT ( 'NONE',  ( -23.33693525117809386, 0.000000000000000000, 5.746789908705562944 ) ) ;
#25163=CARTESIAN_POINT ( 'NONE',  ( -19.16905877885434606, -0.1191753592594168992, 6.617892454864216845 ) ) ;
#25164=EDGE_CURVE ( 'NONE', #49938, #37899, #46536, .T. ) ;
#25165=CARTESIAN_POINT ( 'NONE',  ( -15.88130887279446490, 0.000000000000000000, 3.050160814894388839 ) ) ;
#25166=LINE ( 'NONE', #7261, #40324 ) ;
#25167=CARTESIAN_POINT ( 'NONE',  ( -19.45503627000849889, -1.000000000000000000, 7.556996783084074742 ) ) ;
#25168=FACE_OUTER_BOUND ( 'NONE', #25980, .T. ) ;
#25169=ORIENTED_EDGE ( 'NONE', *, *, #24608, .T. ) ;
#25170=CARTESIAN_POINT ( 'NONE',  ( -16.81345671998191449, 0.000000000000000000, 3.412238694616132495 ) ) ;
#25171=CARTESIAN_POINT ( 'NONE',  ( -14.94916102560700821, 0.000000000000000000, 2.688082935172642962 ) ) ;
#25172=ORIENTED_EDGE ( 'NONE', *, *, #26390, .T. ) ;
#25173=CARTESIAN_POINT ( 'NONE',  ( 2.072287782118878319, 0.000000000000000000, -2.950529333540147015 ) ) ;
#25174=LINE ( 'NONE', #50710, #8774 ) ;
#25175=CARTESIAN_POINT ( 'NONE',  ( -11.60690912192075075, 0.000000000000000000, 3.083425182114127416 ) ) ;
#25176=EDGE_CURVE ( 'NONE', #6270, #48144, #50802, .T. ) ;
#25177=DIRECTION ( 'NONE',  ( -0.005961354470445682716, -0.6427876096865404731, 0.7660212471507180654 ) ) ;
#25178=DIRECTION ( 'NONE',  ( -0.5449076811759708816, 0.6444004775717707689, 0.5364919789714475140 ) ) ;
#25179=EDGE_CURVE ( 'NONE', #22744, #48082, #29221, .T. ) ;
#25180=VECTOR ( 'NONE', #8707, 1000.000000000000114 ) ;
#25181=VERTEX_POINT ( 'NONE', #16437 ) ;
#25182=ORIENTED_EDGE ( 'NONE', *, *, #7927, .F. ) ;
#25183=EDGE_CURVE ( 'NONE', #20216, #10313, #7112, .T. ) ;
#25184=DIRECTION ( 'NONE',  ( 0.005961354470445682716, -0.6427876096865404731, -0.7660212471507180654 ) ) ;
#25185=LINE ( 'NONE', #29982, #8665 ) ;
#25187=ADVANCED_FACE ( 'NONE', ( #7655 ), #20720, .F. ) ;
#25188=VECTOR ( 'NONE', #113, 1000.000000000000227 ) ;
#25189=LINE ( 'NONE', #7558, #6521 ) ;
#25190=FACE_OUTER_BOUND ( 'NONE', #22588, .T. ) ;
#25191=DIRECTION ( 'NONE',  ( -0.5364919789714478471, 0.6444004775717705469, -0.5449076811759709926 ) ) ;
#25192=PLANE ( 'NONE',  #41923 ) ;
#25193=EDGE_CURVE ( 'NONE', #13033, #25808, #55931, .T. ) ;
#25194=DIRECTION ( 'NONE',  ( 0.007781995580012663651, -3.146120232559066537E-19, -0.9999697198139514409 ) ) ;
#25196=CARTESIAN_POINT ( 'NONE',  ( -19.45503627000849889, -1.000000000000000000, 7.556996783084074742 ) ) ;
#25197=ORIENTED_EDGE ( 'NONE', *, *, #52228, .T. ) ;
#25198=DIRECTION ( 'NONE',  ( 0.007781995580012663651, 0.000000000000000000, -0.9999697198139515519 ) ) ;
#25199=VERTEX_POINT ( 'NONE', #15893 ) ;
#25200=VERTEX_POINT ( 'NONE', #20433 ) ;
#25201=VERTEX_POINT ( 'NONE', #46847 ) ;
#25202=ORIENTED_EDGE ( 'NONE', *, *, #25731, .F. ) ;
#25203=ORIENTED_EDGE ( 'NONE', *, *, #14271, .T. ) ;
#25204=VERTEX_POINT ( 'NONE', #25524 ) ;
#25205=FACE_OUTER_BOUND ( 'NONE', #31099, .T. ) ;
#25206=CARTESIAN_POINT ( 'NONE',  ( -15.84391369215092737, -5.051250379848164940, 2.874473923470473480 ) ) ;
#25207=DIRECTION ( 'NONE',  ( -0.005002170337468016433, -0.7660444431189770143, 0.6427681459581293666 ) ) ;
#25209=PLANE ( 'NONE',  #46710 ) ;
#25211=FACE_OUTER_BOUND ( 'NONE', #39153, .T. ) ;
#25212=ORIENTED_EDGE ( 'NONE', *, *, #18813, .F. ) ;
#25214=CARTESIAN_POINT ( 'NONE',  ( -14.42766274591465425, 0.000000000000000000, 7.293452206636453106 ) ) ;
#25215=DIRECTION ( 'NONE',  ( -0.6427681459581293666, -0.7660444431189770143, -0.005002170337467561935 ) ) ;
#25216=ORIENTED_EDGE ( 'NONE', *, *, #8320, .T. ) ;
#25217=CARTESIAN_POINT ( 'NONE',  ( 2.072287782118878319, 0.000000000000000000, -2.950529333540147015 ) ) ;
#25218=EDGE_LOOP ( 'NONE', ( #17494, #2443, #24356, #33839 ) ) ;
#25219=ADVANCED_FACE ( 'NONE', ( #33498 ), #24983, .F. ) ;
#25220=ADVANCED_FACE ( 'NONE', ( #51391 ), #17030, .F. ) ;
#25221=AXIS2_PLACEMENT_3D ( 'NONE', #10580, #1474, #46031 ) ;
#25222=CARTESIAN_POINT ( 'NONE',  ( -7.851256608156574224, 5.553015032381929394, -0.1686788792590568631 ) ) ;
#25223=DIRECTION ( 'NONE',  ( -0.005002170337468016433, -0.7660444431189770143, 0.6427681459581293666 ) ) ;
#25225=DIRECTION ( 'NONE',  ( 0.7660212471507180654, -0.6427876096865404731, 0.005961354470445141482 ) ) ;
#25226=DIRECTION ( 'NONE',  ( 0.5449076811759707706, 0.6444004775717708799, -0.5364919789714476250 ) ) ;
#25227=DIRECTION ( 'NONE',  ( 0.007781995580012663651, -3.146120232559066537E-19, -0.9999697198139514409 ) ) ;
#25228=CARTESIAN_POINT ( 'NONE',  ( -19.12962290826653700, 0.000000000000000000, 14.40064212555863854 ) ) ;
#25229=DIRECTION ( 'NONE',  ( -0.9999697198139514409, -0.000000000000000000, -0.007781995580013368816 ) ) ;
#25230=CARTESIAN_POINT ( 'NONE',  ( -14.02149608406334380, -0.1166911823299071477, 2.228051675397754394 ) ) ;
#25231=ORIENTED_EDGE ( 'NONE', *, *, #25780, .F. ) ;
#25233=ORIENTED_EDGE ( 'NONE', *, *, #6917, .T. ) ;
#25234=CARTESIAN_POINT ( 'NONE',  ( 2.072287782118878319, 0.000000000000000000, -2.950529333540147015 ) ) ;
#25235=CARTESIAN_POINT ( 'NONE',  ( -10.21587248490277844, 0.000000000000000000, 3.463582620675918378 ) ) ;
#25236=CARTESIAN_POINT ( 'NONE',  ( -19.74467861466184715, -3.594132820645662196, 4.436153168894599652 ) ) ;
#25237=DIRECTION ( 'NONE',  ( -0.7660212471507179544, -0.6427876096865405842, -0.005961354470445141482 ) ) ;
#25238=DIRECTION ( 'NONE',  ( 0.5364919789714477361, 0.6444004775717706579, 0.5449076811759711036 ) ) ;
#25239=LINE ( 'NONE', #24377, #55643 ) ;
#25240=EDGE_LOOP ( 'NONE', ( #28965, #821, #47392, #43273 ) ) ;
#25241=CARTESIAN_POINT ( 'NONE',  ( -17.26532721389163072, 0.000000000000000000, 13.67648636611514590 ) ) ;
#25242=DIRECTION ( 'NONE',  ( -0.005961354470445682716, -0.6427876096865404731, 0.7660212471507180654 ) ) ;
#25243=CARTESIAN_POINT ( 'NONE',  ( -22.40634380310664397, 0.000000000000000000, 5.584705972946605534 ) ) ;
#25244=DIRECTION ( 'NONE',  ( 0.005002170337468016433, -0.7660444431189770143, -0.6427681459581293666 ) ) ;
#25245=FACE_OUTER_BOUND ( 'NONE', #37783, .T. ) ;
#25246=DIRECTION ( 'NONE',  ( 0.005002170337468016433, -0.7660444431189770143, -0.6427681459581293666 ) ) ;
#25247=EDGE_CURVE ( 'NONE', #8547, #722, #41714, .T. ) ;
#25248=CARTESIAN_POINT ( 'NONE',  ( -14.15882808514179736, 0.000000000000000000, 6.756886256735718632 ) ) ;
#25249=CARTESIAN_POINT ( 'NONE',  ( -23.33771345073609638, -0.1191753592594197858, 5.846786880686956955 ) ) ;
#25250=VERTEX_POINT ( 'NONE', #11644 ) ;
#25251=DIRECTION ( 'NONE',  ( 0.6427681459581294776, -0.7660444431189769032, 0.005002170337467562802 ) ) ;
#25252=PLANE ( 'NONE',  #21443 ) ;
#25253=EDGE_LOOP ( 'NONE', ( #22674, #52541, #32932, #43787 ) ) ;
#25254=EDGE_CURVE ( 'NONE', #26165, #6886, #12754, .T. ) ;
#25255=EDGE_LOOP ( 'NONE', ( #52432, #28655, #28533, #7191 ) ) ;
#25256=CARTESIAN_POINT ( 'NONE',  ( -11.83276954743108256, 0.000000000000000000, 6.405656112318003359 ) ) ;
#25257=ADVANCED_FACE ( 'NONE', ( #28960 ), #46252, .F. ) ;
#25258=AXIS2_PLACEMENT_3D ( 'NONE', #4825, #21856, #9360 ) ;
#25259=VERTEX_POINT ( 'NONE', #26361 ) ;
#25261=CARTESIAN_POINT ( 'NONE',  ( -12.56204939715046720, 0.000000000000000000, 6.399980687897988574 ) ) ;
#25262=ORIENTED_EDGE ( 'NONE', *, *, #23798, .F. ) ;
#25263=VERTEX_POINT ( 'NONE', #30072 ) ;
#25264=ORIENTED_EDGE ( 'NONE', *, *, #31100, .T. ) ;
#25265=FACE_OUTER_BOUND ( 'NONE', #8371, .T. ) ;
#25266=CARTESIAN_POINT ( 'NONE',  ( -14.56888064431065821, -0.1191753592594197858, 12.58947452739191064 ) ) ;
#25267=CARTESIAN_POINT ( 'NONE',  ( -14.94916102560700821, 0.000000000000000000, 2.688082935172642962 ) ) ;
#25269=ORIENTED_EDGE ( 'NONE', *, *, #39942, .F. ) ;
#25270=CARTESIAN_POINT ( 'NONE',  ( -10.81400064959561469, -0.1159828484229834950, 7.418898672974625796 ) ) ;
#25271=LINE ( 'NONE', #17037, #38173 ) ;
#25272=ORIENTED_EDGE ( 'NONE', *, *, #23589, .F. ) ;
#25273=LINE ( 'NONE', #38044, #2821 ) ;
#25274=DIRECTION ( 'NONE',  ( -0.7660212471507179544, -0.6427876096865405842, -0.005961354470445141482 ) ) ;
#25275=ORIENTED_EDGE ( 'NONE', *, *, #7360, .T. ) ;
#25276=PLANE ( 'NONE',  #6744 ) ;
#25277=CARTESIAN_POINT ( 'NONE',  ( -19.78515715608675762, 1.969473882990073754, 6.707120304835959779 ) ) ;
#25278=EDGE_CURVE ( 'NONE', #7048, #17764, #34602, .T. ) ;
#25279=VERTEX_POINT ( 'NONE', #17571 ) ;
#25280=LINE ( 'NONE', #26375, #48180 ) ;
#25281=EDGE_CURVE ( 'NONE', #48572, #34537, #26950, .T. ) ;
#25282=ADVANCED_FACE ( 'NONE', ( #34909 ), #13862, .F. ) ;
#25283=LINE ( 'NONE', #4276, #20018 ) ;
#25284=ORIENTED_EDGE ( 'NONE', *, *, #21752, .T. ) ;
#25285=DIRECTION ( 'NONE',  ( -0.5364919789714478471, 0.6444004775717705469, -0.5449076811759709926 ) ) ;
#25286=PLANE ( 'NONE',  #4793 ) ;
#25287=DIRECTION ( 'NONE',  ( 0.5449076811759707706, 0.6444004775717708799, -0.5364919789714476250 ) ) ;
#25288=CARTESIAN_POINT ( 'NONE',  ( -17.40110780339754371, 0.000000000000000000, 5.423651820623570430 ) ) ;
#25289=ORIENTED_EDGE ( 'NONE', *, *, #10620, .F. ) ;
#25290=VECTOR ( 'NONE', #18228, 999.9999999999998863 ) ;
#25291=DIRECTION ( 'NONE',  ( 0.007781995580012662783, 0.000000000000000000, -0.9999697198139514409 ) ) ;
#25292=PLANE ( 'NONE',  #32340 ) ;
#25293=CARTESIAN_POINT ( 'NONE',  ( -10.71056757118597069, 0.000000000000000000, 7.322379500780528794 ) ) ;
#25294=FACE_OUTER_BOUND ( 'NONE', #52622, .T. ) ;
#25295=LINE ( 'NONE', #42599, #26747 ) ;
#25296=DIRECTION ( 'NONE',  ( 0.007781995580012663651, 0.000000000000000000, -0.9999697198139515519 ) ) ;
#25297=EDGE_CURVE ( 'NONE', #23151, #23833, #48515, .T. ) ;
#25299=VERTEX_POINT ( 'NONE', #21826 ) ;
#25301=ORIENTED_EDGE ( 'NONE', *, *, #24049, .F. ) ;
#25302=CARTESIAN_POINT ( 'NONE',  ( -19.60834386242827776, 0.000000000000000000, 4.298478389818581213 ) ) ;
#25303=PLANE ( 'NONE',  #55373 ) ;
#25304=PLANE ( 'NONE',  #11340 ) ;
#25305=DIRECTION ( 'NONE',  ( -0.9999697198139514409, -0.000000000000000000, -0.007781995580013368816 ) ) ;
#25306=DIRECTION ( 'NONE',  ( -0.5449076811759708816, 0.6444004775717707689, 0.5364919789714475140 ) ) ;
#25307=ORIENTED_EDGE ( 'NONE', *, *, #24144, .F. ) ;
#25308=VERTEX_POINT ( 'NONE', #48210 ) ;
#25309=DIRECTION ( 'NONE',  ( -0.005961354470445682716, -0.6427876096865404731, 0.7660212471507180654 ) ) ;
#25310=DIRECTION ( 'NONE',  ( -0.005961354470445682716, -0.6427876096865404731, 0.7660212471507180654 ) ) ;
#25313=ORIENTED_EDGE ( 'NONE', *, *, #46376, .T. ) ;
#25314=CARTESIAN_POINT ( 'NONE',  ( -24.26908309836554878, 0.000000000000000000, 6.108867788427308376 ) ) ;
#25315=ADVANCED_FACE ( 'NONE', ( #47386 ), #21575, .F. ) ;
#25316=ORIENTED_EDGE ( 'NONE', *, *, #37666, .F. ) ;
#25317=FACE_OUTER_BOUND ( 'NONE', #50060, .T. ) ;
#25318=ORIENTED_EDGE ( 'NONE', *, *, #3134, .T. ) ;
#25319=VERTEX_POINT ( 'NONE', #9633 ) ;
#25320=VERTEX_POINT ( 'NONE', #22672 ) ;
#25321=CARTESIAN_POINT ( 'NONE',  ( -17.74404816805336793, 0.000000000000000000, 3.574322630375089460 ) ) ;
#25322=CARTESIAN_POINT ( 'NONE',  ( 2.072287782118878319, 0.000000000000000000, -2.950529333540147015 ) ) ;
#25323=CARTESIAN_POINT ( 'NONE',  ( -13.64701913762987573, 1.095915999411505526, 1.947931961135673129 ) ) ;
#25324=EDGE_CURVE ( 'NONE', #16295, #38023, #53060, .T. ) ;
#25326=FACE_OUTER_BOUND ( 'NONE', #1464, .T. ) ;
#25327=ORIENTED_EDGE ( 'NONE', *, *, #13822, .T. ) ;
#25328=EDGE_CURVE ( 'NONE', #49293, #30466, #38889, .T. ) ;
#25329=EDGE_CURVE ( 'NONE', #48860, #28185, #13335, .T. ) ;
#25330=ORIENTED_EDGE ( 'NONE', *, *, #25353, .T. ) ;
#25331=EDGE_LOOP ( 'NONE', ( #45488, #50601, #36175, #42621 ) ) ;
#25332=DIRECTION ( 'NONE',  ( -0.5449076811759708816, 0.6444004775717707689, 0.5364919789714475140 ) ) ;
#25333=FACE_OUTER_BOUND ( 'NONE', #28884, .T. ) ;
#25334=VERTEX_POINT ( 'NONE', #44264 ) ;
#25335=DIRECTION ( 'NONE',  ( 0.9999697198139515519, 0.000000000000000000, 0.007781995580013368816 ) ) ;
#25336=ADVANCED_FACE ( 'NONE', ( #30367 ), #43421, .F. ) ;
#25337=ORIENTED_EDGE ( 'NONE', *, *, #46582, .T. ) ;
#25338=PLANE ( 'NONE',  #54141 ) ;
#25339=CARTESIAN_POINT ( 'NONE',  ( -14.43628490643050277, 0.000000000000000000, 8.401381316409748834 ) ) ;
#25340=EDGE_LOOP ( 'NONE', ( #29146, #26698, #14934, #9841 ) ) ;
#25341=EDGE_CURVE ( 'NONE', #38808, #12870, #43150, .T. ) ;
#25342=PLANE ( 'NONE',  #46767 ) ;
#25343=EDGE_LOOP ( 'NONE', ( #33237, #52193, #72, #6999 ) ) ;
#25344=ADVANCED_FACE ( 'NONE', ( #4259 ), #9323, .F. ) ;
#25345=LINE ( 'NONE', #4344, #7417 ) ;
#25346=CARTESIAN_POINT ( 'NONE',  ( -22.40556560354864146, -0.1191753592594197858, 5.484709000965211523 ) ) ;
#25347=EDGE_LOOP ( 'NONE', ( #24525, #49569, #55096, #25368 ) ) ;
#25348=FACE_OUTER_BOUND ( 'NONE', #18537, .T. ) ;
#25349=LINE ( 'NONE', #43252, #42962 ) ;
#25350=CARTESIAN_POINT ( 'NONE',  ( -13.80469194557137769, 2.391131607591508335, 1.967853275232125609 ) ) ;
#25351=LINE ( 'NONE', #55169, #19199 ) ;
#25352=ORIENTED_EDGE ( 'NONE', *, *, #10225, .T. ) ;
#25353=EDGE_CURVE ( 'NONE', #35444, #30427, #47957, .T. ) ;
#25354=ORIENTED_EDGE ( 'NONE', *, *, #22408, .F. ) ;
#25355=CARTESIAN_POINT ( 'NONE',  ( -15.97319677381126013, -1.327505506330657781, 3.043498820269260552 ) ) ;
#25357=LINE ( 'NONE', #42659, #18688 ) ;
#25358=DIRECTION ( 'NONE',  ( 0.005961354470445682716, -0.6427876096865404731, -0.7660212471507180654 ) ) ;
#25359=FACE_OUTER_BOUND ( 'NONE', #1622, .T. ) ;
#25360=EDGE_CURVE ( 'NONE', #36655, #48938, #8497, .T. ) ;
#25361=PLANE ( 'NONE',  #20415 ) ;
#25362=EDGE_LOOP ( 'NONE', ( #21424, #35071, #34614, #42685 ) ) ;
#25363=DIRECTION ( 'NONE',  ( 0.9999697198139515519, 0.000000000000000000, 0.007781995580013368816 ) ) ;
#25364=PLANE ( 'NONE',  #49464 ) ;
#25365=CARTESIAN_POINT ( 'NONE',  ( -17.43272239195565376, 0.000000000000000000, 9.486058556458980107 ) ) ;
#25366=ORIENTED_EDGE ( 'NONE', *, *, #17134, .F. ) ;
#25367=DIRECTION ( 'NONE',  ( 0.7660212471507180654, -0.6427876096865404731, 0.005961354470445141482 ) ) ;
#25368=ORIENTED_EDGE ( 'NONE', *, *, #44572, .F. ) ;
#25369=PRODUCT_DEFINITION_FORMATION_WITH_SPECIFIED_SOURCE ( 'ANY', '', #53221, .NOT_KNOWN. ) ;
#25371=FACE_OUTER_BOUND ( 'NONE', #41883, .T. ) ;
#25372=PLANE ( 'NONE',  #29613 ) ;
#25374=ORIENTED_EDGE ( 'NONE', *, *, #27906, .F. ) ;
#25375=ORIENTED_EDGE ( 'NONE', *, *, #2504, .F. ) ;
#25376=CARTESIAN_POINT ( 'NONE',  ( -31.72782227498118601, 0.000000000000000000, 9.205484770164058972 ) ) ;
#25377=LINE ( 'NONE', #42678, #6828 ) ;
#25378=FACE_OUTER_BOUND ( 'NONE', #32815, .T. ) ;
#25379=DIRECTION ( 'NONE',  ( -0.9999697198139514409, -0.000000000000000000, -0.007781995580013368816 ) ) ;
#25380=DIRECTION ( 'NONE',  ( 0.5364919789714477361, 0.6444004775717706579, 0.5449076811759711036 ) ) ;
#25381=CARTESIAN_POINT ( 'NONE',  ( -17.33011717104096405, -0.1117717739993967785, 9.949979618152523742 ) ) ;
#25382=ADVANCED_FACE ( 'NONE', ( #9056 ), #43674, .F. ) ;
#25383=EDGE_LOOP ( 'NONE', ( #26239, #11656, #6540, #826 ) ) ;
#25384=CARTESIAN_POINT ( 'NONE',  ( -17.60792775650470077, -3.270328918600661883, 3.616497610996559420 ) ) ;
#25385=FACE_OUTER_BOUND ( 'NONE', #13757, .T. ) ;
#25386=LINE ( 'NONE', #3790, #43257 ) ;
#25387=EDGE_LOOP ( 'NONE', ( #30710, #49651, #19940, #8721 ) ) ;
#25388=CARTESIAN_POINT ( 'NONE',  ( -15.32400429664943609, 0.000000000000000000, 3.054497887970051284 ) ) ;
#25389=DIRECTION ( 'NONE',  ( -0.5449076811759708816, 0.6444004775717707689, 0.5364919789714475140 ) ) ;
#25390=CARTESIAN_POINT ( 'NONE',  ( -14.94916102560700821, 0.000000000000000000, 2.688082935172642962 ) ) ;
#25391=VERTEX_POINT ( 'NONE', #10165 ) ;
#25392=CARTESIAN_POINT ( 'NONE',  ( -18.67619601524082285, 0.000000000000000000, 3.936400510096834893 ) ) ;
#25393=ORIENTED_EDGE ( 'NONE', *, *, #56233, .F. ) ;
#25394=EDGE_CURVE ( 'NONE', #12113, #5158, #28053, .T. ) ;
#25395=VECTOR ( 'NONE', #52183, 1000.000000000000227 ) ;
#25396=ORIENTED_EDGE ( 'NONE', *, *, #35003, .T. ) ;
#25397=VERTEX_POINT ( 'NONE', #45358 ) ;
#25398=ORIENTED_EDGE ( 'NONE', *, *, #43167, .T. ) ;
#25399=CARTESIAN_POINT ( 'NONE',  ( -9.808144436391993182, 0.000000000000000000, 10.77986332834118777 ) ) ;
#25400=EDGE_LOOP ( 'NONE', ( #19133, #51411, #22665, #34057 ) ) ;
#25401=DIRECTION ( 'NONE',  ( -0.005002170337468016433, -0.7660444431189770143, 0.6427681459581293666 ) ) ;
#25402=ORIENTED_EDGE ( 'NONE', *, *, #48918, .T. ) ;
#25403=CARTESIAN_POINT ( 'NONE',  ( -25.20278734466900517, 0.000000000000000000, 6.670939612111840944 ) ) ;
#25404=EDGE_CURVE ( 'NONE', #42504, #21903, #40272, .T. ) ;
#25405=ORIENTED_EDGE ( 'NONE', *, *, #12269, .F. ) ;
#25406=ORIENTED_EDGE ( 'NONE', *, *, #10498, .F. ) ;
#25407=ADVANCED_FACE ( 'NONE', ( #1650 ), #54175, .F. ) ;
#25408=LINE ( 'NONE', #39310, #23845 ) ;
#25409=CARTESIAN_POINT ( 'NONE',  ( -17.74560456716937296, 0.000000000000000000, 3.774316574337878372 ) ) ;
#25410=DIRECTION ( 'NONE',  ( 0.005002170337468016433, -0.7660444431189770143, -0.6427681459581293666 ) ) ;
#25412=DIRECTION ( 'NONE',  ( 0.005002170337468016433, -0.7660444431189770143, -0.6427681459581293666 ) ) ;
#25413=ORIENTED_EDGE ( 'NONE', *, *, #25858, .T. ) ;
#25415=ORIENTED_EDGE ( 'NONE', *, *, #458, .T. ) ;
#25417=LINE ( 'NONE', #39038, #4931 ) ;
#25418=CARTESIAN_POINT ( 'NONE',  ( -11.16813870662720909, 0.000000000000000000, 6.410828423202016069 ) ) ;
#25419=ADVANCED_FACE ( 'NONE', ( #36872 ), #23251, .F. ) ;
#25421=DIRECTION ( 'NONE',  ( 0.000000000000000000, -0.000000000000000000, -1.000000000000000000 ) ) ;
#25422=FACE_OUTER_BOUND ( 'NONE', #16587, .T. ) ;
#25423=VERTEX_POINT ( 'NONE', #2488 ) ;
#25424=LINE ( 'NONE', #42476, #14795 ) ;
#25425=LINE ( 'NONE', #119, #41290 ) ;
#25427=LINE ( 'NONE', #8693, #31585 ) ;
#25428=DIRECTION ( 'NONE',  ( 0.000000000000000000, -1.000000000000000000, 0.000000000000000000 ) ) ;
#25429=LINE ( 'NONE', #40094, #29074 ) ;
#25430=DIRECTION ( 'NONE',  ( -0.6427681459581293666, -0.7660444431189770143, -0.005002170337467561935 ) ) ;
#25431=DIRECTION ( 'NONE',  ( 0.005961354470445682716, -0.6427876096865404731, -0.7660212471507180654 ) ) ;
#25432=AXIS2_PLACEMENT_3D ( 'NONE', #54401, #7017, #55521 ) ;
#25433=ORIENTED_EDGE ( 'NONE', *, *, #15801, .F. ) ;
#25434=ORIENTED_EDGE ( 'NONE', *, *, #16928, .F. ) ;
#25436=DIRECTION ( 'NONE',  ( 0.9999697198139515519, 0.000000000000000000, 0.007781995580013368816 ) ) ;
#25437=CARTESIAN_POINT ( 'NONE',  ( -24.26986129792355129, -0.1191753592594197858, 6.208864760408702388 ) ) ;
#25438=DIRECTION ( 'NONE',  ( 0.007781995580012662783, 0.000000000000000000, -0.9999697198139514409 ) ) ;
#25439=DIRECTION ( 'NONE',  ( 0.000000000000000000, -1.000000000000000000, 0.000000000000000000 ) ) ;
#25440=EDGE_CURVE ( 'NONE', #20904, #9112, #40573, .T. ) ;
#25441=DIRECTION ( 'NONE',  ( 0.000000000000000000, -0.000000000000000000, -1.000000000000000000 ) ) ;
#25442=DIRECTION ( 'NONE',  ( 0.7660212471507180654, -0.6427876096865404731, 0.005961354470445141482 ) ) ;
#25443=CARTESIAN_POINT ( 'NONE',  ( -10.94028622754223967, 0.000000000000000000, 11.14038480894692995 ) ) ;
#25444=DIRECTION ( 'NONE',  ( 0.005002170337468016433, -0.7660444431189770143, -0.6427681459581293666 ) ) ;
#25445=EDGE_CURVE ( 'NONE', #49287, #55547, #18977, .T. ) ;
#25446=ADVANCED_FACE ( 'NONE', ( #27486 ), #53601, .F. ) ;
#25447=DIRECTION ( 'NONE',  ( 0.6427681459581294776, -0.7660444431189769032, 0.005002170337467562802 ) ) ;
#25448=VERTEX_POINT ( 'NONE', #45633 ) ;
#25449=CARTESIAN_POINT ( 'NONE',  ( -9.110551994824897193, -1.000000000000000000, 3.538847790438064411 ) ) ;
#25450=EDGE_CURVE ( 'NONE', #41560, #42137, #10467, .T. ) ;
#25451=ADVANCED_FACE ( 'NONE', ( #53349 ), #48805, .F. ) ;
#25452=ADVANCED_FACE ( 'NONE', ( #27210 ), #32333, .F. ) ;
#25453=VERTEX_POINT ( 'NONE', #14443 ) ;
#25454=ORIENTED_EDGE ( 'NONE', *, *, #55907, .T. ) ;
#25455=VERTEX_POINT ( 'NONE', #1366 ) ;
#25456=VERTEX_POINT ( 'NONE', #18710 ) ;
#25457=EDGE_LOOP ( 'NONE', ( #29647, #39330, #33391, #5157 ) ) ;
#25459=CARTESIAN_POINT ( 'NONE',  ( -15.46582147666606488, -0.1117717739994045917, 9.225823858709038205 ) ) ;
#25460=CARTESIAN_POINT ( 'NONE',  ( -12.70037056462282088, 3.848249166794011522, 1.492407668973236845 ) ) ;
#25461=DIRECTION ( 'NONE',  ( -0.9999697198139514409, -0.000000000000000000, -0.007781995580013368816 ) ) ;
#25462=VECTOR ( 'NONE', #14266, 999.9999999999998863 ) ;
#25463=EDGE_LOOP ( 'NONE', ( #9139, #33078, #62, #27766 ) ) ;
#25464=CARTESIAN_POINT ( 'NONE',  ( -21.47263955680318404, 0.000000000000000000, 5.022634149262071190 ) ) ;
#25465=EDGE_CURVE ( 'NONE', #37343, #49177, #49350, .T. ) ;
#25466=ORIENTED_EDGE ( 'NONE', *, *, #32249, .F. ) ;
#25467=PLANE ( 'NONE',  #52210 ) ;
#25468=ORIENTED_EDGE ( 'NONE', *, *, #28468, .T. ) ;
#25469=AXIS2_PLACEMENT_3D ( 'NONE', #513, #5347, #203 ) ;
#25470=EDGE_CURVE ( 'NONE', #41524, #48104, #6211, .T. ) ;
#25471=DIRECTION ( 'NONE',  ( -0.9999697198139514409, -0.000000000000000000, -0.007781995580013368816 ) ) ;
#25472=EDGE_CURVE ( 'NONE', #18589, #16426, #1903, .T. ) ;
#25473=DIRECTION ( 'NONE',  ( 0.005961354470445682716, -0.6427876096865404731, -0.7660212471507180654 ) ) ;
#25474=DIRECTION ( 'NONE',  ( 0.005961354470445682716, -0.6427876096865404731, -0.7660212471507180654 ) ) ;
#25475=EDGE_LOOP ( 'NONE', ( #26327, #9052, #42475, #45661 ) ) ;
#25476=CARTESIAN_POINT ( 'NONE',  ( -17.20973601995061131, 0.000000000000000000, 6.533137329512866742 ) ) ;
#25477=VERTEX_POINT ( 'NONE', #49648 ) ;
#25478=EDGE_CURVE ( 'NONE', #441, #29890, #10746, .T. ) ;
#25479=CARTESIAN_POINT ( 'NONE',  ( -31.72782227498118601, 0.000000000000000000, 9.205484770164058972 ) ) ;
#25480=DIRECTION ( 'NONE',  ( 0.8531650599175529814, -0.4028455766673920135, -0.3313982828793697877 ) ) ;
#25481=DIRECTION ( 'NONE',  ( 0.6427681459581294776, -0.7660444431189769032, 0.005002170337467562802 ) ) ;
#25482=FACE_OUTER_BOUND ( 'NONE', #33316, .T. ) ;
#25483=CARTESIAN_POINT ( 'NONE',  ( -20.38711805380392406, 1.905425754524007642, 4.540187675463392303 ) ) ;
#25484=LINE ( 'NONE', #47640, #53892 ) ;
#25485=PLANE ( 'NONE',  #41166 ) ;
#25487=ORIENTED_EDGE ( 'NONE', *, *, #10020, .F. ) ;
#25489=ORIENTED_EDGE ( 'NONE', *, *, #20970, .F. ) ;
#25490=VECTOR ( 'NONE', #27841, 1000.000000000000227 ) ;
#25491=VECTOR ( 'NONE', #311, 999.9999999999998863 ) ;
#25492=CARTESIAN_POINT ( 'NONE',  ( -16.94256912529133174, -4.079838673713161334, 9.958711274498135424 ) ) ;
#25493=DIRECTION ( 'NONE',  ( 0.007781995580012663651, 0.000000000000000000, -0.9999697198139515519 ) ) ;
#25494=FACE_OUTER_BOUND ( 'NONE', #19036, .T. ) ;
#25495=CARTESIAN_POINT ( 'NONE',  ( -17.85327294482519633, -1.327505506330656893, 5.795411938479114511 ) ) ;
#25496=DIRECTION ( 'NONE',  ( 0.007781995580012662783, 0.000000000000000000, -0.9999697198139514409 ) ) ;
#25497=FACE_OUTER_BOUND ( 'NONE', #36928, .T. ) ;
#25498=ORIENTED_EDGE ( 'NONE', *, *, #12906, .F. ) ;
#25499=PLANE ( 'NONE',  #27528 ) ;
#25500=LINE ( 'NONE', #46228, #33096 ) ;
#25501=DIRECTION ( 'NONE',  ( -0.5449076811759708816, 0.6444004775717707689, 0.5364919789714475140 ) ) ;
#25502=AXIS2_PLACEMENT_3D ( 'NONE', #19255, #15544, #24091 ) ;
#25503=DIRECTION ( 'NONE',  ( 0.000000000000000000, -1.000000000000000000, 0.000000000000000000 ) ) ;
#25504=DIRECTION ( 'NONE',  ( 0.6427681459581294776, -0.7660444431189769032, 0.005002170337467562802 ) ) ;
#25505=CARTESIAN_POINT ( 'NONE',  ( -15.46920792515735243, -0.1191753592594181482, 8.862677968554882213 ) ) ;
#25506=CARTESIAN_POINT ( 'NONE',  ( -21.47419595591918906, 0.000000000000000000, 5.222628093224860102 ) ) ;
#25507=ORIENTED_EDGE ( 'NONE', *, *, #28090, .F. ) ;
#25508=AXIS2_PLACEMENT_3D ( 'NONE', #18130, #48524, #9639 ) ;
#25509=LINE ( 'NONE', #55610, #50294 ) ;
#25510=DIRECTION ( 'NONE',  ( -0.9999697198139514409, -0.000000000000000000, -0.007781995580013368816 ) ) ;
#25511=ORIENTED_EDGE ( 'NONE', *, *, #46279, .T. ) ;
#25513=LINE ( 'NONE', #54770, #14709 ) ;
#25514=EDGE_CURVE ( 'NONE', #329, #14660, #33694, .T. ) ;
#25515=EDGE_CURVE ( 'NONE', #13391, #33224, #37973, .T. ) ;
#25516=ORIENTED_EDGE ( 'NONE', *, *, #15748, .F. ) ;
#25517=EDGE_CURVE ( 'NONE', #30666, #25884, #33993, .T. ) ;
#25518=ORIENTED_EDGE ( 'NONE', *, *, #24498, .F. ) ;
#25520=ORIENTED_EDGE ( 'NONE', *, *, #23547, .T. ) ;
#25522=ORIENTED_EDGE ( 'NONE', *, *, #38891, .F. ) ;
#25523=DIRECTION ( 'NONE',  ( 0.5364919789714477361, 0.6444004775717706579, 0.5449076811759711036 ) ) ;
#25524=CARTESIAN_POINT ( 'NONE',  ( -12.99926341332800739, 0.000000000000000000, 2.872583502847308790 ) ) ;
#25525=VECTOR ( 'NONE', #43050, 999.9999999999998863 ) ;
#25526=VECTOR ( 'NONE', #18138, 999.9999999999998863 ) ;
#25527=ORIENTED_EDGE ( 'NONE', *, *, #41292, .T. ) ;
#25528=VERTEX_POINT ( 'NONE', #11577 ) ;
#25529=EDGE_CURVE ( 'NONE', #35066, #28129, #51318, .T. ) ;
#25530=VECTOR ( 'NONE', #12096, 1000.000000000000227 ) ;
#25532=DIRECTION ( 'NONE',  ( 0.005002170337468016433, -0.7660444431189770143, -0.6427681459581293666 ) ) ;
#25533=ORIENTED_EDGE ( 'NONE', *, *, #11938, .T. ) ;
#25534=ADVANCED_FACE ( 'NONE', ( #7582 ), #2736, .F. ) ;
#25535=DIRECTION ( 'NONE',  ( 0.005961354470445682716, -0.6427876096865404731, -0.7660212471507180654 ) ) ;
#25536=DIRECTION ( 'NONE',  ( 0.5449076811759707706, 0.6444004775717708799, -0.5364919789714476250 ) ) ;
#25537=ORIENTED_EDGE ( 'NONE', *, *, #34115, .F. ) ;
#25538=FACE_OUTER_BOUND ( 'NONE', #7919, .T. ) ;
#25539=VERTEX_POINT ( 'NONE', #3026 ) ;
#25540=EDGE_CURVE ( 'NONE', #50681, #41476, #47050, .T. ) ;
#25541=LINE ( 'NONE', #42858, #17335 ) ;
#25542=ADVANCED_FACE ( 'NONE', ( #16113 ), #7895, .F. ) ;
#25543=AXIS2_PLACEMENT_3D ( 'NONE', #36733, #15166, #32482 ) ;
#25544=CARTESIAN_POINT ( 'NONE',  ( -10.86644437236699190, 1.095915999411505082, 2.900801997477032934 ) ) ;
#25545=ORIENTED_EDGE ( 'NONE', *, *, #10311, .F. ) ;
#25546=PLANE ( 'NONE',  #54858 ) ;
#25547=CARTESIAN_POINT ( 'NONE',  ( -15.80432911540621532, 0.000000000000000000, 5.066746251785837707 ) ) ;
#25548=FACE_OUTER_BOUND ( 'NONE', #20490, .T. ) ;
#25549=LINE ( 'NONE', #43697, #46424 ) ;
#25550=ORIENTED_EDGE ( 'NONE', *, *, #2171, .F. ) ;
#25551=DIRECTION ( 'NONE',  ( -0.5449076811759708816, 0.6444004775717707689, 0.5364919789714475140 ) ) ;
#25552=CARTESIAN_POINT ( 'NONE',  ( -10.20437627088164589, 0.000000000000000000, 1.986343807644861847 ) ) ;
#25553=CARTESIAN_POINT ( 'NONE',  ( -9.542064456761055524, 0.000000000000000000, 10.59726798936431180 ) ) ;
#25554=CARTESIAN_POINT ( 'NONE',  ( -17.57658898651670043, -1.003701604285656579, 5.156521124944394074 ) ) ;
#25555=DIRECTION ( 'NONE',  ( 0.9321478471874541372, 0.000000000000000000, -0.3620778797217453771 ) ) ;
#25556=LINE ( 'NONE', #15929, #46981 ) ;
#25557=DIRECTION ( 'NONE',  ( 0.5364919789714477361, 0.6444004775717706579, 0.5449076811759711036 ) ) ;
#25558=DIRECTION ( 'NONE',  ( 0.007781995580012663651, 0.000000000000000000, -0.9999697198139515519 ) ) ;
#25559=ORIENTED_EDGE ( 'NONE', *, *, #42500, .T. ) ;
#25560=PLANE ( 'NONE',  #10590 ) ;
#25561=EDGE_LOOP ( 'NONE', ( #10605, #18281, #37316, #21489 ) ) ;
#25562=DIRECTION ( 'NONE',  ( 0.005002170337468016433, -0.7660444431189770143, -0.6427681459581293666 ) ) ;
#25564=VECTOR ( 'NONE', #16287, 1000.000000000000000 ) ;
#25565=VECTOR ( 'NONE', #49791, 1000.000000000000227 ) ;
#25566=FACE_OUTER_BOUND ( 'NONE', #9819, .T. ) ;
#25567=PLANE ( 'NONE',  #43282 ) ;
#25569=ORIENTED_EDGE ( 'NONE', *, *, #35117, .F. ) ;
#25570=VECTOR ( 'NONE', #5390, 1000.000000000000000 ) ;
#25571=ORIENTED_EDGE ( 'NONE', *, *, #28833, .F. ) ;
#25572=CARTESIAN_POINT ( 'NONE',  ( -10.94028622754223967, 0.000000000000000000, 11.14038480894692995 ) ) ;
#25573=CARTESIAN_POINT ( 'NONE',  ( -17.72157301408583763, -5.536956232915663634, 12.65268099554350911 ) ) ;
#25574=ORIENTED_EDGE ( 'NONE', *, *, #640, .T. ) ;
#25575=DIRECTION ( 'NONE',  ( 0.000000000000000000, -0.000000000000000000, -1.000000000000000000 ) ) ;
#25577=ORIENTED_EDGE ( 'NONE', *, *, #20249, .T. ) ;
#25578=CARTESIAN_POINT ( 'NONE',  ( -10.94028622754223967, 0.000000000000000000, 11.14038480894692995 ) ) ;
#25579=AXIS2_PLACEMENT_3D ( 'NONE', #49855, #27742, #28014 ) ;
#25580=ORIENTED_EDGE ( 'NONE', *, *, #27181, .T. ) ;
#25581=DIRECTION ( 'NONE',  ( 0.000000000000000000, -1.000000000000000000, 0.000000000000000000 ) ) ;
#25582=EDGE_CURVE ( 'NONE', #54876, #43321, #29150, .T. ) ;
#25583=ADVANCED_FACE ( 'NONE', ( #46773 ), #16661, .F. ) ;
#25584=ORIENTED_EDGE ( 'NONE', *, *, #26249, .T. ) ;
#25585=ORIENTED_EDGE ( 'NONE', *, *, #45164, .F. ) ;
#25586=ORIENTED_EDGE ( 'NONE', *, *, #49587, .T. ) ;
#25587=LINE ( 'NONE', #39207, #13898 ) ;
#25588=FACE_OUTER_BOUND ( 'NONE', #50226, .T. ) ;
#25589=DIRECTION ( 'NONE',  ( 0.007781995580012663651, -3.146120232559066537E-19, -0.9999697198139514409 ) ) ;
#25590=PLANE ( 'NONE',  #25759 ) ;
#25591=EDGE_LOOP ( 'NONE', ( #35050, #16668, #20578, #54715 ) ) ;
#25592=ORIENTED_EDGE ( 'NONE', *, *, #25697, .T. ) ;
#25593=AXIS2_PLACEMENT_3D ( 'NONE', #17981, #48642, #13987 ) ;
#25594=ORIENTED_EDGE ( 'NONE', *, *, #10903, .T. ) ;
#25595=CARTESIAN_POINT ( 'NONE',  ( -16.79925329029790149, 0.000000000000000000, 13.49544742625427496 ) ) ;
#25596=LINE ( 'NONE', #21051, #7696 ) ;
#25597=ORIENTED_EDGE ( 'NONE', *, *, #2751, .T. ) ;
#25598=VECTOR ( 'NONE', #30776, 1000.000000000000227 ) ;
#25600=ORIENTED_EDGE ( 'NONE', *, *, #36713, .T. ) ;
#25601=DIRECTION ( 'NONE',  ( 0.000000000000000000, -0.000000000000000000, -1.000000000000000000 ) ) ;
#25602=CARTESIAN_POINT ( 'NONE',  ( -17.74560456716937296, 0.000000000000000000, 3.774316574337878372 ) ) ;
#25603=AXIS2_PLACEMENT_3D ( 'NONE', #17861, #18384, #14158 ) ;
#25604=AXIS2_PLACEMENT_3D ( 'NONE', #13610, #34095, #43179 ) ;
#25605=ORIENTED_EDGE ( 'NONE', *, *, #35255, .F. ) ;
#25606=CARTESIAN_POINT ( 'NONE',  ( -15.85727731971092780, -5.536956232915663634, 11.92852523610001647 ) ) ;
#25607=ORIENTED_EDGE ( 'NONE', *, *, #50078, .F. ) ;
#25608=EDGE_CURVE ( 'NONE', #54304, #7819, #3874, .T. ) ;
#25609=AXIS2_PLACEMENT_3D ( 'NONE', #50791, #12485, #17018 ) ;
#25610=DIRECTION ( 'NONE',  ( -0.5449076811759708816, 0.6444004775717707689, 0.5364919789714475140 ) ) ;
#25611=CARTESIAN_POINT ( 'NONE',  ( -21.59172106477361908, 2.229229656569007734, 4.997765353639686658 ) ) ;
#25612=VECTOR ( 'NONE', #23747, 999.9999999999998863 ) ;
#25613=ORIENTED_EDGE ( 'NONE', *, *, #17522, .T. ) ;
#25614=EDGE_CURVE ( 'NONE', #46401, #16128, #54428, .T. ) ;
#25615=LINE ( 'NONE', #42941, #2330 ) ;
#25616=LINE ( 'NONE', #38116, #13933 ) ;
#25617=LINE ( 'NONE', #52850, #11047 ) ;
#25618=EDGE_CURVE ( 'NONE', #38527, #23133, #45936, .T. ) ;
#25619=VERTEX_POINT ( 'NONE', #32856 ) ;
#25620=PLANE ( 'NONE',  #47337 ) ;
#25621=ADVANCED_FACE ( 'NONE', ( #50174 ), #7045, .F. ) ;
#25622=LINE ( 'NONE', #52326, #51216 ) ;
#25624=DIRECTION ( 'NONE',  ( 0.007781995580012663651, 0.000000000000000000, -0.9999697198139515519 ) ) ;
#25625=DIRECTION ( 'NONE',  ( -0.5364919789714478471, 0.6444004775717705469, -0.5449076811759709926 ) ) ;
#25626=CARTESIAN_POINT ( 'NONE',  ( -11.72846197273706537, -3.432230869623159819, 6.870540248819963836 ) ) ;
#25627=LINE ( 'NONE', #55177, #16770 ) ;
#25628=ORIENTED_EDGE ( 'NONE', *, *, #54297, .F. ) ;
#25629=DIRECTION ( 'NONE',  ( 0.007781995580012663651, 0.000000000000000000, -0.9999697198139515519 ) ) ;
#25630=CARTESIAN_POINT ( 'NONE',  ( 2.072287782118878319, 0.000000000000000000, -2.950529333540147015 ) ) ;
#25631=DIRECTION ( 'NONE',  ( -0.005002170337468016433, -0.7660444431189770143, 0.6427681459581293666 ) ) ;
#25632=EDGE_LOOP ( 'NONE', ( #47, #34599, #16109, #9951 ) ) ;
#25633=LINE ( 'NONE', #35027, #19324 ) ;
#25634=CARTESIAN_POINT ( 'NONE',  ( 2.072287782118878319, 0.000000000000000000, -2.950529333540147015 ) ) ;
#25635=EDGE_LOOP ( 'NONE', ( #6814, #30191, #4844, #54849 ) ) ;
#25637=DIRECTION ( 'NONE',  ( 0.007781995580012663651, -3.146120232559066537E-19, -0.9999697198139514409 ) ) ;
#25638=VECTOR ( 'NONE', #51436, 1000.000000000000227 ) ;
#25639=EDGE_CURVE ( 'NONE', #46062, #25455, #37385, .T. ) ;
#25640=CARTESIAN_POINT ( 'NONE',  ( -16.33317936670417225, 0.000000000000000000, 13.31440848639340224 ) ) ;
#25643=ORIENTED_EDGE ( 'NONE', *, *, #41587, .F. ) ;
#25644=FACE_OUTER_BOUND ( 'NONE', #49140, .T. ) ;
#25645=PLANE ( 'NONE',  #17741 ) ;
#25646=AXIS2_PLACEMENT_3D ( 'NONE', #32991, #1506, #50303 ) ;
#25647=CARTESIAN_POINT ( 'NONE',  ( -17.16584333050165867, 0.2864062442990034651, 4.019159061553319034 ) ) ;
#25648=EDGE_CURVE ( 'NONE', #6528, #40301, #50477, .T. ) ;
#25649=VECTOR ( 'NONE', #27703, 1000.000000000000227 ) ;
#25650=CARTESIAN_POINT ( 'NONE',  ( -11.79385045274640653, 0.000000000000000000, 1.404636026004276284 ) ) ;
#25651=VECTOR ( 'NONE', #43105, 1000.000000000000227 ) ;
#25652=LINE ( 'NONE', #43533, #47331 ) ;
#25653=ADVANCED_FACE ( 'NONE', ( #4463 ), #13534, .F. ) ;
#25654=LINE ( 'NONE', #11755, #50293 ) ;
#25655=VERTEX_POINT ( 'NONE', #753 ) ;
#25656=CARTESIAN_POINT ( 'NONE',  ( -19.83058694132466115, 4.495856970884009485, 11.96266175778294816 ) ) ;
#25657=EDGE_CURVE ( 'NONE', #41831, #42740, #17501, .T. ) ;
#25658=EDGE_CURVE ( 'NONE', #53603, #7239, #52438, .T. ) ;
#25659=VECTOR ( 'NONE', #31953, 999.9999999999998863 ) ;
#25660=CARTESIAN_POINT ( 'NONE',  ( -16.53317331066696383, 0.000000000000000000, 13.31285208727739899 ) ) ;
#25661=VECTOR ( 'NONE', #28425, 1000.000000000000227 ) ;
#25662=ORIENTED_EDGE ( 'NONE', *, *, #17021, .T. ) ;
#25663=CARTESIAN_POINT ( 'NONE',  ( -21.47263955680318404, 0.000000000000000000, 5.022634149262071190 ) ) ;
#25664=LINE ( 'NONE', #56063, #9587 ) ;
#25665=DIRECTION ( 'NONE',  ( 0.005961354470445682716, -0.6427876096865404731, -0.7660212471507180654 ) ) ;
#25666=ORIENTED_EDGE ( 'NONE', *, *, #50126, .F. ) ;
#25668=DIRECTION ( 'NONE',  ( 0.9999697198139515519, 0.000000000000000000, 0.007781995580013368816 ) ) ;
#25669=VECTOR ( 'NONE', #32878, 1000.000000000000227 ) ;
#25670=ORIENTED_EDGE ( 'NONE', *, *, #35106, .T. ) ;
#25671=AXIS2_PLACEMENT_3D ( 'NONE', #26304, #17500, #8151 ) ;
#25672=EDGE_CURVE ( 'NONE', #36758, #23095, #34837, .T. ) ;
#25673=ORIENTED_EDGE ( 'NONE', *, *, #19176, .F. ) ;
#25674=VERTEX_POINT ( 'NONE', #8735 ) ;
#25675=VERTEX_POINT ( 'NONE', #56135 ) ;
#25676=CARTESIAN_POINT ( 'NONE',  ( -21.47419595591918906, 0.000000000000000000, 5.222628093224860102 ) ) ;
#25677=ORIENTED_EDGE ( 'NONE', *, *, #9618, .F. ) ;
#25678=AXIS2_PLACEMENT_3D ( 'NONE', #6100, #1787, #36183 ) ;
#25681=PLANE ( 'NONE',  #11363 ) ;
#25683=PLANE ( 'NONE',  #26628 ) ;
#25684=AXIS2_PLACEMENT_3D ( 'NONE', #34395, #52282, #25575 ) ;
#25685=ORIENTED_EDGE ( 'NONE', *, *, #26188, .F. ) ;
#25686=CARTESIAN_POINT ( 'NONE',  ( -33.59211796935609584, 0.000000000000000000, 9.929640529607549837 ) ) ;
#25688=DIRECTION ( 'NONE',  ( -0.6427681459581293666, -0.7660444431189770143, -0.005002170337467561935 ) ) ;
#25689=CARTESIAN_POINT ( 'NONE',  ( -15.93671887550372013, -0.1191753592594204797, 9.228371760044637995 ) ) ;
#25690=VECTOR ( 'NONE', #3397, 1000.000000000000000 ) ;
#25691=FACE_OUTER_BOUND ( 'NONE', #18002, .T. ) ;
#25692=ORIENTED_EDGE ( 'NONE', *, *, #12877, .T. ) ;
#25693=AXIS2_PLACEMENT_3D ( 'NONE', #27293, #633, #35536 ) ;
#25694=AXIS2_PLACEMENT_3D ( 'NONE', #35233, #43194, #581 ) ;
#25695=ORIENTED_EDGE ( 'NONE', *, *, #5405, .T. ) ;
#25696=CARTESIAN_POINT ( 'NONE',  ( -8.875996589204540044, 0.000000000000000000, 10.41778544861944233 ) ) ;
#25697=EDGE_CURVE ( 'NONE', #26758, #15321, #17224, .T. ) ;
#25698=DIRECTION ( 'NONE',  ( -0.7660212471507179544, -0.6427876096865405842, -0.005961354470445141482 ) ) ;
#25699=LINE ( 'NONE', #38189, #33328 ) ;
#25700=VECTOR ( 'NONE', #29219, 999.9999999999998863 ) ;
#25701=VECTOR ( 'NONE', #13311, 1000.000000000000000 ) ;
#25702=DIRECTION ( 'NONE',  ( 0.5364919789714477361, 0.6444004775717706579, 0.5449076811759711036 ) ) ;
#25703=CARTESIAN_POINT ( 'NONE',  ( -13.22668023795434067, 0.000000000000000000, 6.394808377013974976 ) ) ;
#25704=CARTESIAN_POINT ( 'NONE',  ( -18.66354898467281132, 0.000000000000000000, 14.21960318569776582 ) ) ;
#25705=EDGE_LOOP ( 'NONE', ( #52805, #36626, #51445, #56194 ) ) ;
#25706=CARTESIAN_POINT ( 'NONE',  ( -22.15388463660123719, -4.241740624735662379, 5.351308525247191916 ) ) ;
#25707=DIRECTION ( 'NONE',  ( 0.7660212471507180654, -0.6427876096865404731, 0.005961354470445141482 ) ) ;
#25708=EDGE_LOOP ( 'NONE', ( #50280, #34062, #6423, #6818 ) ) ;
#25709=EDGE_CURVE ( 'NONE', #9950, #33621, #21770, .T. ) ;
#25710=DIRECTION ( 'NONE',  ( 0.9999697198139515519, 0.000000000000000000, 0.007781995580013368816 ) ) ;
#25711=LINE ( 'NONE', #423, #41464 ) ;
#25712=LINE ( 'NONE', #20880, #26840 ) ;
#25714=EDGE_CURVE ( 'NONE', #20361, #52593, #22352, .T. ) ;
#25715=DIRECTION ( 'NONE',  ( -0.5364919789714478471, 0.6444004775717705469, -0.5449076811759709926 ) ) ;
#25716=ORIENTED_EDGE ( 'NONE', *, *, #49039, .T. ) ;
#25717=VECTOR ( 'NONE', #48878, 1000.000000000000114 ) ;
#25718=ORIENTED_EDGE ( 'NONE', *, *, #2580, .F. ) ;
#25719=DIRECTION ( 'NONE',  ( 0.000000000000000000, -0.000000000000000000, -1.000000000000000000 ) ) ;
#25720=DIRECTION ( 'NONE',  ( -0.5449076811759708816, 0.6444004775717707689, 0.5364919789714475140 ) ) ;
#25721=DIRECTION ( 'NONE',  ( 0.007781995580012662783, 0.000000000000000000, -0.9999697198139514409 ) ) ;
#25722=EDGE_CURVE ( 'NONE', #11534, #55481, #39674, .T. ) ;
#25723=AXIS2_PLACEMENT_3D ( 'NONE', #27503, #44532, #6484 ) ;
#25724=ADVANCED_FACE ( 'NONE', ( #16966 ), #18070, .F. ) ;
#25725=FACE_OUTER_BOUND ( 'NONE', #52654, .T. ) ;
#25726=ADVANCED_FACE ( 'NONE', ( #30006 ), #9003, .F. ) ;
#25727=CARTESIAN_POINT ( 'NONE',  ( -16.89925026227929195, -0.1191753592594197858, 13.49466922669627422 ) ) ;
#25728=AXIS2_PLACEMENT_3D ( 'NONE', #16739, #7961, #32934 ) ;
#25730=DIRECTION ( 'NONE',  ( 0.005961354470445682716, -0.6427876096865404731, -0.7660212471507180654 ) ) ;
#25731=EDGE_CURVE ( 'NONE', #35444, #32268, #47315, .T. ) ;
#25732=VERTEX_POINT ( 'NONE', #51594 ) ;
#25733=LINE ( 'NONE', #12098, #12355 ) ;
#25734=CARTESIAN_POINT ( 'NONE',  ( -27.99845268667336384, -0.1191753592594197858, 7.657176279295684118 ) ) ;
#25735=VECTOR ( 'NONE', #33368, 1000.000000000000227 ) ;
#25736=PLANE ( 'NONE',  #55563 ) ;
#25737=ORIENTED_EDGE ( 'NONE', *, *, #7978, .F. ) ;
#25738=CARTESIAN_POINT ( 'NONE',  ( -15.40103151951671734, 0.000000000000000000, 12.95233060667165681 ) ) ;
#25739=VECTOR ( 'NONE', #824, 1000.000000000000227 ) ;
#25741=ORIENTED_EDGE ( 'NONE', *, *, #21286, .T. ) ;
#25742=ORIENTED_EDGE ( 'NONE', *, *, #35725, .F. ) ;
#25743=ADVANCED_FACE ( 'NONE', ( #4186 ), #25752, .F. ) ;
#25744=VECTOR ( 'NONE', #34721, 999.9999999999998863 ) ;
#25745=VERTEX_POINT ( 'NONE', #26054 ) ;
#25746=ORIENTED_EDGE ( 'NONE', *, *, #30329, .T. ) ;
#25747=VECTOR ( 'NONE', #27125, 1000.000000000000114 ) ;
#25748=ORIENTED_EDGE ( 'NONE', *, *, #41514, .T. ) ;
#25749=ORIENTED_EDGE ( 'NONE', *, *, #44720, .F. ) ;
#25750=LINE ( 'NONE', #17222, #26009 ) ;
#25751=CARTESIAN_POINT ( 'NONE',  ( -12.23851102634202448, -0.1191753592594197858, 11.68427982808754884 ) ) ;
#25752=PLANE ( 'NONE',  #28568 ) ;
#25753=ORIENTED_EDGE ( 'NONE', *, *, #2591, .F. ) ;
#25754=CARTESIAN_POINT ( 'NONE',  ( -14.15020592462595062, 0.000000000000000000, 5.648957146962426457 ) ) ;
#25755=ORIENTED_EDGE ( 'NONE', *, *, #9896, .F. ) ;
#25756=DIRECTION ( 'NONE',  ( 0.005961354470445682716, -0.6427876096865404731, -0.7660212471507180654 ) ) ;
#25757=EDGE_LOOP ( 'NONE', ( #10535, #52214, #30176, #25269 ) ) ;
#25758=FACE_OUTER_BOUND ( 'NONE', #26108, .T. ) ;
#25759=AXIS2_PLACEMENT_3D ( 'NONE', #4024, #21348, #8569 ) ;
#25760=PLANE ( 'NONE',  #42806 ) ;
#25761=DIRECTION ( 'NONE',  ( -0.5449076811759708816, 0.6444004775717707689, 0.5364919789714475140 ) ) ;
#25762=EDGE_LOOP ( 'NONE', ( #36495, #41237, #35616, #24459 ) ) ;
#25763=PLANE ( 'NONE',  #27411 ) ;
#25764=VECTOR ( 'NONE', #19960, 999.9999999999998863 ) ;
#25765=ORIENTED_EDGE ( 'NONE', *, *, #49458, .F. ) ;
#25766=CARTESIAN_POINT ( 'NONE',  ( -18.34187781110085069, 0.000000000000000000, 6.893658810118608038 ) ) ;
#25767=EDGE_CURVE ( 'NONE', #17866, #8893, #43367, .T. ) ;
#25768=DIRECTION ( 'NONE',  ( -0.005002170337468016433, -0.7660444431189770143, 0.6427681459581293666 ) ) ;
#25769=AXIS2_PLACEMENT_3D ( 'NONE', #49296, #43909, #36510 ) ;
#25770=FACE_OUTER_BOUND ( 'NONE', #2065, .T. ) ;
#25771=DIRECTION ( 'NONE',  ( 0.000000000000000000, -0.000000000000000000, -1.000000000000000000 ) ) ;
#25773=FACE_OUTER_BOUND ( 'NONE', #34775, .T. ) ;
#25775=AXIS2_PLACEMENT_3D ( 'NONE', #2034, #19089, #15658 ) ;
#25778=CARTESIAN_POINT ( 'NONE',  ( -16.27471411925786882, 0.000000000000000000, 5.801749746533357843 ) ) ;
#25779=EDGE_LOOP ( 'NONE', ( #40008, #4117, #26479, #41478, #39027 ) ) ;
#25780=EDGE_CURVE ( 'NONE', #51442, #47161, #161, .T. ) ;
#25781=ADVANCED_FACE ( 'NONE', ( #33006 ), #31702, .F. ) ;
#25782=VECTOR ( 'NONE', #43991, 999.9999999999998863 ) ;
#25783=FACE_OUTER_BOUND ( 'NONE', #1907, .T. ) ;
#25784=LINE ( 'NONE', #35421, #26928 ) ;
#25785=FACE_OUTER_BOUND ( 'NONE', #39082, .T. ) ;
#25786=CARTESIAN_POINT ( 'NONE',  ( -12.23851102634202448, -0.1191753592594197858, 11.68427982808754884 ) ) ;
#25787=CARTESIAN_POINT ( 'NONE',  ( -16.81267852042391198, -0.1191753592594197858, 3.312241722634738039 ) ) ;
#25788=EDGE_CURVE ( 'NONE', #3308, #32995, #14647, .T. ) ;
#25789=DIRECTION ( 'NONE',  ( 0.000000000000000000, -0.000000000000000000, -1.000000000000000000 ) ) ;
#25790=AXIS2_PLACEMENT_3D ( 'NONE', #11814, #42749, #38503 ) ;
#25791=DIRECTION ( 'NONE',  ( 0.007781995580012663651, 0.000000000000000000, -0.9999697198139515519 ) ) ;
#25792=VECTOR ( 'NONE', #26279, 1000.000000000000227 ) ;
#25794=ORIENTED_EDGE ( 'NONE', *, *, #31764, .T. ) ;
#25796=DIRECTION ( 'NONE',  ( -0.5364919789714478471, 0.6444004775717705469, -0.5449076811759709926 ) ) ;
#25797=DIRECTION ( 'NONE',  ( 0.6427681459581294776, -0.7660444431189769032, 0.005002170337467562802 ) ) ;
#25798=CARTESIAN_POINT ( 'NONE',  ( -18.42254072940788134, 0.1245042932765029059, 3.833899844102495624 ) ) ;
#25799=ADVANCED_FACE ( 'NONE', ( #11708 ), #10108, .F. ) ;
#25800=LINE ( 'NONE', #43127, #18524 ) ;
#25801=DIRECTION ( 'NONE',  ( 0.000000000000000000, -0.000000000000000000, -1.000000000000000000 ) ) ;
#25802=DIRECTION ( 'NONE',  ( 0.9999697198139515519, 0.000000000000000000, 0.007781995580013368816 ) ) ;
#25803=ORIENTED_EDGE ( 'NONE', *, *, #9910, .T. ) ;
#25804=EDGE_CURVE ( 'NONE', #39023, #20767, #10400, .T. ) ;
#25805=VECTOR ( 'NONE', #1982, 1000.000000000000227 ) ;
#25806=DIRECTION ( 'NONE',  ( -0.005961354470445682716, -0.6427876096865404731, 0.7660212471507180654 ) ) ;
#25807=FACE_OUTER_BOUND ( 'NONE', #9228, .T. ) ;
#25808=VERTEX_POINT ( 'NONE', #15978 ) ;
#25809=VECTOR ( 'NONE', #21058, 999.9999999999998863 ) ;
#25810=ADVANCED_FACE ( 'NONE', ( #36501 ), #53820, .F. ) ;
#25811=EDGE_LOOP ( 'NONE', ( #12426, #36420, #54386, #51243 ) ) ;
#25812=LINE ( 'NONE', #13849, #49201 ) ;
#25813=VECTOR ( 'NONE', #54516, 1000.000000000000227 ) ;
#25814=ADVANCED_FACE ( 'NONE', ( #29024 ), #50324, .F. ) ;
#25815=ORIENTED_EDGE ( 'NONE', *, *, #30628, .T. ) ;
#25816=ORIENTED_EDGE ( 'NONE', *, *, #48870, .F. ) ;
#25817=VERTEX_POINT ( 'NONE', #48749 ) ;
#25818=VECTOR ( 'NONE', #34861, 1000.000000000000227 ) ;
#25819=ORIENTED_EDGE ( 'NONE', *, *, #2104, .F. ) ;
#25820=CARTESIAN_POINT ( 'NONE',  ( -13.07066190154808361, 0.000000000000000000, 12.04713590736729678 ) ) ;
#25821=VECTOR ( 'NONE', #10995, 999.9999999999998863 ) ;
#25822=ORIENTED_EDGE ( 'NONE', *, *, #3561, .F. ) ;
#25823=CARTESIAN_POINT ( 'NONE',  ( -13.66389425413188086, 0.000000000000000000, 2.867411191963296080 ) ) ;
#25825=VECTOR ( 'NONE', #3209, 999.9999999999998863 ) ;
#25826=ORIENTED_EDGE ( 'NONE', *, *, #6616, .T. ) ;
#25827=ORIENTED_EDGE ( 'NONE', *, *, #42096, .F. ) ;
#25828=VECTOR ( 'NONE', #31872, 999.9999999999998863 ) ;
#25829=AXIS2_PLACEMENT_3D ( 'NONE', #12171, #7344, #37756 ) ;
#25830=CARTESIAN_POINT ( 'NONE',  ( -17.36532418587302473, -0.1191753592594177458, 13.67570816655714516 ) ) ;
#25831=VERTEX_POINT ( 'NONE', #11441 ) ;
#25832=CARTESIAN_POINT ( 'NONE',  ( -11.87243407472968926, 0.000000000000000000, 11.50246268866867361 ) ) ;
#25833=ORIENTED_EDGE ( 'NONE', *, *, #12242, .T. ) ;
#25834=DIRECTION ( 'NONE',  ( 0.6427681459581294776, -0.7660444431189769032, 0.005002170337467562802 ) ) ;
#25835=EDGE_CURVE ( 'NONE', #4032, #8206, #23185, .T. ) ;
#25836=EDGE_LOOP ( 'NONE', ( #5065, #26382, #30533, #4255 ) ) ;
#25837=DIRECTION ( 'NONE',  ( 0.007781995580012662783, 0.000000000000000000, -0.9999697198139514409 ) ) ;
#25838=EDGE_CURVE ( 'NONE', #83, #27011, #46068, .T. ) ;
#25839=AXIS2_PLACEMENT_3D ( 'NONE', #37165, #41691, #6792 ) ;
#25840=CARTESIAN_POINT ( 'NONE',  ( -16.50360637555614218, -4.727446477803164626, 3.141052004737669545 ) ) ;
#25841=VERTEX_POINT ( 'NONE', #2879 ) ;
#25842=PLANE ( 'NONE',  #48502 ) ;
#25843=DIRECTION ( 'NONE',  ( 0.7660212471507180654, -0.6427876096865404731, 0.005961354470445141482 ) ) ;
#25844=DIRECTION ( 'NONE',  ( 0.5364919789714477361, 0.6444004775717706579, 0.5449076811759711036 ) ) ;
#25845=VECTOR ( 'NONE', #9852, 1000.000000000000227 ) ;
#25846=DIRECTION ( 'NONE',  ( -0.9999697198139514409, -0.000000000000000000, -0.007781995580013368816 ) ) ;
#25847=ORIENTED_EDGE ( 'NONE', *, *, #28402, .T. ) ;
#25848=VECTOR ( 'NONE', #40857, 999.9999999999998863 ) ;
#25849=ADVANCED_FACE ( 'NONE', ( #1600 ), #20210, .F. ) ;
#25850=EDGE_CURVE ( 'NONE', #53959, #30417, #36241, .T. ) ;
#25851=EDGE_CURVE ( 'NONE', #24469, #35938, #22619, .T. ) ;
#25852=FACE_OUTER_BOUND ( 'NONE', #1250, .T. ) ;
#25853=CARTESIAN_POINT ( 'NONE',  ( -19.60912206198628027, -0.1191753592594197858, 4.398475361799976113 ) ) ;
#25854=CARTESIAN_POINT ( 'NONE',  ( -22.40634380310664397, 0.000000000000000000, 5.584705972946605534 ) ) ;
#25855=CARTESIAN_POINT ( 'NONE',  ( 2.072287782118878319, 0.000000000000000000, -2.950529333540147015 ) ) ;
#25856=AXIS2_PLACEMENT_3D ( 'NONE', #13606, #26971, #52512 ) ;
#25857=DIRECTION ( 'NONE',  ( -0.7660212471507179544, -0.6427876096865405842, -0.005961354470445141482 ) ) ;
#25858=EDGE_CURVE ( 'NONE', #47896, #43283, #44461, .T. ) ;
#25859=DIRECTION ( 'NONE',  ( -0.6427681459581293666, -0.7660444431189770143, -0.005002170337467561935 ) ) ;
#25860=DIRECTION ( 'NONE',  ( -0.5364919789714478471, 0.6444004775717705469, -0.5449076811759709926 ) ) ;
#25861=DIRECTION ( 'NONE',  ( 0.005961354470445682716, -0.6427876096865404731, -0.7660212471507180654 ) ) ;
#25862=AXIS2_PLACEMENT_3D ( 'NONE', #9029, #52468, #504 ) ;
#25863=CARTESIAN_POINT ( 'NONE',  ( -8.409922665610809034, 0.000000000000000000, 10.23674650875856962 ) ) ;
#25864=EDGE_LOOP ( 'NONE', ( #37689, #34969, #8889, #2797 ) ) ;
#25866=VECTOR ( 'NONE', #30944, 1000.000000000000114 ) ;
#25867=LINE ( 'NONE', #4296, #17836 ) ;
#25868=ORIENTED_EDGE ( 'NONE', *, *, #25478, .F. ) ;
#25869=CARTESIAN_POINT ( 'NONE',  ( -11.43033398677498091, -0.3560938001956562293, 1.706272219544479718 ) ) ;
#25870=LINE ( 'NONE', #30695, #35482 ) ;
#25871=VECTOR ( 'NONE', #9734, 1000.000000000000000 ) ;
#25872=CARTESIAN_POINT ( 'NONE',  ( -17.74560456716937296, 0.000000000000000000, 3.774316574337878372 ) ) ;
#25873=FACE_OUTER_BOUND ( 'NONE', #12347, .T. ) ;
#25874=EDGE_CURVE ( 'NONE', #12052, #23249, #35676, .T. ) ;
#25875=CARTESIAN_POINT ( 'NONE',  ( -26.13337879274045505, 0.000000000000000000, 6.833023547870798353 ) ) ;
#25876=EDGE_LOOP ( 'NONE', ( #15664, #45368, #17087, #22137 ) ) ;
#25877=AXIS2_PLACEMENT_3D ( 'NONE', #52813, #9107, #52284 ) ;
#25878=EDGE_CURVE ( 'NONE', #53765, #51817, #45051, .T. ) ;
#25879=AXIS2_PLACEMENT_3D ( 'NONE', #11539, #20312, #20621 ) ;
#25880=ORIENTED_EDGE ( 'NONE', *, *, #3393, .F. ) ;
#25881=EDGE_CURVE ( 'NONE', #33602, #19374, #1298, .T. ) ;
#25882=PLANE ( 'NONE',  #44981 ) ;
#25883=CARTESIAN_POINT ( 'NONE',  ( -14.17572954220636205, -0.8417996532631565332, 3.569803139150924398 ) ) ;
#25884=VERTEX_POINT ( 'NONE', #22883 ) ;
#25885=DIRECTION ( 'NONE',  ( 0.000000000000000000, -0.000000000000000000, -1.000000000000000000 ) ) ;
#25886=EDGE_CURVE ( 'NONE', #53080, #44261, #40207, .T. ) ;
#25887=EDGE_LOOP ( 'NONE', ( #13546, #8478, #54955, #13110 ) ) ;
#25888=PLANE ( 'NONE',  #14082 ) ;
#25889=ORIENTED_EDGE ( 'NONE', *, *, #16958, .T. ) ;
#25890=CARTESIAN_POINT ( 'NONE',  ( -17.74482636761137044, -0.1191753592594197858, 3.674319602356483916 ) ) ;
#25891=EDGE_CURVE ( 'NONE', #34091, #17338, #37845, .T. ) ;
#25892=AXIS2_PLACEMENT_3D ( 'NONE', #49815, #41006, #10913 ) ;
#25894=VERTEX_POINT ( 'NONE', #12561 ) ;
#25895=ORIENTED_EDGE ( 'NONE', *, *, #5132, .T. ) ;
#25896=VECTOR ( 'NONE', #34122, 999.9999999999998863 ) ;
#25897=DIRECTION ( 'NONE',  ( -0.8531650599175529814, -0.4028455766673920135, 0.3313982828793697877 ) ) ;
#25898=PLANE ( 'NONE',  #26896 ) ;
#25899=VECTOR ( 'NONE', #2151, 1000.000000000000000 ) ;
#25900=CARTESIAN_POINT ( 'NONE',  ( -12.13851405436063047, 0.000000000000000000, 11.68505802764555135 ) ) ;
#25901=LINE ( 'NONE', #33838, #42985 ) ;
#25902=ORIENTED_EDGE ( 'NONE', *, *, #35397, .T. ) ;
#25903=VECTOR ( 'NONE', #36893, 999.9999999999998863 ) ;
#25904=ORIENTED_EDGE ( 'NONE', *, *, #11679, .T. ) ;
#25905=VERTEX_POINT ( 'NONE', #51465 ) ;
#25907=AXIS2_PLACEMENT_3D ( 'NONE', #31895, #30014, #10038 ) ;
#25908=DIRECTION ( 'NONE',  ( -0.9999697198139514409, -0.000000000000000000, -0.007781995580013368816 ) ) ;
#25909=EDGE_LOOP ( 'NONE', ( #44631, #12897, #31130, #44108 ) ) ;
#25910=FACE_OUTER_BOUND ( 'NONE', #30235, .T. ) ;
#25911=EDGE_LOOP ( 'NONE', ( #37581, #35067, #6965, #7526 ) ) ;
#25912=DIRECTION ( 'NONE',  ( 0.6427681459581294776, -0.7660444431189769032, 0.005002170337467562802 ) ) ;
#25913=DIRECTION ( 'NONE',  ( 0.000000000000000000, -1.000000000000000000, 0.000000000000000000 ) ) ;
#25914=AXIS2_PLACEMENT_3D ( 'NONE', #22647, #48785, #35713 ) ;
#25915=EDGE_LOOP ( 'NONE', ( #32762, #40571, #4665, #39083 ) ) ;
#25916=VECTOR ( 'NONE', #8150, 1000.000000000000114 ) ;
#25917=DIRECTION ( 'NONE',  ( 0.007781995580012662783, 0.000000000000000000, -0.9999697198139514409 ) ) ;
#25918=VECTOR ( 'NONE', #51059, 999.9999999999998863 ) ;
#25919=EDGE_LOOP ( 'NONE', ( #35364, #53875, #46565, #50170 ) ) ;
#25920=AXIS2_PLACEMENT_3D ( 'NONE', #23988, #19737, #53529 ) ;
#25921=CARTESIAN_POINT ( 'NONE',  ( -9.808144436391993182, 0.000000000000000000, 10.77986332834118777 ) ) ;
#25922=AXIS2_PLACEMENT_3D ( 'NONE', #23609, #18221, #1479 ) ;
#25923=ORIENTED_EDGE ( 'NONE', *, *, #11979, .F. ) ;
#25924=CARTESIAN_POINT ( 'NONE',  ( -20.54049170961573267, 0.000000000000000000, 4.660556269540326646 ) ) ;
#25925=CARTESIAN_POINT ( 'NONE',  ( -15.07504926568683423, 0.000000000000000000, 5.072421676205853380 ) ) ;
#25926=CARTESIAN_POINT ( 'NONE',  ( -16.79925329029790149, 0.000000000000000000, 13.49544742625427496 ) ) ;
#25927=ORIENTED_EDGE ( 'NONE', *, *, #52591, .T. ) ;
#25928=EDGE_CURVE ( 'NONE', #49012, #17790, #51163, .T. ) ;
#25929=CARTESIAN_POINT ( 'NONE',  ( -26.13415699229845757, -0.1191753592594197858, 6.933020519852192365 ) ) ;
#25930=CARTESIAN_POINT ( 'NONE',  ( -27.06552663992790997, 0.000000000000000000, 7.195101427592543786 ) ) ;
#25931=FACE_OUTER_BOUND ( 'NONE', #53419, .T. ) ;
#25932=LINE ( 'NONE', #17118, #27731 ) ;
#25933=EDGE_CURVE ( 'NONE', #55170, #47218, #42637, .T. ) ;
#25934=LINE ( 'NONE', #35018, #31247 ) ;
#25935=DIRECTION ( 'NONE',  ( 0.000000000000000000, -1.000000000000000000, 0.000000000000000000 ) ) ;
#25937=FACE_OUTER_BOUND ( 'NONE', #55842, .T. ) ;
#25938=VERTEX_POINT ( 'NONE', #8283 ) ;
#25939=DIRECTION ( 'NONE',  ( 0.000000000000000000, -0.000000000000000000, -1.000000000000000000 ) ) ;
#25940=VECTOR ( 'NONE', #33222, 1000.000000000000227 ) ;
#25942=CARTESIAN_POINT ( 'NONE',  ( -21.37767238905108513, -3.270328918600657886, 10.35291257913092977 ) ) ;
#25943=ORIENTED_EDGE ( 'NONE', *, *, #36885, .T. ) ;
#25945=CARTESIAN_POINT ( 'NONE',  ( -18.19747506107908563, 0.000000000000000000, 14.03856424583689311 ) ) ;
#25946=VECTOR ( 'NONE', #54591, 999.9999999999998863 ) ;
#25947=ORIENTED_EDGE ( 'NONE', *, *, #41429, .T. ) ;
#25948=DIRECTION ( 'NONE',  ( 0.6427681459581294776, -0.7660444431189769032, 0.005002170337467562802 ) ) ;
#25949=AXIS2_PLACEMENT_3D ( 'NONE', #36673, #2832, #45449 ) ;
#25950=DIRECTION ( 'NONE',  ( 0.5364919789714477361, 0.6444004775717706579, 0.5449076811759711036 ) ) ;
#25952=ORIENTED_EDGE ( 'NONE', *, *, #8217, .T. ) ;
#25953=AXIS2_PLACEMENT_3D ( 'NONE', #41955, #12464, #20092 ) ;
#25954=VECTOR ( 'NONE', #26818, 1000.000000000000227 ) ;
#25955=ORIENTED_EDGE ( 'NONE', *, *, #20818, .T. ) ;
#25957=CARTESIAN_POINT ( 'NONE',  ( -20.79160881769003666, -2.622721114510659479, 4.873809532974441971 ) ) ;
#25959=VECTOR ( 'NONE', #13763, 1000.000000000000227 ) ;
#25960=DIRECTION ( 'NONE',  ( 0.005002170337468016433, -0.7660444431189770143, -0.6427681459581293666 ) ) ;
#25961=VECTOR ( 'NONE', #26901, 1000.000000000000227 ) ;
#25962=LINE ( 'NONE', #39002, #33750 ) ;
#25963=DIRECTION ( 'NONE',  ( 0.000000000000000000, -1.000000000000000000, 0.000000000000000000 ) ) ;
#25965=LINE ( 'NONE', #55467, #51001 ) ;
#25966=EDGE_CURVE ( 'NONE', #21242, #47865, #16512, .T. ) ;
#25967=VECTOR ( 'NONE', #11697, 999.9999999999998863 ) ;
#25968=VECTOR ( 'NONE', #33958, 1000.000000000000227 ) ;
#25969=CARTESIAN_POINT ( 'NONE',  ( -17.67724697029697367, 0.000000000000000000, 6.898831121002622524 ) ) ;
#25970=ORIENTED_EDGE ( 'NONE', *, *, #18873, .T. ) ;
#25971=ADVANCED_FACE ( 'NONE', ( #3182 ), #42379, .F. ) ;
#25972=DIRECTION ( 'NONE',  ( -0.005961354470445682716, -0.6427876096865404731, 0.7660212471507180654 ) ) ;
#25973=LINE ( 'NONE', #29080, #1422 ) ;
#25974=FACE_OUTER_BOUND ( 'NONE', #4711, .T. ) ;
#25975=ORIENTED_EDGE ( 'NONE', *, *, #5406, .F. ) ;
#25976=FACE_OUTER_BOUND ( 'NONE', #34737, .T. ) ;
#25977=EDGE_CURVE ( 'NONE', #54798, #7497, #25596, .T. ) ;
#25978=ORIENTED_EDGE ( 'NONE', *, *, #15289, .T. ) ;
#25979=VECTOR ( 'NONE', #24892, 999.9999999999998863 ) ;
#25980=EDGE_LOOP ( 'NONE', ( #16000, #12627, #52140, #38381 ) ) ;
#25981=ORIENTED_EDGE ( 'NONE', *, *, #38789, .F. ) ;
#25982=ORIENTED_EDGE ( 'NONE', *, *, #2687, .T. ) ;
#25983=DIRECTION ( 'NONE',  ( 0.5364919789714477361, 0.6444004775717706579, 0.5449076811759711036 ) ) ;
#25984=VECTOR ( 'NONE', #9088, 1000.000000000000114 ) ;
#25985=ORIENTED_EDGE ( 'NONE', *, *, #17742, .T. ) ;
#25986=CARTESIAN_POINT ( 'NONE',  ( -12.77353955513438599, 0.000000000000000000, 7.875663101813041855 ) ) ;
#25988=DIRECTION ( 'NONE',  ( -0.9999697198139514409, -0.000000000000000000, -0.007781995580013368816 ) ) ;
#25989=VECTOR ( 'NONE', #36284, 1000.000000000000227 ) ;
#25990=EDGE_LOOP ( 'NONE', ( #52988, #8147, #52486, #50031 ) ) ;
#25991=LINE ( 'NONE', #96, #9398 ) ;
#25992=ORIENTED_EDGE ( 'NONE', *, *, #16073, .T. ) ;
#25993=VECTOR ( 'NONE', #44840, 999.9999999999998863 ) ;
#25994=LINE ( 'NONE', #8666, #27499 ) ;
#25995=CARTESIAN_POINT ( 'NONE',  ( 2.072287782118878319, 0.000000000000000000, -2.950529333540147015 ) ) ;
#25996=LINE ( 'NONE', #9207, #22254 ) ;
#25997=CARTESIAN_POINT ( 'NONE',  ( -19.79569077582305070, 0.000000000000000000, 14.58012466630350445 ) ) ;
#25998=EDGE_CURVE ( 'NONE', #41698, #15410, #43236, .T. ) ;
#25999=LINE ( 'NONE', #39315, #33764 ) ;
#26001=AXIS2_PLACEMENT_3D ( 'NONE', #20013, #7250, #38180 ) ;
#26002=ADVANCED_FACE ( 'NONE', ( #20517 ), #4332, .F. ) ;
#26003=EDGE_LOOP ( 'NONE', ( #33827, #28522, #25947, #16273 ) ) ;
#26004=AXIS2_PLACEMENT_3D ( 'NONE', #51255, #8368, #12376 ) ;
#26005=LINE ( 'NONE', #12648, #30373 ) ;
#26006=FACE_OUTER_BOUND ( 'NONE', #12615, .T. ) ;
#26008=ADVANCED_FACE ( 'NONE', ( #25333 ), #17098, .F. ) ;
#26009=VECTOR ( 'NONE', #9000, 1000.000000000000227 ) ;
#26010=CARTESIAN_POINT ( 'NONE',  ( -31.72626587586518099, 0.000000000000000000, 9.005490826201270949 ) ) ;
#26011=AXIS2_PLACEMENT_3D ( 'NONE', #43278, #17693, #21936 ) ;
#26012=DIRECTION ( 'NONE',  ( 0.007781995580012663651, -3.146120232559066537E-19, -0.9999697198139514409 ) ) ;
#26013=CARTESIAN_POINT ( 'NONE',  ( -9.808144436391993182, 0.000000000000000000, 10.77986332834118777 ) ) ;
#26014=DIRECTION ( 'NONE',  ( 0.5449076811759707706, 0.6444004775717708799, -0.5364919789714476250 ) ) ;
#26015=ORIENTED_EDGE ( 'NONE', *, *, #37193, .F. ) ;
#26016=DIRECTION ( 'NONE',  ( 0.007781995580012662783, 0.000000000000000000, -0.9999697198139514409 ) ) ;
#26017=FACE_OUTER_BOUND ( 'NONE', #6813, .T. ) ;
#26018=ORIENTED_EDGE ( 'NONE', *, *, #9197, .T. ) ;
#26019=PLANE ( 'NONE',  #56066 ) ;
#26022=DIRECTION ( 'NONE',  ( 0.9999697198139515519, 0.000000000000000000, 0.007781995580013368816 ) ) ;
#26023=AXIS2_PLACEMENT_3D ( 'NONE', #3979, #4286, #16762 ) ;
#26024=ADVANCED_FACE ( 'NONE', ( #38384 ), #29305, .F. ) ;
#26025=ORIENTED_EDGE ( 'NONE', *, *, #49948, .F. ) ;
#26026=ORIENTED_EDGE ( 'NONE', *, *, #6200, .F. ) ;
#26027=CARTESIAN_POINT ( 'NONE',  ( -31.72704407542318350, -0.1191753592594197858, 9.105487798182664960 ) ) ;
#26028=LINE ( 'NONE', #31404, #12256 ) ;
#26029=DIRECTION ( 'NONE',  ( 0.9999697198139515519, 0.000000000000000000, 0.007781995580013368816 ) ) ;
#26030=DIRECTION ( 'NONE',  ( 0.005961354470445682716, -0.6427876096865404731, -0.7660212471507180654 ) ) ;
#26031=AXIS2_PLACEMENT_3D ( 'NONE', #15730, #46381, #11500 ) ;
#26032=DIRECTION ( 'NONE',  ( 0.7660212471507180654, -0.6427876096865404731, 0.005961354470445141482 ) ) ;
#26033=CARTESIAN_POINT ( 'NONE',  ( -19.14237710917700142, -3.432230869623161595, 4.207364329806451586 ) ) ;
#26034=CARTESIAN_POINT ( 'NONE',  ( -23.33693525117809386, 0.000000000000000000, 5.746789908705562944 ) ) ;
#26035=ORIENTED_EDGE ( 'NONE', *, *, #2032, .F. ) ;
#26036=FACE_OUTER_BOUND ( 'NONE', #37117, .T. ) ;
#26037=VECTOR ( 'NONE', #22996, 1000.000000000000227 ) ;
#26038=CARTESIAN_POINT ( 'NONE',  ( -15.00929495654107448, 2.714935509636508204, 2.425430953408422408 ) ) ;
#26039=ORIENTED_EDGE ( 'NONE', *, *, #3306, .T. ) ;
#26040=DIRECTION ( 'NONE',  ( 0.000000000000000000, -1.000000000000000000, 0.000000000000000000 ) ) ;
#26041=ORIENTED_EDGE ( 'NONE', *, *, #18334, .T. ) ;
#26042=CARTESIAN_POINT ( 'NONE',  ( -18.66354898467281132, 0.000000000000000000, 14.21960318569776582 ) ) ;
#26043=ORIENTED_EDGE ( 'NONE', *, *, #42389, .F. ) ;
#26044=AXIS2_PLACEMENT_3D ( 'NONE', #2897, #37862, #30921 ) ;
#26045=EDGE_CURVE ( 'NONE', #39606, #24516, #46619, .T. ) ;
#26046=VERTEX_POINT ( 'NONE', #3470 ) ;
#26047=ORIENTED_EDGE ( 'NONE', *, *, #19061, .F. ) ;
#26048=VECTOR ( 'NONE', #32152, 1000.000000000000227 ) ;
#26049=VERTEX_POINT ( 'NONE', #38956 ) ;
#26050=ORIENTED_EDGE ( 'NONE', *, *, #2101, .F. ) ;
#26051=VERTEX_POINT ( 'NONE', #34677 ) ;
#26052=DIRECTION ( 'NONE',  ( 0.000000000000000000, -0.000000000000000000, -1.000000000000000000 ) ) ;
#26053=PLANE ( 'NONE',  #55574 ) ;
#26054=CARTESIAN_POINT ( 'NONE',  ( -10.87032476607480547, 0.000000000000000000, 2.150487256055822805 ) ) ;
#26055=EDGE_CURVE ( 'NONE', #21341, #1854, #52002, .T. ) ;
#26056=VERTEX_POINT ( 'NONE', #13113 ) ;
#26057=DIRECTION ( 'NONE',  ( 0.000000000000000000, -1.000000000000000000, 0.000000000000000000 ) ) ;
#26058=ORIENTED_EDGE ( 'NONE', *, *, #50328, .F. ) ;
#26059=EDGE_CURVE ( 'NONE', #38090, #54919, #16241, .T. ) ;
#26061=EDGE_CURVE ( 'NONE', #47842, #31761, #38100, .T. ) ;
#26062=DIRECTION ( 'NONE',  ( -0.7660212471507179544, -0.6427876096865405842, -0.005961354470445141482 ) ) ;
#26063=LINE ( 'NONE', #43374, #25059 ) ;
#26064=EDGE_CURVE ( 'NONE', #29013, #52907, #12275, .T. ) ;
#26065=ORIENTED_EDGE ( 'NONE', *, *, #48019, .T. ) ;
#26066=LINE ( 'NONE', #51866, #42802 ) ;
#26067=EDGE_LOOP ( 'NONE', ( #11514, #23647, #34146, #34402 ) ) ;
#26068=DIRECTION ( 'NONE',  ( -0.6427681459581293666, -0.7660444431189770143, -0.005002170337467561935 ) ) ;
#26069=EDGE_CURVE ( 'NONE', #36809, #27546, #14254, .T. ) ;
#26070=DIRECTION ( 'NONE',  ( 0.007781995580012663651, 0.000000000000000000, -0.9999697198139515519 ) ) ;
#26071=EDGE_CURVE ( 'NONE', #49012, #17246, #35265, .T. ) ;
#26072=LINE ( 'NONE', #21528, #22397 ) ;
#26073=VECTOR ( 'NONE', #981, 1000.000000000000227 ) ;
#26074=DIRECTION ( 'NONE',  ( 0.007781995580012662783, 0.000000000000000000, -0.9999697198139514409 ) ) ;
#26075=CARTESIAN_POINT ( 'NONE',  ( -25.20278734466900517, 0.000000000000000000, 6.670939612111840944 ) ) ;
#26076=CARTESIAN_POINT ( 'NONE',  ( -11.17708129266966743, 0.000000000000000000, 7.559931525015129772 ) ) ;
#26077=LINE ( 'NONE', #44230, #50235 ) ;
#26078=DIRECTION ( 'NONE',  ( 0.007781995580012663651, 0.000000000000000000, -0.9999697198139515519 ) ) ;
#26079=ORIENTED_EDGE ( 'NONE', *, *, #40433, .T. ) ;
#26081=APPLICATION_CONTEXT ( 'automotive_design' ) ;
#26083=VECTOR ( 'NONE', #29402, 999.9999999999998863 ) ;
#26084=CARTESIAN_POINT ( 'NONE',  ( -10.28842178966973897, 0.000000000000000000, 0.8776935365639153552 ) ) ;
#26085=FACE_OUTER_BOUND ( 'NONE', #40831, .T. ) ;
#26086=CARTESIAN_POINT ( 'NONE',  ( -19.80914291367107438, 1.743523803501506819, 7.437284542042184476 ) ) ;
#26088=CARTESIAN_POINT ( 'NONE',  ( -15.45196360412565895, -0.1191753592594177180, 6.646819749008290756 ) ) ;
#26089=PLANE ( 'NONE',  #13234 ) ;
#26090=EDGE_CURVE ( 'NONE', #54495, #38297, #44590, .T. ) ;
#26091=CARTESIAN_POINT ( 'NONE',  ( -14.00280974873554030, 0.000000000000000000, 12.40921378708904044 ) ) ;
#26093=CARTESIAN_POINT ( 'NONE',  ( 2.072287782118878319, 0.000000000000000000, -2.950529333540147015 ) ) ;
#26094=PLANE ( 'NONE',  #52142 ) ;
#26095=DIRECTION ( 'NONE',  ( -0.9999697198139514409, -0.000000000000000000, -0.007781995580013368816 ) ) ;
#26096=DIRECTION ( 'NONE',  ( -0.9999697198139514409, -0.000000000000000000, -0.007781995580013368816 ) ) ;
#26097=DIRECTION ( 'NONE',  ( -0.7660212471507179544, -0.6427876096865405842, -0.005961354470445141482 ) ) ;
#26098=LINE ( 'NONE', #16712, #532 ) ;
#26099=LINE ( 'NONE', #21556, #5672 ) ;
#26100=CARTESIAN_POINT ( 'NONE',  ( -15.60102546347950536, 0.000000000000000000, 12.95077420755565356 ) ) ;
#26102=ORIENTED_EDGE ( 'NONE', *, *, #45867, .T. ) ;
#26103=LINE ( 'NONE', #43409, #16524 ) ;
#26104=ORIENTED_EDGE ( 'NONE', *, *, #52371, .T. ) ;
#26105=EDGE_CURVE ( 'NONE', #45704, #3681, #9970, .T. ) ;
#26106=AXIS2_PLACEMENT_3D ( 'NONE', #47815, #46967, #22241 ) ;
#26107=EDGE_LOOP ( 'NONE', ( #11841, #8885, #11145 ) ) ;
#26108=EDGE_LOOP ( 'NONE', ( #41535, #37072, #7182, #23591 ) ) ;
#26110=ORIENTED_EDGE ( 'NONE', *, *, #45445, .T. ) ;
#26111=CARTESIAN_POINT ( 'NONE',  ( -17.61711527485669038, 1.905425754524005200, 6.851535249505179337 ) ) ;
#26112=CARTESIAN_POINT ( 'NONE',  ( -15.40103151951671734, 0.000000000000000000, 12.95233060667165681 ) ) ;
#26113=VECTOR ( 'NONE', #338, 999.9999999999998863 ) ;
#26114=ORIENTED_EDGE ( 'NONE', *, *, #17643, .F. ) ;
#26115=ADVANCED_FACE ( 'NONE', ( #13656 ), #39797, .F. ) ;
#26117=VERTEX_POINT ( 'NONE', #875 ) ;
#26118=DIRECTION ( 'NONE',  ( -0.5364919789714478471, 0.6444004775717705469, -0.5449076811759709926 ) ) ;
#26119=DIRECTION ( 'NONE',  ( 0.007781995580012663651, -3.146120232559066537E-19, -0.9999697198139514409 ) ) ;
#26120=VERTEX_POINT ( 'NONE', #9404 ) ;
#26121=DIRECTION ( 'NONE',  ( 0.000000000000000000, -0.000000000000000000, -1.000000000000000000 ) ) ;
#26122=EDGE_LOOP ( 'NONE', ( #43174, #4400, #29215, #31564 ) ) ;
#26123=CARTESIAN_POINT ( 'NONE',  ( -16.66604408758459144, 0.000000000000000000, 9.692031080521234188 ) ) ;
#26124=EDGE_CURVE ( 'NONE', #23769, #25116, #31266, .T. ) ;
#26125=EDGE_CURVE ( 'NONE', #22884, #51007, #39527, .T. ) ;
#26126=LINE ( 'NONE', #25544, #55366 ) ;
#26127=ORIENTED_EDGE ( 'NONE', *, *, #35101, .F. ) ;
#26128=PLANE ( 'NONE',  #53049 ) ;
#26129=DIRECTION ( 'NONE',  ( 0.007781995580012663651, 0.000000000000000000, -0.9999697198139515519 ) ) ;
#26130=CARTESIAN_POINT ( 'NONE',  ( -1.086233639165236964, 0.000000000000000000, -2.796443541562362078 ) ) ;
#26131=LINE ( 'NONE', #47977, #1115 ) ;
#26132=ORIENTED_EDGE ( 'NONE', *, *, #45705, .T. ) ;
#26135=DIRECTION ( 'NONE',  ( -0.5364919789714478471, 0.6444004775717705469, -0.5449076811759709926 ) ) ;
#26137=DIRECTION ( 'NONE',  ( 0.007781995580012663651, 0.000000000000000000, -0.9999697198139515519 ) ) ;
#26139=CARTESIAN_POINT ( 'NONE',  ( -32.47108885958310509, -1.000000000000000000, 15.83124721154520387 ) ) ;
#26140=LINE ( 'NONE', #39178, #26149 ) ;
#26141=EDGE_CURVE ( 'NONE', #39352, #9106, #22741, .T. ) ;
#26142=LINE ( 'NONE', #34946, #32022 ) ;
#26143=CARTESIAN_POINT ( 'NONE',  ( -23.33849165029409889, 0.000000000000000000, 5.946783852668351855 ) ) ;
#26144=CARTESIAN_POINT ( 'NONE',  ( -24.27063949748155380, 0.000000000000000000, 6.308861732390097288 ) ) ;
#26145=ORIENTED_EDGE ( 'NONE', *, *, #47235, .F. ) ;
#26146=FACE_OUTER_BOUND ( 'NONE', #28252, .T. ) ;
#26147=CARTESIAN_POINT ( 'NONE',  ( -8.947017916834877127, -0.1191753592594194527, 6.693699176569870346 ) ) ;
#26148=CARTESIAN_POINT ( 'NONE',  ( -14.53131197095933125, -0.1191753592594181482, 7.761980682317608959 ) ) ;
#26149=VECTOR ( 'NONE', #17311, 1000.000000000000114 ) ;
#26150=DIRECTION ( 'NONE',  ( -0.7660212471507179544, -0.6427876096865405842, -0.005961354470445141482 ) ) ;
#26151=CARTESIAN_POINT ( 'NONE',  ( -14.97870454676872320, -0.1191753592594188005, 5.542506551003013371 ) ) ;
#26152=CARTESIAN_POINT ( 'NONE',  ( -14.13427925798353435, 0.000000000000000000, 3.602414686710813996 ) ) ;
#26153=ORIENTED_EDGE ( 'NONE', *, *, #16493, .F. ) ;
#26154=ORIENTED_EDGE ( 'NONE', *, *, #14012, .F. ) ;
#26155=FACE_OUTER_BOUND ( 'NONE', #12820, .T. ) ;
#26156=DIRECTION ( 'NONE',  ( 0.7660212471507180654, -0.6427876096865404731, 0.005961354470445141482 ) ) ;
#26157=ORIENTED_EDGE ( 'NONE', *, *, #54241, .F. ) ;
#26158=ADVANCED_FACE ( 'NONE', ( #23032 ), #9122, .F. ) ;
#26159=CARTESIAN_POINT ( 'NONE',  ( -10.34095773887371372, -0.1191753592594177180, 6.686594778456397492 ) ) ;
#26160=VERTEX_POINT ( 'NONE', #17944 ) ;
#26161=DIRECTION ( 'NONE',  ( 0.005002170337468016433, -0.7660444431189770143, -0.6427681459581293666 ) ) ;
#26162=EDGE_CURVE ( 'NONE', #10075, #50517, #5702, .T. ) ;
#26163=ORIENTED_EDGE ( 'NONE', *, *, #20758, .F. ) ;
#26164=PLANE ( 'NONE',  #16602 ) ;
#26165=VERTEX_POINT ( 'NONE', #53145 ) ;
#26166=EDGE_LOOP ( 'NONE', ( #37760, #900, #19764, #42643 ) ) ;
#26167=ORIENTED_EDGE ( 'NONE', *, *, #45596, .F. ) ;
#26168=EDGE_CURVE ( 'NONE', #10990, #37130, #44049, .T. ) ;
#26169=CARTESIAN_POINT ( 'NONE',  ( -29.86197018149027116, 0.000000000000000000, 8.281335066757780083 ) ) ;
#26170=CARTESIAN_POINT ( 'NONE',  ( -24.27063949748155380, 0.000000000000000000, 6.308861732390097288 ) ) ;
#26171=DIRECTION ( 'NONE',  ( 0.007781995580012663651, 0.000000000000000000, -0.9999697198139515519 ) ) ;
#26172=EDGE_CURVE ( 'NONE', #50596, #22114, #5172, .T. ) ;
#26173=EDGE_CURVE ( 'NONE', #28890, #29609, #18481, .T. ) ;
#26174=ADVANCED_FACE ( 'NONE', ( #26434 ), #35522, .F. ) ;
#26175=CARTESIAN_POINT ( 'NONE',  ( -18.67775241435682432, 0.000000000000000000, 4.136394454059623804 ) ) ;
#26176=ORIENTED_EDGE ( 'NONE', *, *, #13357, .F. ) ;
#26177=ORIENTED_EDGE ( 'NONE', *, *, #24062, .T. ) ;
#26178=ORIENTED_EDGE ( 'NONE', *, *, #8816, .T. ) ;
#26179=DIRECTION ( 'NONE',  ( 0.7660212471507180654, -0.6427876096865404731, 0.005961354470445141482 ) ) ;
#26180=ORIENTED_EDGE ( 'NONE', *, *, #38815, .F. ) ;
#26182=ORIENTED_EDGE ( 'NONE', *, *, #9718, .T. ) ;
#26183=CARTESIAN_POINT ( 'NONE',  ( -18.69499589319012145, 0.4483081953215045656, 3.929399642557045880 ) ) ;
#26184=DIRECTION ( 'NONE',  ( 0.9999697198139515519, 0.000000000000000000, 0.007781995580013368816 ) ) ;
#26185=AXIS2_PLACEMENT_3D ( 'NONE', #35853, #5199, #5736 ) ;
#26187=DIRECTION ( 'NONE',  ( 0.005002170337468016433, -0.7660444431189770143, -0.6427681459581293666 ) ) ;
#26188=EDGE_CURVE ( 'NONE', #13435, #593, #43750, .T. ) ;
#26189=ORIENTED_EDGE ( 'NONE', *, *, #33678, .T. ) ;
#26190=EDGE_CURVE ( 'NONE', #16343, #31427, #24410, .T. ) ;
#26191=CARTESIAN_POINT ( 'NONE',  ( -16.26566120875878596, -1.651309408375658538, 5.710146992570346747 ) ) ;
#26192=EDGE_LOOP ( 'NONE', ( #4737, #13913, #48776, #41796, #45410 ) ) ;
#26193=PLANE ( 'NONE',  #9619 ) ;
#26194=CARTESIAN_POINT ( 'NONE',  ( -24.26908309836554878, 0.000000000000000000, 6.108867788427308376 ) ) ;
#26195=EDGE_CURVE ( 'NONE', #42767, #20663, #19613, .T. ) ;
#26196=LINE ( 'NONE', #43500, #13772 ) ;
#26197=EDGE_LOOP ( 'NONE', ( #15889, #23076, #19127, #18171 ) ) ;
#26198=LINE ( 'NONE', #1928, #29294 ) ;
#26199=EDGE_CURVE ( 'NONE', #29379, #6398, #11362, .T. ) ;
#26200=LINE ( 'NONE', #25355, #22823 ) ;
#26201=LINE ( 'NONE', #4603, #15816 ) ;
#26202=LINE ( 'NONE', #30474, #10458 ) ;
#26203=DIRECTION ( 'NONE',  ( 0.000000000000000000, -1.000000000000000000, 0.000000000000000000 ) ) ;
#26204=LINE ( 'NONE', #39553, #43345 ) ;
#26205=DIRECTION ( 'NONE',  ( -0.5449076811759708816, 0.6444004775717707689, 0.5364919789714475140 ) ) ;
#26206=EDGE_LOOP ( 'NONE', ( #49758, #33774, #40504, #32643 ) ) ;
#26207=CARTESIAN_POINT ( 'NONE',  ( 2.072287782118878319, 0.000000000000000000, -2.950529333540147015 ) ) ;
#26209=CARTESIAN_POINT ( 'NONE',  ( -17.19117404452963171, 0.000000000000000000, 4.147963350671305172 ) ) ;
#26210=ORIENTED_EDGE ( 'NONE', *, *, #42139, .T. ) ;
#26211=CARTESIAN_POINT ( 'NONE',  ( -13.07066190154808361, 0.000000000000000000, 12.04713590736729678 ) ) ;
#26212=ORIENTED_EDGE ( 'NONE', *, *, #5333, .T. ) ;
#26213=LINE ( 'NONE', #34720, #23476 ) ;
#26214=CARTESIAN_POINT ( 'NONE',  ( -11.60116101491018448, 0.000000000000000000, 2.344805775598597375 ) ) ;
#26215=CARTESIAN_POINT ( 'NONE',  ( -18.71224913745325935, -1.813211359398156919, 4.091943217255450627 ) ) ;
#26216=DIRECTION ( 'NONE',  ( -0.9999697198139514409, -0.000000000000000000, -0.007781995580013368816 ) ) ;
#26217=ORIENTED_EDGE ( 'NONE', *, *, #29372, .T. ) ;
#26218=ORIENTED_EDGE ( 'NONE', *, *, #38050, .T. ) ;
#26219=DIRECTION ( 'NONE',  ( -0.9999697198139514409, -0.000000000000000000, -0.007781995580013368816 ) ) ;
#26220=CARTESIAN_POINT ( 'NONE',  ( -21.82403829489863156, -4.403642575758161648, 5.218019484613594550 ) ) ;
#26221=CARTESIAN_POINT ( 'NONE',  ( -22.40634380310664397, 0.000000000000000000, 5.584705972946605534 ) ) ;
#26222=LINE ( 'NONE', #18241, #48375 ) ;
#26223=CARTESIAN_POINT ( 'NONE',  ( -27.06630483948590893, -0.1191753592594197858, 7.295098399573937797 ) ) ;
#26224=LINE ( 'NONE', #6324, #34914 ) ;
#26225=EDGE_LOOP ( 'NONE', ( #30133, #36936, #42071, #44893 ) ) ;
#26226=DIRECTION ( 'NONE',  ( 0.6427681459581294776, -0.7660444431189769032, 0.005002170337467562802 ) ) ;
#26227=PLANE ( 'NONE',  #11546 ) ;
#26228=ORIENTED_EDGE ( 'NONE', *, *, #54229, .F. ) ;
#26229=DIRECTION ( 'NONE',  ( -0.005961354470445682716, -0.6427876096865404731, 0.7660212471507180654 ) ) ;
#26230=FACE_OUTER_BOUND ( 'NONE', #36137, .T. ) ;
#26231=CARTESIAN_POINT ( 'NONE',  ( -18.29747203306047609, -0.1191753592594177458, 14.03778604627889059 ) ) ;
#26232=ADVANCED_FACE ( 'NONE', ( #32114 ), #28695, .F. ) ;
#26233=EDGE_CURVE ( 'NONE', #29241, #7820, #11064, .T. ) ;
#26234=ORIENTED_EDGE ( 'NONE', *, *, #9923, .T. ) ;
#26235=CARTESIAN_POINT ( 'NONE',  ( 0.000000000000000000, -1.000000000000000000, 0.000000000000000000 ) ) ;
#26236=ORIENTED_EDGE ( 'NONE', *, *, #31747, .T. ) ;
#26238=ORIENTED_EDGE ( 'NONE', *, *, #1732, .F. ) ;
#26239=ORIENTED_EDGE ( 'NONE', *, *, #26297, .F. ) ;
#26240=EDGE_LOOP ( 'NONE', ( #55487, #25571, #30845 ) ) ;
#26241=LINE ( 'NONE', #42705, #15732 ) ;
#26242=VERTEX_POINT ( 'NONE', #44889 ) ;
#26244=ORIENTED_EDGE ( 'NONE', *, *, #13299, .T. ) ;
#26245=LINE ( 'NONE', #13477, #53084 ) ;
#26246=ORIENTED_EDGE ( 'NONE', *, *, #28454, .T. ) ;
#26247=PLANE ( 'NONE',  #4736 ) ;
#26248=ORIENTED_EDGE ( 'NONE', *, *, #30632, .F. ) ;
#26249=EDGE_CURVE ( 'NONE', #41786, #49493, #45425, .T. ) ;
#26250=CARTESIAN_POINT ( 'NONE',  ( -29.86352658060627618, 0.000000000000000000, 8.481329010720569883 ) ) ;
#26251=DIRECTION ( 'NONE',  ( 0.007781995580012663651, 0.000000000000000000, -0.9999697198139515519 ) ) ;
#26252=CARTESIAN_POINT ( 'NONE',  ( -23.33771345073609638, -0.1191753592594197858, 5.846786880686956955 ) ) ;
#26253=ADVANCED_FACE ( 'NONE', ( #36361 ), #19038, .F. ) ;
#26254=DIRECTION ( 'NONE',  ( -0.5364919789714478471, 0.6444004775717705469, -0.5449076811759709926 ) ) ;
#26255=CARTESIAN_POINT ( 'NONE',  ( -18.37467513599760949, 0.6102101463440048335, 5.020127754809787568 ) ) ;
#26256=ORIENTED_EDGE ( 'NONE', *, *, #49108, .T. ) ;
#26257=EDGE_CURVE ( 'NONE', #29027, #32158, #31823, .T. ) ;
#26258=ORIENTED_EDGE ( 'NONE', *, *, #44121, .T. ) ;
#26259=CARTESIAN_POINT ( 'NONE',  ( -13.03662610889668194, 0.000000000000000000, 7.673609645198246731 ) ) ;
#26260=LINE ( 'NONE', #52392, #8539 ) ;
#26261=EDGE_CURVE ( 'NONE', #47262, #53298, #1978, .T. ) ;
#26262=PLANE ( 'NONE',  #3405 ) ;
#26263=DIRECTION ( 'NONE',  ( -0.7660212471507179544, -0.6427876096865405842, -0.005961354470445141482 ) ) ;
#26264=DIRECTION ( 'NONE',  ( 0.000000000000000000, -1.000000000000000000, 0.000000000000000000 ) ) ;
#26265=CARTESIAN_POINT ( 'NONE',  ( -15.96710241509184058, -0.1191753592594218814, 13.13259134697452879 ) ) ;
#26266=ORIENTED_EDGE ( 'NONE', *, *, #3309, .F. ) ;
#26267=CARTESIAN_POINT ( 'NONE',  ( -19.56339837965643369, -0.02924509082106617128, 7.278025012417948858 ) ) ;
#26268=EDGE_CURVE ( 'NONE', #56189, #33548, #46013, .T. ) ;
#26269=LINE ( 'NONE', #12656, #50310 ) ;
#26270=EDGE_LOOP ( 'NONE', ( #37459, #51461, #45066, #18067 ) ) ;
#26271=CARTESIAN_POINT ( 'NONE',  ( -11.20636620717317378, 0.000000000000000000, 11.32298014792380414 ) ) ;
#26272=CARTESIAN_POINT ( 'NONE',  ( -17.20398791294004326, 0.000000000000000000, 5.794517922997338921 ) ) ;
#26273=EDGE_CURVE ( 'NONE', #23095, #48219, #49959, .T. ) ;
#26274=DIRECTION ( 'NONE',  ( -0.005002170337468016433, -0.7660444431189770143, 0.6427681459581293666 ) ) ;
#26275=DIRECTION ( 'NONE',  ( 0.5449076811759707706, 0.6444004775717708799, -0.5364919789714476250 ) ) ;
#26276=FACE_OUTER_BOUND ( 'NONE', #56141, .T. ) ;
#26277=EDGE_LOOP ( 'NONE', ( #22162, #35978, #9907, #17874 ) ) ;
#26278=ORIENTED_EDGE ( 'NONE', *, *, #52056, .T. ) ;
#26279=DIRECTION ( 'NONE',  ( -0.9999697198139514409, -0.000000000000000000, -0.007781995580013368816 ) ) ;
#26280=DIRECTION ( 'NONE',  ( 0.000000000000000000, -1.000000000000000000, 0.000000000000000000 ) ) ;
#26281=LINE ( 'NONE', #48417, #25180 ) ;
#26282=CARTESIAN_POINT ( 'NONE',  ( -13.08486533123210194, 0.000000000000000000, 1.963927175729152541 ) ) ;
#26283=PLANE ( 'NONE',  #41223 ) ;
#26285=DIRECTION ( 'NONE',  ( -0.005002170337468016433, -0.7660444431189770143, 0.6427681459581293666 ) ) ;
#26286=EDGE_LOOP ( 'NONE', ( #13754, #44367, #16365, #38946 ) ) ;
#26287=CARTESIAN_POINT ( 'NONE',  ( -19.09948665707623405, -1.165603555308156514, 4.263021500068094660 ) ) ;
#26289=ORIENTED_EDGE ( 'NONE', *, *, #5596, .F. ) ;
#26290=LINE ( 'NONE', #17791, #43726 ) ;
#26291=ORIENTED_EDGE ( 'NONE', *, *, #40529, .T. ) ;
#26292=FACE_OUTER_BOUND ( 'NONE', #19032, .T. ) ;
#26293=DIRECTION ( 'NONE',  ( -0.8531650599175529814, -0.4028455766673920135, 0.3313982828793697877 ) ) ;
#26294=EDGE_CURVE ( 'NONE', #46009, #30960, #2275, .T. ) ;
#26296=EDGE_LOOP ( 'NONE', ( #4007, #20670, #28375, #44209 ) ) ;
#26297=EDGE_CURVE ( 'NONE', #54363, #35325, #6278, .T. ) ;
#26298=EDGE_CURVE ( 'NONE', #40212, #19762, #10553, .T. ) ;
#26300=ORIENTED_EDGE ( 'NONE', *, *, #37225, .F. ) ;
#26301=VERTEX_POINT ( 'NONE', #27566 ) ;
#26302=EDGE_LOOP ( 'NONE', ( #17596, #4516, #31687, #3736 ) ) ;
#26303=LINE ( 'NONE', #39086, #6070 ) ;
#26304=CARTESIAN_POINT ( 'NONE',  ( -23.33849165029409889, 0.000000000000000000, 5.946783852668351855 ) ) ;
#26305=CARTESIAN_POINT ( 'NONE',  ( -8.975993561185934055, -0.1191753592594197858, 10.41700724906143982 ) ) ;
#26307=CARTESIAN_POINT ( 'NONE',  ( -20.30408966804592907, -1.489407457353158160, 4.720599178244390792 ) ) ;
#26308=ORIENTED_EDGE ( 'NONE', *, *, #11973, .T. ) ;
#26309=ORIENTED_EDGE ( 'NONE', *, *, #46434, .F. ) ;
#26310=EDGE_CURVE ( 'NONE', #17219, #6448, #27871, .T. ) ;
#26311=CARTESIAN_POINT ( 'NONE',  ( -15.13495153988577968, 0.000000000000000000, 12.76973526769478084 ) ) ;
#26312=CARTESIAN_POINT ( 'NONE',  ( -26.13415699229845757, -0.1191753592594197858, 6.933020519852192365 ) ) ;
#26313=CARTESIAN_POINT ( 'NONE',  ( -15.86710544311044302, 0.000000000000000000, 13.13336954653252953 ) ) ;
#26314=EDGE_LOOP ( 'NONE', ( #28319, #47658, #33619, #44604 ) ) ;
#26315=CARTESIAN_POINT ( 'NONE',  ( -16.99924723426068951, 0.000000000000000000, 13.49389102713827171 ) ) ;
#26316=ORIENTED_EDGE ( 'NONE', *, *, #51856, .T. ) ;
#26317=LINE ( 'NONE', #43631, #37354 ) ;
#26318=CARTESIAN_POINT ( 'NONE',  ( -12.80458192191714595, 0.000000000000000000, 11.86454056839041726 ) ) ;
#26319=EDGE_CURVE ( 'NONE', #33688, #29013, #2554, .T. ) ;
#26320=VECTOR ( 'NONE', #33661, 1000.000000000000227 ) ;
#26321=DIRECTION ( 'NONE',  ( 0.6427681459581294776, -0.7660444431189769032, 0.005002170337467562802 ) ) ;
#26322=LINE ( 'NONE', #5326, #16812 ) ;
#26323=ADVANCED_FACE ( 'NONE', ( #40896 ), #6009, .F. ) ;
#26324=CARTESIAN_POINT ( 'NONE',  ( -15.10534619985566351, 0.000000000000000000, 8.965512652746287614 ) ) ;
#26325=DIRECTION ( 'NONE',  ( -0.5449076811759708816, 0.6444004775717707689, 0.5364919789714475140 ) ) ;
#26327=ORIENTED_EDGE ( 'NONE', *, *, #36561, .T. ) ;
#26328=FACE_OUTER_BOUND ( 'NONE', #54562, .T. ) ;
#26329=LINE ( 'NONE', #4755, #18359 ) ;
#26330=DIRECTION ( 'NONE',  ( 0.007781995580012662783, 0.000000000000000000, -0.9999697198139514409 ) ) ;
#26331=DIRECTION ( 'NONE',  ( -0.6427681459581293666, -0.7660444431189770143, -0.005002170337467561935 ) ) ;
#26332=ADVANCED_FACE ( 'NONE', ( #11902 ), #7962, .F. ) ;
#26333=DIRECTION ( 'NONE',  ( 0.6427681459581294776, -0.7660444431189769032, 0.005002170337467562802 ) ) ;
#26334=CARTESIAN_POINT ( 'NONE',  ( -26.13337879274045505, 0.000000000000000000, 6.833023547870798353 ) ) ;
#26336=LINE ( 'NONE', #39418, #52933 ) ;
#26338=LINE ( 'NONE', #43120, #43856 ) ;
#26339=CARTESIAN_POINT ( 'NONE',  ( 2.072287782118878319, 0.000000000000000000, -2.950529333540147015 ) ) ;
#26340=DIRECTION ( 'NONE',  ( -0.7660212471507179544, -0.6427876096865405842, -0.005961354470445141482 ) ) ;
#26341=ADVANCED_FACE ( 'NONE', ( #55095 ), #34076, .F. ) ;
#26342=CARTESIAN_POINT ( 'NONE',  ( -14.94838282604900748, -0.1191753592594197858, 2.588085963191248506 ) ) ;
#26343=PLANE ( 'NONE',  #46648 ) ;
#26344=LINE ( 'NONE', #20703, #51323 ) ;
#26345=EDGE_CURVE ( 'NONE', #36770, #43426, #42007, .T. ) ;
#26346=DIRECTION ( 'NONE',  ( 0.000000000000000000, -0.000000000000000000, -1.000000000000000000 ) ) ;
#26348=ORIENTED_EDGE ( 'NONE', *, *, #46440, .T. ) ;
#26349=DIRECTION ( 'NONE',  ( -0.005002170337468016433, -0.7660444431189770143, 0.6427681459581293666 ) ) ;
#26350=EDGE_CURVE ( 'NONE', #38597, #11166, #29817, .T. ) ;
#26351=ORIENTED_EDGE ( 'NONE', *, *, #19180, .F. ) ;
#26352=VECTOR ( 'NONE', #16525, 1000.000000000000227 ) ;
#26353=EDGE_CURVE ( 'NONE', #25456, #34036, #25271, .T. ) ;
#26354=EDGE_CURVE ( 'NONE', #40757, #3468, #12499, .T. ) ;
#26355=VECTOR ( 'NONE', #32824, 999.9999999999998863 ) ;
#26356=ORIENTED_EDGE ( 'NONE', *, *, #15474, .T. ) ;
#26357=ORIENTED_EDGE ( 'NONE', *, *, #35772, .T. ) ;
#26358=ORIENTED_EDGE ( 'NONE', *, *, #27041, .T. ) ;
#26359=ORIENTED_EDGE ( 'NONE', *, *, #34913, .F. ) ;
#26360=DIRECTION ( 'NONE',  ( 0.000000000000000000, -0.000000000000000000, -1.000000000000000000 ) ) ;
#26361=CARTESIAN_POINT ( 'NONE',  ( -15.83782052860693845, 0.000000000000000000, 9.370320923623856046 ) ) ;
#26362=EDGE_CURVE ( 'NONE', #41698, #4596, #33769, .T. ) ;
#26363=ORIENTED_EDGE ( 'NONE', *, *, #37593, .F. ) ;
#26364=ORIENTED_EDGE ( 'NONE', *, *, #15378, .F. ) ;
#26365=ADVANCED_FACE ( 'NONE', ( #38608 ), #55939, .F. ) ;
#26366=FACE_OUTER_BOUND ( 'NONE', #41709, .T. ) ;
#26368=VERTEX_POINT ( 'NONE', #7664 ) ;
#26369=DIRECTION ( 'NONE',  ( -0.005961354470445682716, -0.6427876096865404731, 0.7660212471507180654 ) ) ;
#26370=CARTESIAN_POINT ( 'NONE',  ( -15.58059336140243190, -5.213152330870663320, 11.28963442256529426 ) ) ;
#26371=ORIENTED_EDGE ( 'NONE', *, *, #4935, .T. ) ;
#26372=CARTESIAN_POINT ( 'NONE',  ( -15.07827343091642014, -4.079838673713162223, 9.234555515054644559 ) ) ;
#26373=VERTEX_POINT ( 'NONE', #38041 ) ;
#26374=VECTOR ( 'NONE', #37470, 999.9999999999998863 ) ;
#26375=CARTESIAN_POINT ( 'NONE',  ( -16.81345671998191449, 0.000000000000000000, 3.412238694616132495 ) ) ;
#26376=CARTESIAN_POINT ( 'NONE',  ( -10.49818613958752600, -0.3560938001956550081, 1.344194339822732953 ) ) ;
#26377=PLANE ( 'NONE',  #21458 ) ;
#26378=VERTEX_POINT ( 'NONE', #15898 ) ;
#26379=CARTESIAN_POINT ( 'NONE',  ( -26.13493519185646008, 0.000000000000000000, 7.033017491833586377 ) ) ;
#26380=PLANE ( 'NONE',  #46480 ) ;
#26381=DIRECTION ( 'NONE',  ( 0.6427681459581294776, -0.7660444431189769032, 0.005002170337467562802 ) ) ;
#26382=ORIENTED_EDGE ( 'NONE', *, *, #54320, .T. ) ;
#26383=CARTESIAN_POINT ( 'NONE',  ( -15.88053067323646417, -0.1191753592594197858, 2.950163842912994383 ) ) ;
#26384=ORIENTED_EDGE ( 'NONE', *, *, #34896, .F. ) ;
#26385=VECTOR ( 'NONE', #47188, 1000.000000000000114 ) ;
#26386=CARTESIAN_POINT ( 'NONE',  ( -16.33317936670417225, 0.000000000000000000, 13.31440848639340224 ) ) ;
#26387=DIRECTION ( 'NONE',  ( 0.6427681459581294776, -0.7660444431189769032, 0.005002170337467562802 ) ) ;
#26388=CARTESIAN_POINT ( 'NONE',  ( -11.81839927990466954, 0.000000000000000000, 4.559107596029180698 ) ) ;
#26389=LINE ( 'NONE', #30395, #36858 ) ;
#26390=EDGE_CURVE ( 'NONE', #51781, #12809, #33243, .T. ) ;
#26391=CARTESIAN_POINT ( 'NONE',  ( -16.53317331066696383, 0.000000000000000000, 13.31285208727739899 ) ) ;
#26392=CARTESIAN_POINT ( 'NONE',  ( 1.086233639165236964, 0.000000000000000000, 2.796443541562362078 ) ) ;
#26393=DIRECTION ( 'NONE',  ( 0.000000000000000000, 1.000000000000000000, 0.000000000000000000 ) ) ;
#26394=VECTOR ( 'NONE', #27534, 999.9999999999998863 ) ;
#26395=FACE_OUTER_BOUND ( 'NONE', #77, .T. ) ;
#26397=CARTESIAN_POINT ( 'NONE',  ( -22.40478740399063895, 0.000000000000000000, 5.384712028983816623 ) ) ;
#26398=ORIENTED_EDGE ( 'NONE', *, *, #47031, .T. ) ;
#26399=LINE ( 'NONE', #3700, #46559 ) ;
#26400=CARTESIAN_POINT ( 'NONE',  ( -18.78639633340495152, 0.000000000000000000, 4.304874975546248983 ) ) ;
#26401=DIRECTION ( 'NONE',  ( 0.000000000000000000, -0.000000000000000000, -1.000000000000000000 ) ) ;
#26402=ADVANCED_FACE ( 'NONE', ( #11650 ), #37780, .F. ) ;
#26403=CARTESIAN_POINT ( 'NONE',  ( -18.72385110809067399, 3.200641362704007786, 9.407098503644062859 ) ) ;
#26404=EDGE_CURVE ( 'NONE', #29543, #13781, #29538, .T. ) ;
#26405=LINE ( 'NONE', #51689, #19668 ) ;
#26406=EDGE_CURVE ( 'NONE', #47842, #30584, #24988, .T. ) ;
#26407=DIRECTION ( 'NONE',  ( -0.7660212471507179544, -0.6427876096865405842, -0.005961354470445141482 ) ) ;
#26409=ORIENTED_EDGE ( 'NONE', *, *, #33559, .F. ) ;
#26410=DIRECTION ( 'NONE',  ( -0.7660212471507179544, -0.6427876096865405842, -0.005961354470445141482 ) ) ;
#26411=CARTESIAN_POINT ( 'NONE',  ( -26.13415699229845757, -0.1191753592594197858, 6.933020519852192365 ) ) ;
#26412=ORIENTED_EDGE ( 'NONE', *, *, #12613, .T. ) ;
#26413=LINE ( 'NONE', #38937, #8458 ) ;
#26414=VECTOR ( 'NONE', #41151, 999.9999999999998863 ) ;
#26415=VECTOR ( 'NONE', #15909, 1000.000000000000227 ) ;
#26416=ORIENTED_EDGE ( 'NONE', *, *, #34388, .F. ) ;
#26417=ADVANCED_FACE ( 'NONE', ( #20727 ), #55350, .F. ) ;
#26418=CARTESIAN_POINT ( 'NONE',  ( -21.18998281933104622, 5.629170628041515023, 4.733240658386350219 ) ) ;
#26419=ORIENTED_EDGE ( 'NONE', *, *, #3841, .T. ) ;
#26420=PLANE ( 'NONE',  #45621 ) ;
#26421=ADVANCED_FACE ( 'NONE', ( #38308 ), #15512, .F. ) ;
#26422=EDGE_LOOP ( 'NONE', ( #49407, #52372, #43781, #33853 ) ) ;
#26423=ORIENTED_EDGE ( 'NONE', *, *, #52554, .T. ) ;
#26424=ORIENTED_EDGE ( 'NONE', *, *, #24062, .F. ) ;
#26425=DIRECTION ( 'NONE',  ( 0.7660212471507180654, -0.6427876096865404731, 0.005961354470445141482 ) ) ;
#26426=CARTESIAN_POINT ( 'NONE',  ( -16.99924723426068951, 0.000000000000000000, 13.49389102713827171 ) ) ;
#26427=CARTESIAN_POINT ( 'NONE',  ( -13.50281940485377064, 0.000000000000000000, 7.869987677393025294 ) ) ;
#26428=ADVANCED_FACE ( 'NONE', ( #32837 ), #27775, .F. ) ;
#26429=LINE ( 'NONE', #872, #21123 ) ;
#26430=ORIENTED_EDGE ( 'NONE', *, *, #32786, .F. ) ;
#26431=ORIENTED_EDGE ( 'NONE', *, *, #54894, .T. ) ;
#26432=AXIS2_PLACEMENT_3D ( 'NONE', #15600, #42010, #2814 ) ;
#26433=EDGE_CURVE ( 'NONE', #51326, #16268, #16097, .T. ) ;
#26434=FACE_OUTER_BOUND ( 'NONE', #29534, .T. ) ;
#26435=VERTEX_POINT ( 'NONE', #28879 ) ;
#26436=CARTESIAN_POINT ( 'NONE',  ( -20.54049170961573267, 0.000000000000000000, 4.660556269540326646 ) ) ;
#26437=ORIENTED_EDGE ( 'NONE', *, *, #43942, .F. ) ;
#26438=CARTESIAN_POINT ( 'NONE',  ( -13.01650773435970443, 0.000000000000000000, 5.088441722393895361 ) ) ;
#26439=DIRECTION ( 'NONE',  ( 0.007781995580012663651, -3.146120232559066537E-19, -0.9999697198139514409 ) ) ;
#26440=VERTEX_POINT ( 'NONE', #45345 ) ;
#26441=PLANE ( 'NONE',  #5075 ) ;
#26442=ORIENTED_EDGE ( 'NONE', *, *, #36479, .T. ) ;
#26443=FACE_OUTER_BOUND ( 'NONE', #28013, .T. ) ;
#26444=ORIENTED_EDGE ( 'NONE', *, *, #28812, .T. ) ;
#26445=CARTESIAN_POINT ( 'NONE',  ( -21.27912796733415135, -3.756034771668161909, 5.027019887704494039 ) ) ;
#26446=CARTESIAN_POINT ( 'NONE',  ( -11.17233041452177211, 0.000000000000000000, 6.949453885754755866 ) ) ;
#26447=DIRECTION ( 'NONE',  ( -0.5364919789714478471, 0.6444004775717705469, -0.5449076811759709926 ) ) ;
#26448=EDGE_LOOP ( 'NONE', ( #5358, #762, #32330, #32922 ) ) ;
#26449=CIRCLE ( 'NONE', #50930, 2.125000000000000000 ) ;
#26450=CARTESIAN_POINT ( 'NONE',  ( 2.072287782118878319, 0.000000000000000000, -2.950529333540147015 ) ) ;
#26451=VECTOR ( 'NONE', #38969, 1000.000000000000227 ) ;
#26452=CARTESIAN_POINT ( 'NONE',  ( -12.09010799418281579, 0.000000000000000000, 5.464983249187678638 ) ) ;
#26453=DIRECTION ( 'NONE',  ( -0.9999697198139514409, -0.000000000000000000, -0.007781995580013368816 ) ) ;
#26454=EDGE_CURVE ( 'NONE', #30915, #9089, #7030, .T. ) ;
#26455=DIRECTION ( 'NONE',  ( 0.005961354470445682716, -0.6427876096865404731, -0.7660212471507180654 ) ) ;
#26456=DIRECTION ( 'NONE',  ( -0.005961354470445682716, -0.6427876096865404731, 0.7660212471507180654 ) ) ;
#26457=LINE ( 'NONE', #644, #10721 ) ;
#26458=EDGE_CURVE ( 'NONE', #21645, #28247, #37113, .T. ) ;
#26459=SURFACE_STYLE_USAGE ( .BOTH. , #21922 ) ;
#26460=VECTOR ( 'NONE', #47592, 999.9999999999998863 ) ;
#26461=ORIENTED_EDGE ( 'NONE', *, *, #17019, .F. ) ;
#26462=DIRECTION ( 'NONE',  ( 0.005002170337468016433, -0.7660444431189770143, -0.6427681459581293666 ) ) ;
#26464=CARTESIAN_POINT ( 'NONE',  ( -13.73672976910459909, 0.000000000000000000, 12.22661844811216270 ) ) ;
#26465=ORIENTED_EDGE ( 'NONE', *, *, #12982, .F. ) ;
#26466=LINE ( 'NONE', #4067, #24758 ) ;
#26467=PLANE ( 'NONE',  #30896 ) ;
#26468=ORIENTED_EDGE ( 'NONE', *, *, #30967, .F. ) ;
#26469=ADVANCED_FACE ( 'NONE', ( #7280 ), #19792, .F. ) ;
#26470=ADVANCED_FACE ( 'NONE', ( #54164 ), #2720, .F. ) ;
#26471=EDGE_CURVE ( 'NONE', #42993, #29692, #45618, .T. ) ;
#26472=LINE ( 'NONE', #17384, #13501 ) ;
#26473=DIRECTION ( 'NONE',  ( 0.9999697198139515519, 0.000000000000000000, 0.007781995580013368816 ) ) ;
#26474=AXIS2_PLACEMENT_3D ( 'NONE', #25217, #3888, #20923 ) ;
#26475=DIRECTION ( 'NONE',  ( 0.7660212471507180654, -0.6427876096865404731, 0.005961354470445141482 ) ) ;
#26476=VECTOR ( 'NONE', #12441, 1000.000000000000227 ) ;
#26477=ADVANCED_FACE ( 'NONE', ( #54412 ), #3008, .F. ) ;
#26478=CARTESIAN_POINT ( 'NONE',  ( -18.22541471764576215, -0.1191753592594165800, 4.778575762111413994 ) ) ;
#26479=ORIENTED_EDGE ( 'NONE', *, *, #55113, .T. ) ;
#26480=EDGE_LOOP ( 'NONE', ( #17128, #31180, #44337, #15184 ) ) ;
#26481=DIRECTION ( 'NONE',  ( 0.007781995580012663651, 0.000000000000000000, -0.9999697198139515519 ) ) ;
#26482=DIRECTION ( 'NONE',  ( 0.000000000000000000, -0.000000000000000000, -1.000000000000000000 ) ) ;
#26483=FACE_OUTER_BOUND ( 'NONE', #55775, .T. ) ;
#26484=DIRECTION ( 'NONE',  ( 0.5449076811759707706, 0.6444004775717708799, -0.5364919789714476250 ) ) ;
#26485=DIRECTION ( 'NONE',  ( 0.5364919789714477361, 0.6444004775717706579, 0.5449076811759711036 ) ) ;
#26486=ADVANCED_FACE ( 'NONE', ( #20337 ), #6457, .F. ) ;
#26487=CARTESIAN_POINT ( 'NONE',  ( -18.67775241435682432, 0.000000000000000000, 4.136394454059623804 ) ) ;
#26488=ORIENTED_EDGE ( 'NONE', *, *, #50187, .F. ) ;
#26489=DIRECTION ( 'NONE',  ( 0.9999697198139515519, 0.000000000000000000, 0.007781995580013368816 ) ) ;
#26490=EDGE_CURVE ( 'NONE', #47842, #18253, #37371, .T. ) ;
#26491=LINE ( 'NONE', #34462, #2461 ) ;
#26492=ORIENTED_EDGE ( 'NONE', *, *, #26071, .F. ) ;
#26493=EDGE_CURVE ( 'NONE', #9089, #46401, #41085, .T. ) ;
#26494=CARTESIAN_POINT ( 'NONE',  ( -13.70716283399377922, -4.727446477803165514, 2.054818365572432803 ) ) ;
#26496=PLANE ( 'NONE',  #47682 ) ;
#26497=PLANE ( 'NONE',  #39314 ) ;
#26498=ORIENTED_EDGE ( 'NONE', *, *, #53692, .F. ) ;
#26499=AXIS2_PLACEMENT_3D ( 'NONE', #32517, #28233, #50662 ) ;
#26501=VECTOR ( 'NONE', #37488, 999.9999999999998863 ) ;
#26502=DIRECTION ( 'NONE',  ( -0.7660212471507179544, -0.6427876096865405842, -0.005961354470445141482 ) ) ;
#26503=ORIENTED_EDGE ( 'NONE', *, *, #50355, .F. ) ;
#26504=ORIENTED_EDGE ( 'NONE', *, *, #18114, .F. ) ;
#26505=VECTOR ( 'NONE', #16645, 999.9999999999998863 ) ;
#26506=EDGE_LOOP ( 'NONE', ( #23524, #49010, #15590, #33295 ) ) ;
#26507=AXIS2_PLACEMENT_3D ( 'NONE', #15102, #29250, #32428 ) ;
#26508=ORIENTED_EDGE ( 'NONE', *, *, #13316, .T. ) ;
#26509=DIRECTION ( 'NONE',  ( -0.9999697198139514409, -0.000000000000000000, -0.007781995580013368816 ) ) ;
#26510=ORIENTED_EDGE ( 'NONE', *, *, #53206, .F. ) ;
#26511=DIRECTION ( 'NONE',  ( -0.7660212471507179544, -0.6427876096865405842, -0.005961354470445141482 ) ) ;
#26512=ORIENTED_EDGE ( 'NONE', *, *, #50722, .T. ) ;
#26513=CARTESIAN_POINT ( 'NONE',  ( -14.00280974873554030, 0.000000000000000000, 12.40921378708904044 ) ) ;
#26514=EDGE_LOOP ( 'NONE', ( #38224, #19025, #45266, #7744 ) ) ;
#26515=CARTESIAN_POINT ( 'NONE',  ( -27.06708303904391144, 0.000000000000000000, 7.395095371555332697 ) ) ;
#26516=VECTOR ( 'NONE', #21142, 1000.000000000000114 ) ;
#26517=VERTEX_POINT ( 'NONE', #36551 ) ;
#26518=DIRECTION ( 'NONE',  ( 0.005002170337468016433, -0.7660444431189770143, -0.6427681459581293666 ) ) ;
#26519=DIRECTION ( 'NONE',  ( -0.3620778797217461542, -0.000000000000000000, -0.9321478471874538041 ) ) ;
#26520=CARTESIAN_POINT ( 'NONE',  ( -9.031591052444445822, -0.1191753592594191058, 3.742128014318059748 ) ) ;
#26521=DIRECTION ( 'NONE',  ( 0.005002170337468016433, -0.7660444431189770143, -0.6427681459581293666 ) ) ;
#26522=CARTESIAN_POINT ( 'NONE',  ( -11.67244013076689946, 0.000000000000000000, 11.50401908778467863 ) ) ;
#26523=VERTEX_POINT ( 'NONE', #14980 ) ;
#26524=EDGE_CURVE ( 'NONE', #54227, #44519, #28300, .T. ) ;
#26525=VERTEX_POINT ( 'NONE', #32315 ) ;
#26526=DIRECTION ( 'NONE',  ( -0.5364919789714478471, 0.6444004775717705469, -0.5449076811759709926 ) ) ;
#26527=FACE_OUTER_BOUND ( 'NONE', #35602, .T. ) ;
#26528=EDGE_CURVE ( 'NONE', #19226, #27412, #23501, .T. ) ;
#26529=VECTOR ( 'NONE', #54461, 1000.000000000000114 ) ;
#26530=LINE ( 'NONE', #9803, #23361 ) ;
#26531=DIRECTION ( 'NONE',  ( 0.007781995580012663651, -3.146120232559066537E-19, -0.9999697198139514409 ) ) ;
#26532=DIRECTION ( 'NONE',  ( 0.000000000000000000, -0.000000000000000000, -1.000000000000000000 ) ) ;
#26533=CARTESIAN_POINT ( 'NONE',  ( -18.67775241435682432, 0.000000000000000000, 4.136394454059623804 ) ) ;
#26534=VERTEX_POINT ( 'NONE', #19508 ) ;
#26535=AXIS2_PLACEMENT_3D ( 'NONE', #10606, #44642, #2603 ) ;
#26536=DIRECTION ( 'NONE',  ( -0.005002170337468016433, -0.7660444431189770143, 0.6427681459581293666 ) ) ;
#26537=DIRECTION ( 'NONE',  ( 0.5449076811759707706, 0.6444004775717708799, -0.5364919789714476250 ) ) ;
#26538=EDGE_LOOP ( 'NONE', ( #56127, #14320, #18064, #49268 ) ) ;
#26539=EDGE_CURVE ( 'NONE', #33244, #27552, #36855, .T. ) ;
#26540=EDGE_CURVE ( 'NONE', #45468, #48012, #20642, .T. ) ;
#26541=EDGE_CURVE ( 'NONE', #36489, #6114, #56118, .T. ) ;
#26542=VECTOR ( 'NONE', #9893, 999.9999999999998863 ) ;
#26546=EDGE_CURVE ( 'NONE', #53450, #20294, #55260, .T. ) ;
#26547=DIRECTION ( 'NONE',  ( 0.9999697198139515519, 0.000000000000000000, 0.007781995580013368816 ) ) ;
#26548=FACE_OUTER_BOUND ( 'NONE', #47179, .T. ) ;
#26549=ORIENTED_EDGE ( 'NONE', *, *, #9612, .T. ) ;
#26550=AXIS2_PLACEMENT_3D ( 'NONE', #48661, #44647, #39847 ) ;
#26551=VECTOR ( 'NONE', #23804, 1000.000000000000114 ) ;
#26552=EDGE_LOOP ( 'NONE', ( #7172, #37381, #44512, #44936 ) ) ;
#26553=DIRECTION ( 'NONE',  ( 0.7660212471507180654, -0.6427876096865404731, 0.005961354470445141482 ) ) ;
#26554=LINE ( 'NONE', #22018, #10452 ) ;
#26556=FACE_OUTER_BOUND ( 'NONE', #45262, .T. ) ;
#26557=VECTOR ( 'NONE', #13355, 1000.000000000000227 ) ;
#26559=DIRECTION ( 'NONE',  ( 0.000000000000000000, -0.000000000000000000, -1.000000000000000000 ) ) ;
#26560=AXIS2_PLACEMENT_3D ( 'NONE', #35986, #26884, #19171 ) ;
#26561=CARTESIAN_POINT ( 'NONE',  ( -13.03087800188611567, 0.000000000000000000, 6.934990238682716246 ) ) ;
#26562=ADVANCED_FACE ( 'NONE', ( #17203 ), #39066, .F. ) ;
#26563=PLANE ( 'NONE',  #8755 ) ;
#26564=DIRECTION ( 'NONE',  ( 0.000000000000000000, -1.000000000000000000, 0.000000000000000000 ) ) ;
#26565=ADVANCED_FACE ( 'NONE', ( #47292 ), #42493, .F. ) ;
#26566=VERTEX_POINT ( 'NONE', #8401 ) ;
#26567=CARTESIAN_POINT ( 'NONE',  ( -10.47421230394850866, 0.000000000000000000, 10.95934586908605723 ) ) ;
#26568=VERTEX_POINT ( 'NONE', #37953 ) ;
#26569=DIRECTION ( 'NONE',  ( 0.007781995580012663651, 0.000000000000000000, -0.9999697198139515519 ) ) ;
#26571=CARTESIAN_POINT ( 'NONE',  ( -15.13495153988577968, 0.000000000000000000, 12.76973526769478084 ) ) ;
#26572=VERTEX_POINT ( 'NONE', #4161 ) ;
#26573=EDGE_CURVE ( 'NONE', #37960, #17288, #33972, .T. ) ;
#26574=AXIS2_PLACEMENT_3D ( 'NONE', #25875, #55977, #43206 ) ;
#26575=ORIENTED_EDGE ( 'NONE', *, *, #1808, .F. ) ;
#26576=EDGE_CURVE ( 'NONE', #35922, #20993, #42750, .T. ) ;
#26577=ORIENTED_EDGE ( 'NONE', *, *, #7426, .T. ) ;
#26578=EDGE_LOOP ( 'NONE', ( #48725, #36367, #39363, #11518 ) ) ;
#26579=ORIENTED_EDGE ( 'NONE', *, *, #3593, .T. ) ;
#26580=EDGE_LOOP ( 'NONE', ( #5213, #54200, #31190, #20297 ) ) ;
#26581=AXIS2_PLACEMENT_3D ( 'NONE', #14240, #32395, #49701 ) ;
#26582=FACE_OUTER_BOUND ( 'NONE', #8417, .T. ) ;
#26583=CARTESIAN_POINT ( 'NONE',  ( -5.362734387325203578, 5.246864883482168729, 5.301441730927289875 ) ) ;
#26584=DIRECTION ( 'NONE',  ( -0.5449076811759708816, 0.6444004775717707689, 0.5364919789714475140 ) ) ;
#26585=VECTOR ( 'NONE', #140, 999.9999999999998863 ) ;
#26586=VECTOR ( 'NONE', #36078, 999.9999999999998863 ) ;
#26587=ORIENTED_EDGE ( 'NONE', *, *, #20658, .F. ) ;
#26588=LINE ( 'NONE', #43905, #1349 ) ;
#26589=ORIENTED_EDGE ( 'NONE', *, *, #41658, .T. ) ;
#26590=ORIENTED_EDGE ( 'NONE', *, *, #2013, .T. ) ;
#26592=VECTOR ( 'NONE', #33759, 1000.000000000000227 ) ;
#26593=VECTOR ( 'NONE', #31855, 1000.000000000000114 ) ;
#26594=PLANE ( 'NONE',  #42086 ) ;
#26595=DIRECTION ( 'NONE',  ( 0.005002170337468016433, -0.7660444431189770143, -0.6427681459581293666 ) ) ;
#26596=CARTESIAN_POINT ( 'NONE',  ( -4.545936964608350728, -6.455664940184357548, 4.984169873386830041 ) ) ;
#26597=ORIENTED_EDGE ( 'NONE', *, *, #38402, .F. ) ;
#26598=DIRECTION ( 'NONE',  ( -0.005961354470445682716, -0.6427876096865404731, 0.7660212471507180654 ) ) ;
#26599=ORIENTED_EDGE ( 'NONE', *, *, #2135, .T. ) ;
#26600=DIRECTION ( 'NONE',  ( -0.005002170337468016433, -0.7660444431189770143, 0.6427681459581293666 ) ) ;
#26601=VECTOR ( 'NONE', #32538, 999.9999999999998863 ) ;
#26602=CARTESIAN_POINT ( 'NONE',  ( -10.74029228357944987, 0.000000000000000000, 11.14194120806293320 ) ) ;
#26603=CARTESIAN_POINT ( 'NONE',  ( -19.12962290826653700, 0.000000000000000000, 14.40064212555863854 ) ) ;
#26604=CARTESIAN_POINT ( 'NONE',  ( -24.26986129792355129, -0.1191753592594197858, 6.208864760408702388 ) ) ;
#26606=LINE ( 'NONE', #8447, #31192 ) ;
#26607=FACE_OUTER_BOUND ( 'NONE', #54848, .T. ) ;
#26608=ORIENTED_EDGE ( 'NONE', *, *, #36120, .F. ) ;
#26609=CARTESIAN_POINT ( 'NONE',  ( -12.75473883498668570, 0.000000000000000000, 5.459810938303666816 ) ) ;
#26611=EDGE_CURVE ( 'NONE', #18181, #32585, #20891, .T. ) ;
#26612=CARTESIAN_POINT ( 'NONE',  ( -17.40553825601883275, 0.000000000000000000, 5.992955467844123696 ) ) ;
#26613=DIRECTION ( 'NONE',  ( -0.6427681459581293666, -0.7660444431189770143, -0.005002170337467561935 ) ) ;
#26614=DIRECTION ( 'NONE',  ( -0.6246952433987893460, -0.7422098413412802076, 0.2426528472758542054 ) ) ;
#26615=AXIS2_PLACEMENT_3D ( 'NONE', #52354, #22243, #25960 ) ;
#26617=DIRECTION ( 'NONE',  ( 0.005961354470445682716, -0.6427876096865404731, -0.7660212471507180654 ) ) ;
#26618=EDGE_CURVE ( 'NONE', #28751, #35036, #38504, .T. ) ;
#26619=EDGE_CURVE ( 'NONE', #19450, #2403, #29986, .T. ) ;
#26620=CARTESIAN_POINT ( 'NONE',  ( -15.87975247367846166, 0.000000000000000000, 2.850166870931599927 ) ) ;
#26621=LINE ( 'NONE', #16704, #21053 ) ;
#26622=ORIENTED_EDGE ( 'NONE', *, *, #32280, .F. ) ;
#26623=VECTOR ( 'NONE', #22338, 999.9999999999998863 ) ;
#26624=CARTESIAN_POINT ( 'NONE',  ( -12.15116108492864377, 0.000000000000000000, 1.401855352044617975 ) ) ;
#26625=PLANE ( 'NONE',  #48496 ) ;
#26626=DIRECTION ( 'NONE',  ( -0.9321478471874540261, 0.000000000000000000, 0.3620778797217457656 ) ) ;
#26627=AXIS2_PLACEMENT_3D ( 'NONE', #48954, #23119, #31365 ) ;
#26628=AXIS2_PLACEMENT_3D ( 'NONE', #26515, #52632, #44139 ) ;
#26629=LINE ( 'NONE', #43947, #37317 ) ;
#26630=CARTESIAN_POINT ( 'NONE',  ( -19.32961685222932147, 0.000000000000000000, 14.39908572644263351 ) ) ;
#26631=CARTESIAN_POINT ( 'NONE',  ( -14.01545677930355183, 0.000000000000000000, 2.126011111488108174 ) ) ;
#26632=CARTESIAN_POINT ( 'NONE',  ( -14.20280369269832832, 0.000000000000000000, 12.40765738797303719 ) ) ;
#26633=VECTOR ( 'NONE', #41033, 1000.000000000000000 ) ;
#26634=VECTOR ( 'NONE', #39765, 1000.000000000000000 ) ;
#26636=PLANE ( 'NONE',  #50977 ) ;
#26637=EDGE_LOOP ( 'NONE', ( #809, #15458, #34755, #35967 ) ) ;
#26639=ORIENTED_EDGE ( 'NONE', *, *, #26956, .T. ) ;
#26640=ORIENTED_EDGE ( 'NONE', *, *, #35815, .F. ) ;
#26641=VERTEX_POINT ( 'NONE', #55536 ) ;
#26642=VECTOR ( 'NONE', #41536, 1000.000000000000227 ) ;
#26643=EDGE_CURVE ( 'NONE', #5703, #42294, #12945, .T. ) ;
#26644=ORIENTED_EDGE ( 'NONE', *, *, #27193, .T. ) ;
#26645=DIRECTION ( 'NONE',  ( 0.7660212471507180654, -0.6427876096865404731, 0.005961354470445141482 ) ) ;
#26646=EDGE_CURVE ( 'NONE', #36770, #13988, #11815, .T. ) ;
#26647=DIRECTION ( 'NONE',  ( 0.000000000000000000, -1.000000000000000000, 0.000000000000000000 ) ) ;
#26648=VECTOR ( 'NONE', #1613, 999.9999999999998863 ) ;
#26649=ORIENTED_EDGE ( 'NONE', *, *, #667, .F. ) ;
#26650=ORIENTED_EDGE ( 'NONE', *, *, #41847, .F. ) ;
#26651=EDGE_CURVE ( 'NONE', #24469, #25199, #38806, .T. ) ;
#26652=VECTOR ( 'NONE', #16137, 999.9999999999998863 ) ;
#26653=DIRECTION ( 'NONE',  ( 0.5449076811759707706, 0.6444004775717708799, -0.5364919789714476250 ) ) ;
#26654=ORIENTED_EDGE ( 'NONE', *, *, #11248, .T. ) ;
#26655=VECTOR ( 'NONE', #54854, 999.9999999999998863 ) ;
#26656=DIRECTION ( 'NONE',  ( 0.007781995580012662783, 0.000000000000000000, -0.9999697198139514409 ) ) ;
#26657=CARTESIAN_POINT ( 'NONE',  ( -12.53706982000896630, -1.651309408375658538, 4.261835473683364128 ) ) ;
#26658=ORIENTED_EDGE ( 'NONE', *, *, #48812, .T. ) ;
#26659=LINE ( 'NONE', #35456, #43688 ) ;
#26660=VECTOR ( 'NONE', #37487, 1000.000000000000114 ) ;
#26661=ORIENTED_EDGE ( 'NONE', *, *, #44278, .F. ) ;
#26662=DIRECTION ( 'NONE',  ( 0.7660212471507180654, -0.6427876096865404731, 0.005961354470445141482 ) ) ;
#26663=LINE ( 'NONE', #29627, #45614 ) ;
#26664=VECTOR ( 'NONE', #2719, 1000.000000000000227 ) ;
#26665=DIRECTION ( 'NONE',  ( -0.005961354470445682716, -0.6427876096865404731, 0.7660212471507180654 ) ) ;
#26666=FACE_OUTER_BOUND ( 'NONE', #4532, .T. ) ;
#26667=VECTOR ( 'NONE', #53514, 999.9999999999998863 ) ;
#26668=ORIENTED_EDGE ( 'NONE', *, *, #51142, .T. ) ;
#26669=DIRECTION ( 'NONE',  ( 0.5364919789714477361, 0.6444004775717706579, 0.5449076811759711036 ) ) ;
#26670=CARTESIAN_POINT ( 'NONE',  ( -18.13900981363277864, 0.000000000000000000, 6.525905505976847820 ) ) ;
#26671=DIRECTION ( 'NONE',  ( -0.7660212471507179544, -0.6427876096865405842, -0.005961354470445141482 ) ) ;
#26673=CARTESIAN_POINT ( 'NONE',  ( -14.93495759592298988, 0.000000000000000000, 12.77129166681078409 ) ) ;
#26674=ADVANCED_FACE ( 'NONE', ( #7871 ), #12411, .F. ) ;
#26675=EDGE_LOOP ( 'NONE', ( #31439, #6414, #32408, #41824 ) ) ;
#26677=FACE_OUTER_BOUND ( 'NONE', #54023, .T. ) ;
#26678=LINE ( 'NONE', #18151, #16936 ) ;
#26679=DIRECTION ( 'NONE',  ( -0.5449076811759708816, 0.6444004775717707689, 0.5364919789714475140 ) ) ;
#26680=PLANE ( 'NONE',  #34135 ) ;
#26681=DIRECTION ( 'NONE',  ( 0.007781995580012663651, 0.000000000000000000, -0.9999697198139515519 ) ) ;
#26682=DIRECTION ( 'NONE',  ( 0.9999697198139515519, 0.000000000000000000, 0.007781995580013368816 ) ) ;
#26683=EDGE_CURVE ( 'NONE', #36758, #5924, #5287, .T. ) ;
#26685=VECTOR ( 'NONE', #24553, 1000.000000000000114 ) ;
#26686=CARTESIAN_POINT ( 'NONE',  ( 2.072287782118878319, 0.000000000000000000, -2.950529333540147015 ) ) ;
#26687=CARTESIAN_POINT ( 'NONE',  ( -23.33693525117809386, 0.000000000000000000, 5.746789908705562944 ) ) ;
#26688=EDGE_LOOP ( 'NONE', ( #54173, #2874, #3155, #19540 ) ) ;
#26689=CARTESIAN_POINT ( 'NONE',  ( -17.04576418467708621, 1.257817950434005683, 3.262954439389057271 ) ) ;
#26690=LINE ( 'NONE', #18164, #50304 ) ;
#26691=FACE_OUTER_BOUND ( 'NONE', #3575, .T. ) ;
#26693=CARTESIAN_POINT ( 'NONE',  ( -15.76334127827276888, -0.5179957512181551094, 3.655068085059692606 ) ) ;
#26694=PLANE ( 'NONE',  #13695 ) ;
#26695=FACE_OUTER_BOUND ( 'NONE', #23578, .T. ) ;
#26696=PLANE ( 'NONE',  #3911 ) ;
#26697=ADVANCED_FACE ( 'NONE', ( #1273 ), #22598, .F. ) ;
#26698=ORIENTED_EDGE ( 'NONE', *, *, #44578, .T. ) ;
#26699=VECTOR ( 'NONE', #3826, 1000.000000000000114 ) ;
#26700=ORIENTED_EDGE ( 'NONE', *, *, #126, .F. ) ;
#26701=DIRECTION ( 'NONE',  ( 0.9999697198139515519, 0.000000000000000000, 0.007781995580013368816 ) ) ;
#26702=AXIS2_PLACEMENT_3D ( 'NONE', #39982, #5367, #39145 ) ;
#26703=LINE ( 'NONE', #44311, #49482 ) ;
#26704=AXIS2_PLACEMENT_3D ( 'NONE', #51342, #11850, #12455 ) ;
#26705=EDGE_LOOP ( 'NONE', ( #6361, #8675, #37044, #29086 ) ) ;
#26707=ORIENTED_EDGE ( 'NONE', *, *, #29536, .T. ) ;
#26708=CARTESIAN_POINT ( 'NONE',  ( -16.81190032086591302, 0.000000000000000000, 3.212244750653343583 ) ) ;
#26709=VECTOR ( 'NONE', #43807, 999.9999999999998863 ) ;
#26710=VERTEX_POINT ( 'NONE', #35651 ) ;
#26711=VECTOR ( 'NONE', #44368, 1000.000000000000114 ) ;
#26712=EDGE_LOOP ( 'NONE', ( #41598, #55862, #18766, #43146 ) ) ;
#26714=PLANE ( 'NONE',  #13021 ) ;
#26716=CARTESIAN_POINT ( 'NONE',  ( -28.93137873341882127, 0.000000000000000000, 8.119251130998824451 ) ) ;
#26717=LINE ( 'NONE', #53408, #11146 ) ;
#26718=VERTEX_POINT ( 'NONE', #30577 ) ;
#26719=EDGE_CURVE ( 'NONE', #44507, #51210, #34810, .T. ) ;
#26720=ORIENTED_EDGE ( 'NONE', *, *, #43834, .T. ) ;
#26721=AXIS2_PLACEMENT_3D ( 'NONE', #40555, #36848, #32832 ) ;
#26722=CARTESIAN_POINT ( 'NONE',  ( -12.60458797795435615, 0.000000000000000000, 11.86609696750642229 ) ) ;
#26723=VECTOR ( 'NONE', #5708, 1000.000000000000000 ) ;
#26724=ORIENTED_EDGE ( 'NONE', *, *, #27440, .F. ) ;
#26725=LINE ( 'NONE', #26436, #12823 ) ;
#26726=ORIENTED_EDGE ( 'NONE', *, *, #27772, .F. ) ;
#26727=VECTOR ( 'NONE', #8045, 1000.000000000000114 ) ;
#26728=DIRECTION ( 'NONE',  ( 0.000000000000000000, -1.000000000000000000, 0.000000000000000000 ) ) ;
#26729=CARTESIAN_POINT ( 'NONE',  ( -12.70458494993575194, -0.1191753592594197858, 11.86531876794841978 ) ) ;
#26730=EDGE_CURVE ( 'NONE', #55847, #26836, #27132, .T. ) ;
#26731=ORIENTED_EDGE ( 'NONE', *, *, #35746, .F. ) ;
#26732=CARTESIAN_POINT ( 'NONE',  ( -28.92982233430281980, 0.000000000000000000, 7.919257187036034651 ) ) ;
#26733=VECTOR ( 'NONE', #8518, 999.9999999999998863 ) ;
#26734=ORIENTED_EDGE ( 'NONE', *, *, #46429, .T. ) ;
#26735=EDGE_CURVE ( 'NONE', #428, #18282, #47881, .T. ) ;
#26736=EDGE_CURVE ( 'NONE', #54123, #17188, #35960, .T. ) ;
#26737=CARTESIAN_POINT ( 'NONE',  ( -22.40634380310664397, 0.000000000000000000, 5.584705972946605534 ) ) ;
#26738=AXIS2_PLACEMENT_3D ( 'NONE', #6343, #40709, #28767 ) ;
#26739=VECTOR ( 'NONE', #11096, 1000.000000000000114 ) ;
#26740=VERTEX_POINT ( 'NONE', #52125 ) ;
#26741=LINE ( 'NONE', #44601, #24913 ) ;
#26742=LINE ( 'NONE', #31582, #39362 ) ;
#26743=AXIS2_PLACEMENT_3D ( 'NONE', #48449, #51853, #34286 ) ;
#26744=LINE ( 'NONE', #8299, #30115 ) ;
#26745=ADVANCED_FACE ( 'NONE', ( #13243 ), #4703, .F. ) ;
#26746=VERTEX_POINT ( 'NONE', #52419 ) ;
#26747=VECTOR ( 'NONE', #55660, 999.9999999999998863 ) ;
#26748=CARTESIAN_POINT ( 'NONE',  ( -10.67320487561729969, 0.000000000000000000, 2.521353358429592184 ) ) ;
#26749=EDGE_CURVE ( 'NONE', #28760, #33629, #4995, .T. ) ;
#26750=PLANE ( 'NONE',  #50978 ) ;
#26751=PLANE ( 'NONE',  #33994 ) ;
#26752=LINE ( 'NONE', #895, #16862 ) ;
#26753=PLANE ( 'NONE',  #13135 ) ;
#26754=EDGE_CURVE ( 'NONE', #1987, #18030, #39652, .T. ) ;
#26755=PLANE ( 'NONE',  #11591 ) ;
#26756=AXIS2_PLACEMENT_3D ( 'NONE', #19919, #28745, #46052 ) ;
#26757=AXIS2_PLACEMENT_3D ( 'NONE', #38785, #39328, #12921 ) ;
#26758=VERTEX_POINT ( 'NONE', #13776 ) ;
#26759=PLANE ( 'NONE',  #26185 ) ;
#26760=DIRECTION ( 'NONE',  ( -0.6246952433987893460, -0.7422098413412802076, 0.2426528472758542054 ) ) ;
#26761=LINE ( 'NONE', #39822, #1484 ) ;
#26762=EDGE_LOOP ( 'NONE', ( #15845, #50878, #25992, #47094 ) ) ;
#26763=CARTESIAN_POINT ( 'NONE',  ( -15.82887794256448366, 0.000000000000000000, 8.221217821810743231 ) ) ;
#26764=FACE_OUTER_BOUND ( 'NONE', #26506, .T. ) ;
#26765=VERTEX_POINT ( 'NONE', #31101 ) ;
#26766=ADVANCED_FACE ( 'NONE', ( #48423 ), #44684, .F. ) ;
#26767=CARTESIAN_POINT ( 'NONE',  ( -1.086233639165236964, 0.000000000000000000, -2.796443541562362078 ) ) ;
#26768=CARTESIAN_POINT ( 'NONE',  ( -9.808144436391993182, 0.000000000000000000, 10.77986332834118777 ) ) ;
#26769=DIRECTION ( 'NONE',  ( -0.7660212471507179544, -0.6427876096865405842, -0.005961354470445141482 ) ) ;
#26770=PLANE ( 'NONE',  #31114 ) ;
#26771=VECTOR ( 'NONE', #25436, 999.9999999999998863 ) ;
#26772=EDGE_CURVE ( 'NONE', #49950, #35486, #40456, .T. ) ;
#26773=ORIENTED_EDGE ( 'NONE', *, *, #17502, .F. ) ;
#26775=DIRECTION ( 'NONE',  ( 0.5449076811759707706, 0.6444004775717708799, -0.5364919789714476250 ) ) ;
#26776=CARTESIAN_POINT ( 'NONE',  ( -19.62132281647664556, -0.1134144341942082690, 4.403214549183394055 ) ) ;
#26778=VECTOR ( 'NONE', #9221, 1000.000000000000227 ) ;
#26780=DIRECTION ( 'NONE',  ( 0.5364919789714477361, 0.6444004775717706579, 0.5449076811759711036 ) ) ;
#26781=LINE ( 'NONE', #13998, #3153 ) ;
#26782=AXIS2_PLACEMENT_3D ( 'NONE', #50756, #12453, #16134 ) ;
#26783=ORIENTED_EDGE ( 'NONE', *, *, #55222, .T. ) ;
#26784=LINE ( 'NONE', #48348, #44648 ) ;
#26786=VECTOR ( 'NONE', #44898, 999.9999999999998863 ) ;
#26787=VECTOR ( 'NONE', #56225, 999.9999999999998863 ) ;
#26788=VERTEX_POINT ( 'NONE', #9503 ) ;
#26789=DIRECTION ( 'NONE',  ( -0.6427681459581293666, -0.7660444431189770143, -0.005002170337467561935 ) ) ;
#26790=DIRECTION ( 'NONE',  ( 0.007781995580012662783, 0.000000000000000000, -0.9999697198139514409 ) ) ;
#26791=LINE ( 'NONE', #39287, #52033 ) ;
#26792=AXIS2_PLACEMENT_3D ( 'NONE', #54458, #46220, #7328 ) ;
#26793=ORIENTED_EDGE ( 'NONE', *, *, #8568, .F. ) ;
#26794=AXIS2_PLACEMENT_3D ( 'NONE', #3732, #7734, #29875 ) ;
#26795=CARTESIAN_POINT ( 'NONE',  ( -12.15116108492864377, 0.000000000000000000, 1.401855352044617975 ) ) ;
#26796=EDGE_CURVE ( 'NONE', #31672, #48670, #1545, .T. ) ;
#26797=ORIENTED_EDGE ( 'NONE', *, *, #34736, .T. ) ;
#26798=VECTOR ( 'NONE', #33617, 1000.000000000000227 ) ;
#26799=VERTEX_POINT ( 'NONE', #5260 ) ;
#26801=ORIENTED_EDGE ( 'NONE', *, *, #19657, .F. ) ;
#26802=ORIENTED_EDGE ( 'NONE', *, *, #47755, .T. ) ;
#26804=VERTEX_POINT ( 'NONE', #52935 ) ;
#26805=CARTESIAN_POINT ( 'NONE',  ( -12.76270579218648571, -2.460819163488157546, 5.678023567659291615 ) ) ;
#26806=PLANE ( 'NONE',  #21356 ) ;
#26807=ADVANCED_FACE ( 'NONE', ( #19122 ), #49530, .F. ) ;
#26808=ORIENTED_EDGE ( 'NONE', *, *, #2447, .F. ) ;
#26809=CARTESIAN_POINT ( 'NONE',  ( -19.26252944426717306, 0.000000000000000000, 5.778497876809297829 ) ) ;
#26810=VERTEX_POINT ( 'NONE', #1243 ) ;
#26811=CARTESIAN_POINT ( 'NONE',  ( -4.243673151615032779, 6.695908571362696016, -1.569986807829671038 ) ) ;
#26812=ORIENTED_EDGE ( 'NONE', *, *, #45210, .F. ) ;
#26813=EDGE_CURVE ( 'NONE', #54636, #25808, #27955, .T. ) ;
#26814=AXIS2_PLACEMENT_3D ( 'NONE', #13087, #51695, #594 ) ;
#26815=LINE ( 'NONE', #1231, #12867 ) ;
#26816=CARTESIAN_POINT ( 'NONE',  ( -19.32961685222932147, 0.000000000000000000, 14.39908572644263351 ) ) ;
#26817=AXIS2_PLACEMENT_3D ( 'NONE', #21332, #26156, #34393 ) ;
#26818=DIRECTION ( 'NONE',  ( 0.007781995580012663651, -3.146120232559066537E-19, -0.9999697198139514409 ) ) ;
#26819=LINE ( 'NONE', #45249, #41134 ) ;
#26820=CARTESIAN_POINT ( 'NONE',  ( -18.12995690313369224, -1.651309408375657428, 6.434302752013834947 ) ) ;
#26821=PLANE ( 'NONE',  #21077 ) ;
#26822=VECTOR ( 'NONE', #26078, 999.9999999999998863 ) ;
#26823=ORIENTED_EDGE ( 'NONE', *, *, #8122, .T. ) ;
#26824=ORIENTED_EDGE ( 'NONE', *, *, #26173, .F. ) ;
#26826=PLANE ( 'NONE',  #23752 ) ;
#26827=DIRECTION ( 'NONE',  ( -0.7660212471507179544, -0.6427876096865405842, -0.005961354470445141482 ) ) ;
#26828=VECTOR ( 'NONE', #43775, 1000.000000000000227 ) ;
#26830=CARTESIAN_POINT ( 'NONE',  ( -14.94916102560700821, 0.000000000000000000, 2.688082935172642962 ) ) ;
#26831=VECTOR ( 'NONE', #43317, 1000.000000000000227 ) ;
#26833=ORIENTED_EDGE ( 'NONE', *, *, #11105, .T. ) ;
#26834=DIRECTION ( 'NONE',  ( -0.5364919789714478471, 0.6444004775717705469, -0.5449076811759709926 ) ) ;
#26835=DIRECTION ( 'NONE',  ( 0.007781995580012663651, -3.146120232559066537E-19, -0.9999697198139514409 ) ) ;
#26836=VERTEX_POINT ( 'NONE', #6109 ) ;
#26837=CARTESIAN_POINT ( 'NONE',  ( -14.99307481429513622, -0.1191753592594185784, 7.389055067291834256 ) ) ;
#26838=CARTESIAN_POINT ( 'NONE',  ( -20.13687485811055211, 1.581621852479006440, 7.298878075135696086 ) ) ;
#26839=VERTEX_POINT ( 'NONE', #1796 ) ;
#26840=VECTOR ( 'NONE', #16084, 1000.000000000000227 ) ;
#26841=ADVANCED_FACE ( 'NONE', ( #49228 ), #31374, .F. ) ;
#26843=CARTESIAN_POINT ( 'NONE',  ( -13.67407281376373263, 0.000000000000000000, 4.175334245699378499 ) ) ;
#26844=AXIS2_PLACEMENT_3D ( 'NONE', #53554, #27165, #36253 ) ;
#26845=AXIS2_PLACEMENT_3D ( 'NONE', #17860, #13844, #27197 ) ;
#26847=CARTESIAN_POINT ( 'NONE',  ( -16.33317936670417225, 0.000000000000000000, 13.31440848639340224 ) ) ;
#26848=VECTOR ( 'NONE', #36938, 1000.000000000000000 ) ;
#26849=FACE_OUTER_BOUND ( 'NONE', #9079, .T. ) ;
#26850=ORIENTED_EDGE ( 'NONE', *, *, #38165, .F. ) ;
#26851=VECTOR ( 'NONE', #6447, 999.9999999999998863 ) ;
#26852=EDGE_LOOP ( 'NONE', ( #30037, #38721, #12243, #51603 ) ) ;
#26853=DIRECTION ( 'NONE',  ( 0.2426528472758541499, 0.7422098413412800966, 0.6246952433987894571 ) ) ;
#26854=LINE ( 'NONE', #52667, #42211 ) ;
#26855=DIRECTION ( 'NONE',  ( 0.007781995580012663651, 0.000000000000000000, -0.9999697198139515519 ) ) ;
#26856=DIRECTION ( 'NONE',  ( 0.000000000000000000, -1.000000000000000000, 0.000000000000000000 ) ) ;
#26857=LINE ( 'NONE', #18050, #22175 ) ;
#26858=EDGE_LOOP ( 'NONE', ( #31697, #13970, #29519, #17423 ) ) ;
#26860=DIRECTION ( 'NONE',  ( 0.005002170337468016433, -0.7660444431189770143, -0.6427681459581293666 ) ) ;
#26861=VECTOR ( 'NONE', #15059, 999.9999999999998863 ) ;
#26862=LINE ( 'NONE', #39909, #1475 ) ;
#26863=DIRECTION ( 'NONE',  ( 0.007781995580012663651, -3.146120232559066537E-19, -0.9999697198139514409 ) ) ;
#26864=VERTEX_POINT ( 'NONE', #36446 ) ;
#26865=DIRECTION ( 'NONE',  ( 0.6427681459581294776, -0.7660444431189769032, 0.005002170337467562802 ) ) ;
#26866=ORIENTED_EDGE ( 'NONE', *, *, #41610, .T. ) ;
#26867=CARTESIAN_POINT ( 'NONE',  ( -11.25506635995362359, -1.813211359398158029, 1.195320179481486722 ) ) ;
#26868=AXIS2_PLACEMENT_3D ( 'NONE', #28495, #2378, #53502 ) ;
#26869=EDGE_CURVE ( 'NONE', #49537, #53352, #14595, .T. ) ;
#26870=LINE ( 'NONE', #49274, #16644 ) ;
#26871=EDGE_LOOP ( 'NONE', ( #4427, #17825, #35251, #30529 ) ) ;
#26872=PLANE ( 'NONE',  #17237 ) ;
#26873=VECTOR ( 'NONE', #33197, 1000.000000000000000 ) ;
#26874=ADVANCED_FACE ( 'NONE', ( #23409 ), #26826, .F. ) ;
#26876=ORIENTED_EDGE ( 'NONE', *, *, #47928, .F. ) ;
#26877=VECTOR ( 'NONE', #13616, 1000.000000000000227 ) ;
#26879=CARTESIAN_POINT ( 'NONE',  ( -27.99923088623136636, 0.000000000000000000, 7.757173251277078130 ) ) ;
#26880=VECTOR ( 'NONE', #25285, 1000.000000000000000 ) ;
#26881=EDGE_LOOP ( 'NONE', ( #19786, #17671, #39751, #40429 ) ) ;
#26882=EDGE_CURVE ( 'NONE', #3963, #28164, #10648, .T. ) ;
#26883=ORIENTED_EDGE ( 'NONE', *, *, #9607, .T. ) ;
#26884=DIRECTION ( 'NONE',  ( 0.000000000000000000, -1.000000000000000000, 0.000000000000000000 ) ) ;
#26885=CARTESIAN_POINT ( 'NONE',  ( -11.40636015113596180, 0.000000000000000000, 11.32142374880780089 ) ) ;
#26886=ORIENTED_EDGE ( 'NONE', *, *, #9159, .T. ) ;
#26887=EDGE_CURVE ( 'NONE', #49177, #32990, #53248, .T. ) ;
#26889=EDGE_CURVE ( 'NONE', #22744, #17816, #5805, .T. ) ;
#26890=ADVANCED_FACE ( 'NONE', ( #9801 ), #5513, .F. ) ;
#26891=VECTOR ( 'NONE', #29631, 999.9999999999998863 ) ;
#26892=VERTEX_POINT ( 'NONE', #23127 ) ;
#26893=LINE ( 'NONE', #23189, #18586 ) ;
#26894=VERTEX_POINT ( 'NONE', #36192 ) ;
#26895=ORIENTED_EDGE ( 'NONE', *, *, #39444, .T. ) ;
#26896=AXIS2_PLACEMENT_3D ( 'NONE', #9701, #43225, #4323 ) ;
#26897=AXIS2_PLACEMENT_3D ( 'NONE', #4370, #59, #22233 ) ;
#26898=FACE_OUTER_BOUND ( 'NONE', #26688, .T. ) ;
#26899=FACE_OUTER_BOUND ( 'NONE', #26003, .T. ) ;
#26900=LINE ( 'NONE', #1308, #20507 ) ;
#26901=DIRECTION ( 'NONE',  ( 0.007781995580012662783, 0.000000000000000000, -0.9999697198139514409 ) ) ;
#26902=EDGE_LOOP ( 'NONE', ( #15982, #5687, #11117, #17161 ) ) ;
#26904=ORIENTED_EDGE ( 'NONE', *, *, #49772, .T. ) ;
#26905=EDGE_CURVE ( 'NONE', #34917, #2726, #53495, .T. ) ;
#26906=FACE_OUTER_BOUND ( 'NONE', #28764, .T. ) ;
#26907=VECTOR ( 'NONE', #51946, 999.9999999999998863 ) ;
#26908=ADVANCED_FACE ( 'NONE', ( #11726 ), #32737, .F. ) ;
#26909=CARTESIAN_POINT ( 'NONE',  ( -12.13851405436063047, 0.000000000000000000, 11.68505802764555135 ) ) ;
#26910=CARTESIAN_POINT ( 'NONE',  ( -18.67619601524082285, 0.000000000000000000, 3.936400510096834893 ) ) ;
#26911=CARTESIAN_POINT ( 'NONE',  ( -14.42424669531936132, -3.917936722690662954, 2.359185689018677312 ) ) ;
#26912=LINE ( 'NONE', #2071, #43048 ) ;
#26913=EDGE_CURVE ( 'NONE', #1004, #37960, #20804, .T. ) ;
#26914=LINE ( 'NONE', #30033, #10329 ) ;
#26915=DIRECTION ( 'NONE',  ( 0.007781995580012663651, -3.146120232559066537E-19, -0.9999697198139514409 ) ) ;
#26917=PLANE ( 'NONE',  #1153 ) ;
#26918=VECTOR ( 'NONE', #46036, 999.9999999999998863 ) ;
#26920=CARTESIAN_POINT ( 'NONE',  ( -19.08265387484136255, 0.000000000000000000, 8.365222198729652447 ) ) ;
#26921=LINE ( 'NONE', #8766, #605 ) ;
#26922=AXIS2_PLACEMENT_3D ( 'NONE', #28592, #16354, #25444 ) ;
#26923=DIRECTION ( 'NONE',  ( -0.5364919789714478471, 0.6444004775717705469, -0.5449076811759709926 ) ) ;
#26925=CARTESIAN_POINT ( 'NONE',  ( -13.43961370871902972, -4.889348428825662118, 9.926587849587082957 ) ) ;
#26926=ADVANCED_FACE ( 'NONE', ( #46643 ), #7194, .F. ) ;
#26927=CARTESIAN_POINT ( 'NONE',  ( -17.26532721389163072, 0.000000000000000000, 13.67648636611514590 ) ) ;
#26928=VECTOR ( 'NONE', #43108, 1000.000000000000000 ) ;
#26929=PLANE ( 'NONE',  #12105 ) ;
#26930=ORIENTED_EDGE ( 'NONE', *, *, #23360, .T. ) ;
#26931=LINE ( 'NONE', #18682, #47464 ) ;
#26932=CARTESIAN_POINT ( 'NONE',  ( 2.072287782118878319, 0.000000000000000000, -2.950529333540147015 ) ) ;
#26933=LINE ( 'NONE', #35182, #10073 ) ;
#26934=VECTOR ( 'NONE', #7600, 1000.000000000000114 ) ;
#26936=PLANE ( 'NONE',  #42105 ) ;
#26937=LINE ( 'NONE', #4772, #12339 ) ;
#26939=VECTOR ( 'NONE', #49646, 1000.000000000000227 ) ;
#26940=AXIS2_PLACEMENT_3D ( 'NONE', #33815, #6578, #23894 ) ;
#26942=DIRECTION ( 'NONE',  ( 0.007781995580012663651, 0.000000000000000000, -0.9999697198139515519 ) ) ;
#26943=ORIENTED_EDGE ( 'NONE', *, *, #51670, .T. ) ;
#26944=VECTOR ( 'NONE', #4871, 999.9999999999998863 ) ;
#26945=EDGE_LOOP ( 'NONE', ( #19462, #13522, #4069, #37539 ) ) ;
#26946=ORIENTED_EDGE ( 'NONE', *, *, #29681, .T. ) ;
#26947=ORIENTED_EDGE ( 'NONE', *, *, #54240, .T. ) ;
#26948=ORIENTED_EDGE ( 'NONE', *, *, #1241, .T. ) ;
#26949=CARTESIAN_POINT ( 'NONE',  ( -17.47589215640082827, 2.876837460659009693, 3.378375551940059562 ) ) ;
#26950=LINE ( 'NONE', #51918, #41215 ) ;
#26951=EDGE_CURVE ( 'NONE', #37046, #23668, #20230, .T. ) ;
#26952=EDGE_CURVE ( 'NONE', #49895, #54809, #33329, .T. ) ;
#26954=VECTOR ( 'NONE', #8337, 1000.000000000000114 ) ;
#26955=ORIENTED_EDGE ( 'NONE', *, *, #33091, .T. ) ;
#26956=EDGE_CURVE ( 'NONE', #15321, #35294, #24243, .T. ) ;
#26957=AXIS2_PLACEMENT_3D ( 'NONE', #1563, #31391, #48711 ) ;
#26959=ORIENTED_EDGE ( 'NONE', *, *, #45115, .T. ) ;
#26960=DIRECTION ( 'NONE',  ( -0.5364919789714478471, 0.6444004775717705469, -0.5449076811759709926 ) ) ;
#26961=FACE_OUTER_BOUND ( 'NONE', #6495, .T. ) ;
#26962=ORIENTED_EDGE ( 'NONE', *, *, #5208, .T. ) ;
#26963=CARTESIAN_POINT ( 'NONE',  ( 2.072287782118878319, 0.000000000000000000, -2.950529333540147015 ) ) ;
#26964=ORIENTED_EDGE ( 'NONE', *, *, #20901, .T. ) ;
#26965=VECTOR ( 'NONE', #11164, 1000.000000000000000 ) ;
#26966=FACE_OUTER_BOUND ( 'NONE', #41771, .T. ) ;
#26967=CARTESIAN_POINT ( 'NONE',  ( -27.99923088623136636, 0.000000000000000000, 7.757173251277078130 ) ) ;
#26968=FACE_OUTER_BOUND ( 'NONE', #5028, .T. ) ;
#26969=DIRECTION ( 'NONE',  ( 0.005961354470445682716, -0.6427876096865404731, -0.7660212471507180654 ) ) ;
#26970=ORIENTED_EDGE ( 'NONE', *, *, #26055, .F. ) ;
#26971=DIRECTION ( 'NONE',  ( 0.7660212471507180654, -0.6427876096865404731, 0.005961354470445141482 ) ) ;
#26972=CARTESIAN_POINT ( 'NONE',  ( -6.520961821973863870, -6.264410134614024628, -0.6854105512135232336 ) ) ;
#26973=PLANE ( 'NONE',  #15749 ) ;
#26974=VERTEX_POINT ( 'NONE', #50047 ) ;
#26975=FACE_OUTER_BOUND ( 'NONE', #50993, .T. ) ;
#26976=ORIENTED_EDGE ( 'NONE', *, *, #47442, .F. ) ;
#26977=EDGE_CURVE ( 'NONE', #48888, #35555, #46345, .T. ) ;
#26978=DIRECTION ( 'NONE',  ( 0.9999697198139515519, 0.000000000000000000, 0.007781995580013368816 ) ) ;
#26979=DIRECTION ( 'NONE',  ( -0.7660212471507179544, -0.6427876096865405842, -0.005961354470445141482 ) ) ;
#26980=DIRECTION ( 'NONE',  ( 0.007781995580012662783, 0.000000000000000000, -0.9999697198139514409 ) ) ;
#26981=CARTESIAN_POINT ( 'NONE',  ( -17.49357527494113285, 0.1245042932765033361, 3.880752594646831533 ) ) ;
#26982=CARTESIAN_POINT ( 'NONE',  ( -19.72141823409769046, 0.000000000000000000, 5.036262558525757882 ) ) ;
#26983=ADVANCED_FACE ( 'NONE', ( #41811 ), #3206, .F. ) ;
#26984=DIRECTION ( 'NONE',  ( 0.000000000000000000, -1.000000000000000000, 0.000000000000000000 ) ) ;
#26985=PLANE ( 'NONE',  #23436 ) ;
#26986=LINE ( 'NONE', #1941, #17553 ) ;
#26987=EDGE_CURVE ( 'NONE', #15529, #9986, #28485, .T. ) ;
#26988=LINE ( 'NONE', #30406, #47747 ) ;
#26990=PLANE ( 'NONE',  #28445 ) ;
#26991=CARTESIAN_POINT ( 'NONE',  ( -11.30636317915456779, -0.1191753592594197858, 11.32220194836580340 ) ) ;
#26992=CARTESIAN_POINT ( 'NONE',  ( -14.15595403163651866, 0.000000000000000000, 6.387576553477955166 ) ) ;
#26994=DIRECTION ( 'NONE',  ( 0.6246952433987894571, -0.7422098413412800966, -0.2426528472758541777 ) ) ;
#26995=EDGE_CURVE ( 'NONE', #4182, #24424, #41276, .T. ) ;
#26996=DIRECTION ( 'NONE',  ( 0.6427681459581294776, -0.7660444431189769032, 0.005002170337467562802 ) ) ;
#26997=FACE_OUTER_BOUND ( 'NONE', #28604, .T. ) ;
#26998=CARTESIAN_POINT ( 'NONE',  ( -23.33849165029409889, 0.000000000000000000, 5.946783852668351855 ) ) ;
#26999=EDGE_LOOP ( 'NONE', ( #48206, #51849, #48003, #41916 ) ) ;
#27000=VECTOR ( 'NONE', #26855, 999.9999999999998863 ) ;
#27001=ORIENTED_EDGE ( 'NONE', *, *, #52916, .T. ) ;
#27002=DIRECTION ( 'NONE',  ( -0.7660212471507179544, -0.6427876096865405842, -0.005961354470445141482 ) ) ;
#27003=FACE_OUTER_BOUND ( 'NONE', #44288, .T. ) ;
#27004=VECTOR ( 'NONE', #55661, 1000.000000000000227 ) ;
#27005=VERTEX_POINT ( 'NONE', #19959 ) ;
#27006=PLANE ( 'NONE',  #48520 ) ;
#27007=ORIENTED_EDGE ( 'NONE', *, *, #19321, .T. ) ;
#27008=LINE ( 'NONE', #44316, #41964 ) ;
#27009=EDGE_LOOP ( 'NONE', ( #21610, #51834, #8650, #41581 ) ) ;
#27010=ORIENTED_EDGE ( 'NONE', *, *, #26045, .F. ) ;
#27011=VERTEX_POINT ( 'NONE', #54580 ) ;
#27013=CARTESIAN_POINT ( 'NONE',  ( 2.072287782118878319, 0.000000000000000000, -2.950529333540147015 ) ) ;
#27014=LINE ( 'NONE', #9396, #23020 ) ;
#27015=ADVANCED_FACE ( 'NONE', ( #15692 ), #33030, .F. ) ;
#27016=DIRECTION ( 'NONE',  ( 0.005002170337468016433, -0.7660444431189770143, -0.6427681459581293666 ) ) ;
#27017=VERTEX_POINT ( 'NONE', #26452 ) ;
#27018=ORIENTED_EDGE ( 'NONE', *, *, #50534, .T. ) ;
#27019=EDGE_CURVE ( 'NONE', #41786, #44220, #26200, .T. ) ;
#27020=ADVANCED_FACE ( 'NONE', ( #22215 ), #39242, .F. ) ;
#27021=DIRECTION ( 'NONE',  ( -0.5364919789714478471, 0.6444004775717705469, -0.5449076811759709926 ) ) ;
#27022=ORIENTED_EDGE ( 'NONE', *, *, #4284, .F. ) ;
#27023=FACE_OUTER_BOUND ( 'NONE', #11130, .T. ) ;
#27024=ORIENTED_EDGE ( 'NONE', *, *, #46929, .T. ) ;
#27025=LINE ( 'NONE', #31272, #9722 ) ;
#27026=CARTESIAN_POINT ( 'NONE',  ( -21.47341775636118655, -0.1191753592594197858, 5.122631121243466090 ) ) ;
#27027=VERTEX_POINT ( 'NONE', #30744 ) ;
#27028=DIRECTION ( 'NONE',  ( 0.007781995580012663651, 0.000000000000000000, -0.9999697198139515519 ) ) ;
#27029=VERTEX_POINT ( 'NONE', #29637 ) ;
#27030=EDGE_CURVE ( 'NONE', #51526, #31162, #13137, .T. ) ;
#27031=FACE_OUTER_BOUND ( 'NONE', #11785, .T. ) ;
#27032=ORIENTED_EDGE ( 'NONE', *, *, #31807, .F. ) ;
#27033=LINE ( 'NONE', #53162, #18596 ) ;
#27034=LINE ( 'NONE', #44343, #50162 ) ;
#27035=DIRECTION ( 'NONE',  ( 0.007781995580012663651, -3.146120232559066537E-19, -0.9999697198139514409 ) ) ;
#27036=EDGE_LOOP ( 'NONE', ( #18559, #7370, #42164 ) ) ;
#27037=VECTOR ( 'NONE', #17766, 999.9999999999998863 ) ;
#27038=CARTESIAN_POINT ( 'NONE',  ( -34.64355613791357769, -1.000000000000000000, 10.23836012842048326 ) ) ;
#27041=EDGE_CURVE ( 'NONE', #27886, #48678, #17674, .T. ) ;
#27042=DIRECTION ( 'NONE',  ( 0.007781995580012662783, 0.000000000000000000, -0.9999697198139514409 ) ) ;
#27043=LINE ( 'NONE', #10273, #1625 ) ;
#27045=ORIENTED_EDGE ( 'NONE', *, *, #33116, .F. ) ;
#27046=PLANE ( 'NONE',  #36166 ) ;
#27047=DIRECTION ( 'NONE',  ( 0.005002170337468016433, -0.7660444431189770143, -0.6427681459581293666 ) ) ;
#27048=LINE ( 'NONE', #17685, #19648 ) ;
#27049=ORIENTED_EDGE ( 'NONE', *, *, #22595, .F. ) ;
#27050=DIRECTION ( 'NONE',  ( 0.005002170337468016433, -0.7660444431189770143, -0.6427681459581293666 ) ) ;
#27051=PLANE ( 'NONE',  #5488 ) ;
#27052=ORIENTED_EDGE ( 'NONE', *, *, #22906, .T. ) ;
#27053=CARTESIAN_POINT ( 'NONE',  ( -15.60102546347950536, 0.000000000000000000, 12.95077420755565356 ) ) ;
#27054=EDGE_CURVE ( 'NONE', #27257, #29102, #30169, .T. ) ;
#27055=FACE_OUTER_BOUND ( 'NONE', #39135, .T. ) ;
#27056=CARTESIAN_POINT ( 'NONE',  ( -12.56336705153974620, 0.000000000000000000, 6.569296447192962241 ) ) ;
#27057=DIRECTION ( 'NONE',  ( 0.007781995580012662783, 0.000000000000000000, -0.9999697198139514409 ) ) ;
#27058=EDGE_LOOP ( 'NONE', ( #14614, #1285, #24818, #19441 ) ) ;
#27059=ORIENTED_EDGE ( 'NONE', *, *, #18551, .F. ) ;
#27060=LINE ( 'NONE', #35871, #4954 ) ;
#27061=DIRECTION ( 'NONE',  ( 0.5364919789714477361, 0.6444004775717706579, 0.5449076811759711036 ) ) ;
#27062=PLANE ( 'NONE',  #11584 ) ;
#27063=ADVANCED_FACE ( 'NONE', ( #8044 ), #12581, .F. ) ;
#27064=CARTESIAN_POINT ( 'NONE',  ( -15.87975247367846166, 0.000000000000000000, 2.850166870931599927 ) ) ;
#27065=LINE ( 'NONE', #39841, #3796 ) ;
#27066=DIRECTION ( 'NONE',  ( -0.5364919789714478471, 0.6444004775717705469, -0.5449076811759709926 ) ) ;
#27067=ORIENTED_EDGE ( 'NONE', *, *, #49750, .T. ) ;
#27068=ADVANCED_FACE ( 'NONE', ( #46943 ), #52324, .F. ) ;
#27069=FACE_OUTER_BOUND ( 'NONE', #25876, .T. ) ;
#27070=EDGE_CURVE ( 'NONE', #51439, #26046, #48045, .T. ) ;
#27072=EDGE_LOOP ( 'NONE', ( #23977, #41727, #12271, #2025 ) ) ;
#27073=CARTESIAN_POINT ( 'NONE',  ( -12.15271748404464880, 0.000000000000000000, 1.601849296007406664 ) ) ;
#27074=EDGE_CURVE ( 'NONE', #25250, #47436, #4052, .T. ) ;
#27075=PLANE ( 'NONE',  #16830 ) ;
#27076=CARTESIAN_POINT ( 'NONE',  ( -9.542064456761055524, 0.000000000000000000, 10.59726798936431180 ) ) ;
#27077=ORIENTED_EDGE ( 'NONE', *, *, #30532, .F. ) ;
#27078=VECTOR ( 'NONE', #23061, 1000.000000000000227 ) ;
#27079=LINE ( 'NONE', #48081, #34846 ) ;
#27081=ORIENTED_EDGE ( 'NONE', *, *, #34188, .F. ) ;
#27082=EDGE_CURVE ( 'NONE', #24756, #13654, #43772, .T. ) ;
#27084=ORIENTED_EDGE ( 'NONE', *, *, #15511, .F. ) ;
#27086=CARTESIAN_POINT ( 'NONE',  ( -18.24840714568802014, -0.1191753592594162470, 7.733053388173527942 ) ) ;
#27087=ORIENTED_EDGE ( 'NONE', *, *, #11789, .F. ) ;
#27088=CARTESIAN_POINT ( 'NONE',  ( -14.16457619215236541, 0.000000000000000000, 7.495505663251248230 ) ) ;
#27089=CARTESIAN_POINT ( 'NONE',  ( -16.33317936670417225, 0.000000000000000000, 13.31440848639340224 ) ) ;
#27090=EDGE_CURVE ( 'NONE', #37629, #1446, #47486, .T. ) ;
#27091=ORIENTED_EDGE ( 'NONE', *, *, #48033, .T. ) ;
#27092=CARTESIAN_POINT ( 'NONE',  ( -14.46888367232926420, 0.000000000000000000, 12.59025272694991315 ) ) ;
#27093=ORIENTED_EDGE ( 'NONE', *, *, #12165, .F. ) ;
#27094=LINE ( 'NONE', #44399, #23193 ) ;
#27095=ORIENTED_EDGE ( 'NONE', *, *, #21807, .T. ) ;
#27096=ADVANCED_FACE ( 'NONE', ( #21916 ), #8599, .F. ) ;
#27098=LINE ( 'NONE', #26816, #285 ) ;
#27099=LINE ( 'NONE', #18277, #562 ) ;
#27100=LINE ( 'NONE', #27660, #37477 ) ;
#27101=CARTESIAN_POINT ( 'NONE',  ( -13.07066190154808361, 0.000000000000000000, 12.04713590736729678 ) ) ;
#27105=CARTESIAN_POINT ( 'NONE',  ( -16.79925329029790149, 0.000000000000000000, 13.49544742625427496 ) ) ;
#27106=LINE ( 'NONE', #6110, #24868 ) ;
#27108=DIRECTION ( 'NONE',  ( -0.5364919789714478471, 0.6444004775717705469, -0.5449076811759709926 ) ) ;
#27109=ORIENTED_EDGE ( 'NONE', *, *, #6314, .T. ) ;
#27110=FACE_OUTER_BOUND ( 'NONE', #11756, .T. ) ;
#27112=VERTEX_POINT ( 'NONE', #40 ) ;
#27114=DIRECTION ( 'NONE',  ( -0.7660212471507179544, -0.6427876096865405842, -0.005961354470445141482 ) ) ;
#27115=EDGE_LOOP ( 'NONE', ( #4799, #44517, #14775, #6383 ) ) ;
#27116=AXIS2_PLACEMENT_3D ( 'NONE', #7142, #55376, #15935 ) ;
#27118=FACE_OUTER_BOUND ( 'NONE', #16025, .T. ) ;
#27119=ADVANCED_FACE ( 'NONE', ( #21662 ), #25620, .F. ) ;
#27120=DIRECTION ( 'NONE',  ( -0.9321478471874540261, 0.000000000000000000, 0.3620778797217457656 ) ) ;
#27121=CARTESIAN_POINT ( 'NONE',  ( -14.13870971060482162, 0.000000000000000000, 4.171718333931368150 ) ) ;
#27122=DIRECTION ( 'NONE',  ( 0.005002170337468016433, -0.7660444431189770143, -0.6427681459581293666 ) ) ;
#27123=VERTEX_POINT ( 'NONE', #56026 ) ;
#27124=ORIENTED_EDGE ( 'NONE', *, *, #29442, .F. ) ;
#27125=DIRECTION ( 'NONE',  ( 0.5449076811759707706, 0.6444004775717708799, -0.5364919789714476250 ) ) ;
#27126=PLANE ( 'NONE',  #25892 ) ;
#27127=CARTESIAN_POINT ( 'NONE',  ( 3.004435629306332345, -1.000000000000000000, -3.312607213261892003 ) ) ;
#27128=EDGE_CURVE ( 'NONE', #24033, #39633, #34429, .T. ) ;
#27129=PLANE ( 'NONE',  #3753 ) ;
#27130=DIRECTION ( 'NONE',  ( 0.007781995580012663651, 0.000000000000000000, -0.9999697198139515519 ) ) ;
#27131=EDGE_LOOP ( 'NONE', ( #38545, #3259, #6983, #21314 ) ) ;
#27132=LINE ( 'NONE', #35371, #13739 ) ;
#27133=DIRECTION ( 'NONE',  ( 0.000000000000000000, -0.000000000000000000, -1.000000000000000000 ) ) ;
#27134=ADVANCED_FACE ( 'NONE', ( #19055 ), #36130, .F. ) ;
#27135=CARTESIAN_POINT ( 'NONE',  ( -16.79925329029790149, 0.000000000000000000, 13.49544742625427496 ) ) ;
#27136=DIRECTION ( 'NONE',  ( 0.7660212471507180654, -0.6427876096865404731, 0.005961354470445141482 ) ) ;
#27137=ORIENTED_EDGE ( 'NONE', *, *, #35281, .F. ) ;
#27138=CARTESIAN_POINT ( 'NONE',  ( -17.35017059011151375, 1.553641160433663071, 12.97584759397192045 ) ) ;
#27139=ORIENTED_EDGE ( 'NONE', *, *, #22600, .T. ) ;
#27140=CARTESIAN_POINT ( 'NONE',  ( -14.93495759592298988, 0.000000000000000000, 12.77129166681078409 ) ) ;
#27141=PLANE ( 'NONE',  #45657 ) ;
#27142=ORIENTED_EDGE ( 'NONE', *, *, #26404, .T. ) ;
#27143=CARTESIAN_POINT ( 'NONE',  ( -10.27421835998572064, 0.000000000000000000, 10.96090226820206048 ) ) ;
#27144=EDGE_CURVE ( 'NONE', #55458, #35036, #53167, .T. ) ;
#27145=ORIENTED_EDGE ( 'NONE', *, *, #39608, .T. ) ;
#27146=ADVANCED_FACE ( 'NONE', ( #35544 ), #31292, .F. ) ;
#27147=VERTEX_POINT ( 'NONE', #27589 ) ;
#27148=VERTEX_POINT ( 'NONE', #49154 ) ;
#27149=LINE ( 'NONE', #27997, #22129 ) ;
#27150=VERTEX_POINT ( 'NONE', #14526 ) ;
#27151=ORIENTED_EDGE ( 'NONE', *, *, #37079, .F. ) ;
#27152=LINE ( 'NONE', #45050, #30220 ) ;
#27153=CARTESIAN_POINT ( 'NONE',  ( -20.64507249176656956, 4.981562823951512620, 4.542241061477253261 ) ) ;
#27154=ORIENTED_EDGE ( 'NONE', *, *, #1320, .T. ) ;
#27155=EDGE_CURVE ( 'NONE', #17736, #52910, #5447, .T. ) ;
#27157=ORIENTED_EDGE ( 'NONE', *, *, #12410, .T. ) ;
#27158=LINE ( 'NONE', #52699, #11322 ) ;
#27159=ORIENTED_EDGE ( 'NONE', *, *, #10177, .T. ) ;
#27160=ORIENTED_EDGE ( 'NONE', *, *, #17206, .T. ) ;
#27161=ADVANCED_FACE ( 'NONE', ( #22761 ), #39814, .T. ) ;
#27162=CARTESIAN_POINT ( 'NONE',  ( -9.808144436391993182, 0.000000000000000000, 10.77986332834118777 ) ) ;
#27163=PLANE ( 'NONE',  #49343 ) ;
#27164=LINE ( 'NONE', #10704, #18737 ) ;
#27165=DIRECTION ( 'NONE',  ( -0.005961354470445682716, -0.6427876096865404731, 0.7660212471507180654 ) ) ;
#27166=ORIENTED_EDGE ( 'NONE', *, *, #47901, .F. ) ;
#27167=LINE ( 'NONE', #9579, #11060 ) ;
#27168=ORIENTED_EDGE ( 'NONE', *, *, #15461, .T. ) ;
#27170=FACE_OUTER_BOUND ( 'NONE', #44257, .T. ) ;
#27171=DIRECTION ( 'NONE',  ( 0.9999697198139515519, 0.000000000000000000, 0.007781995580013368816 ) ) ;
#27173=LINE ( 'NONE', #10715, #22115 ) ;
#27174=CARTESIAN_POINT ( 'NONE',  ( -14.59472444693005500, 0.000000000000000000, 3.060173312390066513 ) ) ;
#27175=ORIENTED_EDGE ( 'NONE', *, *, #32043, .T. ) ;
#27176=LINE ( 'NONE', #48777, #45587 ) ;
#27177=ORIENTED_EDGE ( 'NONE', *, *, #52393, .T. ) ;
#27178=PLANE ( 'NONE',  #35594 ) ;
#27179=CARTESIAN_POINT ( 'NONE',  ( -15.13495153988577968, 0.000000000000000000, 12.76973526769478084 ) ) ;
#27181=EDGE_CURVE ( 'NONE', #31243, #52679, #52853, .T. ) ;
#27183=LINE ( 'NONE', #26925, #12283 ) ;
#27184=CARTESIAN_POINT ( 'NONE',  ( 2.072287782118878319, 0.000000000000000000, -2.950529333540147015 ) ) ;
#27185=FACE_OUTER_BOUND ( 'NONE', #7286, .T. ) ;
#27186=EDGE_CURVE ( 'NONE', #42836, #40959, #53690, .T. ) ;
#27187=ORIENTED_EDGE ( 'NONE', *, *, #50667, .T. ) ;
#27188=EDGE_CURVE ( 'NONE', #13585, #8019, #40078, .T. ) ;
#27189=CARTESIAN_POINT ( 'NONE',  ( -11.20636620717317378, 0.000000000000000000, 11.32298014792380414 ) ) ;
#27190=CARTESIAN_POINT ( 'NONE',  ( -8.446367469219440594, -0.08969168290429911650, 5.248751129891273237 ) ) ;
#27191=CARTESIAN_POINT ( 'NONE',  ( -18.29325764774754859, 3.848249166794010634, 3.664874947303708996 ) ) ;
#27192=EDGE_CURVE ( 'NONE', #52348, #38688, #9730, .T. ) ;
#27193=EDGE_CURVE ( 'NONE', #9089, #42380, #32133, .T. ) ;
#27194=EDGE_CURVE ( 'NONE', #83, #32693, #893, .T. ) ;
#27195=CARTESIAN_POINT ( 'NONE',  ( -14.66887761629205222, 0.000000000000000000, 12.58869632783390990 ) ) ;
#27196=DIRECTION ( 'NONE',  ( -0.6427681459581293666, -0.7660444431189770143, -0.005002170337467561935 ) ) ;
#27197=DIRECTION ( 'NONE',  ( -0.005002170337468016433, -0.7660444431189770143, 0.6427681459581293666 ) ) ;
#27198=DIRECTION ( 'NONE',  ( -0.005002170337468016433, -0.7660444431189770143, 0.6427681459581293666 ) ) ;
#27200=CARTESIAN_POINT ( 'NONE',  ( -16.25365031537483063, 0.000000000000000000, 3.095096183115911614 ) ) ;
#27201=ORIENTED_EDGE ( 'NONE', *, *, #22357, .F. ) ;
#27202=ADVANCED_FACE ( 'NONE', ( #44073 ), #45194, .F. ) ;
#27203=ADVANCED_FACE ( 'NONE', ( #35284 ), #52580, .F. ) ;
#27204=ORIENTED_EDGE ( 'NONE', *, *, #44317, .F. ) ;
#27205=ORIENTED_EDGE ( 'NONE', *, *, #17277, .F. ) ;
#27206=EDGE_LOOP ( 'NONE', ( #10318, #55802, #38170, #40436 ) ) ;
#27207=ADVANCED_FACE ( 'NONE', ( #30991 ), #26750, .F. ) ;
#27208=EDGE_LOOP ( 'NONE', ( #52449, #24792, #41597, #36803, #25366 ) ) ;
#27209=CARTESIAN_POINT ( 'NONE',  ( -18.80807110705793406, 0.000000000000000000, 7.090036842313388377 ) ) ;
#27210=FACE_OUTER_BOUND ( 'NONE', #7227, .T. ) ;
#27211=EDGE_CURVE ( 'NONE', #3728, #28007, #5190, .T. ) ;
#27212=EDGE_LOOP ( 'NONE', ( #24288, #49586, #3669, #7823 ) ) ;
#27213=ORIENTED_EDGE ( 'NONE', *, *, #23735, .F. ) ;
#27214=ORIENTED_EDGE ( 'NONE', *, *, #17369, .F. ) ;
#27215=AXIS2_PLACEMENT_3D ( 'NONE', #32302, #10437, #45335 ) ;
#27216=CARTESIAN_POINT ( 'NONE',  ( -13.07066190154808361, 0.000000000000000000, 12.04713590736729678 ) ) ;
#27217=ORIENTED_EDGE ( 'NONE', *, *, #40347, .F. ) ;
#27218=FACE_OUTER_BOUND ( 'NONE', #29262, .T. ) ;
#27219=CARTESIAN_POINT ( 'NONE',  ( -25.20278734466900517, 0.000000000000000000, 6.670939612111840944 ) ) ;
#27220=ORIENTED_EDGE ( 'NONE', *, *, #25297, .F. ) ;
#27221=DIRECTION ( 'NONE',  ( 0.7660212471507180654, -0.6427876096865404731, 0.005961354470445141482 ) ) ;
#27222=ORIENTED_EDGE ( 'NONE', *, *, #21047, .T. ) ;
#27223=DIRECTION ( 'NONE',  ( -0.9999697198139514409, -0.000000000000000000, -0.007781995580013368816 ) ) ;
#27224=LINE ( 'NONE', #40590, #13040 ) ;
#27225=CARTESIAN_POINT ( 'NONE',  ( -11.30636317915456779, -0.1191753592594197858, 11.32220194836580340 ) ) ;
#27226=DIRECTION ( 'NONE',  ( -0.2426528472758541499, 0.7422098413412800966, -0.6246952433987894571 ) ) ;
#27227=VERTEX_POINT ( 'NONE', #9987 ) ;
#27228=PLANE ( 'NONE',  #25856 ) ;
#27229=PLANE ( 'NONE',  #37454 ) ;
#27230=DIRECTION ( 'NONE',  ( -0.6427681459581293666, -0.7660444431189770143, -0.005002170337467561935 ) ) ;
#27231=VERTEX_POINT ( 'NONE', #27038 ) ;
#27232=FACE_OUTER_BOUND ( 'NONE', #11533, .T. ) ;
#27233=ORIENTED_EDGE ( 'NONE', *, *, #6621, .T. ) ;
#27234=LINE ( 'NONE', #26386, #48301 ) ;
#27236=LINE ( 'NONE', #40011, #49397 ) ;
#27237=DIRECTION ( 'NONE',  ( 0.000000000000000000, -1.000000000000000000, 0.000000000000000000 ) ) ;
#27238=LINE ( 'NONE', #35229, #23232 ) ;
#27239=LINE ( 'NONE', #22704, #15881 ) ;
#27240=CARTESIAN_POINT ( 'NONE',  ( -17.74560456716937296, 0.000000000000000000, 3.774316574337878372 ) ) ;
#27241=DIRECTION ( 'NONE',  ( 0.000000000000000000, -1.000000000000000000, 0.000000000000000000 ) ) ;
#27242=( LENGTH_UNIT ( ) NAMED_UNIT ( * ) SI_UNIT ( .MILLI., .METRE. ) );
#27243=DIRECTION ( 'NONE',  ( 0.007781995580012662783, 0.000000000000000000, -0.9999697198139514409 ) ) ;
#27244=ORIENTED_EDGE ( 'NONE', *, *, #43017, .T. ) ;
#27245=CARTESIAN_POINT ( 'NONE',  ( -11.27738753480351264, -0.1191753592594194527, 7.598893875874236592 ) ) ;
#27246=CARTESIAN_POINT ( 'NONE',  ( -12.30890265829330410, 0.000000000000000000, 7.879279013581050428 ) ) ;
#27248=DIRECTION ( 'NONE',  ( -0.5449076811759708816, 0.6444004775717707689, 0.5364919789714475140 ) ) ;
#27249=ADVANCED_FACE ( 'NONE', ( #14274 ), #18807, .F. ) ;
#27251=DIRECTION ( 'NONE',  ( -0.3620778797217456546, 0.000000000000000000, -0.9321478471874540261 ) ) ;
#27252=ADVANCED_FACE ( 'NONE', ( #3127 ), #7386, .F. ) ;
#27253=PLANE ( 'NONE',  #12425 ) ;
#27254=DIRECTION ( 'NONE',  ( -0.6427681459581293666, -0.7660444431189770143, -0.005002170337467561935 ) ) ;
#27255=ORIENTED_EDGE ( 'NONE', *, *, #29169, .T. ) ;
#27256=AXIS2_PLACEMENT_3D ( 'NONE', #54527, #14542, #23357 ) ;
#27257=VERTEX_POINT ( 'NONE', #37210 ) ;
#27258=CARTESIAN_POINT ( 'NONE',  ( -14.78014544495433924, -1.003701604285654359, 4.070287485779154224 ) ) ;
#27259=DIRECTION ( 'NONE',  ( 0.005002170337468016433, -0.7660444431189770143, -0.6427681459581293666 ) ) ;
#27260=ORIENTED_EDGE ( 'NONE', *, *, #46067, .T. ) ;
#27261=LINE ( 'NONE', #10530, #37665 ) ;
#27264=ADVANCED_FACE ( 'NONE', ( #50569 ), #7133, .F. ) ;
#27265=VERTEX_POINT ( 'NONE', #46276 ) ;
#27266=ORIENTED_EDGE ( 'NONE', *, *, #39323, .T. ) ;
#27267=EDGE_LOOP ( 'NONE', ( #19854, #31381, #35139, #55550 ) ) ;
#27268=ADVANCED_FACE ( 'NONE', ( #36962 ), #54514, .F. ) ;
#27269=DIRECTION ( 'NONE',  ( -0.3620778797217461542, 0.000000000000000000, -0.9321478471874538041 ) ) ;
#27270=LINE ( 'NONE', #49953, #53158 ) ;
#27271=CARTESIAN_POINT ( 'NONE',  ( -29.86197018149027116, 0.000000000000000000, 8.281335066757780083 ) ) ;
#27272=EDGE_CURVE ( 'NONE', #21119, #1201, #19332, .T. ) ;
#27273=VECTOR ( 'NONE', #41475, 999.9999999999998863 ) ;
#27274=DIRECTION ( 'NONE',  ( 0.007781995580012662783, 0.000000000000000000, -0.9999697198139514409 ) ) ;
#27275=ORIENTED_EDGE ( 'NONE', *, *, #19770, .F. ) ;
#27276=VERTEX_POINT ( 'NONE', #55109 ) ;
#27277=EDGE_CURVE ( 'NONE', #14069, #19074, #24429, .T. ) ;
#27278=CARTESIAN_POINT ( 'NONE',  ( -17.95227482402690811, -0.3560938001956556742, 3.843233064070847416 ) ) ;
#27279=VERTEX_POINT ( 'NONE', #16200 ) ;
#27280=DIRECTION ( 'NONE',  ( -0.6427681459581293666, -0.7660444431189770143, -0.005002170337467561935 ) ) ;
#27282=LINE ( 'NONE', #17657, #7004 ) ;
#27283=DIRECTION ( 'NONE',  ( -0.6427681459581293666, -0.7660444431189770143, -0.005002170337467561935 ) ) ;
#27284=ORIENTED_EDGE ( 'NONE', *, *, #172, .T. ) ;
#27285=VECTOR ( 'NONE', #55647, 1000.000000000000227 ) ;
#27286=CARTESIAN_POINT ( 'NONE',  ( -10.28764359011173646, -0.1191753592594197858, 0.7776965645825208995 ) ) ;
#27287=ORIENTED_EDGE ( 'NONE', *, *, #50191, .F. ) ;
#27290=DIRECTION ( 'NONE',  ( -0.6427681459581293666, -0.7660444431189770143, -0.005002170337467561935 ) ) ;
#27291=VERTEX_POINT ( 'NONE', #53986 ) ;
#27292=FACE_OUTER_BOUND ( 'NONE', #15101, .T. ) ;
#27293=CARTESIAN_POINT ( 'NONE',  ( -8.875996589204540044, 0.000000000000000000, 10.41778544861944233 ) ) ;
#27294=CARTESIAN_POINT ( 'NONE',  ( -10.84028925556084388, -0.1191753592594197858, 11.14116300850493246 ) ) ;
#27295=VERTEX_POINT ( 'NONE', #50825 ) ;
#27296=DIRECTION ( 'NONE',  ( 0.005961354470445682716, -0.6427876096865404731, -0.7660212471507180654 ) ) ;
#27297=DIRECTION ( 'NONE',  ( -0.5364919789714478471, 0.6444004775717705469, -0.5449076811759709926 ) ) ;
#27298=CARTESIAN_POINT ( 'NONE',  ( -18.39746900504187010, 0.000000000000000000, 14.03700784672088808 ) ) ;
#27299=FACE_OUTER_BOUND ( 'NONE', #45112, .T. ) ;
#27300=FACE_OUTER_BOUND ( 'NONE', #54285, .T. ) ;
#27302=ORIENTED_EDGE ( 'NONE', *, *, #31747, .F. ) ;
#27304=CARTESIAN_POINT ( 'NONE',  ( -22.85266645506453997, 5.305366725996512045, 14.46508349092411372 ) ) ;
#27305=CARTESIAN_POINT ( 'NONE',  ( -14.55450947277682161, -0.1941918491731548790, 2.654099391803227181 ) ) ;
#27306=ORIENTED_EDGE ( 'NONE', *, *, #21946, .F. ) ;
#27307=DIRECTION ( 'NONE',  ( -0.7660212471507179544, -0.6427876096865405842, -0.005961354470445141482 ) ) ;
#27308=CARTESIAN_POINT ( 'NONE',  ( -27.06552663992790997, 0.000000000000000000, 7.195101427592543786 ) ) ;
#27309=ORIENTED_EDGE ( 'NONE', *, *, #11846, .T. ) ;
#27310=ADVANCED_FACE ( 'NONE', ( #11921 ), #28982, .F. ) ;
#27311=LINE ( 'NONE', #44625, #2572 ) ;
#27313=VECTOR ( 'NONE', #176, 1000.000000000000114 ) ;
#27314=DIRECTION ( 'NONE',  ( -0.005002170337468016433, -0.7660444431189770143, 0.6427681459581293666 ) ) ;
#27315=EDGE_CURVE ( 'NONE', #21327, #55867, #45727, .T. ) ;
#27316=EDGE_CURVE ( 'NONE', #15809, #22275, #54812, .T. ) ;
#27317=DIRECTION ( 'NONE',  ( 0.007781995580012662783, 0.000000000000000000, -0.9999697198139514409 ) ) ;
#27318=LINE ( 'NONE', #44094, #38364 ) ;
#27319=VERTEX_POINT ( 'NONE', #54264 ) ;
#27320=EDGE_LOOP ( 'NONE', ( #10911, #53449, #293, #14047, #12246 ) ) ;
#27321=DIRECTION ( 'NONE',  ( -0.6427681459581293666, -0.7660444431189770143, -0.005002170337467561935 ) ) ;
#27322=LINE ( 'NONE', #53713, #9603 ) ;
#27323=DIRECTION ( 'NONE',  ( 0.5449076811759707706, 0.6444004775717708799, -0.5364919789714476250 ) ) ;
#27324=DIRECTION ( 'NONE',  ( 0.005961354470445682716, -0.6427876096865404731, -0.7660212471507180654 ) ) ;
#27325=DIRECTION ( 'NONE',  ( -0.9999697198139514409, -0.000000000000000000, -0.007781995580013368816 ) ) ;
#27326=ORIENTED_EDGE ( 'NONE', *, *, #37662, .T. ) ;
#27327=DIRECTION ( 'NONE',  ( 0.6427681459581294776, -0.7660444431189769032, 0.005002170337467562802 ) ) ;
#27328=ORIENTED_EDGE ( 'NONE', *, *, #12847, .F. ) ;
#27329=DIRECTION ( 'NONE',  ( 0.007781995580012662783, 0.000000000000000000, -0.9999697198139514409 ) ) ;
#27330=AXIS2_PLACEMENT_3D ( 'NONE', #1980, #41184, #54501 ) ;
#27331=FACE_OUTER_BOUND ( 'NONE', #56187, .T. ) ;
#27332=ORIENTED_EDGE ( 'NONE', *, *, #24767, .F. ) ;
#27333=DIRECTION ( 'NONE',  ( 0.9999697198139515519, 0.000000000000000000, 0.007781995580013368816 ) ) ;
#27334=DIRECTION ( 'NONE',  ( -0.7660212471507179544, -0.6427876096865405842, -0.005961354470445141482 ) ) ;
#27335=DIRECTION ( 'NONE',  ( 0.9999697198139515519, 0.000000000000000000, 0.007781995580013368816 ) ) ;
#27336=ORIENTED_EDGE ( 'NONE', *, *, #38202, .T. ) ;
#27337=DIRECTION ( 'NONE',  ( 0.005002170337468016433, -0.7660444431189770143, -0.6427681459581293666 ) ) ;
#27338=ORIENTED_EDGE ( 'NONE', *, *, #14486, .T. ) ;
#27339=EDGE_CURVE ( 'NONE', #41467, #35980, #15923, .T. ) ;
#27340=EDGE_LOOP ( 'NONE', ( #53276, #34592, #13943, #35840 ) ) ;
#27341=ORIENTED_EDGE ( 'NONE', *, *, #10545, .T. ) ;
#27342=EDGE_CURVE ( 'NONE', #51521, #40951, #10826, .T. ) ;
#27343=ORIENTED_EDGE ( 'NONE', *, *, #24596, .F. ) ;
#27344=LINE ( 'NONE', #44664, #19381 ) ;
#27345=ORIENTED_EDGE ( 'NONE', *, *, #9191, .F. ) ;
#27346=DIRECTION ( 'NONE',  ( 0.007781995580012663651, -3.146120232559066537E-19, -0.9999697198139514409 ) ) ;
#27347=FACE_OUTER_BOUND ( 'NONE', #27206, .T. ) ;
#27348=AXIS2_PLACEMENT_3D ( 'NONE', #40252, #31480, #1342 ) ;
#27349=VECTOR ( 'NONE', #12841, 999.9999999999998863 ) ;
#27350=ORIENTED_EDGE ( 'NONE', *, *, #24319, .T. ) ;
#27351=EDGE_CURVE ( 'NONE', #4025, #38304, #41201, .T. ) ;
#27352=VERTEX_POINT ( 'NONE', #49977 ) ;
#27353=CARTESIAN_POINT ( 'NONE',  ( -14.46888367232926420, 0.000000000000000000, 12.59025272694991315 ) ) ;
#27354=ORIENTED_EDGE ( 'NONE', *, *, #14826, .T. ) ;
#27355=CARTESIAN_POINT ( 'NONE',  ( -10.94028622754223967, 0.000000000000000000, 11.14038480894692995 ) ) ;
#27356=CARTESIAN_POINT ( 'NONE',  ( 2.072287782118878319, 0.000000000000000000, -2.950529333540147015 ) ) ;
#27357=AXIS2_PLACEMENT_3D ( 'NONE', #47789, #4602, #35014 ) ;
#27360=DIRECTION ( 'NONE',  ( 0.005961354470445682716, -0.6427876096865404731, -0.7660212471507180654 ) ) ;
#27361=DIRECTION ( 'NONE',  ( 0.007781995580012663651, 0.000000000000000000, -0.9999697198139515519 ) ) ;
#27362=CARTESIAN_POINT ( 'NONE',  ( -15.97845555265929285, 2.714935509636507316, 7.543567584037618623 ) ) ;
#27363=EDGE_LOOP ( 'NONE', ( #55244, #14863, #38378, #49642 ) ) ;
#27364=ORIENTED_EDGE ( 'NONE', *, *, #26298, .T. ) ;
#27365=DIRECTION ( 'NONE',  ( -0.8531650599175527594, 0.4028455766673922356, 0.3313982828793700652 ) ) ;
#27366=PLANE ( 'NONE',  #51167 ) ;
#27368=VECTOR ( 'NONE', #4041, 1000.000000000000227 ) ;
#27369=LINE ( 'NONE', #17755, #47839 ) ;
#27370=DIRECTION ( 'NONE',  ( 0.5364919789714477361, 0.6444004775717706579, 0.5449076811759711036 ) ) ;
#27371=ORIENTED_EDGE ( 'NONE', *, *, #7873, .T. ) ;
#27372=CARTESIAN_POINT ( 'NONE',  ( -11.87243407472968926, 0.000000000000000000, 11.50246268866867361 ) ) ;
#27373=DIRECTION ( 'NONE',  ( -0.5449076811759708816, 0.6444004775717707689, 0.5364919789714475140 ) ) ;
#27374=EDGE_LOOP ( 'NONE', ( #19300, #45861, #45177, #21045 ) ) ;
#27375=DIRECTION ( 'NONE',  ( 0.000000000000000000, -0.000000000000000000, -1.000000000000000000 ) ) ;
#27376=EDGE_CURVE ( 'NONE', #52765, #42286, #20156, .T. ) ;
#27378=ORIENTED_EDGE ( 'NONE', *, *, #37481, .F. ) ;
#27379=PLANE ( 'NONE',  #14365 ) ;
#27380=CARTESIAN_POINT ( 'NONE',  ( -17.31821934845932631, 1.581621852479005774, 3.358454237843607082 ) ) ;
#27381=EDGE_CURVE ( 'NONE', #39217, #53467, #37491, .T. ) ;
#27382=DIRECTION ( 'NONE',  ( 0.007781995580012663651, -3.146120232559066537E-19, -0.9999697198139514409 ) ) ;
#27383=ADVANCED_FACE ( 'NONE', ( #17304 ), #3978, .F. ) ;
#27384=EDGE_CURVE ( 'NONE', #14373, #8011, #46874, .T. ) ;
#27385=DIRECTION ( 'NONE',  ( 0.000000000000000000, -0.000000000000000000, -1.000000000000000000 ) ) ;
#27386=LINE ( 'NONE', #45279, #37377 ) ;
#27387=ORIENTED_EDGE ( 'NONE', *, *, #27978, .T. ) ;
#27388=ORIENTED_EDGE ( 'NONE', *, *, #55147, .F. ) ;
#27389=DIRECTION ( 'NONE',  ( 0.6427681459581294776, -0.7660444431189769032, 0.005002170337467562802 ) ) ;
#27390=CARTESIAN_POINT ( 'NONE',  ( -19.60834386242827776, 0.000000000000000000, 4.298478389818581213 ) ) ;
#27391=CARTESIAN_POINT ( 'NONE',  ( -12.29740644427217156, 0.000000000000000000, 6.402040200549994786 ) ) ;
#27392=VECTOR ( 'NONE', #5219, 1000.000000000000227 ) ;
#27393=AXIS2_PLACEMENT_3D ( 'NONE', #31214, #5650, #6234 ) ;
#27394=PRODUCT_DEFINITION ( 'UNKNOWN', '', #25369, #50699 ) ;
#27395=CARTESIAN_POINT ( 'NONE',  ( -11.67244013076689946, 0.000000000000000000, 11.50401908778467863 ) ) ;
#27397=ORIENTED_EDGE ( 'NONE', *, *, #2594, .T. ) ;
#27399=CARTESIAN_POINT ( 'NONE',  ( -18.34056015671156459, 0.000000000000000000, 6.724343050823632595 ) ) ;
#27400=ADVANCED_FACE ( 'NONE', ( #38911 ), #7981, .F. ) ;
#27401=LINE ( 'NONE', #2407, #17828 ) ;
#27402=CARTESIAN_POINT ( 'NONE',  ( -13.24105050548075724, 0.000000000000000000, 8.241356893302796749 ) ) ;
#27403=AXIS2_PLACEMENT_3D ( 'NONE', #40601, #40009, #30930 ) ;
#27404=ORIENTED_EDGE ( 'NONE', *, *, #2128, .T. ) ;
#27405=CARTESIAN_POINT ( 'NONE',  ( -18.10994763196841006, -1.651309408375658760, 3.863154378167301228 ) ) ;
#27406=ORIENTED_EDGE ( 'NONE', *, *, #10563, .F. ) ;
#27408=FACE_OUTER_BOUND ( 'NONE', #30498, .T. ) ;
#27409=ORIENTED_EDGE ( 'NONE', *, *, #1085, .T. ) ;
#27410=DIRECTION ( 'NONE',  ( -0.5364919789714478471, 0.6444004775717705469, -0.5449076811759709926 ) ) ;
#27411=AXIS2_PLACEMENT_3D ( 'NONE', #12702, #21213, #29164 ) ;
#27412=VERTEX_POINT ( 'NONE', #34627 ) ;
#27413=EDGE_LOOP ( 'NONE', ( #4864, #32090, #36720, #16441 ) ) ;
#27414=ORIENTED_EDGE ( 'NONE', *, *, #8882, .T. ) ;
#27415=DIRECTION ( 'NONE',  ( 0.007781995580012662783, 0.000000000000000000, -0.9999697198139514409 ) ) ;
#27416=ORIENTED_EDGE ( 'NONE', *, *, #50118, .F. ) ;
#27418=DIRECTION ( 'NONE',  ( 0.005002170337468016433, -0.7660444431189770143, -0.6427681459581293666 ) ) ;
#27419=CARTESIAN_POINT ( 'NONE',  ( -13.00457969848779705, -2.784623065533159636, 1.843897454566881144 ) ) ;
#27420=ORIENTED_EDGE ( 'NONE', *, *, #2638, .F. ) ;
#27421=VERTEX_POINT ( 'NONE', #43183 ) ;
#27422=DIRECTION ( 'NONE',  ( 0.5364919789714477361, 0.6444004775717706579, 0.5449076811759711036 ) ) ;
#27423=ADVANCED_FACE ( 'NONE', ( #17052 ), #34938, .F. ) ;
#27425=VECTOR ( 'NONE', #40477, 1000.000000000000114 ) ;
#27427=CARTESIAN_POINT ( 'NONE',  ( -24.27063949748155380, 0.000000000000000000, 6.308861732390097288 ) ) ;
#27428=LINE ( 'NONE', #760, #52998 ) ;
#27431=AXIS2_PLACEMENT_3D ( 'NONE', #6326, #45476, #23627 ) ;
#27433=DIRECTION ( 'NONE',  ( 0.5449076811759707706, 0.6444004775717708799, -0.5364919789714476250 ) ) ;
#27434=EDGE_LOOP ( 'NONE', ( #41925, #2596, #20387, #569 ) ) ;
#27435=EDGE_CURVE ( 'NONE', #17107, #5134, #4539, .T. ) ;
#27436=AXIS2_PLACEMENT_3D ( 'NONE', #51634, #3385, #33741 ) ;
#27437=VECTOR ( 'NONE', #16992, 1000.000000000000227 ) ;
#27438=DIRECTION ( 'NONE',  ( 0.005002170337468016433, -0.7660444431189770143, -0.6427681459581293666 ) ) ;
#27439=EDGE_CURVE ( 'NONE', #15806, #11344, #47719, .T. ) ;
#27440=EDGE_CURVE ( 'NONE', #42498, #51400, #8829, .T. ) ;
#27441=DIRECTION ( 'NONE',  ( 0.007781995580012663651, 0.000000000000000000, -0.9999697198139515519 ) ) ;
#27442=VECTOR ( 'NONE', #14697, 999.9999999999998863 ) ;
#27443=VECTOR ( 'NONE', #46494, 1000.000000000000227 ) ;
#27445=DIRECTION ( 'NONE',  ( 0.007781995580012662783, 0.000000000000000000, -0.9999697198139514409 ) ) ;
#27446=CARTESIAN_POINT ( 'NONE',  ( -19.51511390298037441, -5.536956232915666298, 4.284996200178408543 ) ) ;
#27447=CARTESIAN_POINT ( 'NONE',  ( -18.62376508501084516, 0.000000000000000000, 9.107457517013187953 ) ) ;
#27448=ORIENTED_EDGE ( 'NONE', *, *, #23176, .F. ) ;
#27449=PLANE ( 'NONE',  #31984 ) ;
#27450=EDGE_CURVE ( 'NONE', #9775, #37986, #8235, .T. ) ;
#27451=ORIENTED_EDGE ( 'NONE', *, *, #18189, .F. ) ;
#27452=PLANE ( 'NONE',  #21114 ) ;
#27453=CARTESIAN_POINT ( 'NONE',  ( -18.50832163360941607, 4.657758921906512306, 3.722585503579211252 ) ) ;
#27454=ADVANCED_FACE ( 'NONE', ( #25852 ), #34099, .F. ) ;
#27455=PLANE ( 'NONE',  #27215 ) ;
#27456=VECTOR ( 'NONE', #13204, 999.9999999999998863 ) ;
#27457=LINE ( 'NONE', #10138, #18659 ) ;
#27458=VECTOR ( 'NONE', #35322, 1000.000000000000227 ) ;
#27459=EDGE_CURVE ( 'NONE', #48603, #25745, #51417, .T. ) ;
#27460=DIRECTION ( 'NONE',  ( 0.9999697198139515519, 0.000000000000000000, 0.007781995580013368816 ) ) ;
#27462=ORIENTED_EDGE ( 'NONE', *, *, #4878, .T. ) ;
#27463=CARTESIAN_POINT ( 'NONE',  ( -13.45815220315852834, 0.000000000000000000, 2.130348184563771063 ) ) ;
#27464=FACE_OUTER_BOUND ( 'NONE', #20772, .T. ) ;
#27465=DIRECTION ( 'NONE',  ( 0.000000000000000000, -0.000000000000000000, -1.000000000000000000 ) ) ;
#27466=VECTOR ( 'NONE', #546, 999.9999999999998863 ) ;
#27468=CARTESIAN_POINT ( 'NONE',  ( -10.78260220767254118, -0.1191753592594188005, 3.728501240626274527 ) ) ;
#27469=CARTESIAN_POINT ( 'NONE',  ( -14.63627885039329257, 0.000000000000000000, 8.399824917293743809 ) ) ;
#27470=VECTOR ( 'NONE', #6800, 999.9999999999998863 ) ;
#27472=EDGE_CURVE ( 'NONE', #19882, #39633, #51673, .T. ) ;
#27473=CARTESIAN_POINT ( 'NONE',  ( -1.086233639165236964, -1.000000000000000000, -2.796443541562362078 ) ) ;
#27474=VECTOR ( 'NONE', #18179, 1000.000000000000227 ) ;
#27475=DIRECTION ( 'NONE',  ( 0.000000000000000000, -1.000000000000000000, 0.000000000000000000 ) ) ;
#27476=VECTOR ( 'NONE', #50156, 999.9999999999998863 ) ;
#27477=VECTOR ( 'NONE', #12074, 1000.000000000000114 ) ;
#27478=ORIENTED_EDGE ( 'NONE', *, *, #36259, .T. ) ;
#27479=VECTOR ( 'NONE', #5549, 1000.000000000000000 ) ;
#27480=VERTEX_POINT ( 'NONE', #47133 ) ;
#27481=ORIENTED_EDGE ( 'NONE', *, *, #8357, .F. ) ;
#27482=AXIS2_PLACEMENT_3D ( 'NONE', #52266, #12529, #38924 ) ;
#27483=ORIENTED_EDGE ( 'NONE', *, *, #8364, .T. ) ;
#27484=ORIENTED_EDGE ( 'NONE', *, *, #28759, .F. ) ;
#27485=CARTESIAN_POINT ( 'NONE',  ( -2.579292853887890757, -4.639166217699263406, -2.216488638059722849 ) ) ;
#27486=FACE_OUTER_BOUND ( 'NONE', #32696, .T. ) ;
#27487=ORIENTED_EDGE ( 'NONE', *, *, #16164, .T. ) ;
#27489=VECTOR ( 'NONE', #29829, 1000.000000000000227 ) ;
#27490=EDGE_CURVE ( 'NONE', #19740, #26046, #52254, .T. ) ;
#27491=ORIENTED_EDGE ( 'NONE', *, *, #5979, .F. ) ;
#27492=AXIS2_PLACEMENT_3D ( 'NONE', #35143, #16965, #39087 ) ;
#27494=CARTESIAN_POINT ( 'NONE',  ( -11.20636620717317378, 0.000000000000000000, 11.32298014792380414 ) ) ;
#27495=LINE ( 'NONE', #9640, #21416 ) ;
#27496=EDGE_LOOP ( 'NONE', ( #15151, #12619, #32045, #32337 ) ) ;
#27497=DIRECTION ( 'NONE',  ( 0.007781995580012663651, -3.146120232559066537E-19, -0.9999697198139514409 ) ) ;
#27498=EDGE_CURVE ( 'NONE', #37937, #9627, #30681, .T. ) ;
#27499=VECTOR ( 'NONE', #43316, 1000.000000000000227 ) ;
#27500=ADVANCED_FACE ( 'NONE', ( #47981 ), #20743, .F. ) ;
#27501=VERTEX_POINT ( 'NONE', #38060 ) ;
#27502=DIRECTION ( 'NONE',  ( 0.007781995580012663651, -3.146120232559066537E-19, -0.9999697198139514409 ) ) ;
#27503=CARTESIAN_POINT ( 'NONE',  ( -15.87975247367846166, 0.000000000000000000, 2.850166870931599927 ) ) ;
#27504=VECTOR ( 'NONE', #42256, 1000.000000000000227 ) ;
#27505=EDGE_CURVE ( 'NONE', #50409, #33297, #33793, .T. ) ;
#27506=DIRECTION ( 'NONE',  ( 0.3313982828793700097, 0.4028455766673915694, 0.8531650599175529814 ) ) ;
#27507=FACE_OUTER_BOUND ( 'NONE', #52018, .T. ) ;
#27508=LINE ( 'NONE', #24093, #23191 ) ;
#27509=CARTESIAN_POINT ( 'NONE',  ( 1.971453974394196562, 0.000000000000000000, 10.00639841352631088 ) ) ;
#27510=PLANE ( 'NONE',  #8511 ) ;
#27511=AXIS2_PLACEMENT_3D ( 'NONE', #53806, #15736, #23700 ) ;
#27512=ORIENTED_EDGE ( 'NONE', *, *, #2594, .F. ) ;
#27513=LINE ( 'NONE', #35766, #31036 ) ;
#27514=ORIENTED_EDGE ( 'NONE', *, *, #33646, .T. ) ;
#27515=VECTOR ( 'NONE', #46636, 1000.000000000000227 ) ;
#27516=VECTOR ( 'NONE', #48400, 999.9999999999998863 ) ;
#27517=DIRECTION ( 'NONE',  ( 0.007781995580012663651, 0.000000000000000000, -0.9999697198139515519 ) ) ;
#27518=CARTESIAN_POINT ( 'NONE',  ( -15.86710544311044302, 0.000000000000000000, 13.13336954653252953 ) ) ;
#27519=CARTESIAN_POINT ( 'NONE',  ( -27.06630483948590893, -0.1191753592594197858, 7.295098399573937797 ) ) ;
#27520=EDGE_CURVE ( 'NONE', #29311, #2552, #4818, .T. ) ;
#27521=LINE ( 'NONE', #53376, #52243 ) ;
#27522=FACE_OUTER_BOUND ( 'NONE', #19524, .T. ) ;
#27523=DIRECTION ( 'NONE',  ( 0.000000000000000000, -1.000000000000000000, 0.000000000000000000 ) ) ;
#27525=EDGE_CURVE ( 'NONE', #38808, #43441, #31217, .T. ) ;
#27526=VECTOR ( 'NONE', #36352, 999.9999999999998863 ) ;
#27527=FACE_OUTER_BOUND ( 'NONE', #9119, .T. ) ;
#27528=AXIS2_PLACEMENT_3D ( 'NONE', #12728, #39125, #3919 ) ;
#27529=EDGE_CURVE ( 'NONE', #39202, #6097, #44839, .T. ) ;
#27530=CARTESIAN_POINT ( 'NONE',  ( -10.47421230394850866, 0.000000000000000000, 10.95934586908605723 ) ) ;
#27531=ORIENTED_EDGE ( 'NONE', *, *, #43529, .T. ) ;
#27532=CARTESIAN_POINT ( 'NONE',  ( -20.27093655581709797, -1.975113310420657520, 7.797349324992047137 ) ) ;
#27533=CARTESIAN_POINT ( 'NONE',  ( -12.70458494993575194, -0.1191753592594197858, 11.86531876794841978 ) ) ;
#27534=DIRECTION ( 'NONE',  ( 0.007781995580012663651, 0.000000000000000000, -0.9999697198139515519 ) ) ;
#27535=DIRECTION ( 'NONE',  ( 0.5449076811759707706, 0.6444004775717708799, -0.5364919789714476250 ) ) ;
#27536=EDGE_CURVE ( 'NONE', #20287, #49088, #23277, .T. ) ;
#27537=LINE ( 'NONE', #32083, #50888 ) ;
#27538=DIRECTION ( 'NONE',  ( 0.000000000000000000, -0.000000000000000000, -1.000000000000000000 ) ) ;
#27539=DIRECTION ( 'NONE',  ( -0.5364919789714478471, 0.6444004775717705469, -0.5449076811759709926 ) ) ;
#27540=ORIENTED_EDGE ( 'NONE', *, *, #10159, .T. ) ;
#27542=AXIS2_PLACEMENT_3D ( 'NONE', #34680, #42928, #8579 ) ;
#27543=LINE ( 'NONE', #23005, #44033 ) ;
#27545=VECTOR ( 'NONE', #11845, 1000.000000000000227 ) ;
#27546=VERTEX_POINT ( 'NONE', #13890 ) ;
#27547=DIRECTION ( 'NONE',  ( -0.005961354470445682716, -0.6427876096865404731, 0.7660212471507180654 ) ) ;
#27548=VECTOR ( 'NONE', #4482, 1000.000000000000227 ) ;
#27549=ORIENTED_EDGE ( 'NONE', *, *, #39377, .T. ) ;
#27551=ORIENTED_EDGE ( 'NONE', *, *, #50261, .T. ) ;
#27552=VERTEX_POINT ( 'NONE', #35225 ) ;
#27553=VERTEX_POINT ( 'NONE', #44291 ) ;
#27554=CARTESIAN_POINT ( 'NONE',  ( -17.20686196644532728, 0.000000000000000000, 6.163827626255103276 ) ) ;
#27555=VECTOR ( 'NONE', #45700, 1000.000000000000227 ) ;
#27556=CARTESIAN_POINT ( 'NONE',  ( 2.072287782118878319, 0.000000000000000000, -2.950529333540147015 ) ) ;
#27557=PLANE ( 'NONE',  #49358 ) ;
#27558=ADVANCED_FACE ( 'NONE', ( #48545 ), #22699, .F. ) ;
#27559=VECTOR ( 'NONE', #24426, 1000.000000000000227 ) ;
#27560=CARTESIAN_POINT ( 'NONE',  ( -16.43317633868556626, -0.1191753592594197858, 13.31363028683540151 ) ) ;
#27561=ORIENTED_EDGE ( 'NONE', *, *, #48204, .T. ) ;
#27562=ADVANCED_FACE ( 'NONE', ( #9353 ), #1393, .F. ) ;
#27563=ORIENTED_EDGE ( 'NONE', *, *, #26540, .T. ) ;
#27564=AXIS2_PLACEMENT_3D ( 'NONE', #19851, #40872, #11332 ) ;
#27565=AXIS2_PLACEMENT_3D ( 'NONE', #6957, #14903, #28509 ) ;
#27566=CARTESIAN_POINT ( 'NONE',  ( -11.34358382343173410, 0.000000000000000000, 3.254800454061105963 ) ) ;
#27567=EDGE_LOOP ( 'NONE', ( #23190, #23260, #806, #11017 ) ) ;
#27568=EDGE_CURVE ( 'NONE', #43270, #428, #1096, .T. ) ;
#27569=DIRECTION ( 'NONE',  ( -0.9999697198139514409, -0.000000000000000000, -0.007781995580013368816 ) ) ;
#27570=ORIENTED_EDGE ( 'NONE', *, *, #40533, .F. ) ;
#27571=CARTESIAN_POINT ( 'NONE',  ( -20.54049170961573267, 0.000000000000000000, 4.660556269540326646 ) ) ;
#27572=PLANE ( 'NONE',  #17652 ) ;
#27573=EDGE_CURVE ( 'NONE', #3951, #931, #833, .T. ) ;
#27574=EDGE_CURVE ( 'NONE', #50902, #10838, #18434, .T. ) ;
#27575=ADVANCED_FACE ( 'NONE', ( #26677 ), #43997, .F. ) ;
#27576=ORIENTED_EDGE ( 'NONE', *, *, #16680, .T. ) ;
#27577=DIRECTION ( 'NONE',  ( -0.9999697198139514409, -0.000000000000000000, -0.007781995580013368816 ) ) ;
#27578=ORIENTED_EDGE ( 'NONE', *, *, #9618, .T. ) ;
#27579=ADVANCED_FACE ( 'NONE', ( #49089 ), #18740, .F. ) ;
#27580=VECTOR ( 'NONE', #52705, 1000.000000000000227 ) ;
#27581=DIRECTION ( 'NONE',  ( 0.000000000000000000, -0.000000000000000000, -1.000000000000000000 ) ) ;
#27582=AXIS2_PLACEMENT_3D ( 'NONE', #26235, #35062, #21120 ) ;
#27583=VERTEX_POINT ( 'NONE', #53090 ) ;
#27584=CARTESIAN_POINT ( 'NONE',  ( -17.46532115785441519, 0.000000000000000000, 13.67492996699914265 ) ) ;
#27585=CARTESIAN_POINT ( 'NONE',  ( -10.06709704724974763, 0.4073222041869798971, 1.076279759381168599 ) ) ;
#27586=PLANE ( 'NONE',  #53689 ) ;
#27587=ORIENTED_EDGE ( 'NONE', *, *, #35223, .T. ) ;
#27588=VECTOR ( 'NONE', #16324, 1000.000000000000227 ) ;
#27589=CARTESIAN_POINT ( 'NONE',  ( -16.41364898034673558, -0.1191753592594159833, 9.593992249496130498 ) ) ;
#27590=CARTESIAN_POINT ( 'NONE',  ( -12.13851405436063047, 0.000000000000000000, 11.68505802764555135 ) ) ;
#27592=EDGE_CURVE ( 'NONE', #21318, #29013, #48833, .T. ) ;
#27593=VECTOR ( 'NONE', #1855, 999.9999999999998863 ) ;
#27594=CARTESIAN_POINT ( 'NONE',  ( -18.19747506107908563, 0.000000000000000000, 14.03856424583689311 ) ) ;
#27595=PLANE ( 'NONE',  #3146 ) ;
#27596=FACE_OUTER_BOUND ( 'NONE', #13548, .T. ) ;
#27597=EDGE_CURVE ( 'NONE', #14368, #4104, #44546, .T. ) ;
#27599=ORIENTED_EDGE ( 'NONE', *, *, #55023, .T. ) ;
#27600=CARTESIAN_POINT ( 'NONE',  ( -3.184385661761863773, -6.114012816731704270, -1.981450042443219539 ) ) ;
#27601=CARTESIAN_POINT ( 'NONE',  ( -15.40103151951671734, 0.000000000000000000, 12.95233060667165681 ) ) ;
#27602=EDGE_CURVE ( 'NONE', #18340, #26523, #5121, .T. ) ;
#27604=ORIENTED_EDGE ( 'NONE', *, *, #25614, .F. ) ;
#27605=VECTOR ( 'NONE', #5090, 1000.000000000000000 ) ;
#27606=PLANE ( 'NONE',  #55611 ) ;
#27607=LINE ( 'NONE', #40928, #53560 ) ;
#27608=ORIENTED_EDGE ( 'NONE', *, *, #26188, .T. ) ;
#27609=VECTOR ( 'NONE', #7316, 1000.000000000000227 ) ;
#27610=EDGE_CURVE ( 'NONE', #26525, #19811, #53373, .T. ) ;
#27612=DIRECTION ( 'NONE',  ( 0.007781995580012663651, -3.146120232559066537E-19, -0.9999697198139514409 ) ) ;
#27613=EDGE_CURVE ( 'NONE', #34665, #40913, #27234, .T. ) ;
#27614=CARTESIAN_POINT ( 'NONE',  ( -19.91123888593303803, 0.7721120973665051013, 5.882689981159765047 ) ) ;
#27615=ORIENTED_EDGE ( 'NONE', *, *, #5751, .T. ) ;
#27616=VECTOR ( 'NONE', #43594, 999.9999999999998863 ) ;
#27617=AXIS2_PLACEMENT_3D ( 'NONE', #12871, #16559, #7482 ) ;
#27618=ORIENTED_EDGE ( 'NONE', *, *, #18745, .F. ) ;
#27619=PLANE ( 'NONE',  #38606 ) ;
#27620=DIRECTION ( 'NONE',  ( 0.007781995580012663651, 0.000000000000000000, -0.9999697198139515519 ) ) ;
#27621=CARTESIAN_POINT ( 'NONE',  ( -16.36399307677613280, -0.1191753592594193417, 4.423729705925692812 ) ) ;
#27622=CARTESIAN_POINT ( 'NONE',  ( -27.99767448711536133, 0.000000000000000000, 7.557179307314289218 ) ) ;
#27623=ORIENTED_EDGE ( 'NONE', *, *, #15567, .F. ) ;
#27625=ORIENTED_EDGE ( 'NONE', *, *, #17770, .T. ) ;
#27626=CARTESIAN_POINT ( 'NONE',  ( -17.65293688786543314, 0.000000000000000000, 3.775037735645530912 ) ) ;
#27627=AXIS2_PLACEMENT_3D ( 'NONE', #55099, #29545, #479 ) ;
#27628=PLANE ( 'NONE',  #39571 ) ;
#27629=ORIENTED_EDGE ( 'NONE', *, *, #19798, .F. ) ;
#27630=VECTOR ( 'NONE', #45715, 1000.000000000000114 ) ;
#27631=CARTESIAN_POINT ( 'NONE',  ( -13.68433194158294164, 3.848249166794009746, 8.512412852383034689 ) ) ;
#27632=CARTESIAN_POINT ( 'NONE',  ( -31.72626587586518099, 0.000000000000000000, 9.005490826201270949 ) ) ;
#27633=VECTOR ( 'NONE', #17306, 1000.000000000000000 ) ;
#27635=ORIENTED_EDGE ( 'NONE', *, *, #41123, .T. ) ;
#27636=CARTESIAN_POINT ( 'NONE',  ( -13.63673279712320507, -0.1191753592594197858, 12.22739664767016521 ) ) ;
#27637=ORIENTED_EDGE ( 'NONE', *, *, #35791, .T. ) ;
#27638=ORIENTED_EDGE ( 'NONE', *, *, #12053, .F. ) ;
#27639=ORIENTED_EDGE ( 'NONE', *, *, #8058, .F. ) ;
#27640=DIRECTION ( 'NONE',  ( -0.5364919789714478471, 0.6444004775717705469, -0.5449076811759709926 ) ) ;
#27641=AXIS2_PLACEMENT_3D ( 'NONE', #36831, #2700, #27753 ) ;
#27642=ORIENTED_EDGE ( 'NONE', *, *, #14569, .T. ) ;
#27643=AXIS2_PLACEMENT_3D ( 'NONE', #41650, #20063, #28894 ) ;
#27644=CARTESIAN_POINT ( 'NONE',  ( -17.22566268659302580, 0.000000000000000000, 8.579679789764480091 ) ) ;
#27645=VERTEX_POINT ( 'NONE', #43700 ) ;
#27646=DIRECTION ( 'NONE',  ( -0.3313982828793700097, 0.4028455766673915694, -0.8531650599175529814 ) ) ;
#27647=CARTESIAN_POINT ( 'NONE',  ( -18.40664086144219169, -1.975113310420657520, 7.073193565548556272 ) ) ;
#27648=AXIS2_PLACEMENT_3D ( 'NONE', #42950, #25358, #12304 ) ;
#27649=EDGE_CURVE ( 'NONE', #32585, #12755, #17902, .T. ) ;
#27650=EDGE_CURVE ( 'NONE', #43814, #44524, #19835, .T. ) ;
#27651=ORIENTED_EDGE ( 'NONE', *, *, #1326, .F. ) ;
#27652=LINE ( 'NONE', #35603, #4985 ) ;
#27654=ADVANCED_FACE ( 'NONE', ( #53912 ), #45966, .F. ) ;
#27655=VECTOR ( 'NONE', #19435, 1000.000000000000227 ) ;
#27656=DIRECTION ( 'NONE',  ( -0.6427681459581293666, -0.7660444431189770143, -0.005002170337467561935 ) ) ;
#27657=VECTOR ( 'NONE', #52391, 999.9999999999998863 ) ;
#27658=PLANE ( 'NONE',  #54686 ) ;
#27659=DIRECTION ( 'NONE',  ( -0.3620778797217457656, 0.000000000000000000, -0.9321478471874539151 ) ) ;
#27660=CARTESIAN_POINT ( 'NONE',  ( -19.79006065298467121, -3.594132820645660420, 10.26764763322216112 ) ) ;
#27662=PLANE ( 'NONE',  #11939 ) ;
#27663=CARTESIAN_POINT ( 'NONE',  ( 2.072287782118878319, 0.000000000000000000, -2.950529333540147015 ) ) ;
#27664=ORIENTED_EDGE ( 'NONE', *, *, #6171, .T. ) ;
#27666=DIRECTION ( 'NONE',  ( 0.9999697198139515519, 0.000000000000000000, 0.007781995580013368816 ) ) ;
#27667=DIRECTION ( 'NONE',  ( 0.7660212471507180654, -0.6427876096865404731, 0.005961354470445141482 ) ) ;
#27668=PLANE ( 'NONE',  #42401 ) ;
#27669=VECTOR ( 'NONE', #17259, 1000.000000000000227 ) ;
#27670=CARTESIAN_POINT ( 'NONE',  ( -15.13495153988577968, 0.000000000000000000, 12.76973526769478084 ) ) ;
#27673=DIRECTION ( 'NONE',  ( -0.6427681459581293666, -0.7660444431189770143, -0.005002170337467561935 ) ) ;
#27674=CARTESIAN_POINT ( 'NONE',  ( -10.43598480340254397, 0.000000000000000000, 6.047194144364267387 ) ) ;
#27676=LINE ( 'NONE', #5268, #35679 ) ;
#27677=DIRECTION ( 'NONE',  ( 0.007781995580012662783, 0.000000000000000000, -0.9999697198139514409 ) ) ;
#27678=VECTOR ( 'NONE', #15706, 999.9999999999998863 ) ;
#27679=VERTEX_POINT ( 'NONE', #10768 ) ;
#27680=PLANE ( 'NONE',  #4390 ) ;
#27681=CARTESIAN_POINT ( 'NONE',  ( -17.85580488533350518, 0.000000000000000000, 4.142791039787291574 ) ) ;
#27682=VECTOR ( 'NONE', #29771, 1000.000000000000227 ) ;
#27683=DIRECTION ( 'NONE',  ( -0.8531650599175527594, 0.4028455766673922356, 0.3313982828793700652 ) ) ;
#27684=ADVANCED_FACE ( 'NONE', ( #11021 ), #37730, .F. ) ;
#27685=LINE ( 'NONE', #49810, #30551 ) ;
#27686=FACE_OUTER_BOUND ( 'NONE', #41275, .T. ) ;
#27687=ORIENTED_EDGE ( 'NONE', *, *, #55673, .F. ) ;
#27688=VECTOR ( 'NONE', #1527, 1000.000000000000227 ) ;
#27689=VECTOR ( 'NONE', #4061, 1000.000000000000227 ) ;
#27691=ORIENTED_EDGE ( 'NONE', *, *, #53935, .F. ) ;
#27692=AXIS2_PLACEMENT_3D ( 'NONE', #38467, #4122, #8367 ) ;
#27693=PLANE ( 'NONE',  #27565 ) ;
#27694=DIRECTION ( 'NONE',  ( -0.6427681459581293666, -0.7660444431189770143, -0.005002170337467561935 ) ) ;
#27695=DIRECTION ( 'NONE',  ( 0.5364919789714477361, 0.6444004775717706579, 0.5449076811759711036 ) ) ;
#27696=ADVANCED_FACE ( 'NONE', ( #20090 ), #15029, .F. ) ;
#27697=AXIS2_PLACEMENT_3D ( 'NONE', #55309, #16404, #38567 ) ;
#27698=DIRECTION ( 'NONE',  ( 0.007781995580012663651, 0.000000000000000000, -0.9999697198139515519 ) ) ;
#27699=ADVANCED_FACE ( 'NONE', ( #41433 ), #16142, .F. ) ;
#27700=CARTESIAN_POINT ( 'NONE',  ( -12.72887235343914725, 0.000000000000000000, 2.136023608983785849 ) ) ;
#27701=ORIENTED_EDGE ( 'NONE', *, *, #381, .T. ) ;
#27702=DIRECTION ( 'NONE',  ( 0.000000000000000000, -1.000000000000000000, 0.000000000000000000 ) ) ;
#27703=DIRECTION ( 'NONE',  ( -0.9999697198139514409, -0.000000000000000000, -0.007781995580013368816 ) ) ;
#27704=VECTOR ( 'NONE', #43357, 1000.000000000000000 ) ;
#27705=DIRECTION ( 'NONE',  ( 0.005961354470445682716, -0.6427876096865404731, -0.7660212471507180654 ) ) ;
#27707=PLANE ( 'NONE',  #9692 ) ;
#27708=ORIENTED_EDGE ( 'NONE', *, *, #36904, .F. ) ;
#27709=DIRECTION ( 'NONE',  ( 0.005961354470445682716, -0.6427876096865404731, -0.7660212471507180654 ) ) ;
#27710=VERTEX_POINT ( 'NONE', #41953 ) ;
#27711=FACE_OUTER_BOUND ( 'NONE', #37106, .T. ) ;
#27712=DIRECTION ( 'NONE',  ( 0.005961354470445682716, -0.6427876096865404731, -0.7660212471507180654 ) ) ;
#27713=EDGE_LOOP ( 'NONE', ( #40497, #24537, #23408, #29230 ) ) ;
#27714=LINE ( 'NONE', #1591, #12709 ) ;
#27715=ORIENTED_EDGE ( 'NONE', *, *, #36943, .F. ) ;
#27716=VECTOR ( 'NONE', #51826, 1000.000000000000000 ) ;
#27717=ORIENTED_EDGE ( 'NONE', *, *, #44544, .F. ) ;
#27718=ORIENTED_EDGE ( 'NONE', *, *, #20528, .T. ) ;
#27720=ORIENTED_EDGE ( 'NONE', *, *, #41395, .T. ) ;
#27721=AXIS2_PLACEMENT_3D ( 'NONE', #21875, #38079, #55391 ) ;
#27722=ORIENTED_EDGE ( 'NONE', *, *, #17215, .T. ) ;
#27723=DIRECTION ( 'NONE',  ( 0.000000000000000000, -1.000000000000000000, 0.000000000000000000 ) ) ;
#27724=CARTESIAN_POINT ( 'NONE',  ( -29.86352658060627618, 0.000000000000000000, 8.481329010720569883 ) ) ;
#27725=VECTOR ( 'NONE', #53565, 1000.000000000000227 ) ;
#27726=ORIENTED_EDGE ( 'NONE', *, *, #28272, .T. ) ;
#27727=EDGE_CURVE ( 'NONE', #50963, #15779, #15848, .T. ) ;
#27728=ORIENTED_EDGE ( 'NONE', *, *, #53929, .T. ) ;
#27729=CARTESIAN_POINT ( 'NONE',  ( -10.22449464541862341, 0.000000000000000000, 4.571511730449213218 ) ) ;
#27730=ORIENTED_EDGE ( 'NONE', *, *, #6596, .F. ) ;
#27731=VECTOR ( 'NONE', #21664, 1000.000000000000227 ) ;
#27732=ORIENTED_EDGE ( 'NONE', *, *, #55868, .T. ) ;
#27733=EDGE_CURVE ( 'NONE', #39217, #2132, #50509, .T. ) ;
#27734=EDGE_CURVE ( 'NONE', #3468, #26120, #3059, .T. ) ;
#27735=VECTOR ( 'NONE', #17660, 1000.000000000000227 ) ;
#27736=VECTOR ( 'NONE', #31351, 1000.000000000000227 ) ;
#27737=LINE ( 'NONE', #10702, #4801 ) ;
#27738=DIRECTION ( 'NONE',  ( 0.000000000000000000, -1.000000000000000000, 0.000000000000000000 ) ) ;
#27740=CARTESIAN_POINT ( 'NONE',  ( -26.13415699229845757, -0.1191753592594197858, 6.933020519852192365 ) ) ;
#27741=ORIENTED_EDGE ( 'NONE', *, *, #1578, .T. ) ;
#27742=DIRECTION ( 'NONE',  ( 0.000000000000000000, -1.000000000000000000, 0.000000000000000000 ) ) ;
#27743=VERTEX_POINT ( 'NONE', #28077 ) ;
#27744=VECTOR ( 'NONE', #27683, 999.9999999999998863 ) ;
#27745=VECTOR ( 'NONE', #25536, 1000.000000000000114 ) ;
#27746=AXIS2_PLACEMENT_3D ( 'NONE', #53932, #32906, #46234 ) ;
#27747=CARTESIAN_POINT ( 'NONE',  ( -14.94916102560700821, 0.000000000000000000, 2.688082935172642962 ) ) ;
#27748=EDGE_CURVE ( 'NONE', #36809, #26836, #11604, .T. ) ;
#27749=VECTOR ( 'NONE', #31688, 999.9999999999998863 ) ;
#27750=LINE ( 'NONE', #45070, #45123 ) ;
#27751=VECTOR ( 'NONE', #50444, 1000.000000000000227 ) ;
#27752=LINE ( 'NONE', #19191, #12267 ) ;
#27753=DIRECTION ( 'NONE',  ( 0.005002170337468016433, -0.7660444431189770143, -0.6427681459581293666 ) ) ;
#27754=FACE_OUTER_BOUND ( 'NONE', #23637, .T. ) ;
#27755=DIRECTION ( 'NONE',  ( 0.000000000000000000, -1.000000000000000000, 0.000000000000000000 ) ) ;
#27756=EDGE_LOOP ( 'NONE', ( #12838, #8659, #49417, #12895 ) ) ;
#27757=CARTESIAN_POINT ( 'NONE',  ( 1.086233639165236964, 0.000000000000000000, 2.796443541562362078 ) ) ;
#27759=CARTESIAN_POINT ( 'NONE',  ( -13.94446387365259810, 0.000000000000000000, 4.911894139562900996 ) ) ;
#27760=DIRECTION ( 'NONE',  ( -0.7660212471507179544, -0.6427876096865405842, -0.005961354470445141482 ) ) ;
#27761=DIRECTION ( 'NONE',  ( -0.7660212471507179544, -0.6427876096865405842, -0.005961354470445141482 ) ) ;
#27762=FACE_OUTER_BOUND ( 'NONE', #29951, .T. ) ;
#27763=DIRECTION ( 'NONE',  ( 0.6427681459581294776, -0.7660444431189769032, 0.005002170337467562802 ) ) ;
#27764=AXIS2_PLACEMENT_3D ( 'NONE', #9166, #29922, #17402 ) ;
#27766=ORIENTED_EDGE ( 'NONE', *, *, #25515, .F. ) ;
#27767=CARTESIAN_POINT ( 'NONE',  ( -23.33693525117809386, 0.000000000000000000, 5.746789908705562944 ) ) ;
#27768=LINE ( 'NONE', #49874, #53919 ) ;
#27769=DIRECTION ( 'NONE',  ( -0.5364919789714478471, 0.6444004775717705469, -0.5449076811759709926 ) ) ;
#27770=VECTOR ( 'NONE', #21393, 1000.000000000000227 ) ;
#27772=EDGE_CURVE ( 'NONE', #9097, #52074, #6236, .T. ) ;
#27773=VECTOR ( 'NONE', #3691, 1000.000000000000000 ) ;
#27774=CARTESIAN_POINT ( 'NONE',  ( -17.31625929850056878, -0.1191753592594162470, 7.370975508451782510 ) ) ;
#27775=PLANE ( 'NONE',  #5512 ) ;
#27776=LINE ( 'NONE', #45619, #26542 ) ;
#27777=AXIS2_PLACEMENT_3D ( 'NONE', #55306, #29185, #12152 ) ;
#27778=AXIS2_PLACEMENT_3D ( 'NONE', #49788, #37556, #6352 ) ;
#27780=CARTESIAN_POINT ( 'NONE',  ( -12.55630129013990448, 0.000000000000000000, 5.661361281382457200 ) ) ;
#27782=EDGE_CURVE ( 'NONE', #42852, #6281, #32612, .T. ) ;
#27783=ORIENTED_EDGE ( 'NONE', *, *, #24695, .F. ) ;
#27784=VECTOR ( 'NONE', #45946, 1000.000000000000000 ) ;
#27785=EDGE_CURVE ( 'NONE', #22811, #32117, #45382, .T. ) ;
#27786=EDGE_CURVE ( 'NONE', #15806, #45145, #2221, .T. ) ;
#27787=AXIS2_PLACEMENT_3D ( 'NONE', #40948, #19372, #15144 ) ;
#27788=EDGE_LOOP ( 'NONE', ( #32791, #20872, #29624, #20489 ) ) ;
#27789=VECTOR ( 'NONE', #49249, 1000.000000000000227 ) ;
#27790=ORIENTED_EDGE ( 'NONE', *, *, #51672, .F. ) ;
#27791=ORIENTED_EDGE ( 'NONE', *, *, #55505, .F. ) ;
#27792=VERTEX_POINT ( 'NONE', #54204 ) ;
#27793=DIRECTION ( 'NONE',  ( 0.9999697198139515519, 0.000000000000000000, 0.007781995580013368816 ) ) ;
#27794=EDGE_CURVE ( 'NONE', #54764, #43539, #24103, .T. ) ;
#27795=CARTESIAN_POINT ( 'NONE',  ( -13.08408713167409942, -0.1191753592594197858, 1.863930203747758085 ) ) ;
#27796=ORIENTED_EDGE ( 'NONE', *, *, #16105, .T. ) ;
#27797=EDGE_CURVE ( 'NONE', #9219, #40567, #50205, .T. ) ;
#27798=ORIENTED_EDGE ( 'NONE', *, *, #27459, .F. ) ;
#27799=ORIENTED_EDGE ( 'NONE', *, *, #27650, .T. ) ;
#27800=ADVANCED_FACE ( 'NONE', ( #17248 ), #38003, .F. ) ;
#27801=VECTOR ( 'NONE', #38809, 999.9999999999998863 ) ;
#27802=DIRECTION ( 'NONE',  ( 0.000000000000000000, -0.000000000000000000, -1.000000000000000000 ) ) ;
#27803=LINE ( 'NONE', #15285, #33729 ) ;
#27804=FACE_OUTER_BOUND ( 'NONE', #18302, .T. ) ;
#27805=EDGE_LOOP ( 'NONE', ( #44887, #18477, #39025, #45305 ) ) ;
#27806=VECTOR ( 'NONE', #47426, 999.9999999999998863 ) ;
#27807=CARTESIAN_POINT ( 'NONE',  ( -15.52856807626791813, -2.460819163488160655, 2.834631295277566743 ) ) ;
#27808=EDGE_CURVE ( 'NONE', #24601, #25044, #47346, .T. ) ;
#27809=VERTEX_POINT ( 'NONE', #29484 ) ;
#27810=DIRECTION ( 'NONE',  ( -0.6427681459581293666, -0.7660444431189770143, -0.005002170337467561935 ) ) ;
#27811=VECTOR ( 'NONE', #39000, 1000.000000000000227 ) ;
#27813=ADVANCED_FACE ( 'NONE', ( #25783 ), #55304, .F. ) ;
#27814=FACE_OUTER_BOUND ( 'NONE', #4190, .T. ) ;
#27815=DIRECTION ( 'NONE',  ( 0.7660212471507180654, -0.6427876096865404731, 0.005961354470445141482 ) ) ;
#27816=VECTOR ( 'NONE', #31464, 1000.000000000000000 ) ;
#27818=DIRECTION ( 'NONE',  ( 0.000000000000000000, -0.000000000000000000, -1.000000000000000000 ) ) ;
#27819=DIRECTION ( 'NONE',  ( -0.5449076811759708816, 0.6444004775717707689, 0.5364919789714475140 ) ) ;
#27820=CARTESIAN_POINT ( 'NONE',  ( -8.108005289889504752, 5.801717509616975299, -0.06894897205205396951 ) ) ;
#27822=FACE_OUTER_BOUND ( 'NONE', #29706, .T. ) ;
#27823=VERTEX_POINT ( 'NONE', #4486 ) ;
#27824=VECTOR ( 'NONE', #35917, 999.9999999999998863 ) ;
#27825=CARTESIAN_POINT ( 'NONE',  ( -17.94484721929616455, 1.743523803501505709, 6.713128782598690947 ) ) ;
#27826=DIRECTION ( 'NONE',  ( 0.7660212471507180654, -0.6427876096865404731, 0.005961354470445141482 ) ) ;
#27827=DIRECTION ( 'NONE',  ( 0.6427681459581294776, -0.7660444431189769032, 0.005002170337467562802 ) ) ;
#27828=DIRECTION ( 'NONE',  ( -0.7660212471507179544, -0.6427876096865405842, -0.005961354470445141482 ) ) ;
#27829=DIRECTION ( 'NONE',  ( 0.007781995580012663651, -3.146120232559066537E-19, -0.9999697198139514409 ) ) ;
#27830=DIRECTION ( 'NONE',  ( 0.005002170337468016433, -0.7660444431189770143, -0.6427681459581293666 ) ) ;
#27831=DIRECTION ( 'NONE',  ( 0.007781995580012662783, 0.000000000000000000, -0.9999697198139514409 ) ) ;
#27832=VECTOR ( 'NONE', #37772, 999.9999999999998863 ) ;
#27833=AXIS2_PLACEMENT_3D ( 'NONE', #13381, #42892, #47433 ) ;
#27834=CARTESIAN_POINT ( 'NONE',  ( -16.46321184919952785, 0.000000000000000000, 4.322954534386297176 ) ) ;
#27835=PLANE ( 'NONE',  #50995 ) ;
#27836=ORIENTED_EDGE ( 'NONE', *, *, #7414, .F. ) ;
#27837=DIRECTION ( 'NONE',  ( -0.005002170337468016433, -0.7660444431189770143, 0.6427681459581293666 ) ) ;
#27838=PLANE ( 'NONE',  #38516 ) ;
#27840=LINE ( 'NONE', #1113, #48510 ) ;
#27841=DIRECTION ( 'NONE',  ( 0.007781995580012663651, -3.146120232559066537E-19, -0.9999697198139514409 ) ) ;
#27842=EDGE_CURVE ( 'NONE', #10018, #14930, #21795, .T. ) ;
#27843=FACE_OUTER_BOUND ( 'NONE', #30432, .T. ) ;
#27844=DIRECTION ( 'NONE',  ( 0.9999697198139515519, 0.000000000000000000, 0.007781995580013368816 ) ) ;
#27845=CARTESIAN_POINT ( 'NONE',  ( -17.19536575242419474, 0.000000000000000000, 4.686588813224045857 ) ) ;
#27846=AXIS2_PLACEMENT_3D ( 'NONE', #19056, #49731, #6856 ) ;
#27847=ORIENTED_EDGE ( 'NONE', *, *, #13239, .T. ) ;
#27848=ORIENTED_EDGE ( 'NONE', *, *, #52909, .T. ) ;
#27849=CARTESIAN_POINT ( 'NONE',  ( -31.72626587586518099, 0.000000000000000000, 9.005490826201270949 ) ) ;
#27851=DIRECTION ( 'NONE',  ( -0.5364919789714478471, 0.6444004775717705469, -0.5449076811759709926 ) ) ;
#27852=ORIENTED_EDGE ( 'NONE', *, *, #45197, .T. ) ;
#27853=DIRECTION ( 'NONE',  ( 0.5364919789714477361, 0.6444004775717706579, 0.5449076811759711036 ) ) ;
#27854=VECTOR ( 'NONE', #54098, 1000.000000000000227 ) ;
#27855=ORIENTED_EDGE ( 'NONE', *, *, #55608, .T. ) ;
#27858=VECTOR ( 'NONE', #25637, 1000.000000000000227 ) ;
#27859=ORIENTED_EDGE ( 'NONE', *, *, #5661, .F. ) ;
#27860=ORIENTED_EDGE ( 'NONE', *, *, #14359, .F. ) ;
#27861=ORIENTED_EDGE ( 'NONE', *, *, #30439, .T. ) ;
#27862=LINE ( 'NONE', #23317, #46515 ) ;
#27863=CARTESIAN_POINT ( 'NONE',  ( -16.99924723426068951, 0.000000000000000000, 13.49389102713827171 ) ) ;
#27864=DIRECTION ( 'NONE',  ( -0.6427681459581293666, -0.7660444431189770143, -0.005002170337467561935 ) ) ;
#27865=VECTOR ( 'NONE', #32876, 999.9999999999998863 ) ;
#27866=EDGE_CURVE ( 'NONE', #40728, #44870, #8765, .T. ) ;
#27867=ORIENTED_EDGE ( 'NONE', *, *, #2516, .F. ) ;
#27868=ORIENTED_EDGE ( 'NONE', *, *, #30885, .T. ) ;
#27869=EDGE_CURVE ( 'NONE', #20518, #35510, #46805, .T. ) ;
#27870=AXIS2_PLACEMENT_3D ( 'NONE', #3518, #29670, #55196 ) ;
#27871=LINE ( 'NONE', #45179, #27273 ) ;
#27872=ORIENTED_EDGE ( 'NONE', *, *, #30959, .T. ) ;
#27873=CARTESIAN_POINT ( 'NONE',  ( -18.16355864079104165, 0.000000000000000000, 9.680377076001752457 ) ) ;
#27874=ORIENTED_EDGE ( 'NONE', *, *, #28887, .T. ) ;
#27875=DIRECTION ( 'NONE',  ( 0.9999697198139515519, 0.000000000000000000, 0.007781995580013368816 ) ) ;
#27876=CARTESIAN_POINT ( 'NONE',  ( -15.86710544311044302, 0.000000000000000000, 13.13336954653252953 ) ) ;
#27877=EDGE_CURVE ( 'NONE', #15287, #9855, #55892, .T. ) ;
#27878=ORIENTED_EDGE ( 'NONE', *, *, #52080, .F. ) ;
#27880=ADVANCED_FACE ( 'NONE', ( #51884 ), #13001, .F. ) ;
#27881=DIRECTION ( 'NONE',  ( -0.3620778797217455991, 0.000000000000000000, -0.9321478471874540261 ) ) ;
#27882=ORIENTED_EDGE ( 'NONE', *, *, #49876, .T. ) ;
#27883=DIRECTION ( 'NONE',  ( 0.005961354470445682716, -0.6427876096865404731, -0.7660212471507180654 ) ) ;
#27884=CARTESIAN_POINT ( 'NONE',  ( -15.50102849149811135, -0.1191753592594197858, 12.95155240711365430 ) ) ;
#27885=CARTESIAN_POINT ( 'NONE',  ( -15.07085755779227121, 0.000000000000000000, 4.533796213653115359 ) ) ;
#27886=VERTEX_POINT ( 'NONE', #30326 ) ;
#27887=DIRECTION ( 'NONE',  ( 0.5364919789714477361, 0.6444004775717706579, 0.5449076811759711036 ) ) ;
#27888=DIRECTION ( 'NONE',  ( -0.5449076811759708816, 0.6444004775717707689, 0.5364919789714475140 ) ) ;
#27889=DIRECTION ( 'NONE',  ( 0.5449076811759707706, 0.6444004775717708799, -0.5364919789714476250 ) ) ;
#27890=CARTESIAN_POINT ( 'NONE',  ( -13.56467548170849113, -0.1191753592594185229, 2.968186363502689051 ) ) ;
#27891=DIRECTION ( 'NONE',  ( -0.5364919789714478471, 0.6444004775717705469, -0.5449076811759709926 ) ) ;
#27892=DIRECTION ( 'NONE',  ( 0.9999697198139515519, 0.000000000000000000, 0.007781995580013368816 ) ) ;
#27893=VECTOR ( 'NONE', #54922, 1000.000000000000000 ) ;
#27895=ORIENTED_EDGE ( 'NONE', *, *, #38149, .T. ) ;
#27896=DIRECTION ( 'NONE',  ( -0.5364919789714478471, 0.6444004775717705469, -0.5449076811759709926 ) ) ;
#27898=CARTESIAN_POINT ( 'NONE',  ( -15.09672403933981499, 0.000000000000000000, 7.857583542972994550 ) ) ;
#27900=ORIENTED_EDGE ( 'NONE', *, *, #8048, .T. ) ;
#27901=PLANE ( 'NONE',  #41100 ) ;
#27902=CARTESIAN_POINT ( 'NONE',  ( -15.16696776448257822, 4.010151117816512567, 2.445352267504874444 ) ) ;
#27903=EDGE_CURVE ( 'NONE', #40567, #43820, #21232, .T. ) ;
#27904=VECTOR ( 'NONE', #47562, 999.9999999999998863 ) ;
#27905=DIRECTION ( 'NONE',  ( 0.007781995580012663651, 0.000000000000000000, -0.9999697198139515519 ) ) ;
#27906=EDGE_CURVE ( 'NONE', #53549, #46700, #189, .T. ) ;
#27907=DIRECTION ( 'NONE',  ( 0.7660212471507180654, -0.6427876096865404731, 0.005961354470445141482 ) ) ;
#27908=CARTESIAN_POINT ( 'NONE',  ( -17.28751876344774274, -0.1191753592594176486, 3.677878475874140740 ) ) ;
#27909=EDGE_LOOP ( 'NONE', ( #29666, #27540, #1646, #53484 ) ) ;
#27910=EDGE_CURVE ( 'NONE', #8254, #8418, #33459, .T. ) ;
#27911=EDGE_LOOP ( 'NONE', ( #43041, #32036, #34291, #2035 ) ) ;
#27912=EDGE_CURVE ( 'NONE', #52707, #52840, #29183, .T. ) ;
#27913=CARTESIAN_POINT ( 'NONE',  ( -10.18275984876991558, -0.1191753592594204103, 0.7785127941096396942 ) ) ;
#27915=EDGE_CURVE ( 'NONE', #43426, #51541, #24941, .T. ) ;
#27916=ADVANCED_FACE ( 'NONE', ( #20688 ), #16400, .F. ) ;
#27917=EDGE_CURVE ( 'NONE', #44396, #48501, #51040, .T. ) ;
#27918=LINE ( 'NONE', #40687, #34766 ) ;
#27919=ORIENTED_EDGE ( 'NONE', *, *, #19588, .T. ) ;
#27920=CARTESIAN_POINT ( 'NONE',  ( -17.83139810946674686, -0.1191753592594197858, 13.85674710641801788 ) ) ;
#27921=ORIENTED_EDGE ( 'NONE', *, *, #18647, .F. ) ;
#27922=DIRECTION ( 'NONE',  ( -0.7660212471507179544, -0.6427876096865405842, -0.005961354470445141482 ) ) ;
#27923=ORIENTED_EDGE ( 'NONE', *, *, #21094, .F. ) ;
#27924=CARTESIAN_POINT ( 'NONE',  ( 2.072287782118878319, 0.000000000000000000, -2.950529333540147015 ) ) ;
#27925=DIRECTION ( 'NONE',  ( 0.007781995580012662783, 0.000000000000000000, -0.9999697198139514409 ) ) ;
#27926=PLANE ( 'NONE',  #7605 ) ;
#27927=VERTEX_POINT ( 'NONE', #12150 ) ;
#27928=PLANE ( 'NONE',  #53749 ) ;
#27930=ORIENTED_EDGE ( 'NONE', *, *, #29853, .F. ) ;
#27931=ADVANCED_FACE ( 'NONE', ( #10135 ), #31463, .F. ) ;
#27932=ORIENTED_EDGE ( 'NONE', *, *, #21867, .T. ) ;
#27933=ORIENTED_EDGE ( 'NONE', *, *, #14689, .T. ) ;
#27934=DIRECTION ( 'NONE',  ( 0.005002170337468016433, -0.7660444431189770143, -0.6427681459581293666 ) ) ;
#27935=ADVANCED_FACE ( 'NONE', ( #1329 ), #27452, .F. ) ;
#27936=ORIENTED_EDGE ( 'NONE', *, *, #35403, .F. ) ;
#27937=CARTESIAN_POINT ( 'NONE',  ( -12.80458192191714595, 0.000000000000000000, 11.86454056839041726 ) ) ;
#27938=ORIENTED_EDGE ( 'NONE', *, *, #47024, .T. ) ;
#27939=LINE ( 'NONE', #37007, #19483 ) ;
#27941=EDGE_CURVE ( 'NONE', #21134, #5084, #35170, .T. ) ;
#27942=VECTOR ( 'NONE', #38977, 999.9999999999998863 ) ;
#27943=ORIENTED_EDGE ( 'NONE', *, *, #2751, .F. ) ;
#27944=FACE_OUTER_BOUND ( 'NONE', #54779, .T. ) ;
#27947=FACE_OUTER_BOUND ( 'NONE', #25037, .T. ) ;
#27948=PLANE ( 'NONE',  #15958 ) ;
#27949=CARTESIAN_POINT ( 'NONE',  ( -4.849237023859344298, 4.749459929012077808, 5.101981916513284254 ) ) ;
#27950=PLANE ( 'NONE',  #49588 ) ;
#27951=DIRECTION ( 'NONE',  ( 0.000000000000000000, -1.000000000000000000, 0.000000000000000000 ) ) ;
#27952=DIRECTION ( 'NONE',  ( 0.6427681459581294776, -0.7660444431189769032, 0.005002170337467562802 ) ) ;
#27953=VERTEX_POINT ( 'NONE', #14420 ) ;
#27955=LINE ( 'NONE', #53759, #36439 ) ;
#27956=PLANE ( 'NONE',  #33010 ) ;
#27958=DIRECTION ( 'NONE',  ( 0.005002170337468016433, -0.7660444431189770143, -0.6427681459581293666 ) ) ;
#27959=CARTESIAN_POINT ( 'NONE',  ( -17.41990852354524577, 0.000000000000000000, 7.839503984132946357 ) ) ;
#27960=ORIENTED_EDGE ( 'NONE', *, *, #7375, .F. ) ;
#27961=CARTESIAN_POINT ( 'NONE',  ( -18.62244743062156260, 0.000000000000000000, 8.938141757718215175 ) ) ;
#27962=LINE ( 'NONE', #50360, #16897 ) ;
#27963=ORIENTED_EDGE ( 'NONE', *, *, #8043, .F. ) ;
#27964=DIRECTION ( 'NONE',  ( -0.5449076811759708816, 0.6444004775717707689, 0.5364919789714475140 ) ) ;
#27965=LINE ( 'NONE', #48707, #47617 ) ;
#27966=ORIENTED_EDGE ( 'NONE', *, *, #34271, .T. ) ;
#27968=FACE_OUTER_BOUND ( 'NONE', #24795, .T. ) ;
#27969=CARTESIAN_POINT ( 'NONE',  ( -11.87243407472968926, 0.000000000000000000, 11.50246268866867361 ) ) ;
#27970=LINE ( 'NONE', #31931, #5130 ) ;
#27971=DIRECTION ( 'NONE',  ( 0.5364919789714477361, 0.6444004775717706579, 0.5449076811759711036 ) ) ;
#27972=VERTEX_POINT ( 'NONE', #26612 ) ;
#27973=VERTEX_POINT ( 'NONE', #52464 ) ;
#27974=LINE ( 'NONE', #28809, #29391 ) ;
#27975=CARTESIAN_POINT ( 'NONE',  ( -16.28489267888972591, 0.000000000000000000, 7.109672800269438042 ) ) ;
#27976=DIRECTION ( 'NONE',  ( 0.5364919789714477361, 0.6444004775717706579, 0.5449076811759711036 ) ) ;
#27977=EDGE_CURVE ( 'NONE', #2279, #10694, #22918, .T. ) ;
#27978=EDGE_CURVE ( 'NONE', #3951, #51394, #39410, .T. ) ;
#27979=VECTOR ( 'NONE', #13223, 1000.000000000000227 ) ;
#27981=DIRECTION ( 'NONE',  ( 0.9999697198139515519, 0.000000000000000000, 0.007781995580013368816 ) ) ;
#27982=VERTEX_POINT ( 'NONE', #26920 ) ;
#27983=EDGE_CURVE ( 'NONE', #52378, #46741, #5055, .T. ) ;
#27984=DIRECTION ( 'NONE',  ( 0.005002170337468016433, -0.7660444431189770143, -0.6427681459581293666 ) ) ;
#27985=DIRECTION ( 'NONE',  ( 0.007781995580012663651, -3.146120232559066537E-19, -0.9999697198139514409 ) ) ;
#27986=PLANE ( 'NONE',  #48680 ) ;
#27987=EDGE_LOOP ( 'NONE', ( #44407, #164, #25086, #53803 ) ) ;
#27988=CARTESIAN_POINT ( 'NONE',  ( -29.86197018149027116, 0.000000000000000000, 8.281335066757780083 ) ) ;
#27989=EDGE_LOOP ( 'NONE', ( #34336, #15238, #41106, #48089 ) ) ;
#27990=CARTESIAN_POINT ( 'NONE',  ( -27.99923088623136636, 0.000000000000000000, 7.757173251277078130 ) ) ;
#27991=CARTESIAN_POINT ( 'NONE',  ( -19.94248935626058383, 3.038739411681508518, 4.331320150471698049 ) ) ;
#27992=ORIENTED_EDGE ( 'NONE', *, *, #50598, .T. ) ;
#27993=DIRECTION ( 'NONE',  ( 0.007781995580012663651, -3.146120232559066537E-19, -0.9999697198139514409 ) ) ;
#27994=ORIENTED_EDGE ( 'NONE', *, *, #51269, .F. ) ;
#27995=ORIENTED_EDGE ( 'NONE', *, *, #19157, .F. ) ;
#27997=CARTESIAN_POINT ( 'NONE',  ( -27.06552663992790997, 0.000000000000000000, 7.195101427592543786 ) ) ;
#27998=ORIENTED_EDGE ( 'NONE', *, *, #438, .T. ) ;
#27999=EDGE_CURVE ( 'NONE', #931, #33376, #30873, .T. ) ;
#28000=ORIENTED_EDGE ( 'NONE', *, *, #46752, .T. ) ;
#28001=LINE ( 'NONE', #23184, #33814 ) ;
#28002=ORIENTED_EDGE ( 'NONE', *, *, #21110, .T. ) ;
#28003=ADVANCED_FACE ( 'NONE', ( #22383 ), #27178, .F. ) ;
#28004=ORIENTED_EDGE ( 'NONE', *, *, #1547, .F. ) ;
#28005=DIRECTION ( 'NONE',  ( -0.5364919789714478471, 0.6444004775717705469, -0.5449076811759709926 ) ) ;
#28006=ORIENTED_EDGE ( 'NONE', *, *, #15907, .F. ) ;
#28007=VERTEX_POINT ( 'NONE', #35420 ) ;
#28008=CARTESIAN_POINT ( 'NONE',  ( -13.03818250801268341, 0.000000000000000000, 7.873603589161035643 ) ) ;
#28009=LINE ( 'NONE', #22626, #17607 ) ;
#28010=LINE ( 'NONE', #45062, #53197 ) ;
#28011=DIRECTION ( 'NONE',  ( -0.5449076811759708816, 0.6444004775717707689, 0.5364919789714475140 ) ) ;
#28012=EDGE_CURVE ( 'NONE', #33376, #23572, #44778, .T. ) ;
#28013=EDGE_LOOP ( 'NONE', ( #36003, #47217, #27664, #31334 ) ) ;
#28014=DIRECTION ( 'NONE',  ( 0.000000000000000000, -0.000000000000000000, -1.000000000000000000 ) ) ;
#28015=ORIENTED_EDGE ( 'NONE', *, *, #36547, .F. ) ;
#28016=VECTOR ( 'NONE', #25629, 999.9999999999998863 ) ;
#28017=ORIENTED_EDGE ( 'NONE', *, *, #19082, .T. ) ;
#28019=UNCERTAINTY_MEASURE_WITH_UNIT (LENGTH_MEASURE( 1.000000000000000082E-05 ), #43780, 'distance_accuracy_value', 'NONE');
#28020=LINE ( 'NONE', #24308, #31510 ) ;
#28021=CARTESIAN_POINT ( 'NONE',  ( -12.12982302922070943, -2.298917212465658721, 1.519608817024182823 ) ) ;
#28022=LINE ( 'NONE', #44771, #23933 ) ;
#28023=LINE ( 'NONE', #15245, #50364 ) ;
#28024=ORIENTED_EDGE ( 'NONE', *, *, #141, .F. ) ;
#28025=PLANE ( 'NONE',  #5713 ) ;
#28026=ORIENTED_EDGE ( 'NONE', *, *, #10563, .T. ) ;
#28027=CARTESIAN_POINT ( 'NONE',  ( -9.486592635183393796, 0.000000000000000000, 3.469258045095933607 ) ) ;
#28028=CARTESIAN_POINT ( 'NONE',  ( -11.40636015113596180, 0.000000000000000000, 11.32142374880780089 ) ) ;
#28029=CARTESIAN_POINT ( 'NONE',  ( -11.77243710274829525, -0.1191753592594197858, 11.50324088822667612 ) ) ;
#28030=PLANE ( 'NONE',  #48563 ) ;
#28031=CARTESIAN_POINT ( 'NONE',  ( -25.20278734466900517, 0.000000000000000000, 6.670939612111840944 ) ) ;
#28032=ORIENTED_EDGE ( 'NONE', *, *, #13043, .T. ) ;
#28033=LINE ( 'NONE', #1884, #43010 ) ;
#28034=DIRECTION ( 'NONE',  ( 0.6246952433987894571, -0.7422098413412800966, -0.2426528472758541777 ) ) ;
#28035=DIRECTION ( 'NONE',  ( 0.000000000000000000, -1.000000000000000000, 0.000000000000000000 ) ) ;
#28036=EDGE_CURVE ( 'NONE', #17736, #46146, #49032, .T. ) ;
#28037=DIRECTION ( 'NONE',  ( -0.6427681459581293666, -0.7660444431189770143, -0.005002170337467561935 ) ) ;
#28038=DIRECTION ( 'NONE',  ( 0.000000000000000000, -0.000000000000000000, -1.000000000000000000 ) ) ;
#28039=EDGE_CURVE ( 'NONE', #34678, #13391, #34869, .T. ) ;
#28040=CARTESIAN_POINT ( 'NONE',  ( -29.86352658060627618, 0.000000000000000000, 8.481329010720569883 ) ) ;
#28042=DIRECTION ( 'NONE',  ( 0.6427681459581294776, -0.7660444431189769032, 0.005002170337467562802 ) ) ;
#28044=LINE ( 'NONE', #45348, #45548 ) ;
#28045=ORIENTED_EDGE ( 'NONE', *, *, #34269, .T. ) ;
#28046=VECTOR ( 'NONE', #2306, 1000.000000000000227 ) ;
#28047=ORIENTED_EDGE ( 'NONE', *, *, #2710, .T. ) ;
#28048=ORIENTED_EDGE ( 'NONE', *, *, #52496, .T. ) ;
#28052=CARTESIAN_POINT ( 'NONE',  ( -16.79925329029790149, 0.000000000000000000, 13.49544742625427496 ) ) ;
#28053=LINE ( 'NONE', #23772, #33963 ) ;
#28054=ORIENTED_EDGE ( 'NONE', *, *, #41614, .F. ) ;
#28055=CARTESIAN_POINT ( 'NONE',  ( -10.49509204652727234, -0.3560938001956556742, 0.9466100262968846213 ) ) ;
#28056=ORIENTED_EDGE ( 'NONE', *, *, #37400, .T. ) ;
#28057=ADVANCED_FACE ( 'NONE', ( #18367 ), #13300, .F. ) ;
#28058=PLANE ( 'NONE',  #54642 ) ;
#28059=EDGE_CURVE ( 'NONE', #35551, #55216, #26329, .T. ) ;
#28060=DIRECTION ( 'NONE',  ( 0.000000000000000000, -1.000000000000000000, 0.000000000000000000 ) ) ;
#28061=CARTESIAN_POINT ( 'NONE',  ( -15.99570089885316015, 0.000000000000000000, 3.957260742896541839 ) ) ;
#28062=ORIENTED_EDGE ( 'NONE', *, *, #52201, .T. ) ;
#28063=CARTESIAN_POINT ( 'NONE',  ( -14.01701317841955508, 0.000000000000000000, 2.326005055450897085 ) ) ;
#28064=PLANE ( 'NONE',  #38211 ) ;
#28065=EDGE_CURVE ( 'NONE', #3615, #19197, #501, .T. ) ;
#28066=FACE_OUTER_BOUND ( 'NONE', #32761, .T. ) ;
#28067=LINE ( 'NONE', #32352, #30929 ) ;
#28068=CARTESIAN_POINT ( 'NONE',  ( -14.80158947260792424, -3.756034771668160577, 8.595664701519920570 ) ) ;
#28069=CARTESIAN_POINT ( 'NONE',  ( -17.68299507730753817, 0.000000000000000000, 7.637450527518151233 ) ) ;
#28070=FACE_OUTER_BOUND ( 'NONE', #7969, .T. ) ;
#28071=FACE_OUTER_BOUND ( 'NONE', #14567, .T. ) ;
#28072=FACE_OUTER_BOUND ( 'NONE', #22589, .T. ) ;
#28073=ORIENTED_EDGE ( 'NONE', *, *, #8216, .F. ) ;
#28074=LINE ( 'NONE', #19262, #55517 ) ;
#28075=ORIENTED_EDGE ( 'NONE', *, *, #4512, .T. ) ;
#28077=CARTESIAN_POINT ( 'NONE',  ( -10.89331719411706523, 0.000000000000000000, 5.104964882117939418 ) ) ;
#28078=LINE ( 'NONE', #32887, #35928 ) ;
#28079=PLANE ( 'NONE',  #43996 ) ;
#28080=DIRECTION ( 'NONE',  ( 0.005961354470445682716, -0.6427876096865404731, -0.7660212471507180654 ) ) ;
#28081=DIRECTION ( 'NONE',  ( -0.5449076811759708816, 0.6444004775717707689, 0.5364919789714475140 ) ) ;
#28082=CARTESIAN_POINT ( 'NONE',  ( -17.73140113748535285, 0.000000000000000000, 13.85752530597602039 ) ) ;
#28083=CARTESIAN_POINT ( 'NONE',  ( -17.66155904838128166, 0.000000000000000000, 4.882966845418824420 ) ) ;
#28084=EDGE_CURVE ( 'NONE', #48176, #26974, #32822, .T. ) ;
#28085=DIRECTION ( 'NONE',  ( 0.000000000000000000, -0.000000000000000000, -1.000000000000000000 ) ) ;
#28087=CARTESIAN_POINT ( 'NONE',  ( -31.72626587586518099, 0.000000000000000000, 9.005490826201270949 ) ) ;
#28088=DIRECTION ( 'NONE',  ( 0.9999697198139515519, 0.000000000000000000, 0.007781995580013368816 ) ) ;
#28089=LINE ( 'NONE', #49103, #2228 ) ;
#28090=EDGE_CURVE ( 'NONE', #37185, #41455, #33125, .T. ) ;
#28091=LINE ( 'NONE', #15313, #53595 ) ;
#28092=CARTESIAN_POINT ( 'NONE',  ( -11.58491270165622922, -1.651309408375658760, 1.328609220115083644 ) ) ;
#28093=ADVANCED_FACE ( 'NONE', ( #20032 ), #37101, .F. ) ;
#28094=DIRECTION ( 'NONE',  ( -0.9999697198139514409, -0.000000000000000000, -0.007781995580013368816 ) ) ;
#28095=CARTESIAN_POINT ( 'NONE',  ( -17.66816326098766865, 1.419719901456505395, 6.074237969063971398 ) ) ;
#28096=DIRECTION ( 'NONE',  ( 0.9999697198139515519, 0.000000000000000000, 0.007781995580013368816 ) ) ;
#28097=EDGE_CURVE ( 'NONE', #16052, #29890, #32300, .T. ) ;
#28098=CARTESIAN_POINT ( 'NONE',  ( -11.13209366544781354, 0.000000000000000000, 1.779118040146054014 ) ) ;
#28099=VERTEX_POINT ( 'NONE', #27759 ) ;
#28100=ORIENTED_EDGE ( 'NONE', *, *, #36857, .T. ) ;
#28101=FACE_OUTER_BOUND ( 'NONE', #3090, .T. ) ;
#28102=FACE_OUTER_BOUND ( 'NONE', #18194, .T. ) ;
#28103=EDGE_CURVE ( 'NONE', #2289, #34545, #40804, .T. ) ;
#28104=ORIENTED_EDGE ( 'NONE', *, *, #7256, .F. ) ;
#28105=DIRECTION ( 'NONE',  ( 0.9999697198139515519, 0.000000000000000000, 0.007781995580013368816 ) ) ;
#28106=ORIENTED_EDGE ( 'NONE', *, *, #49315, .F. ) ;
#28107=CARTESIAN_POINT ( 'NONE',  ( -14.46888367232926420, 0.000000000000000000, 12.59025272694991315 ) ) ;
#28108=ADVANCED_FACE ( 'NONE', ( #50136 ), #54399, .F. ) ;
#28109=AXIS2_PLACEMENT_3D ( 'NONE', #12721, #503, #39412 ) ;
#28110=ORIENTED_EDGE ( 'NONE', *, *, #31225, .T. ) ;
#28111=EDGE_LOOP ( 'NONE', ( #45930, #28795, #33001, #49481 ) ) ;
#28112=ORIENTED_EDGE ( 'NONE', *, *, #14486, .F. ) ;
#28113=DIRECTION ( 'NONE',  ( 0.7660212471507180654, -0.6427876096865404731, 0.005961354470445141482 ) ) ;
#28114=CARTESIAN_POINT ( 'NONE',  ( -19.27977376529886655, 0.000000000000000000, 7.994356096355883068 ) ) ;
#28115=CARTESIAN_POINT ( 'NONE',  ( -9.808144436391993182, 0.000000000000000000, 10.77986332834118777 ) ) ;
#28116=EDGE_LOOP ( 'NONE', ( #1239, #21698, #44447, #19935 ) ) ;
#28117=ORIENTED_EDGE ( 'NONE', *, *, #12449, .F. ) ;
#28118=DIRECTION ( 'NONE',  ( 0.5449076811759707706, 0.6444004775717708799, -0.5364919789714476250 ) ) ;
#28119=ORIENTED_EDGE ( 'NONE', *, *, #3320, .T. ) ;
#28120=DIRECTION ( 'NONE',  ( -0.005002170337468016433, -0.7660444431189770143, 0.6427681459581293666 ) ) ;
#28121=VERTEX_POINT ( 'NONE', #1877 ) ;
#28122=LINE ( 'NONE', #15085, #44846 ) ;
#28123=DIRECTION ( 'NONE',  ( 0.5449076811759707706, 0.6444004775717708799, -0.5364919789714476250 ) ) ;
#28124=ORIENTED_EDGE ( 'NONE', *, *, #1447, .T. ) ;
#28125=FACE_OUTER_BOUND ( 'NONE', #26448, .T. ) ;
#28126=EDGE_CURVE ( 'NONE', #29102, #31757, #37355, .T. ) ;
#28127=CARTESIAN_POINT ( 'NONE',  ( -16.99924723426068951, 0.000000000000000000, 13.49389102713827171 ) ) ;
#28128=EDGE_CURVE ( 'NONE', #6316, #30378, #28574, .T. ) ;
#28129=VERTEX_POINT ( 'NONE', #45898 ) ;
#28130=LINE ( 'NONE', #28712, #19481 ) ;
#28131=PLANE ( 'NONE',  #45701 ) ;
#28132=PLANE ( 'NONE',  #40077 ) ;
#28133=ORIENTED_EDGE ( 'NONE', *, *, #4015, .F. ) ;
#28134=ADVANCED_FACE ( 'NONE', ( #7014 ), #41625, .F. ) ;
#28135=CARTESIAN_POINT ( 'NONE',  ( -14.23769985819993522, 4.495856970884011261, 9.790194479452477339 ) ) ;
#28136=CARTESIAN_POINT ( 'NONE',  ( -21.93104030566808049, -3.917936722690659401, 11.63069420620037242 ) ) ;
#28137=FACE_OUTER_BOUND ( 'NONE', #5400, .T. ) ;
#28138=CARTESIAN_POINT ( 'NONE',  ( -16.81345671998191449, 0.000000000000000000, 3.412238694616132495 ) ) ;
#28139=EDGE_CURVE ( 'NONE', #50963, #53576, #36271, .T. ) ;
#28140=DIRECTION ( 'NONE',  ( 0.9999697198139515519, 0.000000000000000000, 0.007781995580013368816 ) ) ;
#28141=LINE ( 'NONE', #6301, #33370 ) ;
#28142=ADVANCED_FACE ( 'NONE', ( #31997 ), #46162, .F. ) ;
#28143=VECTOR ( 'NONE', #22774, 1000.000000000000227 ) ;
#28144=CARTESIAN_POINT ( 'NONE',  ( -10.33520963186314923, -0.1191753592594177180, 5.947975371940869671 ) ) ;
#28145=ORIENTED_EDGE ( 'NONE', *, *, #12437, .T. ) ;
#28146=DIRECTION ( 'NONE',  ( 0.007781995580012663651, -3.146120232559066537E-19, -0.9999697198139514409 ) ) ;
#28147=DIRECTION ( 'NONE',  ( 0.000000000000000000, -1.000000000000000000, 0.000000000000000000 ) ) ;
#28149=ORIENTED_EDGE ( 'NONE', *, *, #53244, .F. ) ;
#28150=LINE ( 'NONE', #15939, #42879 ) ;
#28151=CARTESIAN_POINT ( 'NONE',  ( -16.53317331066696383, 0.000000000000000000, 13.31285208727739899 ) ) ;
#28153=CARTESIAN_POINT ( 'NONE',  ( -20.54049170961573267, 0.000000000000000000, 4.660556269540326646 ) ) ;
#28154=FACE_OUTER_BOUND ( 'NONE', #25911, .T. ) ;
#28155=EDGE_CURVE ( 'NONE', #27227, #3531, #10434, .T. ) ;
#28157=EDGE_LOOP ( 'NONE', ( #41246, #15339, #32213, #23642 ) ) ;
#28158=ORIENTED_EDGE ( 'NONE', *, *, #3579, .T. ) ;
#28159=DIRECTION ( 'NONE',  ( 0.007781995580012662783, 0.000000000000000000, -0.9999697198139514409 ) ) ;
#28160=LINE ( 'NONE', #19079, #42948 ) ;
#28161=EDGE_CURVE ( 'NONE', #51848, #26799, #49615, .T. ) ;
#28162=ORIENTED_EDGE ( 'NONE', *, *, #30206, .T. ) ;
#28163=CARTESIAN_POINT ( 'NONE',  ( -12.27860572412447304, 0.000000000000000000, 3.986188037040617083 ) ) ;
#28164=VERTEX_POINT ( 'NONE', #28027 ) ;
#28165=LINE ( 'NONE', #54289, #41050 ) ;
#28166=ADVANCED_FACE ( 'NONE', ( #15250 ), #10966, .F. ) ;
#28167=ORIENTED_EDGE ( 'NONE', *, *, #10634, .F. ) ;
#28168=ORIENTED_EDGE ( 'NONE', *, *, #47067, .F. ) ;
#28169=DIRECTION ( 'NONE',  ( -0.6427681459581293666, -0.7660444431189770143, -0.005002170337467561935 ) ) ;
#28170=CARTESIAN_POINT ( 'NONE',  ( -20.96378235145114388, -1.165603555308157846, 4.987177259511585525 ) ) ;
#28171=DIRECTION ( 'NONE',  ( 0.6427681459581294776, -0.7660444431189769032, 0.005002170337467562802 ) ) ;
#28172=ORIENTED_EDGE ( 'NONE', *, *, #21055, .F. ) ;
#28173=VECTOR ( 'NONE', #22203, 1000.000000000000114 ) ;
#28174=DIRECTION ( 'NONE',  ( -0.005002170337468016433, -0.7660444431189770143, 0.6427681459581293666 ) ) ;
#28175=ORIENTED_EDGE ( 'NONE', *, *, #20109, .F. ) ;
#28176=VECTOR ( 'NONE', #37223, 1000.000000000000227 ) ;
#28177=ORIENTED_EDGE ( 'NONE', *, *, #28418, .F. ) ;
#28178=ORIENTED_EDGE ( 'NONE', *, *, #33534, .T. ) ;
#28179=DIRECTION ( 'NONE',  ( 0.007781995580012663651, 0.000000000000000000, -0.9999697198139515519 ) ) ;
#28180=VERTEX_POINT ( 'NONE', #19779 ) ;
#28181=FACE_OUTER_BOUND ( 'NONE', #25887, .T. ) ;
#28182=EDGE_LOOP ( 'NONE', ( #11213, #15536, #11422, #464 ) ) ;
#28183=DIRECTION ( 'NONE',  ( 0.6427681459581294776, -0.7660444431189769032, 0.005002170337467562802 ) ) ;
#28184=CARTESIAN_POINT ( 'NONE',  ( -10.27421835998572064, 0.000000000000000000, 10.96090226820206048 ) ) ;
#28185=VERTEX_POINT ( 'NONE', #42959 ) ;
#28187=EDGE_CURVE ( 'NONE', #32241, #46025, #26466, .T. ) ;
#28188=ORIENTED_EDGE ( 'NONE', *, *, #16262, .F. ) ;
#28189=LINE ( 'NONE', #29318, #26352 ) ;
#28190=DIRECTION ( 'NONE',  ( -0.005002170337468016433, -0.7660444431189770143, 0.6427681459581293666 ) ) ;
#28191=CARTESIAN_POINT ( 'NONE',  ( -14.10280672071693431, -0.1191753592594197858, 12.40843558753103792 ) ) ;
#28192=DIRECTION ( 'NONE',  ( -0.7660212471507179544, -0.6427876096865405842, -0.005961354470445141482 ) ) ;
#28193=CARTESIAN_POINT ( 'NONE',  ( -19.32961685222932147, 0.000000000000000000, 14.39908572644263351 ) ) ;
#28194=DIRECTION ( 'NONE',  ( 0.5364919789714477361, 0.6444004775717706579, 0.5449076811759711036 ) ) ;
#28195=DIRECTION ( 'NONE',  ( 0.7660212471507180654, -0.6427876096865404731, 0.005961354470445141482 ) ) ;
#28196=ORIENTED_EDGE ( 'NONE', *, *, #25360, .F. ) ;
#28197=EDGE_CURVE ( 'NONE', #52488, #19686, #31003, .T. ) ;
#28198=EDGE_CURVE ( 'NONE', #11534, #43483, #41890, .T. ) ;
#28199=EDGE_CURVE ( 'NONE', #39217, #4575, #48322, .T. ) ;
#28200=VECTOR ( 'NONE', #36337, 1000.000000000000000 ) ;
#28202=VECTOR ( 'NONE', #54791, 1000.000000000000000 ) ;
#28204=DIRECTION ( 'NONE',  ( 0.000000000000000000, -0.000000000000000000, -1.000000000000000000 ) ) ;
#28206=LINE ( 'NONE', #37570, #17032 ) ;
#28207=ADVANCED_FACE ( 'NONE', ( #39560 ), #4903, .F. ) ;
#28209=ORIENTED_EDGE ( 'NONE', *, *, #11105, .F. ) ;
#28210=LINE ( 'NONE', #49801, #46742 ) ;
#28211=DIRECTION ( 'NONE',  ( 0.007781995580012662783, 0.000000000000000000, -0.9999697198139514409 ) ) ;
#28212=EDGE_LOOP ( 'NONE', ( #5854, #33311, #32505, #3391 ) ) ;
#28213=DIRECTION ( 'NONE',  ( 0.007781995580012662783, 0.000000000000000000, -0.9999697198139514409 ) ) ;
#28214=PLANE ( 'NONE',  #13165 ) ;
#28215=ORIENTED_EDGE ( 'NONE', *, *, #44612, .T. ) ;
#28217=CARTESIAN_POINT ( 'NONE',  ( -25.20278734466900517, 0.000000000000000000, 6.670939612111840944 ) ) ;
#28218=VECTOR ( 'NONE', #5947, 1000.000000000000227 ) ;
#28219=EDGE_CURVE ( 'NONE', #29871, #42362, #21673, .T. ) ;
#28220=DIRECTION ( 'NONE',  ( 0.6427681459581294776, -0.7660444431189769032, 0.005002170337467562802 ) ) ;
#28221=PLANE ( 'NONE',  #51374 ) ;
#28222=VECTOR ( 'NONE', #36616, 1000.000000000000227 ) ;
#28223=ADVANCED_FACE ( 'NONE', ( #52337 ), #22228, .F. ) ;
#28224=CARTESIAN_POINT ( 'NONE',  ( -14.43341085292522052, 0.000000000000000000, 8.032071613151982703 ) ) ;
#28225=VERTEX_POINT ( 'NONE', #30181 ) ;
#28226=ORIENTED_EDGE ( 'NONE', *, *, #797, .T. ) ;
#28227=EDGE_CURVE ( 'NONE', #32666, #16969, #25633, .T. ) ;
#28228=CARTESIAN_POINT ( 'NONE',  ( -13.07066190154808361, 0.000000000000000000, 12.04713590736729678 ) ) ;
#28229=DIRECTION ( 'NONE',  ( -0.005002170337468016433, -0.7660444431189770143, 0.6427681459581293666 ) ) ;
#28230=DIRECTION ( 'NONE',  ( -0.9999697198139514409, -0.000000000000000000, -0.007781995580013368816 ) ) ;
#28231=CARTESIAN_POINT ( 'NONE',  ( -17.42278257705052980, 0.000000000000000000, 8.208813687390710712 ) ) ;
#28232=EDGE_CURVE ( 'NONE', #54774, #48671, #17388, .T. ) ;
#28233=DIRECTION ( 'NONE',  ( 0.005961354470445682716, -0.6427876096865404731, -0.7660212471507180654 ) ) ;
#28234=DIRECTION ( 'NONE',  ( 0.007781995580012662783, 0.000000000000000000, -0.9999697198139514409 ) ) ;
#28235=ORIENTED_EDGE ( 'NONE', *, *, #44526, .T. ) ;
#28236=CARTESIAN_POINT ( 'NONE',  ( -10.27421835998572064, 0.000000000000000000, 10.96090226820206048 ) ) ;
#28237=CARTESIAN_POINT ( 'NONE',  ( -12.16501668417466853, -0.1191753592594191197, 2.240414692291188725 ) ) ;
#28238=CARTESIAN_POINT ( 'NONE',  ( -13.53673582514181106, 0.000000000000000000, 12.22817484722816772 ) ) ;
#28239=EDGE_LOOP ( 'NONE', ( #26783, #6704, #7273, #53473, #36704, #31201, #10036, #43322 ) ) ;
#28240=DIRECTION ( 'NONE',  ( -0.6427681459581293666, -0.7660444431189770143, -0.005002170337467561935 ) ) ;
#28242=PLANE ( 'NONE',  #12100 ) ;
#28243=ORIENTED_EDGE ( 'NONE', *, *, #14738, .T. ) ;
#28244=VECTOR ( 'NONE', #36217, 999.9999999999998863 ) ;
#28245=VECTOR ( 'NONE', #46862, 999.9999999999998863 ) ;
#28246=CARTESIAN_POINT ( 'NONE',  ( -20.11779259742415249, -3.432230869623158487, 10.12924116631567273 ) ) ;
#28247=VERTEX_POINT ( 'NONE', #47209 ) ;
#28248=ORIENTED_EDGE ( 'NONE', *, *, #18901, .T. ) ;
#28249=ORIENTED_EDGE ( 'NONE', *, *, #18032, .F. ) ;
#28250=VERTEX_POINT ( 'NONE', #4365 ) ;
#28251=VECTOR ( 'NONE', #29043, 1000.000000000000227 ) ;
#28252=EDGE_LOOP ( 'NONE', ( #17131, #25741, #701, #8955 ) ) ;
#28253=CARTESIAN_POINT ( 'NONE',  ( -16.72078904067797822, 0.000000000000000000, 3.412959855923785923 ) ) ;
#28254=ORIENTED_EDGE ( 'NONE', *, *, #53615, .T. ) ;
#28255=ADVANCED_FACE ( 'NONE', ( #52594 ), #17687, .F. ) ;
#28256=ORIENTED_EDGE ( 'NONE', *, *, #49424, .F. ) ;
#28257=LINE ( 'NONE', #41602, #10493 ) ;
#28258=ORIENTED_EDGE ( 'NONE', *, *, #41091, .F. ) ;
#28259=ADVANCED_FACE ( 'NONE', ( #56037 ), #30757, .F. ) ;
#28260=EDGE_LOOP ( 'NONE', ( #49832, #7849, #55789, #8522 ) ) ;
#28261=VECTOR ( 'NONE', #5632, 1000.000000000000227 ) ;
#28262=ORIENTED_EDGE ( 'NONE', *, *, #6221, .T. ) ;
#28263=CARTESIAN_POINT ( 'NONE',  ( -13.08408713167409942, -0.1191753592594197858, 1.863930203747758085 ) ) ;
#28266=DIRECTION ( 'NONE',  ( 0.3620778797217453771, -0.000000000000000000, 0.9321478471874541372 ) ) ;
#28268=DIRECTION ( 'NONE',  ( 0.007781995580012663651, 0.000000000000000000, -0.9999697198139515519 ) ) ;
#28269=ORIENTED_EDGE ( 'NONE', *, *, #40352, .T. ) ;
#28270=EDGE_CURVE ( 'NONE', #19153, #46212, #33403, .T. ) ;
#28271=ADVANCED_FACE ( 'NONE', ( #11799 ), #17129, .F. ) ;
#28272=EDGE_CURVE ( 'NONE', #36112, #33164, #51750, .T. ) ;
#28273=ORIENTED_EDGE ( 'NONE', *, *, #33235, .F. ) ;
#28276=DIRECTION ( 'NONE',  ( 0.9321478471874541372, 0.000000000000000000, -0.3620778797217453771 ) ) ;
#28277=LINE ( 'NONE', #14955, #9473 ) ;
#28278=LINE ( 'NONE', #14132, #13965 ) ;
#28279=CARTESIAN_POINT ( 'NONE',  ( -20.26176469941677993, 0.000000000000000000, 14.76116360616437895 ) ) ;
#28280=ORIENTED_EDGE ( 'NONE', *, *, #13963, .F. ) ;
#28282=ORIENTED_EDGE ( 'NONE', *, *, #14136, .F. ) ;
#28283=VECTOR ( 'NONE', #1501, 1000.000000000000227 ) ;
#28284=VECTOR ( 'NONE', #56023, 1000.000000000000227 ) ;
#28285=CARTESIAN_POINT ( 'NONE',  ( -15.86710544311044302, 0.000000000000000000, 13.13336954653252953 ) ) ;
#28287=CARTESIAN_POINT ( 'NONE',  ( -10.67033082211201567, 0.000000000000000000, 2.152043655171826497 ) ) ;
#28288=DIRECTION ( 'NONE',  ( 0.007781995580012662783, 0.000000000000000000, -0.9999697198139514409 ) ) ;
#28289=PLANE ( 'NONE',  #5984 ) ;
#28290=VECTOR ( 'NONE', #30097, 999.9999999999998863 ) ;
#28291=ORIENTED_EDGE ( 'NONE', *, *, #11846, .F. ) ;
#28292=EDGE_CURVE ( 'NONE', #46770, #52665, #38986, .T. ) ;
#28294=PLANE ( 'NONE',  #19468 ) ;
#28295=CARTESIAN_POINT ( 'NONE',  ( -17.82130721938061413, -0.03739765774599677212, 3.742346127740344031 ) ) ;
#28296=EDGE_CURVE ( 'NONE', #14051, #17689, #8909, .T. ) ;
#28297=DIRECTION ( 'NONE',  ( -0.005002170337468016433, -0.7660444431189770143, 0.6427681459581293666 ) ) ;
#28298=VECTOR ( 'NONE', #15537, 1000.000000000000114 ) ;
#28299=CARTESIAN_POINT ( 'NONE',  ( -16.33317936670417225, 0.000000000000000000, 13.31440848639340224 ) ) ;
#28300=LINE ( 'NONE', #6199, #50851 ) ;
#28301=CARTESIAN_POINT ( 'NONE',  ( -12.33850799832341849, 0.000000000000000000, 11.68350162852954632 ) ) ;
#28302=ADVANCED_FACE ( 'NONE', ( #31599 ), #1181, .F. ) ;
#28303=AXIS2_PLACEMENT_3D ( 'NONE', #46632, #37554, #33321 ) ;
#28304=FACE_OUTER_BOUND ( 'NONE', #45041, .T. ) ;
#28305=CARTESIAN_POINT ( 'NONE',  ( -27.06630483948590893, -0.1191753592594197858, 7.295098399573937797 ) ) ;
#28306=ORIENTED_EDGE ( 'NONE', *, *, #40884, .T. ) ;
#28307=VECTOR ( 'NONE', #30765, 1000.000000000000114 ) ;
#28308=EDGE_LOOP ( 'NONE', ( #36037, #8276, #49644, #23566 ) ) ;
#28309=ORIENTED_EDGE ( 'NONE', *, *, #30967, .T. ) ;
#28310=ORIENTED_EDGE ( 'NONE', *, *, #9315, .T. ) ;
#28312=VECTOR ( 'NONE', #5063, 1000.000000000000227 ) ;
#28313=CARTESIAN_POINT ( 'NONE',  ( -17.74404816805336793, 0.000000000000000000, 3.574322630375089460 ) ) ;
#28314=DIRECTION ( 'NONE',  ( 0.6427681459581294776, -0.7660444431189769032, 0.005002170337467562802 ) ) ;
#28315=AXIS2_PLACEMENT_3D ( 'NONE', #40407, #31612, #48920 ) ;
#28316=VECTOR ( 'NONE', #28977, 999.9999999999998863 ) ;
#28317=ORIENTED_EDGE ( 'NONE', *, *, #41092, .F. ) ;
#28319=ORIENTED_EDGE ( 'NONE', *, *, #29314, .F. ) ;
#28320=ORIENTED_EDGE ( 'NONE', *, *, #25440, .T. ) ;
#28321=VECTOR ( 'NONE', #36861, 1000.000000000000227 ) ;
#28322=VECTOR ( 'NONE', #44485, 1000.000000000000227 ) ;
#28324=LINE ( 'NONE', #11586, #49097 ) ;
#28325=CARTESIAN_POINT ( 'NONE',  ( -13.17065887352947762, -0.1191753592594197858, 12.04635770780929427 ) ) ;
#28326=ORIENTED_EDGE ( 'NONE', *, *, #50659, .T. ) ;
#28327=DIRECTION ( 'NONE',  ( 0.005002170337468016433, -0.7660444431189770143, -0.6427681459581293666 ) ) ;
#28328=ADVANCED_FACE ( 'NONE', ( #53705 ), #27901, .F. ) ;
#28329=CARTESIAN_POINT ( 'NONE',  ( -23.33849165029409889, 0.000000000000000000, 5.946783852668351855 ) ) ;
#28330=DIRECTION ( 'NONE',  ( 0.005002170337468016433, -0.7660444431189770143, -0.6427681459581293666 ) ) ;
#28331=EDGE_CURVE ( 'NONE', #36770, #34091, #14541, .T. ) ;
#28332=ADVANCED_FACE ( 'NONE', ( #22517 ), #23356, .F. ) ;
#28333=LINE ( 'NONE', #36890, #45433 ) ;
#28334=CARTESIAN_POINT ( 'NONE',  ( -16.87007711150675959, -1.813211359398158473, 6.210631339198578793 ) ) ;
#28336=CARTESIAN_POINT ( 'NONE',  ( -17.74560456716937296, 0.000000000000000000, 3.774316574337878372 ) ) ;
#28337=CARTESIAN_POINT ( 'NONE',  ( -18.67775241435682432, 0.000000000000000000, 4.136394454059623804 ) ) ;
#28338=DIRECTION ( 'NONE',  ( -0.6427681459581293666, -0.7660444431189770143, -0.005002170337467561935 ) ) ;
#28339=EDGE_LOOP ( 'NONE', ( #29823, #23535, #52978, #13474 ) ) ;
#28340=CARTESIAN_POINT ( 'NONE',  ( -8.834775662789930095, 0.000000000000000000, 5.120984928305981398 ) ) ;
#28342=CARTESIAN_POINT ( 'NONE',  ( -13.08330893211609869, 0.000000000000000000, 1.763933231766363630 ) ) ;
#28343=LINE ( 'NONE', #41434, #44999 ) ;
#28344=PLANE ( 'NONE',  #6007 ) ;
#28345=AXIS2_PLACEMENT_3D ( 'NONE', #16024, #11181, #23682 ) ;
#28347=DIRECTION ( 'NONE',  ( -0.5449076811759708816, 0.6444004775717707689, 0.5364919789714475140 ) ) ;
#28348=DIRECTION ( 'NONE',  ( 0.007781995580012663651, -3.146120232559066537E-19, -0.9999697198139514409 ) ) ;
#28350=LINE ( 'NONE', #45393, #15120 ) ;
#28352=PLANE ( 'NONE',  #52939 ) ;
#28353=DIRECTION ( 'NONE',  ( 0.6427681459581294776, -0.7660444431189769032, 0.005002170337467562802 ) ) ;
#28354=LINE ( 'NONE', #45677, #36371 ) ;
#28355=LINE ( 'NONE', #28092, #24162 ) ;
#28356=VECTOR ( 'NONE', #39719, 999.9999999999998863 ) ;
#28357=VECTOR ( 'NONE', #6440, 999.9999999999998863 ) ;
#28358=PLANE ( 'NONE',  #41807 ) ;
#28359=CARTESIAN_POINT ( 'NONE',  ( -16.53182346927628643, 3.362543313726509719, 8.821349211107063937 ) ) ;
#28360=EDGE_CURVE ( 'NONE', #47771, #25044, #10000, .T. ) ;
#28361=CARTESIAN_POINT ( 'NONE',  ( -17.74560456716937296, 0.000000000000000000, 3.774316574337878372 ) ) ;
#28362=DIRECTION ( 'NONE',  ( 0.007781995580012662783, 0.000000000000000000, -0.9999697198139514409 ) ) ;
#28363=ORIENTED_EDGE ( 'NONE', *, *, #12117, .T. ) ;
#28364=VECTOR ( 'NONE', #14563, 999.9999999999998863 ) ;
#28365=DIRECTION ( 'NONE',  ( 0.007781995580012662783, 0.000000000000000000, -0.9999697198139514409 ) ) ;
#28366=VECTOR ( 'NONE', #23540, 1000.000000000000227 ) ;
#28367=ORIENTED_EDGE ( 'NONE', *, *, #33000, .T. ) ;
#28368=EDGE_CURVE ( 'NONE', #24940, #26440, #18821, .T. ) ;
#28369=DIRECTION ( 'NONE',  ( 0.007781995580012663651, 0.000000000000000000, -0.9999697198139515519 ) ) ;
#28370=CARTESIAN_POINT ( 'NONE',  ( -18.71304404252910558, -0.1191753592594156086, 7.729437476405517593 ) ) ;
#28371=EDGE_CURVE ( 'NONE', #26525, #55970, #44359, .T. ) ;
#28372=VERTEX_POINT ( 'NONE', #19069 ) ;
#28374=AXIS2_PLACEMENT_3D ( 'NONE', #21531, #47070, #29772 ) ;
#28375=ORIENTED_EDGE ( 'NONE', *, *, #46672, .T. ) ;
#28376=DIRECTION ( 'NONE',  ( 0.007781995580012663651, 0.000000000000000000, -0.9999697198139515519 ) ) ;
#28377=AXIS2_PLACEMENT_3D ( 'NONE', #36240, #10107, #27418 ) ;
#28378=VERTEX_POINT ( 'NONE', #5741 ) ;
#28379=ORIENTED_EDGE ( 'NONE', *, *, #38145, .F. ) ;
#28380=ORIENTED_EDGE ( 'NONE', *, *, #45925, .T. ) ;
#28381=CARTESIAN_POINT ( 'NONE',  ( -16.81190032086591302, 0.000000000000000000, 3.212244750653343583 ) ) ;
#28382=FACE_OUTER_BOUND ( 'NONE', #53409, .T. ) ;
#28383=DIRECTION ( 'NONE',  ( 0.007781995580012663651, 0.000000000000000000, -0.9999697198139515519 ) ) ;
#28384=VECTOR ( 'NONE', #48097, 999.9999999999998863 ) ;
#28385=VERTEX_POINT ( 'NONE', #52866 ) ;
#28386=ORIENTED_EDGE ( 'NONE', *, *, #9837, .F. ) ;
#28387=AXIS2_PLACEMENT_3D ( 'NONE', #3444, #20761, #55386 ) ;
#28388=LINE ( 'NONE', #55349, #8502 ) ;
#28389=CARTESIAN_POINT ( 'NONE',  ( -14.47385752816844473, -3.917936722690661178, 8.734071168426410736 ) ) ;
#28390=ORIENTED_EDGE ( 'NONE', *, *, #20979, .T. ) ;
#28391=VECTOR ( 'NONE', #602, 999.9999999999998863 ) ;
#28392=CARTESIAN_POINT ( 'NONE',  ( -15.03495456790438389, -0.1191753592594197858, 12.77051346725278158 ) ) ;
#28393=ADVANCED_FACE ( 'NONE', ( #18225 ), #40093, .F. ) ;
#28394=ORIENTED_EDGE ( 'NONE', *, *, #16582, .T. ) ;
#28395=DIRECTION ( 'NONE',  ( 0.5449076811759707706, 0.6444004775717708799, -0.5364919789714476250 ) ) ;
#28396=DIRECTION ( 'NONE',  ( 0.9999697198139515519, 0.000000000000000000, 0.007781995580013368816 ) ) ;
#28397=AXIS2_PLACEMENT_3D ( 'NONE', #39351, #4443, #56119 ) ;
#28398=VECTOR ( 'NONE', #7206, 999.9999999999998863 ) ;
#28399=ADVANCED_FACE ( 'NONE', ( #39824 ), #45207, .F. ) ;
#28400=EDGE_LOOP ( 'NONE', ( #33721, #33830, #25586, #48291 ) ) ;
#28401=FACE_OUTER_BOUND ( 'NONE', #48321, .T. ) ;
#28402=EDGE_CURVE ( 'NONE', #20845, #37899, #48633, .T. ) ;
#28403=EDGE_CURVE ( 'NONE', #24227, #12251, #2011, .T. ) ;
#28404=AXIS2_PLACEMENT_3D ( 'NONE', #5997, #18782, #27269 ) ;
#28405=DIRECTION ( 'NONE',  ( 0.005002170337468016433, -0.7660444431189770143, -0.6427681459581293666 ) ) ;
#28407=VERTEX_POINT ( 'NONE', #53180 ) ;
#28408=DIRECTION ( 'NONE',  ( 0.9999697198139515519, 0.000000000000000000, 0.007781995580013368816 ) ) ;
#28409=PLANE ( 'NONE',  #21231 ) ;
#28410=DIRECTION ( 'NONE',  ( -0.2426528472758542054, 0.7422098413412800966, -0.6246952433987894571 ) ) ;
#28411=ORIENTED_EDGE ( 'NONE', *, *, #14823, .F. ) ;
#28412=CARTESIAN_POINT ( 'NONE',  ( -20.54204810873173415, 0.000000000000000000, 4.860550213503115558 ) ) ;
#28413=DIRECTION ( 'NONE',  ( 0.5449076811759707706, 0.6444004775717708799, -0.5364919789714476250 ) ) ;
#28414=DIRECTION ( 'NONE',  ( 0.007781995580012663651, 0.000000000000000000, -0.9999697198139515519 ) ) ;
#28415=CARTESIAN_POINT ( 'NONE',  ( -17.97681294474074676, -3.108426967578160394, 8.766194593337463203 ) ) ;
#28416=CARTESIAN_POINT ( 'NONE',  ( -8.024318355659660895, -1.000000000000000000, 6.335291332000425157 ) ) ;
#28417=CARTESIAN_POINT ( 'NONE',  ( -14.66887761629205222, 0.000000000000000000, 12.58869632783390990 ) ) ;
#28418=EDGE_CURVE ( 'NONE', #34831, #56081, #49167, .T. ) ;
#28419=CARTESIAN_POINT ( 'NONE',  ( -22.40634380310664397, 0.000000000000000000, 5.584705972946605534 ) ) ;
#28420=VECTOR ( 'NONE', #17100, 1000.000000000000000 ) ;
#28421=ORIENTED_EDGE ( 'NONE', *, *, #53944, .F. ) ;
#28422=FACE_OUTER_BOUND ( 'NONE', #4458, .T. ) ;
#28425=DIRECTION ( 'NONE',  ( -0.5449076811759708816, 0.6444004775717707689, 0.5364919789714475140 ) ) ;
#28426=DIRECTION ( 'NONE',  ( -0.9999697198139514409, -0.000000000000000000, -0.007781995580013368816 ) ) ;
#28427=VECTOR ( 'NONE', #5580, 999.9999999999998863 ) ;
#28428=CARTESIAN_POINT ( 'NONE',  ( -18.80651470794193258, 0.000000000000000000, 6.890042898350599465 ) ) ;
#28430=DIRECTION ( 'NONE',  ( 0.007781995580012663651, 0.000000000000000000, -0.9999697198139515519 ) ) ;
#28431=DIRECTION ( 'NONE',  ( 0.5364919789714477361, 0.6444004775717706579, 0.5449076811759711036 ) ) ;
#28432=ORIENTED_EDGE ( 'NONE', *, *, #37169, .T. ) ;
#28433=VERTEX_POINT ( 'NONE', #26763 ) ;
#28434=PLANE ( 'NONE',  #49519 ) ;
#28435=VECTOR ( 'NONE', #53532, 1000.000000000000227 ) ;
#28436=VECTOR ( 'NONE', #38707, 999.9999999999998863 ) ;
#28437=DIRECTION ( 'NONE',  ( 0.000000000000000000, -0.000000000000000000, -1.000000000000000000 ) ) ;
#28438=EDGE_LOOP ( 'NONE', ( #22534, #5258, #38747, #52421 ) ) ;
#28439=DIRECTION ( 'NONE',  ( -0.005002170337468016433, -0.7660444431189770143, 0.6427681459581293666 ) ) ;
#28440=ADVANCED_FACE ( 'NONE', ( #5203 ), #27606, .F. ) ;
#28441=VERTEX_POINT ( 'NONE', #35556 ) ;
#28442=FACE_OUTER_BOUND ( 'NONE', #22754, .T. ) ;
#28443=VECTOR ( 'NONE', #44091, 1000.000000000000114 ) ;
#28444=ORIENTED_EDGE ( 'NONE', *, *, #47737, .F. ) ;
#28445=AXIS2_PLACEMENT_3D ( 'NONE', #31230, #18755, #14223 ) ;
#28447=DIRECTION ( 'NONE',  ( -0.5364919789714478471, 0.6444004775717705469, -0.5449076811759709926 ) ) ;
#28448=LINE ( 'NONE', #28170, #40476 ) ;
#28449=DIRECTION ( 'NONE',  ( 0.000000000000000000, -1.000000000000000000, 0.000000000000000000 ) ) ;
#28450=ADVANCED_FACE ( 'NONE', ( #13976 ), #9744, .F. ) ;
#28451=ORIENTED_EDGE ( 'NONE', *, *, #5860, .F. ) ;
#28452=CARTESIAN_POINT ( 'NONE',  ( -29.86197018149027116, 0.000000000000000000, 8.281335066757780083 ) ) ;
#28453=VERTEX_POINT ( 'NONE', #50839 ) ;
#28454=EDGE_CURVE ( 'NONE', #42368, #16476, #55123, .T. ) ;
#28455=EDGE_CURVE ( 'NONE', #5924, #20285, #20171, .T. ) ;
#28456=ORIENTED_EDGE ( 'NONE', *, *, #5091, .F. ) ;
#28457=EDGE_LOOP ( 'NONE', ( #55934, #37321, #20709, #25985 ) ) ;
#28458=LINE ( 'NONE', #31889, #13225 ) ;
#28459=VECTOR ( 'NONE', #52308, 1000.000000000000227 ) ;
#28460=ORIENTED_EDGE ( 'NONE', *, *, #15883, .F. ) ;
#28461=DIRECTION ( 'NONE',  ( -0.005002170337468016433, -0.7660444431189770143, 0.6427681459581293666 ) ) ;
#28462=ADVANCED_FACE ( 'NONE', ( #11935 ), #42040, .F. ) ;
#28463=VERTEX_POINT ( 'NONE', #50583 ) ;
#28464=AXIS2_PLACEMENT_3D ( 'NONE', #34496, #21729, #39322 ) ;
#28465=DIRECTION ( 'NONE',  ( 0.007781995580012662783, 0.000000000000000000, -0.9999697198139514409 ) ) ;
#28466=DIRECTION ( 'NONE',  ( 0.007781995580012663651, 0.000000000000000000, -0.9999697198139515519 ) ) ;
#28467=ORIENTED_EDGE ( 'NONE', *, *, #25998, .F. ) ;
#28468=EDGE_CURVE ( 'NONE', #16069, #24033, #37813, .T. ) ;
#28469=CARTESIAN_POINT ( 'NONE',  ( -12.70458494993575194, -0.1191753592594197858, 11.86531876794841978 ) ) ;
#28470=VECTOR ( 'NONE', #20383, 999.9999999999998863 ) ;
#28471=ORIENTED_EDGE ( 'NONE', *, *, #32024, .T. ) ;
#28472=EDGE_CURVE ( 'NONE', #11761, #51416, #19646, .T. ) ;
#28473=CARTESIAN_POINT ( 'NONE',  ( -2.730566055856384011, -5.007877867457373178, -2.157728989155597077 ) ) ;
#28474=DIRECTION ( 'NONE',  ( -0.9999697198139514409, -0.000000000000000000, -0.007781995580013368816 ) ) ;
#28475=DIRECTION ( 'NONE',  ( 0.007781995580012663651, -3.146120232559066537E-19, -0.9999697198139514409 ) ) ;
#28476=DIRECTION ( 'NONE',  ( 0.005002170337468016433, -0.7660444431189770143, -0.6427681459581293666 ) ) ;
#28477=PLANE ( 'NONE',  #25107 ) ;
#28478=VECTOR ( 'NONE', #25589, 1000.000000000000227 ) ;
#28479=PLANE ( 'NONE',  #53655 ) ;
#28480=FACE_OUTER_BOUND ( 'NONE', #34551, .T. ) ;
#28481=ORIENTED_EDGE ( 'NONE', *, *, #29047, .T. ) ;
#28483=EDGE_CURVE ( 'NONE', #44124, #36489, #33531, .T. ) ;
#28484=ORIENTED_EDGE ( 'NONE', *, *, #5408, .F. ) ;
#28485=LINE ( 'NONE', #6631, #15546 ) ;
#28486=DIRECTION ( 'NONE',  ( -0.5449076811759708816, 0.6444004775717707689, 0.5364919789714475140 ) ) ;
#28487=LINE ( 'NONE', #11162, #28527 ) ;
#28488=DIRECTION ( 'NONE',  ( 0.007781995580012662783, 0.000000000000000000, -0.9999697198139514409 ) ) ;
#28489=EDGE_CURVE ( 'NONE', #15384, #51591, #29263, .T. ) ;
#28490=VECTOR ( 'NONE', #15510, 999.9999999999998863 ) ;
#28491=VECTOR ( 'NONE', #26853, 1000.000000000000114 ) ;
#28492=CARTESIAN_POINT ( 'NONE',  ( -15.88130887279446490, 0.000000000000000000, 3.050160814894388839 ) ) ;
#28493=EDGE_LOOP ( 'NONE', ( #54944, #34132, #16230, #30742 ) ) ;
#28494=DIRECTION ( 'NONE',  ( 0.007781995580012663651, -3.146120232559066537E-19, -0.9999697198139514409 ) ) ;
#28495=CARTESIAN_POINT ( 'NONE',  ( -10.00813838035478298, 0.000000000000000000, 10.77830692922518452 ) ) ;
#28496=ORIENTED_EDGE ( 'NONE', *, *, #22324, .T. ) ;
#28497=LINE ( 'NONE', #45815, #21146 ) ;
#28498=DIRECTION ( 'NONE',  ( 0.007781995580012663651, -3.146120232559066537E-19, -0.9999697198139514409 ) ) ;
#28499=ORIENTED_EDGE ( 'NONE', *, *, #54259, .F. ) ;
#28500=PLANE ( 'NONE',  #17104 ) ;
#28502=CARTESIAN_POINT ( 'NONE',  ( -17.37561052637969183, 1.095915999411505526, 3.396243480022655081 ) ) ;
#28503=CARTESIAN_POINT ( 'NONE',  ( -26.13415699229845757, -0.1191753592594197858, 6.933020519852192365 ) ) ;
#28505=AXIS2_PLACEMENT_3D ( 'NONE', #37082, #32801, #20301 ) ;
#28506=ORIENTED_EDGE ( 'NONE', *, *, #28483, .T. ) ;
#28507=ORIENTED_EDGE ( 'NONE', *, *, #27877, .T. ) ;
#28508=AXIS2_PLACEMENT_3D ( 'NONE', #37200, #54504, #15603 ) ;
#28509=DIRECTION ( 'NONE',  ( 0.6427681459581294776, -0.7660444431189769032, 0.005002170337467562802 ) ) ;
#28510=PLANE ( 'NONE',  #45808 ) ;
#28511=CARTESIAN_POINT ( 'NONE',  ( -9.496532450088523092, 0.000000000000000000, 4.746502914164204334 ) ) ;
#28512=VECTOR ( 'NONE', #55369, 1000.000000000000227 ) ;
#28513=DIRECTION ( 'NONE',  ( 0.007781995580012663651, 0.000000000000000000, -0.9999697198139515519 ) ) ;
#28515=CARTESIAN_POINT ( 'NONE',  ( -17.83139810946674686, -0.1191753592594197858, 13.85674710641801788 ) ) ;
#28516=ADVANCED_FACE ( 'NONE', ( #7697 ), #46292, .F. ) ;
#28518=FACE_OUTER_BOUND ( 'NONE', #52094, .T. ) ;
#28519=LINE ( 'NONE', #45845, #24139 ) ;
#28520=DIRECTION ( 'NONE',  ( 0.007781995580012663651, 0.000000000000000000, -0.9999697198139515519 ) ) ;
#28521=VECTOR ( 'NONE', #21464, 999.9999999999998863 ) ;
#28522=ORIENTED_EDGE ( 'NONE', *, *, #44246, .F. ) ;
#28523=VECTOR ( 'NONE', #19234, 999.9999999999998863 ) ;
#28524=FACE_OUTER_BOUND ( 'NONE', #21924, .T. ) ;
#28525=CARTESIAN_POINT ( 'NONE',  ( -15.13495153988577968, 0.000000000000000000, 12.76973526769478084 ) ) ;
#28526=DIRECTION ( 'NONE',  ( 0.5449076811759707706, 0.6444004775717708799, -0.5364919789714476250 ) ) ;
#28527=VECTOR ( 'NONE', #50637, 1000.000000000000227 ) ;
#28528=ORIENTED_EDGE ( 'NONE', *, *, #3925, .T. ) ;
#28529=PLANE ( 'NONE',  #53102 ) ;
#28530=ORIENTED_EDGE ( 'NONE', *, *, #11804, .T. ) ;
#28531=ADVANCED_FACE ( 'NONE', ( #54275 ), #55379, .F. ) ;
#28532=VECTOR ( 'NONE', #50081, 1000.000000000000227 ) ;
#28533=ORIENTED_EDGE ( 'NONE', *, *, #21854, .T. ) ;
#28534=ORIENTED_EDGE ( 'NONE', *, *, #20247, .F. ) ;
#28535=AXIS2_PLACEMENT_3D ( 'NONE', #17984, #52880, #39836 ) ;
#28536=ORIENTED_EDGE ( 'NONE', *, *, #39003, .F. ) ;
#28537=ORIENTED_EDGE ( 'NONE', *, *, #18661, .F. ) ;
#28538=CARTESIAN_POINT ( 'NONE',  ( -23.33849165029409889, 0.000000000000000000, 5.946783852668351855 ) ) ;
#28539=ORIENTED_EDGE ( 'NONE', *, *, #15191, .F. ) ;
#28540=ORIENTED_EDGE ( 'NONE', *, *, #43243, .F. ) ;
#28541=CARTESIAN_POINT ( 'NONE',  ( -14.96433427924230841, -0.1191753592594198830, 3.695958034714191154 ) ) ;
#28542=EDGE_CURVE ( 'NONE', #23008, #38521, #7398, .T. ) ;
#28543=ORIENTED_EDGE ( 'NONE', *, *, #44378, .F. ) ;
#28544=ORIENTED_EDGE ( 'NONE', *, *, #22469, .F. ) ;
#28545=EDGE_CURVE ( 'NONE', #39497, #349, #28150, .T. ) ;
#28546=EDGE_LOOP ( 'NONE', ( #45601, #27625, #29896, #3974 ) ) ;
#28547=AXIS2_PLACEMENT_3D ( 'NONE', #48560, #16861, #31536 ) ;
#28548=LINE ( 'NONE', #45877, #42899 ) ;
#28549=VECTOR ( 'NONE', #14651, 999.9999999999998863 ) ;
#28550=FACE_OUTER_BOUND ( 'NONE', #49643, .T. ) ;
#28551=CARTESIAN_POINT ( 'NONE',  ( -18.67619601524082285, 0.000000000000000000, 3.936400510096834893 ) ) ;
#28552=DIRECTION ( 'NONE',  ( -0.005002170337468016433, -0.7660444431189770143, 0.6427681459581293666 ) ) ;
#28553=CARTESIAN_POINT ( 'NONE',  ( -11.77243710274829525, -0.1191753592594197858, 11.50324088822667612 ) ) ;
#28554=VECTOR ( 'NONE', #40161, 1000.000000000000227 ) ;
#28555=EDGE_LOOP ( 'NONE', ( #22621, #17078, #47132, #5754 ) ) ;
#28556=ADVANCED_FACE ( 'NONE', ( #33276 ), #45459, .F. ) ;
#28557=ORIENTED_EDGE ( 'NONE', *, *, #32555, .T. ) ;
#28558=CARTESIAN_POINT ( 'NONE',  ( -12.70458494993575194, -0.1191753592594197858, 11.86531876794841978 ) ) ;
#28559=LINE ( 'NONE', #20616, #52064 ) ;
#28562=ADVANCED_FACE ( 'NONE', ( #32972 ), #41216, .F. ) ;
#28563=VECTOR ( 'NONE', #28465, 1000.000000000000227 ) ;
#28565=FACE_OUTER_BOUND ( 'NONE', #27374, .T. ) ;
#28566=VECTOR ( 'NONE', #3995, 1000.000000000000114 ) ;
#28567=CARTESIAN_POINT ( 'NONE',  ( 3.004435629306332345, -1.000000000000000000, -3.312607213261892003 ) ) ;
#28568=AXIS2_PLACEMENT_3D ( 'NONE', #21509, #12970, #47616 ) ;
#28569=CARTESIAN_POINT ( 'NONE',  ( -12.18513505871164604, -0.1191753592594185784, 4.825582615095539651 ) ) ;
#28570=ORIENTED_EDGE ( 'NONE', *, *, #35584, .F. ) ;
#28571=LINE ( 'NONE', #7011, #11127 ) ;
#28572=ORIENTED_EDGE ( 'NONE', *, *, #15048, .T. ) ;
#28573=VECTOR ( 'NONE', #30398, 1000.000000000000000 ) ;
#28574=LINE ( 'NONE', #6185, #10220 ) ;
#28575=CARTESIAN_POINT ( 'NONE',  ( -12.60458797795435615, 0.000000000000000000, 11.86609696750642229 ) ) ;
#28576=DIRECTION ( 'NONE',  ( -0.8531650599175527594, 0.4028455766673922356, 0.3313982828793700652 ) ) ;
#28577=LINE ( 'NONE', #45902, #54029 ) ;
#28578=LINE ( 'NONE', #2996, #1463 ) ;
#28579=VECTOR ( 'NONE', #30709, 999.9999999999998863 ) ;
#28580=AXIS2_PLACEMENT_3D ( 'NONE', #16327, #12071, #46727 ) ;
#28581=ORIENTED_EDGE ( 'NONE', *, *, #16630, .F. ) ;
#28582=LINE ( 'NONE', #23496, #13058 ) ;
#28583=FACE_OUTER_BOUND ( 'NONE', #50924, .T. ) ;
#28584=CARTESIAN_POINT ( 'NONE',  ( -27.99923088623136636, 0.000000000000000000, 7.757173251277078130 ) ) ;
#28585=EDGE_CURVE ( 'NONE', #40214, #20884, #32685, .T. ) ;
#28586=DIRECTION ( 'NONE',  ( 0.5364919789714477361, 0.6444004775717706579, 0.5449076811759711036 ) ) ;
#28587=CARTESIAN_POINT ( 'NONE',  ( -10.00813838035478298, 0.000000000000000000, 10.77830692922518452 ) ) ;
#28588=EDGE_CURVE ( 'NONE', #13341, #6886, #28995, .T. ) ;
#28589=DIRECTION ( 'NONE',  ( -0.9999697198139514409, -0.000000000000000000, -0.007781995580013368816 ) ) ;
#28590=LINE ( 'NONE', #38505, #52837 ) ;
#28591=VECTOR ( 'NONE', #7276, 999.9999999999998863 ) ;
#28592=CARTESIAN_POINT ( 'NONE',  ( -28.93137873341882127, 0.000000000000000000, 8.119251130998824451 ) ) ;
#28593=AXIS2_PLACEMENT_3D ( 'NONE', #3708, #25310, #17077 ) ;
#28594=EDGE_CURVE ( 'NONE', #20073, #52488, #46038, .T. ) ;
#28595=DIRECTION ( 'NONE',  ( -0.3620778797217456546, 0.000000000000000000, -0.9321478471874540261 ) ) ;
#28596=ORIENTED_EDGE ( 'NONE', *, *, #53760, .F. ) ;
#28597=VECTOR ( 'NONE', #1033, 999.9999999999998863 ) ;
#28598=ADVANCED_FACE ( 'NONE', ( #2841 ), #39182, .F. ) ;
#28599=EDGE_CURVE ( 'NONE', #41034, #15196, #39487, .T. ) ;
#28600=EDGE_CURVE ( 'NONE', #12202, #46860, #12791, .T. ) ;
#28601=ORIENTED_EDGE ( 'NONE', *, *, #11451, .F. ) ;
#28602=VECTOR ( 'NONE', #21078, 1000.000000000000227 ) ;
#28603=ORIENTED_EDGE ( 'NONE', *, *, #10419, .T. ) ;
#28604=EDGE_LOOP ( 'NONE', ( #36800, #43090, #7349, #45046 ) ) ;
#28605=AXIS2_PLACEMENT_3D ( 'NONE', #320, #12834, #47184 ) ;
#28606=VECTOR ( 'NONE', #3608, 999.9999999999998863 ) ;
#28607=ORIENTED_EDGE ( 'NONE', *, *, #41769, .T. ) ;
#28608=ORIENTED_EDGE ( 'NONE', *, *, #35224, .T. ) ;
#28609=CARTESIAN_POINT ( 'NONE',  ( -16.87359065091598254, 2.714935509636508204, 3.149586712851912829 ) ) ;
#28610=CARTESIAN_POINT ( 'NONE',  ( -14.41616653189352348, 0.000000000000000000, 5.816213393605395687 ) ) ;
#28611=CARTESIAN_POINT ( 'NONE',  ( -17.74482636761137044, -0.1191753592594197858, 3.674319602356483916 ) ) ;
#28612=VECTOR ( 'NONE', #45141, 1000.000000000000000 ) ;
#28613=VECTOR ( 'NONE', #8733, 999.9999999999998863 ) ;
#28614=ORIENTED_EDGE ( 'NONE', *, *, #17855, .F. ) ;
#28615=DIRECTION ( 'NONE',  ( -0.5449076811759708816, 0.6444004775717707689, 0.5364919789714475140 ) ) ;
#28616=EDGE_CURVE ( 'NONE', #46025, #37342, #34641, .T. ) ;
#28617=ORIENTED_EDGE ( 'NONE', *, *, #27194, .F. ) ;
#28618=ORIENTED_EDGE ( 'NONE', *, *, #8160, .F. ) ;
#28619=VECTOR ( 'NONE', #15734, 1000.000000000000227 ) ;
#28620=ADVANCED_FACE ( 'NONE', ( #22154 ), #21611, .F. ) ;
#28621=AXIS2_PLACEMENT_3D ( 'NONE', #2641, #12000, #38129 ) ;
#28623=ADVANCED_FACE ( 'NONE', ( #26146 ), #43200, .F. ) ;
#28624=LINE ( 'NONE', #33171, #24598 ) ;
#28625=CARTESIAN_POINT ( 'NONE',  ( -17.23272844799286929, 0.000000000000000000, 9.487614955574981579 ) ) ;
#28626=ORIENTED_EDGE ( 'NONE', *, *, #54748, .F. ) ;
#28628=EDGE_LOOP ( 'NONE', ( #52831, #8370, #7801, #46656 ) ) ;
#28629=ADVANCED_FACE ( 'NONE', ( #17912 ), #43454, .F. ) ;
#28630=DIRECTION ( 'NONE',  ( 0.007781995580012662783, 0.000000000000000000, -0.9999697198139514409 ) ) ;
#28631=DIRECTION ( 'NONE',  ( 0.5364919789714477361, 0.6444004775717706579, 0.5449076811759711036 ) ) ;
#28632=ADVANCED_FACE ( 'NONE', ( #4298 ), #17066, .F. ) ;
#28633=VECTOR ( 'NONE', #916, 1000.000000000000227 ) ;
#28634=LINE ( 'NONE', #11010, #6463 ) ;
#28635=CARTESIAN_POINT ( 'NONE',  ( -14.94916102560700821, 0.000000000000000000, 2.688082935172642962 ) ) ;
#28637=LINE ( 'NONE', #45129, #42889 ) ;
#28638=LINE ( 'NONE', #28337, #49365 ) ;
#28639=VECTOR ( 'NONE', #8257, 1000.000000000000227 ) ;
#28640=LINE ( 'NONE', #38557, #18502 ) ;
#28641=CARTESIAN_POINT ( 'NONE',  ( -14.93495759592298988, 0.000000000000000000, 12.77129166681078409 ) ) ;
#28642=ORIENTED_EDGE ( 'NONE', *, *, #28126, .T. ) ;
#28643=DIRECTION ( 'NONE',  ( 0.007781995580012663651, -3.146120232559066537E-19, -0.9999697198139514409 ) ) ;
#28644=ORIENTED_EDGE ( 'NONE', *, *, #39697, .T. ) ;
#28645=VECTOR ( 'NONE', #26014, 1000.000000000000114 ) ;
#28647=LINE ( 'NONE', #49917, #31378 ) ;
#28648=PLANE ( 'NONE',  #17802 ) ;
#28649=AXIS2_PLACEMENT_3D ( 'NONE', #36073, #576, #13368 ) ;
#28650=LINE ( 'NONE', #7080, #2370 ) ;
#28651=DIRECTION ( 'NONE',  ( 0.7660212471507180654, -0.6427876096865404731, 0.005961354470445141482 ) ) ;
#28652=AXIS2_PLACEMENT_3D ( 'NONE', #36320, #45136, #6497 ) ;
#28653=DIRECTION ( 'NONE',  ( 0.007781995580012663651, 0.000000000000000000, -0.9999697198139515519 ) ) ;
#28654=AXIS2_PLACEMENT_3D ( 'NONE', #25995, #21451, #20861 ) ;
#28655=ORIENTED_EDGE ( 'NONE', *, *, #30891, .T. ) ;
#28656=DIRECTION ( 'NONE',  ( 0.9999697198139515519, 0.000000000000000000, 0.007781995580013368816 ) ) ;
#28657=LINE ( 'NONE', #15859, #33895 ) ;
#28658=LINE ( 'NONE', #27533, #35819 ) ;
#28659=VECTOR ( 'NONE', #2451, 1000.000000000000227 ) ;
#28660=LINE ( 'NONE', #45978, #33648 ) ;
#28661=CARTESIAN_POINT ( 'NONE',  ( -20.54204810873173415, 0.000000000000000000, 4.860550213503115558 ) ) ;
#28662=VECTOR ( 'NONE', #16337, 999.9999999999998863 ) ;
#28663=VECTOR ( 'NONE', #11840, 999.9999999999998863 ) ;
#28664=DIRECTION ( 'NONE',  ( 0.007781995580012663651, 0.000000000000000000, -0.9999697198139515519 ) ) ;
#28665=PLANE ( 'NONE',  #1247 ) ;
#28666=DIRECTION ( 'NONE',  ( 0.9999697198139515519, 0.000000000000000000, 0.007781995580013368816 ) ) ;
#28667=DIRECTION ( 'NONE',  ( -0.7660212471507179544, -0.6427876096865405842, -0.005961354470445141482 ) ) ;
#28668=ORIENTED_EDGE ( 'NONE', *, *, #1443, .F. ) ;
#28669=VECTOR ( 'NONE', #6823, 999.9999999999998863 ) ;
#28670=VECTOR ( 'NONE', #21800, 999.9999999999998863 ) ;
#28672=EDGE_LOOP ( 'NONE', ( #28990, #27091, #51471, #25880 ) ) ;
#28673=FACE_OUTER_BOUND ( 'NONE', #45304, .T. ) ;
#28674=DIRECTION ( 'NONE',  ( 0.5449076811759707706, 0.6444004775717708799, -0.5364919789714476250 ) ) ;
#28675=ADVANCED_FACE ( 'NONE', ( #46887 ), #21015, .F. ) ;
#28676=ADVANCED_FACE ( 'NONE', ( #30694 ), #38649, .F. ) ;
#28677=ORIENTED_EDGE ( 'NONE', *, *, #1630, .T. ) ;
#28678=EDGE_LOOP ( 'NONE', ( #24482, #23366, #22802, #45313 ) ) ;
#28679=PLANE ( 'NONE',  #22937 ) ;
#28681=VECTOR ( 'NONE', #29433, 999.9999999999998863 ) ;
#28682=VERTEX_POINT ( 'NONE', #51962 ) ;
#28683=EDGE_LOOP ( 'NONE', ( #21824, #11767, #45182, #32692 ) ) ;
#28684=ORIENTED_EDGE ( 'NONE', *, *, #46592, .T. ) ;
#28685=CARTESIAN_POINT ( 'NONE',  ( -17.21991457958245775, 0.000000000000000000, 7.841060383248950494 ) ) ;
#28686=LINE ( 'NONE', #37463, #54125 ) ;
#28688=LINE ( 'NONE', #6824, #11290 ) ;
#28689=AXIS2_PLACEMENT_3D ( 'NONE', #28946, #7345, #24659 ) ;
#28690=ORIENTED_EDGE ( 'NONE', *, *, #38855, .F. ) ;
#28691=VERTEX_POINT ( 'NONE', #17613 ) ;
#28692=EDGE_CURVE ( 'NONE', #45599, #53284, #42884, .T. ) ;
#28693=VECTOR ( 'NONE', #34571, 1000.000000000000000 ) ;
#28694=DIRECTION ( 'NONE',  ( 0.005961354470445682716, -0.6427876096865404731, -0.7660212471507180654 ) ) ;
#28695=PLANE ( 'NONE',  #37238 ) ;
#28696=ORIENTED_EDGE ( 'NONE', *, *, #25928, .F. ) ;
#28697=FACE_OUTER_BOUND ( 'NONE', #8430, .T. ) ;
#28698=ORIENTED_EDGE ( 'NONE', *, *, #54787, .T. ) ;
#28699=CARTESIAN_POINT ( 'NONE',  ( -14.01545677930355183, 0.000000000000000000, 2.126011111488108174 ) ) ;
#28700=CARTESIAN_POINT ( 'NONE',  ( -15.78478530592635920, -3.270328918600659218, 8.180445300800458952 ) ) ;
#28701=VECTOR ( 'NONE', #36252, 999.9999999999998863 ) ;
#28702=EDGE_LOOP ( 'NONE', ( #18405, #52901, #46051, #52339 ) ) ;
#28703=ADVANCED_FACE ( 'NONE', ( #29576 ), #3991, .F. ) ;
#28704=VECTOR ( 'NONE', #17439, 999.9999999999998863 ) ;
#28705=DIRECTION ( 'NONE',  ( 0.005002170337468016433, -0.7660444431189770143, -0.6427681459581293666 ) ) ;
#28706=EDGE_CURVE ( 'NONE', #18997, #32684, #26399, .T. ) ;
#28707=AXIS2_PLACEMENT_3D ( 'NONE', #21573, #26645, #30654 ) ;
#28708=FACE_OUTER_BOUND ( 'NONE', #28555, .T. ) ;
#28709=VECTOR ( 'NONE', #55455, 1000.000000000000000 ) ;
#28710=ORIENTED_EDGE ( 'NONE', *, *, #2937, .T. ) ;
#28711=EDGE_CURVE ( 'NONE', #21327, #37913, #34111, .T. ) ;
#28712=CARTESIAN_POINT ( 'NONE',  ( -23.33693525117809386, 0.000000000000000000, 5.746789908705562944 ) ) ;
#28713=CARTESIAN_POINT ( 'NONE',  ( 2.072287782118878319, 0.000000000000000000, -2.950529333540147015 ) ) ;
#28714=CARTESIAN_POINT ( 'NONE',  ( -16.06709938707323460, 0.000000000000000000, 13.13181314741652628 ) ) ;
#28715=ADVANCED_FACE ( 'NONE', ( #47733 ), #26990, .F. ) ;
#28716=ORIENTED_EDGE ( 'NONE', *, *, #46368, .T. ) ;
#28717=DIRECTION ( 'NONE',  ( 0.007781995580012662783, 0.000000000000000000, -0.9999697198139514409 ) ) ;
#28718=CARTESIAN_POINT ( 'NONE',  ( -19.62794756868486346, -0.1191753592594171213, 5.875657136580680451 ) ) ;
#28719=ADVANCED_FACE ( 'NONE', ( #32079 ), #44852, .F. ) ;
#28720=LINE ( 'NONE', #2298, #53926 ) ;
#28721=CARTESIAN_POINT ( 'NONE',  ( -29.86274838104827367, -0.1191753592594197858, 8.381332038739175871 ) ) ;
#28722=DIRECTION ( 'NONE',  ( 0.007781995580012663651, -3.146120232559066537E-19, -0.9999697198139514409 ) ) ;
#28723=PLANE ( 'NONE',  #25221 ) ;
#28724=VECTOR ( 'NONE', #27888, 1000.000000000000227 ) ;
#28726=ORIENTED_EDGE ( 'NONE', *, *, #24328, .F. ) ;
#28727=CARTESIAN_POINT ( 'NONE',  ( -13.00944197295985916, 0.000000000000000000, 4.180506556583391209 ) ) ;
#28729=VERTEX_POINT ( 'NONE', #10207 ) ;
#28730=CARTESIAN_POINT ( 'NONE',  ( -13.08330893211609869, 0.000000000000000000, 1.763933231766363630 ) ) ;
#28732=VECTOR ( 'NONE', #33142, 999.9999999999998863 ) ;
#28733=CARTESIAN_POINT ( 'NONE',  ( -18.69005161448685115, -0.1191753592594169547, 4.774959850343403645 ) ) ;
#28734=CARTESIAN_POINT ( 'NONE',  ( -17.89488364610653903, -0.8417996532631562001, 3.805443821891801193 ) ) ;
#28735=PLANE ( 'NONE',  #35665 ) ;
#28736=ORIENTED_EDGE ( 'NONE', *, *, #47286, .T. ) ;
#28737=VECTOR ( 'NONE', #30186, 1000.000000000000227 ) ;
#28740=LINE ( 'NONE', #46596, #44734 ) ;
#28741=EDGE_CURVE ( 'NONE', #52604, #17849, #48559, .T. ) ;
#28742=CARTESIAN_POINT ( 'NONE',  ( -9.031895553247439423, 0.000000000000000000, 4.750118825932213795 ) ) ;
#28743=AXIS2_PLACEMENT_3D ( 'NONE', #39103, #46795, #12139 ) ;
#28744=ORIENTED_EDGE ( 'NONE', *, *, #20282, .F. ) ;
#28745=DIRECTION ( 'NONE',  ( -0.7660212471507179544, -0.6427876096865405842, -0.005961354470445141482 ) ) ;
#28746=ORIENTED_EDGE ( 'NONE', *, *, #1471, .T. ) ;
#28747=CARTESIAN_POINT ( 'NONE',  ( -25.20200914511100265, -0.1191753592594197858, 6.570942640130446932 ) ) ;
#28748=ADVANCED_FACE ( 'NONE', ( #23553 ), #53383, .F. ) ;
#28749=EDGE_CURVE ( 'NONE', #50088, #27679, #5668, .T. ) ;
#28750=VECTOR ( 'NONE', #6873, 1000.000000000000227 ) ;
#28751=VERTEX_POINT ( 'NONE', #9675 ) ;
#28752=ORIENTED_EDGE ( 'NONE', *, *, #40228, .T. ) ;
#28753=FACE_OUTER_BOUND ( 'NONE', #36989, .T. ) ;
#28754=CARTESIAN_POINT ( 'NONE',  ( -15.88130887279446490, 0.000000000000000000, 3.050160814894388839 ) ) ;
#28755=CARTESIAN_POINT ( 'NONE',  ( -18.83646877814363663, -0.8417996532631553119, 5.380192537759650229 ) ) ;
#28756=ORIENTED_EDGE ( 'NONE', *, *, #38532, .T. ) ;
#28757=DIRECTION ( 'NONE',  ( 0.005002170337468016433, -0.7660444431189770143, -0.6427681459581293666 ) ) ;
#28758=ORIENTED_EDGE ( 'NONE', *, *, #29681, .F. ) ;
#28759=EDGE_CURVE ( 'NONE', #46034, #31630, #44301, .T. ) ;
#28760=VERTEX_POINT ( 'NONE', #1110 ) ;
#28761=ORIENTED_EDGE ( 'NONE', *, *, #2052, .T. ) ;
#28762=DIRECTION ( 'NONE',  ( 0.5449076811759707706, 0.6444004775717708799, -0.5364919789714476250 ) ) ;
#28763=DIRECTION ( 'NONE',  ( -0.9321478471874540261, 0.000000000000000000, 0.3620778797217457656 ) ) ;
#28764=EDGE_LOOP ( 'NONE', ( #4176, #28756, #26026, #25393 ) ) ;
#28765=FACE_OUTER_BOUND ( 'NONE', #22358, .T. ) ;
#28767=DIRECTION ( 'NONE',  ( 0.6427681459581294776, -0.7660444431189769032, 0.005002170337467562802 ) ) ;
#28768=FACE_OUTER_BOUND ( 'NONE', #46843, .T. ) ;
#28770=VECTOR ( 'NONE', #31878, 999.9999999999998863 ) ;
#28771=DIRECTION ( 'NONE',  ( 0.2426528472758542054, 0.7422098413412800966, 0.6246952433987894571 ) ) ;
#28772=ORIENTED_EDGE ( 'NONE', *, *, #13636, .T. ) ;
#28773=EDGE_CURVE ( 'NONE', #17943, #2828, #45146, .T. ) ;
#28774=VECTOR ( 'NONE', #8979, 999.9999999999998863 ) ;
#28775=LINE ( 'NONE', #24773, #30089 ) ;
#28776=LINE ( 'NONE', #41268, #46537 ) ;
#28777=DIRECTION ( 'NONE',  ( -0.005002170337468016433, -0.7660444431189770143, 0.6427681459581293666 ) ) ;
#28778=DIRECTION ( 'NONE',  ( -0.5449076811759708816, 0.6444004775717707689, 0.5364919789714475140 ) ) ;
#28779=CARTESIAN_POINT ( 'NONE',  ( -15.87975247367846166, 0.000000000000000000, 2.850166870931599927 ) ) ;
#28780=DIRECTION ( 'NONE',  ( 0.005961354470445682716, -0.6427876096865404731, -0.7660212471507180654 ) ) ;
#28781=ORIENTED_EDGE ( 'NONE', *, *, #44059, .F. ) ;
#28783=EDGE_LOOP ( 'NONE', ( #16473, #51532, #41354, #35073 ) ) ;
#28784=VECTOR ( 'NONE', #54142, 1000.000000000000114 ) ;
#28785=DIRECTION ( 'NONE',  ( 0.000000000000000000, -1.000000000000000000, 0.000000000000000000 ) ) ;
#28786=EDGE_CURVE ( 'NONE', #27546, #38691, #18446, .T. ) ;
#28787=CARTESIAN_POINT ( 'NONE',  ( -24.27063949748155380, 0.000000000000000000, 6.308861732390097288 ) ) ;
#28788=LINE ( 'NONE', #1318, #44946 ) ;
#28789=CARTESIAN_POINT ( 'NONE',  ( -18.36514955148751582, 0.6102101463440047224, 3.796110601923448069 ) ) ;
#28790=DIRECTION ( 'NONE',  ( -0.7660212471507179544, -0.6427876096865405842, -0.005961354470445141482 ) ) ;
#28791=DIRECTION ( 'NONE',  ( 0.000000000000000000, -1.000000000000000000, 0.000000000000000000 ) ) ;
#28792=ORIENTED_EDGE ( 'NONE', *, *, #17936, .T. ) ;
#28793=CARTESIAN_POINT ( 'NONE',  ( -13.73672976910459909, 0.000000000000000000, 12.22661844811216270 ) ) ;
#28794=DIRECTION ( 'NONE',  ( -0.5364919789714478471, 0.6444004775717705469, -0.5449076811759709926 ) ) ;
#28795=ORIENTED_EDGE ( 'NONE', *, *, #4093, .T. ) ;
#28796=DIRECTION ( 'NONE',  ( 0.9999697198139515519, 0.000000000000000000, 0.007781995580013368816 ) ) ;
#28797=LINE ( 'NONE', #3506, #54013 ) ;
#28798=VERTEX_POINT ( 'NONE', #44011 ) ;
#28799=EDGE_CURVE ( 'NONE', #15255, #31, #49394, .T. ) ;
#28802=DIRECTION ( 'NONE',  ( -0.5364919789714478471, 0.6444004775717705469, -0.5449076811759709926 ) ) ;
#28803=EDGE_CURVE ( 'NONE', #22744, #24469, #1687, .T. ) ;
#28804=EDGE_CURVE ( 'NONE', #49949, #39181, #48846, .T. ) ;
#28805=LINE ( 'NONE', #28503, #17819 ) ;
#28806=LINE ( 'NONE', #32760, #44640 ) ;
#28807=VERTEX_POINT ( 'NONE', #49102 ) ;
#28808=VERTEX_POINT ( 'NONE', #27245 ) ;
#28809=CARTESIAN_POINT ( 'NONE',  ( -16.81345671998191449, 0.000000000000000000, 3.412238694616132495 ) ) ;
#28810=CARTESIAN_POINT ( 'NONE',  ( -31.72782227498118601, 0.000000000000000000, 9.205484770164058972 ) ) ;
#28811=DIRECTION ( 'NONE',  ( 0.9999697198139515519, 0.000000000000000000, 0.007781995580013368816 ) ) ;
#28812=EDGE_CURVE ( 'NONE', #46187, #42035, #53640, .T. ) ;
#28813=CARTESIAN_POINT ( 'NONE',  ( -30.79567442779373110, 0.000000000000000000, 8.843406890442315316 ) ) ;
#28814=CARTESIAN_POINT ( 'NONE',  ( -16.71591784297447703, 1.419719901456506728, 3.129665398755458572 ) ) ;
#28815=EDGE_CURVE ( 'NONE', #41698, #18658, #5971, .T. ) ;
#28816=FACE_OUTER_BOUND ( 'NONE', #22545, .T. ) ;
#28817=ORIENTED_EDGE ( 'NONE', *, *, #50789, .T. ) ;
#28818=PLANE ( 'NONE',  #18386 ) ;
#28819=ADVANCED_FACE ( 'NONE', ( #44557 ), #22995, .F. ) ;
#28820=LINE ( 'NONE', #7225, #29582 ) ;
#28821=VECTOR ( 'NONE', #52741, 999.9999999999998863 ) ;
#28822=FACE_OUTER_BOUND ( 'NONE', #40633, .T. ) ;
#28824=LINE ( 'NONE', #16577, #51953 ) ;
#28825=CARTESIAN_POINT ( 'NONE',  ( -18.22828877115104618, -0.1191753592594170102, 5.147885465369180125 ) ) ;
#28826=PLANE ( 'NONE',  #35717 ) ;
#28827=EDGE_CURVE ( 'NONE', #5706, #24756, #35236, .T. ) ;
#28828=EDGE_LOOP ( 'NONE', ( #38962, #46769, #55424, #56150 ) ) ;
#28829=VECTOR ( 'NONE', #46647, 999.9999999999998863 ) ;
#28830=EDGE_CURVE ( 'NONE', #45510, #52648, #30941, .T. ) ;
#28831=CARTESIAN_POINT ( 'NONE',  ( -19.05158305253015527, 3.038739411681507185, 9.268692036737574469 ) ) ;
#28832=EDGE_LOOP ( 'NONE', ( #51588, #54786, #36786, #26492 ) ) ;
#28833=EDGE_CURVE ( 'NONE', #13341, #49603, #844, .T. ) ;
#28834=ORIENTED_EDGE ( 'NONE', *, *, #36107, .T. ) ;
#28835=ORIENTED_EDGE ( 'NONE', *, *, #19334, .T. ) ;
#28836=ORIENTED_EDGE ( 'NONE', *, *, #4885, .F. ) ;
#28837=ORIENTED_EDGE ( 'NONE', *, *, #49744, .F. ) ;
#28838=DIRECTION ( 'NONE',  ( 0.9999697198139515519, 0.000000000000000000, 0.007781995580013368816 ) ) ;
#28839=EDGE_LOOP ( 'NONE', ( #20144, #155, #32359, #8041 ) ) ;
#28841=DIRECTION ( 'NONE',  ( 0.000000000000000000, -0.000000000000000000, -1.000000000000000000 ) ) ;
#28842=ORIENTED_EDGE ( 'NONE', *, *, #14757, .F. ) ;
#28843=ORIENTED_EDGE ( 'NONE', *, *, #45431, .F. ) ;
#28844=PLANE ( 'NONE',  #240 ) ;
#28845=DIRECTION ( 'NONE',  ( -0.5449076811759708816, 0.6444004775717707689, 0.5364919789714475140 ) ) ;
#28847=CARTESIAN_POINT ( 'NONE',  ( -20.79233874698950757, 1.257817950434006571, 7.022065141322721082 ) ) ;
#28848=ORIENTED_EDGE ( 'NONE', *, *, #23016, .F. ) ;
#28849=DIRECTION ( 'NONE',  ( -0.6427681459581293666, -0.7660444431189770143, -0.005002170337467561935 ) ) ;
#28850=ORIENTED_EDGE ( 'NONE', *, *, #14953, .F. ) ;
#28851=ORIENTED_EDGE ( 'NONE', *, *, #41292, .F. ) ;
#28852=PLANE ( 'NONE',  #51196 ) ;
#28853=EDGE_CURVE ( 'NONE', #26568, #19155, #6791, .T. ) ;
#28854=CARTESIAN_POINT ( 'NONE',  ( -30.79411802867772607, 0.000000000000000000, 8.643412946479525516 ) ) ;
#28856=DIRECTION ( 'NONE',  ( -0.005961354470445682716, -0.6427876096865404731, 0.7660212471507180654 ) ) ;
#28857=CARTESIAN_POINT ( 'NONE',  ( 1.086233639165236964, 0.000000000000000000, 2.796443541562362078 ) ) ;
#28858=CARTESIAN_POINT ( 'NONE',  ( -15.44046739010452818, -0.1191753592594188005, 5.169580935977237779 ) ) ;
#28859=ORIENTED_EDGE ( 'NONE', *, *, #21713, .F. ) ;
#28860=LINE ( 'NONE', #41623, #12022 ) ;
#28861=ORIENTED_EDGE ( 'NONE', *, *, #22476, .T. ) ;
#28862=EDGE_CURVE ( 'NONE', #54123, #15809, #37742, .T. ) ;
#28863=VECTOR ( 'NONE', #5526, 1000.000000000000227 ) ;
#28865=FACE_OUTER_BOUND ( 'NONE', #48810, .T. ) ;
#28866=CARTESIAN_POINT ( 'NONE',  ( -8.409922665610809034, 0.000000000000000000, 10.23674650875856962 ) ) ;
#28867=DIRECTION ( 'NONE',  ( -0.005002170337468016433, -0.7660444431189770143, 0.6427681459581293666 ) ) ;
#28868=EDGE_CURVE ( 'NONE', #24781, #20661, #11033, .T. ) ;
#28869=EDGE_CURVE ( 'NONE', #54798, #30130, #6506, .T. ) ;
#28870=CARTESIAN_POINT ( 'NONE',  ( -21.47341775636118655, -0.1191753592594197858, 5.122631121243466090 ) ) ;
#28871=ORIENTED_EDGE ( 'NONE', *, *, #16339, .F. ) ;
#28872=ORIENTED_EDGE ( 'NONE', *, *, #53075, .F. ) ;
#28873=LINE ( 'NONE', #7275, #43899 ) ;
#28874=CARTESIAN_POINT ( 'NONE',  ( 2.072287782118878319, 0.000000000000000000, -2.950529333540147015 ) ) ;
#28875=CARTESIAN_POINT ( 'NONE',  ( -20.54049170961573267, 0.000000000000000000, 4.660556269540326646 ) ) ;
#28876=LINE ( 'NONE', #37676, #30074 ) ;
#28877=EDGE_CURVE ( 'NONE', #35256, #50946, #24648, .T. ) ;
#28878=DIRECTION ( 'NONE',  ( 0.000000000000000000, 0.000000000000000000, -1.000000000000000000 ) ) ;
#28879=CARTESIAN_POINT ( 'NONE',  ( -9.214449502844235695, 0.000000000000000000, 3.271369869658160567 ) ) ;
#28880=CARTESIAN_POINT ( 'NONE',  ( -14.94838282604903057, -0.1191753592594194527, 2.588085963191248506 ) ) ;
#28881=ADVANCED_FACE ( 'NONE', ( #37430 ), #49926, .F. ) ;
#28884=EDGE_LOOP ( 'NONE', ( #8742, #44113, #32164, #33440, #13010 ) ) ;
#28885=ADVANCED_FACE ( 'NONE', ( #2524 ), #28352, .F. ) ;
#28886=ORIENTED_EDGE ( 'NONE', *, *, #28472, .T. ) ;
#28887=EDGE_CURVE ( 'NONE', #13455, #10554, #23816, .T. ) ;
#28888=ORIENTED_EDGE ( 'NONE', *, *, #50493, .T. ) ;
#28889=EDGE_LOOP ( 'NONE', ( #40130, #8925, #52996, #50944 ) ) ;
#28890=VERTEX_POINT ( 'NONE', #41443 ) ;
#28891=ORIENTED_EDGE ( 'NONE', *, *, #22396, .F. ) ;
#28892=LINE ( 'NONE', #16366, #41394 ) ;
#28893=FACE_OUTER_BOUND ( 'NONE', #39438, .T. ) ;
#28894=DIRECTION ( 'NONE',  ( 0.005002170337468016433, -0.7660444431189770143, -0.6427681459581293666 ) ) ;
#28895=VECTOR ( 'NONE', #25363, 999.9999999999998863 ) ;
#28896=ORIENTED_EDGE ( 'NONE', *, *, #20832, .F. ) ;
#28897=CARTESIAN_POINT ( 'NONE',  ( -24.26986129792355129, -0.1191753592594197858, 6.208864760408702388 ) ) ;
#28898=VERTEX_POINT ( 'NONE', #45675 ) ;
#28899=LINE ( 'NONE', #46195, #24965 ) ;
#28902=DIRECTION ( 'NONE',  ( -0.005961354470445682716, -0.6427876096865404731, 0.7660212471507180654 ) ) ;
#28903=CARTESIAN_POINT ( 'NONE',  ( -11.56765945739309487, 0.2864062442990042978, 1.166065645416680008 ) ) ;
#28904=ORIENTED_EDGE ( 'NONE', *, *, #8754, .T. ) ;
#28905=CARTESIAN_POINT ( 'NONE',  ( -19.06984000643095456, 0.000000000000000000, 6.718667626403617810 ) ) ;
#28906=ADVANCED_FACE ( 'NONE', ( #33206 ), #41147, .F. ) ;
#28907=VERTEX_POINT ( 'NONE', #20400 ) ;
#28908=DIRECTION ( 'NONE',  ( 0.5449076811759707706, 0.6444004775717708799, -0.5364919789714476250 ) ) ;
#28910=LINE ( 'NONE', #46204, #10324 ) ;
#28911=LINE ( 'NONE', #28068, #26934 ) ;
#28913=FACE_OUTER_BOUND ( 'NONE', #28702, .T. ) ;
#28914=LINE ( 'NONE', #45957, #17474 ) ;
#28915=DIRECTION ( 'NONE',  ( -0.5449076811759708816, 0.6444004775717707689, 0.5364919789714475140 ) ) ;
#28916=EDGE_CURVE ( 'NONE', #50409, #53549, #20100, .T. ) ;
#28917=PLANE ( 'NONE',  #11252 ) ;
#28918=CARTESIAN_POINT ( 'NONE',  ( -10.22162059191334116, 0.000000000000000000, 4.202202027191447087 ) ) ;
#28919=ORIENTED_EDGE ( 'NONE', *, *, #33018, .T. ) ;
#28921=ORIENTED_EDGE ( 'NONE', *, *, #13098, .F. ) ;
#28922=EDGE_CURVE ( 'NONE', #21908, #11209, #28657, .T. ) ;
#28923=EDGE_CURVE ( 'NONE', #21327, #12775, #7086, .T. ) ;
#28924=ADVANCED_FACE ( 'NONE', ( #41690 ), #50519, .F. ) ;
#28925=DIRECTION ( 'NONE',  ( 0.005002170337468016433, -0.7660444431189770143, -0.6427681459581293666 ) ) ;
#28926=CARTESIAN_POINT ( 'NONE',  ( -15.56998309669674718, 0.000000000000000000, 8.961896740978279041 ) ) ;
#28927=DIRECTION ( 'NONE',  ( 0.5449076811759707706, 0.6444004775717708799, -0.5364919789714476250 ) ) ;
#28928=DIRECTION ( 'NONE',  ( -0.7660212471507179544, -0.6427876096865405842, -0.005961354470445141482 ) ) ;
#28929=DIRECTION ( 'NONE',  ( -0.005961354470445682716, -0.6427876096865404731, 0.7660212471507180654 ) ) ;
#28930=CARTESIAN_POINT ( 'NONE',  ( -18.63760471526975593, 0.9340140483890051470, 3.891610400377997436 ) ) ;
#28933=DIRECTION ( 'NONE',  ( -0.5364919789714478471, 0.6444004775717705469, -0.5449076811759709926 ) ) ;
#28934=DIRECTION ( 'NONE',  ( 0.005961354470445682716, -0.6427876096865404731, -0.7660212471507180654 ) ) ;
#28935=LINE ( 'NONE', #41966, #20396 ) ;
#28936=DIRECTION ( 'NONE',  ( 0.007781995580012662783, 0.000000000000000000, -0.9999697198139514409 ) ) ;
#28937=LINE ( 'NONE', #2527, #570 ) ;
#28938=DIRECTION ( 'NONE',  ( -0.5364919789714478471, 0.6444004775717705469, -0.5449076811759709926 ) ) ;
#28939=ADVANCED_FACE ( 'NONE', ( #42276 ), #15043, .F. ) ;
#28940=CARTESIAN_POINT ( 'NONE',  ( -17.32134905586179130, -3.432230869623160263, 9.043007527150438207 ) ) ;
#28941=PLANE ( 'NONE',  #27746 ) ;
#28942=LINE ( 'NONE', #20959, #22003 ) ;
#28943=ORIENTED_EDGE ( 'NONE', *, *, #30548, .F. ) ;
#28944=EDGE_CURVE ( 'NONE', #42380, #18980, #49684, .T. ) ;
#28945=LINE ( 'NONE', #46238, #23999 ) ;
#28946=CARTESIAN_POINT ( 'NONE',  ( -10.27421835998572064, 0.000000000000000000, 10.96090226820206048 ) ) ;
#28947=ORIENTED_EDGE ( 'NONE', *, *, #39668, .F. ) ;
#28948=EDGE_CURVE ( 'NONE', #43321, #41488, #34579, .T. ) ;
#28949=DIRECTION ( 'NONE',  ( 0.7660212471507180654, -0.6427876096865404731, 0.005961354470445141482 ) ) ;
#28950=CARTESIAN_POINT ( 'NONE',  ( -16.28333627977372089, 0.000000000000000000, 6.909678856306649131 ) ) ;
#28951=ADVANCED_FACE ( 'NONE', ( #30339 ), #56172, .F. ) ;
#28952=VERTEX_POINT ( 'NONE', #38274 ) ;
#28953=VERTEX_POINT ( 'NONE', #51895 ) ;
#28954=DIRECTION ( 'NONE',  ( 0.6427681459581294776, -0.7660444431189769032, 0.005002170337467562802 ) ) ;
#28955=ORIENTED_EDGE ( 'NONE', *, *, #53470, .F. ) ;
#28956=VERTEX_POINT ( 'NONE', #42811 ) ;
#28957=ORIENTED_EDGE ( 'NONE', *, *, #2887, .F. ) ;
#28958=FACE_OUTER_BOUND ( 'NONE', #42446, .T. ) ;
#28959=CARTESIAN_POINT ( 'NONE',  ( -17.74404816805336793, 0.000000000000000000, 3.574322630375089460 ) ) ;
#28960=FACE_OUTER_BOUND ( 'NONE', #6601, .T. ) ;
#28961=ORIENTED_EDGE ( 'NONE', *, *, #10498, .T. ) ;
#28962=ORIENTED_EDGE ( 'NONE', *, *, #37666, .T. ) ;
#28963=LINE ( 'NONE', #20726, #19390 ) ;
#28964=DIRECTION ( 'NONE',  ( 0.005961354470445682716, -0.6427876096865404731, -0.7660212471507180654 ) ) ;
#28965=ORIENTED_EDGE ( 'NONE', *, *, #9412, .T. ) ;
#28966=CARTESIAN_POINT ( 'NONE',  ( 2.072287782118878319, 0.000000000000000000, -2.950529333540147015 ) ) ;
#28967=ORIENTED_EDGE ( 'NONE', *, *, #9718, .F. ) ;
#28968=LINE ( 'NONE', #26312, #52099 ) ;
#28969=CARTESIAN_POINT ( 'NONE',  ( -16.85955541371576771, 3.200641362704007786, 8.682942744200573770 ) ) ;
#28970=EDGE_LOOP ( 'NONE', ( #43543, #29040, #29063, #1541, #47384 ) ) ;
#28971=PLANE ( 'NONE',  #13731 ) ;
#28972=EDGE_CURVE ( 'NONE', #16128, #2673, #21243, .T. ) ;
#28973=CARTESIAN_POINT ( 'NONE',  ( -11.85736786543846932, -1.975113310420660184, 1.424109018569633234 ) ) ;
#28974=VERTEX_POINT ( 'NONE', #7932 ) ;
#28975=DIRECTION ( 'NONE',  ( 0.6427681459581294776, -0.7660444431189769032, 0.005002170337467562802 ) ) ;
#28977=DIRECTION ( 'NONE',  ( 0.9999697198139515519, 0.000000000000000000, 0.007781995580013368816 ) ) ;
#28978=ORIENTED_EDGE ( 'NONE', *, *, #8767, .F. ) ;
#28979=ADVANCED_FACE ( 'NONE', ( #201 ), #25499, .F. ) ;
#28980=EDGE_CURVE ( 'NONE', #39017, #43351, #55597, .T. ) ;
#28981=ADVANCED_FACE ( 'NONE', ( #47938 ), #13012, .F. ) ;
#28982=PLANE ( 'NONE',  #26507 ) ;
#28983=DIRECTION ( 'NONE',  ( -0.005002170337468016433, -0.7660444431189770143, 0.6427681459581293666 ) ) ;
#28984=CARTESIAN_POINT ( 'NONE',  ( -17.26532721389163072, 0.000000000000000000, 13.67648636611514590 ) ) ;
#28985=LINE ( 'NONE', #28415, #2327 ) ;
#28986=EDGE_CURVE ( 'NONE', #29764, #47771, #43398, .T. ) ;
#28987=DIRECTION ( 'NONE',  ( 0.000000000000000000, 1.000000000000000000, 0.000000000000000000 ) ) ;
#28988=DIRECTION ( 'NONE',  ( 0.000000000000000000, -0.000000000000000000, -1.000000000000000000 ) ) ;
#28989=CARTESIAN_POINT ( 'NONE',  ( -28.93137873341882127, 0.000000000000000000, 8.119251130998824451 ) ) ;
#28990=ORIENTED_EDGE ( 'NONE', *, *, #8329, .F. ) ;
#28991=FACE_OUTER_BOUND ( 'NONE', #34565, .T. ) ;
#28992=DIRECTION ( 'NONE',  ( -0.5364919789714478471, 0.6444004775717705469, -0.5449076811759709926 ) ) ;
#28993=LINE ( 'NONE', #3437, #13297 ) ;
#28994=ORIENTED_EDGE ( 'NONE', *, *, #8740, .F. ) ;
#28995=LINE ( 'NONE', #49991, #37447 ) ;
#28996=DIRECTION ( 'NONE',  ( 0.5364919789714477361, 0.6444004775717706579, 0.5449076811759711036 ) ) ;
#28997=DIRECTION ( 'NONE',  ( 0.9999697198139515519, 0.000000000000000000, 0.007781995580013368816 ) ) ;
#28998=DIRECTION ( 'NONE',  ( -0.6427681459581293666, -0.7660444431189770143, -0.005002170337467561935 ) ) ;
#28999=EDGE_CURVE ( 'NONE', #46991, #51210, #30636, .T. ) ;
#29000=CARTESIAN_POINT ( 'NONE',  ( -20.56670277481199349, 0.4483081953215036219, 5.605877047346789155 ) ) ;
#29001=ORIENTED_EDGE ( 'NONE', *, *, #9500, .T. ) ;
#29002=ORIENTED_EDGE ( 'NONE', *, *, #15690, .F. ) ;
#29003=EDGE_CURVE ( 'NONE', #32478, #21588, #26338, .T. ) ;
#29004=DIRECTION ( 'NONE',  ( -0.7660212471507179544, -0.6427876096865405842, -0.005961354470445141482 ) ) ;
#29005=DIRECTION ( 'NONE',  ( 0.9999697198139515519, 0.000000000000000000, 0.007781995580013368816 ) ) ;
#29006=ADVANCED_FACE ( 'NONE', ( #38012 ), #55901, .F. ) ;
#29007=ORIENTED_EDGE ( 'NONE', *, *, #38025, .F. ) ;
#29008=CARTESIAN_POINT ( 'NONE',  ( -12.72599829993386322, 0.000000000000000000, 1.766713905726021938 ) ) ;
#29009=VERTEX_POINT ( 'NONE', #8191 ) ;
#29010=CARTESIAN_POINT ( 'NONE',  ( -12.40227819300294954, -2.622721114510660367, 1.615108615478732190 ) ) ;
#29012=VERTEX_POINT ( 'NONE', #17851 ) ;
#29013=VERTEX_POINT ( 'NONE', #35718 ) ;
#29014=VERTEX_POINT ( 'NONE', #35180 ) ;
#29015=LINE ( 'NONE', #45480, #38380 ) ;
#29016=DIRECTION ( 'NONE',  ( 0.5364919789714477361, 0.6444004775717706579, 0.5449076811759711036 ) ) ;
#29017=LINE ( 'NONE', #46313, #41174 ) ;
#29018=EDGE_LOOP ( 'NONE', ( #33307, #19921, #42369, #48235 ) ) ;
#29019=DIRECTION ( 'NONE',  ( 0.6427681459581294776, -0.7660444431189769032, 0.005002170337467562802 ) ) ;
#29020=VERTEX_POINT ( 'NONE', #52474 ) ;
#29021=EDGE_LOOP ( 'NONE', ( #34287, #44805, #8491, #36303 ) ) ;
#29022=ORIENTED_EDGE ( 'NONE', *, *, #1647, .T. ) ;
#29023=LINE ( 'NONE', #12560, #22261 ) ;
#29024=FACE_OUTER_BOUND ( 'NONE', #35030, .T. ) ;
#29025=VERTEX_POINT ( 'NONE', #53033 ) ;
#29026=DIRECTION ( 'NONE',  ( 0.3313982828793700097, 0.4028455766673915694, 0.8531650599175529814 ) ) ;
#29027=VERTEX_POINT ( 'NONE', #14150 ) ;
#29028=CARTESIAN_POINT ( 'NONE',  ( 2.072287782118878319, 0.000000000000000000, -2.950529333540147015 ) ) ;
#29030=ORIENTED_EDGE ( 'NONE', *, *, #22495, .T. ) ;
#29032=ORIENTED_EDGE ( 'NONE', *, *, #5251, .F. ) ;
#29033=VECTOR ( 'NONE', #15293, 999.9999999999998863 ) ;
#29034=LINE ( 'NONE', #11981, #45516 ) ;
#29035=CARTESIAN_POINT ( 'NONE',  ( -14.14290141849938465, 0.000000000000000000, 4.710343796484107948 ) ) ;
#29036=DIRECTION ( 'NONE',  ( 0.000000000000000000, -0.000000000000000000, -1.000000000000000000 ) ) ;
#29037=LINE ( 'NONE', #46336, #2127 ) ;
#29038=CARTESIAN_POINT ( 'NONE',  ( -20.69024277472754392, 2.229229656569007290, 8.576659702205136071 ) ) ;
#29039=FACE_OUTER_BOUND ( 'NONE', #9379, .T. ) ;
#29040=ORIENTED_EDGE ( 'NONE', *, *, #9376, .T. ) ;
#29041=ADVANCED_FACE ( 'NONE', ( #22927 ), #53577, .F. ) ;
#29042=EDGE_LOOP ( 'NONE', ( #52300, #11934, #55421, #1407 ) ) ;
#29043=DIRECTION ( 'NONE',  ( 0.007781995580012663651, -3.146120232559066537E-19, -0.9999697198139514409 ) ) ;
#29044=DIRECTION ( 'NONE',  ( 0.6427681459581294776, -0.7660444431189769032, 0.005002170337467562802 ) ) ;
#29045=DIRECTION ( 'NONE',  ( -0.9999697198139514409, -0.000000000000000000, -0.007781995580013368816 ) ) ;
#29046=ADVANCED_FACE ( 'NONE', ( #31475 ), #13838, .F. ) ;
#29047=EDGE_CURVE ( 'NONE', #18224, #34917, #31164, .T. ) ;
#29048=CARTESIAN_POINT ( 'NONE',  ( -12.33850799832341849, 0.000000000000000000, 11.68350162852954632 ) ) ;
#29049=DIRECTION ( 'NONE',  ( 0.7660212471507180654, -0.6427876096865404731, 0.005961354470445141482 ) ) ;
#29050=CARTESIAN_POINT ( 'NONE',  ( -19.06696595292567054, 0.000000000000000000, 6.349357923145855231 ) ) ;
#29051=ORIENTED_EDGE ( 'NONE', *, *, #3553, .F. ) ;
#29052=CARTESIAN_POINT ( 'NONE',  ( -20.54126990917373519, -0.1191753592594197858, 4.760553241521720658 ) ) ;
#29053=DIRECTION ( 'NONE',  ( 0.000000000000000000, -1.000000000000000000, 0.000000000000000000 ) ) ;
#29054=VERTEX_POINT ( 'NONE', #48489 ) ;
#29055=CARTESIAN_POINT ( 'NONE',  ( -15.18422100874571434, -5.375054281893165253, 2.607895842203279191 ) ) ;
#29056=FACE_OUTER_BOUND ( 'NONE', #42054, .T. ) ;
#29057=ORIENTED_EDGE ( 'NONE', *, *, #6811, .T. ) ;
#29059=DIRECTION ( 'NONE',  ( -0.5449076811759708816, 0.6444004775717707689, 0.5364919789714475140 ) ) ;
#29060=PLANE ( 'NONE',  #6898 ) ;
#29061=CARTESIAN_POINT ( 'NONE',  ( -13.96302584907357236, 0.000000000000000000, 7.297068118404461678 ) ) ;
#29062=PLANE ( 'NONE',  #2918 ) ;
#29063=ORIENTED_EDGE ( 'NONE', *, *, #18230, .T. ) ;
#29064=ORIENTED_EDGE ( 'NONE', *, *, #36544, .T. ) ;
#29065=PLANE ( 'NONE',  #16738 ) ;
#29066=PLANE ( 'NONE',  #33141 ) ;
#29067=DIRECTION ( 'NONE',  ( 0.9999697198139515519, 0.000000000000000000, 0.007781995580013368816 ) ) ;
#29068=DIRECTION ( 'NONE',  ( -0.5364919789714478471, 0.6444004775717705469, -0.5449076811759709926 ) ) ;
#29069=CARTESIAN_POINT ( 'NONE',  ( -10.74029228357944987, 0.000000000000000000, 11.14194120806293320 ) ) ;
#29070=CARTESIAN_POINT ( 'NONE',  ( -16.81345671998191449, 0.000000000000000000, 3.412238694616132495 ) ) ;
#29071=ORIENTED_EDGE ( 'NONE', *, *, #15048, .F. ) ;
#29072=CARTESIAN_POINT ( 'NONE',  ( -12.58558820878208451, 4.819660872929013351, 1.416829184615139736 ) ) ;
#29073=ADVANCED_FACE ( 'NONE', ( #35429 ), #4766, .F. ) ;
#29074=VECTOR ( 'NONE', #12396, 999.9999999999998863 ) ;
#29075=LINE ( 'NONE', #16293, #53216 ) ;
#29076=CARTESIAN_POINT ( 'NONE',  ( -12.73905091307099546, 0.000000000000000000, 3.443946662719867824 ) ) ;
#29077=EDGE_LOOP ( 'NONE', ( #4398, #16741, #50396, #25585 ) ) ;
#29078=EDGE_CURVE ( 'NONE', #46919, #38778, #48190, .T. ) ;
#29080=CARTESIAN_POINT ( 'NONE',  ( -15.86710544311044302, 0.000000000000000000, 13.13336954653252953 ) ) ;
#29081=FACE_OUTER_BOUND ( 'NONE', #18564, .T. ) ;
#29082=EDGE_LOOP ( 'NONE', ( #978, #21335, #31461, #21467, #54957 ) ) ;
#29083=LINE ( 'NONE', #54107, #44048 ) ;
#29084=EDGE_CURVE ( 'NONE', #49698, #9775, #44243, .T. ) ;
#29086=ORIENTED_EDGE ( 'NONE', *, *, #558, .T. ) ;
#29087=ORIENTED_EDGE ( 'NONE', *, *, #51435, .F. ) ;
#29088=ORIENTED_EDGE ( 'NONE', *, *, #51854, .T. ) ;
#29089=CARTESIAN_POINT ( 'NONE',  ( -14.20280369269832832, 0.000000000000000000, 12.40765738797303719 ) ) ;
#29091=VECTOR ( 'NONE', #28589, 1000.000000000000227 ) ;
#29092=ORIENTED_EDGE ( 'NONE', *, *, #28139, .T. ) ;
#29093=CARTESIAN_POINT ( 'NONE',  ( -14.66887761629205222, 0.000000000000000000, 12.58869632783390990 ) ) ;
#29094=ORIENTED_EDGE ( 'NONE', *, *, #46890, .F. ) ;
#29095=EDGE_LOOP ( 'NONE', ( #48963, #49236, #26579, #1839 ) ) ;
#29096=CARTESIAN_POINT ( 'NONE',  ( -16.76798113924479239, -2.784623065533159636, 7.765225900080996446 ) ) ;
#29097=LINE ( 'NONE', #6995, #35776 ) ;
#29098=DIRECTION ( 'NONE',  ( -0.5449076811759708816, 0.6444004775717707689, 0.5364919789714475140 ) ) ;
#29100=EDGE_CURVE ( 'NONE', #52840, #46950, #43943, .T. ) ;
#29101=DIRECTION ( 'NONE',  ( 0.7660212471507180654, -0.6427876096865404731, 0.005961354470445141482 ) ) ;
#29102=VERTEX_POINT ( 'NONE', #5066 ) ;
#29103=ORIENTED_EDGE ( 'NONE', *, *, #47699, .F. ) ;
#29104=VECTOR ( 'NONE', #15913, 1000.000000000000227 ) ;
#29105=DIRECTION ( 'NONE',  ( 0.007781995580012663651, 0.000000000000000000, -0.9999697198139515519 ) ) ;
#29106=LINE ( 'NONE', #2697, #46624 ) ;
#29108=EDGE_CURVE ( 'NONE', #43993, #36408, #9608, .T. ) ;
#29109=EDGE_CURVE ( 'NONE', #23095, #45238, #26931, .T. ) ;
#29110=VECTOR ( 'NONE', #3921, 999.9999999999998863 ) ;
#29111=FACE_OUTER_BOUND ( 'NONE', #48866, .T. ) ;
#29113=CARTESIAN_POINT ( 'NONE',  ( -15.88130887279446490, 0.000000000000000000, 3.050160814894388839 ) ) ;
#29114=PLANE ( 'NONE',  #40453 ) ;
#29115=VERTEX_POINT ( 'NONE', #36025 ) ;
#29116=DIRECTION ( 'NONE',  ( -0.6427681459581293666, -0.7660444431189770143, -0.005002170337467561935 ) ) ;
#29117=DIRECTION ( 'NONE',  ( -0.9999697198139514409, -0.000000000000000000, -0.007781995580013368816 ) ) ;
#29118=ORIENTED_EDGE ( 'NONE', *, *, #24192, .T. ) ;
#29119=FACE_OUTER_BOUND ( 'NONE', #42996, .T. ) ;
#29120=CARTESIAN_POINT ( 'NONE',  ( -13.23662005285947174, 0.000000000000000000, 7.672053246082242595 ) ) ;
#29121=PLANE ( 'NONE',  #9993 ) ;
#29122=DIRECTION ( 'NONE',  ( 0.000000000000000000, -0.000000000000000000, -1.000000000000000000 ) ) ;
#29124=DIRECTION ( 'NONE',  ( 0.007781995580012662783, 0.000000000000000000, -0.9999697198139514409 ) ) ;
#29125=EDGE_CURVE ( 'NONE', #55742, #32296, #786, .T. ) ;
#29126=ORIENTED_EDGE ( 'NONE', *, *, #26524, .T. ) ;
#29127=ORIENTED_EDGE ( 'NONE', *, *, #30206, .F. ) ;
#29128=CARTESIAN_POINT ( 'NONE',  ( -15.52954537527145185, -5.698858183938162902, 12.06693170300650308 ) ) ;
#29129=FACE_OUTER_BOUND ( 'NONE', #34096, .T. ) ;
#29130=CARTESIAN_POINT ( 'NONE',  ( -20.82430447243409333, -2.622721114510657703, 9.075130952061487122 ) ) ;
#29131=VECTOR ( 'NONE', #205, 999.9999999999998863 ) ;
#29132=VECTOR ( 'NONE', #20674, 1000.000000000000000 ) ;
#29133=DIRECTION ( 'NONE',  ( 0.007781995580012663651, -3.146120232559066537E-19, -0.9999697198139514409 ) ) ;
#29134=DIRECTION ( 'NONE',  ( 0.6427681459581294776, -0.7660444431189769032, 0.005002170337467562802 ) ) ;
#29136=CARTESIAN_POINT ( 'NONE',  ( -23.33693525117809386, 0.000000000000000000, 5.746789908705562944 ) ) ;
#29137=DIRECTION ( 'NONE',  ( 0.007781995580012662783, 0.000000000000000000, -0.9999697198139514409 ) ) ;
#29138=LINE ( 'NONE', #51301, #7447 ) ;
#29139=ORIENTED_EDGE ( 'NONE', *, *, #31628, .T. ) ;
#29140=CARTESIAN_POINT ( 'NONE',  ( 2.072287782118878319, 0.000000000000000000, -2.950529333540147015 ) ) ;
#29141=EDGE_LOOP ( 'NONE', ( #16430, #11414, #11955 ) ) ;
#29142=ADVANCED_FACE ( 'NONE', ( #44494 ), #31736, .F. ) ;
#29143=AXIS2_PLACEMENT_3D ( 'NONE', #28966, #49433, #46015 ) ;
#29144=ORIENTED_EDGE ( 'NONE', *, *, #47487, .F. ) ;
#29145=VERTEX_POINT ( 'NONE', #27463 ) ;
#29146=ORIENTED_EDGE ( 'NONE', *, *, #13639, .F. ) ;
#29147=VERTEX_POINT ( 'NONE', #52732 ) ;
#29148=DIRECTION ( 'NONE',  ( -0.5364919789714478471, 0.6444004775717705469, -0.5449076811759709926 ) ) ;
#29149=DIRECTION ( 'NONE',  ( -0.005002170337468016433, -0.7660444431189770143, 0.6427681459581293666 ) ) ;
#29150=LINE ( 'NONE', #51004, #13088 ) ;
#29151=ADVANCED_FACE ( 'NONE', ( #22652 ), #39963, .F. ) ;
#29152=ORIENTED_EDGE ( 'NONE', *, *, #19914, .T. ) ;
#29153=VERTEX_POINT ( 'NONE', #45611 ) ;
#29154=ORIENTED_EDGE ( 'NONE', *, *, #27082, .T. ) ;
#29155=FACE_OUTER_BOUND ( 'NONE', #46664, .T. ) ;
#29156=EDGE_CURVE ( 'NONE', #12964, #17849, #46171, .T. ) ;
#29157=EDGE_LOOP ( 'NONE', ( #51149, #11912, #22253, #20258 ) ) ;
#29158=EDGE_CURVE ( 'NONE', #31213, #10988, #54995, .T. ) ;
#29160=CARTESIAN_POINT ( 'NONE',  ( -10.19678563399013527, -0.07627425201977861002, 0.7424042488757021108 ) ) ;
#29161=CARTESIAN_POINT ( 'NONE',  ( -14.15439763252051364, 0.000000000000000000, 6.187582609515166254 ) ) ;
#29163=VERTEX_POINT ( 'NONE', #24325 ) ;
#29164=DIRECTION ( 'NONE',  ( 0.005002170337468016433, -0.7660444431189770143, -0.6427681459581293666 ) ) ;
#29165=EDGE_LOOP ( 'NONE', ( #937, #31502, #24348, #22538 ) ) ;
#29166=AXIS2_PLACEMENT_3D ( 'NONE', #14431, #10147, #40559 ) ;
#29167=VECTOR ( 'NONE', #28194, 999.9999999999998863 ) ;
#29168=DIRECTION ( 'NONE',  ( 0.9321478471874541372, 0.000000000000000000, -0.3620778797217453771 ) ) ;
#29169=EDGE_CURVE ( 'NONE', #20216, #15750, #6725, .T. ) ;
#29170=PLANE ( 'NONE',  #16636 ) ;
#29171=EDGE_CURVE ( 'NONE', #19445, #51083, #15792, .T. ) ;
#29172=CARTESIAN_POINT ( 'NONE',  ( -13.97320440870542413, 0.000000000000000000, 8.604991172140545430 ) ) ;
#29173=AXIS2_PLACEMENT_3D ( 'NONE', #3855, #38215, #25441 ) ;
#29174=DIRECTION ( 'NONE',  ( 0.9999697198139515519, 0.000000000000000000, 0.007781995580013368816 ) ) ;
#29175=FACE_OUTER_BOUND ( 'NONE', #34467, .T. ) ;
#29176=CARTESIAN_POINT ( 'NONE',  ( -22.40478740399063895, 0.000000000000000000, 5.384712028983816623 ) ) ;
#29177=DIRECTION ( 'NONE',  ( 0.7660212471507180654, -0.6427876096865404731, 0.005961354470445141482 ) ) ;
#29178=DIRECTION ( 'NONE',  ( 0.5449076811759707706, 0.6444004775717708799, -0.5364919789714476250 ) ) ;
#29179=EDGE_LOOP ( 'NONE', ( #50799, #37379, #40971, #49700 ) ) ;
#29180=CARTESIAN_POINT ( 'NONE',  ( -14.93495759592298988, 0.000000000000000000, 12.77129166681078409 ) ) ;
#29181=ORIENTED_EDGE ( 'NONE', *, *, #11319, .F. ) ;
#29182=EDGE_CURVE ( 'NONE', #29459, #13435, #28033, .T. ) ;
#29183=LINE ( 'NONE', #51618, #27443 ) ;
#29184=CARTESIAN_POINT ( 'NONE',  ( -27.06552663992790997, 0.000000000000000000, 7.195101427592543786 ) ) ;
#29185=DIRECTION ( 'NONE',  ( 0.7660212471507180654, -0.6427876096865404731, 0.005961354470445141482 ) ) ;
#29186=VECTOR ( 'NONE', #2749, 1000.000000000000227 ) ;
#29187=DIRECTION ( 'NONE',  ( -0.6427681459581293666, -0.7660444431189770143, -0.005002170337467561935 ) ) ;
#29188=DIRECTION ( 'NONE',  ( 0.9999697198139515519, 0.000000000000000000, 0.007781995580013368816 ) ) ;
#29189=AXIS2_PLACEMENT_3D ( 'NONE', #16975, #55566, #38540 ) ;
#29190=EDGE_CURVE ( 'NONE', #52307, #52077, #37363, .T. ) ;
#29192=EDGE_LOOP ( 'NONE', ( #3877, #1391, #52383, #15754 ) ) ;
#29193=CARTESIAN_POINT ( 'NONE',  ( -10.78547626117782521, -0.1191753592594183703, 4.097810943884039325 ) ) ;
#29194=DIRECTION ( 'NONE',  ( 0.007781995580012663651, 0.000000000000000000, -0.9999697198139515519 ) ) ;
#29195=LINE ( 'NONE', #12162, #10408 ) ;
#29196=FACE_OUTER_BOUND ( 'NONE', #45627, .T. ) ;
#29197=DIRECTION ( 'NONE',  ( 0.005961354470445682716, -0.6427876096865404731, -0.7660212471507180654 ) ) ;
#29198=CARTESIAN_POINT ( 'NONE',  ( -15.40103151951671734, 0.000000000000000000, 12.95233060667165681 ) ) ;
#29199=CARTESIAN_POINT ( 'NONE',  ( -12.98732645422466092, 1.419719901456506728, 1.681353879868476842 ) ) ;
#29200=DIRECTION ( 'NONE',  ( -0.005961354470445682716, -0.6427876096865404731, 0.7660212471507180654 ) ) ;
#29201=EDGE_LOOP ( 'NONE', ( #52517, #41518, #39440, #1014 ) ) ;
#29202=LINE ( 'NONE', #55073, #33082 ) ;
#29203=LINE ( 'NONE', #3648, #55000 ) ;
#29204=ORIENTED_EDGE ( 'NONE', *, *, #27983, .F. ) ;
#29205=AXIS2_PLACEMENT_3D ( 'NONE', #43939, #38859, #52189 ) ;
#29206=VERTEX_POINT ( 'NONE', #45340 ) ;
#29207=FACE_OUTER_BOUND ( 'NONE', #40544, .T. ) ;
#29208=VECTOR ( 'NONE', #21259, 1000.000000000000227 ) ;
#29209=VECTOR ( 'NONE', #10572, 1000.000000000000000 ) ;
#29210=ORIENTED_EDGE ( 'NONE', *, *, #52981, .T. ) ;
#29211=EDGE_CURVE ( 'NONE', #39021, #56226, #28873, .T. ) ;
#29212=ORIENTED_EDGE ( 'NONE', *, *, #45969, .T. ) ;
#29213=PLANE ( 'NONE',  #54652 ) ;
#29214=AXIS2_PLACEMENT_3D ( 'NONE', #5003, #8989, #39659 ) ;
#29215=ORIENTED_EDGE ( 'NONE', *, *, #7986, .F. ) ;
#29216=ORIENTED_EDGE ( 'NONE', *, *, #27490, .T. ) ;
#29217=VECTOR ( 'NONE', #18500, 1000.000000000000114 ) ;
#29218=ORIENTED_EDGE ( 'NONE', *, *, #48105, .F. ) ;
#29219=DIRECTION ( 'NONE',  ( 0.9999697198139515519, 0.000000000000000000, 0.007781995580013368816 ) ) ;
#29220=DIRECTION ( 'NONE',  ( 0.007781995580012663651, -3.146120232559066537E-19, -0.9999697198139514409 ) ) ;
#29221=LINE ( 'NONE', #20977, #31245 ) ;
#29223=EDGE_CURVE ( 'NONE', #10342, #20845, #2999, .T. ) ;
#29224=VERTEX_POINT ( 'NONE', #50718 ) ;
#29225=VECTOR ( 'NONE', #30803, 1000.000000000000227 ) ;
#29226=EDGE_LOOP ( 'NONE', ( #21900, #47742, #38980 ) ) ;
#29228=CARTESIAN_POINT ( 'NONE',  ( -12.64689790204744746, -0.1191753592594185784, 4.452657000069766724 ) ) ;
#29229=CARTESIAN_POINT ( 'NONE',  ( -18.67775241435682432, 0.000000000000000000, 4.136394454059623804 ) ) ;
#29230=ORIENTED_EDGE ( 'NONE', *, *, #40399, .F. ) ;
#29231=PLANE ( 'NONE',  #46365 ) ;
#29232=ORIENTED_EDGE ( 'NONE', *, *, #33888, .F. ) ;
#29233=CARTESIAN_POINT ( 'NONE',  ( 2.072287782118878319, 0.000000000000000000, -2.950529333540147015 ) ) ;
#29234=CARTESIAN_POINT ( 'NONE',  ( -16.99924723426068951, 0.000000000000000000, 13.49389102713827171 ) ) ;
#29235=ORIENTED_EDGE ( 'NONE', *, *, #9792, .F. ) ;
#29236=CARTESIAN_POINT ( 'NONE',  ( -17.74560456716937296, 0.000000000000000000, 3.774316574337878372 ) ) ;
#29237=EDGE_CURVE ( 'NONE', #50606, #25455, #6192, .T. ) ;
#29238=VECTOR ( 'NONE', #9524, 1000.000000000000000 ) ;
#29239=EDGE_CURVE ( 'NONE', #39009, #28807, #28582, .T. ) ;
#29240=LINE ( 'NONE', #49723, #52657 ) ;
#29241=VERTEX_POINT ( 'NONE', #54158 ) ;
#29242=PLANE ( 'NONE',  #6797 ) ;
#29243=DIRECTION ( 'NONE',  ( 0.9999697198139515519, 0.000000000000000000, 0.007781995580013368816 ) ) ;
#29244=AXIS2_PLACEMENT_3D ( 'NONE', #23084, #19084, #23376 ) ;
#29245=CARTESIAN_POINT ( 'NONE',  ( -14.94916102560700821, 0.000000000000000000, 2.688082935172642962 ) ) ;
#29246=ORIENTED_EDGE ( 'NONE', *, *, #32424, .T. ) ;
#29247=AXIS2_PLACEMENT_3D ( 'NONE', #19284, #1953, #36625 ) ;
#29248=EDGE_CURVE ( 'NONE', #36041, #17041, #40812, .T. ) ;
#29249=VECTOR ( 'NONE', #18671, 1000.000000000000227 ) ;
#29250=DIRECTION ( 'NONE',  ( 0.000000000000000000, -1.000000000000000000, 0.000000000000000000 ) ) ;
#29251=CARTESIAN_POINT ( 'NONE',  ( -12.60458797795435615, 0.000000000000000000, 11.86609696750642229 ) ) ;
#29252=LINE ( 'NONE', #51419, #10417 ) ;
#29253=LINE ( 'NONE', #33797, #38619 ) ;
#29254=PLANE ( 'NONE',  #48516 ) ;
#29255=DIRECTION ( 'NONE',  ( -0.5449076811759708816, 0.6444004775717707689, 0.5364919789714475140 ) ) ;
#29256=AXIS2_PLACEMENT_3D ( 'NONE', #4096, #26229, #43540 ) ;
#29257=CARTESIAN_POINT ( 'NONE',  ( -18.39746900504187010, 0.000000000000000000, 14.03700784672088808 ) ) ;
#29258=VECTOR ( 'NONE', #36901, 1000.000000000000227 ) ;
#29259=ORIENTED_EDGE ( 'NONE', *, *, #5132, .F. ) ;
#29260=LINE ( 'NONE', #37502, #23506 ) ;
#29261=PLANE ( 'NONE',  #34171 ) ;
#29262=EDGE_LOOP ( 'NONE', ( #26930, #20947, #19534, #1453 ) ) ;
#29263=LINE ( 'NONE', #6870, #11185 ) ;
#29264=CARTESIAN_POINT ( 'NONE',  ( -10.37421533196711465, -0.1191753592594197858, 10.96012406864405975 ) ) ;
#29265=DIRECTION ( 'NONE',  ( -0.9999697198139514409, -0.000000000000000000, -0.007781995580013368816 ) ) ;
#29266=AXIS2_PLACEMENT_3D ( 'NONE', #28336, #11596, #23532 ) ;
#29267=VECTOR ( 'NONE', #18847, 1000.000000000000114 ) ;
#29268=CARTESIAN_POINT ( 'NONE',  ( -30.79567442779373110, 0.000000000000000000, 8.843406890442315316 ) ) ;
#29269=LINE ( 'NONE', #29000, #52874 ) ;
#29270=ORIENTED_EDGE ( 'NONE', *, *, #2194, .T. ) ;
#29271=ORIENTED_EDGE ( 'NONE', *, *, #35746, .T. ) ;
#29272=PLANE ( 'NONE',  #35911 ) ;
#29273=CARTESIAN_POINT ( 'NONE',  ( -9.110551994824897193, -1.000000000000000000, 3.538847790438064411 ) ) ;
#29274=EDGE_CURVE ( 'NONE', #44937, #1477, #41377, .T. ) ;
#29275=VECTOR ( 'NONE', #38537, 1000.000000000000227 ) ;
#29276=FACE_OUTER_BOUND ( 'NONE', #7047, .T. ) ;
#29277=ORIENTED_EDGE ( 'NONE', *, *, #20451, .T. ) ;
#29278=CARTESIAN_POINT ( 'NONE',  ( -27.06708303904391144, 0.000000000000000000, 7.395095371555332697 ) ) ;
#29279=EDGE_CURVE ( 'NONE', #17736, #13096, #32571, .T. ) ;
#29280=VECTOR ( 'NONE', #15575, 999.9999999999998863 ) ;
#29281=ORIENTED_EDGE ( 'NONE', *, *, #28980, .F. ) ;
#29282=CARTESIAN_POINT ( 'NONE',  ( -11.55387398669053312, -2.137015261443158565, 4.677054874402827522 ) ) ;
#29284=VERTEX_POINT ( 'NONE', #36541 ) ;
#29285=VERTEX_POINT ( 'NONE', #54407 ) ;
#29286=EDGE_CURVE ( 'NONE', #41600, #50762, #14974, .T. ) ;
#29287=LINE ( 'NONE', #19671, #17558 ) ;
#29288=VECTOR ( 'NONE', #11418, 1000.000000000000227 ) ;
#29289=DIRECTION ( 'NONE',  ( 0.000000000000000000, -1.000000000000000000, 0.000000000000000000 ) ) ;
#29290=DIRECTION ( 'NONE',  ( -0.7660212471507179544, -0.6427876096865405842, -0.005961354470445141482 ) ) ;
#29291=EDGE_CURVE ( 'NONE', #20189, #54113, #32831, .T. ) ;
#29292=EDGE_CURVE ( 'NONE', #29930, #6164, #47584, .T. ) ;
#29293=ADVANCED_FACE ( 'NONE', ( #42204 ), #7554, .F. ) ;
#29294=VECTOR ( 'NONE', #13676, 1000.000000000000114 ) ;
#29295=AXIS2_PLACEMENT_3D ( 'NONE', #13899, #7471, #5397 ) ;
#29296=DIRECTION ( 'NONE',  ( 0.9999697198139515519, 0.000000000000000000, 0.007781995580013368816 ) ) ;
#29297=EDGE_LOOP ( 'NONE', ( #43356, #33410, #49834, #17285 ) ) ;
#29298=EDGE_CURVE ( 'NONE', #51007, #48125, #3310, .T. ) ;
#29299=ADVANCED_BREP_SHAPE_REPRESENTATION ( '', ( #3992, #2610 ), #48882 ) ;
#29300=ORIENTED_EDGE ( 'NONE', *, *, #34492, .T. ) ;
#29301=VECTOR ( 'NONE', #3170, 999.9999999999998863 ) ;
#29302=ORIENTED_EDGE ( 'NONE', *, *, #23423, .T. ) ;
#29303=DIRECTION ( 'NONE',  ( 0.5449076811759707706, 0.6444004775717708799, -0.5364919789714476250 ) ) ;
#29304=VECTOR ( 'NONE', #34716, 1000.000000000000227 ) ;
#29305=PLANE ( 'NONE',  #4988 ) ;
#29306=ORIENTED_EDGE ( 'NONE', *, *, #24418, .F. ) ;
#29307=DIRECTION ( 'NONE',  ( -0.005002170337468016433, -0.7660444431189770143, 0.6427681459581293666 ) ) ;
#29308=ORIENTED_EDGE ( 'NONE', *, *, #2735, .T. ) ;
#29309=FACE_OUTER_BOUND ( 'NONE', #42238, .T. ) ;
#29310=DIRECTION ( 'NONE',  ( -0.005961354470445682716, -0.6427876096865404731, 0.7660212471507180654 ) ) ;
#29311=VERTEX_POINT ( 'NONE', #34515 ) ;
#29312=DIRECTION ( 'NONE',  ( 0.007781995580012663651, 0.000000000000000000, -0.9999697198139515519 ) ) ;
#29313=VECTOR ( 'NONE', #7669, 1000.000000000000227 ) ;
#29314=EDGE_CURVE ( 'NONE', #41229, #26160, #12087, .T. ) ;
#29315=EDGE_LOOP ( 'NONE', ( #21941, #46766, #17731, #32193 ) ) ;
#29316=AXIS2_PLACEMENT_3D ( 'NONE', #31820, #4861, #1444 ) ;
#29317=ADVANCED_FACE ( 'NONE', ( #8705 ), #43045, .F. ) ;
#29318=CARTESIAN_POINT ( 'NONE',  ( -19.48141096923159665, 1.905425754524007198, 7.575691008948671978 ) ) ;
#29319=DIRECTION ( 'NONE',  ( 0.007781995580012663651, -3.146120232559066537E-19, -0.9999697198139514409 ) ) ;
#29320=ORIENTED_EDGE ( 'NONE', *, *, #19770, .T. ) ;
#29321=LINE ( 'NONE', #21376, #44047 ) ;
#29322=EDGE_CURVE ( 'NONE', #12293, #30283, #29731, .T. ) ;
#29323=CARTESIAN_POINT ( 'NONE',  ( 2.072287782118878319, 0.000000000000000000, -2.950529333540147015 ) ) ;
#29324=PLANE ( 'NONE',  #43676 ) ;
#29325=ORIENTED_EDGE ( 'NONE', *, *, #3309, .T. ) ;
#29326=VECTOR ( 'NONE', #43011, 1000.000000000000114 ) ;
#29327=ADVANCED_FACE ( 'NONE', ( #34801 ), #3847, .F. ) ;
#29328=ORIENTED_EDGE ( 'NONE', *, *, #9788, .F. ) ;
#29330=CARTESIAN_POINT ( 'NONE',  ( -9.808144436391993182, 0.000000000000000000, 10.77986332834118777 ) ) ;
#29331=VECTOR ( 'NONE', #10013, 1000.000000000000000 ) ;
#29332=LINE ( 'NONE', #50351, #5961 ) ;
#29333=LINE ( 'NONE', #19705, #16733 ) ;
#29334=EDGE_CURVE ( 'NONE', #24768, #36870, #20885, .T. ) ;
#29335=LINE ( 'NONE', #16266, #22470 ) ;
#29336=FACE_OUTER_BOUND ( 'NONE', #11285, .T. ) ;
#29337=ORIENTED_EDGE ( 'NONE', *, *, #31451, .F. ) ;
#29338=DIRECTION ( 'NONE',  ( -0.005002170337468016433, -0.7660444431189770143, 0.6427681459581293666 ) ) ;
#29339=CARTESIAN_POINT ( 'NONE',  ( 3.520599301005862269, 0.000000000000000000, 0.7780620552096689790 ) ) ;
#29340=ORIENTED_EDGE ( 'NONE', *, *, #47121, .F. ) ;
#29341=VECTOR ( 'NONE', #22607, 1000.000000000000227 ) ;
#29342=LINE ( 'NONE', #54904, #6880 ) ;
#29343=VERTEX_POINT ( 'NONE', #43342 ) ;
#29344=VECTOR ( 'NONE', #14035, 999.9999999999998863 ) ;
#29347=CARTESIAN_POINT ( 'NONE',  ( -14.99525971934085788, 3.200641362704007786, 7.958786984757082017 ) ) ;
#29348=LINE ( 'NONE', #22157, #21414 ) ;
#29351=VERTEX_POINT ( 'NONE', #33964 ) ;
#29352=AXIS2_PLACEMENT_3D ( 'NONE', #38016, #42282, #16416 ) ;
#29353=AXIS2_PLACEMENT_3D ( 'NONE', #13903, #40024, #23290 ) ;
#29354=EDGE_LOOP ( 'NONE', ( #11580, #54042, #5762, #52983 ) ) ;
#29355=CARTESIAN_POINT ( 'NONE',  ( -15.99883398164889847, 2.229229656569006401, 2.825298075309216284 ) ) ;
#29356=LINE ( 'NONE', #3516, #2274 ) ;
#29357=CARTESIAN_POINT ( 'NONE',  ( -1.086233639165236964, 0.000000000000000000, -2.796443541562362078 ) ) ;
#29358=LINE ( 'NONE', #50381, #35138 ) ;
#29359=DIRECTION ( 'NONE',  ( 0.007781995580012663651, 0.000000000000000000, -0.9999697198139515519 ) ) ;
#29360=CARTESIAN_POINT ( 'NONE',  ( -13.50126300573776739, 0.000000000000000000, 7.669993733430236382 ) ) ;
#29361=ORIENTED_EDGE ( 'NONE', *, *, #2698, .F. ) ;
#29362=LINE ( 'NONE', #21109, #14746 ) ;
#29363=DIRECTION ( 'NONE',  ( -0.005002170337468016433, -0.7660444431189770143, 0.6427681459581293666 ) ) ;
#29364=DIRECTION ( 'NONE',  ( 0.5364919789714477361, 0.6444004775717706579, 0.5449076811759711036 ) ) ;
#29365=ORIENTED_EDGE ( 'NONE', *, *, #54492, .F. ) ;
#29366=VECTOR ( 'NONE', #6088, 999.9999999999998863 ) ;
#29367=DIRECTION ( 'NONE',  ( 0.9999697198139515519, 0.000000000000000000, 0.007781995580013368816 ) ) ;
#29368=PLANE ( 'NONE',  #48570 ) ;
#29369=VECTOR ( 'NONE', #10485, 999.9999999999998863 ) ;
#29370=LINE ( 'NONE', #3794, #32937 ) ;
#29371=EDGE_CURVE ( 'NONE', #16343, #54122, #39060, .T. ) ;
#29372=EDGE_CURVE ( 'NONE', #30427, #34934, #38498, .T. ) ;
#29373=EDGE_LOOP ( 'NONE', ( #17274, #19746, #35818, #53938 ) ) ;
#29374=CARTESIAN_POINT ( 'NONE',  ( -14.01623497886155256, -0.1191753592594197858, 2.226008083469502630 ) ) ;
#29375=VECTOR ( 'NONE', #32559, 999.9999999999998863 ) ;
#29377=ADVANCED_FACE ( 'NONE', ( #29424 ), #20636, .F. ) ;
#29378=ORIENTED_EDGE ( 'NONE', *, *, #10065, .F. ) ;
#29379=VERTEX_POINT ( 'NONE', #47283 ) ;
#29380=EDGE_LOOP ( 'NONE', ( #54916, #29094, #39931, #5421 ) ) ;
#29381=VECTOR ( 'NONE', #7168, 1000.000000000000227 ) ;
#29382=LINE ( 'NONE', #37327, #48362 ) ;
#29383=ORIENTED_EDGE ( 'NONE', *, *, #19957, .F. ) ;
#29384=CARTESIAN_POINT ( 'NONE',  ( -8.140418508869350589, -9.937499621474987777, 6.380388574284866721 ) ) ;
#29385=VECTOR ( 'NONE', #29243, 999.9999999999998863 ) ;
#29386=ORIENTED_EDGE ( 'NONE', *, *, #14772, .T. ) ;
#29387=DIRECTION ( 'NONE',  ( 0.5449076811759707706, 0.6444004775717708799, -0.5364919789714476250 ) ) ;
#29388=ORIENTED_EDGE ( 'NONE', *, *, #4519, .F. ) ;
#29389=ORIENTED_EDGE ( 'NONE', *, *, #11525, .F. ) ;
#29390=VECTOR ( 'NONE', #14077, 1000.000000000000227 ) ;
#29391=VECTOR ( 'NONE', #37047, 999.9999999999998863 ) ;
#29392=LINE ( 'NONE', #35080, #29326 ) ;
#29393=LINE ( 'NONE', #37632, #368 ) ;
#29394=DIRECTION ( 'NONE',  ( -0.6427681459581293666, -0.7660444431189770143, -0.005002170337467561935 ) ) ;
#29395=DIRECTION ( 'NONE',  ( 0.005961354470445682716, -0.6427876096865404731, -0.7660212471507180654 ) ) ;
#29397=ORIENTED_EDGE ( 'NONE', *, *, #6963, .T. ) ;
#29398=ORIENTED_EDGE ( 'NONE', *, *, #25281, .F. ) ;
#29400=PLANE ( 'NONE',  #15778 ) ;
#29401=EDGE_CURVE ( 'NONE', #37529, #25528, #16633, .T. ) ;
#29402=DIRECTION ( 'NONE',  ( 0.007781995580012663651, 0.000000000000000000, -0.9999697198139515519 ) ) ;
#29403=AXIS2_PLACEMENT_3D ( 'NONE', #49851, #2436, #19758 ) ;
#29404=DIRECTION ( 'NONE',  ( 0.005002170337468016433, -0.7660444431189770143, -0.6427681459581293666 ) ) ;
#29405=VECTOR ( 'NONE', #12556, 999.9999999999998863 ) ;
#29406=EDGE_CURVE ( 'NONE', #30427, #2840, #24879, .T. ) ;
#29407=FACE_OUTER_BOUND ( 'NONE', #36931, .T. ) ;
#29408=LINE ( 'NONE', #43328, #10542 ) ;
#29409=ORIENTED_EDGE ( 'NONE', *, *, #14316, .T. ) ;
#29411=EDGE_CURVE ( 'NONE', #32655, #54876, #42488, .T. ) ;
#29413=VECTOR ( 'NONE', #47264, 999.9999999999998863 ) ;
#29414=ORIENTED_EDGE ( 'NONE', *, *, #45300, .F. ) ;
#29415=CARTESIAN_POINT ( 'NONE',  ( -13.08486533123210194, 0.000000000000000000, 1.963927175729152541 ) ) ;
#29416=FACE_OUTER_BOUND ( 'NONE', #23715, .T. ) ;
#29417=DIRECTION ( 'NONE',  ( 0.6427681459581294776, -0.7660444431189769032, 0.005002170337467562802 ) ) ;
#29418=EDGE_CURVE ( 'NONE', #53080, #51439, #3576, .T. ) ;
#29419=PLANE ( 'NONE',  #35940 ) ;
#29420=PLANE ( 'NONE',  #30465 ) ;
#29421=EDGE_LOOP ( 'NONE', ( #18190, #10245, #5740, #34413 ) ) ;
#29422=VERTEX_POINT ( 'NONE', #12402 ) ;
#29423=VECTOR ( 'NONE', #24678, 999.9999999999998863 ) ;
#29424=FACE_OUTER_BOUND ( 'NONE', #6053, .T. ) ;
#29425=PLANE ( 'NONE',  #54896 ) ;
#29426=CARTESIAN_POINT ( 'NONE',  ( -14.62478263637216180, 0.000000000000000000, 6.922586104262684614 ) ) ;
#29427=VECTOR ( 'NONE', #46646, 1000.000000000000227 ) ;
#29428=LINE ( 'NONE', #54687, #2843 ) ;
#29429=PLANE ( 'NONE',  #49370 ) ;
#29430=CARTESIAN_POINT ( 'NONE',  ( -7.547956548905578877, -7.259220043554206470, -0.2864909223855121034 ) ) ;
#29431=PLANE ( 'NONE',  #13851 ) ;
#29432=VECTOR ( 'NONE', #14367, 999.9999999999998863 ) ;
#29433=DIRECTION ( 'NONE',  ( 0.9999697198139515519, 0.000000000000000000, 0.007781995580013368816 ) ) ;
#29434=VECTOR ( 'NONE', #25117, 1000.000000000000000 ) ;
#29435=DIRECTION ( 'NONE',  ( -0.005961354470445682716, -0.6427876096865404731, 0.7660212471507180654 ) ) ;
#29436=DIRECTION ( 'NONE',  ( 0.005002170337468016433, -0.7660444431189770143, -0.6427681459581293666 ) ) ;
#29437=EDGE_LOOP ( 'NONE', ( #53605, #7808, #44361, #47773 ) ) ;
#29438=LINE ( 'NONE', #29744, #14126 ) ;
#29440=EDGE_LOOP ( 'NONE', ( #19311, #27726, #46286, #52035 ) ) ;
#29441=ORIENTED_EDGE ( 'NONE', *, *, #49205, .F. ) ;
#29442=EDGE_CURVE ( 'NONE', #5827, #43300, #16939, .T. ) ;
#29443=ADVANCED_FACE ( 'NONE', ( #52666 ), #23153, .F. ) ;
#29444=VECTOR ( 'NONE', #4497, 1000.000000000000227 ) ;
#29445=EDGE_LOOP ( 'NONE', ( #40708, #27629, #51576, #29818 ) ) ;
#29446=ORIENTED_EDGE ( 'NONE', *, *, #51446, .F. ) ;
#29447=EDGE_LOOP ( 'NONE', ( #39059, #10858, #55155, #15155 ) ) ;
#29448=AXIS2_PLACEMENT_3D ( 'NONE', #43164, #51095, #4270 ) ;
#29449=ORIENTED_EDGE ( 'NONE', *, *, #53243, .T. ) ;
#29450=CARTESIAN_POINT ( 'NONE',  ( -18.12044783821180260, 0.000000000000000000, 4.140731527135287138 ) ) ;
#29452=DIRECTION ( 'NONE',  ( 0.005961354470445682716, -0.6427876096865404731, -0.7660212471507180654 ) ) ;
#29453=VECTOR ( 'NONE', #46028, 1000.000000000000000 ) ;
#29454=ORIENTED_EDGE ( 'NONE', *, *, #8882, .F. ) ;
#29455=DIRECTION ( 'NONE',  ( -0.5449076811759708816, 0.6444004775717707689, 0.5364919789714475140 ) ) ;
#29456=VERTEX_POINT ( 'NONE', #35954 ) ;
#29459=VERTEX_POINT ( 'NONE', #40481 ) ;
#29460=EDGE_CURVE ( 'NONE', #24424, #52991, #724, .T. ) ;
#29461=VECTOR ( 'NONE', #6613, 999.9999999999998863 ) ;
#29462=VECTOR ( 'NONE', #17966, 1000.000000000000227 ) ;
#29464=AXIS2_PLACEMENT_3D ( 'NONE', #38690, #51715, #12825 ) ;
#29465=DIRECTION ( 'NONE',  ( 0.2426528472758541499, 0.7422098413412800966, 0.6246952433987894571 ) ) ;
#29467=ORIENTED_EDGE ( 'NONE', *, *, #6950, .F. ) ;
#29468=CARTESIAN_POINT ( 'NONE',  ( -10.27421835998572064, 0.000000000000000000, 10.96090226820206048 ) ) ;
#29469=EDGE_LOOP ( 'NONE', ( #42388, #15425, #24142, #47926 ) ) ;
#29470=VECTOR ( 'NONE', #13618, 1000.000000000000114 ) ;
#29471=CARTESIAN_POINT ( 'NONE',  ( -13.92222681985565202, -5.536956232915666298, 2.112528921847934615 ) ) ;
#29472=DIRECTION ( 'NONE',  ( 0.6427681459581294776, -0.7660444431189769032, 0.005002170337467562802 ) ) ;
#29473=VECTOR ( 'NONE', #7490, 999.9999999999998863 ) ;
#29474=DIRECTION ( 'NONE',  ( -0.005002170337468016433, -0.7660444431189770143, 0.6427681459581293666 ) ) ;
#29475=AXIS2_PLACEMENT_3D ( 'NONE', #25167, #50702, #42473 ) ;
#29476=LINE ( 'NONE', #46485, #35879 ) ;
#29477=DIRECTION ( 'NONE',  ( 0.000000000000000000, -1.000000000000000000, 0.000000000000000000 ) ) ;
#29478=LINE ( 'NONE', #25228, #38501 ) ;
#29479=LINE ( 'NONE', #11851, #27504 ) ;
#29481=EDGE_LOOP ( 'NONE', ( #17997, #5377, #6852, #29325 ) ) ;
#29482=DIRECTION ( 'NONE',  ( 0.000000000000000000, -0.000000000000000000, -1.000000000000000000 ) ) ;
#29483=ORIENTED_EDGE ( 'NONE', *, *, #10651, .T. ) ;
#29484=CARTESIAN_POINT ( 'NONE',  ( -17.89735928879674631, 0.000000000000000000, 9.482442644690969757 ) ) ;
#29485=CARTESIAN_POINT ( 'NONE',  ( -28.93137873341882127, 0.000000000000000000, 8.119251130998824451 ) ) ;
#29486=LINE ( 'NONE', #11316, #11420 ) ;
#29487=EDGE_CURVE ( 'NONE', #5703, #33009, #22853, .T. ) ;
#29488=DIRECTION ( 'NONE',  ( 0.5364919789714477361, 0.6444004775717706579, 0.5449076811759711036 ) ) ;
#29489=DIRECTION ( 'NONE',  ( 0.5364919789714477361, 0.6444004775717706579, 0.5449076811759711036 ) ) ;
#29490=VECTOR ( 'NONE', #24267, 999.9999999999998863 ) ;
#29491=CARTESIAN_POINT ( 'NONE',  ( -16.79925329029790149, 0.000000000000000000, 13.49544742625427496 ) ) ;
#29493=VECTOR ( 'NONE', #35681, 1000.000000000000114 ) ;
#29494=ORIENTED_EDGE ( 'NONE', *, *, #21110, .F. ) ;
#29497=DIRECTION ( 'NONE',  ( 0.9999697198139515519, 0.000000000000000000, 0.007781995580013368816 ) ) ;
#29498=CARTESIAN_POINT ( 'NONE',  ( -13.83644591565411375, -1.003701604285657911, 2.223843262371220320 ) ) ;
#29499=AXIS2_PLACEMENT_3D ( 'NONE', #42477, #32366, #45137 ) ;
#29500=ADVANCED_FACE ( 'NONE', ( #17778 ), #47875, .F. ) ;
#29501=LINE ( 'NONE', #2780, #9196 ) ;
#29502=VECTOR ( 'NONE', #41813, 999.9999999999998863 ) ;
#29503=DIRECTION ( 'NONE',  ( -0.6427681459581293666, -0.7660444431189770143, -0.005002170337467561935 ) ) ;
#29504=ADVANCED_FACE ( 'NONE', ( #9820 ), #44431, .F. ) ;
#29505=FACE_OUTER_BOUND ( 'NONE', #16238, .T. ) ;
#29506=EDGE_CURVE ( 'NONE', #28751, #9630, #9230, .T. ) ;
#29507=LINE ( 'NONE', #38581, #9312 ) ;
#29508=ORIENTED_EDGE ( 'NONE', *, *, #46961, .F. ) ;
#29509=DIRECTION ( 'NONE',  ( 0.5449076811759707706, 0.6444004775717708799, -0.5364919789714476250 ) ) ;
#29510=VECTOR ( 'NONE', #9131, 999.9999999999998863 ) ;
#29511=DIRECTION ( 'NONE',  ( 0.5364919789714477361, 0.6444004775717706579, 0.5449076811759711036 ) ) ;
#29512=VECTOR ( 'NONE', #54310, 1000.000000000000000 ) ;
#29513=VERTEX_POINT ( 'NONE', #39343 ) ;
#29514=VECTOR ( 'NONE', #29265, 1000.000000000000227 ) ;
#29515=ORIENTED_EDGE ( 'NONE', *, *, #3314, .T. ) ;
#29516=CARTESIAN_POINT ( 'NONE',  ( -11.07315700445993478, 0.000000000000000000, 7.519563802190774027 ) ) ;
#29517=ADVANCED_FACE ( 'NONE', ( #52119 ), #979, .F. ) ;
#29518=AXIS2_PLACEMENT_3D ( 'NONE', #2161, #53851, #10969 ) ;
#29519=ORIENTED_EDGE ( 'NONE', *, *, #27019, .F. ) ;
#29520=AXIS2_PLACEMENT_3D ( 'NONE', #29615, #8020, #21049 ) ;
#29521=EDGE_CURVE ( 'NONE', #25319, #41949, #13236, .T. ) ;
#29522=LINE ( 'NONE', #33490, #1194 ) ;
#29523=ADVANCED_FACE ( 'NONE', ( #52956 ), #14072, .F. ) ;
#29524=VECTOR ( 'NONE', #4569, 1000.000000000000227 ) ;
#29525=EDGE_LOOP ( 'NONE', ( #6038, #36565, #35910, #49198 ) ) ;
#29526=VECTOR ( 'NONE', #36389, 1000.000000000000000 ) ;
#29527=ORIENTED_EDGE ( 'NONE', *, *, #37514, .F. ) ;
#29528=VERTEX_POINT ( 'NONE', #44175 ) ;
#29529=PLANE ( 'NONE',  #40257 ) ;
#29530=CARTESIAN_POINT ( 'NONE',  ( -16.40135577234480735, -0.1191753592594181482, 9.224755848276627646 ) ) ;
#29531=CARTESIAN_POINT ( 'NONE',  ( -19.44046948079687454, 4.657758921906512306, 4.084663383300955353 ) ) ;
#29532=EDGE_CURVE ( 'NONE', #11534, #28953, #22017, .T. ) ;
#29533=EDGE_LOOP ( 'NONE', ( #39672, #23002, #31814, #49434 ) ) ;
#29534=EDGE_LOOP ( 'NONE', ( #29259, #46247, #26802 ) ) ;
#29535=VECTOR ( 'NONE', #13634, 1000.000000000000227 ) ;
#29536=EDGE_CURVE ( 'NONE', #485, #53740, #18605, .T. ) ;
#29537=PLANE ( 'NONE',  #4892 ) ;
#29538=LINE ( 'NONE', #7367, #35459 ) ;
#29539=VECTOR ( 'NONE', #33630, 999.9999999999998863 ) ;
#29540=ORIENTED_EDGE ( 'NONE', *, *, #45979, .T. ) ;
#29541=CARTESIAN_POINT ( 'NONE',  ( -15.24161218666607809, -4.889348428825665671, 2.645685084382324970 ) ) ;
#29542=CARTESIAN_POINT ( 'NONE',  ( -10.19862816387108140, 0.000000000000000000, 1.247724401129331806 ) ) ;
#29543=VERTEX_POINT ( 'NONE', #14362 ) ;
#29544=VECTOR ( 'NONE', #7207, 999.9999999999998863 ) ;
#29545=DIRECTION ( 'NONE',  ( 0.7660212471507180654, -0.6427876096865404731, 0.005961354470445141482 ) ) ;
#29546=CARTESIAN_POINT ( 'NONE',  ( -12.29297599165088783, 0.000000000000000000, 5.832736553329440632 ) ) ;
#29548=CARTESIAN_POINT ( 'NONE',  ( -14.67944861483846708, 2.876837460659008361, 2.292141912774824153 ) ) ;
#29549=VECTOR ( 'NONE', #14810, 999.9999999999998863 ) ;
#29550=CARTESIAN_POINT ( 'NONE',  ( -21.25413238913553471, -1.489407457353157049, 7.382129924272583743 ) ) ;
#29552=VECTOR ( 'NONE', #41852, 1000.000000000000227 ) ;
#29553=ORIENTED_EDGE ( 'NONE', *, *, #18873, .F. ) ;
#29554=FACE_OUTER_BOUND ( 'NONE', #50269, .T. ) ;
#29555=FACE_OUTER_BOUND ( 'NONE', #38561, .T. ) ;
#29556=LINE ( 'NONE', #34624, #44792 ) ;
#29557=DIRECTION ( 'NONE',  ( 0.007781995580012662783, 0.000000000000000000, -0.9999697198139514409 ) ) ;
#29558=EDGE_LOOP ( 'NONE', ( #23777, #34513, #1034, #42676 ) ) ;
#29559=VECTOR ( 'NONE', #55821, 999.9999999999998863 ) ;
#29560=AXIS2_PLACEMENT_3D ( 'NONE', #11530, #28266, #49600 ) ;
#29561=DIRECTION ( 'NONE',  ( -0.9999697198139514409, -0.000000000000000000, -0.007781995580013368816 ) ) ;
#29562=DIRECTION ( 'NONE',  ( 0.6246952433987893460, 0.7422098413412802076, -0.2426528472758539279 ) ) ;
#29563=LINE ( 'NONE', #51947, #38487 ) ;
#29564=VECTOR ( 'NONE', #7219, 1000.000000000000227 ) ;
#29565=EDGE_CURVE ( 'NONE', #6357, #34966, #48978, .T. ) ;
#29566=LINE ( 'NONE', #42337, #13258 ) ;
#29567=CARTESIAN_POINT ( 'NONE',  ( -13.49132319083263987, 0.000000000000000000, 6.392748864361969652 ) ) ;
#29568=DIRECTION ( 'NONE',  ( -0.5364919789714478471, 0.6444004775717705469, -0.5449076811759709926 ) ) ;
#29569=AXIS2_PLACEMENT_3D ( 'NONE', #36487, #2110, #54360 ) ;
#29570=VECTOR ( 'NONE', #26547, 999.9999999999998863 ) ;
#29571=CARTESIAN_POINT ( 'NONE',  ( -13.93871576664203182, 0.000000000000000000, 4.173274733047372287 ) ) ;
#29572=VERTEX_POINT ( 'NONE', #432 ) ;
#29574=CARTESIAN_POINT ( 'NONE',  ( -13.86960054602229953, 0.000000000000000000, 8.605797441356008548 ) ) ;
#29575=ORIENTED_EDGE ( 'NONE', *, *, #20247, .T. ) ;
#29576=FACE_OUTER_BOUND ( 'NONE', #11004, .T. ) ;
#29577=DIRECTION ( 'NONE',  ( 0.000000000000000000, -0.000000000000000000, -1.000000000000000000 ) ) ;
#29578=DIRECTION ( 'NONE',  ( 0.007781995580012663651, -3.146120232559066537E-19, -0.9999697198139514409 ) ) ;
#29579=DIRECTION ( 'NONE',  ( 0.007781995580012663651, -3.146120232559066537E-19, -0.9999697198139514409 ) ) ;
#29580=EDGE_CURVE ( 'NONE', #49166, #24915, #10077, .T. ) ;
#29582=VECTOR ( 'NONE', #51223, 999.9999999999998863 ) ;
#29583=ORIENTED_EDGE ( 'NONE', *, *, #40021, .F. ) ;
#29584=ORIENTED_EDGE ( 'NONE', *, *, #135, .F. ) ;
#29585=DIRECTION ( 'NONE',  ( -0.5364919789714478471, 0.6444004775717705469, -0.5449076811759709926 ) ) ;
#29587=ORIENTED_EDGE ( 'NONE', *, *, #34237, .F. ) ;
#29588=VECTOR ( 'NONE', #30554, 1000.000000000000114 ) ;
#29589=CARTESIAN_POINT ( 'NONE',  ( -14.51694170343292178, -0.1191753592594181482, 5.915432166028785410 ) ) ;
#29590=ORIENTED_EDGE ( 'NONE', *, *, #2163, .T. ) ;
#29591=EDGE_CURVE ( 'NONE', #23572, #36955, #43875, .T. ) ;
#29592=LINE ( 'NONE', #37240, #5042 ) ;
#29593=VECTOR ( 'NONE', #27829, 1000.000000000000227 ) ;
#29594=ORIENTED_EDGE ( 'NONE', *, *, #45485, .F. ) ;
#29595=CARTESIAN_POINT ( 'NONE',  ( -17.46532115785441519, 0.000000000000000000, 13.67492996699914265 ) ) ;
#29596=EDGE_CURVE ( 'NONE', #55560, #2, #4989, .T. ) ;
#29597=VECTOR ( 'NONE', #45968, 999.9999999999998863 ) ;
#29598=VECTOR ( 'NONE', #12637, 999.9999999999998863 ) ;
#29599=ORIENTED_EDGE ( 'NONE', *, *, #38878, .F. ) ;
#29600=ORIENTED_EDGE ( 'NONE', *, *, #9461, .F. ) ;
#29601=ORIENTED_EDGE ( 'NONE', *, *, #26172, .T. ) ;
#29602=DIRECTION ( 'NONE',  ( 0.007781995580012663651, 0.000000000000000000, -0.9999697198139515519 ) ) ;
#29603=PLANE ( 'NONE',  #39587 ) ;
#29604=LINE ( 'NONE', #42629, #53855 ) ;
#29606=EDGE_CURVE ( 'NONE', #41331, #34820, #48415, .T. ) ;
#29607=AXIS2_PLACEMENT_3D ( 'NONE', #54965, #33637, #20863 ) ;
#29608=CARTESIAN_POINT ( 'NONE',  ( -20.54049170961573267, 0.000000000000000000, 4.660556269540326646 ) ) ;
#29609=VERTEX_POINT ( 'NONE', #19722 ) ;
#29610=VECTOR ( 'NONE', #29016, 999.9999999999998863 ) ;
#29611=ORIENTED_EDGE ( 'NONE', *, *, #11801, .F. ) ;
#29612=ADVANCED_FACE ( 'NONE', ( #54607 ), #24517, .F. ) ;
#29613=AXIS2_PLACEMENT_3D ( 'NONE', #19718, #20256, #19975 ) ;
#29614=ORIENTED_EDGE ( 'NONE', *, *, #51878, .F. ) ;
#29615=CARTESIAN_POINT ( 'NONE',  ( -11.67244013076689946, 0.000000000000000000, 11.50401908778467863 ) ) ;
#29616=CARTESIAN_POINT ( 'NONE',  ( -22.40556560354864146, -0.1191753592594197858, 5.484709000965211523 ) ) ;
#29617=EDGE_LOOP ( 'NONE', ( #45363, #56204, #19080, #21515 ) ) ;
#29618=CARTESIAN_POINT ( 'NONE',  ( 2.072287782118878319, 0.000000000000000000, -2.950529333540147015 ) ) ;
#29619=EDGE_LOOP ( 'NONE', ( #27728, #37934, #43221, #11906, #9321 ) ) ;
#29620=DIRECTION ( 'NONE',  ( -0.5449076811759708816, 0.6444004775717707689, 0.5364919789714475140 ) ) ;
#29621=CARTESIAN_POINT ( 'NONE',  ( 2.072287782118878319, 0.000000000000000000, -2.950529333540147015 ) ) ;
#29622=ORIENTED_EDGE ( 'NONE', *, *, #34451, .F. ) ;
#29623=PLANE ( 'NONE',  #44006 ) ;
#29624=ORIENTED_EDGE ( 'NONE', *, *, #56114, .F. ) ;
#29625=AXIS2_PLACEMENT_3D ( 'NONE', #47414, #51674, #21005 ) ;
#29626=LINE ( 'NONE', #30161, #972 ) ;
#29627=CARTESIAN_POINT ( 'NONE',  ( 1.086233639165236964, 0.000000000000000000, 2.796443541562362078 ) ) ;
#29628=ORIENTED_EDGE ( 'NONE', *, *, #30079, .T. ) ;
#29629=LINE ( 'NONE', #38706, #12325 ) ;
#29630=PLANE ( 'NONE',  #301 ) ;
#29631=DIRECTION ( 'NONE',  ( 0.9999697198139515519, 0.000000000000000000, 0.007781995580013368816 ) ) ;
#29632=DIRECTION ( 'NONE',  ( -0.7660212471507179544, -0.6427876096865405842, -0.005961354470445141482 ) ) ;
#29633=VECTOR ( 'NONE', #48248, 1000.000000000000000 ) ;
#29634=ORIENTED_EDGE ( 'NONE', *, *, #32325, .T. ) ;
#29635=ADVANCED_FACE ( 'NONE', ( #2094 ), #37298, .F. ) ;
#29636=ORIENTED_EDGE ( 'NONE', *, *, #16339, .T. ) ;
#29637=CARTESIAN_POINT ( 'NONE',  ( -17.22123223397174030, 0.000000000000000000, 8.010376142543925937 ) ) ;
#29638=VECTOR ( 'NONE', #5473, 1000.000000000000227 ) ;
#29639=LINE ( 'NONE', #46944, #26727 ) ;
#29640=EDGE_CURVE ( 'NONE', #50295, #44275, #6657, .T. ) ;
#29641=DIRECTION ( 'NONE',  ( -0.5449076811759708816, 0.6444004775717707689, 0.5364919789714475140 ) ) ;
#29642=FACE_OUTER_BOUND ( 'NONE', #5996, .T. ) ;
#29643=DIRECTION ( 'NONE',  ( -0.6427681459581293666, -0.7660444431189770143, -0.005002170337467561935 ) ) ;
#29644=AXIS2_PLACEMENT_3D ( 'NONE', #3060, #16401, #8184 ) ;
#29645=EDGE_CURVE ( 'NONE', #24756, #1435, #7216, .T. ) ;
#29646=PLANE ( 'NONE',  #23150 ) ;
#29647=ORIENTED_EDGE ( 'NONE', *, *, #26524, .F. ) ;
#29648=EDGE_CURVE ( 'NONE', #40648, #42565, #2924, .T. ) ;
#29649=CARTESIAN_POINT ( 'NONE',  ( -21.63461151687438999, 4.495856970884011261, 4.942108183378046249 ) ) ;
#29650=LINE ( 'NONE', #3766, #14187 ) ;
#29651=EDGE_LOOP ( 'NONE', ( #15439, #7704, #51645, #47074, #48447 ) ) ;
#29652=DIRECTION ( 'NONE',  ( 0.9999697198139515519, 0.000000000000000000, 0.007781995580013368816 ) ) ;
#29653=ORIENTED_EDGE ( 'NONE', *, *, #38954, .T. ) ;
#29654=EDGE_CURVE ( 'NONE', #1287, #46991, #15440, .T. ) ;
#29655=ADVANCED_FACE ( 'NONE', ( #36214 ), #27693, .F. ) ;
#29656=EDGE_CURVE ( 'NONE', #12179, #28185, #27974, .T. ) ;
#29657=FACE_OUTER_BOUND ( 'NONE', #19477, .T. ) ;
#29658=DIRECTION ( 'NONE',  ( 0.9999697198139515519, 0.000000000000000000, 0.007781995580013368816 ) ) ;
#29659=VECTOR ( 'NONE', #47336, 1000.000000000000227 ) ;
#29661=FACE_OUTER_BOUND ( 'NONE', #30766, .T. ) ;
#29662=AXIS2_PLACEMENT_3D ( 'NONE', #28959, #30366, #30901 ) ;
#29665=AXIS2_PLACEMENT_3D ( 'NONE', #29268, #3149, #45749 ) ;
#29666=ORIENTED_EDGE ( 'NONE', *, *, #18011, .T. ) ;
#29667=CARTESIAN_POINT ( 'NONE',  ( -9.949673132908477768, 0.000000000000000000, 3.265648189365135234 ) ) ;
#29668=CARTESIAN_POINT ( 'NONE',  ( -10.47421230394850866, 0.000000000000000000, 10.95934586908605723 ) ) ;
#29669=CARTESIAN_POINT ( 'NONE',  ( -12.52887840947635745, 0.000000000000000000, 2.137580008099788209 ) ) ;
#29670=DIRECTION ( 'NONE',  ( 0.000000000000000000, -1.000000000000000000, 0.000000000000000000 ) ) ;
#29671=DIRECTION ( 'NONE',  ( -0.005002170337468016433, -0.7660444431189770143, 0.6427681459581293666 ) ) ;
#29672=EDGE_CURVE ( 'NONE', #16268, #46898, #32234, .T. ) ;
#29673=DIRECTION ( 'NONE',  ( -0.005961354470445682716, -0.6427876096865404731, 0.7660212471507180654 ) ) ;
#29674=VERTEX_POINT ( 'NONE', #11487 ) ;
#29675=CARTESIAN_POINT ( 'NONE',  ( -17.39535969638698276, 0.000000000000000000, 4.685032414108041721 ) ) ;
#29676=AXIS2_PLACEMENT_3D ( 'NONE', #1454, #47774, #30976 ) ;
#29677=EDGE_CURVE ( 'NONE', #41065, #25334, #15197, .T. ) ;
#29678=CARTESIAN_POINT ( 'NONE',  ( -18.16819014657557574, 0.000000000000000000, 10.27551562292821963 ) ) ;
#29679=CARTESIAN_POINT ( 'NONE',  ( -17.73140113748535285, 0.000000000000000000, 13.85752530597602039 ) ) ;
#29680=ORIENTED_EDGE ( 'NONE', *, *, #16450, .T. ) ;
#29681=EDGE_CURVE ( 'NONE', #54483, #46200, #40751, .T. ) ;
#29682=DIRECTION ( 'NONE',  ( 0.9999697198139515519, 0.000000000000000000, 0.007781995580013368816 ) ) ;
#29683=DIRECTION ( 'NONE',  ( 0.9999697198139515519, 0.000000000000000000, 0.007781995580013368816 ) ) ;
#29684=CARTESIAN_POINT ( 'NONE',  ( -16.33317936670417225, 0.000000000000000000, 13.31440848639340224 ) ) ;
#29685=ORIENTED_EDGE ( 'NONE', *, *, #52157, .F. ) ;
#29686=EDGE_CURVE ( 'NONE', #41830, #55275, #50072, .T. ) ;
#29687=CARTESIAN_POINT ( 'NONE',  ( -17.74560456716937296, 0.000000000000000000, 3.774316574337878372 ) ) ;
#29688=VECTOR ( 'NONE', #6141, 999.9999999999998863 ) ;
#29689=ORIENTED_EDGE ( 'NONE', *, *, #27315, .T. ) ;
#29690=ORIENTED_EDGE ( 'NONE', *, *, #26736, .T. ) ;
#29691=VECTOR ( 'NONE', #51205, 999.9999999999998863 ) ;
#29692=VERTEX_POINT ( 'NONE', #41574 ) ;
#29693=ORIENTED_EDGE ( 'NONE', *, *, #718, .T. ) ;
#29694=LINE ( 'NONE', #46987, #324 ) ;
#29695=ORIENTED_EDGE ( 'NONE', *, *, #40018, .F. ) ;
#29696=CARTESIAN_POINT ( 'NONE',  ( -12.80458192191714595, 0.000000000000000000, 11.86454056839041726 ) ) ;
#29697=AXIS2_PLACEMENT_3D ( 'NONE', #2372, #28790, #36746 ) ;
#29698=ORIENTED_EDGE ( 'NONE', *, *, #6218, .F. ) ;
#29700=ORIENTED_EDGE ( 'NONE', *, *, #25780, .T. ) ;
#29701=ORIENTED_EDGE ( 'NONE', *, *, #36719, .F. ) ;
#29702=LINE ( 'NONE', #56087, #3002 ) ;
#29703=LINE ( 'NONE', #25409, #43173 ) ;
#29704=DIRECTION ( 'NONE',  ( -0.5449076811759708816, 0.6444004775717707689, 0.5364919789714475140 ) ) ;
#29705=LINE ( 'NONE', #33389, #37788 ) ;
#29706=EDGE_LOOP ( 'NONE', ( #31673, #53599, #54243, #24021 ) ) ;
#29707=VERTEX_POINT ( 'NONE', #54348 ) ;
#29709=CARTESIAN_POINT ( 'NONE',  ( -26.13337879274045505, 0.000000000000000000, 6.833023547870798353 ) ) ;
#29711=LINE ( 'NONE', #25165, #20639 ) ;
#29712=PLANE ( 'NONE',  #4184 ) ;
#29713=CARTESIAN_POINT ( 'NONE',  ( -14.94916102560700821, 0.000000000000000000, 2.688082935172642962 ) ) ;
#29714=DIRECTION ( 'NONE',  ( 0.007781995580012663651, -3.146120232559066537E-19, -0.9999697198139514409 ) ) ;
#29715=EDGE_LOOP ( 'NONE', ( #23455, #22948, #17216, #4017 ) ) ;
#29716=CARTESIAN_POINT ( 'NONE',  ( -13.13740128043607669, -0.1191753592594177180, 7.772828417621633790 ) ) ;
#29717=LINE ( 'NONE', #53630, #15862 ) ;
#29718=ORIENTED_EDGE ( 'NONE', *, *, #36324, .T. ) ;
#29719=EDGE_CURVE ( 'NONE', #27017, #54363, #1817, .T. ) ;
#29720=EDGE_CURVE ( 'NONE', #21115, #37239, #6385, .T. ) ;
#29721=DIRECTION ( 'NONE',  ( 0.007781995580012663651, -3.146120232559066537E-19, -0.9999697198139514409 ) ) ;
#29722=DIRECTION ( 'NONE',  ( 0.9999697198139515519, 0.000000000000000000, 0.007781995580013368816 ) ) ;
#29723=FACE_OUTER_BOUND ( 'NONE', #52066, .T. ) ;
#29724=FACE_OUTER_BOUND ( 'NONE', #20479, .T. ) ;
#29725=ADVANCED_FACE ( 'NONE', ( #2657 ), #31935, .F. ) ;
#29726=DIRECTION ( 'NONE',  ( -0.005002170337468016433, -0.7660444431189770143, 0.6427681459581293666 ) ) ;
#29727=VECTOR ( 'NONE', #43047, 999.9999999999998863 ) ;
#29728=VERTEX_POINT ( 'NONE', #45020 ) ;
#29730=ORIENTED_EDGE ( 'NONE', *, *, #28128, .T. ) ;
#29731=LINE ( 'NONE', #46744, #48445 ) ;
#29732=FACE_OUTER_BOUND ( 'NONE', #23841, .T. ) ;
#29734=VECTOR ( 'NONE', #4607, 1000.000000000000227 ) ;
#29736=CARTESIAN_POINT ( 'NONE',  ( -15.64335043210865450, -1.489407457353158160, 2.910209779635662741 ) ) ;
#29737=CARTESIAN_POINT ( 'NONE',  ( -16.81190032086591302, 0.000000000000000000, 3.212244750653343583 ) ) ;
#29738=CARTESIAN_POINT ( 'NONE',  ( -10.27421835998572064, 0.000000000000000000, 10.96090226820206048 ) ) ;
#29739=DIRECTION ( 'NONE',  ( 0.005961354470445682716, -0.6427876096865404731, -0.7660212471507180654 ) ) ;
#29741=EDGE_CURVE ( 'NONE', #11699, #32747, #54088, .T. ) ;
#29742=PLANE ( 'NONE',  #21065 ) ;
#29743=EDGE_LOOP ( 'NONE', ( #55888, #26039, #10143, #29527 ) ) ;
#29744=CARTESIAN_POINT ( 'NONE',  ( -11.77243710274829525, -0.1191753592594197858, 11.50324088822667612 ) ) ;
#29745=ORIENTED_EDGE ( 'NONE', *, *, #276, .T. ) ;
#29747=EDGE_LOOP ( 'NONE', ( #4173, #815, #18445, #48617 ) ) ;
#29748=EDGE_CURVE ( 'NONE', #41698, #17269, #38737, .T. ) ;
#29749=EDGE_LOOP ( 'NONE', ( #50046, #11065, #48106, #22609 ) ) ;
#29751=ORIENTED_EDGE ( 'NONE', *, *, #18939, .T. ) ;
#29752=ORIENTED_EDGE ( 'NONE', *, *, #19920, .F. ) ;
#29753=CARTESIAN_POINT ( 'NONE',  ( -18.86354292863559579, 0.000000000000000000, 14.21804678658176080 ) ) ;
#29754=DIRECTION ( 'NONE',  ( -0.5364919789714478471, 0.6444004775717705469, -0.5449076811759709926 ) ) ;
#29755=DIRECTION ( 'NONE',  ( 0.9999697198139515519, 0.000000000000000000, 0.007781995580013368816 ) ) ;
#29756=ORIENTED_EDGE ( 'NONE', *, *, #30217, .F. ) ;
#29757=DIRECTION ( 'NONE',  ( 0.007781995580012663651, -3.146120232559066537E-19, -0.9999697198139514409 ) ) ;
#29758=ORIENTED_EDGE ( 'NONE', *, *, #43366, .T. ) ;
#29759=DIRECTION ( 'NONE',  ( 0.005002170337468016433, -0.7660444431189770143, -0.6427681459581293666 ) ) ;
#29760=ORIENTED_EDGE ( 'NONE', *, *, #16499, .T. ) ;
#29761=CARTESIAN_POINT ( 'NONE',  ( -17.93139508144814442, 0.000000000000000000, 13.85596890686001537 ) ) ;
#29762=CARTESIAN_POINT ( 'NONE',  ( -15.35693653959682692, 0.000000000000000000, 7.286220383100434184 ) ) ;
#29763=LINE ( 'NONE', #47059, #12336 ) ;
#29764=VERTEX_POINT ( 'NONE', #42425 ) ;
#29765=PLANE ( 'NONE',  #26474 ) ;
#29766=EDGE_LOOP ( 'NONE', ( #55017, #12602, #47435, #18706 ) ) ;
#29768=PLANE ( 'NONE',  #40967 ) ;
#29769=DIRECTION ( 'NONE',  ( 0.5364919789714477361, 0.6444004775717706579, 0.5449076811759711036 ) ) ;
#29771=DIRECTION ( 'NONE',  ( -0.5449076811759708816, 0.6444004775717707689, 0.5364919789714475140 ) ) ;
#29772=DIRECTION ( 'NONE',  ( -0.005002170337468016433, -0.7660444431189770143, 0.6427681459581293666 ) ) ;
#29773=DIRECTION ( 'NONE',  ( 0.007781995580012663651, 0.000000000000000000, -0.9999697198139515519 ) ) ;
#29774=CARTESIAN_POINT ( 'NONE',  ( -14.69598771881120136, 0.000000000000000000, 2.490047132166154586 ) ) ;
#29776=ORIENTED_EDGE ( 'NONE', *, *, #26404, .F. ) ;
#29777=CARTESIAN_POINT ( 'NONE',  ( 2.072287782118878319, 0.000000000000000000, -2.950529333540147015 ) ) ;
#29778=VERTEX_POINT ( 'NONE', #29667 ) ;
#29779=EDGE_CURVE ( 'NONE', #12044, #35264, #24809, .T. ) ;
#29780=DIRECTION ( 'NONE',  ( -0.7660212471507179544, -0.6427876096865405842, -0.005961354470445141482 ) ) ;
#29781=FACE_OUTER_BOUND ( 'NONE', #49841, .T. ) ;
#29782=DIRECTION ( 'NONE',  ( 0.007781995580012663651, 0.000000000000000000, -0.9999697198139515519 ) ) ;
#29783=CARTESIAN_POINT ( 'NONE',  ( -22.40634380310664397, 0.000000000000000000, 5.584705972946605534 ) ) ;
#29784=FACE_OUTER_BOUND ( 'NONE', #3250, .T. ) ;
#29785=EDGE_CURVE ( 'NONE', #39202, #2126, #47219, .T. ) ;
#29786=EDGE_CURVE ( 'NONE', #23249, #17775, #16282, .T. ) ;
#29787=CARTESIAN_POINT ( 'NONE',  ( -10.47421230394850866, 0.000000000000000000, 10.95934586908605723 ) ) ;
#29788=ORIENTED_EDGE ( 'NONE', *, *, #6136, .F. ) ;
#29789=DIRECTION ( 'NONE',  ( 0.5449076811759707706, 0.6444004775717708799, -0.5364919789714476250 ) ) ;
#29790=DIRECTION ( 'NONE',  ( -0.005002170337468016433, -0.7660444431189770143, 0.6427681459581293666 ) ) ;
#29791=CARTESIAN_POINT ( 'NONE',  ( -18.35337402512197968, 0.000000000000000000, 8.370897623149668121 ) ) ;
#29793=FACE_OUTER_BOUND ( 'NONE', #8149, .T. ) ;
#29794=FACE_OUTER_BOUND ( 'NONE', #41172, .T. ) ;
#29796=ORIENTED_EDGE ( 'NONE', *, *, #29125, .T. ) ;
#29797=LINE ( 'NONE', #42823, #36694 ) ;
#29798=DIRECTION ( 'NONE',  ( 0.9999697198139515519, 0.000000000000000000, 0.007781995580013368816 ) ) ;
#29799=ORIENTED_EDGE ( 'NONE', *, *, #49719, .F. ) ;
#29800=ORIENTED_EDGE ( 'NONE', *, *, #46440, .F. ) ;
#29801=CARTESIAN_POINT ( 'NONE',  ( -20.54126990917373519, -0.1191753592594197858, 4.760553241521720658 ) ) ;
#29802=VECTOR ( 'NONE', #16471, 999.9999999999998863 ) ;
#29803=ORIENTED_EDGE ( 'NONE', *, *, #48909, .F. ) ;
#29804=ADVANCED_FACE ( 'NONE', ( #25644 ), #29065, .F. ) ;
#29805=ORIENTED_EDGE ( 'NONE', *, *, #18806, .T. ) ;
#29806=ORIENTED_EDGE ( 'NONE', *, *, #48541, .T. ) ;
#29808=ADVANCED_FACE ( 'NONE', ( #43284 ), #17141, .F. ) ;
#29809=PLANE ( 'NONE',  #8514 ) ;
#29810=CARTESIAN_POINT ( 'NONE',  ( -13.60688120397264278, -2.946525016555662457, 2.072686293655027434 ) ) ;
#29811=ADVANCED_FACE ( 'NONE', ( #34452 ), #42677, .F. ) ;
#29812=DIRECTION ( 'NONE',  ( 0.005961354470445682716, -0.6427876096865404731, -0.7660212471507180654 ) ) ;
#29813=ORIENTED_EDGE ( 'NONE', *, *, #33053, .F. ) ;
#29814=EDGE_CURVE ( 'NONE', #52782, #21764, #8625, .T. ) ;
#29815=EDGE_LOOP ( 'NONE', ( #29103, #7890, #39609 ) ) ;
#29816=DIRECTION ( 'NONE',  ( 0.005002170337468016433, -0.7660444431189770143, -0.6427681459581293666 ) ) ;
#29817=LINE ( 'NONE', #42851, #2765 ) ;
#29818=ORIENTED_EDGE ( 'NONE', *, *, #1134, .T. ) ;
#29819=LINE ( 'NONE', #3957, #40017 ) ;
#29820=CARTESIAN_POINT ( 'NONE',  ( -17.08865463677785357, 3.524445264749009876, 3.207297269127415085 ) ) ;
#29821=ORIENTED_EDGE ( 'NONE', *, *, #7959, .F. ) ;
#29822=LINE ( 'NONE', #55638, #7548 ) ;
#29823=ORIENTED_EDGE ( 'NONE', *, *, #31173, .T. ) ;
#29824=CARTESIAN_POINT ( 'NONE',  ( -20.02296364123857586, 1.376441525734817484, 6.094901730887621660 ) ) ;
#29825=ADVANCED_FACE ( 'NONE', ( #16028 ), #33350, .F. ) ;
#29826=DIRECTION ( 'NONE',  ( 0.5364919789714477361, 0.6444004775717706579, 0.5449076811759711036 ) ) ;
#29827=ORIENTED_EDGE ( 'NONE', *, *, #23424, .F. ) ;
#29828=LINE ( 'NONE', #30092, #26880 ) ;
#29829=DIRECTION ( 'NONE',  ( 0.007781995580012662783, 0.000000000000000000, -0.9999697198139514409 ) ) ;
#29830=CARTESIAN_POINT ( 'NONE',  ( -11.13365006456381856, 0.000000000000000000, 1.979111984108842037 ) ) ;
#29831=CARTESIAN_POINT ( 'NONE',  ( -17.79123777228383929, 5.467268677019013978, 3.418218180132968076 ) ) ;
#29832=EDGE_CURVE ( 'NONE', #51442, #30522, #42128, .T. ) ;
#29833=ORIENTED_EDGE ( 'NONE', *, *, #3784, .F. ) ;
#29834=VECTOR ( 'NONE', #49163, 1000.000000000000227 ) ;
#29835=EDGE_CURVE ( 'NONE', #21379, #40714, #53194, .T. ) ;
#29837=DIRECTION ( 'NONE',  ( 0.007781995580012663651, 0.000000000000000000, -0.9999697198139515519 ) ) ;
#29838=CARTESIAN_POINT ( 'NONE',  ( -10.67763532823858341, 0.000000000000000000, 3.090657005650145450 ) ) ;
#29839=CARTESIAN_POINT ( 'NONE',  ( -25.20123094555300369, 0.000000000000000000, 6.470945668149052032 ) ) ;
#29840=LINE ( 'NONE', #56221, #15830 ) ;
#29841=EDGE_CURVE ( 'NONE', #33876, #7777, #4374, .T. ) ;
#29842=PLANE ( 'NONE',  #19741 ) ;
#29843=DIRECTION ( 'NONE',  ( -0.5449076811759708816, 0.6444004775717707689, 0.5364919789714475140 ) ) ;
#29844=ORIENTED_EDGE ( 'NONE', *, *, #31402, .T. ) ;
#29848=CARTESIAN_POINT ( 'NONE',  ( -2.579292853887890757, -4.639166217699263406, -2.216488638059722849 ) ) ;
#29849=FACE_OUTER_BOUND ( 'NONE', #4841, .T. ) ;
#29850=FACE_OUTER_BOUND ( 'NONE', #33026, .T. ) ;
#29851=LINE ( 'NONE', #46893, #20565 ) ;
#29852=LINE ( 'NONE', #38931, #19309 ) ;
#29853=EDGE_CURVE ( 'NONE', #28798, #23596, #13702, .T. ) ;
#29857=CARTESIAN_POINT ( 'NONE',  ( -1.300095020133916979, 4.816411402586080470, 3.723374632896542025 ) ) ;
#29859=CARTESIAN_POINT ( 'NONE',  ( -25.20123094555300369, 0.000000000000000000, 6.470945668149052032 ) ) ;
#29860=ORIENTED_EDGE ( 'NONE', *, *, #32641, .F. ) ;
#29861=DIRECTION ( 'NONE',  ( 0.007781995580012662783, 0.000000000000000000, -0.9999697198139514409 ) ) ;
#29862=ORIENTED_EDGE ( 'NONE', *, *, #19666, .T. ) ;
#29863=CARTESIAN_POINT ( 'NONE',  ( -13.11728290589909918, -0.1191753592594190225, 5.187660494817285084 ) ) ;
#29864=ORIENTED_EDGE ( 'NONE', *, *, #24813, .T. ) ;
#29865=ORIENTED_EDGE ( 'NONE', *, *, #7894, .F. ) ;
#29867=CARTESIAN_POINT ( 'NONE',  ( -9.388691517149283072, -0.1191753592594190225, 3.739348975930303354 ) ) ;
#29868=DIRECTION ( 'NONE',  ( -0.6427681459581293666, -0.7660444431189770143, -0.005002170337467561935 ) ) ;
#29869=PLANE ( 'NONE',  #32106 ) ;
#29870=LINE ( 'NONE', #34670, #29405 ) ;
#29871=VERTEX_POINT ( 'NONE', #52351 ) ;
#29872=EDGE_CURVE ( 'NONE', #42922, #25139, #14300, .T. ) ;
#29873=VERTEX_POINT ( 'NONE', #21942 ) ;
#29874=ORIENTED_EDGE ( 'NONE', *, *, #48008, .F. ) ;
#29875=DIRECTION ( 'NONE',  ( 0.000000000000000000, -0.000000000000000000, -1.000000000000000000 ) ) ;
#29876=DIRECTION ( 'NONE',  ( 0.9999697198139515519, 0.000000000000000000, 0.007781995580013368816 ) ) ;
#29877=EDGE_LOOP ( 'NONE', ( #34528, #22640, #2204, #33436 ) ) ;
#29878=PLANE ( 'NONE',  #55664 ) ;
#29879=EDGE_LOOP ( 'NONE', ( #25662, #27326, #31108, #35381 ) ) ;
#29880=LINE ( 'NONE', #52006, #48714 ) ;
#29881=DIRECTION ( 'NONE',  ( -0.9999697198139514409, -0.000000000000000000, -0.007781995580013368816 ) ) ;
#29882=EDGE_CURVE ( 'NONE', #35428, #1353, #35567, .T. ) ;
#29883=EDGE_LOOP ( 'NONE', ( #15604, #4248, #15882, #10679 ) ) ;
#29884=DIRECTION ( 'NONE',  ( 0.9999697198139515519, 0.000000000000000000, 0.007781995580013368816 ) ) ;
#29885=ORIENTED_EDGE ( 'NONE', *, *, #55256, .T. ) ;
#29886=EDGE_CURVE ( 'NONE', #30608, #42734, #9165, .T. ) ;
#29887=EDGE_CURVE ( 'NONE', #18842, #636, #35040, .T. ) ;
#29888=DIRECTION ( 'NONE',  ( 0.000000000000000000, -1.000000000000000000, 0.000000000000000000 ) ) ;
#29889=CARTESIAN_POINT ( 'NONE',  ( -20.16176772743538237, -0.1191753592594197858, 14.76194180572237968 ) ) ;
#29890=VERTEX_POINT ( 'NONE', #915 ) ;
#29891=LINE ( 'NONE', #35, #36859 ) ;
#29892=LINE ( 'NONE', #26194, #22092 ) ;
#29893=DIRECTION ( 'NONE',  ( -0.6427681459581293666, -0.7660444431189770143, -0.005002170337467561935 ) ) ;
#29894=CARTESIAN_POINT ( 'NONE',  ( -18.67619601524082285, 0.000000000000000000, 3.936400510096834893 ) ) ;
#29895=ADVANCED_FACE ( 'NONE', ( #48065 ), #662, .F. ) ;
#29896=ORIENTED_EDGE ( 'NONE', *, *, #28853, .T. ) ;
#29897=ADVANCED_FACE ( 'NONE', ( #34727 ), #64, .F. ) ;
#29899=LINE ( 'NONE', #34704, #6751 ) ;
#29900=FACE_OUTER_BOUND ( 'NONE', #10885, .T. ) ;
#29901=CARTESIAN_POINT ( 'NONE',  ( -20.18761153005478093, 0.000000000000000000, 5.232640590720539109 ) ) ;
#29902=ADVANCED_FACE ( 'NONE', ( #40104 ), #18528, .F. ) ;
#29903=LINE ( 'NONE', #3498, #31550 ) ;
#29904=DIRECTION ( 'NONE',  ( -0.7660212471507179544, -0.6427876096865405842, -0.005961354470445141482 ) ) ;
#29905=VERTEX_POINT ( 'NONE', #13449 ) ;
#29906=DIRECTION ( 'NONE',  ( 0.5449076811759707706, 0.6444004775717708799, -0.5364919789714476250 ) ) ;
#29907=CARTESIAN_POINT ( 'NONE',  ( -18.67619601524082285, 0.000000000000000000, 3.936400510096834893 ) ) ;
#29909=ORIENTED_EDGE ( 'NONE', *, *, #54800, .F. ) ;
#29910=DIRECTION ( 'NONE',  ( -0.005961354470445682716, -0.6427876096865404731, 0.7660212471507180654 ) ) ;
#29911=FACE_OUTER_BOUND ( 'NONE', #40576, .T. ) ;
#29913=EDGE_CURVE ( 'NONE', #47218, #16890, #21685, .T. ) ;
#29914=DIRECTION ( 'NONE',  ( 0.7660212471507180654, -0.6427876096865404731, 0.005961354470445141482 ) ) ;
#29915=CARTESIAN_POINT ( 'NONE',  ( -18.78927038691023554, 0.000000000000000000, 4.674184678804012449 ) ) ;
#29916=LINE ( 'NONE', #4072, #25064 ) ;
#29918=ADVANCED_FACE ( 'NONE', ( #22239 ), #39574, .F. ) ;
#29919=ORIENTED_EDGE ( 'NONE', *, *, #46289, .T. ) ;
#29920=EDGE_LOOP ( 'NONE', ( #25868, #51460, #10279, #35823 ) ) ;
#29922=DIRECTION ( 'NONE',  ( -0.005961354470445682716, -0.6427876096865404731, 0.7660212471507180654 ) ) ;
#29923=DIRECTION ( 'NONE',  ( 0.7660212471507180654, -0.6427876096865404731, 0.005961354470445141482 ) ) ;
#29924=CARTESIAN_POINT ( 'NONE',  ( -13.17675323224890249, -1.327505506330657781, 1.957265181104025142 ) ) ;
#29925=LINE ( 'NONE', #31325, #21059 ) ;
#29927=ORIENTED_EDGE ( 'NONE', *, *, #45213, .T. ) ;
#29928=CARTESIAN_POINT ( 'NONE',  ( -10.29984434460210352, -0.1134144341942118078, 0.7824357519659358440 ) ) ;
#29929=FACE_OUTER_BOUND ( 'NONE', #14174, .T. ) ;
#29930=VERTEX_POINT ( 'NONE', #52046 ) ;
#29932=CARTESIAN_POINT ( 'NONE',  ( -16.99924723426068951, 0.000000000000000000, 13.49389102713827171 ) ) ;
#29933=DIRECTION ( 'NONE',  ( -0.005002170337468016433, -0.7660444431189770143, 0.6427681459581293666 ) ) ;
#29934=EDGE_LOOP ( 'NONE', ( #36466, #18720, #32797, #53351 ) ) ;
#29935=DIRECTION ( 'NONE',  ( 0.007781995580012663651, -3.146120232559066537E-19, -0.9999697198139514409 ) ) ;
#29936=EDGE_CURVE ( 'NONE', #44124, #42368, #35304, .T. ) ;
#29938=VECTOR ( 'NONE', #18324, 1000.000000000000227 ) ;
#29939=ORIENTED_EDGE ( 'NONE', *, *, #2429, .T. ) ;
#29940=ORIENTED_EDGE ( 'NONE', *, *, #34068, .T. ) ;
#29942=DIRECTION ( 'NONE',  ( -0.6427681459581293666, -0.7660444431189770143, -0.005002170337467561935 ) ) ;
#29943=VERTEX_POINT ( 'NONE', #30499 ) ;
#29944=EDGE_CURVE ( 'NONE', #49575, #15364, #27060, .T. ) ;
#29945=CARTESIAN_POINT ( 'NONE',  ( -18.39746900504187010, 0.000000000000000000, 14.03700784672088808 ) ) ;
#29946=EDGE_CURVE ( 'NONE', #34361, #37913, #17401, .T. ) ;
#29947=ORIENTED_EDGE ( 'NONE', *, *, #31364, .T. ) ;
#29948=LINE ( 'NONE', #3266, #54010 ) ;
#29949=VERTEX_POINT ( 'NONE', #42289 ) ;
#29950=CARTESIAN_POINT ( 'NONE',  ( -12.27728806973519404, 0.000000000000000000, 3.816872277745642084 ) ) ;
#29951=EDGE_LOOP ( 'NONE', ( #26946, #24173, #16963, #19296 ) ) ;
#29952=EDGE_CURVE ( 'NONE', #42667, #19558, #24962, .T. ) ;
#29953=CARTESIAN_POINT ( 'NONE',  ( -14.20280369269832832, 0.000000000000000000, 12.40765738797303719 ) ) ;
#29954=CARTESIAN_POINT ( 'NONE',  ( -26.13337879274045505, 0.000000000000000000, 6.833023547870798353 ) ) ;
#29955=FACE_OUTER_BOUND ( 'NONE', #51012, .T. ) ;
#29956=DIRECTION ( 'NONE',  ( -0.005961354470445682716, -0.6427876096865404731, 0.7660212471507180654 ) ) ;
#29958=EDGE_LOOP ( 'NONE', ( #2366, #8517, #39644, #34357 ) ) ;
#29959=VERTEX_POINT ( 'NONE', #20412 ) ;
#29960=EDGE_CURVE ( 'NONE', #35804, #46919, #28945, .T. ) ;
#29961=DIRECTION ( 'NONE',  ( 0.000000000000000000, -0.000000000000000000, -1.000000000000000000 ) ) ;
#29962=PLANE ( 'NONE',  #28464 ) ;
#29963=EDGE_CURVE ( 'NONE', #48365, #28099, #29202, .T. ) ;
#29964=CARTESIAN_POINT ( 'NONE',  ( -27.06552663992790997, 0.000000000000000000, 7.195101427592543786 ) ) ;
#29965=CARTESIAN_POINT ( 'NONE',  ( -24.27063949748155380, 0.000000000000000000, 6.308861732390097288 ) ) ;
#29966=EDGE_CURVE ( 'NONE', #17816, #25674, #55327, .T. ) ;
#29967=LINE ( 'NONE', #47270, #14972 ) ;
#29968=PLANE ( 'NONE',  #13254 ) ;
#29969=ORIENTED_EDGE ( 'NONE', *, *, #19652, .F. ) ;
#29970=CARTESIAN_POINT ( 'NONE',  ( -21.47263955680318404, 0.000000000000000000, 5.022634149262071190 ) ) ;
#29971=CARTESIAN_POINT ( 'NONE',  ( -15.91660050096674262, -0.1191753592594193972, 6.643203837240283960 ) ) ;
#29972=ORIENTED_EDGE ( 'NONE', *, *, #22094, .F. ) ;
#29973=ADVANCED_FACE ( 'NONE', ( #33744 ), #16422, .F. ) ;
#29974=CARTESIAN_POINT ( 'NONE',  ( -16.75372128362536728, 0.000000000000000000, 7.644682351054170155 ) ) ;
#29975=LINE ( 'NONE', #54079, #14241 ) ;
#29976=DIRECTION ( 'NONE',  ( 0.5364919789714477361, 0.6444004775717706579, 0.5449076811759711036 ) ) ;
#29977=CARTESIAN_POINT ( 'NONE',  ( 2.072287782118878319, 0.000000000000000000, -2.950529333540147015 ) ) ;
#29978=AXIS2_PLACEMENT_3D ( 'NONE', #43515, #35028, #16626 ) ;
#29979=VERTEX_POINT ( 'NONE', #33482 ) ;
#29980=ORIENTED_EDGE ( 'NONE', *, *, #32454, .T. ) ;
#29981=CARTESIAN_POINT ( 'NONE',  ( -14.00280974873554030, 0.000000000000000000, 12.40921378708904044 ) ) ;
#29982=CARTESIAN_POINT ( 'NONE',  ( -15.96710241509184058, -0.1191753592594218814, 13.13259134697452879 ) ) ;
#29983=CARTESIAN_POINT ( 'NONE',  ( 2.072287782118878319, 0.000000000000000000, -2.950529333540147015 ) ) ;
#29984=PLANE ( 'NONE',  #7400 ) ;
#29985=CARTESIAN_POINT ( 'NONE',  ( -10.27421835998572064, 0.000000000000000000, 10.96090226820206048 ) ) ;
#29986=LINE ( 'NONE', #33676, #26460 ) ;
#29987=PLANE ( 'NONE',  #8423 ) ;
#29989=LINE ( 'NONE', #7874, #53173 ) ;
#29990=DIRECTION ( 'NONE',  ( 0.007781995580012663651, -3.146120232559066537E-19, -0.9999697198139514409 ) ) ;
#29991=CARTESIAN_POINT ( 'NONE',  ( 2.072287782118878319, 0.000000000000000000, -2.950529333540147015 ) ) ;
#29992=ORIENTED_EDGE ( 'NONE', *, *, #42603, .F. ) ;
#29993=PLANE ( 'NONE',  #4152 ) ;
#29994=ADVANCED_FACE ( 'NONE', ( #49940 ), #41980, .F. ) ;
#29996=VERTEX_POINT ( 'NONE', #2535 ) ;
#29997=VECTOR ( 'NONE', #53411, 999.9999999999998863 ) ;
#29998=EDGE_CURVE ( 'NONE', #23767, #38400, #19855, .T. ) ;
#29999=ORIENTED_EDGE ( 'NONE', *, *, #48608, .F. ) ;
#30000=ORIENTED_EDGE ( 'NONE', *, *, #38292, .F. ) ;
#30001=ORIENTED_EDGE ( 'NONE', *, *, #8388, .F. ) ;
#30002=ORIENTED_EDGE ( 'NONE', *, *, #12885, .T. ) ;
#30003=ORIENTED_EDGE ( 'NONE', *, *, #15474, .F. ) ;
#30004=CARTESIAN_POINT ( 'NONE',  ( -18.09269438770527216, 0.2864062442990030766, 3.700610803468898258 ) ) ;
#30005=DIRECTION ( 'NONE',  ( 0.6246952433987893460, 0.7422098413412802076, -0.2426528472758539279 ) ) ;
#30006=FACE_OUTER_BOUND ( 'NONE', #16513, .T. ) ;
#30007=ADVANCED_FACE ( 'NONE', ( #11628 ), #20112, .F. ) ;
#30008=EDGE_CURVE ( 'NONE', #34747, #53648, #37446, .T. ) ;
#30009=EDGE_CURVE ( 'NONE', #25732, #44724, #45406, .T. ) ;
#30010=AXIS2_PLACEMENT_3D ( 'NONE', #41483, #11373, #54508 ) ;
#30011=ORIENTED_EDGE ( 'NONE', *, *, #47737, .T. ) ;
#30012=PLANE ( 'NONE',  #31318 ) ;
#30014=DIRECTION ( 'NONE',  ( -0.005961354470445682716, -0.6427876096865404731, 0.7660212471507180654 ) ) ;
#30015=EDGE_CURVE ( 'NONE', #11380, #2600, #11042, .T. ) ;
#30016=EDGE_LOOP ( 'NONE', ( #48681, #48582, #53322, #31659 ) ) ;
#30017=VECTOR ( 'NONE', #43945, 999.9999999999998863 ) ;
#30018=FACE_OUTER_BOUND ( 'NONE', #53478, .T. ) ;
#30019=PLANE ( 'NONE',  #36449 ) ;
#30020=CARTESIAN_POINT ( 'NONE',  ( -29.86197018149027116, 0.000000000000000000, 8.281335066757780083 ) ) ;
#30022=CARTESIAN_POINT ( 'NONE',  ( -19.18564475023670113, -3.432230869623159819, 9.767163286593927296 ) ) ;
#30023=ORIENTED_EDGE ( 'NONE', *, *, #29171, .T. ) ;
#30024=LINE ( 'NONE', #47334, #10134 ) ;
#30025=CARTESIAN_POINT ( 'NONE',  ( -9.043391767268570192, 0.000000000000000000, 6.227357638963272102 ) ) ;
#30026=EDGE_CURVE ( 'NONE', #55375, #27710, #15871, .T. ) ;
#30028=DIRECTION ( 'NONE',  ( -0.6427681459581293666, -0.7660444431189770143, -0.005002170337467561935 ) ) ;
#30029=CARTESIAN_POINT ( 'NONE',  ( -18.26565146671972073, -0.1191753592594149563, 9.948911607720113182 ) ) ;
#30030=DIRECTION ( 'NONE',  ( 0.5449076811759707706, 0.6444004775717708799, -0.5364919789714476250 ) ) ;
#30031=CARTESIAN_POINT ( 'NONE',  ( -26.13337879274045505, 0.000000000000000000, 6.833023547870798353 ) ) ;
#30032=EDGE_CURVE ( 'NONE', #50886, #44511, #50528, .T. ) ;
#30033=CARTESIAN_POINT ( 'NONE',  ( -14.90901332651993805, 0.9340140483890027046, 2.443298881491017038 ) ) ;
#30034=DIRECTION ( 'NONE',  ( 0.005002170337468016433, -0.7660444431189770143, -0.6427681459581293666 ) ) ;
#30035=ORIENTED_EDGE ( 'NONE', *, *, #7778, .T. ) ;
#30037=ORIENTED_EDGE ( 'NONE', *, *, #45168, .F. ) ;
#30038=VECTOR ( 'NONE', #49688, 999.9999999999998863 ) ;
#30040=VECTOR ( 'NONE', #23527, 1000.000000000000114 ) ;
#30042=DIRECTION ( 'NONE',  ( -0.9999697198139514409, -0.000000000000000000, -0.007781995580013368816 ) ) ;
#30043=LINE ( 'NONE', #191, #23605 ) ;
#30044=CARTESIAN_POINT ( 'NONE',  ( -13.10486132850893348, -4.565544526780663581, 1.826029526484286958 ) ) ;
#30045=LINE ( 'NONE', #33728, #21363 ) ;
#30046=ADVANCED_FACE ( 'NONE', ( #2248 ), #32634, .F. ) ;
#30047=DIRECTION ( 'NONE',  ( 0.9999697198139515519, 0.000000000000000000, 0.007781995580013368816 ) ) ;
#30048=PLANE ( 'NONE',  #7569 ) ;
#30050=EDGE_LOOP ( 'NONE', ( #38435, #45293, #42572, #13488 ) ) ;
#30052=DIRECTION ( 'NONE',  ( 0.007781995580012663651, -3.146120232559066537E-19, -0.9999697198139514409 ) ) ;
#30053=CARTESIAN_POINT ( 'NONE',  ( -26.13415699229845757, -0.1191753592594197858, 6.933020519852192365 ) ) ;
#30054=CARTESIAN_POINT ( 'NONE',  ( -12.67560930558469323, -0.1191753592594190225, 8.142010695456853853 ) ) ;
#30055=DIRECTION ( 'NONE',  ( -0.005002170337468016433, -0.7660444431189770143, 0.6427681459581293666 ) ) ;
#30056=DIRECTION ( 'NONE',  ( 0.000000000000000000, -0.000000000000000000, -1.000000000000000000 ) ) ;
#30057=CARTESIAN_POINT ( 'NONE',  ( -17.74404816805336793, 0.000000000000000000, 3.574322630375089460 ) ) ;
#30058=EDGE_LOOP ( 'NONE', ( #26423, #41990, #29306, #30973 ) ) ;
#30059=VECTOR ( 'NONE', #39799, 1000.000000000000227 ) ;
#30060=DIRECTION ( 'NONE',  ( 0.007781995580012662783, 0.000000000000000000, -0.9999697198139514409 ) ) ;
#30061=LINE ( 'NONE', #33220, #8887 ) ;
#30062=VERTEX_POINT ( 'NONE', #50225 ) ;
#30063=ORIENTED_EDGE ( 'NONE', *, *, #54176, .T. ) ;
#30064=CARTESIAN_POINT ( 'NONE',  ( 2.072287782118878319, 0.000000000000000000, -2.950529333540147015 ) ) ;
#30065=ORIENTED_EDGE ( 'NONE', *, *, #19743, .T. ) ;
#30066=ORIENTED_EDGE ( 'NONE', *, *, #8575, .T. ) ;
#30067=EDGE_LOOP ( 'NONE', ( #35743, #12124, #39268, #199 ) ) ;
#30068=ORIENTED_EDGE ( 'NONE', *, *, #22087, .T. ) ;
#30069=CARTESIAN_POINT ( 'NONE',  ( -18.40804000358828318, 2.876837460659008361, 3.740453431661805883 ) ) ;
#30070=ORIENTED_EDGE ( 'NONE', *, *, #12194, .T. ) ;
#30072=CARTESIAN_POINT ( 'NONE',  ( -11.23199219178955310, -0.1134144341942142642, 1.144513631687679611 ) ) ;
#30073=EDGE_CURVE ( 'NONE', #8011, #56197, #45989, .T. ) ;
#30074=VECTOR ( 'NONE', #24587, 1000.000000000000227 ) ;
#30075=AXIS2_PLACEMENT_3D ( 'NONE', #13876, #1380, #1919 ) ;
#30076=ORIENTED_EDGE ( 'NONE', *, *, #21885, .T. ) ;
#30077=ORIENTED_EDGE ( 'NONE', *, *, #14504, .T. ) ;
#30078=ADVANCED_FACE ( 'NONE', ( #34589 ), #17559, .F. ) ;
#30079=EDGE_CURVE ( 'NONE', #53603, #24506, #13323, .T. ) ;
#30080=AXIS2_PLACEMENT_3D ( 'NONE', #51485, #8896, #13428 ) ;
#30082=ORIENTED_EDGE ( 'NONE', *, *, #23515, .T. ) ;
#30083=CARTESIAN_POINT ( 'NONE',  ( -19.11062313909426535, 4.819660872929013351, 3.951374342667357542 ) ) ;
#30084=DIRECTION ( 'NONE',  ( -0.9999697198139514409, -0.000000000000000000, -0.007781995580013368816 ) ) ;
#30085=ORIENTED_EDGE ( 'NONE', *, *, #8837, .F. ) ;
#30086=DIRECTION ( 'NONE',  ( -0.005002170337468016433, -0.7660444431189770143, 0.6427681459581293666 ) ) ;
#30087=ORIENTED_EDGE ( 'NONE', *, *, #33800, .F. ) ;
#30088=CARTESIAN_POINT ( 'NONE',  ( -16.53317331066696383, 0.000000000000000000, 13.31285208727739899 ) ) ;
#30089=VECTOR ( 'NONE', #42392, 1000.000000000000227 ) ;
#30090=CARTESIAN_POINT ( 'NONE',  ( -11.63564965697357501, 0.000000000000000000, 6.776522214691770074 ) ) ;
#30091=ORIENTED_EDGE ( 'NONE', *, *, #36245, .T. ) ;
#30092=CARTESIAN_POINT ( 'NONE',  ( -13.08760808424579736, 3.200641362704010451, 1.663485951785882877 ) ) ;
#30093=DIRECTION ( 'NONE',  ( 0.9999697198139515519, 0.000000000000000000, 0.007781995580013368816 ) ) ;
#30094=PLANE ( 'NONE',  #41177 ) ;
#30095=DIRECTION ( 'NONE',  ( -0.5364919789714478471, 0.6444004775717705469, -0.5449076811759709926 ) ) ;
#30096=VERTEX_POINT ( 'NONE', #51636 ) ;
#30097=DIRECTION ( 'NONE',  ( 0.5364919789714477361, 0.6444004775717706579, 0.5449076811759711036 ) ) ;
#30098=LINE ( 'NONE', #8524, #39600 ) ;
#30099=CARTESIAN_POINT ( 'NONE',  ( -21.47419595591918906, 0.000000000000000000, 5.222628093224860102 ) ) ;
#30100=CARTESIAN_POINT ( 'NONE',  ( 2.072287782118878319, 0.000000000000000000, -2.950529333540147015 ) ) ;
#30101=DIRECTION ( 'NONE',  ( 0.5364919789714477361, 0.6444004775717706579, 0.5449076811759711036 ) ) ;
#30102=ADVANCED_FACE ( 'NONE', ( #46831 ), #34048, .F. ) ;
#30103=DIRECTION ( 'NONE',  ( 0.5364919789714477361, 0.6444004775717706579, 0.5449076811759711036 ) ) ;
#30104=CARTESIAN_POINT ( 'NONE',  ( -19.79127492296584734, -1.786397712959882034, 6.691370479880283106 ) ) ;
#30105=DIRECTION ( 'NONE',  ( 0.007781995580012663651, 0.000000000000000000, -0.9999697198139515519 ) ) ;
#30106=FACE_OUTER_BOUND ( 'NONE', #50437, .T. ) ;
#30107=ORIENTED_EDGE ( 'NONE', *, *, #39078, .T. ) ;
#30109=EDGE_CURVE ( 'NONE', #14557, #30246, #43406, .T. ) ;
#30110=PLANE ( 'NONE',  #52281 ) ;
#30111=VERTEX_POINT ( 'NONE', #12481 ) ;
#30112=DIRECTION ( 'NONE',  ( 0.7660212471507180654, -0.6427876096865404731, 0.005961354470445141482 ) ) ;
#30113=DIRECTION ( 'NONE',  ( -0.9999697198139514409, -0.000000000000000000, -0.007781995580013368816 ) ) ;
#30114=VECTOR ( 'NONE', #16720, 999.9999999999998863 ) ;
#30115=VECTOR ( 'NONE', #17113, 999.9999999999998863 ) ;
#30116=ADVANCED_FACE ( 'NONE', ( #7940 ), #47670, .F. ) ;
#30118=DIRECTION ( 'NONE',  ( 0.6427681459581294776, -0.7660444431189769032, 0.005002170337467562802 ) ) ;
#30119=DIRECTION ( 'NONE',  ( -0.5449076811759708816, 0.6444004775717707689, 0.5364919789714475140 ) ) ;
#30120=ORIENTED_EDGE ( 'NONE', *, *, #14271, .F. ) ;
#30121=VECTOR ( 'NONE', #5957, 1000.000000000000227 ) ;
#30122=ORIENTED_EDGE ( 'NONE', *, *, #41986, .F. ) ;
#30123=PLANE ( 'NONE',  #46754 ) ;
#30124=PLANE ( 'NONE',  #50358 ) ;
#30125=ORIENTED_EDGE ( 'NONE', *, *, #13831, .F. ) ;
#30126=CARTESIAN_POINT ( 'NONE',  ( 2.072287782118878319, 0.000000000000000000, -2.950529333540147015 ) ) ;
#30127=EDGE_LOOP ( 'NONE', ( #315, #33632, #34525, #6077 ) ) ;
#30128=DIRECTION ( 'NONE',  ( 0.005961354470445682716, -0.6427876096865404731, -0.7660212471507180654 ) ) ;
#30129=VECTOR ( 'NONE', #33174, 999.9999999999998863 ) ;
#30130=VERTEX_POINT ( 'NONE', #3647 ) ;
#30131=DIRECTION ( 'NONE',  ( 0.007781995580012663651, -3.146120232559066537E-19, -0.9999697198139514409 ) ) ;
#30132=VERTEX_POINT ( 'NONE', #20962 ) ;
#30133=ORIENTED_EDGE ( 'NONE', *, *, #48709, .F. ) ;
#30134=ORIENTED_EDGE ( 'NONE', *, *, #3482, .F. ) ;
#30135=DIRECTION ( 'NONE',  ( 0.007781995580012663651, 0.000000000000000000, -0.9999697198139515519 ) ) ;
#30136=EDGE_CURVE ( 'NONE', #35585, #28807, #25509, .T. ) ;
#30137=CARTESIAN_POINT ( 'NONE',  ( -20.54204810873173415, 0.000000000000000000, 4.860550213503115558 ) ) ;
#30138=DIRECTION ( 'NONE',  ( 0.000000000000000000, -1.000000000000000000, 0.000000000000000000 ) ) ;
#30139=EDGE_CURVE ( 'NONE', #39543, #3963, #8199, .T. ) ;
#30140=DIRECTION ( 'NONE',  ( 0.007781995580012663651, -3.146120232559066537E-19, -0.9999697198139514409 ) ) ;
#30141=EDGE_LOOP ( 'NONE', ( #54374, #7429, #41262, #35737 ) ) ;
#30142=ORIENTED_EDGE ( 'NONE', *, *, #27193, .F. ) ;
#30143=VECTOR ( 'NONE', #11867, 1000.000000000000227 ) ;
#30144=EDGE_CURVE ( 'NONE', #26056, #11768, #29797, .T. ) ;
#30145=EDGE_CURVE ( 'NONE', #3478, #13447, #21254, .T. ) ;
#30147=CARTESIAN_POINT ( 'NONE',  ( -17.46532115785441519, 0.000000000000000000, 13.67492996699914265 ) ) ;
#30148=ORIENTED_EDGE ( 'NONE', *, *, #37441, .F. ) ;
#30149=AXIS2_PLACEMENT_3D ( 'NONE', #52612, #35575, #39585 ) ;
#30150=CARTESIAN_POINT ( 'NONE',  ( -14.93495759592298988, 0.000000000000000000, 12.77129166681078409 ) ) ;
#30151=ORIENTED_EDGE ( 'NONE', *, *, #23745, .F. ) ;
#30152=CARTESIAN_POINT ( 'NONE',  ( -8.862326071713864550, -0.04157877016374941087, 4.177890584275355756 ) ) ;
#30153=CARTESIAN_POINT ( 'NONE',  ( -19.04209547915586143, -1.651309408375658760, 4.225232257889047105 ) ) ;
#30154=AXIS2_PLACEMENT_3D ( 'NONE', #43129, #13319, #26346 ) ;
#30155=VECTOR ( 'NONE', #41736, 999.9999999999998863 ) ;
#30156=ORIENTED_EDGE ( 'NONE', *, *, #32629, .T. ) ;
#30158=ORIENTED_EDGE ( 'NONE', *, *, #5282, .F. ) ;
#30159=ADVANCED_FACE ( 'NONE', ( #39133 ), #13022, .F. ) ;
#30160=VECTOR ( 'NONE', #24395, 1000.000000000000114 ) ;
#30161=CARTESIAN_POINT ( 'NONE',  ( -11.72533226533460038, 1.581621852479005774, 1.185986959513134487 ) ) ;
#30163=ORIENTED_EDGE ( 'NONE', *, *, #29872, .F. ) ;
#30164=DIRECTION ( 'NONE',  ( 0.5364919789714477361, 0.6444004775717706579, 0.5449076811759711036 ) ) ;
#30165=CARTESIAN_POINT ( 'NONE',  ( -21.47263955680318404, 0.000000000000000000, 5.022634149262071190 ) ) ;
#30166=CARTESIAN_POINT ( 'NONE',  ( -13.53118798318999794, 5.305366725996512045, 10.84430469370666117 ) ) ;
#30167=VERTEX_POINT ( 'NONE', #55914 ) ;
#30168=DIRECTION ( 'NONE',  ( -0.6427681459581293666, -0.7660444431189770143, -0.005002170337467561935 ) ) ;
#30169=LINE ( 'NONE', #47197, #44581 ) ;
#30170=DIRECTION ( 'NONE',  ( -0.6427681459581293666, -0.7660444431189770143, -0.005002170337467561935 ) ) ;
#30171=VECTOR ( 'NONE', #10707, 1000.000000000000227 ) ;
#30172=CARTESIAN_POINT ( 'NONE',  ( -26.13415699229845757, -0.1191753592594197858, 6.933020519852192365 ) ) ;
#30173=PLANE ( 'NONE',  #23069 ) ;
#30174=PLANE ( 'NONE',  #54226 ) ;
#30175=FACE_OUTER_BOUND ( 'NONE', #44624, .T. ) ;
#30176=ORIENTED_EDGE ( 'NONE', *, *, #20665, .F. ) ;
#30177=CARTESIAN_POINT ( 'NONE',  ( -10.86170260555895695, 0.000000000000000000, 1.042558146282530629 ) ) ;
#30178=DIRECTION ( 'NONE',  ( 0.7660212471507180654, -0.6427876096865404731, 0.005961354470445141482 ) ) ;
#30179=CARTESIAN_POINT ( 'NONE',  ( -18.32906394269043560, 0.000000000000000000, 5.247104237792575177 ) ) ;
#30180=ORIENTED_EDGE ( 'NONE', *, *, #40352, .F. ) ;
#30181=CARTESIAN_POINT ( 'NONE',  ( -14.05230480659183989, -0.1191753592594174960, 5.919048077796793095 ) ) ;
#30182=DIRECTION ( 'NONE',  ( 0.5449076811759707706, 0.6444004775717708799, -0.5364919789714476250 ) ) ;
#30184=AXIS2_PLACEMENT_3D ( 'NONE', #9266, #47908, #13278 ) ;
#30185=LINE ( 'NONE', #12317, #12608 ) ;
#30186=DIRECTION ( 'NONE',  ( -0.5449076811759708816, 0.6444004775717707689, 0.5364919789714475140 ) ) ;
#30187=ADVANCED_FACE ( 'NONE', ( #17014 ), #34333, .F. ) ;
#30188=AXIS2_PLACEMENT_3D ( 'NONE', #278, #9949, #27254 ) ;
#30189=PLANE ( 'NONE',  #26011 ) ;
#30191=ORIENTED_EDGE ( 'NONE', *, *, #34401, .F. ) ;
#30192=VERTEX_POINT ( 'NONE', #4245 ) ;
#30193=CARTESIAN_POINT ( 'NONE',  ( -13.43470767021154089, -4.403642575758163424, 1.959318567117884546 ) ) ;
#30194=CARTESIAN_POINT ( 'NONE',  ( -13.27065584551087163, 0.000000000000000000, 12.04557950825129176 ) ) ;
#30195=AXIS2_PLACEMENT_3D ( 'NONE', #24137, #1432, #41168 ) ;
#30196=LINE ( 'NONE', #48067, #6048 ) ;
#30198=VECTOR ( 'NONE', #13426, 999.9999999999998863 ) ;
#30199=LINE ( 'NONE', #13705, #41122 ) ;
#30200=VECTOR ( 'NONE', #10430, 1000.000000000000227 ) ;
#30201=LINE ( 'NONE', #26223, #41009 ) ;
#30202=DIRECTION ( 'NONE',  ( -0.7660212471507179544, -0.6427876096865405842, -0.005961354470445141482 ) ) ;
#30203=VERTEX_POINT ( 'NONE', #51903 ) ;
#30204=ADVANCED_FACE ( 'NONE', ( #30350 ), #28852, .F. ) ;
#30205=DIRECTION ( 'NONE',  ( 0.000000000000000000, -1.000000000000000000, 0.000000000000000000 ) ) ;
#30206=EDGE_CURVE ( 'NONE', #31801, #50295, #20615, .T. ) ;
#30208=LINE ( 'NONE', #42983, #45994 ) ;
#30209=VECTOR ( 'NONE', #38345, 999.9999999999998863 ) ;
#30210=ORIENTED_EDGE ( 'NONE', *, *, #6611, .F. ) ;
#30211=DIRECTION ( 'NONE',  ( 0.005002170337468016433, -0.7660444431189770143, -0.6427681459581293666 ) ) ;
#30212=ADVANCED_FACE ( 'NONE', ( #24857 ), #33941, .F. ) ;
#30213=DIRECTION ( 'NONE',  ( 0.9999697198139515519, 0.000000000000000000, 0.007781995580013368816 ) ) ;
#30215=ORIENTED_EDGE ( 'NONE', *, *, #44200, .F. ) ;
#30216=CARTESIAN_POINT ( 'NONE',  ( -11.21901323774118708, 0.000000000000000000, 1.039777472322872098 ) ) ;
#30217=EDGE_CURVE ( 'NONE', #32158, #17870, #15485, .T. ) ;
#30218=VECTOR ( 'NONE', #30030, 1000.000000000000114 ) ;
#30219=ORIENTED_EDGE ( 'NONE', *, *, #23733, .F. ) ;
#30220=VECTOR ( 'NONE', #18333, 1000.000000000000227 ) ;
#30222=VERTEX_POINT ( 'NONE', #46718 ) ;
#30223=VERTEX_POINT ( 'NONE', #33643 ) ;
#30224=ORIENTED_EDGE ( 'NONE', *, *, #3418, .T. ) ;
#30225=DIRECTION ( 'NONE',  ( 0.005002170337468016433, -0.7660444431189770143, -0.6427681459581293666 ) ) ;
#30227=AXIS2_PLACEMENT_3D ( 'NONE', #46334, #41800, #28190 ) ;
#30228=FACE_OUTER_BOUND ( 'NONE', #29877, .T. ) ;
#30229=EDGE_CURVE ( 'NONE', #22478, #13447, #20307, .T. ) ;
#30230=ORIENTED_EDGE ( 'NONE', *, *, #34070, .F. ) ;
#30231=PLANE ( 'NONE',  #30434 ) ;
#30233=FACE_OUTER_BOUND ( 'NONE', #53786, .T. ) ;
#30234=VECTOR ( 'NONE', #34128, 999.9999999999998863 ) ;
#30235=EDGE_LOOP ( 'NONE', ( #15464, #47169, #38174, #31182 ) ) ;
#30236=EDGE_CURVE ( 'NONE', #22227, #55768, #50696, .T. ) ;
#30237=CARTESIAN_POINT ( 'NONE',  ( -13.48844913732735762, 0.000000000000000000, 6.023439161104203521 ) ) ;
#30238=DIRECTION ( 'NONE',  ( -0.5364919789714478471, 0.6444004775717705469, -0.5449076811759709926 ) ) ;
#30239=DIRECTION ( 'NONE',  ( 0.005961354470445682716, -0.6427876096865404731, -0.7660212471507180654 ) ) ;
#30240=FACE_OUTER_BOUND ( 'NONE', #25915, .T. ) ;
#30242=CARTESIAN_POINT ( 'NONE',  ( -8.577437216038198642, 0.000000000000000000, 6.061657791436306120 ) ) ;
#30243=ORIENTED_EDGE ( 'NONE', *, *, #22692, .T. ) ;
#30244=VECTOR ( 'NONE', #49221, 1000.000000000000114 ) ;
#30245=AXIS2_PLACEMENT_3D ( 'NONE', #5815, #17762, #18885 ) ;
#30246=VERTEX_POINT ( 'NONE', #2978 ) ;
#30247=FACE_OUTER_BOUND ( 'NONE', #21432, .T. ) ;
#30248=CARTESIAN_POINT ( 'NONE',  ( -18.66354898467281132, 0.000000000000000000, 14.21960318569776582 ) ) ;
#30249=LINE ( 'NONE', #12385, #50546 ) ;
#30250=AXIS2_PLACEMENT_3D ( 'NONE', #55141, #24209, #28169 ) ;
#30251=VECTOR ( 'NONE', #5401, 999.9999999999998863 ) ;
#30252=CARTESIAN_POINT ( 'NONE',  ( 2.072287782118878319, 0.000000000000000000, -2.950529333540147015 ) ) ;
#30253=CARTESIAN_POINT ( 'NONE',  ( -11.26735747905060414, -0.1191753592594181482, 6.310053251662615992 ) ) ;
#30254=DIRECTION ( 'NONE',  ( -0.005961354470445682716, -0.6427876096865404731, 0.7660212471507180654 ) ) ;
#30255=ORIENTED_EDGE ( 'NONE', *, *, #15586, .T. ) ;
#30256=CARTESIAN_POINT ( 'NONE',  ( -14.66887761629205222, 0.000000000000000000, 12.58869632783390990 ) ) ;
#30257=DIRECTION ( 'NONE',  ( -0.005961354470445682716, -0.6427876096865404731, 0.7660212471507180654 ) ) ;
#30258=ORIENTED_EDGE ( 'NONE', *, *, #46003, .T. ) ;
#30259=CARTESIAN_POINT ( 'NONE',  ( -9.513398082562453340, 0.000000000000000000, 6.913700467289853435 ) ) ;
#30260=LINE ( 'NONE', #47278, #31500 ) ;
#30261=EDGE_CURVE ( 'NONE', #4723, #9720, #54659, .T. ) ;
#30263=DIRECTION ( 'NONE',  ( -0.005961354470445682716, -0.6427876096865404731, 0.7660212471507180654 ) ) ;
#30264=ORIENTED_EDGE ( 'NONE', *, *, #1785, .T. ) ;
#30265=AXIS2_PLACEMENT_3D ( 'NONE', #37544, #46070, #7178 ) ;
#30266=EDGE_LOOP ( 'NONE', ( #42635, #35056, #32593, #49638 ) ) ;
#30267=DIRECTION ( 'NONE',  ( -0.005002170337468016433, -0.7660444431189770143, 0.6427681459581293666 ) ) ;
#30268=LINE ( 'NONE', #32514, #34032 ) ;
#30269=DIRECTION ( 'NONE',  ( 0.7660212471507180654, -0.6427876096865404731, 0.005961354470445141482 ) ) ;
#30270=VECTOR ( 'NONE', #37859, 999.9999999999998863 ) ;
#30271=LINE ( 'NONE', #39347, #40038 ) ;
#30272=DIRECTION ( 'NONE',  ( -0.6427681459581293666, -0.7660444431189770143, -0.005002170337467561935 ) ) ;
#30273=AXIS2_PLACEMENT_3D ( 'NONE', #12197, #20438, #42576 ) ;
#30274=DIRECTION ( 'NONE',  ( 0.9999697198139515519, 0.000000000000000000, 0.007781995580013368816 ) ) ;
#30275=FACE_OUTER_BOUND ( 'NONE', #17229, .T. ) ;
#30276=VERTEX_POINT ( 'NONE', #37643 ) ;
#30277=EDGE_CURVE ( 'NONE', #36770, #38019, #15768, .T. ) ;
#30278=DIRECTION ( 'NONE',  ( -0.005002170337468016433, -0.7660444431189770143, 0.6427681459581293666 ) ) ;
#30279=LINE ( 'NONE', #52424, #2417 ) ;
#30280=VECTOR ( 'NONE', #28383, 999.9999999999998863 ) ;
#30281=EDGE_LOOP ( 'NONE', ( #41758, #41862, #46651, #5250 ) ) ;
#30282=DIRECTION ( 'NONE',  ( 0.007781995580012663651, 0.000000000000000000, -0.9999697198139515519 ) ) ;
#30283=VERTEX_POINT ( 'NONE', #16070 ) ;
#30284=DIRECTION ( 'NONE',  ( 0.7660212471507180654, -0.6427876096865404731, 0.005961354470445141482 ) ) ;
#30285=AXIS2_PLACEMENT_3D ( 'NONE', #17898, #5385, #27230 ) ;
#30286=EDGE_LOOP ( 'NONE', ( #34682, #18623, #25468, #56139 ) ) ;
#30289=EDGE_CURVE ( 'NONE', #52782, #7637, #16610, .T. ) ;
#30290=VECTOR ( 'NONE', #352, 1000.000000000000114 ) ;
#30291=EDGE_LOOP ( 'NONE', ( #12811, #32648, #22038, #8158 ) ) ;
#30292=VERTEX_POINT ( 'NONE', #11535 ) ;
#30293=VECTOR ( 'NONE', #41076, 1000.000000000000227 ) ;
#30294=VERTEX_POINT ( 'NONE', #24304 ) ;
#30295=EDGE_LOOP ( 'NONE', ( #14900, #26866, #20005, #47241 ) ) ;
#30296=CARTESIAN_POINT ( 'NONE',  ( -17.26532721389163072, 0.000000000000000000, 13.67648636611514590 ) ) ;
#30297=LINE ( 'NONE', #39374, #1173 ) ;
#30299=EDGE_CURVE ( 'NONE', #25456, #50706, #42176, .T. ) ;
#30300=VERTEX_POINT ( 'NONE', #11235 ) ;
#30301=LINE ( 'NONE', #55558, #21297 ) ;
#30302=ORIENTED_EDGE ( 'NONE', *, *, #31634, .F. ) ;
#30304=EDGE_CURVE ( 'NONE', #19686, #20073, #38185, .T. ) ;
#30305=CARTESIAN_POINT ( 'NONE',  ( -16.81345671998191449, 0.000000000000000000, 3.412238694616132495 ) ) ;
#30306=VECTOR ( 'NONE', #29296, 999.9999999999998863 ) ;
#30307=PLANE ( 'NONE',  #35047 ) ;
#30308=ORIENTED_EDGE ( 'NONE', *, *, #52802, .T. ) ;
#30309=CARTESIAN_POINT ( 'NONE',  ( -15.61019731987982873, -1.975113310420657520, 5.986959926383320862 ) ) ;
#30310=VECTOR ( 'NONE', #36193, 999.9999999999998863 ) ;
#30311=ORIENTED_EDGE ( 'NONE', *, *, #51039, .F. ) ;
#30312=CARTESIAN_POINT ( 'NONE',  ( -18.06838721921171498, 3.524445264749008988, 9.683911437457039639 ) ) ;
#30313=CARTESIAN_POINT ( 'NONE',  ( -22.40634380310664397, 0.000000000000000000, 5.584705972946605534 ) ) ;
#30314=VECTOR ( 'NONE', #22055, 999.9999999999998863 ) ;
#30315=DIRECTION ( 'NONE',  ( 0.9999697198139515519, 0.000000000000000000, 0.007781995580013368816 ) ) ;
#30316=CARTESIAN_POINT ( 'NONE',  ( 2.072287782118878319, 0.000000000000000000, -2.950529333540147015 ) ) ;
#30317=DIRECTION ( 'NONE',  ( 0.007781995580012663651, -3.146120232559066537E-19, -0.9999697198139514409 ) ) ;
#30318=PLANE ( 'NONE',  #39408 ) ;
#30319=LINE ( 'NONE', #22377, #42044 ) ;
#30320=VECTOR ( 'NONE', #20358, 999.9999999999998863 ) ;
#30321=LINE ( 'NONE', #47642, #3220 ) ;
#30322=ORIENTED_EDGE ( 'NONE', *, *, #43197, .F. ) ;
#30323=CARTESIAN_POINT ( 'NONE',  ( -19.60912206198628027, -0.1191753592594197858, 4.398475361799976113 ) ) ;
#30324=EDGE_CURVE ( 'NONE', #26517, #37130, #55502, .T. ) ;
#30325=VECTOR ( 'NONE', #52459, 999.9999999999998863 ) ;
#30326=CARTESIAN_POINT ( 'NONE',  ( -15.90797834045089587, -0.1191753592594207017, 5.535274727466993561 ) ) ;
#30327=FACE_OUTER_BOUND ( 'NONE', #3081, .T. ) ;
#30328=DIRECTION ( 'NONE',  ( -0.5449076811759708816, 0.6444004775717707689, 0.5364919789714475140 ) ) ;
#30329=EDGE_CURVE ( 'NONE', #25044, #3649, #19767, .T. ) ;
#30330=DIRECTION ( 'NONE',  ( 0.6427681459581294776, -0.7660444431189769032, 0.005002170337467562802 ) ) ;
#30331=DIRECTION ( 'NONE',  ( 0.000000000000000000, 1.000000000000000000, 0.000000000000000000 ) ) ;
#30332=DIRECTION ( 'NONE',  ( -0.005961354470445682716, -0.6427876096865404731, 0.7660212471507180654 ) ) ;
#30333=AXIS2_PLACEMENT_3D ( 'NONE', #28587, #18966, #10449 ) ;
#30334=DIRECTION ( 'NONE',  ( -0.7660212471507179544, -0.6427876096865405842, -0.005961354470445141482 ) ) ;
#30335=VECTOR ( 'NONE', #7530, 1000.000000000000227 ) ;
#30337=ORIENTED_EDGE ( 'NONE', *, *, #22568, .F. ) ;
#30338=EDGE_CURVE ( 'NONE', #39017, #50804, #54387, .T. ) ;
#30339=FACE_OUTER_BOUND ( 'NONE', #38183, .T. ) ;
#30340=DIRECTION ( 'NONE',  ( -0.7660212471507179544, -0.6427876096865405842, -0.005961354470445141482 ) ) ;
#30341=DIRECTION ( 'NONE',  ( 0.6427681459581294776, -0.7660444431189769032, 0.005002170337467562802 ) ) ;
#30342=EDGE_CURVE ( 'NONE', #38273, #22275, #45887, .T. ) ;
#30343=ADVANCED_FACE ( 'NONE', ( #18023 ), #8110, .F. ) ;
#30344=EDGE_CURVE ( 'NONE', #37808, #45566, #39321, .T. ) ;
#30345=DIRECTION ( 'NONE',  ( -0.3313982828793700097, 0.4028455766673915694, -0.8531650599175529814 ) ) ;
#30346=CARTESIAN_POINT ( 'NONE',  ( -14.01701317841955508, 0.000000000000000000, 2.326005055450897085 ) ) ;
#30347=CARTESIAN_POINT ( 'NONE',  ( -22.40478740399063895, 0.000000000000000000, 5.384712028983816623 ) ) ;
#30348=DIRECTION ( 'NONE',  ( 0.5449076811759707706, 0.6444004775717708799, -0.5364919789714476250 ) ) ;
#30349=AXIS2_PLACEMENT_3D ( 'NONE', #13543, #24689, #50810 ) ;
#30350=FACE_OUTER_BOUND ( 'NONE', #40541, .T. ) ;
#30351=CARTESIAN_POINT ( 'NONE',  ( -9.353677591794285817, 2.186419275952748986, 2.912935481226179402 ) ) ;
#30352=VECTOR ( 'NONE', #50531, 1000.000000000000227 ) ;
#30353=ORIENTED_EDGE ( 'NONE', *, *, #8424, .F. ) ;
#30354=CARTESIAN_POINT ( 'NONE',  ( -19.60990026154428278, 0.000000000000000000, 4.498472333781370125 ) ) ;
#30355=AXIS2_PLACEMENT_3D ( 'NONE', #33869, #51190, #12302 ) ;
#30356=ORIENTED_EDGE ( 'NONE', *, *, #4762, .T. ) ;
#30357=EDGE_CURVE ( 'NONE', #2187, #14051, #4673, .T. ) ;
#30358=EDGE_CURVE ( 'NONE', #21510, #37821, #43852, .T. ) ;
#30359=ORIENTED_EDGE ( 'NONE', *, *, #28980, .T. ) ;
#30360=ORIENTED_EDGE ( 'NONE', *, *, #54295, .F. ) ;
#30361=VECTOR ( 'NONE', #18667, 999.9999999999998863 ) ;
#30362=ORIENTED_EDGE ( 'NONE', *, *, #39654, .T. ) ;
#30363=EDGE_CURVE ( 'NONE', #49603, #54423, #9212, .T. ) ;
#30364=VECTOR ( 'NONE', #5564, 999.9999999999998863 ) ;
#30365=ORIENTED_EDGE ( 'NONE', *, *, #29645, .F. ) ;
#30366=DIRECTION ( 'NONE',  ( 0.005961354470445682716, -0.6427876096865404731, -0.7660212471507180654 ) ) ;
#30367=FACE_OUTER_BOUND ( 'NONE', #29077, .T. ) ;
#30369=ADVANCED_FACE ( 'NONE', ( #30247 ), #408, .F. ) ;
#30370=ORIENTED_EDGE ( 'NONE', *, *, #891, .F. ) ;
#30371=EDGE_CURVE ( 'NONE', #15287, #51394, #26005, .T. ) ;
#30372=AXIS2_PLACEMENT_3D ( 'NONE', #13774, #30576, #52124 ) ;
#30373=VECTOR ( 'NONE', #17752, 1000.000000000000227 ) ;
#30374=CARTESIAN_POINT ( 'NONE',  ( -12.78414981984007071, -5.213152330870663320, 10.20340078340005974 ) ) ;
#30375=ORIENTED_EDGE ( 'NONE', *, *, #7980, .F. ) ;
#30376=LINE ( 'NONE', #47694, #19179 ) ;
#30377=DIRECTION ( 'NONE',  ( 0.007781995580012663651, 0.000000000000000000, -0.9999697198139515519 ) ) ;
#30378=VERTEX_POINT ( 'NONE', #43323 ) ;
#30379=DIRECTION ( 'NONE',  ( 0.007781995580012663651, -3.146120232559066537E-19, -0.9999697198139514409 ) ) ;
#30380=ORIENTED_EDGE ( 'NONE', *, *, #41778, .T. ) ;
#30381=DIRECTION ( 'NONE',  ( -0.6427681459581293666, -0.7660444431189770143, -0.005002170337467561935 ) ) ;
#30382=VECTOR ( 'NONE', #16708, 999.9999999999998863 ) ;
#30383=DIRECTION ( 'NONE',  ( 0.5449076811759707706, 0.6444004775717708799, -0.5364919789714476250 ) ) ;
#30384=ORIENTED_EDGE ( 'NONE', *, *, #35611, .F. ) ;
#30385=DIRECTION ( 'NONE',  ( 0.5364919789714477361, 0.6444004775717706579, 0.5449076811759711036 ) ) ;
#30386=LINE ( 'NONE', #21842, #35648 ) ;
#30387=LINE ( 'NONE', #3424, #5803 ) ;
#30389=DIRECTION ( 'NONE',  ( -0.9999697198139514409, 0.000000000000000000, -0.007781995580013368816 ) ) ;
#30390=ORIENTED_EDGE ( 'NONE', *, *, #51327, .T. ) ;
#30391=VECTOR ( 'NONE', #16622, 1000.000000000000227 ) ;
#30392=DIRECTION ( 'NONE',  ( 0.005002170337468016433, -0.7660444431189770143, -0.6427681459581293666 ) ) ;
#30394=DIRECTION ( 'NONE',  ( -0.005002170337468016433, -0.7660444431189770143, 0.6427681459581293666 ) ) ;
#30395=CARTESIAN_POINT ( 'NONE',  ( -16.53317331066696383, 0.000000000000000000, 13.31285208727739899 ) ) ;
#30396=VECTOR ( 'NONE', #16194, 1000.000000000000227 ) ;
#30397=CARTESIAN_POINT ( 'NONE',  ( -15.09516764022381174, 0.000000000000000000, 7.657589599010205639 ) ) ;
#30398=DIRECTION ( 'NONE',  ( -0.5364919789714478471, 0.6444004775717705469, -0.5449076811759709926 ) ) ;
#30399=DIRECTION ( 'NONE',  ( 0.000000000000000000, -0.000000000000000000, -1.000000000000000000 ) ) ;
#30400=PLANE ( 'NONE',  #257 ) ;
#30401=VECTOR ( 'NONE', #13192, 1000.000000000000227 ) ;
#30402=DIRECTION ( 'NONE',  ( 0.005002170337468016433, -0.7660444431189770143, -0.6427681459581293666 ) ) ;
#30403=VECTOR ( 'NONE', #15424, 1000.000000000000227 ) ;
#30405=VECTOR ( 'NONE', #23362, 999.9999999999998863 ) ;
#30406=CARTESIAN_POINT ( 'NONE',  ( -20.56906454177918064, -5.051250379848161387, 12.96161735426753303 ) ) ;
#30407=VERTEX_POINT ( 'NONE', #4415 ) ;
#30408=DIRECTION ( 'NONE',  ( 0.005961354470445682716, -0.6427876096865404731, -0.7660212471507180654 ) ) ;
#30409=LINE ( 'NONE', #35784, #17273 ) ;
#30410=AXIS2_PLACEMENT_3D ( 'NONE', #42805, #51355, #47351 ) ;
#30411=EDGE_CURVE ( 'NONE', #15538, #11444, #17444, .T. ) ;
#30412=EDGE_CURVE ( 'NONE', #30623, #40953, #34780, .T. ) ;
#30414=EDGE_CURVE ( 'NONE', #25905, #37607, #13489, .T. ) ;
#30415=DIRECTION ( 'NONE',  ( -0.9999697198139514409, -0.000000000000000000, -0.007781995580013368816 ) ) ;
#30416=LINE ( 'NONE', #35243, #47401 ) ;
#30417=VERTEX_POINT ( 'NONE', #39037 ) ;
#30418=VECTOR ( 'NONE', #47041, 999.9999999999998863 ) ;
#30419=VECTOR ( 'NONE', #8461, 999.9999999999998863 ) ;
#30420=VERTEX_POINT ( 'NONE', #12915 ) ;
#30422=FACE_OUTER_BOUND ( 'NONE', #5226, .T. ) ;
#30423=ORIENTED_EDGE ( 'NONE', *, *, #101, .F. ) ;
#30424=LINE ( 'NONE', #8856, #21179 ) ;
#30425=ORIENTED_EDGE ( 'NONE', *, *, #40140, .F. ) ;
#30426=DIRECTION ( 'NONE',  ( -0.005961354470445682716, -0.6427876096865404731, 0.7660212471507180654 ) ) ;
#30427=VERTEX_POINT ( 'NONE', #39625 ) ;
#30428=DIRECTION ( 'NONE',  ( 0.007781995580012663651, 0.000000000000000000, -0.9999697198139515519 ) ) ;
#30429=EDGE_CURVE ( 'NONE', #6407, #26740, #43019, .T. ) ;
#30430=VECTOR ( 'NONE', #3000, 999.9999999999998863 ) ;
#30431=VERTEX_POINT ( 'NONE', #55803 ) ;
#30432=EDGE_LOOP ( 'NONE', ( #54346, #11110, #29601, #13259 ) ) ;
#30434=AXIS2_PLACEMENT_3D ( 'NONE', #94, #55224, #47546 ) ;
#30435=CARTESIAN_POINT ( 'NONE',  ( -14.46888367232926420, 0.000000000000000000, 12.59025272694991315 ) ) ;
#30436=FACE_OUTER_BOUND ( 'NONE', #764, .T. ) ;
#30437=VECTOR ( 'NONE', #2453, 1000.000000000000227 ) ;
#30438=CARTESIAN_POINT ( 'NONE',  ( -10.74029228357944987, 0.000000000000000000, 11.14194120806293320 ) ) ;
#30439=EDGE_CURVE ( 'NONE', #50871, #26864, #13748, .T. ) ;
#30440=DIRECTION ( 'NONE',  ( 0.9999697198139515519, 0.000000000000000000, 0.007781995580013368816 ) ) ;
#30441=EDGE_LOOP ( 'NONE', ( #56002, #37543, #6523 ) ) ;
#30442=VECTOR ( 'NONE', #40797, 999.9999999999998863 ) ;
#30443=EDGE_LOOP ( 'NONE', ( #28110, #14287, #28962, #7942 ) ) ;
#30445=ORIENTED_EDGE ( 'NONE', *, *, #18569, .F. ) ;
#30447=AXIS2_PLACEMENT_3D ( 'NONE', #27089, #43080, #4193 ) ;
#30448=ADVANCED_FACE ( 'NONE', ( #21148 ), #47854, .F. ) ;
#30449=DIRECTION ( 'NONE',  ( 0.5364919789714477361, 0.6444004775717706579, 0.5449076811759711036 ) ) ;
#30450=ORIENTED_EDGE ( 'NONE', *, *, #49369, .F. ) ;
#30451=LINE ( 'NONE', #12563, #20275 ) ;
#30452=EDGE_CURVE ( 'NONE', #29102, #19178, #47263, .T. ) ;
#30453=ORIENTED_EDGE ( 'NONE', *, *, #46894, .F. ) ;
#30454=PLANE ( 'NONE',  #36922 ) ;
#30455=CARTESIAN_POINT ( 'NONE',  ( -26.13415699229845757, -0.1191753592594197858, 6.933020519852192365 ) ) ;
#30456=AXIS2_PLACEMENT_3D ( 'NONE', #32508, #49548, #28220 ) ;
#30457=EDGE_LOOP ( 'NONE', ( #47545, #28536, #45479, #27462, #31887 ) ) ;
#30458=AXIS2_PLACEMENT_3D ( 'NONE', #29753, #22044, #39373 ) ;
#30459=EDGE_CURVE ( 'NONE', #15204, #19054, #13208, .T. ) ;
#30460=DIRECTION ( 'NONE',  ( 0.5449076811759707706, 0.6444004775717708799, -0.5364919789714476250 ) ) ;
#30461=VECTOR ( 'NONE', #2400, 1000.000000000000227 ) ;
#30462=ORIENTED_EDGE ( 'NONE', *, *, #51310, .F. ) ;
#30463=AXIS2_PLACEMENT_3D ( 'NONE', #19446, #10385, #24532 ) ;
#30464=LINE ( 'NONE', #34164, #28173 ) ;
#30465=AXIS2_PLACEMENT_3D ( 'NONE', #24875, #8127, #50974 ) ;
#30466=VERTEX_POINT ( 'NONE', #17179 ) ;
#30467=CARTESIAN_POINT ( 'NONE',  ( -17.25977937193981404, 5.305366725996510269, 12.29261621259364112 ) ) ;
#30468=CARTESIAN_POINT ( 'NONE',  ( -10.27421835998572064, 0.000000000000000000, 10.96090226820206048 ) ) ;
#30469=PLANE ( 'NONE',  #39147 ) ;
#30470=ORIENTED_EDGE ( 'NONE', *, *, #31290, .T. ) ;
#30471=CARTESIAN_POINT ( 'NONE',  ( -14.05517886009712036, -0.1191753592594174960, 6.288357781054557449 ) ) ;
#30472=CARTESIAN_POINT ( 'NONE',  ( -13.73672976910459909, 0.000000000000000000, 12.22661844811216270 ) ) ;
#30473=DIRECTION ( 'NONE',  ( 0.7660212471507180654, -0.6427876096865404731, 0.005961354470445141482 ) ) ;
#30474=CARTESIAN_POINT ( 'NONE',  ( -16.93204742750033631, 5.467268677019011314, 12.43102267950012951 ) ) ;
#30475=FACE_OUTER_BOUND ( 'NONE', #55825, .T. ) ;
#30476=CARTESIAN_POINT ( 'NONE',  ( 2.072287782118878319, 0.000000000000000000, -2.950529333540147015 ) ) ;
#30477=AXIS2_PLACEMENT_3D ( 'NONE', #55680, #55981, #282 ) ;
#30478=PLANE ( 'NONE',  #54864 ) ;
#30479=ORIENTED_EDGE ( 'NONE', *, *, #13184, .T. ) ;
#30480=DIRECTION ( 'NONE',  ( 0.9999697198139515519, 0.000000000000000000, 0.007781995580013368816 ) ) ;
#30481=FACE_OUTER_BOUND ( 'NONE', #11889, .T. ) ;
#30482=LINE ( 'NONE', #48631, #35070 ) ;
#30483=VERTEX_POINT ( 'NONE', #8957 ) ;
#30484=CARTESIAN_POINT ( 'NONE',  ( -27.99923088623136636, 0.000000000000000000, 7.757173251277078130 ) ) ;
#30485=VECTOR ( 'NONE', #17760, 1000.000000000000114 ) ;
#30486=VERTEX_POINT ( 'NONE', #26259 ) ;
#30487=ADVANCED_FACE ( 'NONE', ( #37932 ), #50961, .F. ) ;
#30488=FACE_OUTER_BOUND ( 'NONE', #50018, .T. ) ;
#30489=CARTESIAN_POINT ( 'NONE',  ( -10.44554592974990470, 0.000000000000000000, 7.275778347011597980 ) ) ;
#30490=AXIS2_PLACEMENT_3D ( 'NONE', #24177, #50573, #10830 ) ;
#30491=ADVANCED_FACE ( 'NONE', ( #55239 ), #32813, .F. ) ;
#30492=EDGE_CURVE ( 'NONE', #30714, #46212, #33946, .T. ) ;
#30493=LINE ( 'NONE', #51506, #50471 ) ;
#30495=EDGE_LOOP ( 'NONE', ( #10866, #30380, #36724, #2900 ) ) ;
#30496=VECTOR ( 'NONE', #14735, 1000.000000000000227 ) ;
#30497=AXIS2_PLACEMENT_3D ( 'NONE', #54573, #37270, #2360 ) ;
#30498=EDGE_LOOP ( 'NONE', ( #42319, #13623, #40495, #43290 ) ) ;
#30499=CARTESIAN_POINT ( 'NONE',  ( -15.98863513745331311, 0.000000000000000000, 3.049325577086037242 ) ) ;
#30500=DIRECTION ( 'NONE',  ( -0.005002170337468016433, -0.7660444431189770143, 0.6427681459581293666 ) ) ;
#30501=DIRECTION ( 'NONE',  ( 0.9999697198139515519, 0.000000000000000000, 0.007781995580013368816 ) ) ;
#30502=VECTOR ( 'NONE', #40744, 999.9999999999998863 ) ;
#30503=LINE ( 'NONE', #8629, #33870 ) ;
#30504=VECTOR ( 'NONE', #2747, 999.9999999999998863 ) ;
#30505=DIRECTION ( 'NONE',  ( 0.000000000000000000, -0.000000000000000000, -1.000000000000000000 ) ) ;
#30506=DIRECTION ( 'NONE',  ( 0.005961354470445682716, -0.6427876096865404731, -0.7660212471507180654 ) ) ;
#30507=VERTEX_POINT ( 'NONE', #54980 ) ;
#30509=AXIS2_PLACEMENT_3D ( 'NONE', #21345, #33300, #29868 ) ;
#30510=AXIS2_PLACEMENT_3D ( 'NONE', #19138, #53781, #3511 ) ;
#30511=DIRECTION ( 'NONE',  ( -0.5364919789714478471, 0.6444004775717705469, -0.5449076811759709926 ) ) ;
#30512=ORIENTED_EDGE ( 'NONE', *, *, #7588, .F. ) ;
#30514=CARTESIAN_POINT ( 'NONE',  ( -19.15756256483321351, -0.1191753592594164135, 5.140653641833157650 ) ) ;
#30516=ORIENTED_EDGE ( 'NONE', *, *, #55307, .T. ) ;
#30517=DIRECTION ( 'NONE',  ( 0.005961354470445682716, -0.6427876096865404731, -0.7660212471507180654 ) ) ;
#30518=ORIENTED_EDGE ( 'NONE', *, *, #4284, .T. ) ;
#30519=ADVANCED_FACE ( 'NONE', ( #15491 ), #20026, .F. ) ;
#30520=VECTOR ( 'NONE', #1579, 999.9999999999998863 ) ;
#30521=ORIENTED_EDGE ( 'NONE', *, *, #35668, .F. ) ;
#30522=VERTEX_POINT ( 'NONE', #41881 ) ;
#30523=EDGE_CURVE ( 'NONE', #10129, #4038, #50435, .T. ) ;
#30524=ORIENTED_EDGE ( 'NONE', *, *, #52228, .F. ) ;
#30525=CARTESIAN_POINT ( 'NONE',  ( -8.375886872959409146, 0.000000000000000000, 5.863220246589520457 ) ) ;
#30526=VECTOR ( 'NONE', #8842, 999.9999999999998863 ) ;
#30527=ORIENTED_EDGE ( 'NONE', *, *, #52270, .F. ) ;
#30529=ORIENTED_EDGE ( 'NONE', *, *, #36181, .F. ) ;
#30530=CARTESIAN_POINT ( 'NONE',  ( -17.73140113748535285, 0.000000000000000000, 13.85752530597602039 ) ) ;
#30531=VECTOR ( 'NONE', #29798, 999.9999999999998863 ) ;
#30532=EDGE_CURVE ( 'NONE', #36489, #17725, #3563, .T. ) ;
#30533=ORIENTED_EDGE ( 'NONE', *, *, #39830, .T. ) ;
#30534=LINE ( 'NONE', #51794, #8380 ) ;
#30535=EDGE_LOOP ( 'NONE', ( #46475, #42048, #48460, #25233 ) ) ;
#30536=VECTOR ( 'NONE', #18674, 1000.000000000000227 ) ;
#30537=PLANE ( 'NONE',  #5745 ) ;
#30538=CARTESIAN_POINT ( 'NONE',  ( -14.93495759592298988, 0.000000000000000000, 12.77129166681078409 ) ) ;
#30539=DIRECTION ( 'NONE',  ( -0.9999697198139514409, -0.000000000000000000, -0.007781995580013368816 ) ) ;
#30540=CARTESIAN_POINT ( 'NONE',  ( -18.85791280579721985, -3.594132820645661308, 9.905569753500415686 ) ) ;
#30541=LINE ( 'NONE', #47850, #50094 ) ;
#30543=ADVANCED_FACE ( 'NONE', ( #29407 ), #7847, .F. ) ;
#30544=VERTEX_POINT ( 'NONE', #38191 ) ;
#30546=DIRECTION ( 'NONE',  ( 0.9999697198139515519, 0.000000000000000000, 0.007781995580013368816 ) ) ;
#30547=DIRECTION ( 'NONE',  ( -0.5364919789714478471, 0.6444004775717705469, -0.5449076811759709926 ) ) ;
#30548=EDGE_CURVE ( 'NONE', #27352, #3917, #33396, .T. ) ;
#30549=VECTOR ( 'NONE', #4461, 999.9999999999998863 ) ;
#30550=DIRECTION ( 'NONE',  ( 0.5449076811759707706, 0.6444004775717708799, -0.5364919789714476250 ) ) ;
#30551=VECTOR ( 'NONE', #10072, 1000.000000000000000 ) ;
#30552=CARTESIAN_POINT ( 'NONE',  ( -19.22961988024793101, -0.1191753592594177458, 14.39986392600063603 ) ) ;
#30553=PLANE ( 'NONE',  #19500 ) ;
#30554=DIRECTION ( 'NONE',  ( -0.6246952433987894571, 0.7422098413412802076, 0.2426528472758539834 ) ) ;
#30555=ORIENTED_EDGE ( 'NONE', *, *, #50277, .F. ) ;
#30556=CARTESIAN_POINT ( 'NONE',  ( -19.55346843781402910, -2.379430070215138304, 7.303589053828619448 ) ) ;
#30557=ADVANCED_FACE ( 'NONE', ( #46156 ), #33651, .T. ) ;
#30558=CARTESIAN_POINT ( 'NONE',  ( -12.70458494993575194, -0.1191753592594197858, 11.86531876794841978 ) ) ;
#30559=EDGE_LOOP ( 'NONE', ( #28017, #12562, #39538, #20672 ) ) ;
#30560=FACE_OUTER_BOUND ( 'NONE', #29141, .T. ) ;
#30561=DIRECTION ( 'NONE',  ( -0.9999697198139514409, -0.000000000000000000, -0.007781995580013368816 ) ) ;
#30562=EDGE_CURVE ( 'NONE', #46828, #47750, #37348, .T. ) ;
#30564=ADVANCED_FACE ( 'NONE', ( #11792 ), #20870, .F. ) ;
#30566=VECTOR ( 'NONE', #46925, 1000.000000000000227 ) ;
#30567=CARTESIAN_POINT ( 'NONE',  ( -20.54049170961573267, 0.000000000000000000, 4.660556269540326646 ) ) ;
#30568=ORIENTED_EDGE ( 'NONE', *, *, #21018, .T. ) ;
#30569=ORIENTED_EDGE ( 'NONE', *, *, #19110, .F. ) ;
#30570=CARTESIAN_POINT ( 'NONE',  ( -20.10835023650160736, -0.9956879032862070433, 5.875079047949166799 ) ) ;
#30571=DIRECTION ( 'NONE',  ( 0.000000000000000000, -1.000000000000000000, 0.000000000000000000 ) ) ;
#30572=FACE_OUTER_BOUND ( 'NONE', #3332, .T. ) ;
#30573=EDGE_CURVE ( 'NONE', #52239, #38033, #16618, .T. ) ;
#30574=CARTESIAN_POINT ( 'NONE',  ( -14.01545677930355183, 0.000000000000000000, 2.126011111488108174 ) ) ;
#30575=AXIS2_PLACEMENT_3D ( 'NONE', #48135, #31105, #47599 ) ;
#30576=DIRECTION ( 'NONE',  ( 0.000000000000000000, -1.000000000000000000, 0.000000000000000000 ) ) ;
#30577=CARTESIAN_POINT ( 'NONE',  ( -15.08079737269739873, 0.000000000000000000, 5.811041082721382978 ) ) ;
#30578=FACE_OUTER_BOUND ( 'NONE', #13605, .T. ) ;
#30579=ORIENTED_EDGE ( 'NONE', *, *, #17770, .F. ) ;
#30581=CARTESIAN_POINT ( 'NONE',  ( -16.81190032086591302, 0.000000000000000000, 3.212244750653343583 ) ) ;
#30582=AXIS2_PLACEMENT_3D ( 'NONE', #53508, #44702, #5819 ) ;
#30583=CARTESIAN_POINT ( 'NONE',  ( -16.75659533713064775, 0.000000000000000000, 8.013992054311934510 ) ) ;
#30584=VERTEX_POINT ( 'NONE', #37096 ) ;
#30585=CARTESIAN_POINT ( 'NONE',  ( -22.02261458013905226, 4.333955019861509328, 12.54841105031995241 ) ) ;
#30586=EDGE_LOOP ( 'NONE', ( #20564, #48664, #45786, #32654 ) ) ;
#30587=DIRECTION ( 'NONE',  ( -0.005961354470445682716, -0.6427876096865404731, 0.7660212471507180654 ) ) ;
#30588=DIRECTION ( 'NONE',  ( -0.6427681459581293666, -0.7660444431189770143, -0.005002170337467561935 ) ) ;
#30589=VERTEX_POINT ( 'NONE', #7008 ) ;
#30590=VECTOR ( 'NONE', #42092, 1000.000000000000227 ) ;
#30591=ORIENTED_EDGE ( 'NONE', *, *, #17450, .F. ) ;
#30592=ORIENTED_EDGE ( 'NONE', *, *, #2822, .F. ) ;
#30593=VECTOR ( 'NONE', #910, 1000.000000000000000 ) ;
#30594=ORIENTED_EDGE ( 'NONE', *, *, #12054, .F. ) ;
#30595=ORIENTED_EDGE ( 'NONE', *, *, #7882, .T. ) ;
#30596=VERTEX_POINT ( 'NONE', #24310 ) ;
#30597=LINE ( 'NONE', #51851, #12286 ) ;
#30598=DIRECTION ( 'NONE',  ( -0.005002170337468016433, -0.7660444431189770143, 0.6427681459581293666 ) ) ;
#30599=CARTESIAN_POINT ( 'NONE',  ( -16.78706339993119556, 0.9340140483890039258, 4.934862808901015363 ) ) ;
#30600=ORIENTED_EDGE ( 'NONE', *, *, #32567, .F. ) ;
#30601=CARTESIAN_POINT ( 'NONE',  ( -4.394946353583525145, 7.064620221120807564, -1.511227158925545266 ) ) ;
#30602=EDGE_CURVE ( 'NONE', #34227, #15529, #41620, .T. ) ;
#30603=ORIENTED_EDGE ( 'NONE', *, *, #12768, .F. ) ;
#30604=ORIENTED_EDGE ( 'NONE', *, *, #51779, .T. ) ;
#30605=CARTESIAN_POINT ( 'NONE',  ( -17.74482636761137044, -0.1191753592594197858, 3.674319602356483916 ) ) ;
#30606=LINE ( 'NONE', #47909, #43908 ) ;
#30607=LINE ( 'NONE', #47910, #6900 ) ;
#30608=VERTEX_POINT ( 'NONE', #46417 ) ;
#30609=DIRECTION ( 'NONE',  ( 0.6427681459581294776, -0.7660444431189769032, 0.005002170337467562802 ) ) ;
#30610=ORIENTED_EDGE ( 'NONE', *, *, #14473, .T. ) ;
#30611=EDGE_CURVE ( 'NONE', #50804, #11380, #4679, .T. ) ;
#30612=LINE ( 'NONE', #13284, #10098 ) ;
#30613=DIRECTION ( 'NONE',  ( 0.005961354470445682716, -0.6427876096865404731, -0.7660212471507180654 ) ) ;
#30614=ADVANCED_FACE ( 'NONE', ( #17183 ), #30553, .F. ) ;
#30615=EDGE_CURVE ( 'NONE', #19873, #20126, #43327, .T. ) ;
#30617=AXIS2_PLACEMENT_3D ( 'NONE', #29983, #12940, #4991 ) ;
#30618=LINE ( 'NONE', #48467, #48549 ) ;
#30619=DIRECTION ( 'NONE',  ( -0.7660212471507179544, -0.6427876096865405842, -0.005961354470445141482 ) ) ;
#30620=CARTESIAN_POINT ( 'NONE',  ( -8.944172994845175140, -0.1191753592594181482, 6.328132810502664185 ) ) ;
#30621=FACE_OUTER_BOUND ( 'NONE', #48857, .T. ) ;
#30622=DIRECTION ( 'NONE',  ( 0.5449076811759707706, 0.6444004775717708799, -0.5364919789714476250 ) ) ;
#30623=VERTEX_POINT ( 'NONE', #30810 ) ;
#30624=CARTESIAN_POINT ( 'NONE',  ( -9.908141408373387193, -0.1191753592594197858, 10.77908512878318703 ) ) ;
#30625=AXIS2_PLACEMENT_3D ( 'NONE', #22907, #14127, #31721 ) ;
#30626=DIRECTION ( 'NONE',  ( 0.000000000000000000, -1.000000000000000000, 0.000000000000000000 ) ) ;
#30627=CARTESIAN_POINT ( 'NONE',  ( -20.54126990917373519, -0.1191753592594197858, 4.760553241521720658 ) ) ;
#30628=EDGE_CURVE ( 'NONE', #36677, #16658, #13755, .T. ) ;
#30629=CARTESIAN_POINT ( 'NONE',  ( -14.01701317841955508, 0.000000000000000000, 2.326005055450897085 ) ) ;
#30631=DIRECTION ( 'NONE',  ( 0.7660212471507180654, -0.6427876096865404731, 0.005961354470445141482 ) ) ;
#30632=EDGE_CURVE ( 'NONE', #26534, #9630, #52396, .T. ) ;
#30633=LINE ( 'NONE', #48787, #23246 ) ;
#30634=DIRECTION ( 'NONE',  ( 0.005002170337468016433, -0.7660444431189770143, -0.6427681459581293666 ) ) ;
#30635=EDGE_LOOP ( 'NONE', ( #33092, #25080, #53768, #37690 ) ) ;
#30636=LINE ( 'NONE', #3378, #24807 ) ;
#30637=PLANE ( 'NONE',  #5909 ) ;
#30638=CARTESIAN_POINT ( 'NONE',  ( 2.072287782118878319, 0.000000000000000000, -2.950529333540147015 ) ) ;
#30639=EDGE_CURVE ( 'NONE', #32268, #46991, #708, .T. ) ;
#30640=CARTESIAN_POINT ( 'NONE',  ( -11.62415344295244779, 0.000000000000000000, 5.299283401660711768 ) ) ;
#30641=CARTESIAN_POINT ( 'NONE',  ( 2.072287782118878319, 0.000000000000000000, -2.950529333540147015 ) ) ;
#30642=CARTESIAN_POINT ( 'NONE',  ( -16.81190032086591302, 0.000000000000000000, 3.212244750653343583 ) ) ;
#30643=CARTESIAN_POINT ( 'NONE',  ( -10.76248383313556367, -0.1191753592594202577, 1.143333317821924489 ) ) ;
#30644=ADVANCED_FACE ( 'NONE', ( #43858 ), #8116, .F. ) ;
#30645=CARTESIAN_POINT ( 'NONE',  ( -12.80458192191714595, 0.000000000000000000, 11.86454056839041726 ) ) ;
#30647=ORIENTED_EDGE ( 'NONE', *, *, #24819, .T. ) ;
#30648=CARTESIAN_POINT ( 'NONE',  ( -9.748361534556408969, 0.000000000000000000, 3.097888829186164816 ) ) ;
#30649=VERTEX_POINT ( 'NONE', #30253 ) ;
#30650=ORIENTED_EDGE ( 'NONE', *, *, #18344, .F. ) ;
#30651=ORIENTED_EDGE ( 'NONE', *, *, #15639, .F. ) ;
#30652=VERTEX_POINT ( 'NONE', #8685 ) ;
#30653=EDGE_LOOP ( 'NONE', ( #22792, #3474, #8633, #41326 ) ) ;
#30654=DIRECTION ( 'NONE',  ( -0.6427681459581293666, -0.7660444431189770143, -0.005002170337467561935 ) ) ;
#30655=CARTESIAN_POINT ( 'NONE',  ( -11.97318020560097729, 2.391131607591506114, 5.456365251615914680 ) ) ;
#30656=VECTOR ( 'NONE', #10832, 999.9999999999998863 ) ;
#30657=EDGE_LOOP ( 'NONE', ( #14518, #4510, #51477, #53442 ) ) ;
#30658=ORIENTED_EDGE ( 'NONE', *, *, #33957, .T. ) ;
#30659=EDGE_CURVE ( 'NONE', #53347, #39093, #47566, .T. ) ;
#30660=EDGE_CURVE ( 'NONE', #51468, #36412, #22301, .T. ) ;
#30662=ORIENTED_EDGE ( 'NONE', *, *, #19291, .F. ) ;
#30663=EDGE_CURVE ( 'NONE', #24292, #30130, #55811, .T. ) ;
#30664=CARTESIAN_POINT ( 'NONE',  ( -18.32362714986662411, 1.095915999411505082, 5.797425035250995506 ) ) ;
#30666=VERTEX_POINT ( 'NONE', #52649 ) ;
#30667=PLANE ( 'NONE',  #4718 ) ;
#30668=ADVANCED_FACE ( 'NONE', ( #31073 ), #35095, .F. ) ;
#30669=EDGE_CURVE ( 'NONE', #37975, #41809, #13495, .T. ) ;
#30670=EDGE_CURVE ( 'NONE', #6528, #52618, #18028, .T. ) ;
#30671=ORIENTED_EDGE ( 'NONE', *, *, #31225, .F. ) ;
#30672=DIRECTION ( 'NONE',  ( 0.6246952433987893460, 0.7422098413412802076, -0.2426528472758539279 ) ) ;
#30673=LINE ( 'NONE', #12508, #10068 ) ;
#30674=ORIENTED_EDGE ( 'NONE', *, *, #52054, .T. ) ;
#30675=DIRECTION ( 'NONE',  ( -0.005002170337468016433, -0.7660444431189770143, 0.6427681459581293666 ) ) ;
#30676=LINE ( 'NONE', #27509, #2993 ) ;
#30679=CARTESIAN_POINT ( 'NONE',  ( -10.74029228357944987, 0.000000000000000000, 11.14194120806293320 ) ) ;
#30680=ORIENTED_EDGE ( 'NONE', *, *, #40180, .T. ) ;
#30681=LINE ( 'NONE', #3427, #28290 ) ;
#30682=CARTESIAN_POINT ( 'NONE',  ( -15.40103151951671734, 0.000000000000000000, 12.95233060667165681 ) ) ;
#30683=CARTESIAN_POINT ( 'NONE',  ( -17.86442704584935015, 0.000000000000000000, 5.250720149560584638 ) ) ;
#30684=ADVANCED_FACE ( 'NONE', ( #52102 ), #47860, .F. ) ;
#30685=DIRECTION ( 'NONE',  ( 0.007781995580012663651, 0.000000000000000000, -0.9999697198139515519 ) ) ;
#30687=CARTESIAN_POINT ( 'NONE',  ( -21.47263955680318404, 0.000000000000000000, 5.022634149262071190 ) ) ;
#30688=FACE_OUTER_BOUND ( 'NONE', #26192, .T. ) ;
#30689=EDGE_CURVE ( 'NONE', #32551, #37828, #42729, .T. ) ;
#30690=DIRECTION ( 'NONE',  ( -0.005002170337468016433, -0.7660444431189770143, 0.6427681459581293666 ) ) ;
#30691=EDGE_CURVE ( 'NONE', #51521, #39606, #12652, .T. ) ;
#30692=DIRECTION ( 'NONE',  ( 0.007781995580012663651, 0.000000000000000000, -0.9999697198139515519 ) ) ;
#30693=EDGE_LOOP ( 'NONE', ( #5239, #8570, #50135, #45564 ) ) ;
#30694=FACE_OUTER_BOUND ( 'NONE', #41041, .T. ) ;
#30695=CARTESIAN_POINT ( 'NONE',  ( -22.40634380310664397, 0.000000000000000000, 5.584705972946605534 ) ) ;
#30696=CARTESIAN_POINT ( 'NONE',  ( -12.05619391717654310, -3.270328918600659218, 6.732133781913477222 ) ) ;
#30697=EDGE_CURVE ( 'NONE', #3706, #42498, #29967, .T. ) ;
#30698=VECTOR ( 'NONE', #19271, 1000.000000000000000 ) ;
#30700=DIRECTION ( 'NONE',  ( 0.000000000000000000, -1.000000000000000000, 0.000000000000000000 ) ) ;
#30701=FACE_OUTER_BOUND ( 'NONE', #11102, .T. ) ;
#30702=ORIENTED_EDGE ( 'NONE', *, *, #28706, .F. ) ;
#30703=VERTEX_POINT ( 'NONE', #25703 ) ;
#30704=FACE_OUTER_BOUND ( 'NONE', #34053, .T. ) ;
#30705=DIRECTION ( 'NONE',  ( -0.5364919789714478471, 0.6444004775717705469, -0.5449076811759709926 ) ) ;
#30706=ORIENTED_EDGE ( 'NONE', *, *, #34325, .T. ) ;
#30707=CARTESIAN_POINT ( 'NONE',  ( 2.072287782118878319, 0.000000000000000000, -2.950529333540147015 ) ) ;
#30708=EDGE_LOOP ( 'NONE', ( #1955, #2881, #3394, #24480 ) ) ;
#30709=DIRECTION ( 'NONE',  ( 0.5364919789714477361, 0.6444004775717706579, 0.5449076811759711036 ) ) ;
#30710=ORIENTED_EDGE ( 'NONE', *, *, #1447, .F. ) ;
#30711=LINE ( 'NONE', #4571, #19312 ) ;
#30712=EDGE_LOOP ( 'NONE', ( #39137, #53397, #41053, #10821 ) ) ;
#30713=ORIENTED_EDGE ( 'NONE', *, *, #38444, .F. ) ;
#30714=VERTEX_POINT ( 'NONE', #27961 ) ;
#30716=PLANE ( 'NONE',  #16615 ) ;
#30717=DIRECTION ( 'NONE',  ( 0.7660212471507180654, -0.6427876096865404731, 0.005961354470445141482 ) ) ;
#30718=LINE ( 'NONE', #35514, #40247 ) ;
#30719=LINE ( 'NONE', #27560, #22067 ) ;
#30720=EDGE_LOOP ( 'NONE', ( #2914, #9711, #7837, #36822 ) ) ;
#30722=EDGE_LOOP ( 'NONE', ( #30311, #29947, #46186, #44867 ) ) ;
#30723=DIRECTION ( 'NONE',  ( 0.007781995580012663651, 0.000000000000000000, -0.9999697198139515519 ) ) ;
#30724=EDGE_LOOP ( 'NONE', ( #30148, #22036, #22828, #56004, #46520 ) ) ;
#30725=LINE ( 'NONE', #51165, #50180 ) ;
#30726=ORIENTED_EDGE ( 'NONE', *, *, #50461, .T. ) ;
#30727=CARTESIAN_POINT ( 'NONE',  ( -14.00280974873554030, 0.000000000000000000, 12.40921378708904044 ) ) ;
#30728=DIRECTION ( 'NONE',  ( -0.005961354470445682716, -0.6427876096865404731, 0.7660212471507180654 ) ) ;
#30729=EDGE_CURVE ( 'NONE', #9458, #34138, #19128, .T. ) ;
#30730=EDGE_CURVE ( 'NONE', #19740, #4570, #40156, .T. ) ;
#30731=EDGE_CURVE ( 'NONE', #38688, #7205, #48397, .T. ) ;
#30733=ORIENTED_EDGE ( 'NONE', *, *, #55936, .F. ) ;
#30734=FACE_OUTER_BOUND ( 'NONE', #3801, .T. ) ;
#30735=ORIENTED_EDGE ( 'NONE', *, *, #49996, .F. ) ;
#30736=EDGE_CURVE ( 'NONE', #50295, #7467, #14600, .T. ) ;
#30737=DIRECTION ( 'NONE',  ( 0.5449076811759707706, 0.6444004775717708799, -0.5364919789714476250 ) ) ;
#30738=ORIENTED_EDGE ( 'NONE', *, *, #14381, .T. ) ;
#30739=DIRECTION ( 'NONE',  ( 0.9999697198139515519, 0.000000000000000000, 0.007781995580013368816 ) ) ;
#30740=DIRECTION ( 'NONE',  ( -0.5364919789714478471, 0.6444004775717705469, -0.5449076811759709926 ) ) ;
#30741=DIRECTION ( 'NONE',  ( 0.5364919789714477361, 0.6444004775717706579, 0.5449076811759711036 ) ) ;
#30742=ORIENTED_EDGE ( 'NONE', *, *, #26350, .F. ) ;
#30743=CARTESIAN_POINT ( 'NONE',  ( -9.024829791847592375, 0.000000000000000000, 3.842183660121707867 ) ) ;
#30744=CARTESIAN_POINT ( 'NONE',  ( -19.53579455766131900, 0.000000000000000000, 6.884367473930582904 ) ) ;
#30746=CARTESIAN_POINT ( 'NONE',  ( -21.47341775636118655, -0.1191753592594197858, 5.122631121243466090 ) ) ;
#30747=CARTESIAN_POINT ( 'NONE',  ( -13.68556902778486339, 0.000000000000000000, 5.652573058730435918 ) ) ;
#30748=CARTESIAN_POINT ( 'NONE',  ( -30.79411802867772607, 0.000000000000000000, 8.643412946479525516 ) ) ;
#30749=ADVANCED_FACE ( 'NONE', ( #23416 ), #14049, .F. ) ;
#30750=CARTESIAN_POINT ( 'NONE',  ( -15.37130680712323816, 0.000000000000000000, 9.132768899389256845 ) ) ;
#30751=ORIENTED_EDGE ( 'NONE', *, *, #7377, .F. ) ;
#30752=FACE_OUTER_BOUND ( 'NONE', #26637, .T. ) ;
#30753=CARTESIAN_POINT ( 'NONE',  ( -15.32975240366000236, 0.000000000000000000, 3.793117294485577329 ) ) ;
#30754=ADVANCED_FACE ( 'NONE', ( #27110 ), #6369, .F. ) ;
#30755=DIRECTION ( 'NONE',  ( -0.5364919789714478471, 0.6444004775717705469, -0.5449076811759709926 ) ) ;
#30756=ORIENTED_EDGE ( 'NONE', *, *, #12138, .F. ) ;
#30757=PLANE ( 'NONE',  #44709 ) ;
#30758=CARTESIAN_POINT ( 'NONE',  ( -21.47341775636118655, -0.1191753592594197858, 5.122631121243466090 ) ) ;
#30759=ORIENTED_EDGE ( 'NONE', *, *, #49057, .F. ) ;
#30760=DIRECTION ( 'NONE',  ( 0.007781995580012663651, 0.000000000000000000, -0.9999697198139515519 ) ) ;
#30761=ADVANCED_FACE ( 'NONE', ( #45264 ), #40734, .F. ) ;
#30762=CARTESIAN_POINT ( 'NONE',  ( -10.76823194014612639, -0.1191753592594204242, 1.881952724337453642 ) ) ;
#30763=FACE_OUTER_BOUND ( 'NONE', #51347, .T. ) ;
#30764=ADVANCED_FACE ( 'NONE', ( #15182 ), #40464, .F. ) ;
#30765=DIRECTION ( 'NONE',  ( -0.6246952433987894571, 0.7422098413412802076, 0.2426528472758539834 ) ) ;
#30766=EDGE_LOOP ( 'NONE', ( #32750, #16516, #32799, #37924 ) ) ;
#30767=ORIENTED_EDGE ( 'NONE', *, *, #23717, .F. ) ;
#30768=DIRECTION ( 'NONE',  ( -0.5364919789714478471, 0.6444004775717705469, -0.5449076811759709926 ) ) ;
#30769=CARTESIAN_POINT ( 'NONE',  ( -13.73672976910459909, 0.000000000000000000, 12.22661844811216270 ) ) ;
#30770=DIRECTION ( 'NONE',  ( 0.000000000000000000, -0.000000000000000000, -1.000000000000000000 ) ) ;
#30771=DIRECTION ( 'NONE',  ( -0.005961354470445682716, -0.6427876096865404731, 0.7660212471507180654 ) ) ;
#30772=VECTOR ( 'NONE', #10835, 1000.000000000000227 ) ;
#30773=PLANE ( 'NONE',  #11974 ) ;
#30774=CARTESIAN_POINT ( 'NONE',  ( -17.74404816805336793, 0.000000000000000000, 3.574322630375089460 ) ) ;
#30775=ORIENTED_EDGE ( 'NONE', *, *, #1866, .T. ) ;
#30776=DIRECTION ( 'NONE',  ( 0.007781995580012663651, -3.146120232559066537E-19, -0.9999697198139514409 ) ) ;
#30778=ORIENTED_EDGE ( 'NONE', *, *, #3670, .T. ) ;
#30779=DIRECTION ( 'NONE',  ( 0.005961354470445682716, -0.6427876096865404731, -0.7660212471507180654 ) ) ;
#30780=FACE_OUTER_BOUND ( 'NONE', #22783, .T. ) ;
#30781=CARTESIAN_POINT ( 'NONE',  ( -11.14312833067548958, 1.419719901456505395, 3.539692811011753371 ) ) ;
#30782=EDGE_LOOP ( 'NONE', ( #35506, #50542, #32344, #1062 ) ) ;
#30783=DIRECTION ( 'NONE',  ( -0.9999697198139514409, -0.000000000000000000, -0.007781995580013368816 ) ) ;
#30784=EDGE_LOOP ( 'NONE', ( #20713, #44262, #46801, #23330 ) ) ;
#30785=ORIENTED_EDGE ( 'NONE', *, *, #21676, .F. ) ;
#30786=EDGE_LOOP ( 'NONE', ( #49543, #8051, #44567, #55614 ) ) ;
#30787=VERTEX_POINT ( 'NONE', #18587 ) ;
#30788=DIRECTION ( 'NONE',  ( 0.000000000000000000, -0.000000000000000000, -1.000000000000000000 ) ) ;
#30789=ORIENTED_EDGE ( 'NONE', *, *, #33380, .T. ) ;
#30790=DIRECTION ( 'NONE',  ( 0.6427681459581294776, -0.7660444431189769032, 0.005002170337467562802 ) ) ;
#30792=ORIENTED_EDGE ( 'NONE', *, *, #26141, .F. ) ;
#30793=CARTESIAN_POINT ( 'NONE',  ( -14.13715331148882015, 0.000000000000000000, 3.971724389968579239 ) ) ;
#30794=EDGE_LOOP ( 'NONE', ( #12458, #8827, #47382, #20360 ) ) ;
#30795=DIRECTION ( 'NONE',  ( 0.005961354470445682716, -0.6427876096865404731, -0.7660212471507180654 ) ) ;
#30796=ORIENTED_EDGE ( 'NONE', *, *, #14851, .T. ) ;
#30797=ADVANCED_FACE ( 'NONE', ( #53254 ), #10059, .F. ) ;
#30798=ADVANCED_FACE ( 'NONE', ( #9807 ), #39883, .F. ) ;
#30799=FACE_OUTER_BOUND ( 'NONE', #48283, .T. ) ;
#30800=DIRECTION ( 'NONE',  ( 0.5364919789714477361, 0.6444004775717706579, 0.5449076811759711036 ) ) ;
#30801=CARTESIAN_POINT ( 'NONE',  ( -8.580311269543482666, 0.000000000000000000, 6.430967494694069586 ) ) ;
#30802=LINE ( 'NONE', #48102, #47763 ) ;
#30803=DIRECTION ( 'NONE',  ( -0.5449076811759708816, 0.6444004775717707689, 0.5364919789714475140 ) ) ;
#30804=ORIENTED_EDGE ( 'NONE', *, *, #4935, .F. ) ;
#30805=EDGE_LOOP ( 'NONE', ( #34185, #41718, #33484, #39534 ) ) ;
#30806=CARTESIAN_POINT ( 'NONE',  ( -14.94760462649100496, 0.000000000000000000, 2.488088991209854051 ) ) ;
#30807=LINE ( 'NONE', #56095, #3089 ) ;
#30808=PLANE ( 'NONE',  #36941 ) ;
#30809=FACE_OUTER_BOUND ( 'NONE', #26514, .T. ) ;
#30810=CARTESIAN_POINT ( 'NONE',  ( -12.28147977762975707, 0.000000000000000000, 4.355497740298383214 ) ) ;
#30811=LINE ( 'NONE', #47861, #36850 ) ;
#30812=ORIENTED_EDGE ( 'NONE', *, *, #39955, .T. ) ;
#30813=DIRECTION ( 'NONE',  ( 0.7660212471507180654, -0.6427876096865404731, 0.005961354470445141482 ) ) ;
#30814=CARTESIAN_POINT ( 'NONE',  ( -30.79489622823572859, -0.1191753592594197858, 8.743409918460921304 ) ) ;
#30815=ORIENTED_EDGE ( 'NONE', *, *, #45443, .F. ) ;
#30817=DIRECTION ( 'NONE',  ( 0.000000000000000000, -1.000000000000000000, 0.000000000000000000 ) ) ;
#30818=LINE ( 'NONE', #35636, #43181 ) ;
#30819=ADVANCED_FACE ( 'NONE', ( #2075 ), #19411, .F. ) ;
#30820=LINE ( 'NONE', #38796, #536 ) ;
#30821=LINE ( 'NONE', #48124, #27425 ) ;
#30822=ORIENTED_EDGE ( 'NONE', *, *, #46673, .T. ) ;
#30823=EDGE_CURVE ( 'NONE', #15750, #13531, #49538, .T. ) ;
#30825=CARTESIAN_POINT ( 'NONE',  ( -15.61159646202592199, 2.876837460659008361, 2.654219792496569141 ) ) ;
#30826=DIRECTION ( 'NONE',  ( 0.007781995580012663651, -3.146120232559066537E-19, -0.9999697198139514409 ) ) ;
#30827=CARTESIAN_POINT ( 'NONE',  ( -22.40556560354864146, -0.1191753592594197858, 5.484709000965211523 ) ) ;
#30828=DIRECTION ( 'NONE',  ( -0.9999697198139514409, -0.000000000000000000, -0.007781995580013368816 ) ) ;
#30829=ADVANCED_FACE ( 'NONE', ( #36198 ), #53501, .F. ) ;
#30830=DIRECTION ( 'NONE',  ( 0.007781995580012663651, 0.000000000000000000, -0.9999697198139515519 ) ) ;
#30832=FACE_OUTER_BOUND ( 'NONE', #33981, .T. ) ;
#30833=LINE ( 'NONE', #30581, #4210 ) ;
#30834=FACE_OUTER_BOUND ( 'NONE', #22961, .T. ) ;
#30835=ORIENTED_EDGE ( 'NONE', *, *, #21938, .T. ) ;
#30836=DIRECTION ( 'NONE',  ( -0.5449076811759708816, 0.6444004775717707689, 0.5364919789714475140 ) ) ;
#30837=ORIENTED_EDGE ( 'NONE', *, *, #44150, .F. ) ;
#30838=CARTESIAN_POINT ( 'NONE',  ( -19.59569683186026268, 0.000000000000000000, 14.58168106541950948 ) ) ;
#30839=DIRECTION ( 'NONE',  ( -0.005002170337468016433, -0.7660444431189770143, 0.6427681459581293666 ) ) ;
#30840=ORIENTED_EDGE ( 'NONE', *, *, #10270, .F. ) ;
#30841=ORIENTED_EDGE ( 'NONE', *, *, #36719, .T. ) ;
#30842=ORIENTED_EDGE ( 'NONE', *, *, #32582, .F. ) ;
#30843=ORIENTED_EDGE ( 'NONE', *, *, #25514, .F. ) ;
#30844=VERTEX_POINT ( 'NONE', #45003 ) ;
#30845=ORIENTED_EDGE ( 'NONE', *, *, #50850, .T. ) ;
#30846=LINE ( 'NONE', #21199, #39492 ) ;
#30847=LINE ( 'NONE', #43614, #32037 ) ;
#30848=EDGE_CURVE ( 'NONE', #25456, #9641, #11733, .T. ) ;
#30849=DIRECTION ( 'NONE',  ( -0.005961354470445682716, -0.6427876096865404731, 0.7660212471507180654 ) ) ;
#30850=ORIENTED_EDGE ( 'NONE', *, *, #48874, .F. ) ;
#30851=CARTESIAN_POINT ( 'NONE',  ( -11.67244013076689946, 0.000000000000000000, 11.50401908778467863 ) ) ;
#30853=ORIENTED_EDGE ( 'NONE', *, *, #25529, .F. ) ;
#30854=ADVANCED_FACE ( 'NONE', ( #16011 ), #42111, .F. ) ;
#30855=CARTESIAN_POINT ( 'NONE',  ( -10.80272058220951870, -0.1191753592594185784, 6.313669163430627229 ) ) ;
#30856=PLANE ( 'NONE',  #20348 ) ;
#30857=CARTESIAN_POINT ( 'NONE',  ( -18.59502454995801912, 0.000000000000000000, 5.414360484435545295 ) ) ;
#30858=ORIENTED_EDGE ( 'NONE', *, *, #50821, .F. ) ;
#30859=DIRECTION ( 'NONE',  ( 0.000000000000000000, -0.000000000000000000, -1.000000000000000000 ) ) ;
#30860=ORIENTED_EDGE ( 'NONE', *, *, #43720, .T. ) ;
#30861=CARTESIAN_POINT ( 'NONE',  ( -17.55053657858433169, -3.756034771668162797, 3.578708368817510532 ) ) ;
#30862=FACE_OUTER_BOUND ( 'NONE', #21535, .T. ) ;
#30863=ADVANCED_FACE ( 'NONE', ( #33040 ), #6639, .F. ) ;
#30864=VECTOR ( 'NONE', #12079, 999.9999999999998863 ) ;
#30865=LINE ( 'NONE', #1028, #14248 ) ;
#30866=FACE_OUTER_BOUND ( 'NONE', #37969, .T. ) ;
#30867=CARTESIAN_POINT ( 'NONE',  ( -20.06177075545399191, 0.000000000000000000, 14.76272000528038220 ) ) ;
#30869=DIRECTION ( 'NONE',  ( 0.005002170337468016433, -0.7660444431189770143, -0.6427681459581293666 ) ) ;
#30870=PLANE ( 'NONE',  #21346 ) ;
#30871=EDGE_LOOP ( 'NONE', ( #31961, #25212, #51009, #44877 ) ) ;
#30872=CARTESIAN_POINT ( 'NONE',  ( -12.60458797795435615, 0.000000000000000000, 11.86609696750642229 ) ) ;
#30873=LINE ( 'NONE', #36015, #22909 ) ;
#30874=DIRECTION ( 'NONE',  ( 0.005002170337468016433, -0.7660444431189770143, -0.6427681459581293666 ) ) ;
#30875=LINE ( 'NONE', #26086, #53523 ) ;
#30877=PLANE ( 'NONE',  #43139 ) ;
#30878=FACE_OUTER_BOUND ( 'NONE', #51845, .T. ) ;
#30879=DIRECTION ( 'NONE',  ( -0.005002170337468016433, -0.7660444431189770143, 0.6427681459581293666 ) ) ;
#30880=EDGE_LOOP ( 'NONE', ( #13415, #17730, #16237, #34181 ) ) ;
#30881=DIRECTION ( 'NONE',  ( -0.005002170337468016433, -0.7660444431189770143, 0.6427681459581293666 ) ) ;
#30882=CARTESIAN_POINT ( 'NONE',  ( -18.67619601524082285, 0.000000000000000000, 3.936400510096834893 ) ) ;
#30883=FACE_OUTER_BOUND ( 'NONE', #30127, .T. ) ;
#30884=LINE ( 'NONE', #38866, #49077 ) ;
#30885=EDGE_CURVE ( 'NONE', #53603, #11768, #41819, .T. ) ;
#30886=CARTESIAN_POINT ( 'NONE',  ( -30.79567442779373110, 0.000000000000000000, 8.843406890442315316 ) ) ;
#30887=PLANE ( 'NONE',  #32287 ) ;
#30888=LINE ( 'NONE', #9617, #42829 ) ;
#30890=DIRECTION ( 'NONE',  ( 0.005961354470445682716, -0.6427876096865404731, -0.7660212471507180654 ) ) ;
#30891=EDGE_CURVE ( 'NONE', #21366, #36639, #20550, .T. ) ;
#30892=ORIENTED_EDGE ( 'NONE', *, *, #55208, .T. ) ;
#30893=VECTOR ( 'NONE', #9071, 1000.000000000000114 ) ;
#30894=EDGE_CURVE ( 'NONE', #345, #51439, #11469, .T. ) ;
#30895=EDGE_CURVE ( 'NONE', #29778, #22415, #10896, .T. ) ;
#30896=AXIS2_PLACEMENT_3D ( 'NONE', #35296, #906, #18514 ) ;
#30897=ORIENTED_EDGE ( 'NONE', *, *, #52635, .T. ) ;
#30898=ORIENTED_EDGE ( 'NONE', *, *, #45389, .T. ) ;
#30899=ORIENTED_EDGE ( 'NONE', *, *, #25193, .T. ) ;
#30900=VERTEX_POINT ( 'NONE', #50900 ) ;
#30901=DIRECTION ( 'NONE',  ( -0.005002170337468016433, -0.7660444431189770143, 0.6427681459581293666 ) ) ;
#30902=EDGE_CURVE ( 'NONE', #39497, #44937, #37031, .T. ) ;
#30904=EDGE_LOOP ( 'NONE', ( #4933, #51403, #18928, #22489 ) ) ;
#30905=EDGE_CURVE ( 'NONE', #1854, #53450, #15701, .T. ) ;
#30906=ORIENTED_EDGE ( 'NONE', *, *, #32410, .T. ) ;
#30907=EDGE_CURVE ( 'NONE', #22464, #49826, #24501, .T. ) ;
#30909=ORIENTED_EDGE ( 'NONE', *, *, #1471, .F. ) ;
#30910=CARTESIAN_POINT ( 'NONE',  ( -8.571689109027634146, 0.000000000000000000, 5.323038384920776522 ) ) ;
#30911=DIRECTION ( 'NONE',  ( -0.005961354470445682716, -0.6427876096865404731, 0.7660212471507180654 ) ) ;
#30913=DIRECTION ( 'NONE',  ( 0.000000000000000000, -0.000000000000000000, -1.000000000000000000 ) ) ;
#30914=ADVANCED_FACE ( 'NONE', ( #32500 ), #2909, .F. ) ;
#30915=VERTEX_POINT ( 'NONE', #33588 ) ;
#30916=AXIS2_PLACEMENT_3D ( 'NONE', #20986, #16740, #34351 ) ;
#30917=PLANE ( 'NONE',  #30075 ) ;
#30918=PLANE ( 'NONE',  #9334 ) ;
#30919=ADVANCED_FACE ( 'NONE', ( #32745 ), #55179, .F. ) ;
#30920=DIRECTION ( 'NONE',  ( -0.9999697198139514409, -0.000000000000000000, -0.007781995580013368816 ) ) ;
#30921=DIRECTION ( 'NONE',  ( -0.005002170337468016433, -0.7660444431189770143, 0.6427681459581293666 ) ) ;
#30922=VERTEX_POINT ( 'NONE', #37576 ) ;
#30923=CARTESIAN_POINT ( 'NONE',  ( -14.20280369269832832, 0.000000000000000000, 12.40765738797303719 ) ) ;
#30924=CARTESIAN_POINT ( 'NONE',  ( -16.03461999353783440, 0.000000000000000000, 8.958280829210268692 ) ) ;
#30925=LINE ( 'NONE', #18733, #1240 ) ;
#30926=ORIENTED_EDGE ( 'NONE', *, *, #39477, .F. ) ;
#30927=DIRECTION ( 'NONE',  ( 0.007781995580012663651, 0.000000000000000000, -0.9999697198139515519 ) ) ;
#30928=ORIENTED_EDGE ( 'NONE', *, *, #24306, .T. ) ;
#30929=VECTOR ( 'NONE', #41670, 999.9999999999998863 ) ;
#30930=DIRECTION ( 'NONE',  ( 0.005002170337468016433, -0.7660444431189770143, -0.6427681459581293666 ) ) ;
#30931=CARTESIAN_POINT ( 'NONE',  ( -8.704836502503972895, 0.000000000000000000, 4.583338061504010241 ) ) ;
#30932=LINE ( 'NONE', #39173, #10455 ) ;
#30933=CARTESIAN_POINT ( 'NONE',  ( -17.26532721389163072, 0.000000000000000000, 13.67648636611514590 ) ) ;
#30935=DIRECTION ( 'NONE',  ( -0.6246952433987894571, 0.7422098413412802076, 0.2426528472758539834 ) ) ;
#30936=LINE ( 'NONE', #48553, #42480 ) ;
#30937=VECTOR ( 'NONE', #10146, 999.9999999999998863 ) ;
#30938=DIRECTION ( 'NONE',  ( 0.007781995580012663651, 0.000000000000000000, -0.9999697198139515519 ) ) ;
#30939=LINE ( 'NONE', #268, #15997 ) ;
#30940=ORIENTED_EDGE ( 'NONE', *, *, #2447, .T. ) ;
#30941=LINE ( 'NONE', #48251, #4866 ) ;
#30942=DIRECTION ( 'NONE',  ( -0.6427681459581293666, -0.7660444431189770143, -0.005002170337467561935 ) ) ;
#30943=CARTESIAN_POINT ( 'NONE',  ( -12.56492345065575122, 0.000000000000000000, 6.769290391155751152 ) ) ;
#30944=DIRECTION ( 'NONE',  ( 0.5449076811759707706, 0.6444004775717708799, -0.5364919789714476250 ) ) ;
#30945=EDGE_CURVE ( 'NONE', #7012, #15750, #33336, .T. ) ;
#30946=PLANE ( 'NONE',  #35093 ) ;
#30947=DIRECTION ( 'NONE',  ( 0.9999697198139515519, 0.000000000000000000, 0.007781995580013368816 ) ) ;
#30948=ORIENTED_EDGE ( 'NONE', *, *, #3499, .F. ) ;
#30949=ORIENTED_EDGE ( 'NONE', *, *, #12536, .F. ) ;
#30950=LINE ( 'NONE', #17625, #48579 ) ;
#30951=DIRECTION ( 'NONE',  ( 0.9999697198139515519, 0.000000000000000000, 0.007781995580013368816 ) ) ;
#30952=EDGE_CURVE ( 'NONE', #22163, #6183, #28210, .T. ) ;
#30953=VECTOR ( 'NONE', #12164, 999.9999999999998863 ) ;
#30954=VECTOR ( 'NONE', #43093, 1000.000000000000227 ) ;
#30955=VERTEX_POINT ( 'NONE', #42411 ) ;
#30956=DIRECTION ( 'NONE',  ( 0.6427681459581294776, -0.7660444431189769032, 0.005002170337467562802 ) ) ;
#30958=DIRECTION ( 'NONE',  ( 0.5364919789714477361, 0.6444004775717706579, 0.5449076811759711036 ) ) ;
#30959=EDGE_CURVE ( 'NONE', #19103, #44937, #11167, .T. ) ;
#30960=VERTEX_POINT ( 'NONE', #45521 ) ;
#30961=VERTEX_POINT ( 'NONE', #24790 ) ;
#30962=VERTEX_POINT ( 'NONE', #50641 ) ;
#30963=CARTESIAN_POINT ( 'NONE',  ( -12.54269775668131714, 2.553033558614008047, 1.472486354876782810 ) ) ;
#30964=CARTESIAN_POINT ( 'NONE',  ( -12.54193102261348969, 0.000000000000000000, 3.814812765093635871 ) ) ;
#30965=CARTESIAN_POINT ( 'NONE',  ( -14.14158376411010387, 0.000000000000000000, 4.541028037189134281 ) ) ;
#30966=LINE ( 'NONE', #9967, #33005 ) ;
#30967=EDGE_CURVE ( 'NONE', #42922, #50620, #23954, .T. ) ;
#30968=ORIENTED_EDGE ( 'NONE', *, *, #13028, .F. ) ;
#30969=ORIENTED_EDGE ( 'NONE', *, *, #8740, .T. ) ;
#30970=VECTOR ( 'NONE', #46261, 1000.000000000000227 ) ;
#30971=EDGE_CURVE ( 'NONE', #39202, #12878, #343, .T. ) ;
#30972=DIRECTION ( 'NONE',  ( 0.005002170337468016433, -0.7660444431189770143, -0.6427681459581293666 ) ) ;
#30973=ORIENTED_EDGE ( 'NONE', *, *, #18086, .F. ) ;
#30974=LINE ( 'NONE', #9406, #30059 ) ;
#30976=DIRECTION ( 'NONE',  ( -0.6427681459581293666, -0.7660444431189770143, -0.005002170337467561935 ) ) ;
#30977=DIRECTION ( 'NONE',  ( -0.005961354470445682716, -0.6427876096865404731, 0.7660212471507180654 ) ) ;
#30978=EDGE_CURVE ( 'NONE', #13435, #19083, #17126, .T. ) ;
#30979=ORIENTED_EDGE ( 'NONE', *, *, #22007, .F. ) ;
#30980=CARTESIAN_POINT ( 'NONE',  ( -25.20123094555300369, 0.000000000000000000, 6.470945668149052032 ) ) ;
#30981=EDGE_LOOP ( 'NONE', ( #9782, #11197, #24829 ) ) ;
#30982=FACE_OUTER_BOUND ( 'NONE', #54170, .T. ) ;
#30983=ORIENTED_EDGE ( 'NONE', *, *, #52628, .T. ) ;
#30984=LINE ( 'NONE', #48303, #1355 ) ;
#30985=LINE ( 'NONE', #887, #43849 ) ;
#30986=LINE ( 'NONE', #25926, #27349 ) ;
#30987=VERTEX_POINT ( 'NONE', #12310 ) ;
#30988=VECTOR ( 'NONE', #6455, 1000.000000000000227 ) ;
#30989=DIRECTION ( 'NONE',  ( 0.7660212471507180654, -0.6427876096865404731, 0.005961354470445141482 ) ) ;
#30990=VECTOR ( 'NONE', #20225, 1000.000000000000227 ) ;
#30991=FACE_OUTER_BOUND ( 'NONE', #14189, .T. ) ;
#30992=DIRECTION ( 'NONE',  ( 0.000000000000000000, -0.000000000000000000, -1.000000000000000000 ) ) ;
#30993=CARTESIAN_POINT ( 'NONE',  ( 2.072287782118878319, 0.000000000000000000, -2.950529333540147015 ) ) ;
#30994=PLANE ( 'NONE',  #55774 ) ;
#30995=DIRECTION ( 'NONE',  ( -0.005002170337468016433, -0.7660444431189770143, 0.6427681459581293666 ) ) ;
#30996=PLANE ( 'NONE',  #9527 ) ;
#30997=AXIS2_PLACEMENT_3D ( 'NONE', #18313, #9828, #40184 ) ;
#30998=EDGE_LOOP ( 'NONE', ( #44812, #44518, #19990, #32670 ) ) ;
#30999=DIRECTION ( 'NONE',  ( -0.9321478471874540261, 0.000000000000000000, 0.3620778797217457656 ) ) ;
#31000=PLANE ( 'NONE',  #43144 ) ;
#31001=DIRECTION ( 'NONE',  ( -0.6427681459581293666, -0.7660444431189770143, -0.005002170337467561935 ) ) ;
#31002=ORIENTED_EDGE ( 'NONE', *, *, #34843, .T. ) ;
#31003=LINE ( 'NONE', #43514, #40173 ) ;
#31004=DIRECTION ( 'NONE',  ( 0.9999697198139515519, 0.000000000000000000, 0.007781995580013368816 ) ) ;
#31005=ORIENTED_EDGE ( 'NONE', *, *, #25278, .F. ) ;
#31006=ADVANCED_FACE ( 'NONE', ( #12590 ), #9149, .F. ) ;
#31007=DIRECTION ( 'NONE',  ( 0.007781995580012663651, -3.146120232559066537E-19, -0.9999697198139514409 ) ) ;
#31008=DIRECTION ( 'NONE',  ( 0.5449076811759707706, 0.6444004775717708799, -0.5364919789714476250 ) ) ;
#31009=AXIS2_PLACEMENT_3D ( 'NONE', #40285, #13873, #18133 ) ;
#31010=ADVANCED_FACE ( 'NONE', ( #42955 ), #4899, .F. ) ;
#31011=LINE ( 'NONE', #9444, #49554 ) ;
#31012=AXIS2_PLACEMENT_3D ( 'NONE', #18571, #14868, #52924 ) ;
#31013=CARTESIAN_POINT ( 'NONE',  ( -15.88130887279446490, 0.000000000000000000, 3.050160814894388839 ) ) ;
#31014=ORIENTED_EDGE ( 'NONE', *, *, #19743, .F. ) ;
#31015=ORIENTED_EDGE ( 'NONE', *, *, #173, .T. ) ;
#31016=ADVANCED_FACE ( 'NONE', ( #49 ), #4362, .F. ) ;
#31017=DIRECTION ( 'NONE',  ( 0.5364919789714477361, 0.6444004775717706579, 0.5449076811759711036 ) ) ;
#31018=DIRECTION ( 'NONE',  ( 0.7660212471507180654, -0.6427876096865404731, 0.005961354470445141482 ) ) ;
#31019=CARTESIAN_POINT ( 'NONE',  ( -9.766923509977383233, 0.000000000000000000, 5.483062808027726831 ) ) ;
#31020=ADVANCED_FACE ( 'NONE', ( #34437 ), #46951, .F. ) ;
#31021=ADVANCED_FACE ( 'NONE', ( #30481 ), #43783, .F. ) ;
#31023=CARTESIAN_POINT ( 'NONE',  ( -21.47263955680318404, 0.000000000000000000, 5.022634149262071190 ) ) ;
#31024=CARTESIAN_POINT ( 'NONE',  ( -17.96341130604493941, 4.010151117816511679, 3.531585906670110742 ) ) ;
#31025=LINE ( 'NONE', #39004, #16737 ) ;
#31026=ORIENTED_EDGE ( 'NONE', *, *, #46881, .F. ) ;
#31027=DIRECTION ( 'NONE',  ( -0.7660212471507179544, -0.6427876096865405842, -0.005961354470445141482 ) ) ;
#31028=DIRECTION ( 'NONE',  ( 0.007781995580012663651, 0.000000000000000000, -0.9999697198139515519 ) ) ;
#31029=VERTEX_POINT ( 'NONE', #17684 ) ;
#31030=DIRECTION ( 'NONE',  ( 0.6427681459581294776, -0.7660444431189769032, 0.005002170337467562802 ) ) ;
#31031=VECTOR ( 'NONE', #19841, 999.9999999999998863 ) ;
#31032=FACE_OUTER_BOUND ( 'NONE', #52143, .T. ) ;
#31033=LINE ( 'NONE', #48663, #17548 ) ;
#31034=VERTEX_POINT ( 'NONE', #8609 ) ;
#31035=AXIS2_PLACEMENT_3D ( 'NONE', #7489, #12023, #50080 ) ;
#31036=VECTOR ( 'NONE', #1390, 999.9999999999998863 ) ;
#31037=PLANE ( 'NONE',  #54768 ) ;
#31039=ORIENTED_EDGE ( 'NONE', *, *, #16396, .F. ) ;
#31040=EDGE_CURVE ( 'NONE', #21773, #2815, #38983, .T. ) ;
#31041=ORIENTED_EDGE ( 'NONE', *, *, #51080, .F. ) ;
#31042=VECTOR ( 'NONE', #26942, 999.9999999999998863 ) ;
#31043=ORIENTED_EDGE ( 'NONE', *, *, #20352, .T. ) ;
#31044=VECTOR ( 'NONE', #29561, 1000.000000000000227 ) ;
#31045=EDGE_CURVE ( 'NONE', #44182, #5782, #34713, .T. ) ;
#31046=VERTEX_POINT ( 'NONE', #13148 ) ;
#31048=ORIENTED_EDGE ( 'NONE', *, *, #34700, .T. ) ;
#31049=CARTESIAN_POINT ( 'NONE',  ( -14.82067173329432563, 1.905425754524005200, 5.765301610339943039 ) ) ;
#31050=CARTESIAN_POINT ( 'NONE',  ( -14.56888064431065821, -0.1191753592594197858, 12.58947452739191064 ) ) ;
#31052=ORIENTED_EDGE ( 'NONE', *, *, #49383, .T. ) ;
#31054=EDGE_LOOP ( 'NONE', ( #23306, #3137, #13497, #28175 ) ) ;
#31055=DIRECTION ( 'NONE',  ( 0.6427681459581294776, -0.7660444431189769032, 0.005002170337467562802 ) ) ;
#31056=VECTOR ( 'NONE', #54323, 1000.000000000000227 ) ;
#31057=ORIENTED_EDGE ( 'NONE', *, *, #52829, .F. ) ;
#31058=ADVANCED_FACE ( 'NONE', ( #21926 ), #35024, .F. ) ;
#31059=CARTESIAN_POINT ( 'NONE',  ( -17.74404816805336793, 0.000000000000000000, 3.574322630375089460 ) ) ;
#31060=LINE ( 'NONE', #49219, #52870 ) ;
#31061=DIRECTION ( 'NONE',  ( -0.005002170337468016433, -0.7660444431189770143, 0.6427681459581293666 ) ) ;
#31063=CARTESIAN_POINT ( 'NONE',  ( -17.23833534428622372, 2.553033558614007603, 7.767238996852877442 ) ) ;
#31064=PLANE ( 'NONE',  #13832 ) ;
#31065=EDGE_LOOP ( 'NONE', ( #11186, #10767, #12966, #3705 ) ) ;
#31066=ORIENTED_EDGE ( 'NONE', *, *, #13350, .T. ) ;
#31067=CARTESIAN_POINT ( 'NONE',  ( -12.98834176436399623, -3.270328918600660995, 7.094211661635224431 ) ) ;
#31068=LINE ( 'NONE', #9504, #10370 ) ;
#31070=CARTESIAN_POINT ( 'NONE',  ( -19.76861662533108799, -0.8417996532631553119, 5.742270417481394773 ) ) ;
#31071=CARTESIAN_POINT ( 'NONE',  ( -16.01294521988485542, 0.000000000000000000, 6.173118962443128410 ) ) ;
#31072=ORIENTED_EDGE ( 'NONE', *, *, #53852, .T. ) ;
#31073=FACE_OUTER_BOUND ( 'NONE', #9728, .T. ) ;
#31074=LINE ( 'NONE', #48965, #54056 ) ;
#31075=ORIENTED_EDGE ( 'NONE', *, *, #45570, .F. ) ;
#31076=VECTOR ( 'NONE', #52382, 1000.000000000000114 ) ;
#31078=CARTESIAN_POINT ( 'NONE',  ( -19.23669273636768295, -2.946525016555658905, 8.989866006152718469 ) ) ;
#31080=VECTOR ( 'NONE', #7281, 1000.000000000000227 ) ;
#31081=VECTOR ( 'NONE', #34502, 1000.000000000000227 ) ;
#31082=CARTESIAN_POINT ( 'NONE',  ( -9.542064456761055524, 0.000000000000000000, 10.59726798936431180 ) ) ;
#31083=DIRECTION ( 'NONE',  ( 0.9999697198139515519, 0.000000000000000000, 0.007781995580013368816 ) ) ;
#31084=DIRECTION ( 'NONE',  ( -0.5364919789714478471, 0.6444004775717705469, -0.5449076811759709926 ) ) ;
#31085=CARTESIAN_POINT ( 'NONE',  ( -9.971347906561460306, 0.000000000000000000, 6.050810056132276848 ) ) ;
#31086=CARTESIAN_POINT ( 'NONE',  ( -19.60912206198628027, -0.1191753592594197858, 4.398475361799976113 ) ) ;
#31087=VERTEX_POINT ( 'NONE', #30753 ) ;
#31088=VECTOR ( 'NONE', #14089, 999.9999999999998863 ) ;
#31089=VECTOR ( 'NONE', #20939, 999.9999999999998863 ) ;
#31090=ORIENTED_EDGE ( 'NONE', *, *, #46792, .T. ) ;
#31091=DIRECTION ( 'NONE',  ( 0.9999697198139515519, 0.000000000000000000, 0.007781995580013368816 ) ) ;
#31092=DIRECTION ( 'NONE',  ( 0.007781995580012663651, -3.146120232559066537E-19, -0.9999697198139514409 ) ) ;
#31093=LINE ( 'NONE', #13238, #39689 ) ;
#31094=EDGE_CURVE ( 'NONE', #15067, #9201, #33877, .T. ) ;
#31095=ADVANCED_FACE ( 'NONE', ( #8053 ), #25364, .F. ) ;
#31096=CARTESIAN_POINT ( 'NONE',  ( -15.14133055664494520, -3.108426967578160838, 2.663553012464920933 ) ) ;
#31097=VECTOR ( 'NONE', #30093, 999.9999999999998863 ) ;
#31098=CARTESIAN_POINT ( 'NONE',  ( -11.67244013076689946, 0.000000000000000000, 11.50401908778467863 ) ) ;
#31099=EDGE_LOOP ( 'NONE', ( #55669, #1984, #52073, #44455 ) ) ;
#31100=EDGE_CURVE ( 'NONE', #18224, #11899, #14285, .T. ) ;
#31101=CARTESIAN_POINT ( 'NONE',  ( -12.08016817927768827, 0.000000000000000000, 4.187738380119410131 ) ) ;
#31102=VECTOR ( 'NONE', #13406, 999.9999999999998863 ) ;
#31103=CARTESIAN_POINT ( 'NONE',  ( -9.046265820773848887, 0.000000000000000000, 6.596667342221034680 ) ) ;
#31105=DIRECTION ( 'NONE',  ( 0.005961354470445682716, -0.6427876096865404731, -0.7660212471507180654 ) ) ;
#31106=ORIENTED_EDGE ( 'NONE', *, *, #11307, .T. ) ;
#31107=PLANE ( 'NONE',  #4745 ) ;
#31108=ORIENTED_EDGE ( 'NONE', *, *, #25529, .T. ) ;
#31109=CARTESIAN_POINT ( 'NONE',  ( -13.10003858486740214, -0.1191753592594189115, 2.971802275270698956 ) ) ;
#31110=VECTOR ( 'NONE', #21067, 1000.000000000000114 ) ;
#31111=LINE ( 'NONE', #22035, #10292 ) ;
#31112=EDGE_LOOP ( 'NONE', ( #11579, #11890, #4447, #54221 ) ) ;
#31113=LINE ( 'NONE', #36231, #3621 ) ;
#31114=AXIS2_PLACEMENT_3D ( 'NONE', #9752, #47809, #22782 ) ;
#31115=ORIENTED_EDGE ( 'NONE', *, *, #17717, .T. ) ;
#31116=ORIENTED_EDGE ( 'NONE', *, *, #2135, .F. ) ;
#31117=ORIENTED_EDGE ( 'NONE', *, *, #52634, .F. ) ;
#31118=LINE ( 'NONE', #30069, #2091 ) ;
#31119=ORIENTED_EDGE ( 'NONE', *, *, #49776, .T. ) ;
#31120=ORIENTED_EDGE ( 'NONE', *, *, #20232, .T. ) ;
#31121=VECTOR ( 'NONE', #9958, 1000.000000000000227 ) ;
#31122=PLANE ( 'NONE',  #25671 ) ;
#31123=DIRECTION ( 'NONE',  ( 0.005002170337468016433, -0.7660444431189770143, -0.6427681459581293666 ) ) ;
#31124=ORIENTED_EDGE ( 'NONE', *, *, #37045, .F. ) ;
#31125=AXIS2_PLACEMENT_3D ( 'NONE', #13244, #47882, #43884 ) ;
#31126=AXIS2_PLACEMENT_3D ( 'NONE', #21310, #51954, #21605 ) ;
#31127=ORIENTED_EDGE ( 'NONE', *, *, #3561, .T. ) ;
#31128=CARTESIAN_POINT ( 'NONE',  ( -16.40420069433451289, -0.1191753592594190225, 9.590322214343837359 ) ) ;
#31129=ORIENTED_EDGE ( 'NONE', *, *, #6086, .T. ) ;
#31130=ORIENTED_EDGE ( 'NONE', *, *, #13620, .F. ) ;
#31131=EDGE_CURVE ( 'NONE', #29285, #2305, #52863, .T. ) ;
#31132=AXIS2_PLACEMENT_3D ( 'NONE', #24676, #6532, #49706 ) ;
#31133=AXIS2_PLACEMENT_3D ( 'NONE', #52034, #29910, #34440 ) ;
#31134=DIRECTION ( 'NONE',  ( -0.6427681459581293666, -0.7660444431189770143, -0.005002170337467561935 ) ) ;
#31135=EDGE_CURVE ( 'NONE', #34678, #39202, #649, .T. ) ;
#31136=CARTESIAN_POINT ( 'NONE',  ( -21.47341775636118655, -0.1191753592594197858, 5.122631121243466090 ) ) ;
#31137=DIRECTION ( 'NONE',  ( 0.005961354470445682716, -0.6427876096865404731, -0.7660212471507180654 ) ) ;
#31138=ADVANCED_FACE ( 'NONE', ( #1178 ), #31000, .F. ) ;
#31139=ORIENTED_EDGE ( 'NONE', *, *, #31740, .T. ) ;
#31140=LINE ( 'NONE', #30309, #49133 ) ;
#31141=VERTEX_POINT ( 'NONE', #6306 ) ;
#31142=EDGE_CURVE ( 'NONE', #13383, #14078, #35854, .T. ) ;
#31143=CARTESIAN_POINT ( 'NONE',  ( -10.96854034462895555, 0.1245042932765021287, 1.346207436594613505 ) ) ;
#31144=AXIS2_PLACEMENT_3D ( 'NONE', #29089, #20851, #50406 ) ;
#31145=DIRECTION ( 'NONE',  ( 0.7660212471507180654, -0.6427876096865404731, 0.005961354470445141482 ) ) ;
#31146=DIRECTION ( 'NONE',  ( 0.005961354470445682716, -0.6427876096865404731, -0.7660212471507180654 ) ) ;
#31147=LINE ( 'NONE', #4479, #16871 ) ;
#31149=LINE ( 'NONE', #22072, #42992 ) ;
#31150=DIRECTION ( 'NONE',  ( 0.9321478471874541372, 0.000000000000000000, -0.3620778797217453771 ) ) ;
#31151=ORIENTED_EDGE ( 'NONE', *, *, #13746, .F. ) ;
#31152=DIRECTION ( 'NONE',  ( 0.9999697198139515519, 0.000000000000000000, 0.007781995580013368816 ) ) ;
#31153=VECTOR ( 'NONE', #55039, 1000.000000000000000 ) ;
#31154=DIRECTION ( 'NONE',  ( 0.007781995580012663651, -3.146120232559066537E-19, -0.9999697198139514409 ) ) ;
#31155=DIRECTION ( 'NONE',  ( -0.005002170337468016433, -0.7660444431189770143, 0.6427681459581293666 ) ) ;
#31156=LINE ( 'NONE', #8185, #20847 ) ;
#31157=AXIS2_PLACEMENT_3D ( 'NONE', #8922, #30771, #21691 ) ;
#31158=PLANE ( 'NONE',  #14992 ) ;
#31159=LINE ( 'NONE', #39414, #17720 ) ;
#31160=CARTESIAN_POINT ( 'NONE',  ( 2.072287782118878319, 0.000000000000000000, -2.950529333540147015 ) ) ;
#31161=DIRECTION ( 'NONE',  ( 0.7660212471507180654, -0.6427876096865404731, 0.005961354470445141482 ) ) ;
#31162=VERTEX_POINT ( 'NONE', #14817 ) ;
#31163=AXIS2_PLACEMENT_3D ( 'NONE', #17156, #24828, #80 ) ;
#31164=LINE ( 'NONE', #43652, #32951 ) ;
#31165=LINE ( 'NONE', #44244, #3117 ) ;
#31166=FACE_OUTER_BOUND ( 'NONE', #46886, .T. ) ;
#31167=VECTOR ( 'NONE', #5507, 999.9999999999998863 ) ;
#31168=VECTOR ( 'NONE', #48374, 999.9999999999998863 ) ;
#31169=EDGE_CURVE ( 'NONE', #45628, #41178, #53440, .T. ) ;
#31170=DIRECTION ( 'NONE',  ( -0.5364919789714478471, 0.6444004775717705469, -0.5449076811759709926 ) ) ;
#31171=FACE_OUTER_BOUND ( 'NONE', #28970, .T. ) ;
#31172=CARTESIAN_POINT ( 'NONE',  ( -10.27421835998572064, 0.000000000000000000, 10.96090226820206048 ) ) ;
#31173=EDGE_CURVE ( 'NONE', #14388, #46093, #14538, .T. ) ;
#31174=EDGE_CURVE ( 'NONE', #36024, #51395, #10585, .T. ) ;
#31175=DIRECTION ( 'NONE',  ( 0.5364919789714477361, 0.6444004775717706579, 0.5449076811759711036 ) ) ;
#31176=AXIS2_PLACEMENT_3D ( 'NONE', #37749, #54469, #50220 ) ;
#31177=VECTOR ( 'NONE', #28088, 999.9999999999998863 ) ;
#31178=DIRECTION ( 'NONE',  ( -0.9999697198139514409, -0.000000000000000000, -0.007781995580013368816 ) ) ;
#31179=CARTESIAN_POINT ( 'NONE',  ( -11.35088832955830007, 0.000000000000000000, 4.193413804539424916 ) ) ;
#31180=ORIENTED_EDGE ( 'NONE', *, *, #50755, .T. ) ;
#31181=EDGE_CURVE ( 'NONE', #14703, #34243, #17969, .T. ) ;
#31182=ORIENTED_EDGE ( 'NONE', *, *, #33034, .F. ) ;
#31183=VERTEX_POINT ( 'NONE', #27898 ) ;
#31184=EDGE_LOOP ( 'NONE', ( #43612, #9685, #32499, #2331 ) ) ;
#31185=AXIS2_PLACEMENT_3D ( 'NONE', #43238, #56009, #55416 ) ;
#31186=VERTEX_POINT ( 'NONE', #45204 ) ;
#31187=DIRECTION ( 'NONE',  ( 0.7660212471507180654, -0.6427876096865404731, 0.005961354470445141482 ) ) ;
#31188=DIRECTION ( 'NONE',  ( -0.9999697198139514409, -0.000000000000000000, -0.007781995580013368816 ) ) ;
#31189=VECTOR ( 'NONE', #2635, 1000.000000000000227 ) ;
#31190=ORIENTED_EDGE ( 'NONE', *, *, #29656, .T. ) ;
#31191=ORIENTED_EDGE ( 'NONE', *, *, #10414, .T. ) ;
#31192=VECTOR ( 'NONE', #26325, 1000.000000000000227 ) ;
#31193=PLANE ( 'NONE',  #2066 ) ;
#31194=VERTEX_POINT ( 'NONE', #40384 ) ;
#31197=LINE ( 'NONE', #27219, #31392 ) ;
#31198=ORIENTED_EDGE ( 'NONE', *, *, #43720, .F. ) ;
#31199=DIRECTION ( 'NONE',  ( 0.5449076811759707706, 0.6444004775717708799, -0.5364919789714476250 ) ) ;
#31200=VECTOR ( 'NONE', #31839, 1000.000000000000000 ) ;
#31201=ORIENTED_EDGE ( 'NONE', *, *, #6249, .F. ) ;
#31202=CARTESIAN_POINT ( 'NONE',  ( -9.542064456761055524, 0.000000000000000000, 10.59726798936431180 ) ) ;
#31203=EDGE_CURVE ( 'NONE', #17816, #11120, #36139, .T. ) ;
#31204=DIRECTION ( 'NONE',  ( 0.9321478471874541372, 0.000000000000000000, -0.3620778797217453771 ) ) ;
#31205=AXIS2_PLACEMENT_3D ( 'NONE', #46749, #12094, #3317 ) ;
#31206=LINE ( 'NONE', #44829, #52697 ) ;
#31207=CARTESIAN_POINT ( 'NONE',  ( -17.97791203186454112, 1.257817950434005683, 3.625032319110802259 ) ) ;
#31208=VECTOR ( 'NONE', #18044, 999.9999999999998863 ) ;
#31209=ORIENTED_EDGE ( 'NONE', *, *, #42887, .T. ) ;
#31210=CARTESIAN_POINT ( 'NONE',  ( -12.80323208052646855, 3.362543313726509719, 7.373037692220082207 ) ) ;
#31211=DIRECTION ( 'NONE',  ( 0.6246952433987894571, -0.7422098413412800966, -0.2426528472758541777 ) ) ;
#31212=DIRECTION ( 'NONE',  ( -0.7660212471507179544, -0.6427876096865405842, -0.005961354470445141482 ) ) ;
#31213=VERTEX_POINT ( 'NONE', #44926 ) ;
#31214=CARTESIAN_POINT ( 'NONE',  ( -17.46532115785441519, 0.000000000000000000, 13.67492996699914265 ) ) ;
#31216=ADVANCED_FACE ( 'NONE', ( #6040 ), #1744, .F. ) ;
#31217=LINE ( 'NONE', #14734, #25570 ) ;
#31218=LINE ( 'NONE', #34939, #8795 ) ;
#31219=DIRECTION ( 'NONE',  ( 0.005002170337468016433, -0.7660444431189770143, -0.6427681459581293666 ) ) ;
#31220=DIRECTION ( 'NONE',  ( 0.000000000000000000, -0.000000000000000000, -1.000000000000000000 ) ) ;
#31221=DIRECTION ( 'NONE',  ( -0.9999697198139514409, -0.000000000000000000, -0.007781995580013368816 ) ) ;
#31223=DIRECTION ( 'NONE',  ( 0.000000000000000000, -1.000000000000000000, 0.000000000000000000 ) ) ;
#31224=FACE_OUTER_BOUND ( 'NONE', #35196, .T. ) ;
#31225=EDGE_CURVE ( 'NONE', #10401, #20294, #19066, .T. ) ;
#31226=AXIS2_PLACEMENT_3D ( 'NONE', #29233, #51094, #167 ) ;
#31227=LINE ( 'NONE', #9363, #24749 ) ;
#31228=LINE ( 'NONE', #13901, #25984 ) ;
#31229=VERTEX_POINT ( 'NONE', #23353 ) ;
#31230=CARTESIAN_POINT ( 'NONE',  ( -26.13493519185646008, 0.000000000000000000, 7.033017491833586377 ) ) ;
#31231=DIRECTION ( 'NONE',  ( -0.5449076811759708816, 0.6444004775717707689, 0.5364919789714475140 ) ) ;
#31232=EDGE_CURVE ( 'NONE', #37122, #40408, #40672, .T. ) ;
#31233=DIRECTION ( 'NONE',  ( 0.007781995580012663651, -3.146120232559066537E-19, -0.9999697198139514409 ) ) ;
#31234=VECTOR ( 'NONE', #7983, 999.9999999999998863 ) ;
#31235=FACE_OUTER_BOUND ( 'NONE', #12324, .T. ) ;
#31236=ADVANCED_FACE ( 'NONE', ( #13686 ), #48319, .F. ) ;
#31237=PLANE ( 'NONE',  #20043 ) ;
#31238=DIRECTION ( 'NONE',  ( -0.5364919789714478471, 0.6444004775717705469, -0.5449076811759709926 ) ) ;
#31239=EDGE_CURVE ( 'NONE', #29528, #36994, #5737, .T. ) ;
#31240=DIRECTION ( 'NONE',  ( -0.7660212471507179544, -0.6427876096865405842, -0.005961354470445141482 ) ) ;
#31241=ORIENTED_EDGE ( 'NONE', *, *, #46948, .T. ) ;
#31242=VECTOR ( 'NONE', #50757, 999.9999999999998863 ) ;
#31243=VERTEX_POINT ( 'NONE', #18818 ) ;
#31245=VECTOR ( 'NONE', #11893, 999.9999999999998863 ) ;
#31246=DIRECTION ( 'NONE',  ( 0.9999697198139515519, 0.000000000000000000, 0.007781995580013368816 ) ) ;
#31247=VECTOR ( 'NONE', #56029, 1000.000000000000114 ) ;
#31248=EDGE_CURVE ( 'NONE', #36758, #36001, #40089, .T. ) ;
#31249=ORIENTED_EDGE ( 'NONE', *, *, #10930, .F. ) ;
#31250=DIRECTION ( 'NONE',  ( -0.5364919789714478471, 0.6444004775717705469, -0.5449076811759709926 ) ) ;
#31252=CARTESIAN_POINT ( 'NONE',  ( -18.66354898467281132, 0.000000000000000000, 14.21960318569776582 ) ) ;
#31253=EDGE_CURVE ( 'NONE', #40596, #15338, #54823, .T. ) ;
#31254=VECTOR ( 'NONE', #48070, 999.9999999999998863 ) ;
#31257=ORIENTED_EDGE ( 'NONE', *, *, #53005, .F. ) ;
#31258=ORIENTED_EDGE ( 'NONE', *, *, #37791, .T. ) ;
#31259=CARTESIAN_POINT ( 'NONE',  ( -16.79925329029790149, 0.000000000000000000, 13.49544742625427496 ) ) ;
#31260=DIRECTION ( 'NONE',  ( 0.9999697198139515519, 0.000000000000000000, 0.007781995580013368816 ) ) ;
#31261=DIRECTION ( 'NONE',  ( 0.5449076811759707706, 0.6444004775717708799, -0.5364919789714476250 ) ) ;
#31262=PLANE ( 'NONE',  #41992 ) ;
#31263=EDGE_LOOP ( 'NONE', ( #42064, #33188, #35880, #45556 ) ) ;
#31264=VERTEX_POINT ( 'NONE', #20168 ) ;
#31265=VECTOR ( 'NONE', #53641, 1000.000000000000227 ) ;
#31266=LINE ( 'NONE', #27278, #10052 ) ;
#31267=AXIS2_PLACEMENT_3D ( 'NONE', #36927, #32638, #49943 ) ;
#31268=EDGE_LOOP ( 'NONE', ( #17945, #45883, #18556, #38519 ) ) ;
#31269=PLANE ( 'NONE',  #35521 ) ;
#31270=ORIENTED_EDGE ( 'NONE', *, *, #22202, .F. ) ;
#31271=VECTOR ( 'NONE', #894, 999.9999999999998863 ) ;
#31272=CARTESIAN_POINT ( 'NONE',  ( -18.39746900504187010, 0.000000000000000000, 14.03700784672088808 ) ) ;
#31273=CARTESIAN_POINT ( 'NONE',  ( -12.33850799832341849, 0.000000000000000000, 11.68350162852954632 ) ) ;
#31274=ORIENTED_EDGE ( 'NONE', *, *, #34015, .F. ) ;
#31275=DIRECTION ( 'NONE',  ( 0.6427681459581294776, -0.7660444431189769032, 0.005002170337467562802 ) ) ;
#31276=EDGE_CURVE ( 'NONE', #39446, #50762, #45739, .T. ) ;
#31277=VECTOR ( 'NONE', #15610, 1000.000000000000227 ) ;
#31278=ORIENTED_EDGE ( 'NONE', *, *, #32631, .T. ) ;
#31279=CARTESIAN_POINT ( 'NONE',  ( -17.01269937210870964, 1.743523803501506819, 6.351050902876947291 ) ) ;
#31280=VECTOR ( 'NONE', #27346, 1000.000000000000227 ) ;
#31281=AXIS2_PLACEMENT_3D ( 'NONE', #28989, #50577, #55663 ) ;
#31282=EDGE_LOOP ( 'NONE', ( #39984, #1543, #22173, #12685 ) ) ;
#31283=LINE ( 'NONE', #886, #19612 ) ;
#31284=LINE ( 'NONE', #48614, #4859 ) ;
#31285=VECTOR ( 'NONE', #18759, 999.9999999999998863 ) ;
#31286=VECTOR ( 'NONE', #33156, 1000.000000000000227 ) ;
#31287=LINE ( 'NONE', #23049, #32821 ) ;
#31288=ORIENTED_EDGE ( 'NONE', *, *, #43627, .T. ) ;
#31289=AXIS2_PLACEMENT_3D ( 'NONE', #23057, #1473, #6034 ) ;
#31290=EDGE_CURVE ( 'NONE', #4086, #12666, #24715, .T. ) ;
#31291=FACE_OUTER_BOUND ( 'NONE', #619, .T. ) ;
#31292=PLANE ( 'NONE',  #20127 ) ;
#31293=LINE ( 'NONE', #35843, #23091 ) ;
#31295=LINE ( 'NONE', #14812, #25871 ) ;
#31296=DIRECTION ( 'NONE',  ( 0.005961354470445682716, -0.6427876096865404731, -0.7660212471507180654 ) ) ;
#31297=EDGE_CURVE ( 'NONE', #54809, #1909, #2584, .T. ) ;
#31298=VECTOR ( 'NONE', #12419, 999.9999999999998863 ) ;
#31299=VECTOR ( 'NONE', #2444, 1000.000000000000000 ) ;
#31300=( NAMED_UNIT ( * ) SI_UNIT ( $, .STERADIAN. ) SOLID_ANGLE_UNIT ( ) );
#31301=ORIENTED_EDGE ( 'NONE', *, *, #26168, .T. ) ;
#31302=PLANE ( 'NONE',  #15315 ) ;
#31303=CARTESIAN_POINT ( 'NONE',  ( -18.19192721912726896, 5.305366725996512045, 12.65469409231538833 ) ) ;
#31304=CARTESIAN_POINT ( 'NONE',  ( -17.74482636761137044, -0.1191753592594197858, 3.674319602356483916 ) ) ;
#31305=ORIENTED_EDGE ( 'NONE', *, *, #39409, .F. ) ;
#31306=DIRECTION ( 'NONE',  ( 0.005961354470445682716, -0.6427876096865404731, -0.7660212471507180654 ) ) ;
#31307=DIRECTION ( 'NONE',  ( 0.9999697198139515519, 0.000000000000000000, 0.007781995580013368816 ) ) ;
#31308=ORIENTED_EDGE ( 'NONE', *, *, #20248, .F. ) ;
#31309=LINE ( 'NONE', #13443, #51561 ) ;
#31310=EDGE_CURVE ( 'NONE', #2289, #1437, #49988, .T. ) ;
#31311=LINE ( 'NONE', #52343, #35727 ) ;
#31312=LINE ( 'NONE', #23071, #55913 ) ;
#31313=ADVANCED_FACE ( 'NONE', ( #28422 ), #37219, .F. ) ;
#31314=CARTESIAN_POINT ( 'NONE',  ( -9.752553242450971993, 0.000000000000000000, 3.636514291738904170 ) ) ;
#31315=AXIS2_PLACEMENT_3D ( 'NONE', #27390, #18899, #11751 ) ;
#31316=EDGE_LOOP ( 'NONE', ( #24080, #45473, #41300, #18467 ) ) ;
#31317=VERTEX_POINT ( 'NONE', #6867 ) ;
#31318=AXIS2_PLACEMENT_3D ( 'NONE', #3339, #52153, #51858 ) ;
#31319=CARTESIAN_POINT ( 'NONE',  ( -24.26986129792355129, -0.1191753592594197858, 6.208864760408702388 ) ) ;
#31320=DIRECTION ( 'NONE',  ( 0.000000000000000000, -0.000000000000000000, -1.000000000000000000 ) ) ;
#31322=AXIS2_PLACEMENT_3D ( 'NONE', #52653, #25707, #34791 ) ;
#31323=LINE ( 'NONE', #48651, #42004 ) ;
#31324=ADVANCED_FACE ( 'NONE', ( #23884 ), #36679, .F. ) ;
#31325=CARTESIAN_POINT ( 'NONE',  ( -21.47976836131305234, -2.298917212465657833, 8.798318018248513894 ) ) ;
#31326=FACE_OUTER_BOUND ( 'NONE', #36161, .T. ) ;
#31327=VECTOR ( 'NONE', #12140, 999.9999999999998863 ) ;
#31328=ORIENTED_EDGE ( 'NONE', *, *, #27610, .T. ) ;
#31329=LINE ( 'NONE', #1202, #37382 ) ;
#31330=EDGE_CURVE ( 'NONE', #10301, #17288, #45456, .T. ) ;
#31331=CARTESIAN_POINT ( 'NONE',  ( -15.88130887279446490, 0.000000000000000000, 3.050160814894388839 ) ) ;
#31332=VECTOR ( 'NONE', #1721, 1000.000000000000114 ) ;
#31333=AXIS2_PLACEMENT_3D ( 'NONE', #21514, #49211, #39862 ) ;
#31334=ORIENTED_EDGE ( 'NONE', *, *, #7725, .F. ) ;
#31335=FACE_OUTER_BOUND ( 'NONE', #5202, .T. ) ;
#31336=CARTESIAN_POINT ( 'NONE',  ( 2.072287782118878319, 0.000000000000000000, -2.950529333540147015 ) ) ;
#31337=CARTESIAN_POINT ( 'NONE',  ( -14.57595350043041194, -2.946525016555658905, 7.179476607543993083 ) ) ;
#31338=AXIS2_PLACEMENT_3D ( 'NONE', #36536, #49619, #45336 ) ;
#31339=VERTEX_POINT ( 'NONE', #46288 ) ;
#31340=VECTOR ( 'NONE', #27640, 1000.000000000000000 ) ;
#31341=PLANE ( 'NONE',  #24723 ) ;
#31342=ORIENTED_EDGE ( 'NONE', *, *, #38974, .F. ) ;
#31343=VECTOR ( 'NONE', #39593, 999.9999999999998863 ) ;
#31344=ORIENTED_EDGE ( 'NONE', *, *, #6851, .F. ) ;
#31345=VECTOR ( 'NONE', #5200, 1000.000000000000227 ) ;
#31346=ORIENTED_EDGE ( 'NONE', *, *, #45485, .T. ) ;
#31347=EDGE_LOOP ( 'NONE', ( #38904, #1303, #46683, #48442 ) ) ;
#31348=LINE ( 'NONE', #13726, #43872 ) ;
#31349=ORIENTED_EDGE ( 'NONE', *, *, #8250, .T. ) ;
#31351=DIRECTION ( 'NONE',  ( 0.007781995580012662783, 0.000000000000000000, -0.9999697198139514409 ) ) ;
#31352=ORIENTED_EDGE ( 'NONE', *, *, #20846, .F. ) ;
#31353=DIRECTION ( 'NONE',  ( 0.007781995580012663651, 0.000000000000000000, -0.9999697198139515519 ) ) ;
#31354=EDGE_LOOP ( 'NONE', ( #1146, #8910, #37256, #16609 ) ) ;
#31355=DIRECTION ( 'NONE',  ( 0.007781995580012662783, 0.000000000000000000, -0.9999697198139514409 ) ) ;
#31356=EDGE_CURVE ( 'NONE', #34418, #54919, #40924, .T. ) ;
#31357=ORIENTED_EDGE ( 'NONE', *, *, #11924, .F. ) ;
#31358=VECTOR ( 'NONE', #44100, 999.9999999999998863 ) ;
#31359=DIRECTION ( 'NONE',  ( 0.6427681459581294776, -0.7660444431189769032, 0.005002170337467562802 ) ) ;
#31361=CARTESIAN_POINT ( 'NONE',  ( -0.2408075302807476947, -4.234515647955085171, 3.311911398282993524 ) ) ;
#31362=VECTOR ( 'NONE', #28005, 1000.000000000000000 ) ;
#31364=EDGE_CURVE ( 'NONE', #32426, #14652, #41212, .T. ) ;
#31365=DIRECTION ( 'NONE',  ( 0.000000000000000000, -0.000000000000000000, -1.000000000000000000 ) ) ;
#31366=CARTESIAN_POINT ( 'NONE',  ( -15.92740756652831102, 3.200641362704007786, 8.320864864478828338 ) ) ;
#31367=CARTESIAN_POINT ( 'NONE',  ( -18.04930495852531536, -5.375054281893163477, 12.51427452863701895 ) ) ;
#31368=AXIS2_PLACEMENT_3D ( 'NONE', #14415, #31460, #48775 ) ;
#31369=ORIENTED_EDGE ( 'NONE', *, *, #19994, .F. ) ;
#31370=ADVANCED_FACE ( 'NONE', ( #2008 ), #41502, .F. ) ;
#31371=EDGE_CURVE ( 'NONE', #40825, #49950, #15936, .T. ) ;
#31372=ADVANCED_FACE ( 'NONE', ( #15114 ), #32438, .F. ) ;
#31373=EDGE_LOOP ( 'NONE', ( #1670, #41631, #42203, #9463 ) ) ;
#31374=PLANE ( 'NONE',  #11944 ) ;
#31375=DIRECTION ( 'NONE',  ( 0.9321478471874540261, -0.000000000000000000, -0.3620778797217457101 ) ) ;
#31377=CARTESIAN_POINT ( 'NONE',  ( -23.33771345073609638, -0.1191753592594197858, 5.846786880686956955 ) ) ;
#31378=VECTOR ( 'NONE', #22983, 1000.000000000000227 ) ;
#31379=AXIS2_PLACEMENT_3D ( 'NONE', #13954, #13420, #14268 ) ;
#31380=CARTESIAN_POINT ( 'NONE',  ( -12.17651289819579929, -0.1191753592594186895, 3.717653505322246144 ) ) ;
#31381=ORIENTED_EDGE ( 'NONE', *, *, #52450, .F. ) ;
#31382=CARTESIAN_POINT ( 'NONE',  ( -7.291207867172650126, -7.010517566319160565, -0.3862208295925149693 ) ) ;
#31383=DIRECTION ( 'NONE',  ( 0.007781995580012663651, -3.146120232559066537E-19, -0.9999697198139514409 ) ) ;
#31384=ORIENTED_EDGE ( 'NONE', *, *, #18475, .T. ) ;
#31385=DIRECTION ( 'NONE',  ( 0.9999697198139515519, 0.000000000000000000, 0.007781995580013368816 ) ) ;
#31386=AXIS2_PLACEMENT_3D ( 'NONE', #36262, #32293, #49609 ) ;
#31387=CARTESIAN_POINT ( 'NONE',  ( -15.65448691412668580, 5.143464774974014553, 2.598562622234925623 ) ) ;
#31388=ORIENTED_EDGE ( 'NONE', *, *, #17459, .F. ) ;
#31389=VECTOR ( 'NONE', #17617, 999.9999999999998863 ) ;
#31390=CARTESIAN_POINT ( 'NONE',  ( -9.070553403303552642, 0.000000000000000000, 3.641821772184214101 ) ) ;
#31391=DIRECTION ( 'NONE',  ( -0.005961354470445682716, -0.6427876096865404731, 0.7660212471507180654 ) ) ;
#31392=VECTOR ( 'NONE', #5100, 999.9999999999998863 ) ;
#31393=EDGE_CURVE ( 'NONE', #21230, #51597, #54272, .T. ) ;
#31394=DIRECTION ( 'NONE',  ( 0.7660212471507180654, -0.6427876096865404731, 0.005961354470445141482 ) ) ;
#31395=CARTESIAN_POINT ( 'NONE',  ( -22.40478740399063895, 0.000000000000000000, 5.384712028983816623 ) ) ;
#31396=VECTOR ( 'NONE', #14502, 1000.000000000000227 ) ;
#31397=EDGE_CURVE ( 'NONE', #55983, #25397, #11100, .T. ) ;
#31398=LINE ( 'NONE', #17774, #9304 ) ;
#31400=VECTOR ( 'NONE', #47352, 1000.000000000000114 ) ;
#31401=VERTEX_POINT ( 'NONE', #28727 ) ;
#31402=EDGE_CURVE ( 'NONE', #17816, #35294, #46035, .T. ) ;
#31403=CARTESIAN_POINT ( 'NONE',  ( -19.55525183663760913, 3.686347215771509589, 4.160241867659052240 ) ) ;
#31404=CARTESIAN_POINT ( 'NONE',  ( -13.07066190154808361, 0.000000000000000000, 12.04713590736729678 ) ) ;
#31405=CARTESIAN_POINT ( 'NONE',  ( -12.18721420714108028, -1.813211359398158029, 1.557398059203232377 ) ) ;
#31406=EDGE_CURVE ( 'NONE', #47316, #30844, #13007, .T. ) ;
#31407=CARTESIAN_POINT ( 'NONE',  ( -16.25459574472089130, 0.000000000000000000, 3.216581823729005585 ) ) ;
#31408=PLANE ( 'NONE',  #23950 ) ;
#31409=EDGE_LOOP ( 'NONE', ( #14196, #31116, #3664, #47127 ) ) ;
#31411=CARTESIAN_POINT ( 'NONE',  ( -18.80232300004736956, 0.000000000000000000, 6.351417435797861444 ) ) ;
#31412=VECTOR ( 'NONE', #16947, 999.9999999999998863 ) ;
#31413=DIRECTION ( 'NONE',  ( 0.6427681459581294776, -0.7660444431189769032, 0.005002170337467562802 ) ) ;
#31414=DIRECTION ( 'NONE',  ( 0.7660212471507180654, -0.6427876096865404731, 0.005961354470445141482 ) ) ;
#31415=ORIENTED_EDGE ( 'NONE', *, *, #1320, .F. ) ;
#31416=LINE ( 'NONE', #9833, #34739 ) ;
#31417=EDGE_LOOP ( 'NONE', ( #26104, #38070, #14801, #47778 ) ) ;
#31420=DIRECTION ( 'NONE',  ( 0.9999697198139515519, 0.000000000000000000, 0.007781995580013368816 ) ) ;
#31421=ORIENTED_EDGE ( 'NONE', *, *, #39523, .F. ) ;
#31422=CARTESIAN_POINT ( 'NONE',  ( -10.37421533196711465, -0.1191753592594197858, 10.96012406864405975 ) ) ;
#31423=VECTOR ( 'NONE', #27323, 1000.000000000000114 ) ;
#31424=ORIENTED_EDGE ( 'NONE', *, *, #30670, .T. ) ;
#31425=ORIENTED_EDGE ( 'NONE', *, *, #4388, .T. ) ;
#31426=AXIS2_PLACEMENT_3D ( 'NONE', #18368, #22078, #39115 ) ;
#31427=VERTEX_POINT ( 'NONE', #9295 ) ;
#31430=ORIENTED_EDGE ( 'NONE', *, *, #13979, .F. ) ;
#31431=PLANE ( 'NONE',  #26560 ) ;
#31432=DIRECTION ( 'NONE',  ( 0.9999697198139515519, 0.000000000000000000, 0.007781995580013368816 ) ) ;
#31433=ORIENTED_EDGE ( 'NONE', *, *, #28187, .F. ) ;
#31434=VECTOR ( 'NONE', #1019, 999.9999999999998863 ) ;
#31435=VECTOR ( 'NONE', #22826, 1000.000000000000227 ) ;
#31436=ORIENTED_EDGE ( 'NONE', *, *, #23745, .T. ) ;
#31437=CARTESIAN_POINT ( 'NONE',  ( -20.46176247598743103, -2.784623065533159636, 4.740520492340843717 ) ) ;
#31438=EDGE_LOOP ( 'NONE', ( #21228, #23467, #44095, #1929 ) ) ;
#31439=ORIENTED_EDGE ( 'NONE', *, *, #46792, .F. ) ;
#31441=AXIS2_PLACEMENT_3D ( 'NONE', #46661, #54603, #33599 ) ;
#31442=EDGE_CURVE ( 'NONE', #14652, #10233, #5340, .T. ) ;
#31443=LINE ( 'NONE', #49015, #12045 ) ;
#31444=CARTESIAN_POINT ( 'NONE',  ( -16.79925329029790149, 0.000000000000000000, 13.49544742625427496 ) ) ;
#31445=LINE ( 'NONE', #40527, #45009 ) ;
#31446=FACE_OUTER_BOUND ( 'NONE', #17813, .T. ) ;
#31447=ORIENTED_EDGE ( 'NONE', *, *, #43715, .F. ) ;
#31448=CARTESIAN_POINT ( 'NONE',  ( -14.10280672071693431, -0.1191753592594197858, 12.40843558753103792 ) ) ;
#31449=ORIENTED_EDGE ( 'NONE', *, *, #15883, .T. ) ;
#31450=ADVANCED_FACE ( 'NONE', ( #22649 ), #26089, .F. ) ;
#31451=EDGE_CURVE ( 'NONE', #50934, #46898, #48187, .T. ) ;
#31452=CARTESIAN_POINT ( 'NONE',  ( -12.80458192191714595, 0.000000000000000000, 11.86454056839041726 ) ) ;
#31453=EDGE_CURVE ( 'NONE', #21908, #8254, #39121, .T. ) ;
#31454=AXIS2_PLACEMENT_3D ( 'NONE', #7387, #37800, #46567 ) ;
#31455=LINE ( 'NONE', #52456, #24201 ) ;
#31456=CARTESIAN_POINT ( 'NONE',  ( -30.79411802867772607, 0.000000000000000000, 8.643412946479525516 ) ) ;
#31457=CARTESIAN_POINT ( 'NONE',  ( -16.72941120119383029, 0.000000000000000000, 4.520888965697079875 ) ) ;
#31458=DIRECTION ( 'NONE',  ( 0.000000000000000000, -1.000000000000000000, 0.000000000000000000 ) ) ;
#31459=DIRECTION ( 'NONE',  ( 0.000000000000000000, 1.000000000000000000, 0.000000000000000000 ) ) ;
#31460=DIRECTION ( 'NONE',  ( -0.005961354470445682716, -0.6427876096865404731, 0.7660212471507180654 ) ) ;
#31461=ORIENTED_EDGE ( 'NONE', *, *, #26294, .T. ) ;
#31462=FACE_OUTER_BOUND ( 'NONE', #40532, .T. ) ;
#31463=PLANE ( 'NONE',  #225 ) ;
#31464=DIRECTION ( 'NONE',  ( -0.5364919789714478471, 0.6444004775717705469, -0.5449076811759709926 ) ) ;
#31465=VECTOR ( 'NONE', #40188, 999.9999999999998863 ) ;
#31466=DIRECTION ( 'NONE',  ( 0.6427681459581294776, -0.7660444431189769032, 0.005002170337467562802 ) ) ;
#31467=FACE_OUTER_BOUND ( 'NONE', #52559, .T. ) ;
#31468=CARTESIAN_POINT ( 'NONE',  ( -15.60102546347950536, 0.000000000000000000, 12.95077420755565356 ) ) ;
#31469=ADVANCED_FACE ( 'NONE', ( #9031 ), #47653, .F. ) ;
#31470=CARTESIAN_POINT ( 'NONE',  ( -19.60834386242827776, 0.000000000000000000, 4.298478389818581213 ) ) ;
#31471=AXIS2_PLACEMENT_3D ( 'NONE', #38265, #51041, #16143 ) ;
#31473=ORIENTED_EDGE ( 'NONE', *, *, #4604, .F. ) ;
#31474=EDGE_CURVE ( 'NONE', #43785, #42567, #43395, .T. ) ;
#31475=FACE_OUTER_BOUND ( 'NONE', #22497, .T. ) ;
#31477=LINE ( 'NONE', #5606, #45999 ) ;
#31478=ADVANCED_FACE ( 'NONE', ( #48484 ), #1044, .F. ) ;
#31479=VECTOR ( 'NONE', #16133, 999.9999999999998863 ) ;
#31480=DIRECTION ( 'NONE',  ( -0.005961354470445682716, -0.6427876096865404731, 0.7660212471507180654 ) ) ;
#31481=DIRECTION ( 'NONE',  ( 0.7660212471507180654, -0.6427876096865404731, 0.005961354470445141482 ) ) ;
#31482=LINE ( 'NONE', #48795, #44964 ) ;
#31483=LINE ( 'NONE', #48495, #24702 ) ;
#31484=EDGE_CURVE ( 'NONE', #2493, #38484, #506, .T. ) ;
#31485=AXIS2_PLACEMENT_3D ( 'NONE', #55676, #30700, #43459 ) ;
#31487=CARTESIAN_POINT ( 'NONE',  ( -15.22910602592149765, 0.000000000000000000, 9.133875538749295586 ) ) ;
#31488=ORIENTED_EDGE ( 'NONE', *, *, #37718, .F. ) ;
#31489=AXIS2_PLACEMENT_3D ( 'NONE', #29028, #3475, #25601 ) ;
#31490=VERTEX_POINT ( 'NONE', #17544 ) ;
#31491=ORIENTED_EDGE ( 'NONE', *, *, #31886, .T. ) ;
#31492=ORIENTED_EDGE ( 'NONE', *, *, #55641, .T. ) ;
#31493=ORIENTED_EDGE ( 'NONE', *, *, #34271, .F. ) ;
#31494=DIRECTION ( 'NONE',  ( 0.9999697198139515519, 0.000000000000000000, 0.007781995580013368816 ) ) ;
#31495=CARTESIAN_POINT ( 'NONE',  ( -24.27063949748155380, 0.000000000000000000, 6.308861732390097288 ) ) ;
#31496=ORIENTED_EDGE ( 'NONE', *, *, #43632, .F. ) ;
#31497=VECTOR ( 'NONE', #31028, 999.9999999999998863 ) ;
#31498=ORIENTED_EDGE ( 'NONE', *, *, #25341, .F. ) ;
#31499=ORIENTED_EDGE ( 'NONE', *, *, #1241, .F. ) ;
#31500=VECTOR ( 'NONE', #31083, 999.9999999999998863 ) ;
#31502=ORIENTED_EDGE ( 'NONE', *, *, #4387, .F. ) ;
#31503=DIRECTION ( 'NONE',  ( -0.5449076811759708816, 0.6444004775717707689, 0.5364919789714475140 ) ) ;
#31504=DIRECTION ( 'NONE',  ( 0.5449076811759707706, 0.6444004775717708799, -0.5364919789714476250 ) ) ;
#31506=PLANE ( 'NONE',  #46524 ) ;
#31507=EDGE_CURVE ( 'NONE', #39389, #31631, #43114, .T. ) ;
#31508=ORIENTED_EDGE ( 'NONE', *, *, #2520, .T. ) ;
#31510=VECTOR ( 'NONE', #24565, 999.9999999999998863 ) ;
#31511=CARTESIAN_POINT ( 'NONE',  ( -21.33651914525451687, -3.270328918600659662, 5.064809129883542482 ) ) ;
#31512=CARTESIAN_POINT ( 'NONE',  ( -19.45503627000849889, -1.000000000000000000, 7.556996783084074742 ) ) ;
#31513=EDGE_CURVE ( 'NONE', #34665, #31630, #18373, .T. ) ;
#31514=EDGE_CURVE ( 'NONE', #39217, #10989, #35176, .T. ) ;
#31515=LINE ( 'NONE', #53365, #42722 ) ;
#31516=DIRECTION ( 'NONE',  ( -0.7660212471507179544, -0.6427876096865405842, -0.005961354470445141482 ) ) ;
#31517=ORIENTED_EDGE ( 'NONE', *, *, #46265, .T. ) ;
#31518=LINE ( 'NONE', #47708, #424 ) ;
#31519=DIRECTION ( 'NONE',  ( -0.6427681459581293666, -0.7660444431189770143, -0.005002170337467561935 ) ) ;
#31520=DIRECTION ( 'NONE',  ( 0.007781995580012663651, -3.146120232559066537E-19, -0.9999697198139514409 ) ) ;
#31521=VERTEX_POINT ( 'NONE', #52471 ) ;
#31522=PLANE ( 'NONE',  #27393 ) ;
#31523=ORIENTED_EDGE ( 'NONE', *, *, #6663, .F. ) ;
#31524=CARTESIAN_POINT ( 'NONE',  ( -22.40556560354864146, -0.1191753592594197858, 5.484709000965211523 ) ) ;
#31525=DIRECTION ( 'NONE',  ( 0.007781995580012663651, 0.000000000000000000, -0.9999697198139515519 ) ) ;
#31527=CARTESIAN_POINT ( 'NONE',  ( 2.072287782118878319, 0.000000000000000000, -2.950529333540147015 ) ) ;
#31528=DIRECTION ( 'NONE',  ( -0.7660212471507179544, -0.6427876096865405842, -0.005961354470445141482 ) ) ;
#31529=DIRECTION ( 'NONE',  ( 0.000000000000000000, -0.000000000000000000, -1.000000000000000000 ) ) ;
#31530=LINE ( 'NONE', #40016, #33401 ) ;
#31531=CARTESIAN_POINT ( 'NONE',  ( -8.875996589204540044, 0.000000000000000000, 10.41778544861944233 ) ) ;
#31533=CARTESIAN_POINT ( 'NONE',  ( -12.15271748404464880, 0.000000000000000000, 1.601849296007406664 ) ) ;
#31535=CARTESIAN_POINT ( 'NONE',  ( -22.45197700822111031, 5.467268677019013978, 5.228607578741694795 ) ) ;
#31536=DIRECTION ( 'NONE',  ( 0.000000000000000000, -0.000000000000000000, -1.000000000000000000 ) ) ;
#31537=DIRECTION ( 'NONE',  ( -0.9999697198139514409, -0.000000000000000000, -0.007781995580013368816 ) ) ;
#31538=CARTESIAN_POINT ( 'NONE',  ( -16.53317331066696383, 0.000000000000000000, 13.31285208727739899 ) ) ;
#31539=CARTESIAN_POINT ( 'NONE',  ( -31.72626587586518099, 0.000000000000000000, 9.005490826201270949 ) ) ;
#31541=CARTESIAN_POINT ( 'NONE',  ( -18.15283808406918098, -3.917936722690662954, 3.807497207905658154 ) ) ;
#31542=PLANE ( 'NONE',  #30188 ) ;
#31543=ORIENTED_EDGE ( 'NONE', *, *, #14297, .F. ) ;
#31544=VECTOR ( 'NONE', #11556, 1000.000000000000227 ) ;
#31545=ORIENTED_EDGE ( 'NONE', *, *, #34783, .T. ) ;
#31546=EDGE_CURVE ( 'NONE', #35148, #42919, #52728, .T. ) ;
#31547=LINE ( 'NONE', #6261, #55880 ) ;
#31549=EDGE_CURVE ( 'NONE', #42286, #21767, #30633, .T. ) ;
#31550=VECTOR ( 'NONE', #56030, 999.9999999999998863 ) ;
#31551=ORIENTED_EDGE ( 'NONE', *, *, #33796, .T. ) ;
#31552=CARTESIAN_POINT ( 'NONE',  ( -29.86352658060627618, 0.000000000000000000, 8.481329010720569883 ) ) ;
#31553=EDGE_CURVE ( 'NONE', #25397, #52695, #47934, .T. ) ;
#31555=LINE ( 'NONE', #28107, #15656 ) ;
#31556=ORIENTED_EDGE ( 'NONE', *, *, #17647, .T. ) ;
#31557=ORIENTED_EDGE ( 'NONE', *, *, #5405, .F. ) ;
#31558=ORIENTED_EDGE ( 'NONE', *, *, #8411, .T. ) ;
#31559=CARTESIAN_POINT ( 'NONE',  ( -16.00875351199029240, 0.000000000000000000, 5.634493499890388613 ) ) ;
#31560=DIRECTION ( 'NONE',  ( 0.007781995580012662783, 0.000000000000000000, -0.9999697198139514409 ) ) ;
#31562=LINE ( 'NONE', #9117, #47526 ) ;
#31563=ORIENTED_EDGE ( 'NONE', *, *, #30459, .F. ) ;
#31564=ORIENTED_EDGE ( 'NONE', *, *, #33166, .T. ) ;
#31566=CARTESIAN_POINT ( 'NONE',  ( -20.07452495636445633, -3.432230869623159819, 4.569442209528198795 ) ) ;
#31568=FACE_OUTER_BOUND ( 'NONE', #15596, .T. ) ;
#31569=ADVANCED_FACE ( 'NONE', ( #30878 ), #17255, .F. ) ;
#31570=ORIENTED_EDGE ( 'NONE', *, *, #37437, .T. ) ;
#31572=CARTESIAN_POINT ( 'NONE',  ( -16.93802730567246329, 0.000000000000000000, 5.627261676354369691 ) ) ;
#31573=ORIENTED_EDGE ( 'NONE', *, *, #50726, .F. ) ;
#31574=ADVANCED_FACE ( 'NONE', ( #49325 ), #53328, .F. ) ;
#31576=EDGE_LOOP ( 'NONE', ( #51802, #36560, #30258, #52908 ) ) ;
#31577=EDGE_CURVE ( 'NONE', #5343, #49645, #19784, .T. ) ;
#31578=EDGE_CURVE ( 'NONE', #45628, #9765, #19498, .T. ) ;
#31579=CARTESIAN_POINT ( 'NONE',  ( -25.20123094555300369, 0.000000000000000000, 6.470945668149052032 ) ) ;
#31580=EDGE_LOOP ( 'NONE', ( #17157, #18578, #50313, #53758 ) ) ;
#31581=CARTESIAN_POINT ( 'NONE',  ( -19.25390728375132099, 0.000000000000000000, 4.670568767036004765 ) ) ;
#31582=CARTESIAN_POINT ( 'NONE',  ( -12.69021377840191533, -0.1941918491731548790, 1.929943632359736538 ) ) ;
#31583=DIRECTION ( 'NONE',  ( -0.5449076811759708816, 0.6444004775717707689, 0.5364919789714475140 ) ) ;
#31584=ORIENTED_EDGE ( 'NONE', *, *, #719, .T. ) ;
#31585=VECTOR ( 'NONE', #3837, 1000.000000000000227 ) ;
#31587=DIRECTION ( 'NONE',  ( -0.6427681459581293666, -0.7660444431189770143, -0.005002170337467561935 ) ) ;
#31588=CARTESIAN_POINT ( 'NONE',  ( -16.47626446233665831, 0.000000000000000000, 6.000187291380142618 ) ) ;
#31589=LINE ( 'NONE', #27594, #29549 ) ;
#31590=DIRECTION ( 'NONE',  ( -0.005961354470445682716, -0.6427876096865404731, 0.7660212471507180654 ) ) ;
#31591=CARTESIAN_POINT ( 'NONE',  ( -24.26908309836554878, 0.000000000000000000, 6.108867788427308376 ) ) ;
#31592=EDGE_CURVE ( 'NONE', #15287, #14766, #24042, .T. ) ;
#31594=ORIENTED_EDGE ( 'NONE', *, *, #13055, .F. ) ;
#31595=CARTESIAN_POINT ( 'NONE',  ( -15.13495153988577968, 0.000000000000000000, 12.76973526769478084 ) ) ;
#31596=DIRECTION ( 'NONE',  ( 0.007781995580012663651, -3.146120232559066537E-19, -0.9999697198139514409 ) ) ;
#31597=DIRECTION ( 'NONE',  ( 0.005961354470445682716, -0.6427876096865404731, -0.7660212471507180654 ) ) ;
#31598=VERTEX_POINT ( 'NONE', #44784 ) ;
#31599=FACE_OUTER_BOUND ( 'NONE', #14025, .T. ) ;
#31600=CARTESIAN_POINT ( 'NONE',  ( -18.23116282465632310, -0.1191753592594167882, 5.517195168626942703 ) ) ;
#31601=VERTEX_POINT ( 'NONE', #2162 ) ;
#31602=CARTESIAN_POINT ( 'NONE',  ( -18.19747506107908563, 0.000000000000000000, 14.03856424583689311 ) ) ;
#31603=CARTESIAN_POINT ( 'NONE',  ( -19.62714374037757636, 0.4483081953215045656, 4.291477522278790424 ) ) ;
#31604=DIRECTION ( 'NONE',  ( 0.7660212471507180654, -0.6427876096865404731, 0.005961354470445141482 ) ) ;
#31605=DIRECTION ( 'NONE',  ( 0.5449076811759707706, 0.6444004775717708799, -0.5364919789714476250 ) ) ;
#31606=ORIENTED_EDGE ( 'NONE', *, *, #28868, .F. ) ;
#31607=ORIENTED_EDGE ( 'NONE', *, *, #14001, .T. ) ;
#31608=CARTESIAN_POINT ( 'NONE',  ( -14.93495759592298988, 0.000000000000000000, 12.77129166681078409 ) ) ;
#31609=CARTESIAN_POINT ( 'NONE',  ( -16.53317331066696383, 0.000000000000000000, 13.31285208727739899 ) ) ;
#31610=CARTESIAN_POINT ( 'NONE',  ( -16.48045617023122134, 0.000000000000000000, 6.538812753932882416 ) ) ;
#31611=PLANE ( 'NONE',  #42903 ) ;
#31612=DIRECTION ( 'NONE',  ( 0.005961354470445682716, -0.6427876096865404731, -0.7660212471507180654 ) ) ;
#31613=VERTEX_POINT ( 'NONE', #10971 ) ;
#31614=LINE ( 'NONE', #10017, #4105 ) ;
#31615=ADVANCED_FACE ( 'NONE', ( #6189 ), #28289, .F. ) ;
#31616=ORIENTED_EDGE ( 'NONE', *, *, #18108, .F. ) ;
#31617=CARTESIAN_POINT ( 'NONE',  ( -15.13495153988577968, 0.000000000000000000, 12.76973526769478084 ) ) ;
#31618=LINE ( 'NONE', #9764, #55973 ) ;
#31619=EDGE_LOOP ( 'NONE', ( #7202, #26180, #4862, #23245 ) ) ;
#31620=DIRECTION ( 'NONE',  ( 0.3313982828793700097, 0.4028455766673916805, 0.8531650599175528704 ) ) ;
#31621=DIRECTION ( 'NONE',  ( 0.000000000000000000, -1.000000000000000000, 0.000000000000000000 ) ) ;
#31622=DIRECTION ( 'NONE',  ( 0.007781995580012663651, -3.146120232559066537E-19, -0.9999697198139514409 ) ) ;
#31623=EDGE_CURVE ( 'NONE', #23133, #21974, #41074, .T. ) ;
#31624=VERTEX_POINT ( 'NONE', #32304 ) ;
#31625=AXIS2_PLACEMENT_3D ( 'NONE', #42670, #29914, #12595 ) ;
#31626=FACE_OUTER_BOUND ( 'NONE', #8500, .T. ) ;
#31628=EDGE_CURVE ( 'NONE', #45792, #10825, #37105, .T. ) ;
#31629=EDGE_CURVE ( 'NONE', #27319, #44456, #36844, .T. ) ;
#31630=VERTEX_POINT ( 'NONE', #41374 ) ;
#31631=VERTEX_POINT ( 'NONE', #10727 ) ;
#31632=ORIENTED_EDGE ( 'NONE', *, *, #40581, .F. ) ;
#31633=DIRECTION ( 'NONE',  ( 0.6427681459581294776, -0.7660444431189769032, 0.005002170337467562802 ) ) ;
#31634=EDGE_CURVE ( 'NONE', #35152, #25894, #22923, .T. ) ;
#31636=ORIENTED_EDGE ( 'NONE', *, *, #23891, .T. ) ;
#31637=DIRECTION ( 'NONE',  ( 0.5449076811759707706, 0.6444004775717708799, -0.5364919789714476250 ) ) ;
#31638=LINE ( 'NONE', #18263, #3232 ) ;
#31639=ORIENTED_EDGE ( 'NONE', *, *, #46063, .F. ) ;
#31640=EDGE_CURVE ( 'NONE', #27257, #17489, #9881, .T. ) ;
#31641=ORIENTED_EDGE ( 'NONE', *, *, #46076, .F. ) ;
#31642=CARTESIAN_POINT ( 'NONE',  ( -19.72584868671897596, 0.000000000000000000, 5.605566205746312036 ) ) ;
#31643=VERTEX_POINT ( 'NONE', #19204 ) ;
#31644=ADVANCED_FACE ( 'NONE', ( #2465 ), #32827, .F. ) ;
#31645=CARTESIAN_POINT ( 'NONE',  ( -11.60492197282151139, -1.651309408375657428, 3.899757593961617808 ) ) ;
#31646=DIRECTION ( 'NONE',  ( -0.005961354470445682716, -0.6427876096865404731, 0.7660212471507180654 ) ) ;
#31647=CARTESIAN_POINT ( 'NONE',  ( -19.12962290826653700, 0.000000000000000000, 14.40064212555863854 ) ) ;
#31648=LINE ( 'NONE', #48380, #3962 ) ;
#31649=CARTESIAN_POINT ( 'NONE',  ( -21.00667280355191124, -3.432230869623159819, 4.931520089249944228 ) ) ;
#31650=CARTESIAN_POINT ( 'NONE',  ( -29.86352658060627618, 0.000000000000000000, 8.481329010720569883 ) ) ;
#31651=ORIENTED_EDGE ( 'NONE', *, *, #23456, .T. ) ;
#31652=EDGE_CURVE ( 'NONE', #41949, #27295, #36021, .T. ) ;
#31653=ORIENTED_EDGE ( 'NONE', *, *, #3925, .F. ) ;
#31654=DIRECTION ( 'NONE',  ( -0.6427681459581293666, -0.7660444431189770143, -0.005002170337467561935 ) ) ;
#31655=DIRECTION ( 'NONE',  ( 0.007781995580012663651, -3.146120232559066537E-19, -0.9999697198139514409 ) ) ;
#31656=FACE_OUTER_BOUND ( 'NONE', #22185, .T. ) ;
#31657=EDGE_CURVE ( 'NONE', #1914, #31885, #10439, .T. ) ;
#31659=ORIENTED_EDGE ( 'NONE', *, *, #55833, .T. ) ;
#31661=LINE ( 'NONE', #18588, #17794 ) ;
#31662=VERTEX_POINT ( 'NONE', #18677 ) ;
#31664=CARTESIAN_POINT ( 'NONE',  ( -20.10727089963316061, 4.819660872929009798, 12.60155257131766859 ) ) ;
#31665=ORIENTED_EDGE ( 'NONE', *, *, #19421, .F. ) ;
#31668=DIRECTION ( 'NONE',  ( 0.005002170337468016433, -0.7660444431189770143, -0.6427681459581293666 ) ) ;
#31669=DIRECTION ( 'NONE',  ( 0.007781995580012663651, 0.000000000000000000, -0.9999697198139515519 ) ) ;
#31670=DIRECTION ( 'NONE',  ( 0.000000000000000000, -0.000000000000000000, -1.000000000000000000 ) ) ;
#31671=CARTESIAN_POINT ( 'NONE',  ( -20.31522615006396038, 5.143464774974012776, 4.408952020843655895 ) ) ;
#31672=VERTEX_POINT ( 'NONE', #32004 ) ;
#31673=ORIENTED_EDGE ( 'NONE', *, *, #34451, .T. ) ;
#31674=DIRECTION ( 'NONE',  ( 0.6427681459581294776, -0.7660444431189769032, 0.005002170337467562802 ) ) ;
#31675=PLANE ( 'NONE',  #17695 ) ;
#31676=FACE_OUTER_BOUND ( 'NONE', #10042, .T. ) ;
#31677=CARTESIAN_POINT ( 'NONE',  ( -9.769797563482667258, 0.000000000000000000, 5.852372511285491186 ) ) ;
#31678=CARTESIAN_POINT ( 'NONE',  ( -25.20200914511100265, -0.1191753592594197858, 6.570942640130446932 ) ) ;
#31679=ADVANCED_FACE ( 'NONE', ( #1631 ), #45086, .F. ) ;
#31680=ORIENTED_EDGE ( 'NONE', *, *, #21392, .F. ) ;
#31682=LINE ( 'NONE', #41762, #41094 ) ;
#31683=DIRECTION ( 'NONE',  ( -0.9999697198139514409, -0.000000000000000000, -0.007781995580013368816 ) ) ;
#31684=LINE ( 'NONE', #6395, #27854 ) ;
#31685=ORIENTED_EDGE ( 'NONE', *, *, #12644, .T. ) ;
#31686=DIRECTION ( 'NONE',  ( 0.5449076811759707706, 0.6444004775717708799, -0.5364919789714476250 ) ) ;
#31687=ORIENTED_EDGE ( 'NONE', *, *, #5224, .T. ) ;
#31688=DIRECTION ( 'NONE',  ( 0.5364919789714477361, 0.6444004775717706579, 0.5449076811759711036 ) ) ;
#31689=ADVANCED_FACE ( 'NONE', ( #23223 ), #40550, .F. ) ;
#31690=EDGE_CURVE ( 'NONE', #14373, #52348, #3842, .T. ) ;
#31691=LINE ( 'NONE', #5007, #26623 ) ;
#31692=ORIENTED_EDGE ( 'NONE', *, *, #13350, .F. ) ;
#31693=DIRECTION ( 'NONE',  ( -0.9999697198139514409, -0.000000000000000000, -0.007781995580013368816 ) ) ;
#31694=ORIENTED_EDGE ( 'NONE', *, *, #34221, .T. ) ;
#31695=EDGE_CURVE ( 'NONE', #38002, #27953, #11805, .T. ) ;
#31696=EDGE_LOOP ( 'NONE', ( #24005, #36567, #38368, #31709 ) ) ;
#31697=ORIENTED_EDGE ( 'NONE', *, *, #7457, .T. ) ;
#31698=CARTESIAN_POINT ( 'NONE',  ( -28.93137873341882127, 0.000000000000000000, 8.119251130998824451 ) ) ;
#31699=ORIENTED_EDGE ( 'NONE', *, *, #43124, .F. ) ;
#31700=ORIENTED_EDGE ( 'NONE', *, *, #27188, .T. ) ;
#31701=FACE_OUTER_BOUND ( 'NONE', #13927, .T. ) ;
#31702=PLANE ( 'NONE',  #4095 ) ;
#31703=VERTEX_POINT ( 'NONE', #38204 ) ;
#31704=EDGE_CURVE ( 'NONE', #37525, #20361, #19642, .T. ) ;
#31705=EDGE_LOOP ( 'NONE', ( #34411, #11423, #16882, #18872 ) ) ;
#31706=CARTESIAN_POINT ( 'NONE',  ( -18.32618988918515512, 0.000000000000000000, 4.877794534534811710 ) ) ;
#31707=EDGE_CURVE ( 'NONE', #38106, #35325, #20632, .T. ) ;
#31708=EDGE_LOOP ( 'NONE', ( #9033, #32321, #33922, #21428 ) ) ;
#31709=ORIENTED_EDGE ( 'NONE', *, *, #34854, .F. ) ;
#31710=ADVANCED_FACE ( 'NONE', ( #46739 ), #29420, .F. ) ;
#31711=CARTESIAN_POINT ( 'NONE',  ( -27.99845268667336384, -0.1191753592594197858, 7.657176279295684118 ) ) ;
#31712=DIRECTION ( 'NONE',  ( 0.007781995580012663651, -3.146120232559066537E-19, -0.9999697198139514409 ) ) ;
#31713=EDGE_CURVE ( 'NONE', #51394, #34166, #16629, .T. ) ;
#31714=LINE ( 'NONE', #49017, #31434 ) ;
#31716=ORIENTED_EDGE ( 'NONE', *, *, #35407, .F. ) ;
#31717=LINE ( 'NONE', #10120, #21976 ) ;
#31718=ORIENTED_EDGE ( 'NONE', *, *, #52873, .F. ) ;
#31719=ADVANCED_FACE ( 'NONE', ( #46430 ), #3573, .F. ) ;
#31720=DIRECTION ( 'NONE',  ( 0.7660212471507180654, -0.6427876096865404731, 0.005961354470445141482 ) ) ;
#31721=DIRECTION ( 'NONE',  ( 0.6427681459581294776, -0.7660444431189769032, 0.005002170337467562802 ) ) ;
#31723=FACE_OUTER_BOUND ( 'NONE', #16746, .T. ) ;
#31724=CARTESIAN_POINT ( 'NONE',  ( -22.40478740399063895, 0.000000000000000000, 5.384712028983816623 ) ) ;
#31725=CARTESIAN_POINT ( 'NONE',  ( -22.38231225002310865, -5.536956232915663634, 14.46307039415223272 ) ) ;
#31726=ORIENTED_EDGE ( 'NONE', *, *, #54325, .F. ) ;
#31727=CARTESIAN_POINT ( 'NONE',  ( -10.43155435078125670, 0.000000000000000000, 5.477890497143714121 ) ) ;
#31728=ORIENTED_EDGE ( 'NONE', *, *, #46601, .T. ) ;
#31729=CARTESIAN_POINT ( 'NONE',  ( -13.17065887352947762, -0.1191753592594197858, 12.04635770780929427 ) ) ;
#31730=DIRECTION ( 'NONE',  ( 0.007781995580012662783, 0.000000000000000000, -0.9999697198139514409 ) ) ;
#31731=DIRECTION ( 'NONE',  ( -0.9999697198139514409, -0.000000000000000000, -0.007781995580013368816 ) ) ;
#31732=CARTESIAN_POINT ( 'NONE',  ( -16.84874834815419575, -0.1191753592594177180, 7.005281716962028504 ) ) ;
#31733=DIRECTION ( 'NONE',  ( -0.7660212471507179544, -0.6427876096865405842, -0.005961354470445141482 ) ) ;
#31735=EDGE_LOOP ( 'NONE', ( #29805, #6971, #25070, #48138 ) ) ;
#31736=PLANE ( 'NONE',  #54704 ) ;
#31737=DIRECTION ( 'NONE',  ( 0.005961354470445682716, -0.6427876096865404731, -0.7660212471507180654 ) ) ;
#31738=DIRECTION ( 'NONE',  ( -0.5364919789714478471, 0.6444004775717705469, -0.5449076811759709926 ) ) ;
#31740=EDGE_CURVE ( 'NONE', #22414, #30649, #33664, .T. ) ;
#31741=PLANE ( 'NONE',  #33707 ) ;
#31742=DIRECTION ( 'NONE',  ( -0.005961354470445682716, -0.6427876096865404731, 0.7660212471507180654 ) ) ;
#31743=ADVANCED_FACE ( 'NONE', ( #51285 ), #12398, .F. ) ;
#31744=CARTESIAN_POINT ( 'NONE',  ( -18.63227683361970577, -2.784623065533159636, 8.489381659524488200 ) ) ;
#31745=DIRECTION ( 'NONE',  ( -0.5449076811759708816, 0.6444004775717707689, 0.5364919789714475140 ) ) ;
#31747=EDGE_CURVE ( 'NONE', #24350, #33683, #47023, .T. ) ;
#31748=CARTESIAN_POINT ( 'NONE',  ( -12.15720038968843575, -0.1166911823299083412, 1.503895915954261975 ) ) ;
#31749=EDGE_CURVE ( 'NONE', #26892, #6017, #37664, .T. ) ;
#31750=EDGE_CURVE ( 'NONE', #22811, #40865, #16935, .T. ) ;
#31751=EDGE_CURVE ( 'NONE', #47218, #50133, #38492, .T. ) ;
#31752=ORIENTED_EDGE ( 'NONE', *, *, #6151, .F. ) ;
#31753=EDGE_CURVE ( 'NONE', #39017, #36677, #28578, .T. ) ;
#31754=ORIENTED_EDGE ( 'NONE', *, *, #46138, .T. ) ;
#31755=ORIENTED_EDGE ( 'NONE', *, *, #33930, .T. ) ;
#31756=VERTEX_POINT ( 'NONE', #24578 ) ;
#31757=VERTEX_POINT ( 'NONE', #45903 ) ;
#31758=CARTESIAN_POINT ( 'NONE',  ( -18.76354595665420177, -0.1191753592594177458, 14.21882498613976331 ) ) ;
#31761=VERTEX_POINT ( 'NONE', #7020 ) ;
#31762=ORIENTED_EDGE ( 'NONE', *, *, #46878, .F. ) ;
#31763=AXIS2_PLACEMENT_3D ( 'NONE', #52979, #45039, #32255 ) ;
#31764=EDGE_CURVE ( 'NONE', #38002, #26378, #24323, .T. ) ;
#31765=CARTESIAN_POINT ( 'NONE',  ( -14.20280369269832832, 0.000000000000000000, 12.40765738797303719 ) ) ;
#31766=EDGE_CURVE ( 'NONE', #46034, #19226, #2711, .T. ) ;
#31767=PLANE ( 'NONE',  #10114 ) ;
#31768=LINE ( 'NONE', #550, #47718 ) ;
#31769=VERTEX_POINT ( 'NONE', #7551 ) ;
#31770=CARTESIAN_POINT ( 'NONE',  ( -18.86354292863559579, 0.000000000000000000, 14.21804678658176080 ) ) ;
#31771=ORIENTED_EDGE ( 'NONE', *, *, #26546, .T. ) ;
#31772=EDGE_CURVE ( 'NONE', #24424, #34779, #16085, .T. ) ;
#31773=PLANE ( 'NONE',  #50890 ) ;
#31774=DIRECTION ( 'NONE',  ( 0.9999697198139515519, 0.000000000000000000, 0.007781995580013368816 ) ) ;
#31775=EDGE_CURVE ( 'NONE', #23847, #49612, #20327, .T. ) ;
#31776=LINE ( 'NONE', #49081, #40904 ) ;
#31777=DIRECTION ( 'NONE',  ( 0.6427681459581294776, -0.7660444431189769032, 0.005002170337467562802 ) ) ;
#31778=DIRECTION ( 'NONE',  ( -0.5449076811759708816, 0.6444004775717707689, 0.5364919789714475140 ) ) ;
#31779=DIRECTION ( 'NONE',  ( 0.7660212471507180654, -0.6427876096865404731, 0.005961354470445141482 ) ) ;
#31780=DIRECTION ( 'NONE',  ( 0.005002170337468016433, -0.7660444431189770143, -0.6427681459581293666 ) ) ;
#31781=ORIENTED_EDGE ( 'NONE', *, *, #27381, .T. ) ;
#31782=DIRECTION ( 'NONE',  ( 0.007781995580012662783, 0.000000000000000000, -0.9999697198139514409 ) ) ;
#31784=CARTESIAN_POINT ( 'NONE',  ( -17.74560456716937296, 0.000000000000000000, 3.774316574337878372 ) ) ;
#31785=CARTESIAN_POINT ( 'NONE',  ( -17.46532115785441519, 0.000000000000000000, 13.67492996699914265 ) ) ;
#31786=LINE ( 'NONE', #574, #20403 ) ;
#31787=DIRECTION ( 'NONE',  ( 0.6427681459581294776, -0.7660444431189769032, 0.005002170337467562802 ) ) ;
#31788=DIRECTION ( 'NONE',  ( 0.6427681459581294776, -0.7660444431189769032, 0.005002170337467562802 ) ) ;
#31789=PLANE ( 'NONE',  #24926 ) ;
#31791=LINE ( 'NONE', #23287, #6554 ) ;
#31792=DIRECTION ( 'NONE',  ( 0.007781995580012662783, 0.000000000000000000, -0.9999697198139514409 ) ) ;
#31793=EDGE_LOOP ( 'NONE', ( #30702, #55753, #15576, #39614 ) ) ;
#31794=DIRECTION ( 'NONE',  ( 0.007781995580012663651, -3.146120232559066537E-19, -0.9999697198139514409 ) ) ;
#31795=FACE_OUTER_BOUND ( 'NONE', #32176, .T. ) ;
#31796=CARTESIAN_POINT ( 'NONE',  ( -12.60458797795435615, 0.000000000000000000, 11.86609696750642229 ) ) ;
#31797=DIRECTION ( 'NONE',  ( 0.005961354470445682716, -0.6427876096865404731, -0.7660212471507180654 ) ) ;
#31798=FACE_OUTER_BOUND ( 'NONE', #6279, .T. ) ;
#31800=DIRECTION ( 'NONE',  ( 0.9999697198139515519, 0.000000000000000000, 0.007781995580013368816 ) ) ;
#31801=VERTEX_POINT ( 'NONE', #17772 ) ;
#31802=AXIS2_PLACEMENT_3D ( 'NONE', #18165, #52797, #13905 ) ;
#31803=ORIENTED_EDGE ( 'NONE', *, *, #54497, .F. ) ;
#31804=DIRECTION ( 'NONE',  ( -0.5449076811759708816, 0.6444004775717707689, 0.5364919789714475140 ) ) ;
#31805=CARTESIAN_POINT ( 'NONE',  ( -18.86354292863559579, 0.000000000000000000, 14.21804678658176080 ) ) ;
#31806=EDGE_CURVE ( 'NONE', #3481, #46828, #30820, .T. ) ;
#31807=EDGE_CURVE ( 'NONE', #8140, #13801, #21741, .T. ) ;
#31808=ORIENTED_EDGE ( 'NONE', *, *, #12662, .T. ) ;
#31809=CARTESIAN_POINT ( 'NONE',  ( 2.072287782118878319, 0.000000000000000000, -2.950529333540147015 ) ) ;
#31810=ORIENTED_EDGE ( 'NONE', *, *, #1578, .F. ) ;
#31811=FACE_OUTER_BOUND ( 'NONE', #24473, .T. ) ;
#31812=ADVANCED_FACE ( 'NONE', ( #12933 ), #22313, .F. ) ;
#31813=ORIENTED_EDGE ( 'NONE', *, *, #54287, .T. ) ;
#31814=ORIENTED_EDGE ( 'NONE', *, *, #39639, .F. ) ;
#31815=ORIENTED_EDGE ( 'NONE', *, *, #52886, .F. ) ;
#31816=CARTESIAN_POINT ( 'NONE',  ( -15.05682940326283514, -1.327505506330655782, 4.709178299313876437 ) ) ;
#31817=CARTESIAN_POINT ( 'NONE',  ( -20.90639117353077125, -1.651309408375658760, 4.949388017332537970 ) ) ;
#31818=PLANE ( 'NONE',  #3053 ) ;
#31819=VECTOR ( 'NONE', #48594, 1000.000000000000114 ) ;
#31820=CARTESIAN_POINT ( 'NONE',  ( -19.60990026154428278, 0.000000000000000000, 4.498472333781370125 ) ) ;
#31821=ORIENTED_EDGE ( 'NONE', *, *, #26546, .F. ) ;
#31822=ORIENTED_EDGE ( 'NONE', *, *, #20953, .F. ) ;
#31823=LINE ( 'NONE', #15080, #55394 ) ;
#31824=ORIENTED_EDGE ( 'NONE', *, *, #42151, .T. ) ;
#31825=DIRECTION ( 'NONE',  ( -0.6427681459581293666, -0.7660444431189770143, -0.005002170337467561935 ) ) ;
#31826=VERTEX_POINT ( 'NONE', #31085 ) ;
#31827=CARTESIAN_POINT ( 'NONE',  ( -17.24632744471935908, 4.819660872929012463, 3.227218583223867121 ) ) ;
#31828=PLANE ( 'NONE',  #7678 ) ;
#31829=ORIENTED_EDGE ( 'NONE', *, *, #19334, .F. ) ;
#31830=VECTOR ( 'NONE', #16751, 1000.000000000000000 ) ;
#31831=CARTESIAN_POINT ( 'NONE',  ( -16.86886672269117682, -0.1191753592594181482, 9.590449639766383427 ) ) ;
#31832=ORIENTED_EDGE ( 'NONE', *, *, #42466, .T. ) ;
#31833=ADVANCED_FACE ( 'NONE', ( #8700 ), #22586, .F. ) ;
#31834=VECTOR ( 'NONE', #40556, 1000.000000000000227 ) ;
#31835=CARTESIAN_POINT ( 'NONE',  ( 2.072287782118878319, 0.000000000000000000, -2.950529333540147015 ) ) ;
#31836=ORIENTED_EDGE ( 'NONE', *, *, #21151, .T. ) ;
#31837=EDGE_CURVE ( 'NONE', #39606, #20246, #17464, .T. ) ;
#31838=DIRECTION ( 'NONE',  ( 0.000000000000000000, -0.000000000000000000, -1.000000000000000000 ) ) ;
#31839=DIRECTION ( 'NONE',  ( -0.5364919789714478471, 0.6444004775717705469, -0.5449076811759709926 ) ) ;
#31840=DIRECTION ( 'NONE',  ( 0.5449076811759707706, 0.6444004775717708799, -0.5364919789714476250 ) ) ;
#31841=ORIENTED_EDGE ( 'NONE', *, *, #55088, .T. ) ;
#31842=CARTESIAN_POINT ( 'NONE',  ( -30.79411802867772607, 0.000000000000000000, 8.643412946479525516 ) ) ;
#31843=CARTESIAN_POINT ( 'NONE',  ( -19.72297463321369548, 0.000000000000000000, 5.236256502488546793 ) ) ;
#31844=EDGE_CURVE ( 'NONE', #48219, #3085, #52408, .T. ) ;
#31845=DIRECTION ( 'NONE',  ( 0.000000000000000000, -1.000000000000000000, 0.000000000000000000 ) ) ;
#31846=DIRECTION ( 'NONE',  ( -0.005961354470445682716, -0.6427876096865404731, 0.7660212471507180654 ) ) ;
#31847=DIRECTION ( 'NONE',  ( 0.7660212471507180654, -0.6427876096865404731, 0.005961354470445141482 ) ) ;
#31848=CARTESIAN_POINT ( 'NONE',  ( -12.67829634397052097, -0.1159828484229817602, 8.143054432418114885 ) ) ;
#31850=EDGE_LOOP ( 'NONE', ( #52758, #7306, #25955, #37819 ) ) ;
#31851=CARTESIAN_POINT ( 'NONE',  ( -20.54204810873173415, 0.000000000000000000, 4.860550213503115558 ) ) ;
#31852=CARTESIAN_POINT ( 'NONE',  ( -28.92982233430281980, 0.000000000000000000, 7.919257187036034651 ) ) ;
#31855=DIRECTION ( 'NONE',  ( 0.5449076811759707706, 0.6444004775717708799, -0.5364919789714476250 ) ) ;
#31856=LINE ( 'NONE', #27902, #11837 ) ;
#31857=ORIENTED_EDGE ( 'NONE', *, *, #7068, .T. ) ;
#31859=VECTOR ( 'NONE', #7059, 999.9999999999998863 ) ;
#31860=CARTESIAN_POINT ( 'NONE',  ( -12.08148583366696727, 0.000000000000000000, 4.357054139414387350 ) ) ;
#31861=CARTESIAN_POINT ( 'NONE',  ( -2.428019651919397948, -4.270454567941153634, -2.275248286963848177 ) ) ;
#31862=PLANE ( 'NONE',  #48331 ) ;
#31863=ORIENTED_EDGE ( 'NONE', *, *, #43055, .T. ) ;
#31864=VERTEX_POINT ( 'NONE', #56108 ) ;
#31865=FACE_OUTER_BOUND ( 'NONE', #42346, .T. ) ;
#31866=LINE ( 'NONE', #49484, #29638 ) ;
#31867=EDGE_CURVE ( 'NONE', #2943, #10990, #34509, .T. ) ;
#31868=DIRECTION ( 'NONE',  ( -0.5449076811759708816, 0.6444004775717707689, 0.5364919789714475140 ) ) ;
#31869=ADVANCED_FACE ( 'NONE', ( #125 ), #43337, .F. ) ;
#31870=CARTESIAN_POINT ( 'NONE',  ( -22.40634380310664397, 0.000000000000000000, 5.584705972946605534 ) ) ;
#31871=EDGE_LOOP ( 'NONE', ( #46867, #33985, #30163, #9199 ) ) ;
#31872=DIRECTION ( 'NONE',  ( 0.9999697198139515519, 0.000000000000000000, 0.007781995580013368816 ) ) ;
#31873=ORIENTED_EDGE ( 'NONE', *, *, #38978, .T. ) ;
#31874=PLANE ( 'NONE',  #26535 ) ;
#31875=ADVANCED_FACE ( 'NONE', ( #4982 ), #43583, .F. ) ;
#31877=VECTOR ( 'NONE', #55352, 1000.000000000000227 ) ;
#31878=DIRECTION ( 'NONE',  ( 0.9999697198139515519, 0.000000000000000000, 0.007781995580013368816 ) ) ;
#31880=CARTESIAN_POINT ( 'NONE',  ( -14.38135624321859218, -1.651309408375658760, 2.414842859280319054 ) ) ;
#31881=CARTESIAN_POINT ( 'NONE',  ( -20.10484237718952727, -0.1046793181814243412, 5.884109821959732756 ) ) ;
#31882=LINE ( 'NONE', #6076, #19397 ) ;
#31883=ORIENTED_EDGE ( 'NONE', *, *, #23618, .T. ) ;
#31884=FACE_OUTER_BOUND ( 'NONE', #20831, .T. ) ;
#31885=VERTEX_POINT ( 'NONE', #13764 ) ;
#31886=EDGE_CURVE ( 'NONE', #48900, #35085, #22009, .T. ) ;
#31887=ORIENTED_EDGE ( 'NONE', *, *, #44312, .F. ) ;
#31888=EDGE_LOOP ( 'NONE', ( #43029, #29860, #55782, #11111 ) ) ;
#31889=CARTESIAN_POINT ( 'NONE',  ( -13.77905473773374645, -1.489407457353156827, 2.186054020192172320 ) ) ;
#31890=ORIENTED_EDGE ( 'NONE', *, *, #45354, .T. ) ;
#31891=LINE ( 'NONE', #35596, #3944 ) ;
#31893=ORIENTED_EDGE ( 'NONE', *, *, #34127, .F. ) ;
#31894=DIRECTION ( 'NONE',  ( -0.5449076811759708816, 0.6444004775717707689, 0.5364919789714475140 ) ) ;
#31895=CARTESIAN_POINT ( 'NONE',  ( -22.40634380310664397, 0.000000000000000000, 5.584705972946605534 ) ) ;
#31896=VECTOR ( 'NONE', #17201, 999.9999999999998863 ) ;
#31897=AXIS2_PLACEMENT_3D ( 'NONE', #46938, #28780, #15686 ) ;
#31898=ORIENTED_EDGE ( 'NONE', *, *, #13665, .T. ) ;
#31899=DIRECTION ( 'NONE',  ( 0.7660212471507180654, -0.6427876096865404731, 0.005961354470445141482 ) ) ;
#31900=EDGE_LOOP ( 'NONE', ( #25024, #51146, #2483, #40510, #35931 ) ) ;
#31901=DIRECTION ( 'NONE',  ( -0.005961354470445682716, -0.6427876096865404731, 0.7660212471507180654 ) ) ;
#31902=LINE ( 'NONE', #13738, #22963 ) ;
#31904=CARTESIAN_POINT ( 'NONE',  ( -12.33850799832341849, 0.000000000000000000, 11.68350162852954632 ) ) ;
#31906=DIRECTION ( 'NONE',  ( -0.5364919789714478471, 0.6444004775717705469, -0.5449076811759709926 ) ) ;
#31907=FACE_OUTER_BOUND ( 'NONE', #36991, .T. ) ;
#31908=CARTESIAN_POINT ( 'NONE',  ( -17.18674359190834977, 0.000000000000000000, 3.578659703450752350 ) ) ;
#31909=ORIENTED_EDGE ( 'NONE', *, *, #4717, .T. ) ;
#31910=VERTEX_POINT ( 'NONE', #48410 ) ;
#31911=DIRECTION ( 'NONE',  ( 0.000000000000000000, -0.000000000000000000, -1.000000000000000000 ) ) ;
#31912=ADVANCED_FACE ( 'NONE', ( #426 ), #9522, .F. ) ;
#31914=AXIS2_PLACEMENT_3D ( 'NONE', #39685, #26598, #4472 ) ;
#31915=VECTOR ( 'NONE', #11452, 1000.000000000000227 ) ;
#31917=DIRECTION ( 'NONE',  ( 0.9321478471874540261, 0.000000000000000000, -0.3620778797217457101 ) ) ;
#31918=EDGE_LOOP ( 'NONE', ( #51140, #3600, #15221, #24468 ) ) ;
#31919=DIRECTION ( 'NONE',  ( 0.005002170337468016433, -0.7660444431189770143, -0.6427681459581293666 ) ) ;
#31920=CARTESIAN_POINT ( 'NONE',  ( 2.072287782118878319, 0.000000000000000000, -2.950529333540147015 ) ) ;
#31921=EDGE_LOOP ( 'NONE', ( #25952, #16545, #35501, #49498 ) ) ;
#31922=FACE_OUTER_BOUND ( 'NONE', #51237, .T. ) ;
#31923=DIRECTION ( 'NONE',  ( -0.5449076811759708816, 0.6444004775717707689, 0.5364919789714475140 ) ) ;
#31924=ORIENTED_EDGE ( 'NONE', *, *, #14264, .F. ) ;
#31926=CARTESIAN_POINT ( 'NONE',  ( -21.47419595591918906, 0.000000000000000000, 5.222628093224860102 ) ) ;
#31927=DIRECTION ( 'NONE',  ( -0.7660212471507179544, -0.6427876096865405842, -0.005961354470445141482 ) ) ;
#31928=DIRECTION ( 'NONE',  ( 0.005002170337468016433, -0.7660444431189770143, -0.6427681459581293666 ) ) ;
#31929=EDGE_CURVE ( 'NONE', #5535, #19882, #51822, .T. ) ;
#31930=EDGE_CURVE ( 'NONE', #33244, #4850, #8390, .T. ) ;
#31931=CARTESIAN_POINT ( 'NONE',  ( -15.03495456790438389, -0.1191753592594197858, 12.77051346725278158 ) ) ;
#31933=EDGE_LOOP ( 'NONE', ( #36289, #54898, #13684, #35068 ) ) ;
#31934=EDGE_LOOP ( 'NONE', ( #33131, #33626, #30898, #13709 ) ) ;
#31935=PLANE ( 'NONE',  #24849 ) ;
#31936=LINE ( 'NONE', #10368, #19511 ) ;
#31937=CARTESIAN_POINT ( 'NONE',  ( -19.10230891376690110, -0.1191753592594169270, 8.465072266782243560 ) ) ;
#31938=ADVANCED_FACE ( 'NONE', ( #21475 ), #15192, .F. ) ;
#31941=DIRECTION ( 'NONE',  ( -0.6427681459581293666, -0.7660444431189770143, -0.005002170337467561935 ) ) ;
#31942=EDGE_CURVE ( 'NONE', #2953, #25391, #1812, .T. ) ;
#31943=CARTESIAN_POINT ( 'NONE',  ( -14.93495759592298988, 0.000000000000000000, 12.77129166681078409 ) ) ;
#31944=ORIENTED_EDGE ( 'NONE', *, *, #29966, .F. ) ;
#31945=CARTESIAN_POINT ( 'NONE',  ( 2.072287782118878319, 0.000000000000000000, -2.950529333540147015 ) ) ;
#31946=PLANE ( 'NONE',  #2082 ) ;
#31947=ADVANCED_FACE ( 'NONE', ( #23964 ), #10361, .F. ) ;
#31948=LINE ( 'NONE', #49266, #22327 ) ;
#31949=VECTOR ( 'NONE', #16101, 1000.000000000000114 ) ;
#31950=PLANE ( 'NONE',  #52325 ) ;
#31951=AXIS2_PLACEMENT_3D ( 'NONE', #23053, #44347, #35842 ) ;
#31952=ORIENTED_EDGE ( 'NONE', *, *, #23920, .T. ) ;
#31953=DIRECTION ( 'NONE',  ( 0.9999697198139515519, 0.000000000000000000, 0.007781995580013368816 ) ) ;
#31954=ORIENTED_EDGE ( 'NONE', *, *, #14750, .F. ) ;
#31955=DIRECTION ( 'NONE',  ( -0.005961354470445682716, -0.6427876096865404731, 0.7660212471507180654 ) ) ;
#31956=PLANE ( 'NONE',  #47454 ) ;
#31957=EDGE_CURVE ( 'NONE', #35444, #40739, #27685, .T. ) ;
#31958=ORIENTED_EDGE ( 'NONE', *, *, #32768, .F. ) ;
#31959=CARTESIAN_POINT ( 'NONE',  ( -10.66076323225010469, 0.000000000000000000, 0.9226289047854381309 ) ) ;
#31961=ORIENTED_EDGE ( 'NONE', *, *, #19560, .T. ) ;
#31962=ADVANCED_FACE ( 'NONE', ( #18298 ), #1566, .F. ) ;
#31963=VERTEX_POINT ( 'NONE', #27121 ) ;
#31964=VERTEX_POINT ( 'NONE', #36463 ) ;
#31965=CARTESIAN_POINT ( 'NONE',  ( -15.05648729026585819, 0.000000000000000000, 2.687247697364291366 ) ) ;
#31966=ORIENTED_EDGE ( 'NONE', *, *, #15574, .F. ) ;
#31967=ORIENTED_EDGE ( 'NONE', *, *, #7648, .F. ) ;
#31968=DIRECTION ( 'NONE',  ( 0.007781995580012662783, 0.000000000000000000, -0.9999697198139514409 ) ) ;
#31969=CARTESIAN_POINT ( 'NONE',  ( -1.086233639165236964, 0.000000000000000000, -2.796443541562362078 ) ) ;
#31970=ORIENTED_EDGE ( 'NONE', *, *, #8100, .T. ) ;
#31971=ORIENTED_EDGE ( 'NONE', *, *, #6384, .F. ) ;
#31972=DIRECTION ( 'NONE',  ( 0.5364919789714477361, 0.6444004775717706579, 0.5449076811759711036 ) ) ;
#31973=ORIENTED_EDGE ( 'NONE', *, *, #46894, .T. ) ;
#31974=VECTOR ( 'NONE', #53782, 999.9999999999998863 ) ;
#31975=ORIENTED_EDGE ( 'NONE', *, *, #12667, .F. ) ;
#31976=CARTESIAN_POINT ( 'NONE',  ( -17.26532721389163072, 0.000000000000000000, 13.67648636611514590 ) ) ;
#31977=PLANE ( 'NONE',  #7838 ) ;
#31978=LINE ( 'NONE', #45880, #612 ) ;
#31979=AXIS2_PLACEMENT_3D ( 'NONE', #36992, #27922, #45224 ) ;
#31980=ORIENTED_EDGE ( 'NONE', *, *, #31640, .F. ) ;
#31981=LINE ( 'NONE', #28553, #39201 ) ;
#31982=ORIENTED_EDGE ( 'NONE', *, *, #49922, .F. ) ;
#31983=VECTOR ( 'NONE', #32015, 1000.000000000000000 ) ;
#31984=AXIS2_PLACEMENT_3D ( 'NONE', #22641, #39696, #14135 ) ;
#31985=ADVANCED_FACE ( 'NONE', ( #44427 ), #14064, .F. ) ;
#31986=PLANE ( 'NONE',  #32130 ) ;
#31987=DIRECTION ( 'NONE',  ( -0.6427681459581293666, -0.7660444431189770143, -0.005002170337467561935 ) ) ;
#31988=AXIS2_PLACEMENT_3D ( 'NONE', #27073, #44382, #5481 ) ;
#31989=VECTOR ( 'NONE', #31154, 1000.000000000000227 ) ;
#31990=CARTESIAN_POINT ( 'NONE',  ( -18.25990335970915268, -0.1191753592594171213, 9.210292201204588025 ) ) ;
#31991=PLANE ( 'NONE',  #11425 ) ;
#31992=DIRECTION ( 'NONE',  ( 0.9999697198139515519, 0.000000000000000000, 0.007781995580013368816 ) ) ;
#31993=CARTESIAN_POINT ( 'NONE',  ( -11.20636620717317378, 0.000000000000000000, 11.32298014792380414 ) ) ;
#31995=DIRECTION ( 'NONE',  ( 0.9999697198139515519, 0.000000000000000000, 0.007781995580013368816 ) ) ;
#31996=ORIENTED_EDGE ( 'NONE', *, *, #1158, .T. ) ;
#31997=FACE_OUTER_BOUND ( 'NONE', #22051, .T. ) ;
#31998=CARTESIAN_POINT ( 'NONE',  ( -14.20280369269832832, 0.000000000000000000, 12.40765738797303719 ) ) ;
#31999=DIRECTION ( 'NONE',  ( 0.000000000000000000, -0.000000000000000000, -1.000000000000000000 ) ) ;
#32000=AXIS2_PLACEMENT_3D ( 'NONE', #27663, #6356, #44989 ) ;
#32001=DIRECTION ( 'NONE',  ( 0.9999697198139515519, 0.000000000000000000, 0.007781995580013368816 ) ) ;
#32002=VECTOR ( 'NONE', #29935, 1000.000000000000227 ) ;
#32003=ADVANCED_FACE ( 'NONE', ( #45278 ), #40169, .F. ) ;
#32004=CARTESIAN_POINT ( 'NONE',  ( -11.61397488332059602, 0.000000000000000000, 3.991360347924631125 ) ) ;
#32008=CARTESIAN_POINT ( 'NONE',  ( -15.74363206212979094, -3.270328918600661439, 2.892341851553068999 ) ) ;
#32009=CARTESIAN_POINT ( 'NONE',  ( -14.01701317841955508, 0.000000000000000000, 2.326005055450897085 ) ) ;
#32010=VECTOR ( 'NONE', #50689, 1000.000000000000227 ) ;
#32012=ADVANCED_FACE ( 'NONE', ( #41299 ), #14897, .F. ) ;
#32013=DIRECTION ( 'NONE',  ( -0.6427681459581293666, -0.7660444431189770143, -0.005002170337467561935 ) ) ;
#32014=VECTOR ( 'NONE', #4559, 1000.000000000000000 ) ;
#32015=DIRECTION ( 'NONE',  ( -0.9321478471874541372, -0.000000000000000000, 0.3620778797217454326 ) ) ;
#32016=EDGE_CURVE ( 'NONE', #56039, #3193, #45014, .T. ) ;
#32017=DIRECTION ( 'NONE',  ( 0.5364919789714477361, 0.6444004775717706579, 0.5449076811759711036 ) ) ;
#32018=VECTOR ( 'NONE', #45996, 999.9999999999998863 ) ;
#32019=LINE ( 'NONE', #49341, #46432 ) ;
#32020=VECTOR ( 'NONE', #44440, 999.9999999999998863 ) ;
#32021=ADVANCED_FACE ( 'NONE', ( #2088 ), #28221, .F. ) ;
#32022=VECTOR ( 'NONE', #21859, 999.9999999999998863 ) ;
#32023=ORIENTED_EDGE ( 'NONE', *, *, #23206, .F. ) ;
#32024=EDGE_CURVE ( 'NONE', #13096, #12755, #48713, .T. ) ;
#32025=VECTOR ( 'NONE', #53725, 999.9999999999998863 ) ;
#32026=ORIENTED_EDGE ( 'NONE', *, *, #56114, .T. ) ;
#32027=ORIENTED_EDGE ( 'NONE', *, *, #18757, .F. ) ;
#32028=AXIS2_PLACEMENT_3D ( 'NONE', #13440, #17972, #652 ) ;
#32029=EDGE_LOOP ( 'NONE', ( #55016, #37205, #33570, #39938 ) ) ;
#32030=ORIENTED_EDGE ( 'NONE', *, *, #49518, .T. ) ;
#32031=FACE_OUTER_BOUND ( 'NONE', #48163, .T. ) ;
#32032=DIRECTION ( 'NONE',  ( 0.000000000000000000, -0.000000000000000000, -1.000000000000000000 ) ) ;
#32033=ORIENTED_EDGE ( 'NONE', *, *, #28198, .T. ) ;
#32034=ORIENTED_EDGE ( 'NONE', *, *, #24819, .F. ) ;
#32035=VECTOR ( 'NONE', #48223, 1000.000000000000227 ) ;
#32036=ORIENTED_EDGE ( 'NONE', *, *, #22498, .F. ) ;
#32037=VECTOR ( 'NONE', #43072, 1000.000000000000227 ) ;
#32038=DIRECTION ( 'NONE',  ( 0.7660212471507180654, -0.6427876096865404731, 0.005961354470445141482 ) ) ;
#32039=DIRECTION ( 'NONE',  ( 0.007781995580012662783, 0.000000000000000000, -0.9999697198139514409 ) ) ;
#32040=LINE ( 'NONE', #9916, #45837 ) ;
#32042=CARTESIAN_POINT ( 'NONE',  ( -17.26532721389163072, 0.000000000000000000, 13.67648636611514590 ) ) ;
#32043=EDGE_CURVE ( 'NONE', #35922, #55515, #32226, .T. ) ;
#32044=VECTOR ( 'NONE', #5253, 1000.000000000000227 ) ;
#32045=ORIENTED_EDGE ( 'NONE', *, *, #12667, .T. ) ;
#32046=DIRECTION ( 'NONE',  ( 0.7660212471507180654, -0.6427876096865404731, 0.005961354470445141482 ) ) ;
#32047=EDGE_CURVE ( 'NONE', #41786, #428, #27970, .T. ) ;
#32048=CARTESIAN_POINT ( 'NONE',  ( 2.072287782118878319, 0.000000000000000000, -2.950529333540147015 ) ) ;
#32049=VECTOR ( 'NONE', #23079, 1000.000000000000227 ) ;
#32050=CARTESIAN_POINT ( 'NONE',  ( -12.87254409838392810, 2.391131607591507002, 1.605775395510381287 ) ) ;
#32051=LINE ( 'NONE', #9341, #47806 ) ;
#32052=EDGE_CURVE ( 'NONE', #42377, #41065, #23429, .T. ) ;
#32053=PLANE ( 'NONE',  #55805 ) ;
#32054=LINE ( 'NONE', #15841, #18406 ) ;
#32055=DIRECTION ( 'NONE',  ( -0.7660212471507179544, -0.6427876096865405842, -0.005961354470445141482 ) ) ;
#32056=EDGE_CURVE ( 'NONE', #36173, #41663, #6651, .T. ) ;
#32057=AXIS2_PLACEMENT_3D ( 'NONE', #27076, #4932, #44116 ) ;
#32058=ORIENTED_EDGE ( 'NONE', *, *, #54155, .T. ) ;
#32059=DIRECTION ( 'NONE',  ( 0.000000000000000000, -1.000000000000000000, 0.000000000000000000 ) ) ;
#32060=ORIENTED_EDGE ( 'NONE', *, *, #30324, .T. ) ;
#32061=ADVANCED_FACE ( 'NONE', ( #40745 ), #14357, .F. ) ;
#32062=EDGE_CURVE ( 'NONE', #15806, #28385, #24512, .T. ) ;
#32063=ADVANCED_FACE ( 'NONE', ( #55188 ), #7478, .F. ) ;
#32064=AXIS2_PLACEMENT_3D ( 'NONE', #5444, #9726, #44069 ) ;
#32065=VECTOR ( 'NONE', #34876, 1000.000000000000227 ) ;
#32066=DIRECTION ( 'NONE',  ( 0.5449076811759707706, 0.6444004775717708799, -0.5364919789714476250 ) ) ;
#32067=PLANE ( 'NONE',  #19611 ) ;
#32068=DIRECTION ( 'NONE',  ( 0.5449076811759707706, 0.6444004775717708799, -0.5364919789714476250 ) ) ;
#32069=CARTESIAN_POINT ( 'NONE',  ( -17.88873712828089424, 0.000000000000000000, 8.374513534917676694 ) ) ;
#32070=CARTESIAN_POINT ( 'NONE',  ( -16.51274120858988681, -5.213152330870661544, 11.65171230228703969 ) ) ;
#32071=LINE ( 'NONE', #36074, #17672 ) ;
#32072=CARTESIAN_POINT ( 'NONE',  ( -15.60102546347950536, 0.000000000000000000, 12.95077420755565356 ) ) ;
#32073=VECTOR ( 'NONE', #11424, 999.9999999999998863 ) ;
#32074=FACE_OUTER_BOUND ( 'NONE', #42537, .T. ) ;
#32076=SURFACE_SIDE_STYLE ('',( #1106 ) ) ;
#32077=LINE ( 'NONE', #11032, #4771 ) ;
#32078=EDGE_LOOP ( 'NONE', ( #43332, #321, #33639, #31752 ) ) ;
#32079=FACE_OUTER_BOUND ( 'NONE', #52546, .T. ) ;
#32080=CARTESIAN_POINT ( 'NONE',  ( -14.63931068118123591, -4.727446477803164626, 2.416896245294180012 ) ) ;
#32081=PLANE ( 'NONE',  #13711 ) ;
#32082=LINE ( 'NONE', #49106, #24029 ) ;
#32083=CARTESIAN_POINT ( 'NONE',  ( -16.70141711715487887, 4.172053068839010947, 3.036218986314767943 ) ) ;
#32084=EDGE_CURVE ( 'NONE', #46919, #53826, #37586, .T. ) ;
#32085=CARTESIAN_POINT ( 'NONE',  ( -19.79569077582305070, 0.000000000000000000, 14.58012466630350445 ) ) ;
#32086=LINE ( 'NONE', #53115, #32373 ) ;
#32087=CARTESIAN_POINT ( 'NONE',  ( 1.710209902397132220, -1.000000000000000000, -3.882677180727601041 ) ) ;
#32088=VERTEX_POINT ( 'NONE', #33346 ) ;
#32089=ADVANCED_FACE ( 'NONE', ( #20820 ), #38138, .F. ) ;
#32090=ORIENTED_EDGE ( 'NONE', *, *, #21748, .F. ) ;
#32091=AXIS2_PLACEMENT_3D ( 'NONE', #14577, #1219, #45239 ) ;
#32092=ADVANCED_FACE ( 'NONE', ( #45824 ), #11746, .F. ) ;
#32093=CARTESIAN_POINT ( 'NONE',  ( -14.86643316120819591, 0.000000000000000000, 3.966048965548564453 ) ) ;
#32094=CARTESIAN_POINT ( 'NONE',  ( -10.22868635331318643, 0.000000000000000000, 5.110137193001952127 ) ) ;
#32095=AXIS2_PLACEMENT_3D ( 'NONE', #4475, #47066, #38841 ) ;
#32096=ADVANCED_FACE ( 'NONE', ( #41828 ), #24262, .F. ) ;
#32097=EDGE_LOOP ( 'NONE', ( #5578, #40852, #18022, #55108 ) ) ;
#32098=DIRECTION ( 'NONE',  ( -0.6427681459581293666, -0.7660444431189770143, -0.005002170337467561935 ) ) ;
#32099=VECTOR ( 'NONE', #40233, 999.9999999999998863 ) ;
#32100=ORIENTED_EDGE ( 'NONE', *, *, #42452, .F. ) ;
#32101=CARTESIAN_POINT ( 'NONE',  ( -12.99794575893872839, 0.000000000000000000, 2.703267743552332014 ) ) ;
#32102=EDGE_LOOP ( 'NONE', ( #8055, #45545, #47044, #40313 ) ) ;
#32103=ORIENTED_EDGE ( 'NONE', *, *, #43314, .T. ) ;
#32104=ORIENTED_EDGE ( 'NONE', *, *, #40505, .F. ) ;
#32105=DIRECTION ( 'NONE',  ( 0.9999697198139515519, 0.000000000000000000, 0.007781995580013368816 ) ) ;
#32106=AXIS2_PLACEMENT_3D ( 'NONE', #7724, #38374, #51457 ) ;
#32107=LINE ( 'NONE', #15335, #31396 ) ;
#32108=DIRECTION ( 'NONE',  ( -0.5364919789714478471, 0.6444004775717705469, -0.5449076811759709926 ) ) ;
#32109=VECTOR ( 'NONE', #49973, 999.9999999999998863 ) ;
#32110=ORIENTED_EDGE ( 'NONE', *, *, #54553, .T. ) ;
#32111=EDGE_LOOP ( 'NONE', ( #7730, #6693, #40339, #27549 ) ) ;
#32112=AXIS2_PLACEMENT_3D ( 'NONE', #21554, #21809, #30055 ) ;
#32113=VECTOR ( 'NONE', #15720, 999.9999999999998863 ) ;
#32114=FACE_OUTER_BOUND ( 'NONE', #22721, .T. ) ;
#32115=ORIENTED_EDGE ( 'NONE', *, *, #3653, .F. ) ;
#32116=PLANE ( 'NONE',  #23004 ) ;
#32117=VERTEX_POINT ( 'NONE', #29061 ) ;
#32118=CARTESIAN_POINT ( 'NONE',  ( -10.30934315031560544, -0.1191753592594188005, 2.624188042620991368 ) ) ;
#32119=LINE ( 'NONE', #40902, #53001 ) ;
#32121=DIRECTION ( 'NONE',  ( 0.007781995580012663651, 0.000000000000000000, -0.9999697198139515519 ) ) ;
#32122=VECTOR ( 'NONE', #45183, 999.9999999999998863 ) ;
#32123=LINE ( 'NONE', #1462, #37249 ) ;
#32124=AXIS2_PLACEMENT_3D ( 'NONE', #42441, #21429, #43298 ) ;
#32126=FACE_OUTER_BOUND ( 'NONE', #37221, .T. ) ;
#32127=DIRECTION ( 'NONE',  ( 0.9999697198139515519, 0.000000000000000000, 0.007781995580013368816 ) ) ;
#32128=LINE ( 'NONE', #49451, #29209 ) ;
#32129=ORIENTED_EDGE ( 'NONE', *, *, #23846, .T. ) ;
#32130=AXIS2_PLACEMENT_3D ( 'NONE', #27747, #19189, #27438 ) ;
#32131=EDGE_CURVE ( 'NONE', #36758, #3085, #41570, .T. ) ;
#32132=EDGE_CURVE ( 'NONE', #23151, #53142, #2652, .T. ) ;
#32133=LINE ( 'NONE', #1169, #29217 ) ;
#32134=CARTESIAN_POINT ( 'NONE',  ( -17.74560456716937296, 0.000000000000000000, 3.774316574337878372 ) ) ;
#32135=DIRECTION ( 'NONE',  ( -0.005002170337468016433, -0.7660444431189770143, 0.6427681459581293666 ) ) ;
#32136=VECTOR ( 'NONE', #18716, 999.9999999999998863 ) ;
#32137=DIRECTION ( 'NONE',  ( -0.3313982828793700097, 0.4028455766673915694, -0.8531650599175529814 ) ) ;
#32138=EDGE_CURVE ( 'NONE', #33548, #41210, #28805, .T. ) ;
#32139=FACE_OUTER_BOUND ( 'NONE', #25347, .T. ) ;
#32142=ORIENTED_EDGE ( 'NONE', *, *, #38249, .T. ) ;
#32143=CARTESIAN_POINT ( 'NONE',  ( -15.75281958048178232, 1.905425754524005200, 6.127379490061689360 ) ) ;
#32144=DIRECTION ( 'NONE',  ( 0.005002170337468016433, -0.7660444431189770143, -0.6427681459581293666 ) ) ;
#32146=ORIENTED_EDGE ( 'NONE', *, *, #44909, .T. ) ;
#32147=AXIS2_PLACEMENT_3D ( 'NONE', #44516, #41402, #28314 ) ;
#32148=CARTESIAN_POINT ( 'NONE',  ( -16.53317331066696383, 0.000000000000000000, 13.31285208727739899 ) ) ;
#32149=LINE ( 'NONE', #54002, #51727 ) ;
#32150=VECTOR ( 'NONE', #33332, 1000.000000000000227 ) ;
#32151=CARTESIAN_POINT ( 'NONE',  ( -19.60990026154428278, 0.000000000000000000, 4.498472333781370125 ) ) ;
#32152=DIRECTION ( 'NONE',  ( -0.5449076811759708816, 0.6444004775717707689, 0.5364919789714475140 ) ) ;
#32153=ADVANCED_FACE ( 'NONE', ( #16555 ), #46960, .F. ) ;
#32154=PLANE ( 'NONE',  #43792 ) ;
#32155=ORIENTED_EDGE ( 'NONE', *, *, #26168, .F. ) ;
#32156=VECTOR ( 'NONE', #14432, 999.9999999999998863 ) ;
#32157=AXIS2_PLACEMENT_3D ( 'NONE', #3083, #51063, #20706 ) ;
#32158=VERTEX_POINT ( 'NONE', #7785 ) ;
#32159=ADVANCED_FACE ( 'NONE', ( #12322 ), #2919, .F. ) ;
#32160=DIRECTION ( 'NONE',  ( -0.005961354470445682716, -0.6427876096865404731, 0.7660212471507180654 ) ) ;
#32161=LINE ( 'NONE', #35873, #17840 ) ;
#32162=DIRECTION ( 'NONE',  ( -0.9999697198139514409, -0.000000000000000000, -0.007781995580013368816 ) ) ;
#32163=ADVANCED_FACE ( 'NONE', ( #29661 ), #25372, .F. ) ;
#32164=ORIENTED_EDGE ( 'NONE', *, *, #10539, .T. ) ;
#32165=FACE_OUTER_BOUND ( 'NONE', #42880, .T. ) ;
#32166=EDGE_LOOP ( 'NONE', ( #41339, #45995, #23398, #34047 ) ) ;
#32167=FACE_OUTER_BOUND ( 'NONE', #44320, .T. ) ;
#32168=VECTOR ( 'NONE', #38863, 1000.000000000000227 ) ;
#32169=ORIENTED_EDGE ( 'NONE', *, *, #4522, .T. ) ;
#32170=VECTOR ( 'NONE', #28396, 999.9999999999998863 ) ;
#32171=CARTESIAN_POINT ( 'NONE',  ( -16.81345671998191449, 0.000000000000000000, 3.412238694616132495 ) ) ;
#32173=EDGE_CURVE ( 'NONE', #55867, #49289, #3227, .T. ) ;
#32174=VECTOR ( 'NONE', #47721, 1000.000000000000114 ) ;
#32175=FACE_OUTER_BOUND ( 'NONE', #158, .T. ) ;
#32176=EDGE_LOOP ( 'NONE', ( #35110, #19169, #22413, #50955, #2409 ) ) ;
#32177=CARTESIAN_POINT ( 'NONE',  ( -19.98224170412465028, 0.000000000000000000, 4.543407702002897786 ) ) ;
#32178=VECTOR ( 'NONE', #4533, 1000.000000000000227 ) ;
#32179=ORIENTED_EDGE ( 'NONE', *, *, #6827, .F. ) ;
#32180=ORIENTED_EDGE ( 'NONE', *, *, #40608, .F. ) ;
#32182=DIRECTION ( 'NONE',  ( -0.005961354470445682716, -0.6427876096865404731, 0.7660212471507180654 ) ) ;
#32183=VECTOR ( 'NONE', #27108, 1000.000000000000000 ) ;
#32184=ORIENTED_EDGE ( 'NONE', *, *, #23733, .T. ) ;
#32185=VECTOR ( 'NONE', #40513, 1000.000000000000000 ) ;
#32186=FACE_OUTER_BOUND ( 'NONE', #30535, .T. ) ;
#32187=ORIENTED_EDGE ( 'NONE', *, *, #15200, .F. ) ;
#32188=DIRECTION ( 'NONE',  ( 0.7660212471507180654, -0.6427876096865404731, 0.005961354470445141482 ) ) ;
#32189=DIRECTION ( 'NONE',  ( 0.9999697198139515519, 0.000000000000000000, 0.007781995580013368816 ) ) ;
#32190=AXIS2_PLACEMENT_3D ( 'NONE', #24434, #42031, #6860 ) ;
#32192=CARTESIAN_POINT ( 'NONE',  ( -18.36487023914310512, 0.000000000000000000, 9.848136436180725539 ) ) ;
#32193=ORIENTED_EDGE ( 'NONE', *, *, #18421, .F. ) ;
#32194=VECTOR ( 'NONE', #45544, 999.9999999999998863 ) ;
#32195=PLANE ( 'NONE',  #23762 ) ;
#32196=VECTOR ( 'NONE', #7538, 1000.000000000000000 ) ;
#32197=CARTESIAN_POINT ( 'NONE',  ( -12.55187083751861721, 0.000000000000000000, 5.092057634161903934 ) ) ;
#32198=FACE_OUTER_BOUND ( 'NONE', #27989, .T. ) ;
#32199=CARTESIAN_POINT ( 'NONE',  ( -12.10922913985712412, 0.000000000000000000, 7.922009404736876981 ) ) ;
#32200=LINE ( 'NONE', #19954, #32363 ) ;
#32201=CARTESIAN_POINT ( 'NONE',  ( 2.072287782118878319, 0.000000000000000000, -2.950529333540147015 ) ) ;
#32202=LINE ( 'NONE', #31650, #8399 ) ;
#32203=ORIENTED_EDGE ( 'NONE', *, *, #24520, .F. ) ;
#32204=ADVANCED_FACE ( 'NONE', ( #54344 ), #15435, .F. ) ;
#32205=VERTEX_POINT ( 'NONE', #33050 ) ;
#32206=CARTESIAN_POINT ( 'NONE',  ( -14.94916102560700821, 0.000000000000000000, 2.688082935172642962 ) ) ;
#32207=DIRECTION ( 'NONE',  ( 0.007781995580012663651, 0.000000000000000000, -0.9999697198139515519 ) ) ;
#32208=EDGE_CURVE ( 'NONE', #33959, #34435, #39265, .T. ) ;
#32209=ADVANCED_FACE ( 'NONE', ( #34723 ), #8619, .F. ) ;
#32210=DIRECTION ( 'NONE',  ( -0.9999697198139514409, -0.000000000000000000, -0.007781995580013368816 ) ) ;
#32211=AXIS2_PLACEMENT_3D ( 'NONE', #9533, #43046, #980 ) ;
#32213=ORIENTED_EDGE ( 'NONE', *, *, #53096, .F. ) ;
#32214=VECTOR ( 'NONE', #19464, 999.9999999999998863 ) ;
#32215=DIRECTION ( 'NONE',  ( -0.005961354470445682716, -0.6427876096865404731, 0.7660212471507180654 ) ) ;
#32216=CARTESIAN_POINT ( 'NONE',  ( 2.072287782118878319, 0.000000000000000000, -2.950529333540147015 ) ) ;
#32217=ORIENTED_EDGE ( 'NONE', *, *, #56147, .T. ) ;
#32218=FACE_OUTER_BOUND ( 'NONE', #5988, .T. ) ;
#32219=LINE ( 'NONE', #23139, #28554 ) ;
#32220=VECTOR ( 'NONE', #43331, 999.9999999999998863 ) ;
#32221=ORIENTED_EDGE ( 'NONE', *, *, #49474, .T. ) ;
#32223=FACE_OUTER_BOUND ( 'NONE', #46455, .T. ) ;
#32224=VECTOR ( 'NONE', #25226, 1000.000000000000114 ) ;
#32225=FACE_OUTER_BOUND ( 'NONE', #18896, .T. ) ;
#32226=LINE ( 'NONE', #53264, #37755 ) ;
#32227=ADVANCED_FACE ( 'NONE', ( #13155 ), #43793, .F. ) ;
#32228=DIRECTION ( 'NONE',  ( -0.3620778797217457101, 0.000000000000000000, -0.9321478471874540261 ) ) ;
#32229=ORIENTED_EDGE ( 'NONE', *, *, #41123, .F. ) ;
#32231=VECTOR ( 'NONE', #5243, 1000.000000000000227 ) ;
#32232=ORIENTED_EDGE ( 'NONE', *, *, #7859, .T. ) ;
#32233=VECTOR ( 'NONE', #10284, 1000.000000000000000 ) ;
#32234=LINE ( 'NONE', #33057, #3066 ) ;
#32235=PLANE ( 'NONE',  #34975 ) ;
#32236=DIRECTION ( 'NONE',  ( 0.005002170337468016433, -0.7660444431189770143, -0.6427681459581293666 ) ) ;
#32237=AXIS2_PLACEMENT_3D ( 'NONE', #13305, #30631, #9030 ) ;
#32238=VECTOR ( 'NONE', #35142, 1000.000000000000000 ) ;
#32240=DIRECTION ( 'NONE',  ( -0.5364919789714478471, 0.6444004775717705469, -0.5449076811759709926 ) ) ;
#32241=VERTEX_POINT ( 'NONE', #47507 ) ;
#32243=ADVANCED_FACE ( 'NONE', ( #30763 ), #9160, .F. ) ;
#32244=AXIS2_PLACEMENT_3D ( 'NONE', #29278, #51447, #42620 ) ;
#32246=VECTOR ( 'NONE', #33528, 1000.000000000000227 ) ;
#32247=LINE ( 'NONE', #23694, #55933 ) ;
#32248=ORIENTED_EDGE ( 'NONE', *, *, #49388, .F. ) ;
#32249=EDGE_CURVE ( 'NONE', #19711, #40042, #4910, .T. ) ;
#32250=PLANE ( 'NONE',  #17512 ) ;
#32251=ORIENTED_EDGE ( 'NONE', *, *, #29648, .F. ) ;
#32252=DIRECTION ( 'NONE',  ( -0.5364919789714478471, 0.6444004775717705469, -0.5449076811759709926 ) ) ;
#32253=CARTESIAN_POINT ( 'NONE',  ( -14.61484282146703251, 0.000000000000000000, 5.645341235194416107 ) ) ;
#32254=EDGE_LOOP ( 'NONE', ( #36234, #8860, #13675, #9471 ) ) ;
#32255=DIRECTION ( 'NONE',  ( 0.005002170337468016433, -0.7660444431189770143, -0.6427681459581293666 ) ) ;
#32256=EDGE_CURVE ( 'NONE', #5924, #29543, #658, .T. ) ;
#32257=ORIENTED_EDGE ( 'NONE', *, *, #18491, .F. ) ;
#32258=AXIS2_PLACEMENT_3D ( 'NONE', #30194, #4918, #12604 ) ;
#32259=EDGE_LOOP ( 'NONE', ( #42190, #23465, #39857, #33175, #55131, #53175, #45353, #49803 ) ) ;
#32260=ORIENTED_EDGE ( 'NONE', *, *, #48746, .F. ) ;
#32262=EDGE_LOOP ( 'NONE', ( #7943, #50868, #12826, #38648 ) ) ;
#32263=AXIS2_PLACEMENT_3D ( 'NONE', #45869, #54956, #28841 ) ;
#32264=ORIENTED_EDGE ( 'NONE', *, *, #26646, .T. ) ;
#32265=FACE_OUTER_BOUND ( 'NONE', #35495, .T. ) ;
#32266=AXIS2_PLACEMENT_3D ( 'NONE', #25945, #42668, #38987 ) ;
#32267=ORIENTED_EDGE ( 'NONE', *, *, #43242, .T. ) ;
#32268=VERTEX_POINT ( 'NONE', #21095 ) ;
#32269=FACE_OUTER_BOUND ( 'NONE', #10406, .T. ) ;
#32270=ORIENTED_EDGE ( 'NONE', *, *, #47652, .F. ) ;
#32271=AXIS2_PLACEMENT_3D ( 'NONE', #42030, #3130, #15360 ) ;
#32272=ORIENTED_EDGE ( 'NONE', *, *, #46888, .T. ) ;
#32273=ADVANCED_FACE ( 'NONE', ( #52346 ), #17980, .F. ) ;
#32275=AXIS2_PLACEMENT_3D ( 'NONE', #25392, #30517, #25134 ) ;
#32276=DIRECTION ( 'NONE',  ( 0.9999697198139515519, 0.000000000000000000, 0.007781995580013368816 ) ) ;
#32277=CARTESIAN_POINT ( 'NONE',  ( -15.42897117608339741, -0.1191753592594185229, 3.692342122946178584 ) ) ;
#32278=DIRECTION ( 'NONE',  ( 0.9999697198139515519, 0.000000000000000000, 0.007781995580013368816 ) ) ;
#32279=DIRECTION ( 'NONE',  ( 0.005961354470445682716, -0.6427876096865404731, -0.7660212471507180654 ) ) ;
#32280=EDGE_CURVE ( 'NONE', #10313, #36287, #52040, .T. ) ;
#32281=ORIENTED_EDGE ( 'NONE', *, *, #21580, .T. ) ;
#32282=DIRECTION ( 'NONE',  ( -0.7660212471507179544, -0.6427876096865405842, -0.005961354470445141482 ) ) ;
#32283=EDGE_LOOP ( 'NONE', ( #36317, #16313, #15375, #47643 ) ) ;
#32284=VECTOR ( 'NONE', #20819, 999.9999999999998863 ) ;
#32285=VECTOR ( 'NONE', #13808, 999.9999999999998863 ) ;
#32286=EDGE_CURVE ( 'NONE', #33398, #8024, #13698, .T. ) ;
#32287=AXIS2_PLACEMENT_3D ( 'NONE', #45541, #43949, #1054 ) ;
#32288=CARTESIAN_POINT ( 'NONE',  ( -17.46532115785441519, 0.000000000000000000, 13.67492996699914265 ) ) ;
#32289=EDGE_CURVE ( 'NONE', #21088, #40269, #12598, .T. ) ;
#32290=AXIS2_PLACEMENT_3D ( 'NONE', #35318, #9182, #52616 ) ;
#32291=CARTESIAN_POINT ( 'NONE',  ( -13.08330893211609869, 0.000000000000000000, 1.763933231766363630 ) ) ;
#32292=VECTOR ( 'NONE', #6722, 1000.000000000000227 ) ;
#32293=DIRECTION ( 'NONE',  ( -0.005961354470445682716, -0.6427876096865404731, 0.7660212471507180654 ) ) ;
#32294=LINE ( 'NONE', #49861, #6720 ) ;
#32295=DIRECTION ( 'NONE',  ( -0.6427681459581293666, -0.7660444431189770143, -0.005002170337467561935 ) ) ;
#32296=VERTEX_POINT ( 'NONE', #21680 ) ;
#32297=DIRECTION ( 'NONE',  ( 0.9999697198139515519, 0.000000000000000000, 0.007781995580013368816 ) ) ;
#32298=ORIENTED_EDGE ( 'NONE', *, *, #24328, .T. ) ;
#32299=EDGE_CURVE ( 'NONE', #24601, #47628, #31011, .T. ) ;
#32300=LINE ( 'NONE', #54673, #40127 ) ;
#32301=LINE ( 'NONE', #53325, #13308 ) ;
#32302=CARTESIAN_POINT ( 'NONE',  ( -26.13337879274045505, 0.000000000000000000, 6.833023547870798353 ) ) ;
#32303=CARTESIAN_POINT ( 'NONE',  ( -21.47341775636118655, -0.1191753592594197858, 5.122631121243466090 ) ) ;
#32304=CARTESIAN_POINT ( 'NONE',  ( -10.86457665906423919, 0.000000000000000000, 1.411867849540296094 ) ) ;
#32305=AXIS2_PLACEMENT_3D ( 'NONE', #48989, #10088, #23163 ) ;
#32306=EDGE_CURVE ( 'NONE', #37808, #636, #43521, .T. ) ;
#32307=ORIENTED_EDGE ( 'NONE', *, *, #38449, .T. ) ;
#32308=CARTESIAN_POINT ( 'NONE',  ( -11.91475904335884017, -1.489407457353156827, 1.461898260748682787 ) ) ;
#32309=DIRECTION ( 'NONE',  ( -0.5449076811759708816, 0.6444004775717707689, 0.5364919789714475140 ) ) ;
#32310=CARTESIAN_POINT ( 'NONE',  ( -12.33850799832341849, 0.000000000000000000, 11.68350162852954632 ) ) ;
#32311=AXIS2_PLACEMENT_3D ( 'NONE', #32501, #14887, #23670 ) ;
#32312=FACE_OUTER_BOUND ( 'NONE', #31934, .T. ) ;
#32313=VECTOR ( 'NONE', #11025, 1000.000000000000227 ) ;
#32314=CARTESIAN_POINT ( 'NONE',  ( -11.20636620717317378, 0.000000000000000000, 11.32298014792380414 ) ) ;
#32315=CARTESIAN_POINT ( 'NONE',  ( -10.31221720382088947, -0.1191753592594183703, 2.993497745878755278 ) ) ;
#32316=LINE ( 'NONE', #49632, #2931 ) ;
#32317=VECTOR ( 'NONE', #23541, 1000.000000000000114 ) ;
#32318=VECTOR ( 'NONE', #26251, 999.9999999999998863 ) ;
#32319=CARTESIAN_POINT ( 'NONE',  ( -17.67981966024466800, -0.03228989815065527041, 3.747733265616297160 ) ) ;
#32320=CARTESIAN_POINT ( 'NONE',  ( -21.45016440283565373, -5.536956232915663634, 14.10099251443048729 ) ) ;
#32321=ORIENTED_EDGE ( 'NONE', *, *, #40844, .F. ) ;
#32322=AXIS2_PLACEMENT_3D ( 'NONE', #16021, #33345, #35490 ) ;
#32323=VERTEX_POINT ( 'NONE', #34193 ) ;
#32324=AXIS2_PLACEMENT_3D ( 'NONE', #403, #27360, #18019 ) ;
#32325=EDGE_CURVE ( 'NONE', #54313, #17993, #30493, .T. ) ;
#32326=VECTOR ( 'NONE', #12262, 999.9999999999998863 ) ;
#32327=EDGE_LOOP ( 'NONE', ( #35908, #12327, #32217, #19803 ) ) ;
#32328=VECTOR ( 'NONE', #27317, 1000.000000000000227 ) ;
#32329=EDGE_LOOP ( 'NONE', ( #35201, #26437, #13045, #18463, #17257 ) ) ;
#32330=ORIENTED_EDGE ( 'NONE', *, *, #52157, .T. ) ;
#32331=ORIENTED_EDGE ( 'NONE', *, *, #34231, .F. ) ;
#32332=LINE ( 'NONE', #36042, #51408 ) ;
#32333=PLANE ( 'NONE',  #8594 ) ;
#32334=EDGE_CURVE ( 'NONE', #12044, #29102, #29916, .T. ) ;
#32335=ORIENTED_EDGE ( 'NONE', *, *, #16285, .T. ) ;
#32336=LINE ( 'NONE', #11284, #55795 ) ;
#32337=ORIENTED_EDGE ( 'NONE', *, *, #52736, .F. ) ;
#32338=ADVANCED_FACE ( 'NONE', ( #4625 ), #38732, .F. ) ;
#32339=ADVANCED_FACE ( 'NONE', ( #12866 ), #30189, .F. ) ;
#32340=AXIS2_PLACEMENT_3D ( 'NONE', #24705, #12778, #38333 ) ;
#32341=DIRECTION ( 'NONE',  ( -0.7660212471507179544, -0.6427876096865405842, -0.005961354470445141482 ) ) ;
#32342=CARTESIAN_POINT ( 'NONE',  ( -23.33849165029409889, 0.000000000000000000, 5.946783852668351855 ) ) ;
#32343=CARTESIAN_POINT ( 'NONE',  ( -14.46888367232926420, 0.000000000000000000, 12.59025272694991315 ) ) ;
#32344=ORIENTED_EDGE ( 'NONE', *, *, #15506, .T. ) ;
#32345=VECTOR ( 'NONE', #38069, 999.9999999999998863 ) ;
#32346=DIRECTION ( 'NONE',  ( 0.5364919789714477361, 0.6444004775717706579, 0.5449076811759711036 ) ) ;
#32347=CARTESIAN_POINT ( 'NONE',  ( -18.39746900504187010, 0.000000000000000000, 14.03700784672088808 ) ) ;
#32348=EDGE_CURVE ( 'NONE', #18224, #49166, #10593, .T. ) ;
#32349=VECTOR ( 'NONE', #50075, 999.9999999999998863 ) ;
#32350=FACE_OUTER_BOUND ( 'NONE', #10595, .T. ) ;
#32351=EDGE_CURVE ( 'NONE', #50681, #34828, #31312, .T. ) ;
#32352=CARTESIAN_POINT ( 'NONE',  ( -24.27063949748155380, 0.000000000000000000, 6.308861732390097288 ) ) ;
#32353=DIRECTION ( 'NONE',  ( 0.5449076811759707706, 0.6444004775717708799, -0.5364919789714476250 ) ) ;
#32354=AXIS2_PLACEMENT_3D ( 'NONE', #47347, #13002, #44236 ) ;
#32355=FACE_OUTER_BOUND ( 'NONE', #10874, .T. ) ;
#32356=DIRECTION ( 'NONE',  ( -0.9999697198139514409, -0.000000000000000000, -0.007781995580013368816 ) ) ;
#32357=DIRECTION ( 'NONE',  ( 0.8531650599175529814, -0.4028455766673920135, -0.3313982828793697877 ) ) ;
#32358=CARTESIAN_POINT ( 'NONE',  ( -10.16199474375293299, 7.791337327497334542, 0.7288902856039674027 ) ) ;
#32359=ORIENTED_EDGE ( 'NONE', *, *, #10148, .T. ) ;
#32360=CARTESIAN_POINT ( 'NONE',  ( -20.54049170961573267, 0.000000000000000000, 4.660556269540326646 ) ) ;
#32361=ORIENTED_EDGE ( 'NONE', *, *, #49833, .T. ) ;
#32362=EDGE_CURVE ( 'NONE', #30431, #52995, #40680, .T. ) ;
#32363=VECTOR ( 'NONE', #46083, 1000.000000000000227 ) ;
#32364=CARTESIAN_POINT ( 'NONE',  ( -30.79489622823572859, -0.1191753592594197858, 8.743409918460921304 ) ) ;
#32365=PLANE ( 'NONE',  #28652 ) ;
#32366=DIRECTION ( 'NONE',  ( 0.7660212471507180654, -0.6427876096865404731, 0.005961354470445141482 ) ) ;
#32367=LINE ( 'NONE', #45385, #54067 ) ;
#32368=CARTESIAN_POINT ( 'NONE',  ( -7.804705230638511182, -7.507922520789255039, -0.1867610151785078776 ) ) ;
#32369=CARTESIAN_POINT ( 'NONE',  ( -11.94039625119647141, 2.391131607591507002, 1.243697515788635632 ) ) ;
#32370=DIRECTION ( 'NONE',  ( -0.6427681459581293666, -0.7660444431189770143, -0.005002170337467561935 ) ) ;
#32371=VECTOR ( 'NONE', #8800, 999.9999999999998863 ) ;
#32372=EDGE_CURVE ( 'NONE', #8391, #46530, #10005, .T. ) ;
#32373=VECTOR ( 'NONE', #49403, 999.9999999999998863 ) ;
#32374=CARTESIAN_POINT ( 'NONE',  ( 2.072287782118878319, 0.000000000000000000, -2.950529333540147015 ) ) ;
#32376=FACE_OUTER_BOUND ( 'NONE', #50411, .T. ) ;
#32377=CARTESIAN_POINT ( 'NONE',  ( -18.67619601524082285, 0.000000000000000000, 3.936400510096834893 ) ) ;
#32378=CARTESIAN_POINT ( 'NONE',  ( -33.59056157024009082, 0.000000000000000000, 9.729646585644761814 ) ) ;
#32380=CARTESIAN_POINT ( 'NONE',  ( -24.27063949748155380, 0.000000000000000000, 6.308861732390097288 ) ) ;
#32381=LINE ( 'NONE', #36085, #30038 ) ;
#32382=DIRECTION ( 'NONE',  ( 0.6427681459581294776, -0.7660444431189769032, 0.005002170337467562802 ) ) ;
#32383=CARTESIAN_POINT ( 'NONE',  ( -13.08330893211609869, 0.000000000000000000, 1.763933231766363630 ) ) ;
#32384=DIRECTION ( 'NONE',  ( 0.000000000000000000, 1.000000000000000000, 0.000000000000000000 ) ) ;
#32385=VECTOR ( 'NONE', #22447, 1000.000000000000227 ) ;
#32386=VERTEX_POINT ( 'NONE', #5750 ) ;
#32387=ORIENTED_EDGE ( 'NONE', *, *, #1429, .F. ) ;
#32388=FACE_OUTER_BOUND ( 'NONE', #20722, .T. ) ;
#32389=LINE ( 'NONE', #45991, #47565 ) ;
#32390=ORIENTED_EDGE ( 'NONE', *, *, #37962, .T. ) ;
#32391=CARTESIAN_POINT ( 'NONE',  ( -23.33849165029409889, 0.000000000000000000, 5.946783852668351855 ) ) ;
#32392=AXIS2_PLACEMENT_3D ( 'NONE', #45620, #32840, #40821 ) ;
#32394=ORIENTED_EDGE ( 'NONE', *, *, #41651, .T. ) ;
#32395=DIRECTION ( 'NONE',  ( 0.005961354470445682716, -0.6427876096865404731, -0.7660212471507180654 ) ) ;
#32397=VERTEX_POINT ( 'NONE', #40099 ) ;
#32398=EDGE_LOOP ( 'NONE', ( #34504, #31718, #38875, #25597 ) ) ;
#32399=ADVANCED_FACE ( 'NONE', ( #40393 ), #36398, .F. ) ;
#32400=VERTEX_POINT ( 'NONE', #1490 ) ;
#32401=CARTESIAN_POINT ( 'NONE',  ( -18.26277741321443671, -0.1191753592594162470, 9.579601904462350603 ) ) ;
#32402=CARTESIAN_POINT ( 'NONE',  ( -17.20343699261858816, 2.553033558614008047, 3.282875753485510195 ) ) ;
#32403=CARTESIAN_POINT ( 'NONE',  ( -15.96710241509184058, -0.1191753592594218814, 13.13259134697452879 ) ) ;
#32404=EDGE_CURVE ( 'NONE', #39021, #11131, #19351, .T. ) ;
#32405=ADVANCED_FACE ( 'NONE', ( #49476 ), #44933, .F. ) ;
#32406=EDGE_CURVE ( 'NONE', #35922, #37629, #6313, .T. ) ;
#32408=ORIENTED_EDGE ( 'NONE', *, *, #15912, .T. ) ;
#32409=ORIENTED_EDGE ( 'NONE', *, *, #30139, .T. ) ;
#32410=EDGE_CURVE ( 'NONE', #20361, #20373, #53447, .T. ) ;
#32411=DIRECTION ( 'NONE',  ( -0.2426528472758542054, 0.7422098413412800966, -0.6246952433987894571 ) ) ;
#32412=VERTEX_POINT ( 'NONE', #27056 ) ;
#32413=CARTESIAN_POINT ( 'NONE',  ( -15.89648212642976510, -0.1191753592594206462, 4.058035914435935254 ) ) ;
#32414=ORIENTED_EDGE ( 'NONE', *, *, #11241, .T. ) ;
#32415=DIRECTION ( 'NONE',  ( 0.2426528472758542054, 0.7422098413412800966, 0.6246952433987894571 ) ) ;
#32417=ORIENTED_EDGE ( 'NONE', *, *, #35694, .T. ) ;
#32419=EDGE_CURVE ( 'NONE', #40411, #16890, #13985, .T. ) ;
#32420=EDGE_CURVE ( 'NONE', #44220, #47606, #23363, .T. ) ;
#32421=FACE_OUTER_BOUND ( 'NONE', #26277, .T. ) ;
#32422=ORIENTED_EDGE ( 'NONE', *, *, #17978, .F. ) ;
#32423=FACE_OUTER_BOUND ( 'NONE', #4464, .T. ) ;
#32424=EDGE_CURVE ( 'NONE', #25263, #32502, #40932, .T. ) ;
#32425=LINE ( 'NONE', #49727, #4741 ) ;
#32426=VERTEX_POINT ( 'NONE', #22780 ) ;
#32427=EDGE_CURVE ( 'NONE', #34236, #37134, #2016, .T. ) ;
#32428=DIRECTION ( 'NONE',  ( 0.000000000000000000, -0.000000000000000000, -1.000000000000000000 ) ) ;
#32429=DIRECTION ( 'NONE',  ( -0.8531650599175527594, 0.4028455766673922356, 0.3313982828793700652 ) ) ;
#32430=CARTESIAN_POINT ( 'NONE',  ( -11.30636317915456779, -0.1191753592594197858, 11.32220194836580340 ) ) ;
#32431=DIRECTION ( 'NONE',  ( 0.7660212471507180654, -0.6427876096865404731, 0.005961354470445141482 ) ) ;
#32432=LINE ( 'NONE', #7138, #6810 ) ;
#32433=DIRECTION ( 'NONE',  ( -0.005002170337468016433, -0.7660444431189770143, 0.6427681459581293666 ) ) ;
#32434=AXIS2_PLACEMENT_3D ( 'NONE', #726, #30269, #38500 ) ;
#32436=ORIENTED_EDGE ( 'NONE', *, *, #45917, .F. ) ;
#32437=CARTESIAN_POINT ( 'NONE',  ( -19.12962290826653700, 0.000000000000000000, 14.40064212555863854 ) ) ;
#32438=PLANE ( 'NONE',  #53160 ) ;
#32440=ORIENTED_EDGE ( 'NONE', *, *, #19801, .F. ) ;
#32441=CARTESIAN_POINT ( 'NONE',  ( -12.44241612666018071, 0.7721120973665049902, 1.490354282959377441 ) ) ;
#32442=DIRECTION ( 'NONE',  ( -0.5364919789714478471, 0.6444004775717705469, -0.5449076811759709926 ) ) ;
#32443=VECTOR ( 'NONE', #28488, 1000.000000000000227 ) ;
#32444=LINE ( 'NONE', #41508, #7738 ) ;
#32445=PLANE ( 'NONE',  #45972 ) ;
#32446=DIRECTION ( 'NONE',  ( 0.000000000000000000, -1.000000000000000000, 0.000000000000000000 ) ) ;
#32447=EDGE_LOOP ( 'NONE', ( #14441, #12551, #36127, #6073 ) ) ;
#32449=CARTESIAN_POINT ( 'NONE',  ( -20.47626320180702919, -0.03228989815065526348, 4.833966904781533458 ) ) ;
#32450=ADVANCED_FACE ( 'NONE', ( #15124 ), #32445, .F. ) ;
#32451=LINE ( 'NONE', #53198, #51980 ) ;
#32452=ORIENTED_EDGE ( 'NONE', *, *, #4015, .T. ) ;
#32453=DIRECTION ( 'NONE',  ( -0.9999697198139514409, -0.000000000000000000, -0.007781995580013368816 ) ) ;
#32454=EDGE_CURVE ( 'NONE', #46860, #606, #14295, .T. ) ;
#32455=ORIENTED_EDGE ( 'NONE', *, *, #52200, .F. ) ;
#32456=LINE ( 'NONE', #40692, #20151 ) ;
#32457=ORIENTED_EDGE ( 'NONE', *, *, #20747, .F. ) ;
#32459=FACE_OUTER_BOUND ( 'NONE', #25340, .T. ) ;
#32460=LINE ( 'NONE', #41240, #48609 ) ;
#32461=DIRECTION ( 'NONE',  ( -0.005002170337468016433, -0.7660444431189770143, 0.6427681459581293666 ) ) ;
#32462=EDGE_CURVE ( 'NONE', #47104, #48938, #1188, .T. ) ;
#32463=ADVANCED_FACE ( 'NONE', ( #53188 ), #48911, .F. ) ;
#32464=ADVANCED_FACE ( 'NONE', ( #55128 ), #16216, .F. ) ;
#32465=ORIENTED_EDGE ( 'NONE', *, *, #7648, .T. ) ;
#32466=DIRECTION ( 'NONE',  ( 0.005961354470445682716, -0.6427876096865404731, -0.7660212471507180654 ) ) ;
#32467=VERTEX_POINT ( 'NONE', #49998 ) ;
#32468=ADVANCED_FACE ( 'NONE', ( #11107 ), #15373, .F. ) ;
#32469=EDGE_LOOP ( 'NONE', ( #50302, #8355, #34893, #12351 ) ) ;
#32470=EDGE_LOOP ( 'NONE', ( #30219, #226, #24086, #46055 ) ) ;
#32471=DIRECTION ( 'NONE',  ( 0.5449076811759707706, 0.6444004775717708799, -0.5364919789714476250 ) ) ;
#32472=ORIENTED_EDGE ( 'NONE', *, *, #33166, .F. ) ;
#32473=DIRECTION ( 'NONE',  ( 0.000000000000000000, -0.000000000000000000, -1.000000000000000000 ) ) ;
#32474=VERTEX_POINT ( 'NONE', #11941 ) ;
#32475=FACE_OUTER_BOUND ( 'NONE', #29766, .T. ) ;
#32476=CARTESIAN_POINT ( 'NONE',  ( -18.59658094907401704, 0.000000000000000000, 5.614354428398334207 ) ) ;
#32477=AXIS2_PLACEMENT_3D ( 'NONE', #15362, #11094, #49735 ) ;
#32478=VERTEX_POINT ( 'NONE', #2847 ) ;
#32479=CARTESIAN_POINT ( 'NONE',  ( -14.16589384654164441, 0.000000000000000000, 7.664821422546224561 ) ) ;
#32480=ORIENTED_EDGE ( 'NONE', *, *, #28232, .T. ) ;
#32482=DIRECTION ( 'NONE',  ( -0.005002170337468016433, -0.7660444431189770143, 0.6427681459581293666 ) ) ;
#32483=DIRECTION ( 'NONE',  ( 0.6427681459581294776, -0.7660444431189769032, 0.005002170337467562802 ) ) ;
#32484=FACE_OUTER_BOUND ( 'NONE', #16675, .T. ) ;
#32485=FACE_OUTER_BOUND ( 'NONE', #34756, .T. ) ;
#32486=EDGE_CURVE ( 'NONE', #29459, #10313, #33537, .T. ) ;
#32487=LINE ( 'NONE', #40978, #42320 ) ;
#32488=FACE_OUTER_BOUND ( 'NONE', #3416, .T. ) ;
#32489=DIRECTION ( 'NONE',  ( 0.007781995580012663651, -3.146120232559066537E-19, -0.9999697198139514409 ) ) ;
#32490=ORIENTED_EDGE ( 'NONE', *, *, #19920, .T. ) ;
#32491=EDGE_CURVE ( 'NONE', #19751, #40803, #20485, .T. ) ;
#32492=ORIENTED_EDGE ( 'NONE', *, *, #40344, .F. ) ;
#32494=DIRECTION ( 'NONE',  ( 0.005961354470445682716, -0.6427876096865404731, -0.7660212471507180654 ) ) ;
#32495=CARTESIAN_POINT ( 'NONE',  ( -19.98318713347071096, 0.000000000000000000, 4.664893342615989091 ) ) ;
#32496=ADVANCED_FACE ( 'NONE', ( #7701 ), #25033, .F. ) ;
#32497=DIRECTION ( 'NONE',  ( 0.5364919789714477361, 0.6444004775717706579, 0.5449076811759711036 ) ) ;
#32498=DIRECTION ( 'NONE',  ( 0.6427681459581294776, -0.7660444431189769032, 0.005002170337467562802 ) ) ;
#32499=ORIENTED_EDGE ( 'NONE', *, *, #9707, .T. ) ;
#32500=FACE_OUTER_BOUND ( 'NONE', #38736, .T. ) ;
#32501=CARTESIAN_POINT ( 'NONE',  ( 2.072287782118878319, 0.000000000000000000, -2.950529333540147015 ) ) ;
#32502=VERTEX_POINT ( 'NONE', #50842 ) ;
#32503=LINE ( 'NONE', #6940, #13016 ) ;
#32504=CARTESIAN_POINT ( 'NONE',  ( -3.184760737835581335, 4.114927023055928501, -1.981304350158550776 ) ) ;
#32505=ORIENTED_EDGE ( 'NONE', *, *, #2928, .T. ) ;
#32506=CARTESIAN_POINT ( 'NONE',  ( -20.54204810873173415, 0.000000000000000000, 4.860550213503115558 ) ) ;
#32507=DIRECTION ( 'NONE',  ( -0.005961354470445682716, -0.6427876096865404731, 0.7660212471507180654 ) ) ;
#32508=CARTESIAN_POINT ( 'NONE',  ( -14.66887761629205222, 0.000000000000000000, 12.58869632783390990 ) ) ;
#32509=CARTESIAN_POINT ( 'NONE',  ( -14.46888367232926420, 0.000000000000000000, 12.59025272694991315 ) ) ;
#32511=VERTEX_POINT ( 'NONE', #36982 ) ;
#32513=CARTESIAN_POINT ( 'NONE',  ( -17.74404816805336793, 0.000000000000000000, 3.574322630375089460 ) ) ;
#32514=CARTESIAN_POINT ( 'NONE',  ( -10.37421533196711465, -0.1191753592594197858, 10.96012406864405975 ) ) ;
#32515=LINE ( 'NONE', #23435, #2494 ) ;
#32516=VECTOR ( 'NONE', #37804, 1000.000000000000227 ) ;
#32517=CARTESIAN_POINT ( 'NONE',  ( -23.33693525117809386, 0.000000000000000000, 5.746789908705562944 ) ) ;
#32518=CARTESIAN_POINT ( 'NONE',  ( -9.946799079403195520, 0.000000000000000000, 2.896338486107371324 ) ) ;
#32519=ORIENTED_EDGE ( 'NONE', *, *, #39586, .F. ) ;
#32520=FACE_OUTER_BOUND ( 'NONE', #11125, .T. ) ;
#32521=FACE_OUTER_BOUND ( 'NONE', #24129, .T. ) ;
#32523=EDGE_LOOP ( 'NONE', ( #3829, #26163, #22178, #7863 ) ) ;
#32524=DIRECTION ( 'NONE',  ( 0.9999697198139515519, 0.000000000000000000, 0.007781995580013368816 ) ) ;
#32525=FACE_OUTER_BOUND ( 'NONE', #40002, .T. ) ;
#32526=LINE ( 'NONE', #20280, #25735 ) ;
#32527=ADVANCED_FACE ( 'NONE', ( #15942 ), #41755, .F. ) ;
#32528=ORIENTED_EDGE ( 'NONE', *, *, #32419, .F. ) ;
#32529=CARTESIAN_POINT ( 'NONE',  ( -26.13337879274045505, 0.000000000000000000, 6.833023547870798353 ) ) ;
#32530=ORIENTED_EDGE ( 'NONE', *, *, #19893, .F. ) ;
#32531=ADVANCED_FACE ( 'NONE', ( #7403 ), #16482, .F. ) ;
#32532=ADVANCED_FACE ( 'NONE', ( #28154 ), #42045, .F. ) ;
#32533=EDGE_LOOP ( 'NONE', ( #33326, #5638, #20207, #39215 ) ) ;
#32534=ORIENTED_EDGE ( 'NONE', *, *, #43659, .F. ) ;
#32536=ORIENTED_EDGE ( 'NONE', *, *, #31181, .F. ) ;
#32537=ORIENTED_EDGE ( 'NONE', *, *, #12316, .T. ) ;
#32538=DIRECTION ( 'NONE',  ( 0.9999697198139515519, 0.000000000000000000, 0.007781995580013368816 ) ) ;
#32539=ORIENTED_EDGE ( 'NONE', *, *, #13665, .F. ) ;
#32540=ORIENTED_EDGE ( 'NONE', *, *, #23774, .F. ) ;
#32541=DIRECTION ( 'NONE',  ( -0.005961354470445682716, -0.6427876096865404731, 0.7660212471507180654 ) ) ;
#32542=ORIENTED_EDGE ( 'NONE', *, *, #9954, .T. ) ;
#32543=ORIENTED_EDGE ( 'NONE', *, *, #54830, .T. ) ;
#32544=EDGE_LOOP ( 'NONE', ( #22316, #22964, #49830 ) ) ;
#32545=CARTESIAN_POINT ( 'NONE',  ( -12.74192496657627949, 0.000000000000000000, 3.813256365977633067 ) ) ;
#32546=PLANE ( 'NONE',  #1304 ) ;
#32548=DIRECTION ( 'NONE',  ( -0.005002170337468016433, -0.7660444431189770143, 0.6427681459581293666 ) ) ;
#32549=ORIENTED_EDGE ( 'NONE', *, *, #41880, .F. ) ;
#32550=CARTESIAN_POINT ( 'NONE',  ( -13.47120481629566058, 0.000000000000000000, 3.807580941557616949 ) ) ;
#32551=VERTEX_POINT ( 'NONE', #19651 ) ;
#32552=AXIS2_PLACEMENT_3D ( 'NONE', #35023, #8904, #52333 ) ;
#32553=ORIENTED_EDGE ( 'NONE', *, *, #49173, .T. ) ;
#32554=DIRECTION ( 'NONE',  ( 0.007781995580012663651, 0.000000000000000000, -0.9999697198139515519 ) ) ;
#32555=EDGE_CURVE ( 'NONE', #4269, #26373, #54278, .T. ) ;
#32557=CARTESIAN_POINT ( 'NONE',  ( -15.81552396586975640, -0.03228989815065647778, 3.023577506172806739 ) ) ;
#32558=EDGE_CURVE ( 'NONE', #8547, #23151, #24449, .T. ) ;
#32559=DIRECTION ( 'NONE',  ( 0.9999697198139515519, 0.000000000000000000, 0.007781995580013368816 ) ) ;
#32560=CARTESIAN_POINT ( 'NONE',  ( -14.87661172084004946, 0.000000000000000000, 5.273972019284645540 ) ) ;
#32562=PLANE ( 'NONE',  #48295 ) ;
#32563=ORIENTED_EDGE ( 'NONE', *, *, #19834, .T. ) ;
#32564=DIRECTION ( 'NONE',  ( 0.6427681459581294776, -0.7660444431189769032, 0.005002170337467562802 ) ) ;
#32565=DIRECTION ( 'NONE',  ( 0.9999697198139515519, 0.000000000000000000, 0.007781995580013368816 ) ) ;
#32567=EDGE_CURVE ( 'NONE', #16295, #22163, #24194, .T. ) ;
#32568=DIRECTION ( 'NONE',  ( -0.5449076811759708816, 0.6444004775717707689, 0.5364919789714475140 ) ) ;
#32569=CARTESIAN_POINT ( 'NONE',  ( -13.63251841181027402, 3.848249166794011522, 1.854485548694981611 ) ) ;
#32570=ORIENTED_EDGE ( 'NONE', *, *, #529, .F. ) ;
#32571=LINE ( 'NONE', #24046, #30293 ) ;
#32572=DIRECTION ( 'NONE',  ( 0.5364919789714477361, 0.6444004775717706579, 0.5449076811759711036 ) ) ;
#32573=PLANE ( 'NONE',  #49058 ) ;
#32575=CARTESIAN_POINT ( 'NONE',  ( -20.46460680255002984, 1.419719901456506728, 7.160471608229209473 ) ) ;
#32576=DIRECTION ( 'NONE',  ( 0.005961354470445682716, -0.6427876096865404731, -0.7660212471507180654 ) ) ;
#32577=LINE ( 'NONE', #53339, #35586 ) ;
#32578=CARTESIAN_POINT ( 'NONE',  ( -10.68757514314370916, 0.000000000000000000, 4.367901874718414845 ) ) ;
#32579=CARTESIAN_POINT ( 'NONE',  ( -3.789853545709553462, 5.589773622088367588, -1.746265754542047910 ) ) ;
#32580=EDGE_CURVE ( 'NONE', #30608, #47582, #15638, .T. ) ;
#32582=EDGE_CURVE ( 'NONE', #35922, #49529, #11404, .T. ) ;
#32583=ORIENTED_EDGE ( 'NONE', *, *, #16667, .F. ) ;
#32584=EDGE_CURVE ( 'NONE', #34233, #46872, #21325, .T. ) ;
#32585=VERTEX_POINT ( 'NONE', #56235 ) ;
#32586=ORIENTED_EDGE ( 'NONE', *, *, #32956, .T. ) ;
#32587=VERTEX_POINT ( 'NONE', #17323 ) ;
#32588=EDGE_LOOP ( 'NONE', ( #47954, #5361, #48037, #28534 ) ) ;
#32589=CARTESIAN_POINT ( 'NONE',  ( -19.63656972920071198, -0.1191753592594160388, 6.983586246353969962 ) ) ;
#32590=DIRECTION ( 'NONE',  ( 0.007781995580012662783, 0.000000000000000000, -0.9999697198139514409 ) ) ;
#32591=ORIENTED_EDGE ( 'NONE', *, *, #213, .T. ) ;
#32592=VERTEX_POINT ( 'NONE', #34958 ) ;
#32593=ORIENTED_EDGE ( 'NONE', *, *, #46105, .T. ) ;
#32594=ORIENTED_EDGE ( 'NONE', *, *, #52966, .T. ) ;
#32595=ADVANCED_FACE ( 'NONE', ( #277 ), #4302, .F. ) ;
#32597=LINE ( 'NONE', #40836, #53671 ) ;
#32598=LINE ( 'NONE', #28325, #53154 ) ;
#32599=EDGE_LOOP ( 'NONE', ( #46597, #29051, #43299, #55483 ) ) ;
#32600=FACE_OUTER_BOUND ( 'NONE', #28, .T. ) ;
#32601=LINE ( 'NONE', #50751, #22815 ) ;
#32603=DIRECTION ( 'NONE',  ( -0.5449076811759708816, 0.6444004775717707689, 0.5364919789714475140 ) ) ;
#32604=DIRECTION ( 'NONE',  ( 0.9999697198139515519, 0.000000000000000000, 0.007781995580013368816 ) ) ;
#32605=DIRECTION ( 'NONE',  ( -0.5449076811759708816, 0.6444004775717707689, 0.5364919789714475140 ) ) ;
#32606=CARTESIAN_POINT ( 'NONE',  ( -19.98893524048127190, 0.000000000000000000, 5.403512749131516024 ) ) ;
#32607=CARTESIAN_POINT ( 'NONE',  ( -13.95440368855772562, 0.000000000000000000, 6.189139008631170391 ) ) ;
#32608=DIRECTION ( 'NONE',  ( 0.000000000000000000, -1.000000000000000000, 0.000000000000000000 ) ) ;
#32609=ORIENTED_EDGE ( 'NONE', *, *, #49879, .F. ) ;
#32610=PLANE ( 'NONE',  #36519 ) ;
#32611=ORIENTED_EDGE ( 'NONE', *, *, #47186, .T. ) ;
#32612=LINE ( 'NONE', #28342, #54623 ) ;
#32613=DIRECTION ( 'NONE',  ( -0.6427681459581293666, -0.7660444431189770143, -0.005002170337467561935 ) ) ;
#32614=DIRECTION ( 'NONE',  ( -0.005961354470445682716, -0.6427876096865404731, 0.7660212471507180654 ) ) ;
#32615=LINE ( 'NONE', #19004, #24110 ) ;
#32616=EDGE_CURVE ( 'NONE', #46922, #41711, #34116, .T. ) ;
#32617=CARTESIAN_POINT ( 'NONE',  ( -10.47421230394850866, 0.000000000000000000, 10.95934586908605723 ) ) ;
#32618=LINE ( 'NONE', #33198, #51278 ) ;
#32619=DIRECTION ( 'NONE',  ( 0.9999697198139515519, 0.000000000000000000, 0.007781995580013368816 ) ) ;
#32622=CARTESIAN_POINT ( 'NONE',  ( -11.67244013076689946, 0.000000000000000000, 11.50401908778467863 ) ) ;
#32623=CARTESIAN_POINT ( 'NONE',  ( -11.37100670409528114, 0.000000000000000000, 6.778581727343776286 ) ) ;
#32624=FACE_OUTER_BOUND ( 'NONE', #22566, .T. ) ;
#32625=CARTESIAN_POINT ( 'NONE',  ( 2.072287782118878319, 0.000000000000000000, -2.950529333540147015 ) ) ;
#32626=EDGE_CURVE ( 'NONE', #19674, #49645, #29851, .T. ) ;
#32627=CARTESIAN_POINT ( 'NONE',  ( -26.13337879274045505, 0.000000000000000000, 6.833023547870798353 ) ) ;
#32629=EDGE_CURVE ( 'NONE', #24940, #33221, #39495, .T. ) ;
#32630=DIRECTION ( 'NONE',  ( 0.000000000000000000, -0.000000000000000000, -1.000000000000000000 ) ) ;
#32631=EDGE_CURVE ( 'NONE', #36809, #52840, #21616, .T. ) ;
#32632=LINE ( 'NONE', #10216, #20154 ) ;
#32633=ORIENTED_EDGE ( 'NONE', *, *, #26490, .T. ) ;
#32634=PLANE ( 'NONE',  #3106 ) ;
#32635=ORIENTED_EDGE ( 'NONE', *, *, #10810, .F. ) ;
#32637=LINE ( 'NONE', #11044, #25979 ) ;
#32638=DIRECTION ( 'NONE',  ( -0.7660212471507179544, -0.6427876096865405842, -0.005961354470445141482 ) ) ;
#32639=EDGE_CURVE ( 'NONE', #29014, #53080, #51129, .T. ) ;
#32641=EDGE_CURVE ( 'NONE', #29959, #14373, #21869, .T. ) ;
#32642=DIRECTION ( 'NONE',  ( -0.005961354470445682716, -0.6427876096865404731, 0.7660212471507180654 ) ) ;
#32643=ORIENTED_EDGE ( 'NONE', *, *, #40716, .F. ) ;
#32644=DIRECTION ( 'NONE',  ( 0.5449076811759707706, 0.6444004775717708799, -0.5364919789714476250 ) ) ;
#32645=EDGE_CURVE ( 'NONE', #53603, #33755, #8848, .T. ) ;
#32646=AXIS2_PLACEMENT_3D ( 'NONE', #43646, #5057, #34572 ) ;
#32647=ORIENTED_EDGE ( 'NONE', *, *, #21905, .F. ) ;
#32648=ORIENTED_EDGE ( 'NONE', *, *, #17398, .T. ) ;
#32649=ORIENTED_EDGE ( 'NONE', *, *, #1491, .T. ) ;
#32650=PLANE ( 'NONE',  #20259 ) ;
#32651=PLANE ( 'NONE',  #21421 ) ;
#32652=DIRECTION ( 'NONE',  ( 0.7660212471507180654, -0.6427876096865404731, 0.005961354470445141482 ) ) ;
#32653=ADVANCED_FACE ( 'NONE', ( #51969 ), #7996, .F. ) ;
#32654=ORIENTED_EDGE ( 'NONE', *, *, #41373, .F. ) ;
#32655=VERTEX_POINT ( 'NONE', #17071 ) ;
#32656=ADVANCED_FACE ( 'NONE', ( #12535 ), #42610, .F. ) ;
#32657=DIRECTION ( 'NONE',  ( 0.9999697198139515519, 0.000000000000000000, 0.007781995580013368816 ) ) ;
#32658=ORIENTED_EDGE ( 'NONE', *, *, #54975, .T. ) ;
#32659=DIRECTION ( 'NONE',  ( -0.5364919789714478471, 0.6444004775717705469, -0.5449076811759709926 ) ) ;
#32660=ORIENTED_EDGE ( 'NONE', *, *, #13384, .F. ) ;
#32661=DIRECTION ( 'NONE',  ( 0.000000000000000000, -1.000000000000000000, 0.000000000000000000 ) ) ;
#32662=CARTESIAN_POINT ( 'NONE',  ( -10.88469503360121848, 0.000000000000000000, 3.997035772344645910 ) ) ;
#32663=ORIENTED_EDGE ( 'NONE', *, *, #53792, .F. ) ;
#32664=CARTESIAN_POINT ( 'NONE',  ( -15.88130887279446490, 0.000000000000000000, 3.050160814894388839 ) ) ;
#32665=CARTESIAN_POINT ( 'NONE',  ( -19.60834386242827776, 0.000000000000000000, 4.298478389818581213 ) ) ;
#32666=VERTEX_POINT ( 'NONE', #26151 ) ;
#32667=CARTESIAN_POINT ( 'NONE',  ( -10.22006419279734146, 0.000000000000000000, 4.002208083228659063 ) ) ;
#32668=CARTESIAN_POINT ( 'NONE',  ( -15.10628516568717572, 0.000000000000000000, 9.086167745620324254 ) ) ;
#32669=LINE ( 'NONE', #2570, #8385 ) ;
#32670=ORIENTED_EDGE ( 'NONE', *, *, #36293, .T. ) ;
#32671=DIRECTION ( 'NONE',  ( 0.000000000000000000, -0.000000000000000000, -1.000000000000000000 ) ) ;
#32672=CARTESIAN_POINT ( 'NONE',  ( -18.67619601524082285, 0.000000000000000000, 3.936400510096834893 ) ) ;
#32673=CARTESIAN_POINT ( 'NONE',  ( -14.88367748223989118, 0.000000000000000000, 6.181907185095151469 ) ) ;
#32674=EDGE_CURVE ( 'NONE', #55170, #8704, #3703, .T. ) ;
#32675=DIRECTION ( 'NONE',  ( -0.5449076811759708816, 0.6444004775717707689, 0.5364919789714475140 ) ) ;
#32676=LINE ( 'NONE', #25018, #44866 ) ;
#32677=CARTESIAN_POINT ( 'NONE',  ( -27.06708303904391144, 0.000000000000000000, 7.395095371555332697 ) ) ;
#32678=AXIS2_PLACEMENT_3D ( 'NONE', #17913, #48252, #56232 ) ;
#32680=ORIENTED_EDGE ( 'NONE', *, *, #2651, .F. ) ;
#32681=FACE_OUTER_BOUND ( 'NONE', #32869, .T. ) ;
#32682=DIRECTION ( 'NONE',  ( -0.5449076811759708816, 0.6444004775717707689, 0.5364919789714475140 ) ) ;
#32684=VERTEX_POINT ( 'NONE', #34387 ) ;
#32685=LINE ( 'NONE', #11677, #25661 ) ;
#32686=CARTESIAN_POINT ( 'NONE',  ( -17.74560456716937296, 0.000000000000000000, 3.774316574337878372 ) ) ;
#32687=ADVANCED_FACE ( 'NONE', ( #47147 ), #21023, .F. ) ;
#32688=LINE ( 'NONE', #14824, #3184 ) ;
#32689=CARTESIAN_POINT ( 'NONE',  ( -18.19747506107908563, 0.000000000000000000, 14.03856424583689311 ) ) ;
#32690=EDGE_CURVE ( 'NONE', #34394, #25528, #26405, .T. ) ;
#32691=LINE ( 'NONE', #7151, #13877 ) ;
#32692=ORIENTED_EDGE ( 'NONE', *, *, #35463, .F. ) ;
#32693=VERTEX_POINT ( 'NONE', #12796 ) ;
#32695=CARTESIAN_POINT ( 'NONE',  ( -25.20123094555300369, 0.000000000000000000, 6.470945668149052032 ) ) ;
#32696=EDGE_LOOP ( 'NONE', ( #3162, #49414, #40553, #40372 ) ) ;
#32697=ADVANCED_FACE ( 'NONE', ( #25873 ), #25567, .F. ) ;
#32698=CARTESIAN_POINT ( 'NONE',  ( -12.60458797795435615, 0.000000000000000000, 11.86609696750642229 ) ) ;
#32699=ORIENTED_EDGE ( 'NONE', *, *, #18647, .T. ) ;
#32700=DIRECTION ( 'NONE',  ( -0.005002170337468016433, -0.7660444431189770143, 0.6427681459581293666 ) ) ;
#32701=EDGE_CURVE ( 'NONE', #20126, #52593, #38929, .T. ) ;
#32702=EDGE_LOOP ( 'NONE', ( #35076, #5775, #4306, #4423 ) ) ;
#32703=EDGE_LOOP ( 'NONE', ( #32417, #17421, #30949, #45176 ) ) ;
#32704=DIRECTION ( 'NONE',  ( 0.005961354470445682716, -0.6427876096865404731, -0.7660212471507180654 ) ) ;
#32705=LINE ( 'NONE', #18844, #10564 ) ;
#32707=VERTEX_POINT ( 'NONE', #18762 ) ;
#32708=ADVANCED_FACE ( 'NONE', ( #36338 ), #1117, .F. ) ;
#32709=VECTOR ( 'NONE', #48300, 1000.000000000000000 ) ;
#32710=CARTESIAN_POINT ( 'NONE',  ( -15.90832530584190785, -5.051250379848162275, 11.15122795565880587 ) ) ;
#32712=VECTOR ( 'NONE', #13625, 1000.000000000000227 ) ;
#32713=ORIENTED_EDGE ( 'NONE', *, *, #25648, .F. ) ;
#32714=ADVANCED_FACE ( 'NONE', ( #5409 ), #22716, .F. ) ;
#32715=ORIENTED_EDGE ( 'NONE', *, *, #23636, .F. ) ;
#32718=CARTESIAN_POINT ( 'NONE',  ( -19.52872879626147196, 0.000000000000000000, 5.976432308120079639 ) ) ;
#32719=ORIENTED_EDGE ( 'NONE', *, *, #15443, .T. ) ;
#32720=CARTESIAN_POINT ( 'NONE',  ( -30.79567442779373110, 0.000000000000000000, 8.843406890442315316 ) ) ;
#32721=PLANE ( 'NONE',  #53975 ) ;
#32722=ORIENTED_EDGE ( 'NONE', *, *, #6377, .T. ) ;
#32723=PLANE ( 'NONE',  #7788 ) ;
#32724=VERTEX_POINT ( 'NONE', #48566 ) ;
#32725=CARTESIAN_POINT ( 'NONE',  ( -14.10280672071693431, -0.1191753592594197858, 12.40843558753103792 ) ) ;
#32727=DIRECTION ( 'NONE',  ( 0.9999697198139515519, 0.000000000000000000, 0.007781995580013368816 ) ) ;
#32728=DIRECTION ( 'NONE',  ( -0.005961354470445682716, -0.6427876096865404731, 0.7660212471507180654 ) ) ;
#32729=PLANE ( 'NONE',  #6947 ) ;
#32730=CARTESIAN_POINT ( 'NONE',  ( -20.94784447234964730, -4.403642575758159872, 12.04591360691983581 ) ) ;
#32731=DIRECTION ( 'NONE',  ( -0.6427681459581293666, -0.7660444431189770143, -0.005002170337467561935 ) ) ;
#32734=VECTOR ( 'NONE', #44561, 999.9999999999998863 ) ;
#32735=ORIENTED_EDGE ( 'NONE', *, *, #13620, .T. ) ;
#32737=PLANE ( 'NONE',  #38252 ) ;
#32738=DIRECTION ( 'NONE',  ( -0.6427681459581293666, -0.7660444431189770143, -0.005002170337467561935 ) ) ;
#32739=ADVANCED_FACE ( 'NONE', ( #18452 ), #44306, .F. ) ;
#32740=CARTESIAN_POINT ( 'NONE',  ( -29.86352658060627618, 0.000000000000000000, 8.481329010720569883 ) ) ;
#32741=CARTESIAN_POINT ( 'NONE',  ( -30.79489622823572859, -0.1191753592594197858, 8.743409918460921304 ) ) ;
#32742=DIRECTION ( 'NONE',  ( -0.8531650599175529814, -0.4028455766673920135, 0.3313982828793697877 ) ) ;
#32743=ORIENTED_EDGE ( 'NONE', *, *, #730, .T. ) ;
#32744=ADVANCED_FACE ( 'NONE', ( #26997 ), #27253, .F. ) ;
#32745=FACE_OUTER_BOUND ( 'NONE', #49040, .T. ) ;
#32746=DIRECTION ( 'NONE',  ( 0.000000000000000000, -0.000000000000000000, -1.000000000000000000 ) ) ;
#32747=VERTEX_POINT ( 'NONE', #53390 ) ;
#32748=CARTESIAN_POINT ( 'NONE',  ( -24.26908309836554878, 0.000000000000000000, 6.108867788427308376 ) ) ;
#32749=CARTESIAN_POINT ( 'NONE',  ( -9.440078302826643508, -0.04820958850348456420, 2.690502017889039976 ) ) ;
#32750=ORIENTED_EDGE ( 'NONE', *, *, #36436, .T. ) ;
#32752=EDGE_CURVE ( 'NONE', #37228, #3166, #35242, .T. ) ;
#32753=ADVANCED_FACE ( 'NONE', ( #52538 ), #30946, .F. ) ;
#32754=DIRECTION ( 'NONE',  ( 0.5449076811759707706, 0.6444004775717708799, -0.5364919789714476250 ) ) ;
#32755=CARTESIAN_POINT ( 'NONE',  ( -12.15116108492864377, 0.000000000000000000, 1.401855352044617975 ) ) ;
#32756=VECTOR ( 'NONE', #30920, 1000.000000000000227 ) ;
#32757=DIRECTION ( 'NONE',  ( 0.9999697198139515519, 0.000000000000000000, 0.007781995580013368816 ) ) ;
#32758=DIRECTION ( 'NONE',  ( 0.005002170337468016433, -0.7660444431189770143, -0.6427681459581293666 ) ) ;
#32759=VECTOR ( 'NONE', #37197, 999.9999999999998863 ) ;
#32760=CARTESIAN_POINT ( 'NONE',  ( -12.60458797795435615, 0.000000000000000000, 11.86609696750642229 ) ) ;
#32761=EDGE_LOOP ( 'NONE', ( #15884, #42907, #51159, #46705 ) ) ;
#32762=ORIENTED_EDGE ( 'NONE', *, *, #8841, .F. ) ;
#32763=DIRECTION ( 'NONE',  ( 0.5364919789714477361, 0.6444004775717706579, 0.5449076811759711036 ) ) ;
#32764=PLANE ( 'NONE',  #14098 ) ;
#32765=CARTESIAN_POINT ( 'NONE',  ( -24.26908309836554878, 0.000000000000000000, 6.108867788427308376 ) ) ;
#32766=FACE_OUTER_BOUND ( 'NONE', #19765, .T. ) ;
#32767=PLANE ( 'NONE',  #31035 ) ;
#32768=EDGE_CURVE ( 'NONE', #32655, #29728, #1693, .T. ) ;
#32769=CARTESIAN_POINT ( 'NONE',  ( -19.12962290826653700, 0.000000000000000000, 14.40064212555863854 ) ) ;
#32770=ORIENTED_EDGE ( 'NONE', *, *, #17158, .F. ) ;
#32771=DIRECTION ( 'NONE',  ( 0.5364919789714477361, 0.6444004775717706579, 0.5449076811759711036 ) ) ;
#32772=EDGE_CURVE ( 'NONE', #4025, #20238, #32086, .T. ) ;
#32773=CARTESIAN_POINT ( 'NONE',  ( -15.60102546347950536, 0.000000000000000000, 12.95077420755565356 ) ) ;
#32774=CARTESIAN_POINT ( 'NONE',  ( -16.55824503503297151, 0.1245042932765017124, 3.109744084659005203 ) ) ;
#32775=ORIENTED_EDGE ( 'NONE', *, *, #43951, .F. ) ;
#32776=EDGE_CURVE ( 'NONE', #25320, #12550, #44563, .T. ) ;
#32778=CARTESIAN_POINT ( 'NONE',  ( -15.35561888520754614, 0.000000000000000000, 7.116904623805458741 ) ) ;
#32779=LINE ( 'NONE', #16043, #11214 ) ;
#32780=VERTEX_POINT ( 'NONE', #48259 ) ;
#32781=AXIS2_PLACEMENT_3D ( 'NONE', #39902, #982, #23157 ) ;
#32782=ADVANCED_FACE ( 'NONE', ( #40321 ), #1418, .F. ) ;
#32783=VECTOR ( 'NONE', #53617, 999.9999999999998863 ) ;
#32784=CARTESIAN_POINT ( 'NONE',  ( -10.88912548622250220, 0.000000000000000000, 4.566339419565200508 ) ) ;
#32785=ORIENTED_EDGE ( 'NONE', *, *, #55382, .T. ) ;
#32786=EDGE_CURVE ( 'NONE', #47757, #5305, #40874, .T. ) ;
#32787=ORIENTED_EDGE ( 'NONE', *, *, #26261, .F. ) ;
#32788=ORIENTED_EDGE ( 'NONE', *, *, #41079, .F. ) ;
#32789=ORIENTED_EDGE ( 'NONE', *, *, #39150, .T. ) ;
#32790=VECTOR ( 'NONE', #7760, 999.9999999999998863 ) ;
#32791=ORIENTED_EDGE ( 'NONE', *, *, #4003, .T. ) ;
#32792=LINE ( 'NONE', #33087, #26601 ) ;
#32793=ORIENTED_EDGE ( 'NONE', *, *, #44117, .T. ) ;
#32794=ORIENTED_EDGE ( 'NONE', *, *, #35122, .T. ) ;
#32796=VERTEX_POINT ( 'NONE', #36086 ) ;
#32797=ORIENTED_EDGE ( 'NONE', *, *, #46969, .F. ) ;
#32798=VECTOR ( 'NONE', #6219, 999.9999999999998863 ) ;
#32799=ORIENTED_EDGE ( 'NONE', *, *, #5427, .T. ) ;
#32801=DIRECTION ( 'NONE',  ( -0.005961354470445682716, -0.6427876096865404731, 0.7660212471507180654 ) ) ;
#32803=DIRECTION ( 'NONE',  ( 0.005961354470445682716, -0.6427876096865404731, -0.7660212471507180654 ) ) ;
#32804=DIRECTION ( 'NONE',  ( -0.5449076811759708816, 0.6444004775717707689, 0.5364919789714475140 ) ) ;
#32805=ORIENTED_EDGE ( 'NONE', *, *, #41556, .T. ) ;
#32806=EDGE_LOOP ( 'NONE', ( #50171, #45751, #43008, #25148 ) ) ;
#32807=CARTESIAN_POINT ( 'NONE',  ( -19.22961988024793101, -0.1191753592594177458, 14.39986392600063603 ) ) ;
#32808=DIRECTION ( 'NONE',  ( 0.005961354470445682716, -0.6427876096865404731, -0.7660212471507180654 ) ) ;
#32810=ADVANCED_FACE ( 'NONE', ( #26695 ), #5142, .F. ) ;
#32811=CARTESIAN_POINT ( 'NONE',  ( -16.28908438678428183, 0.000000000000000000, 7.648298262822180504 ) ) ;
#32813=PLANE ( 'NONE',  #21329 ) ;
#32814=CARTESIAN_POINT ( 'NONE',  ( -19.59569683186026268, 0.000000000000000000, 14.58168106541950948 ) ) ;
#32815=EDGE_LOOP ( 'NONE', ( #42125, #35682, #16139, #39983 ) ) ;
#32816=LINE ( 'NONE', #54396, #21105 ) ;
#32817=EDGE_LOOP ( 'NONE', ( #46075, #16051, #53682, #28888 ) ) ;
#32818=EDGE_CURVE ( 'NONE', #55170, #48632, #11333, .T. ) ;
#32819=EDGE_CURVE ( 'NONE', #21126, #7904, #41696, .T. ) ;
#32820=VECTOR ( 'NONE', #48653, 1000.000000000000000 ) ;
#32821=VECTOR ( 'NONE', #14804, 1000.000000000000227 ) ;
#32822=LINE ( 'NONE', #36531, #50087 ) ;
#32823=LINE ( 'NONE', #24574, #4230 ) ;
#32824=DIRECTION ( 'NONE',  ( 0.9999697198139515519, 0.000000000000000000, 0.007781995580013368816 ) ) ;
#32825=FACE_OUTER_BOUND ( 'NONE', #22052, .T. ) ;
#32826=EDGE_CURVE ( 'NONE', #9089, #19669, #2783, .T. ) ;
#32827=PLANE ( 'NONE',  #36830 ) ;
#32829=AXIS2_PLACEMENT_3D ( 'NONE', #638, #17961, #13961 ) ;
#32830=ORIENTED_EDGE ( 'NONE', *, *, #26362, .T. ) ;
#32831=LINE ( 'NONE', #50147, #40258 ) ;
#32832=DIRECTION ( 'NONE',  ( 0.005002170337468016433, -0.7660444431189770143, -0.6427681459581293666 ) ) ;
#32833=DIRECTION ( 'NONE',  ( -0.005002170337468016433, -0.7660444431189770143, 0.6427681459581293666 ) ) ;
#32834=CARTESIAN_POINT ( 'NONE',  ( -19.56442468080716068, -2.784623065533158304, 8.851459539246230079 ) ) ;
#32835=AXIS2_PLACEMENT_3D ( 'NONE', #5635, #14454, #43684 ) ;
#32836=FACE_OUTER_BOUND ( 'NONE', #12211, .T. ) ;
#32837=FACE_OUTER_BOUND ( 'NONE', #6345, .T. ) ;
#32838=DIRECTION ( 'NONE',  ( -0.6427681459581293666, -0.7660444431189770143, -0.005002170337467561935 ) ) ;
#32839=ADVANCED_FACE ( 'NONE', ( #46512 ), #42283, .T. ) ;
#32840=DIRECTION ( 'NONE',  ( 0.7660212471507180654, -0.6427876096865404731, 0.005961354470445141482 ) ) ;
#32841=LINE ( 'NONE', #54415, #22908 ) ;
#32842=ORIENTED_EDGE ( 'NONE', *, *, #3228, .F. ) ;
#32843=ORIENTED_EDGE ( 'NONE', *, *, #29741, .F. ) ;
#32844=EDGE_CURVE ( 'NONE', #33164, #40367, #7630, .T. ) ;
#32845=VECTOR ( 'NONE', #27057, 1000.000000000000227 ) ;
#32846=ADVANCED_FACE ( 'NONE', ( #15053 ), #24655, .F. ) ;
#32847=ORIENTED_EDGE ( 'NONE', *, *, #41715, .F. ) ;
#32848=ORIENTED_EDGE ( 'NONE', *, *, #47892, .T. ) ;
#32849=ORIENTED_EDGE ( 'NONE', *, *, #31546, .T. ) ;
#32850=ADVANCED_FACE ( 'NONE', ( #2245 ), #15868, .F. ) ;
#32851=ORIENTED_EDGE ( 'NONE', *, *, #6358, .F. ) ;
#32852=AXIS2_PLACEMENT_3D ( 'NONE', #13479, #30795, #48094 ) ;
#32853=CARTESIAN_POINT ( 'NONE',  ( 2.072287782118878319, 0.000000000000000000, -2.950529333540147015 ) ) ;
#32854=CARTESIAN_POINT ( 'NONE',  ( -10.43311074989726173, 0.000000000000000000, 5.677884441106503033 ) ) ;
#32855=ADVANCED_FACE ( 'NONE', ( #55070 ), #41975, .F. ) ;
#32856=CARTESIAN_POINT ( 'NONE',  ( -16.96101973371472837, 0.000000000000000000, 8.581739302416485415 ) ) ;
#32857=AXIS2_PLACEMENT_3D ( 'NONE', #12736, #16713, #21250 ) ;
#32858=VECTOR ( 'NONE', #55956, 999.9999999999998863 ) ;
#32859=ORIENTED_EDGE ( 'NONE', *, *, #32690, .T. ) ;
#32860=CARTESIAN_POINT ( 'NONE',  ( -19.86019089980205266, 1.257817950434005461, 6.659987261600974762 ) ) ;
#32861=EDGE_CURVE ( 'NONE', #49508, #42567, #37171, .T. ) ;
#32862=VERTEX_POINT ( 'NONE', #33479 ) ;
#32863=EDGE_LOOP ( 'NONE', ( #32184, #18971, #12745, #20755 ) ) ;
#32864=VECTOR ( 'NONE', #37116, 999.9999999999998863 ) ;
#32865=AXIS2_PLACEMENT_3D ( 'NONE', #35707, #30626, #9026 ) ;
#32868=PLANE ( 'NONE',  #10561 ) ;
#32869=EDGE_LOOP ( 'NONE', ( #38412, #41484, #10692, #20114 ) ) ;
#32870=LINE ( 'NONE', #11005, #28298 ) ;
#32871=ORIENTED_EDGE ( 'NONE', *, *, #19102, .T. ) ;
#32872=CARTESIAN_POINT ( 'NONE',  ( -13.22512383883834097, 0.000000000000000000, 6.194814433051186064 ) ) ;
#32873=VECTOR ( 'NONE', #8369, 999.9999999999998863 ) ;
#32874=CARTESIAN_POINT ( 'NONE',  ( -17.74560456716937296, 0.000000000000000000, 3.774316574337878372 ) ) ;
#32875=CARTESIAN_POINT ( 'NONE',  ( -23.33771345073609638, -0.1191753592594197858, 5.846786880686956955 ) ) ;
#32876=DIRECTION ( 'NONE',  ( 0.007781995580012663651, 0.000000000000000000, -0.9999697198139515519 ) ) ;
#32878=DIRECTION ( 'NONE',  ( -0.9999697198139514409, -0.000000000000000000, -0.007781995580013368816 ) ) ;
#32879=CARTESIAN_POINT ( 'NONE',  ( -21.70540433349056642, -3.108426967578157729, 10.21450611222444316 ) ) ;
#32880=DIRECTION ( 'NONE',  ( -0.005002170337468016433, -0.7660444431189770143, 0.6427681459581293666 ) ) ;
#32881=LINE ( 'NONE', #2216, #256 ) ;
#32882=VERTEX_POINT ( 'NONE', #54471 ) ;
#32884=EDGE_LOOP ( 'NONE', ( #14242, #27095, #42772, #5625 ) ) ;
#32885=ADVANCED_FACE ( 'NONE', ( #45986 ), #50525, .F. ) ;
#32886=DIRECTION ( 'NONE',  ( 0.007781995580012662783, 0.000000000000000000, -0.9999697198139514409 ) ) ;
#32887=CARTESIAN_POINT ( 'NONE',  ( -17.42344502812375140, -2.460819163488158878, 7.488412966268020554 ) ) ;
#32888=PLANE ( 'NONE',  #27777 ) ;
#32889=AXIS2_PLACEMENT_3D ( 'NONE', #21871, #13382, #34648 ) ;
#32890=CARTESIAN_POINT ( 'NONE',  ( -20.55929158756503128, 0.4483081953215033444, 4.653555402000536745 ) ) ;
#32891=FACE_OUTER_BOUND ( 'NONE', #40284, .T. ) ;
#32892=ADVANCED_FACE ( 'NONE', ( #11875 ), #36624, .F. ) ;
#32893=ADVANCED_FACE ( 'NONE', ( #37440 ), #28941, .F. ) ;
#32894=LINE ( 'NONE', #7330, #34778 ) ;
#32895=ORIENTED_EDGE ( 'NONE', *, *, #42407, .F. ) ;
#32896=CARTESIAN_POINT ( 'NONE',  ( -10.62894072970072301, -10.24364977037474667, 0.9102679640985203990 ) ) ;
#32897=AXIS2_PLACEMENT_3D ( 'NONE', #49415, #19029, #18776 ) ;
#32899=DIRECTION ( 'NONE',  ( -0.005961354470445682716, -0.6427876096865404731, 0.7660212471507180654 ) ) ;
#32901=CARTESIAN_POINT ( 'NONE',  ( -17.69736534483395118, 0.000000000000000000, 9.483999043806973006 ) ) ;
#32902=AXIS2_PLACEMENT_3D ( 'NONE', #26450, #35283, #52579 ) ;
#32903=AXIS2_PLACEMENT_3D ( 'NONE', #1621, #53844, #49314 ) ;
#32904=LINE ( 'NONE', #37168, #43642 ) ;
#32905=PLANE ( 'NONE',  #31176 ) ;
#32906=DIRECTION ( 'NONE',  ( 0.7660212471507180654, -0.6427876096865404731, 0.005961354470445141482 ) ) ;
#32907=CARTESIAN_POINT ( 'NONE',  ( -10.29499555079022066, -0.1191753592594194527, 0.7805523157836706805 ) ) ;
#32908=EDGE_CURVE ( 'NONE', #17489, #17469, #7340, .T. ) ;
#32909=ORIENTED_EDGE ( 'NONE', *, *, #13463, .T. ) ;
#32910=AXIS2_PLACEMENT_3D ( 'NONE', #41322, #20838, #55472 ) ;
#32912=VECTOR ( 'NONE', #47428, 1000.000000000000114 ) ;
#32913=ORIENTED_EDGE ( 'NONE', *, *, #50231, .T. ) ;
#32914=CARTESIAN_POINT ( 'NONE',  ( -19.45503627000849889, 0.000000000000000000, 7.556996783084074742 ) ) ;
#32915=LINE ( 'NONE', #1199, #46423 ) ;
#32916=ORIENTED_EDGE ( 'NONE', *, *, #2237, .T. ) ;
#32917=VECTOR ( 'NONE', #25227, 1000.000000000000227 ) ;
#32918=ORIENTED_EDGE ( 'NONE', *, *, #831, .T. ) ;
#32919=LINE ( 'NONE', #8993, #5704 ) ;
#32920=VECTOR ( 'NONE', #52989, 1000.000000000000114 ) ;
#32921=EDGE_CURVE ( 'NONE', #1131, #54123, #45401, .T. ) ;
#32922=ORIENTED_EDGE ( 'NONE', *, *, #12913, .F. ) ;
#32923=ORIENTED_EDGE ( 'NONE', *, *, #28331, .T. ) ;
#32924=EDGE_LOOP ( 'NONE', ( #3720, #29092, #2849, #29752 ) ) ;
#32925=DIRECTION ( 'NONE',  ( 0.6427681459581294776, -0.7660444431189769032, 0.005002170337467562802 ) ) ;
#32928=DIRECTION ( 'NONE',  ( 0.7660212471507180654, -0.6427876096865404731, 0.005961354470445141482 ) ) ;
#32929=CIRCLE ( 'NONE', #12091, 1.000000000000000444 ) ;
#32930=ORIENTED_EDGE ( 'NONE', *, *, #53313, .T. ) ;
#32931=ADVANCED_FACE ( 'NONE', ( #41153 ), #19584, .F. ) ;
#32932=ORIENTED_EDGE ( 'NONE', *, *, #13222, .T. ) ;
#32933=AXIS2_PLACEMENT_3D ( 'NONE', #48005, #47441, #9105 ) ;
#32934=DIRECTION ( 'NONE',  ( 0.000000000000000000, -0.000000000000000000, -1.000000000000000000 ) ) ;
#32935=CARTESIAN_POINT ( 'NONE',  ( -19.32961685222932147, 0.000000000000000000, 14.39908572644263351 ) ) ;
#32937=VECTOR ( 'NONE', #16579, 999.9999999999998863 ) ;
#32938=LINE ( 'NONE', #50253, #30970 ) ;
#32939=VERTEX_POINT ( 'NONE', #209 ) ;
#32941=DIRECTION ( 'NONE',  ( -0.005002170337468016433, -0.7660444431189770143, 0.6427681459581293666 ) ) ;
#32942=ADVANCED_FACE ( 'NONE', ( #29505 ), #55909, .F. ) ;
#32943=AXIS2_PLACEMENT_3D ( 'NONE', #6922, #28192, #24236 ) ;
#32944=VECTOR ( 'NONE', #52105, 999.9999999999998863 ) ;
#32945=ORIENTED_EDGE ( 'NONE', *, *, #42906, .F. ) ;
#32946=CARTESIAN_POINT ( 'NONE',  ( -20.44552454186363022, -3.270328918600659218, 9.990834699409186115 ) ) ;
#32947=EDGE_CURVE ( 'NONE', #47757, #21366, #34328, .T. ) ;
#32948=ADVANCED_FACE ( 'NONE', ( #42820 ), #34045, .F. ) ;
#32949=VECTOR ( 'NONE', #30135, 999.9999999999998863 ) ;
#32950=CARTESIAN_POINT ( 'NONE',  ( -18.14056621274878012, 0.000000000000000000, 6.725899449939636732 ) ) ;
#32951=VECTOR ( 'NONE', #5902, 1000.000000000000227 ) ;
#32952=ORIENTED_EDGE ( 'NONE', *, *, #30329, .F. ) ;
#32953=FACE_OUTER_BOUND ( 'NONE', #4062, .T. ) ;
#32954=CARTESIAN_POINT ( 'NONE',  ( -16.37548929079726534, -0.1191753592594192307, 5.900968518956748454 ) ) ;
#32955=LINE ( 'NONE', #15355, #28316 ) ;
#32956=EDGE_CURVE ( 'NONE', #9006, #14383, #55605, .T. ) ;
#32957=ORIENTED_EDGE ( 'NONE', *, *, #35407, .T. ) ;
#32958=ADVANCED_FACE ( 'NONE', ( #56179 ), #47362, .F. ) ;
#32959=DIRECTION ( 'NONE',  ( -0.005961354470445682716, -0.6427876096865404731, 0.7660212471507180654 ) ) ;
#32960=DIRECTION ( 'NONE',  ( 0.9999697198139515519, 0.000000000000000000, 0.007781995580013368816 ) ) ;
#32961=LINE ( 'NONE', #37801, #46670 ) ;
#32962=CARTESIAN_POINT ( 'NONE',  ( -19.68560291375552040, -0.03739765774599557863, 4.466501887183837560 ) ) ;
#32963=CARTESIAN_POINT ( 'NONE',  ( -14.90567268141948531, 0.000000000000000000, 9.008243043902110614 ) ) ;
#32964=EDGE_CURVE ( 'NONE', #13331, #42326, #26098, .T. ) ;
#32965=DIRECTION ( 'NONE',  ( -0.005961354470445682716, -0.6427876096865404731, 0.7660212471507180654 ) ) ;
#32966=DIRECTION ( 'NONE',  ( -0.7660212471507179544, -0.6427876096865405842, -0.005961354470445141482 ) ) ;
#32967=AXIS2_PLACEMENT_3D ( 'NONE', #18854, #36174, #49509 ) ;
#32968=VERTEX_POINT ( 'NONE', #12735 ) ;
#32969=DIRECTION ( 'NONE',  ( 0.9999697198139515519, 0.000000000000000000, 0.007781995580013368816 ) ) ;
#32971=ORIENTED_EDGE ( 'NONE', *, *, #34420, .F. ) ;
#32972=FACE_OUTER_BOUND ( 'NONE', #51535, .T. ) ;
#32973=DIRECTION ( 'NONE',  ( -0.9321478471874540261, 0.000000000000000000, 0.3620778797217457656 ) ) ;
#32974=AXIS2_PLACEMENT_3D ( 'NONE', #31512, #1381, #5379 ) ;
#32975=ADVANCED_FACE ( 'NONE', ( #8476 ), #51369, .F. ) ;
#32977=AXIS2_PLACEMENT_3D ( 'NONE', #41720, #38040, #2811 ) ;
#32978=CARTESIAN_POINT ( 'NONE',  ( -13.56079194166738944, 2.067327705546507133, 5.541630197524685997 ) ) ;
#32980=EDGE_CURVE ( 'NONE', #21349, #49949, #4240, .T. ) ;
#32981=ORIENTED_EDGE ( 'NONE', *, *, #29286, .T. ) ;
#32983=LINE ( 'NONE', #11946, #12306 ) ;
#32984=VECTOR ( 'NONE', #15457, 1000.000000000000000 ) ;
#32985=AXIS2_PLACEMENT_3D ( 'NONE', #22442, #26671, #49085 ) ;
#32986=PLANE ( 'NONE',  #51085 ) ;
#32987=DIRECTION ( 'NONE',  ( 0.007781995580012663651, 0.000000000000000000, -0.9999697198139515519 ) ) ;
#32989=DIRECTION ( 'NONE',  ( -0.005002170337468016433, -0.7660444431189770143, 0.6427681459581293666 ) ) ;
#32990=VERTEX_POINT ( 'NONE', #34886 ) ;
#32991=CARTESIAN_POINT ( 'NONE',  ( 3.520599301005862269, -1.000000000000000000, 0.7780620552096689790 ) ) ;
#32992=AXIS2_PLACEMENT_3D ( 'NONE', #52985, #51648, #12492 ) ;
#32993=ORIENTED_EDGE ( 'NONE', *, *, #2846, .F. ) ;
#32994=AXIS2_PLACEMENT_3D ( 'NONE', #21745, #4437, #25719 ) ;
#32995=VERTEX_POINT ( 'NONE', #21555 ) ;
#32996=CARTESIAN_POINT ( 'NONE',  ( -16.45902014130496482, 0.000000000000000000, 3.784329071833556046 ) ) ;
#32997=CARTESIAN_POINT ( 'NONE',  ( -18.77489909422165582, 2.714935509636507316, 8.629801223202855809 ) ) ;
#32998=CARTESIAN_POINT ( 'NONE',  ( -29.86197018149027116, 0.000000000000000000, 8.281335066757780083 ) ) ;
#32999=ORIENTED_EDGE ( 'NONE', *, *, #40581, .T. ) ;
#33000=EDGE_CURVE ( 'NONE', #32426, #46062, #8196, .T. ) ;
#33001=ORIENTED_EDGE ( 'NONE', *, *, #40515, .T. ) ;
#33002=ORIENTED_EDGE ( 'NONE', *, *, #38249, .F. ) ;
#33003=VERTEX_POINT ( 'NONE', #51633 ) ;
#33004=PLANE ( 'NONE',  #55820 ) ;
#33005=VECTOR ( 'NONE', #303, 999.9999999999998863 ) ;
#33006=FACE_OUTER_BOUND ( 'NONE', #37362, .T. ) ;
#33007=ORIENTED_EDGE ( 'NONE', *, *, #1711, .F. ) ;
#33008=CARTESIAN_POINT ( 'NONE',  ( -11.20636620717317378, 0.000000000000000000, 11.32298014792380414 ) ) ;
#33009=VERTEX_POINT ( 'NONE', #25505 ) ;
#33010=AXIS2_PLACEMENT_3D ( 'NONE', #44411, #5261, #23410 ) ;
#33011=DIRECTION ( 'NONE',  ( 0.2426528472758541499, 0.7422098413412800966, 0.6246952433987894571 ) ) ;
#33012=LINE ( 'NONE', #50331, #45829 ) ;
#33013=EDGE_CURVE ( 'NONE', #3665, #35650, #52205, .T. ) ;
#33014=ORIENTED_EDGE ( 'NONE', *, *, #26433, .F. ) ;
#33016=VECTOR ( 'NONE', #33386, 1000.000000000000227 ) ;
#33017=ORIENTED_EDGE ( 'NONE', *, *, #8016, .F. ) ;
#33018=EDGE_CURVE ( 'NONE', #3168, #10121, #3384, .T. ) ;
#33019=CARTESIAN_POINT ( 'NONE',  ( -23.33771345073609638, -0.1191753592594197858, 5.846786880686956955 ) ) ;
#33020=LINE ( 'NONE', #6623, #47440 ) ;
#33021=DIRECTION ( 'NONE',  ( -0.5449076811759708816, 0.6444004775717707689, 0.5364919789714475140 ) ) ;
#33022=LINE ( 'NONE', #54574, #51991 ) ;
#33023=CARTESIAN_POINT ( 'NONE',  ( -9.756139500593079106, -1.014955843830462667, 1.876821366356609344 ) ) ;
#33024=AXIS2_PLACEMENT_3D ( 'NONE', #52553, #5426, #5162 ) ;
#33025=DIRECTION ( 'NONE',  ( 0.000000000000000000, -1.000000000000000000, 0.000000000000000000 ) ) ;
#33026=EDGE_LOOP ( 'NONE', ( #16568, #4266, #6838, #16814 ) ) ;
#33027=VECTOR ( 'NONE', #24786, 1000.000000000000227 ) ;
#33028=EDGE_LOOP ( 'NONE', ( #35886, #17043, #1389 ) ) ;
#33029=ADVANCED_FACE ( 'NONE', ( #29794 ), #21810, .F. ) ;
#33030=PLANE ( 'NONE',  #47298 ) ;
#33031=DIRECTION ( 'NONE',  ( 0.7660212471507180654, -0.6427876096865404731, 0.005961354470445141482 ) ) ;
#33032=CARTESIAN_POINT ( 'NONE',  ( -30.79567442779373110, 0.000000000000000000, 8.843406890442315316 ) ) ;
#33033=DIRECTION ( 'NONE',  ( -0.5364919789714478471, 0.6444004775717705469, -0.5449076811759709926 ) ) ;
#33034=EDGE_CURVE ( 'NONE', #1901, #722, #33740, .T. ) ;
#33035=CARTESIAN_POINT ( 'NONE',  ( -16.42896195337263521, 3.848249166794011522, 2.940719187860218575 ) ) ;
#33036=VECTOR ( 'NONE', #1343, 999.9999999999998863 ) ;
#33037=AXIS2_PLACEMENT_3D ( 'NONE', #8480, #38583, #47365 ) ;
#33038=DIRECTION ( 'NONE',  ( 0.005002170337468016433, -0.7660444431189770143, -0.6427681459581293666 ) ) ;
#33039=EDGE_LOOP ( 'NONE', ( #31002, #8029, #5286, #28215 ) ) ;
#33040=FACE_OUTER_BOUND ( 'NONE', #34490, .T. ) ;
#33043=LINE ( 'NONE', #10899, #9352 ) ;
#33044=DIRECTION ( 'NONE',  ( 0.007781995580012663651, -3.146120232559066537E-19, -0.9999697198139514409 ) ) ;
#33045=ORIENTED_EDGE ( 'NONE', *, *, #38789, .T. ) ;
#33046=EDGE_CURVE ( 'NONE', #44540, #33054, #26344, .T. ) ;
#33047=CARTESIAN_POINT ( 'NONE',  ( -14.93495759592298988, 0.000000000000000000, 12.77129166681078409 ) ) ;
#33048=FACE_OUTER_BOUND ( 'NONE', #42861, .T. ) ;
#33049=LINE ( 'NONE', #18891, #527 ) ;
#33050=CARTESIAN_POINT ( 'NONE',  ( -16.03174594003255038, 0.000000000000000000, 8.588971125952504337 ) ) ;
#33051=DIRECTION ( 'NONE',  ( 0.007781995580012663651, 0.000000000000000000, -0.9999697198139515519 ) ) ;
#33052=VECTOR ( 'NONE', #28845, 1000.000000000000227 ) ;
#33053=EDGE_CURVE ( 'NONE', #28751, #3861, #55324, .T. ) ;
#33054=VERTEX_POINT ( 'NONE', #7937 ) ;
#33055=ORIENTED_EDGE ( 'NONE', *, *, #1104, .T. ) ;
#33056=VECTOR ( 'NONE', #16518, 999.9999999999998863 ) ;
#33057=CARTESIAN_POINT ( 'NONE',  ( -20.84338673312048940, 0.7721120973665037690, 6.244767860881510479 ) ) ;
#33059=LINE ( 'NONE', #41576, #17922 ) ;
#33060=VECTOR ( 'NONE', #48835, 999.9999999999998863 ) ;
#33061=CARTESIAN_POINT ( 'NONE',  ( -10.29784693629447467, -0.1191753592594200495, 1.146949229589934616 ) ) ;
#33062=CARTESIAN_POINT ( 'NONE',  ( -18.35780447774326518, 0.000000000000000000, 8.940201270370220499 ) ) ;
#33063=CARTESIAN_POINT ( 'NONE',  ( -18.88442267121436302, -0.3560938001956556742, 4.205310943792594180 ) ) ;
#33064=VERTEX_POINT ( 'NONE', #25248 ) ;
#33065=FACE_OUTER_BOUND ( 'NONE', #38595, .T. ) ;
#33066=CARTESIAN_POINT ( 'NONE',  ( -21.08970118930990978, 3.848249166794010634, 4.751108586468945738 ) ) ;
#33067=LINE ( 'NONE', #50391, #50495 ) ;
#33068=VECTOR ( 'NONE', #22300, 1000.000000000000114 ) ;
#33070=AXIS2_PLACEMENT_3D ( 'NONE', #7956, #55623, #33234 ) ;
#33072=FACE_OUTER_BOUND ( 'NONE', #50750, .T. ) ;
#33073=CARTESIAN_POINT ( 'NONE',  ( -13.27065584551087163, 0.000000000000000000, 12.04557950825129176 ) ) ;
#33075=ORIENTED_EDGE ( 'NONE', *, *, #40018, .T. ) ;
#33076=DIRECTION ( 'NONE',  ( 0.5449076811759707706, 0.6444004775717708799, -0.5364919789714476250 ) ) ;
#33077=ADVANCED_FACE ( 'NONE', ( #32766 ), #5610, .F. ) ;
#33078=ORIENTED_EDGE ( 'NONE', *, *, #41555, .T. ) ;
#33079=AXIS2_PLACEMENT_3D ( 'NONE', #8631, #17406, #18244 ) ;
#33080=VERTEX_POINT ( 'NONE', #13577 ) ;
#33081=VERTEX_POINT ( 'NONE', #15445 ) ;
#33082=VECTOR ( 'NONE', #6802, 999.9999999999998863 ) ;
#33083=EDGE_CURVE ( 'NONE', #3168, #31521, #40255, .T. ) ;
#33084=ORIENTED_EDGE ( 'NONE', *, *, #12599, .F. ) ;
#33086=ORIENTED_EDGE ( 'NONE', *, *, #7779, .F. ) ;
#33087=CARTESIAN_POINT ( 'NONE',  ( -17.74560456716937296, 0.000000000000000000, 3.774316574337878372 ) ) ;
#33088=ORIENTED_EDGE ( 'NONE', *, *, #38050, .F. ) ;
#33089=ADVANCED_FACE ( 'NONE', ( #9616 ), #35186, .F. ) ;
#33090=EDGE_CURVE ( 'NONE', #6826, #48632, #43658, .T. ) ;
#33091=EDGE_CURVE ( 'NONE', #32088, #14924, #14157, .T. ) ;
#33092=ORIENTED_EDGE ( 'NONE', *, *, #34491, .F. ) ;
#33093=DIRECTION ( 'NONE',  ( 0.7660212471507180654, -0.6427876096865404731, 0.005961354470445141482 ) ) ;
#33094=EDGE_LOOP ( 'NONE', ( #20, #14702, #21727, #13875 ) ) ;
#33095=VERTEX_POINT ( 'NONE', #22934 ) ;
#33096=VECTOR ( 'NONE', #29497, 999.9999999999998863 ) ;
#33097=CARTESIAN_POINT ( 'NONE',  ( -20.06177075545399191, 0.000000000000000000, 14.76272000528038220 ) ) ;
#33098=VECTOR ( 'NONE', #42516, 999.9999999999998863 ) ;
#33099=LINE ( 'NONE', #24851, #22148 ) ;
#33100=DIRECTION ( 'NONE',  ( 0.9999697198139515519, 0.000000000000000000, 0.007781995580013368816 ) ) ;
#33101=DIRECTION ( 'NONE',  ( 0.5364919789714477361, 0.6444004775717706579, 0.5449076811759711036 ) ) ;
#33102=ORIENTED_EDGE ( 'NONE', *, *, #52495, .T. ) ;
#33103=CARTESIAN_POINT ( 'NONE',  ( -17.39384106964635990, -5.698858183938163791, 12.79108746244999395 ) ) ;
#33105=ORIENTED_EDGE ( 'NONE', *, *, #55058, .F. ) ;
#33106=ORIENTED_EDGE ( 'NONE', *, *, #19595, .F. ) ;
#33107=EDGE_CURVE ( 'NONE', #10405, #51867, #18690, .T. ) ;
#33108=DIRECTION ( 'NONE',  ( -0.5364919789714478471, 0.6444004775717705469, -0.5449076811759709926 ) ) ;
#33109=DIRECTION ( 'NONE',  ( -0.6427681459581293666, -0.7660444431189770143, -0.005002170337467561935 ) ) ;
#33110=VECTOR ( 'NONE', #44342, 999.9999999999998863 ) ;
#33112=LINE ( 'NONE', #50431, #28784 ) ;
#33113=VECTOR ( 'NONE', #22274, 999.9999999999998863 ) ;
#33114=AXIS2_PLACEMENT_3D ( 'NONE', #12307, #42108, #50356 ) ;
#33115=CARTESIAN_POINT ( 'NONE',  ( -10.00813838035478298, 0.000000000000000000, 10.77830692922518452 ) ) ;
#33116=EDGE_CURVE ( 'NONE', #44540, #41193, #39969, .T. ) ;
#33117=AXIS2_PLACEMENT_3D ( 'NONE', #46999, #48100, #13202 ) ;
#33118=DIRECTION ( 'NONE',  ( 0.9999697198139515519, 0.000000000000000000, 0.007781995580013368816 ) ) ;
#33119=CARTESIAN_POINT ( 'NONE',  ( -12.10735231521451283, 0.000000000000000000, 7.680841468734264765 ) ) ;
#33120=VERTEX_POINT ( 'NONE', #28231 ) ;
#33121=CARTESIAN_POINT ( 'NONE',  ( -14.89960414888230744, 0.000000000000000000, 8.228449645346760377 ) ) ;
#33122=EDGE_LOOP ( 'NONE', ( #12484, #49737, #55613, #11133 ) ) ;
#33123=VECTOR ( 'NONE', #28987, 1000.000000000000000 ) ;
#33124=ADVANCED_FACE ( 'NONE', ( #39426 ), #30887, .F. ) ;
#33125=LINE ( 'NONE', #24037, #25612 ) ;
#33126=LINE ( 'NONE', #45899, #35981 ) ;
#33127=CARTESIAN_POINT ( 'NONE',  ( -9.439064187057317312, -1.805665653504137769, 2.693112798287724541 ) ) ;
#33128=DIRECTION ( 'NONE',  ( 0.005002170337468016433, -0.7660444431189770143, -0.6427681459581293666 ) ) ;
#33129=DIRECTION ( 'NONE',  ( -0.5364919789714478471, 0.6444004775717705469, -0.5449076811759709926 ) ) ;
#33130=VECTOR ( 'NONE', #15648, 999.9999999999998863 ) ;
#33131=ORIENTED_EDGE ( 'NONE', *, *, #5244, .F. ) ;
#33132=VECTOR ( 'NONE', #30546, 999.9999999999998863 ) ;
#33133=EDGE_LOOP ( 'NONE', ( #17212, #38387, #1766, #567 ) ) ;
#33134=CARTESIAN_POINT ( 'NONE',  ( -19.45503627000849889, 0.000000000000000000, 7.556996783084074742 ) ) ;
#33135=CARTESIAN_POINT ( 'NONE',  ( -15.88130887279446490, 0.000000000000000000, 3.050160814894388839 ) ) ;
#33136=DIRECTION ( 'NONE',  ( 0.9999697198139515519, 0.000000000000000000, 0.007781995580013368816 ) ) ;
#33137=CARTESIAN_POINT ( 'NONE',  ( -10.27421835998572064, 0.000000000000000000, 10.96090226820206048 ) ) ;
#33138=CARTESIAN_POINT ( 'NONE',  ( -9.754109641566973465, 0.000000000000000000, 3.836508235701692637 ) ) ;
#33139=CARTESIAN_POINT ( 'NONE',  ( -13.17065887352947762, -0.1191753592594197858, 12.04635770780929427 ) ) ;
#33140=DIRECTION ( 'NONE',  ( 0.5449076811759707706, 0.6444004775717708799, -0.5364919789714476250 ) ) ;
#33141=AXIS2_PLACEMENT_3D ( 'NONE', #29668, #11188, #12329 ) ;
#33142=DIRECTION ( 'NONE',  ( 0.9999697198139515519, 0.000000000000000000, 0.007781995580013368816 ) ) ;
#33143=VECTOR ( 'NONE', #52082, 1000.000000000000227 ) ;
#33144=CARTESIAN_POINT ( 'NONE',  ( -14.51119359642235374, -0.1191753592594179401, 5.176812759513254036 ) ) ;
#33145=VECTOR ( 'NONE', #40540, 1000.000000000000227 ) ;
#33146=ORIENTED_EDGE ( 'NONE', *, *, #21144, .T. ) ;
#33147=VECTOR ( 'NONE', #4747, 999.9999999999998863 ) ;
#33148=VERTEX_POINT ( 'NONE', #53039 ) ;
#33150=VECTOR ( 'NONE', #36956, 1000.000000000000114 ) ;
#33151=VECTOR ( 'NONE', #54044, 1000.000000000000227 ) ;
#33152=ORIENTED_EDGE ( 'NONE', *, *, #12877, .F. ) ;
#33153=ORIENTED_EDGE ( 'NONE', *, *, #37235, .F. ) ;
#33154=DIRECTION ( 'NONE',  ( -0.9999697198139514409, -0.000000000000000000, -0.007781995580013368816 ) ) ;
#33155=CARTESIAN_POINT ( 'NONE',  ( -18.66354898467281132, 0.000000000000000000, 14.21960318569776582 ) ) ;
#33156=DIRECTION ( 'NONE',  ( 0.007781995580012662783, 0.000000000000000000, -0.9999697198139514409 ) ) ;
#33157=VECTOR ( 'NONE', #14141, 1000.000000000000227 ) ;
#33158=EDGE_CURVE ( 'NONE', #370, #51735, #54351, .T. ) ;
#33159=EDGE_CURVE ( 'NONE', #36173, #35938, #5073, .T. ) ;
#33160=VECTOR ( 'NONE', #8222, 999.9999999999998863 ) ;
#33161=VERTEX_POINT ( 'NONE', #19725 ) ;
#33162=DIRECTION ( 'NONE',  ( -0.005961354470445682716, -0.6427876096865404731, 0.7660212471507180654 ) ) ;
#33163=VECTOR ( 'NONE', #28513, 999.9999999999998863 ) ;
#33164=VERTEX_POINT ( 'NONE', #37051 ) ;
#33165=LINE ( 'NONE', #50482, #51267 ) ;
#33166=EDGE_CURVE ( 'NONE', #53467, #6270, #18383, .T. ) ;
#33167=ORIENTED_EDGE ( 'NONE', *, *, #55868, .F. ) ;
#33168=VECTOR ( 'NONE', #1281, 1000.000000000000227 ) ;
#33169=VECTOR ( 'NONE', #31596, 1000.000000000000227 ) ;
#33171=CARTESIAN_POINT ( 'NONE',  ( -24.26908309836554878, 0.000000000000000000, 6.108867788427308376 ) ) ;
#33172=CARTESIAN_POINT ( 'NONE',  ( -19.32961685222932147, 0.000000000000000000, 14.39908572644263351 ) ) ;
#33173=ORIENTED_EDGE ( 'NONE', *, *, #13321, .F. ) ;
#33174=DIRECTION ( 'NONE',  ( 0.9999697198139515519, 0.000000000000000000, 0.007781995580013368816 ) ) ;
#33175=ORIENTED_EDGE ( 'NONE', *, *, #27842, .T. ) ;
#33176=LINE ( 'NONE', #46203, #47288 ) ;
#33177=LINE ( 'NONE', #50496, #3949 ) ;
#33178=EDGE_CURVE ( 'NONE', #42084, #41830, #35434, .T. ) ;
#33179=PLANE ( 'NONE',  #38184 ) ;
#33180=CARTESIAN_POINT ( 'NONE',  ( -11.18898947068464800, 8.786147236437516383, 1.127809914431977978 ) ) ;
#33181=CARTESIAN_POINT ( 'NONE',  ( -19.27270800389901950, 0.000000000000000000, 7.086420930545378027 ) ) ;
#33182=FACE_OUTER_BOUND ( 'NONE', #55082, .T. ) ;
#33183=DIRECTION ( 'NONE',  ( 0.007781995580012663651, -3.146120232559066537E-19, -0.9999697198139514409 ) ) ;
#33185=EDGE_CURVE ( 'NONE', #36655, #10808, #26937, .T. ) ;
#33186=FACE_OUTER_BOUND ( 'NONE', #55678, .T. ) ;
#33187=DIRECTION ( 'NONE',  ( 0.000000000000000000, -0.000000000000000000, -1.000000000000000000 ) ) ;
#33188=ORIENTED_EDGE ( 'NONE', *, *, #32362, .F. ) ;
#33189=DIRECTION ( 'NONE',  ( 0.007781995580012662783, 0.000000000000000000, -0.9999697198139514409 ) ) ;
#33190=VERTEX_POINT ( 'NONE', #44250 ) ;
#33191=VECTOR ( 'NONE', #11734, 1000.000000000000227 ) ;
#33192=EDGE_CURVE ( 'NONE', #12359, #18681, #31482, .T. ) ;
#33193=DIRECTION ( 'NONE',  ( 0.000000000000000000, -0.000000000000000000, -1.000000000000000000 ) ) ;
#33194=LINE ( 'NONE', #42542, #34179 ) ;
#33195=DIRECTION ( 'NONE',  ( -0.7660212471507179544, -0.6427876096865405842, -0.005961354470445141482 ) ) ;
#33197=DIRECTION ( 'NONE',  ( -0.5364919789714478471, 0.6444004775717705469, -0.5449076811759709926 ) ) ;
#33198=CARTESIAN_POINT ( 'NONE',  ( -0.9975486161969306931, 4.078988103069860038, 3.605855335088290925 ) ) ;
#33199=ADVANCED_FACE ( 'NONE', ( #50660 ), #37598, .F. ) ;
#33200=AXIS2_PLACEMENT_3D ( 'NONE', #53093, #6499, #15305 ) ;
#33201=PLANE ( 'NONE',  #48387 ) ;
#33202=AXIS2_PLACEMENT_3D ( 'NONE', #31904, #23118, #1233 ) ;
#33205=FACE_OUTER_BOUND ( 'NONE', #55399, .T. ) ;
#33206=FACE_OUTER_BOUND ( 'NONE', #49872, .T. ) ;
#33207=CARTESIAN_POINT ( 'NONE',  ( -19.17480688586491056, -0.1191753592594168992, 7.356511861379745554 ) ) ;
#33208=CARTESIAN_POINT ( 'NONE',  ( -27.99767448711536133, 0.000000000000000000, 7.557179307314289218 ) ) ;
#33210=VECTOR ( 'NONE', #29976, 999.9999999999998863 ) ;
#33211=VECTOR ( 'NONE', #50420, 1000.000000000000227 ) ;
#33212=DIRECTION ( 'NONE',  ( 0.9999697198139515519, 0.000000000000000000, 0.007781995580013368816 ) ) ;
#33213=PLANE ( 'NONE',  #52043 ) ;
#33214=CARTESIAN_POINT ( 'NONE',  ( -14.66887761629205222, 0.000000000000000000, 12.58869632783390990 ) ) ;
#33215=PLANE ( 'NONE',  #32857 ) ;
#33216=VERTEX_POINT ( 'NONE', #33900 ) ;
#33217=VECTOR ( 'NONE', #869, 1000.000000000000227 ) ;
#33218=VECTOR ( 'NONE', #37359, 999.9999999999998863 ) ;
#33219=CARTESIAN_POINT ( 'NONE',  ( -33.59133976979808978, -0.1191753592594197858, 9.829643557626155825 ) ) ;
#33220=CARTESIAN_POINT ( 'NONE',  ( -18.12108411398644492, 5.305366725996514710, 3.551507220766565442 ) ) ;
#33221=VERTEX_POINT ( 'NONE', #54612 ) ;
#33222=DIRECTION ( 'NONE',  ( 0.007781995580012662783, 0.000000000000000000, -0.9999697198139514409 ) ) ;
#33223=DIRECTION ( 'NONE',  ( 0.000000000000000000, -0.000000000000000000, -1.000000000000000000 ) ) ;
#33224=VERTEX_POINT ( 'NONE', #12021 ) ;
#33225=VERTEX_POINT ( 'NONE', #33061 ) ;
#33226=CARTESIAN_POINT ( 'NONE',  ( -18.39746900504187010, 0.000000000000000000, 14.03700784672088808 ) ) ;
#33227=VECTOR ( 'NONE', #47884, 1000.000000000000000 ) ;
#33228=ORIENTED_EDGE ( 'NONE', *, *, #23577, .F. ) ;
#33229=ORIENTED_EDGE ( 'NONE', *, *, #37507, .T. ) ;
#33230=ORIENTED_EDGE ( 'NONE', *, *, #36244, .F. ) ;
#33231=DIRECTION ( 'NONE',  ( 0.005002170337468016433, -0.7660444431189770143, -0.6427681459581293666 ) ) ;
#33232=CARTESIAN_POINT ( 'NONE',  ( -9.506711009720374861, 0.000000000000000000, 6.054425967900286309 ) ) ;
#33233=AXIS2_PLACEMENT_3D ( 'NONE', #42038, #21013, #7694 ) ;
#33234=DIRECTION ( 'NONE',  ( 0.005002170337468016433, -0.7660444431189770143, -0.6427681459581293666 ) ) ;
#33235=EDGE_CURVE ( 'NONE', #32088, #43237, #16873, .T. ) ;
#33236=VECTOR ( 'NONE', #43528, 999.9999999999998863 ) ;
#33237=ORIENTED_EDGE ( 'NONE', *, *, #44705, .T. ) ;
#33238=ORIENTED_EDGE ( 'NONE', *, *, #53990, .F. ) ;
#33239=EDGE_CURVE ( 'NONE', #50886, #36877, #46968, .T. ) ;
#33240=ADVANCED_FACE ( 'NONE', ( #15723 ), #24269, .F. ) ;
#33241=VECTOR ( 'NONE', #9290, 1000.000000000000227 ) ;
#33242=FACE_OUTER_BOUND ( 'NONE', #50483, .T. ) ;
#33243=LINE ( 'NONE', #29229, #24545 ) ;
#33244=VERTEX_POINT ( 'NONE', #55759 ) ;
#33245=PLANE ( 'NONE',  #44553 ) ;
#33246=VERTEX_POINT ( 'NONE', #55463 ) ;
#33247=CARTESIAN_POINT ( 'NONE',  ( 2.072287782118878319, 0.000000000000000000, -2.950529333540147015 ) ) ;
#33248=CARTESIAN_POINT ( 'NONE',  ( -14.50346148664584156, -0.6798977022406551551, 3.431396672244436008 ) ) ;
#33249=VECTOR ( 'NONE', #29098, 1000.000000000000227 ) ;
#33251=VECTOR ( 'NONE', #48690, 999.9999999999998863 ) ;
#33252=DIRECTION ( 'NONE',  ( 0.6427681459581294776, -0.7660444431189769032, 0.005002170337467562802 ) ) ;
#33253=AXIS2_PLACEMENT_3D ( 'NONE', #20976, #37188, #20719 ) ;
#33254=DIRECTION ( 'NONE',  ( 0.005961354470445682716, -0.6427876096865404731, -0.7660212471507180654 ) ) ;
#33255=VECTOR ( 'NONE', #54912, 1000.000000000000227 ) ;
#33256=ORIENTED_EDGE ( 'NONE', *, *, #47304, .F. ) ;
#33257=CARTESIAN_POINT ( 'NONE',  ( -19.05834379240982202, 0.000000000000000000, 5.241428813372559503 ) ) ;
#33258=CARTESIAN_POINT ( 'NONE',  ( -17.79526646286806724, -0.1191753592594177180, 9.213908112972596598 ) ) ;
#33259=CARTESIAN_POINT ( 'NONE',  ( -13.73672976910459909, 0.000000000000000000, 12.22661844811216270 ) ) ;
#33260=ORIENTED_EDGE ( 'NONE', *, *, #36619, .T. ) ;
#33261=DIRECTION ( 'NONE',  ( 0.007781995580012663651, -3.146120232559066537E-19, -0.9999697198139514409 ) ) ;
#33262=FACE_OUTER_BOUND ( 'NONE', #25038, .T. ) ;
#33263=LINE ( 'NONE', #53988, #36708 ) ;
#33264=DIRECTION ( 'NONE',  ( 0.6246952433987894571, -0.7422098413412800966, -0.2426528472758541777 ) ) ;
#33265=EDGE_CURVE ( 'NONE', #17790, #56189, #29358, .T. ) ;
#33266=DIRECTION ( 'NONE',  ( 0.005002170337468016433, -0.7660444431189770143, -0.6427681459581293666 ) ) ;
#33267=CARTESIAN_POINT ( 'NONE',  ( -11.74754423342346321, 1.581621852479005552, 4.040177157639987193 ) ) ;
#33268=VECTOR ( 'NONE', #46277, 1000.000000000000227 ) ;
#33269=DIRECTION ( 'NONE',  ( -0.005002170337468016433, -0.7660444431189770143, 0.6427681459581293666 ) ) ;
#33270=ORIENTED_EDGE ( 'NONE', *, *, #26124, .T. ) ;
#33271=LINE ( 'NONE', #50579, #12646 ) ;
#33273=DIRECTION ( 'NONE',  ( 0.6427681459581294776, -0.7660444431189769032, 0.005002170337467562802 ) ) ;
#33275=ORIENTED_EDGE ( 'NONE', *, *, #35947, .F. ) ;
#33276=FACE_OUTER_BOUND ( 'NONE', #45281, .T. ) ;
#33277=CARTESIAN_POINT ( 'NONE',  ( -20.87463720344803875, 3.038739411681508518, 4.693398030193443482 ) ) ;
#33278=EDGE_CURVE ( 'NONE', #28372, #41541, #12335, .T. ) ;
#33279=VECTOR ( 'NONE', #20342, 999.9999999999998863 ) ;
#33280=EDGE_CURVE ( 'NONE', #37122, #17347, #16564, .T. ) ;
#33281=LINE ( 'NONE', #16481, #18604 ) ;
#33283=CARTESIAN_POINT ( 'NONE',  ( -17.26532721389163072, 0.000000000000000000, 13.67648636611514590 ) ) ;
#33284=ORIENTED_EDGE ( 'NONE', *, *, #23980, .T. ) ;
#33285=VECTOR ( 'NONE', #31231, 1000.000000000000227 ) ;
#33286=ORIENTED_EDGE ( 'NONE', *, *, #23515, .F. ) ;
#33287=CARTESIAN_POINT ( 'NONE',  ( -19.32961685222932147, 0.000000000000000000, 14.39908572644263351 ) ) ;
#33288=CARTESIAN_POINT ( 'NONE',  ( 2.072287782118878319, 0.000000000000000000, -2.950529333540147015 ) ) ;
#33289=VECTOR ( 'NONE', #6773, 1000.000000000000114 ) ;
#33290=VERTEX_POINT ( 'NONE', #11491 ) ;
#33291=PLANE ( 'NONE',  #7748 ) ;
#33293=DIRECTION ( 'NONE',  ( -0.6427681459581293666, -0.7660444431189770143, -0.005002170337467561935 ) ) ;
#33294=AXIS2_PLACEMENT_3D ( 'NONE', #39774, #5980, #44019 ) ;
#33295=ORIENTED_EDGE ( 'NONE', *, *, #6754, .F. ) ;
#33296=ORIENTED_EDGE ( 'NONE', *, *, #42760, .T. ) ;
#33297=VERTEX_POINT ( 'NONE', #24521 ) ;
#33298=CARTESIAN_POINT ( 'NONE',  ( -11.70037978733358131, -0.1191753592594185229, 2.244030604059197742 ) ) ;
#33299=ADVANCED_FACE ( 'NONE', ( #34205 ), #33354, .F. ) ;
#33300=DIRECTION ( 'NONE',  ( 0.7660212471507180654, -0.6427876096865404731, 0.005961354470445141482 ) ) ;
#33301=LINE ( 'NONE', #4324, #50242 ) ;
#33302=ORIENTED_EDGE ( 'NONE', *, *, #29672, .F. ) ;
#33303=DIRECTION ( 'NONE',  ( -0.005961354470445682716, -0.6427876096865404731, 0.7660212471507180654 ) ) ;
#33305=VERTEX_POINT ( 'NONE', #19982 ) ;
#33306=EDGE_CURVE ( 'NONE', #54123, #20350, #8070, .T. ) ;
#33307=ORIENTED_EDGE ( 'NONE', *, *, #40443, .T. ) ;
#33309=DIRECTION ( 'NONE',  ( -0.5449076811759708816, 0.6444004775717707689, 0.5364919789714475140 ) ) ;
#33310=DIRECTION ( 'NONE',  ( 0.7660212471507180654, -0.6427876096865404731, 0.005961354470445141482 ) ) ;
#33311=ORIENTED_EDGE ( 'NONE', *, *, #31930, .T. ) ;
#33312=CARTESIAN_POINT ( 'NONE',  ( -21.37940959735528423, -5.536956232915666298, 5.009151959621898520 ) ) ;
#33313=ORIENTED_EDGE ( 'NONE', *, *, #6426, .F. ) ;
#33314=LINE ( 'NONE', #45787, #44904 ) ;
#33316=EDGE_LOOP ( 'NONE', ( #6478, #28073, #16535, #43741 ) ) ;
#33317=CARTESIAN_POINT ( 'NONE',  ( -17.96629124694975488, 4.495856970884008597, 11.23850599833945552 ) ) ;
#33319=ADVANCED_FACE ( 'NONE', ( #41835 ), #7487, .F. ) ;
#33320=VECTOR ( 'NONE', #24584, 1000.000000000000114 ) ;
#33321=DIRECTION ( 'NONE',  ( 0.000000000000000000, -0.000000000000000000, -1.000000000000000000 ) ) ;
#33322=CARTESIAN_POINT ( 'NONE',  ( -10.27421835998572064, 0.000000000000000000, 10.96090226820206048 ) ) ;
#33323=LINE ( 'NONE', #15168, #22348 ) ;
#33324=LINE ( 'NONE', #29038, #30590 ) ;
#33325=CARTESIAN_POINT ( 'NONE',  ( -17.74404816805336793, 0.000000000000000000, 3.574322630375089460 ) ) ;
#33326=ORIENTED_EDGE ( 'NONE', *, *, #22969, .T. ) ;
#33327=ORIENTED_EDGE ( 'NONE', *, *, #38444, .T. ) ;
#33328=VECTOR ( 'NONE', #17181, 1000.000000000000000 ) ;
#33329=LINE ( 'NONE', #55436, #18276 ) ;
#33330=PLANE ( 'NONE',  #33951 ) ;
#33331=CARTESIAN_POINT ( 'NONE',  ( -9.359795358673375532, -2.003343105922557488, 2.897185656270504062 ) ) ;
#33332=DIRECTION ( 'NONE',  ( -0.9999697198139514409, -0.000000000000000000, -0.007781995580013368816 ) ) ;
#33333=CARTESIAN_POINT ( 'NONE',  ( -17.33547259272246066, -2.946525016555662457, 3.520997812542008720 ) ) ;
#33334=LINE ( 'NONE', #51492, #24917 ) ;
#33335=EDGE_LOOP ( 'NONE', ( #23507, #44340, #53422, #50470 ) ) ;
#33336=LINE ( 'NONE', #46352, #35899 ) ;
#33337=LINE ( 'NONE', #42666, #20492 ) ;
#33339=FACE_OUTER_BOUND ( 'NONE', #45938, .T. ) ;
#33340=DIRECTION ( 'NONE',  ( 0.8531650599175527594, 0.4028455766673922356, -0.3313982828793700652 ) ) ;
#33341=EDGE_LOOP ( 'NONE', ( #33238, #42343, #30860, #40023 ) ) ;
#33343=LINE ( 'NONE', #15710, #16985 ) ;
#33344=EDGE_CURVE ( 'NONE', #32684, #171, #25120, .T. ) ;
#33345=DIRECTION ( 'NONE',  ( 0.7660212471507180654, -0.6427876096865404731, 0.005961354470445141482 ) ) ;
#33346=CARTESIAN_POINT ( 'NONE',  ( -16.37836334430254581, -0.1191753592594192307, 6.270278222214512809 ) ) ;
#33347=CARTESIAN_POINT ( 'NONE',  ( -12.13851405436063047, 0.000000000000000000, 11.68505802764555135 ) ) ;
#33349=ORIENTED_EDGE ( 'NONE', *, *, #458, .F. ) ;
#33350=PLANE ( 'NONE',  #38508 ) ;
#33351=CARTESIAN_POINT ( 'NONE',  ( -20.44726175016783287, -5.536956232915667186, 4.647074079900152199 ) ) ;
#33352=DIRECTION ( 'NONE',  ( -0.5364919789714478471, 0.6444004775717705469, -0.5449076811759709926 ) ) ;
#33353=EDGE_CURVE ( 'NONE', #7607, #37255, #45836, .T. ) ;
#33354=PLANE ( 'NONE',  #49633 ) ;
#33355=LINE ( 'NONE', #15446, #25564 ) ;
#33356=PLANE ( 'NONE',  #14971 ) ;
#33357=ORIENTED_EDGE ( 'NONE', *, *, #29506, .T. ) ;
#33358=ADVANCED_FACE ( 'NONE', ( #2661 ), #37303, .F. ) ;
#33359=CARTESIAN_POINT ( 'NONE',  ( 2.072287782118878319, 0.000000000000000000, -2.950529333540147015 ) ) ;
#33360=ADVANCED_FACE ( 'NONE', ( #16286 ), #17144, .F. ) ;
#33361=DIRECTION ( 'NONE',  ( -0.005002170337468016433, -0.7660444431189770143, 0.6427681459581293666 ) ) ;
#33362=AXIS2_PLACEMENT_3D ( 'NONE', #52353, #39273, #30770 ) ;
#33364=ORIENTED_EDGE ( 'NONE', *, *, #42686, .T. ) ;
#33366=EDGE_CURVE ( 'NONE', #18631, #10456, #30503, .T. ) ;
#33367=DIRECTION ( 'NONE',  ( 0.6427681459581294776, -0.7660444431189769032, 0.005002170337467562802 ) ) ;
#33368=DIRECTION ( 'NONE',  ( 0.007781995580012662783, 0.000000000000000000, -0.9999697198139514409 ) ) ;
#33370=VECTOR ( 'NONE', #36135, 1000.000000000000227 ) ;
#33371=DIRECTION ( 'NONE',  ( -0.005002170337468016433, -0.7660444431189770143, 0.6427681459581293666 ) ) ;
#33372=EDGE_CURVE ( 'NONE', #34449, #30378, #8330, .T. ) ;
#33373=VERTEX_POINT ( 'NONE', #25650 ) ;
#33374=ADVANCED_FACE ( 'NONE', ( #22530 ), #362, .F. ) ;
#33375=ORIENTED_EDGE ( 'NONE', *, *, #4093, .F. ) ;
#33376=VERTEX_POINT ( 'NONE', #17703 ) ;
#33377=ORIENTED_EDGE ( 'NONE', *, *, #32334, .F. ) ;
#33378=LINE ( 'NONE', #7512, #33857 ) ;
#33379=ORIENTED_EDGE ( 'NONE', *, *, #38661, .T. ) ;
#33380=EDGE_CURVE ( 'NONE', #34545, #1702, #30199, .T. ) ;
#33381=ORIENTED_EDGE ( 'NONE', *, *, #7952, .F. ) ;
#33382=LINE ( 'NONE', #6990, #40398 ) ;
#33383=ORIENTED_EDGE ( 'NONE', *, *, #1427, .T. ) ;
#33384=VERTEX_POINT ( 'NONE', #38740 ) ;
#33385=ADVANCED_FACE ( 'NONE', ( #48342 ), #21415, .F. ) ;
#33386=DIRECTION ( 'NONE',  ( -0.9999697198139514409, -0.000000000000000000, -0.007781995580013368816 ) ) ;
#33387=DIRECTION ( 'NONE',  ( 0.5364919789714477361, 0.6444004775717706579, 0.5449076811759711036 ) ) ;
#33388=LINE ( 'NONE', #15759, #12379 ) ;
#33389=CARTESIAN_POINT ( 'NONE',  ( -12.71487129044241904, 1.095915999411505526, 1.585854081413927474 ) ) ;
#33390=ORIENTED_EDGE ( 'NONE', *, *, #314, .T. ) ;
#33391=ORIENTED_EDGE ( 'NONE', *, *, #47917, .T. ) ;
#33393=DIRECTION ( 'NONE',  ( -0.005002170337468016433, -0.7660444431189770143, 0.6427681459581293666 ) ) ;
#33394=LINE ( 'NONE', #50700, #5207 ) ;
#33395=FACE_OUTER_BOUND ( 'NONE', #52749, .T. ) ;
#33396=LINE ( 'NONE', #28857, #51241 ) ;
#33397=LINE ( 'NONE', #11793, #34982 ) ;
#33398=VERTEX_POINT ( 'NONE', #52608 ) ;
#33399=DIRECTION ( 'NONE',  ( 0.9999697198139515519, 0.000000000000000000, 0.007781995580013368816 ) ) ;
#33401=VECTOR ( 'NONE', #13071, 999.9999999999998863 ) ;
#33402=CARTESIAN_POINT ( 'NONE',  ( -12.81515292046355725, 2.876837460659008361, 1.567986153331332844 ) ) ;
#33403=LINE ( 'NONE', #50709, #29304 ) ;
#33404=DIRECTION ( 'NONE',  ( 0.7660212471507180654, -0.6427876096865404731, 0.005961354470445141482 ) ) ;
#33405=DIRECTION ( 'NONE',  ( 0.005961354470445682716, -0.6427876096865404731, -0.7660212471507180654 ) ) ;
#33407=CARTESIAN_POINT ( 'NONE',  ( -16.44621519763577666, -5.213152330870664208, 3.103262762558621990 ) ) ;
#33408=CARTESIAN_POINT ( 'NONE',  ( -20.11466289002168750, 1.581621852479007106, 4.444687877008841603 ) ) ;
#33409=ORIENTED_EDGE ( 'NONE', *, *, #46909, .F. ) ;
#33410=ORIENTED_EDGE ( 'NONE', *, *, #16983, .T. ) ;
#33411=DIRECTION ( 'NONE',  ( 0.9999697198139515519, 0.000000000000000000, 0.007781995580013368816 ) ) ;
#33413=LINE ( 'NONE', #25437, #49654 ) ;
#33414=ADVANCED_FACE ( 'NONE', ( #47816 ), #43287, .F. ) ;
#33415=ADVANCED_FACE ( 'NONE', ( #21945 ), #17987, .F. ) ;
#33416=PLANE ( 'NONE',  #43675 ) ;
#33417=CARTESIAN_POINT ( 'NONE',  ( -15.88130887279446490, 0.000000000000000000, 3.050160814894388839 ) ) ;
#33418=DIRECTION ( 'NONE',  ( -0.9999697198139514409, -0.000000000000000000, -0.007781995580013368816 ) ) ;
#33419=LINE ( 'NONE', #50725, #47411 ) ;
#33420=EDGE_CURVE ( 'NONE', #20361, #24739, #5218, .T. ) ;
#33421=LINE ( 'NONE', #11818, #36887 ) ;
#33422=DIRECTION ( 'NONE',  ( 0.007781995580012662783, 0.000000000000000000, -0.9999697198139514409 ) ) ;
#33423=ORIENTED_EDGE ( 'NONE', *, *, #15200, .T. ) ;
#33424=ORIENTED_EDGE ( 'NONE', *, *, #13822, .F. ) ;
#33425=EDGE_CURVE ( 'NONE', #17269, #43836, #26222, .T. ) ;
#33426=EDGE_CURVE ( 'NONE', #547, #40934, #12606, .T. ) ;
#33427=EDGE_LOOP ( 'NONE', ( #52912, #4338, #19971, #40431 ) ) ;
#33428=EDGE_LOOP ( 'NONE', ( #35193, #30610, #13189, #38390 ) ) ;
#33429=ORIENTED_EDGE ( 'NONE', *, *, #2580, .T. ) ;
#33431=CARTESIAN_POINT ( 'NONE',  ( -15.40103151951671734, 0.000000000000000000, 12.95233060667165681 ) ) ;
#33432=DIRECTION ( 'NONE',  ( 0.5364919789714477361, 0.6444004775717706579, 0.5449076811759711036 ) ) ;
#33434=EDGE_CURVE ( 'NONE', #44937, #37525, #17404, .T. ) ;
#33435=VECTOR ( 'NONE', #30760, 999.9999999999998863 ) ;
#33436=ORIENTED_EDGE ( 'NONE', *, *, #43243, .T. ) ;
#33437=CARTESIAN_POINT ( 'NONE',  ( -20.54204810873173415, 0.000000000000000000, 4.860550213503115558 ) ) ;
#33438=ORIENTED_EDGE ( 'NONE', *, *, #29322, .F. ) ;
#33439=CARTESIAN_POINT ( 'NONE',  ( -18.11889143909580469, 0.000000000000000000, 3.940737583172497782 ) ) ;
#33440=ORIENTED_EDGE ( 'NONE', *, *, #7076, .T. ) ;
#33442=CARTESIAN_POINT ( 'NONE',  ( -15.60102546347950536, 0.000000000000000000, 12.95077420755565356 ) ) ;
#33443=CARTESIAN_POINT ( 'NONE',  ( -18.34918231722741666, 0.000000000000000000, 7.832272160596925659 ) ) ;
#33444=ORIENTED_EDGE ( 'NONE', *, *, #33631, .F. ) ;
#33445=DIRECTION ( 'NONE',  ( -0.3620778797217457656, 0.000000000000000000, -0.9321478471874539151 ) ) ;
#33447=DIRECTION ( 'NONE',  ( 0.9999697198139515519, 0.000000000000000000, 0.007781995580013368816 ) ) ;
#33448=DIRECTION ( 'NONE',  ( -0.6427681459581293666, -0.7660444431189770143, -0.005002170337467561935 ) ) ;
#33449=LINE ( 'NONE', #28635, #34191 ) ;
#33450=LINE ( 'NONE', #11848, #1398 ) ;
#33451=CARTESIAN_POINT ( 'NONE',  ( -28.92982233430281980, 0.000000000000000000, 7.919257187036034651 ) ) ;
#33452=CARTESIAN_POINT ( 'NONE',  ( -18.86354292863559579, 0.000000000000000000, 14.21804678658176080 ) ) ;
#33453=LINE ( 'NONE', #51343, #2160 ) ;
#33454=DIRECTION ( 'NONE',  ( 0.007781995580012663651, 0.000000000000000000, -0.9999697198139515519 ) ) ;
#33455=ORIENTED_EDGE ( 'NONE', *, *, #40578, .T. ) ;
#33456=FACE_OUTER_BOUND ( 'NONE', #3043, .T. ) ;
#33457=EDGE_LOOP ( 'NONE', ( #53294, #19933, #49132, #35007 ) ) ;
#33458=ADVANCED_FACE ( 'NONE', ( #56054 ), #34455, .F. ) ;
#33459=LINE ( 'NONE', #34313, #16574 ) ;
#33460=DIRECTION ( 'NONE',  ( 0.005002170337468016433, -0.7660444431189770143, -0.6427681459581293666 ) ) ;
#33461=DIRECTION ( 'NONE',  ( 0.6427681459581294776, -0.7660444431189769032, 0.005002170337467562802 ) ) ;
#33462=EDGE_CURVE ( 'NONE', #52707, #46034, #67, .T. ) ;
#33463=DIRECTION ( 'NONE',  ( -0.5364919789714478471, 0.6444004775717705469, -0.5449076811759709926 ) ) ;
#33464=DIRECTION ( 'NONE',  ( -0.7660212471507179544, -0.6427876096865405842, -0.005961354470445141482 ) ) ;
#33465=CARTESIAN_POINT ( 'NONE',  ( -30.79411802867772607, 0.000000000000000000, 8.643412946479525516 ) ) ;
#33467=ORIENTED_EDGE ( 'NONE', *, *, #37593, .T. ) ;
#33468=EDGE_CURVE ( 'NONE', #48904, #46790, #13166, .T. ) ;
#33469=DIRECTION ( 'NONE',  ( -0.9999697198139514409, -0.000000000000000000, -0.007781995580013368816 ) ) ;
#33470=DIRECTION ( 'NONE',  ( 0.007781995580012663651, 0.000000000000000000, -0.9999697198139515519 ) ) ;
#33471=LINE ( 'NONE', #34038, #411 ) ;
#33472=CARTESIAN_POINT ( 'NONE',  ( -22.40634380310664397, 0.000000000000000000, 5.584705972946605534 ) ) ;
#33473=ADVANCED_FACE ( 'NONE', ( #1197 ), #44942, .F. ) ;
#33474=ADVANCED_FACE ( 'NONE', ( #23370 ), #14836, .F. ) ;
#33475=EDGE_CURVE ( 'NONE', #3340, #22086, #45472, .T. ) ;
#33477=FACE_OUTER_BOUND ( 'NONE', #43471, .T. ) ;
#33478=ADVANCED_FACE ( 'NONE', ( #36154 ), #40107, .F. ) ;
#33479=CARTESIAN_POINT ( 'NONE',  ( -17.77802214183636664, -0.1191753592594185784, 6.998049893426011359 ) ) ;
#33480=DIRECTION ( 'NONE',  ( 0.000000000000000000, -0.000000000000000000, -1.000000000000000000 ) ) ;
#33481=ORIENTED_EDGE ( 'NONE', *, *, #16058, .T. ) ;
#33482=CARTESIAN_POINT ( 'NONE',  ( -18.32463349006915010, 0.000000000000000000, 4.677800590572023687 ) ) ;
#33483=DIRECTION ( 'NONE',  ( 0.7660212471507180654, -0.6427876096865404731, 0.005961354470445141482 ) ) ;
#33484=ORIENTED_EDGE ( 'NONE', *, *, #18549, .T. ) ;
#33485=EDGE_LOOP ( 'NONE', ( #16393, #12239, #26266, #44232 ) ) ;
#33486=CARTESIAN_POINT ( 'NONE',  ( -17.06374735823969147, 1.257817950434005461, 5.573753622435739352 ) ) ;
#33487=ORIENTED_EDGE ( 'NONE', *, *, #3788, .T. ) ;
#33488=EDGE_CURVE ( 'NONE', #33893, #17923, #28160, .T. ) ;
#33489=VERTEX_POINT ( 'NONE', #27621 ) ;
#33490=CARTESIAN_POINT ( 'NONE',  ( -18.76354595665420177, -0.1191753592594177458, 14.21882498613976331 ) ) ;
#33491=EDGE_CURVE ( 'NONE', #45690, #44220, #44372, .T. ) ;
#33492=ORIENTED_EDGE ( 'NONE', *, *, #53911, .T. ) ;
#33493=EDGE_LOOP ( 'NONE', ( #40994, #54354, #23732, #11357 ) ) ;
#33494=ORIENTED_EDGE ( 'NONE', *, *, #53238, .T. ) ;
#33495=EDGE_CURVE ( 'NONE', #41657, #18997, #32451, .T. ) ;
#33496=CARTESIAN_POINT ( 'NONE',  ( -17.67880336941297870, 0.000000000000000000, 7.098825064965410547 ) ) ;
#33497=CARTESIAN_POINT ( 'NONE',  ( -11.33496166291588558, 0.000000000000000000, 2.146871344287814232 ) ) ;
#33498=FACE_OUTER_BOUND ( 'NONE', #15650, .T. ) ;
#33499=ADVANCED_FACE ( 'NONE', ( #6583 ), #31611, .F. ) ;
#33500=ORIENTED_EDGE ( 'NONE', *, *, #50933, .T. ) ;
#33501=ORIENTED_EDGE ( 'NONE', *, *, #54985, .T. ) ;
#33503=CARTESIAN_POINT ( 'NONE',  ( -11.83696125532564558, 0.000000000000000000, 6.944281574870742269 ) ) ;
#33504=DIRECTION ( 'NONE',  ( 0.005961354470445682716, -0.6427876096865404731, -0.7660212471507180654 ) ) ;
#33505=ORIENTED_EDGE ( 'NONE', *, *, #54229, .T. ) ;
#33506=PLANE ( 'NONE',  #34588 ) ;
#33507=ORIENTED_EDGE ( 'NONE', *, *, #21989, .T. ) ;
#33508=CARTESIAN_POINT ( 'NONE',  ( -12.77226246836278989, 0.6102101463440035012, 1.623643323592976140 ) ) ;
#33509=DIRECTION ( 'NONE',  ( 0.007781995580012663651, -3.146120232559066537E-19, -0.9999697198139514409 ) ) ;
#33511=ORIENTED_EDGE ( 'NONE', *, *, #38026, .F. ) ;
#33513=DIRECTION ( 'NONE',  ( 0.005961354470445682716, -0.6427876096865404731, -0.7660212471507180654 ) ) ;
#33514=ORIENTED_EDGE ( 'NONE', *, *, #50480, .F. ) ;
#33515=LINE ( 'NONE', #42589, #15865 ) ;
#33516=DIRECTION ( 'NONE',  ( 0.007781995580012663651, 0.000000000000000000, -0.9999697198139515519 ) ) ;
#33517=FACE_OUTER_BOUND ( 'NONE', #30016, .T. ) ;
#33518=EDGE_LOOP ( 'NONE', ( #24408, #47539, #34963, #37713 ) ) ;
#33519=DIRECTION ( 'NONE',  ( 0.000000000000000000, -1.000000000000000000, 0.000000000000000000 ) ) ;
#33520=DIRECTION ( 'NONE',  ( 0.000000000000000000, -0.000000000000000000, -1.000000000000000000 ) ) ;
#33521=DIRECTION ( 'NONE',  ( 0.9999697198139515519, 0.000000000000000000, 0.007781995580013368816 ) ) ;
#33522=DIRECTION ( 'NONE',  ( 0.9999697198139515519, 0.000000000000000000, 0.007781995580013368816 ) ) ;
#33523=DIRECTION ( 'NONE',  ( 0.005961354470445682716, -0.6427876096865404731, -0.7660212471507180654 ) ) ;
#33524=CARTESIAN_POINT ( 'NONE',  ( -21.57722033895402092, 4.981562823951513508, 4.904318941198996029 ) ) ;
#33526=EDGE_LOOP ( 'NONE', ( #51713, #19426, #40501, #3279 ) ) ;
#33527=CARTESIAN_POINT ( 'NONE',  ( -16.72366309418326225, 0.000000000000000000, 3.782269559181549390 ) ) ;
#33528=DIRECTION ( 'NONE',  ( 0.007781995580012662783, 0.000000000000000000, -0.9999697198139514409 ) ) ;
#33529=DIRECTION ( 'NONE',  ( 0.5449076811759707706, 0.6444004775717708799, -0.5364919789714476250 ) ) ;
#33530=ORIENTED_EDGE ( 'NONE', *, *, #208, .F. ) ;
#33531=LINE ( 'NONE', #41505, #2982 ) ;
#33532=DIRECTION ( 'NONE',  ( 0.5449076811759707706, 0.6444004775717708799, -0.5364919789714476250 ) ) ;
#33533=EDGE_CURVE ( 'NONE', #14352, #21126, #6063, .T. ) ;
#33534=EDGE_CURVE ( 'NONE', #12878, #23644, #19659, .T. ) ;
#33535=CARTESIAN_POINT ( 'NONE',  ( -11.22056963685719211, 0.000000000000000000, 1.239771416285661010 ) ) ;
#33536=EDGE_CURVE ( 'NONE', #40102, #44513, #27918, .T. ) ;
#33537=LINE ( 'NONE', #2316, #54127 ) ;
#33538=PLANE ( 'NONE',  #26574 ) ;
#33539=EDGE_LOOP ( 'NONE', ( #19799, #1898, #47099, #44043, #34071 ) ) ;
#33540=ORIENTED_EDGE ( 'NONE', *, *, #40906, .T. ) ;
#33542=DIRECTION ( 'NONE',  ( 0.5364919789714477361, 0.6444004775717706579, 0.5449076811759711036 ) ) ;
#33543=VERTEX_POINT ( 'NONE', #49757 ) ;
#33544=FACE_OUTER_BOUND ( 'NONE', #8938, .T. ) ;
#33545=ORIENTED_EDGE ( 'NONE', *, *, #34015, .T. ) ;
#33546=LINE ( 'NONE', #34400, #24745 ) ;
#33547=ORIENTED_EDGE ( 'NONE', *, *, #51788, .F. ) ;
#33548=VERTEX_POINT ( 'NONE', #2324 ) ;
#33549=ORIENTED_EDGE ( 'NONE', *, *, #10263, .F. ) ;
#33550=PLANE ( 'NONE',  #43763 ) ;
#33551=DIRECTION ( 'NONE',  ( 0.6427681459581294776, -0.7660444431189769032, 0.005002170337467562802 ) ) ;
#33552=DIRECTION ( 'NONE',  ( 0.007781995580012663651, 0.000000000000000000, -0.9999697198139515519 ) ) ;
#33553=DIRECTION ( 'NONE',  ( 0.7660212471507180654, -0.6427876096865404731, 0.005961354470445141482 ) ) ;
#33554=ORIENTED_EDGE ( 'NONE', *, *, #21253, .T. ) ;
#33555=ADVANCED_FACE ( 'NONE', ( #52888 ), #6320, .F. ) ;
#33557=ORIENTED_EDGE ( 'NONE', *, *, #36547, .T. ) ;
#33558=CARTESIAN_POINT ( 'NONE',  ( -10.77487009789602368, -0.6798977022406563764, 1.983085153357455166 ) ) ;
#33559=EDGE_CURVE ( 'NONE', #40825, #28225, #35875, .T. ) ;
#33560=CARTESIAN_POINT ( 'NONE',  ( -27.99767448711536133, 0.000000000000000000, 7.557179307314289218 ) ) ;
#33561=ORIENTED_EDGE ( 'NONE', *, *, #6930, .F. ) ;
#33562=CARTESIAN_POINT ( 'NONE',  ( -17.78951835585749919, -0.1191753592594190225, 8.475288706457071441 ) ) ;
#33563=EDGE_CURVE ( 'NONE', #12727, #2320, #36405, .T. ) ;
#33564=ORIENTED_EDGE ( 'NONE', *, *, #27342, .F. ) ;
#33565=DIRECTION ( 'NONE',  ( -0.5364919789714478471, 0.6444004775717705469, -0.5449076811759709926 ) ) ;
#33566=FACE_OUTER_BOUND ( 'NONE', #38027, .T. ) ;
#33567=ORIENTED_EDGE ( 'NONE', *, *, #32701, .T. ) ;
#33568=EDGE_CURVE ( 'NONE', #12564, #22624, #31323, .T. ) ;
#33569=LINE ( 'NONE', #6915, #44951 ) ;
#33570=ORIENTED_EDGE ( 'NONE', *, *, #9897, .T. ) ;
#33571=AXIS2_PLACEMENT_3D ( 'NONE', #20079, #37408, #35976 ) ;
#33572=LINE ( 'NONE', #7185, #154 ) ;
#33573=CARTESIAN_POINT ( 'NONE',  ( -25.20200914511100265, -0.1191753592594197858, 6.570942640130446932 ) ) ;
#33574=ORIENTED_EDGE ( 'NONE', *, *, #13911, .F. ) ;
#33575=CARTESIAN_POINT ( 'NONE',  ( -18.97020357541589775, -4.889348428825664783, 4.093996603269308920 ) ) ;
#33576=DIRECTION ( 'NONE',  ( -0.7660212471507179544, -0.6427876096865405842, -0.005961354470445141482 ) ) ;
#33577=PLANE ( 'NONE',  #5120 ) ;
#33578=FACE_OUTER_BOUND ( 'NONE', #38513, .T. ) ;
#33580=VERTEX_POINT ( 'NONE', #22788 ) ;
#33581=CARTESIAN_POINT ( 'NONE',  ( -16.99924723426068951, 0.000000000000000000, 13.49389102713827171 ) ) ;
#33582=FACE_OUTER_BOUND ( 'NONE', #29533, .T. ) ;
#33584=CARTESIAN_POINT ( 'NONE',  ( -14.01623497886155256, -0.1191753592594197858, 2.226008083469502630 ) ) ;
#33585=CARTESIAN_POINT ( 'NONE',  ( 2.072287782118878319, 0.000000000000000000, -2.950529333540147015 ) ) ;
#33586=CARTESIAN_POINT ( 'NONE',  ( -25.20278734466900517, 0.000000000000000000, 6.670939612111840944 ) ) ;
#33587=ORIENTED_EDGE ( 'NONE', *, *, #5350, .F. ) ;
#33588=CARTESIAN_POINT ( 'NONE',  ( -12.64402384854216699, -0.1191753592594183703, 4.083347296812000593 ) ) ;
#33589=CARTESIAN_POINT ( 'NONE',  ( -13.07066190154808361, 0.000000000000000000, 12.04713590736729678 ) ) ;
#33590=ORIENTED_EDGE ( 'NONE', *, *, #23661, .T. ) ;
#33591=CARTESIAN_POINT ( 'NONE',  ( -16.47470806322066039, 0.000000000000000000, 5.800193347417353706 ) ) ;
#33592=VERTEX_POINT ( 'NONE', #29589 ) ;
#33594=DIRECTION ( 'NONE',  ( 0.005961354470445682716, -0.6427876096865404731, -0.7660212471507180654 ) ) ;
#33595=CARTESIAN_POINT ( 'NONE',  ( -15.46345981814678616, -0.1191753592594185784, 8.124058562039351727 ) ) ;
#33596=CARTESIAN_POINT ( 'NONE',  ( -9.075990533167328067, 0.000000000000000000, 10.41622904950343909 ) ) ;
#33598=EDGE_CURVE ( 'NONE', #32693, #38304, #37236, .T. ) ;
#33599=DIRECTION ( 'NONE',  ( -0.005002170337468016433, -0.7660444431189770143, 0.6427681459581293666 ) ) ;
#33601=ORIENTED_EDGE ( 'NONE', *, *, #55448, .T. ) ;
#33602=VERTEX_POINT ( 'NONE', #16492 ) ;
#33603=CARTESIAN_POINT ( 'NONE',  ( -16.53317331066696383, 0.000000000000000000, 13.31285208727739899 ) ) ;
#33604=FACE_OUTER_BOUND ( 'NONE', #51245, .T. ) ;
#33605=DIRECTION ( 'NONE',  ( 0.9999697198139515519, 0.000000000000000000, 0.007781995580013368816 ) ) ;
#33607=FACE_OUTER_BOUND ( 'NONE', #47906, .T. ) ;
#33608=DIRECTION ( 'NONE',  ( 0.9999697198139515519, 0.000000000000000000, 0.007781995580013368816 ) ) ;
#33609=ORIENTED_EDGE ( 'NONE', *, *, #51959, .T. ) ;
#33610=PLANE ( 'NONE',  #7484 ) ;
#33611=EDGE_CURVE ( 'NONE', #52077, #13086, #38081, .T. ) ;
#33612=VECTOR ( 'NONE', #44087, 999.9999999999998863 ) ;
#33613=LINE ( 'NONE', #12344, #24180 ) ;
#33614=CARTESIAN_POINT ( 'NONE',  ( -13.73672976910459909, 0.000000000000000000, 12.22661844811216270 ) ) ;
#33615=ORIENTED_EDGE ( 'NONE', *, *, #21775, .T. ) ;
#33617=DIRECTION ( 'NONE',  ( -0.9999697198139514409, -0.000000000000000000, -0.007781995580013368816 ) ) ;
#33618=LINE ( 'NONE', #25390, #2124 ) ;
#33619=ORIENTED_EDGE ( 'NONE', *, *, #10794, .T. ) ;
#33620=CARTESIAN_POINT ( 'NONE',  ( -20.54049170961573267, 0.000000000000000000, 4.660556269540326646 ) ) ;
#33621=VERTEX_POINT ( 'NONE', #8004 ) ;
#33622=ORIENTED_EDGE ( 'NONE', *, *, #54362, .T. ) ;
#33623=ORIENTED_EDGE ( 'NONE', *, *, #46376, .F. ) ;
#33624=EDGE_LOOP ( 'NONE', ( #3527, #44408, #7665, #15967 ) ) ;
#33625=DIRECTION ( 'NONE',  ( -0.005002170337468016433, -0.7660444431189770143, 0.6427681459581293666 ) ) ;
#33626=ORIENTED_EDGE ( 'NONE', *, *, #48172, .F. ) ;
#33627=CARTESIAN_POINT ( 'NONE',  ( -14.73683979275883438, 2.391131607591508335, 2.329931154953872152 ) ) ;
#33628=VECTOR ( 'NONE', #23760, 999.9999999999998863 ) ;
#33629=VERTEX_POINT ( 'NONE', #50849 ) ;
#33630=DIRECTION ( 'NONE',  ( 0.007781995580012663651, 0.000000000000000000, -0.9999697198139515519 ) ) ;
#33631=EDGE_CURVE ( 'NONE', #55501, #2328, #51139, .T. ) ;
#33632=ORIENTED_EDGE ( 'NONE', *, *, #17604, .F. ) ;
#33633=ORIENTED_EDGE ( 'NONE', *, *, #24229, .T. ) ;
#33634=LINE ( 'NONE', #20011, #1271 ) ;
#33635=FACE_OUTER_BOUND ( 'NONE', #17407, .T. ) ;
#33636=CARTESIAN_POINT ( 'NONE',  ( -12.09298204768809626, 0.000000000000000000, 5.834292952445442992 ) ) ;
#33637=DIRECTION ( 'NONE',  ( 0.000000000000000000, -1.000000000000000000, 0.000000000000000000 ) ) ;
#33638=FACE_OUTER_BOUND ( 'NONE', #51912, .T. ) ;
#33639=ORIENTED_EDGE ( 'NONE', *, *, #28219, .T. ) ;
#33640=EDGE_CURVE ( 'NONE', #15599, #25201, #20766, .T. ) ;
#33641=ORIENTED_EDGE ( 'NONE', *, *, #29100, .F. ) ;
#33642=VECTOR ( 'NONE', #38965, 1000.000000000000227 ) ;
#33643=CARTESIAN_POINT ( 'NONE',  ( -14.38935462099992080, 0.000000000000000000, 2.370940423672420305 ) ) ;
#33644=DIRECTION ( 'NONE',  ( 0.3313982828793700097, 0.4028455766673915694, 0.8531650599175529814 ) ) ;
#33645=UNCERTAINTY_MEASURE_WITH_UNIT (LENGTH_MEASURE( 1.000000000000000082E-05 ), #27242, 'distance_accuracy_value', 'NONE');
#33646=EDGE_CURVE ( 'NONE', #19155, #53854, #28740, .T. ) ;
#33647=EDGE_CURVE ( 'NONE', #35388, #24636, #12250, .T. ) ;
#33648=VECTOR ( 'NONE', #11870, 1000.000000000000227 ) ;
#33649=CARTESIAN_POINT ( 'NONE',  ( -12.80458192191714595, 0.000000000000000000, 11.86454056839041726 ) ) ;
#33650=PLANE ( 'NONE',  #43178 ) ;
#33651=PLANE ( 'NONE',  #29475 ) ;
#33652=DIRECTION ( 'NONE',  ( 0.5449076811759707706, 0.6444004775717708799, -0.5364919789714476250 ) ) ;
#33653=ORIENTED_EDGE ( 'NONE', *, *, #51352, .F. ) ;
#33654=DIRECTION ( 'NONE',  ( 0.005961354470445682716, -0.6427876096865404731, -0.7660212471507180654 ) ) ;
#33656=CARTESIAN_POINT ( 'NONE',  ( -28.92982233430281980, 0.000000000000000000, 7.919257187036034651 ) ) ;
#33657=EDGE_LOOP ( 'NONE', ( #26608, #52276, #13721 ) ) ;
#33658=LINE ( 'NONE', #20320, #13466 ) ;
#33659=DIRECTION ( 'NONE',  ( 0.007781995580012662783, 0.000000000000000000, -0.9999697198139514409 ) ) ;
#33660=EDGE_CURVE ( 'NONE', #6407, #35835, #36988, .T. ) ;
#33661=DIRECTION ( 'NONE',  ( -0.9999697198139514409, -0.000000000000000000, -0.007781995580013368816 ) ) ;
#33662=DIRECTION ( 'NONE',  ( 0.9999697198139515519, 0.000000000000000000, 0.007781995580013368816 ) ) ;
#33663=ADVANCED_FACE ( 'NONE', ( #29276 ), #11947, .F. ) ;
#33664=LINE ( 'NONE', #42485, #25968 ) ;
#33665=ORIENTED_EDGE ( 'NONE', *, *, #8488, .T. ) ;
#33667=ORIENTED_EDGE ( 'NONE', *, *, #44883, .T. ) ;
#33668=CARTESIAN_POINT ( 'NONE',  ( -12.55995100094445505, -3.917936722690662954, 1.635029929575186891 ) ) ;
#33670=DIRECTION ( 'NONE',  ( -0.9999697198139514409, -0.000000000000000000, -0.007781995580013368816 ) ) ;
#33671=ADVANCED_FACE ( 'NONE', ( #54284 ), #46302, .F. ) ;
#33672=VECTOR ( 'NONE', #22999, 1000.000000000000114 ) ;
#33673=VECTOR ( 'NONE', #11008, 999.9999999999998863 ) ;
#33674=LINE ( 'NONE', #11813, #34603 ) ;
#33675=CARTESIAN_POINT ( 'NONE',  ( -14.00280974873554030, 0.000000000000000000, 12.40921378708904044 ) ) ;
#33676=CARTESIAN_POINT ( 'NONE',  ( -23.33849165029409889, 0.000000000000000000, 5.946783852668351855 ) ) ;
#33677=FACE_OUTER_BOUND ( 'NONE', #46849, .T. ) ;
#33678=EDGE_CURVE ( 'NONE', #15181, #25884, #50005, .T. ) ;
#33680=CARTESIAN_POINT ( 'NONE',  ( -9.030577898858158647, 0.000000000000000000, 4.580803066637238352 ) ) ;
#33682=CARTESIAN_POINT ( 'NONE',  ( -17.00562625101985503, -3.108426967578162170, 3.387708771908411354 ) ) ;
#33683=VERTEX_POINT ( 'NONE', #20183 ) ;
#33684=CARTESIAN_POINT ( 'NONE',  ( -17.26532721389163072, 0.000000000000000000, 13.67648636611514590 ) ) ;
#33685=VERTEX_POINT ( 'NONE', #2599 ) ;
#33686=ORIENTED_EDGE ( 'NONE', *, *, #24192, .F. ) ;
#33687=VECTOR ( 'NONE', #20729, 999.9999999999998863 ) ;
#33688=VERTEX_POINT ( 'NONE', #11113 ) ;
#33689=EDGE_LOOP ( 'NONE', ( #16979, #36502, #56032, #51906 ) ) ;
#33690=ORIENTED_EDGE ( 'NONE', *, *, #4572, .T. ) ;
#33691=EDGE_LOOP ( 'NONE', ( #8007, #16590, #52682, #32169 ) ) ;
#33692=LINE ( 'NONE', #7892, #15139 ) ;
#33693=DIRECTION ( 'NONE',  ( 0.7660212471507180654, -0.6427876096865404731, 0.005961354470445141482 ) ) ;
#33694=LINE ( 'NONE', #24908, #47540 ) ;
#33695=ORIENTED_EDGE ( 'NONE', *, *, #50821, .T. ) ;
#33696=DIRECTION ( 'NONE',  ( -0.7660212471507179544, -0.6427876096865405842, -0.005961354470445141482 ) ) ;
#33697=EDGE_CURVE ( 'NONE', #6551, #55548, #45756, .T. ) ;
#33698=ORIENTED_EDGE ( 'NONE', *, *, #37443, .T. ) ;
#33699=LINE ( 'NONE', #3880, #55809 ) ;
#33702=CARTESIAN_POINT ( 'NONE',  ( -17.85999659322806821, 0.000000000000000000, 4.681416502340032260 ) ) ;
#33705=LINE ( 'NONE', #55569, #53669 ) ;
#33707=AXIS2_PLACEMENT_3D ( 'NONE', #18965, #10978, #28037 ) ;
#33709=CARTESIAN_POINT ( 'NONE',  ( -15.96710241509184058, -0.1191753592594218814, 13.13259134697452879 ) ) ;
#33710=CARTESIAN_POINT ( 'NONE',  ( -10.94028622754223967, 0.000000000000000000, 11.14038480894692995 ) ) ;
#33711=ADVANCED_FACE ( 'NONE', ( #15644 ), #32986, .F. ) ;
#33712=LINE ( 'NONE', #21221, #7921 ) ;
#33714=DIRECTION ( 'NONE',  ( 0.007781995580012662783, 0.000000000000000000, -0.9999697198139514409 ) ) ;
#33715=PLANE ( 'NONE',  #23835 ) ;
#33716=DIRECTION ( 'NONE',  ( 0.007781995580012662783, 0.000000000000000000, -0.9999697198139514409 ) ) ;
#33717=DIRECTION ( 'NONE',  ( -0.5449076811759708816, 0.6444004775717707689, 0.5364919789714475140 ) ) ;
#33719=ORIENTED_EDGE ( 'NONE', *, *, #29656, .F. ) ;
#33721=ORIENTED_EDGE ( 'NONE', *, *, #32138, .T. ) ;
#33722=CARTESIAN_POINT ( 'NONE',  ( -16.53317331066696383, 0.000000000000000000, 13.31285208727739899 ) ) ;
#33723=LINE ( 'NONE', #37420, #24197 ) ;
#33724=ADVANCED_FACE ( 'NONE', ( #41761 ), #15950, .F. ) ;
#33725=PLANE ( 'NONE',  #13262 ) ;
#33727=DIRECTION ( 'NONE',  ( 0.007781995580012663651, -3.146120232559066537E-19, -0.9999697198139514409 ) ) ;
#33728=CARTESIAN_POINT ( 'NONE',  ( -16.56099755347650770, -4.241740624735664156, 3.178841246916717100 ) ) ;
#33729=VECTOR ( 'NONE', #2496, 1000.000000000000114 ) ;
#33730=EDGE_CURVE ( 'NONE', #4731, #98, #4846, .T. ) ;
#33732=ORIENTED_EDGE ( 'NONE', *, *, #51269, .T. ) ;
#33733=CARTESIAN_POINT ( 'NONE',  ( -18.61196750743211936, -0.03228989815065406305, 4.109811145338044369 ) ) ;
#33735=LINE ( 'NONE', #47086, #16750 ) ;
#33736=DIRECTION ( 'NONE',  ( -0.005961354470445682716, -0.6427876096865404731, 0.7660212471507180654 ) ) ;
#33737=ADVANCED_FACE ( 'NONE', ( #13092 ), #43732, .F. ) ;
#33738=DIRECTION ( 'NONE',  ( -0.5364919789714478471, 0.6444004775717705469, -0.5449076811759709926 ) ) ;
#33739=LINE ( 'NONE', #3643, #51102 ) ;
#33740=LINE ( 'NONE', #30642, #19582 ) ;
#33741=DIRECTION ( 'NONE',  ( 0.000000000000000000, 0.000000000000000000, 1.000000000000000000 ) ) ;
#33742=ORIENTED_EDGE ( 'NONE', *, *, #48440, .F. ) ;
#33743=EDGE_CURVE ( 'NONE', #42918, #15204, #30424, .T. ) ;
#33744=FACE_OUTER_BOUND ( 'NONE', #30871, .T. ) ;
#33745=CARTESIAN_POINT ( 'NONE',  ( -24.26908309836554878, 0.000000000000000000, 6.108867788427308376 ) ) ;
#33747=VECTOR ( 'NONE', #40019, 999.9999999999998863 ) ;
#33748=ORIENTED_EDGE ( 'NONE', *, *, #21447, .F. ) ;
#33749=PLANE ( 'NONE',  #10166 ) ;
#33750=VECTOR ( 'NONE', #47817, 1000.000000000000227 ) ;
#33751=VECTOR ( 'NONE', #3973, 1000.000000000000114 ) ;
#33752=ORIENTED_EDGE ( 'NONE', *, *, #27440, .T. ) ;
#33753=DIRECTION ( 'NONE',  ( -0.7660212471507179544, -0.6427876096865405842, -0.005961354470445141482 ) ) ;
#33754=VECTOR ( 'NONE', #5615, 1000.000000000000114 ) ;
#33755=VERTEX_POINT ( 'NONE', #26159 ) ;
#33756=ORIENTED_EDGE ( 'NONE', *, *, #6022, .F. ) ;
#33757=VECTOR ( 'NONE', #1733, 999.9999999999998863 ) ;
#33758=ORIENTED_EDGE ( 'NONE', *, *, #41386, .T. ) ;
#33759=DIRECTION ( 'NONE',  ( -0.9999697198139514409, -0.000000000000000000, -0.007781995580013368816 ) ) ;
#33761=DIRECTION ( 'NONE',  ( 0.007781995580012663651, -3.146120232559066537E-19, -0.9999697198139514409 ) ) ;
#33762=EDGE_CURVE ( 'NONE', #54772, #48743, #34967, .T. ) ;
#33763=ORIENTED_EDGE ( 'NONE', *, *, #18990, .F. ) ;
#33764=VECTOR ( 'NONE', #104, 999.9999999999998863 ) ;
#33765=ADVANCED_FACE ( 'NONE', ( #286 ), #22169, .F. ) ;
#33766=ORIENTED_EDGE ( 'NONE', *, *, #8320, .F. ) ;
#33768=FACE_OUTER_BOUND ( 'NONE', #13360, .T. ) ;
#33769=LINE ( 'NONE', #3954, #40893 ) ;
#33770=ORIENTED_EDGE ( 'NONE', *, *, #40358, .F. ) ;
#33771=ADVANCED_FACE ( 'NONE', ( #4009 ), #4311, .F. ) ;
#33772=FACE_OUTER_BOUND ( 'NONE', #6547, .T. ) ;
#33773=CARTESIAN_POINT ( 'NONE',  ( -28.93060053386082231, -0.1191753592594197858, 8.019254159017428663 ) ) ;
#33774=ORIENTED_EDGE ( 'NONE', *, *, #20069, .F. ) ;
#33775=LINE ( 'NONE', #33508, #55701 ) ;
#33776=DIRECTION ( 'NONE',  ( 0.5364919789714477361, 0.6444004775717706579, 0.5449076811759711036 ) ) ;
#33777=ADVANCED_FACE ( 'NONE', ( #13392 ), #34656, .F. ) ;
#33778=ADVANCED_FACE ( 'NONE', ( #51977 ), #12803, .F. ) ;
#33779=EDGE_CURVE ( 'NONE', #45468, #19093, #26413, .T. ) ;
#33780=ORIENTED_EDGE ( 'NONE', *, *, #9277, .F. ) ;
#33781=LINE ( 'NONE', #32946, #33150 ) ;
#33782=VECTOR ( 'NONE', #24647, 1000.000000000000227 ) ;
#33783=CARTESIAN_POINT ( 'NONE',  ( -20.65957321758616416, 2.229229656569007734, 4.635687473917941226 ) ) ;
#33784=ORIENTED_EDGE ( 'NONE', *, *, #20249, .F. ) ;
#33785=DIRECTION ( 'NONE',  ( -0.6427681459581293666, -0.7660444431189770143, -0.005002170337467561935 ) ) ;
#33786=PLANE ( 'NONE',  #7505 ) ;
#33787=LINE ( 'NONE', #51414, #20293 ) ;
#33788=VECTOR ( 'NONE', #41522, 1000.000000000000227 ) ;
#33789=CARTESIAN_POINT ( 'NONE',  ( -15.47117689834755261, -2.946525016555661125, 2.796842053098518743 ) ) ;
#33790=EDGE_LOOP ( 'NONE', ( #3537, #20549, #341, #9578 ) ) ;
#33791=AXIS2_PLACEMENT_3D ( 'NONE', #45097, #5611, #6201 ) ;
#33792=VECTOR ( 'NONE', #26016, 1000.000000000000227 ) ;
#33793=LINE ( 'NONE', #12219, #18317 ) ;
#33795=DIRECTION ( 'NONE',  ( -0.005961354470445682716, -0.6427876096865404731, 0.7660212471507180654 ) ) ;
#33796=EDGE_CURVE ( 'NONE', #36235, #18922, #12543, .T. ) ;
#33797=CARTESIAN_POINT ( 'NONE',  ( -16.06709938707323460, 0.000000000000000000, 13.13181314741652628 ) ) ;
#33798=DIRECTION ( 'NONE',  ( -0.005002170337468016433, -0.7660444431189770143, 0.6427681459581293666 ) ) ;
#33799=CARTESIAN_POINT ( 'NONE',  ( -15.60102546347950536, 0.000000000000000000, 12.95077420755565356 ) ) ;
#33800=EDGE_CURVE ( 'NONE', #32412, #47173, #51443, .T. ) ;
#33801=VECTOR ( 'NONE', #27333, 999.9999999999998863 ) ;
#33802=LINE ( 'NONE', #42601, #51226 ) ;
#33803=AXIS2_PLACEMENT_3D ( 'NONE', #46215, #15555, #33193 ) ;
#33804=ORIENTED_EDGE ( 'NONE', *, *, #54330, .T. ) ;
#33806=ADVANCED_FACE ( 'NONE', ( #8259 ), #21334, .F. ) ;
#33808=ORIENTED_EDGE ( 'NONE', *, *, #4520, .F. ) ;
#33809=CARTESIAN_POINT ( 'NONE',  ( -21.84967550273626102, 5.305366725996514710, 4.999818739653546729 ) ) ;
#33810=FACE_OUTER_BOUND ( 'NONE', #21883, .T. ) ;
#33812=FACE_OUTER_BOUND ( 'NONE', #41566, .T. ) ;
#33813=VECTOR ( 'NONE', #40297, 999.9999999999998863 ) ;
#33814=VECTOR ( 'NONE', #36500, 999.9999999999998863 ) ;
#33815=CARTESIAN_POINT ( 'NONE',  ( -15.88130887279446490, 0.000000000000000000, 3.050160814894388839 ) ) ;
#33817=VERTEX_POINT ( 'NONE', #15550 ) ;
#33818=EDGE_LOOP ( 'NONE', ( #2836, #26416, #40224, #30224 ) ) ;
#33819=CARTESIAN_POINT ( 'NONE',  ( -25.20123094555300369, 0.000000000000000000, 6.470945668149052032 ) ) ;
#33820=FACE_OUTER_BOUND ( 'NONE', #737, .T. ) ;
#33821=ORIENTED_EDGE ( 'NONE', *, *, #11219, .F. ) ;
#33822=AXIS2_PLACEMENT_3D ( 'NONE', #52771, #46633, #22435 ) ;
#33824=ORIENTED_EDGE ( 'NONE', *, *, #22370, .T. ) ;
#33825=DIRECTION ( 'NONE',  ( 0.007781995580012663651, -3.146120232559066537E-19, -0.9999697198139514409 ) ) ;
#33827=ORIENTED_EDGE ( 'NONE', *, *, #33598, .F. ) ;
#33828=LINE ( 'NONE', #16498, #51940 ) ;
#33829=ORIENTED_EDGE ( 'NONE', *, *, #46405, .T. ) ;
#33830=ORIENTED_EDGE ( 'NONE', *, *, #14377, .T. ) ;
#33831=ORIENTED_EDGE ( 'NONE', *, *, #37169, .F. ) ;
#33832=CARTESIAN_POINT ( 'NONE',  ( -11.87243407472968926, 0.000000000000000000, 11.50246268866867361 ) ) ;
#33833=VECTOR ( 'NONE', #38942, 999.9999999999998863 ) ;
#33834=LINE ( 'NONE', #51152, #24130 ) ;
#33835=CARTESIAN_POINT ( 'NONE',  ( -19.05259568539925752, 0.000000000000000000, 4.502809406857032570 ) ) ;
#33836=VECTOR ( 'NONE', #15298, 1000.000000000000227 ) ;
#33837=VECTOR ( 'NONE', #28213, 1000.000000000000227 ) ;
#33838=CARTESIAN_POINT ( 'NONE',  ( -21.47263955680318404, 0.000000000000000000, 5.022634149262071190 ) ) ;
#33839=ORIENTED_EDGE ( 'NONE', *, *, #46279, .F. ) ;
#33841=VECTOR ( 'NONE', #23912, 1000.000000000000227 ) ;
#33842=ORIENTED_EDGE ( 'NONE', *, *, #53130, .T. ) ;
#33843=FACE_OUTER_BOUND ( 'NONE', #37069, .T. ) ;
#33844=AXIS2_PLACEMENT_3D ( 'NONE', #26211, #347, #9152 ) ;
#33845=DIRECTION ( 'NONE',  ( -0.9999697198139514409, -0.000000000000000000, -0.007781995580013368816 ) ) ;
#33846=ORIENTED_EDGE ( 'NONE', *, *, #29779, .F. ) ;
#33848=ORIENTED_EDGE ( 'NONE', *, *, #55848, .T. ) ;
#33850=FACE_OUTER_BOUND ( 'NONE', #37765, .T. ) ;
#33851=EDGE_CURVE ( 'NONE', #42922, #45468, #41947, .T. ) ;
#33852=EDGE_CURVE ( 'NONE', #12574, #30915, #29479, .T. ) ;
#33853=ORIENTED_EDGE ( 'NONE', *, *, #41459, .T. ) ;
#33855=EDGE_LOOP ( 'NONE', ( #42561, #45993, #41563, #6003 ) ) ;
#33856=ADVANCED_FACE ( 'NONE', ( #3626 ), #20931, .F. ) ;
#33857=VECTOR ( 'NONE', #25141, 999.9999999999998863 ) ;
#33858=DIRECTION ( 'NONE',  ( 0.000000000000000000, -0.000000000000000000, -1.000000000000000000 ) ) ;
#33859=DIRECTION ( 'NONE',  ( -0.9999697198139514409, -0.000000000000000000, -0.007781995580013368816 ) ) ;
#33860=ORIENTED_EDGE ( 'NONE', *, *, #26125, .T. ) ;
#33861=LINE ( 'NONE', #33575, #49535 ) ;
#33862=DIRECTION ( 'NONE',  ( -0.5449076811759708816, 0.6444004775717707689, 0.5364919789714475140 ) ) ;
#33863=CARTESIAN_POINT ( 'NONE',  ( -27.99767448711536133, 0.000000000000000000, 7.557179307314289218 ) ) ;
#33864=DIRECTION ( 'NONE',  ( 0.007781995580012662783, 0.000000000000000000, -0.9999697198139514409 ) ) ;
#33865=VERTEX_POINT ( 'NONE', #54734 ) ;
#33866=VECTOR ( 'NONE', #24486, 1000.000000000000227 ) ;
#33867=ORIENTED_EDGE ( 'NONE', *, *, #38870, .F. ) ;
#33868=DIRECTION ( 'NONE',  ( 0.007781995580012662783, 0.000000000000000000, -0.9999697198139514409 ) ) ;
#33869=CARTESIAN_POINT ( 'NONE',  ( -19.59569683186026268, 0.000000000000000000, 14.58168106541950948 ) ) ;
#33870=VECTOR ( 'NONE', #26484, 1000.000000000000114 ) ;
#33871=DIRECTION ( 'NONE',  ( -0.5449076811759708816, 0.6444004775717707689, 0.5364919789714475140 ) ) ;
#33872=CARTESIAN_POINT ( 'NONE',  ( -11.30636317915456779, -0.1191753592594197858, 11.32220194836580340 ) ) ;
#33873=FACE_OUTER_BOUND ( 'NONE', #44944, .T. ) ;
#33874=EDGE_CURVE ( 'NONE', #13391, #40480, #12456, .T. ) ;
#33875=PLANE ( 'NONE',  #33114 ) ;
#33876=VERTEX_POINT ( 'NONE', #38256 ) ;
#33877=LINE ( 'NONE', #29649, #14128 ) ;
#33878=EDGE_CURVE ( 'NONE', #14582, #2799, #33453, .T. ) ;
#33879=DIRECTION ( 'NONE',  ( 0.7660212471507180654, -0.6427876096865404731, 0.005961354470445141482 ) ) ;
#33880=ORIENTED_EDGE ( 'NONE', *, *, #37258, .F. ) ;
#33881=VECTOR ( 'NONE', #8342, 1000.000000000000227 ) ;
#33882=LINE ( 'NONE', #51202, #23186 ) ;
#33883=ORIENTED_EDGE ( 'NONE', *, *, #24107, .T. ) ;
#33885=AXIS2_PLACEMENT_3D ( 'NONE', #4664, #43833, #47843 ) ;
#33886=DIRECTION ( 'NONE',  ( -0.005961354470445682716, -0.6427876096865404731, 0.7660212471507180654 ) ) ;
#33887=CARTESIAN_POINT ( 'NONE',  ( -9.342070512798265725, 0.000000000000000000, 10.59882438848031505 ) ) ;
#33888=EDGE_CURVE ( 'NONE', #50295, #30246, #3899, .T. ) ;
#33889=DIRECTION ( 'NONE',  ( 0.9999697198139515519, 0.000000000000000000, 0.007781995580013368816 ) ) ;
#33890=CARTESIAN_POINT ( 'NONE',  ( -23.33849165029409889, 0.000000000000000000, 5.946783852668351855 ) ) ;
#33891=EDGE_CURVE ( 'NONE', #43988, #43441, #24936, .T. ) ;
#33893=VERTEX_POINT ( 'NONE', #16391 ) ;
#33894=AXIS2_PLACEMENT_3D ( 'NONE', #32085, #24387, #2782 ) ;
#33895=VECTOR ( 'NONE', #29194, 999.9999999999998863 ) ;
#33896=VERTEX_POINT ( 'NONE', #47072 ) ;
#33897=CARTESIAN_POINT ( 'NONE',  ( -22.40478740399063895, 0.000000000000000000, 5.384712028983816623 ) ) ;
#33898=FACE_OUTER_BOUND ( 'NONE', #7719, .T. ) ;
#33899=DIRECTION ( 'NONE',  ( 0.007781995580012663651, -3.146120232559066537E-19, -0.9999697198139514409 ) ) ;
#33900=CARTESIAN_POINT ( 'NONE',  ( -20.00186950356889426, -0.008498251296377924008, 6.149207326778157956 ) ) ;
#33901=DIRECTION ( 'NONE',  ( 0.5449076811759707706, 0.6444004775717708799, -0.5364919789714476250 ) ) ;
#33902=DIRECTION ( 'NONE',  ( 0.007781995580012663651, 0.000000000000000000, -0.9999697198139515519 ) ) ;
#33903=ORIENTED_EDGE ( 'NONE', *, *, #51997, .T. ) ;
#33904=CARTESIAN_POINT ( 'NONE',  ( -10.94028622754223967, 0.000000000000000000, 11.14038480894692995 ) ) ;
#33905=DIRECTION ( 'NONE',  ( 0.000000000000000000, -0.000000000000000000, -1.000000000000000000 ) ) ;
#33906=DIRECTION ( 'NONE',  ( 0.6427681459581294776, -0.7660444431189769032, 0.005002170337467562802 ) ) ;
#33907=ORIENTED_EDGE ( 'NONE', *, *, #17717, .F. ) ;
#33908=VECTOR ( 'NONE', #15154, 1000.000000000000227 ) ;
#33909=LINE ( 'NONE', #7229, #41060 ) ;
#33910=DIRECTION ( 'NONE',  ( 0.000000000000000000, -0.000000000000000000, -1.000000000000000000 ) ) ;
#33911=VECTOR ( 'NONE', #28631, 999.9999999999998863 ) ;
#33912=LINE ( 'NONE', #29684, #19356 ) ;
#33913=VERTEX_POINT ( 'NONE', #50198 ) ;
#33914=DIRECTION ( 'NONE',  ( 0.5449076811759707706, 0.6444004775717708799, -0.5364919789714476250 ) ) ;
#33915=AXIS2_PLACEMENT_3D ( 'NONE', #2760, #20085, #11598 ) ;
#33917=ORIENTED_EDGE ( 'NONE', *, *, #14467, .F. ) ;
#33918=ORIENTED_EDGE ( 'NONE', *, *, #9104, .F. ) ;
#33919=EDGE_LOOP ( 'NONE', ( #26248, #14465, #27338, #47251 ) ) ;
#33920=VECTOR ( 'NONE', #46915, 1000.000000000000227 ) ;
#33921=PLANE ( 'NONE',  #37500 ) ;
#33922=ORIENTED_EDGE ( 'NONE', *, *, #13363, .T. ) ;
#33923=FACE_OUTER_BOUND ( 'NONE', #43360, .T. ) ;
#33925=ADVANCED_FACE ( 'NONE', ( #33186 ), #25485, .F. ) ;
#33926=VERTEX_POINT ( 'NONE', #29774 ) ;
#33927=CARTESIAN_POINT ( 'NONE',  ( -12.15929124516513227, -0.1191753592594198830, 1.504708075227162656 ) ) ;
#33928=ORIENTED_EDGE ( 'NONE', *, *, #54801, .F. ) ;
#33929=ORIENTED_EDGE ( 'NONE', *, *, #10071, .T. ) ;
#33930=EDGE_CURVE ( 'NONE', #19674, #34361, #8177, .T. ) ;
#33931=EDGE_CURVE ( 'NONE', #42035, #3660, #20682, .T. ) ;
#33932=AXIS2_PLACEMENT_3D ( 'NONE', #37951, #25439, #21178 ) ;
#33933=VECTOR ( 'NONE', #20040, 1000.000000000000000 ) ;
#33934=CARTESIAN_POINT ( 'NONE',  ( -19.25577499705407902, 1.095915999411505082, 6.159502914972740939 ) ) ;
#33935=LINE ( 'NONE', #4667, #3272 ) ;
#33936=FACE_OUTER_BOUND ( 'NONE', #10937, .T. ) ;
#33937=CARTESIAN_POINT ( 'NONE',  ( -14.39760455647254744, 0.000000000000000000, 3.431039414763832340 ) ) ;
#33938=DIRECTION ( 'NONE',  ( -0.7660212471507179544, -0.6427876096865405842, -0.005961354470445141482 ) ) ;
#33939=ORIENTED_EDGE ( 'NONE', *, *, #20276, .T. ) ;
#33940=EDGE_LOOP ( 'NONE', ( #2643, #32871, #50097, #22041 ) ) ;
#33941=PLANE ( 'NONE',  #47551 ) ;
#33942=LINE ( 'NONE', #43324, #47529 ) ;
#33943=FACE_OUTER_BOUND ( 'NONE', #42155, .T. ) ;
#33944=VECTOR ( 'NONE', #28395, 1000.000000000000114 ) ;
#33945=LINE ( 'NONE', #51268, #53013 ) ;
#33946=LINE ( 'NONE', #24030, #50340 ) ;
#33947=CARTESIAN_POINT ( 'NONE',  ( -15.09384998583453097, 0.000000000000000000, 7.488273839715230196 ) ) ;
#33948=VERTEX_POINT ( 'NONE', #16689 ) ;
#33949=CARTESIAN_POINT ( 'NONE',  ( -12.78951571262592068, -1.975113310420658852, 1.786186898291378000 ) ) ;
#33950=DIRECTION ( 'NONE',  ( -0.7660212471507179544, -0.6427876096865405842, -0.005961354470445141482 ) ) ;
#33951=AXIS2_PLACEMENT_3D ( 'NONE', #54328, #15421, #29044 ) ;
#33952=ORIENTED_EDGE ( 'NONE', *, *, #10080, .T. ) ;
#33953=CARTESIAN_POINT ( 'NONE',  ( -28.92982233430281980, 0.000000000000000000, 7.919257187036034651 ) ) ;
#33954=CARTESIAN_POINT ( 'NONE',  ( -18.19747506107908563, 0.000000000000000000, 14.03856424583689311 ) ) ;
#33955=DIRECTION ( 'NONE',  ( -0.7660212471507179544, -0.6427876096865405842, -0.005961354470445141482 ) ) ;
#33956=LINE ( 'NONE', #56107, #44958 ) ;
#33957=EDGE_CURVE ( 'NONE', #46531, #21352, #50503, .T. ) ;
#33958=DIRECTION ( 'NONE',  ( 0.007781995580012663651, -3.146120232559066537E-19, -0.9999697198139514409 ) ) ;
#33959=VERTEX_POINT ( 'NONE', #42793 ) ;
#33960=VECTOR ( 'NONE', #5327, 1000.000000000000227 ) ;
#33961=EDGE_CURVE ( 'NONE', #48671, #31756, #37997, .T. ) ;
#33962=ORIENTED_EDGE ( 'NONE', *, *, #5655, .T. ) ;
#33963=VECTOR ( 'NONE', #19528, 999.9999999999998863 ) ;
#33964=CARTESIAN_POINT ( 'NONE',  ( -17.43427879107165879, 0.000000000000000000, 9.686052500421766354 ) ) ;
#33966=DIRECTION ( 'NONE',  ( 0.6427681459581294776, -0.7660444431189769032, 0.005002170337467562802 ) ) ;
#33967=EDGE_CURVE ( 'NONE', #41210, #51656, #28640, .T. ) ;
#33968=VECTOR ( 'NONE', #5048, 999.9999999999998863 ) ;
#33969=DIRECTION ( 'NONE',  ( -0.9999697198139514409, -0.000000000000000000, -0.007781995580013368816 ) ) ;
#33970=ADVANCED_FACE ( 'NONE', ( #24365 ), #41675, .F. ) ;
#33971=CARTESIAN_POINT ( 'NONE',  ( -2.881839257824877265, -5.376589517215482950, -2.098969340251471305 ) ) ;
#33972=LINE ( 'NONE', #3583, #13780 ) ;
#33973=DIRECTION ( 'NONE',  ( -0.5449076811759708816, 0.6444004775717707689, 0.5364919789714475140 ) ) ;
#33974=VECTOR ( 'NONE', #19727, 1000.000000000000000 ) ;
#33975=PLANE ( 'NONE',  #11450 ) ;
#33976=VECTOR ( 'NONE', #46516, 1000.000000000000227 ) ;
#33977=CARTESIAN_POINT ( 'NONE',  ( -15.88130887279446490, 0.000000000000000000, 3.050160814894388839 ) ) ;
#33978=DIRECTION ( 'NONE',  ( -0.3313982828793700097, 0.4028455766673915694, -0.8531650599175529814 ) ) ;
#33981=EDGE_LOOP ( 'NONE', ( #22237, #46170, #3338, #14962 ) ) ;
#33982=ORIENTED_EDGE ( 'NONE', *, *, #38926, .F. ) ;
#33983=ADVANCED_FACE ( 'NONE', ( #37413 ), #28917, .F. ) ;
#33984=VECTOR ( 'NONE', #28034, 1000.000000000000227 ) ;
#33985=ORIENTED_EDGE ( 'NONE', *, *, #51672, .T. ) ;
#33986=ORIENTED_EDGE ( 'NONE', *, *, #3264, .T. ) ;
#33987=ORIENTED_EDGE ( 'NONE', *, *, #54952, .T. ) ;
#33988=AXIS2_PLACEMENT_3D ( 'NONE', #43756, #40062, #4872 ) ;
#33989=ORIENTED_EDGE ( 'NONE', *, *, #37366, .F. ) ;
#33990=LINE ( 'NONE', #20061, #40522 ) ;
#33991=DIRECTION ( 'NONE',  ( -0.9999697198139514409, -0.000000000000000000, -0.007781995580013368816 ) ) ;
#33992=EDGE_CURVE ( 'NONE', #35868, #26894, #30319, .T. ) ;
#33993=LINE ( 'NONE', #12431, #4940 ) ;
#33994=AXIS2_PLACEMENT_3D ( 'NONE', #40079, #49156, #44074 ) ;
#33995=VERTEX_POINT ( 'NONE', #13557 ) ;
#33996=EDGE_CURVE ( 'NONE', #45628, #5924, #34308, .T. ) ;
#33997=FACE_OUTER_BOUND ( 'NONE', #54398, .T. ) ;
#33998=ORIENTED_EDGE ( 'NONE', *, *, #10902, .F. ) ;
#33999=VECTOR ( 'NONE', #48826, 999.9999999999998863 ) ;
#34000=DIRECTION ( 'NONE',  ( -0.5449076811759708816, 0.6444004775717707689, 0.5364919789714475140 ) ) ;
#34001=EDGE_LOOP ( 'NONE', ( #3176, #44598, #37624, #33228 ) ) ;
#34002=EDGE_CURVE ( 'NONE', #8988, #26117, #26914, .T. ) ;
#34003=AXIS2_PLACEMENT_3D ( 'NONE', #16592, #16310, #51536 ) ;
#34004=AXIS2_PLACEMENT_3D ( 'NONE', #38340, #32966, #16769 ) ;
#34005=CARTESIAN_POINT ( 'NONE',  ( -21.47341775636118655, -0.1191753592594197858, 5.122631121243466090 ) ) ;
#34006=VECTOR ( 'NONE', #25461, 1000.000000000000227 ) ;
#34007=CARTESIAN_POINT ( 'NONE',  ( -13.06197087640816434, -2.298917212465660054, 1.881686696745927589 ) ) ;
#34008=CARTESIAN_POINT ( 'NONE',  ( -9.607175450607181588, -0.1191753592594187727, 2.260320404213849610 ) ) ;
#34009=ORIENTED_EDGE ( 'NONE', *, *, #22885, .T. ) ;
#34010=FACE_OUTER_BOUND ( 'NONE', #16429, .T. ) ;
#34011=ORIENTED_EDGE ( 'NONE', *, *, #31203, .T. ) ;
#34012=AXIS2_PLACEMENT_3D ( 'NONE', #34707, #26203, #43506 ) ;
#34013=FACE_OUTER_BOUND ( 'NONE', #48454, .T. ) ;
#34014=CARTESIAN_POINT ( 'NONE',  ( -14.46888367232926420, 0.000000000000000000, 12.59025272694991315 ) ) ;
#34015=EDGE_CURVE ( 'NONE', #51439, #21119, #31149, .T. ) ;
#34016=VECTOR ( 'NONE', #53398, 1000.000000000000114 ) ;
#34017=LINE ( 'NONE', #38552, #39664 ) ;
#34018=VECTOR ( 'NONE', #23135, 1000.000000000000227 ) ;
#34019=CARTESIAN_POINT ( 'NONE',  ( -14.01545677930355183, 0.000000000000000000, 2.126011111488108174 ) ) ;
#34020=CARTESIAN_POINT ( 'NONE',  ( 2.072287782118878319, 0.000000000000000000, -2.950529333540147015 ) ) ;
#34021=CARTESIAN_POINT ( 'NONE',  ( -22.40556560354864146, -0.1191753592594197858, 5.484709000965211523 ) ) ;
#34022=CARTESIAN_POINT ( 'NONE',  ( -24.26986129792355129, -0.1191753592594197858, 6.208864760408702388 ) ) ;
#34023=CARTESIAN_POINT ( 'NONE',  ( -14.88235982785061218, 0.000000000000000000, 6.012591425800175138 ) ) ;
#34024=ORIENTED_EDGE ( 'NONE', *, *, #40287, .T. ) ;
#34025=CARTESIAN_POINT ( 'NONE',  ( 2.072287782118878319, 0.000000000000000000, -2.950529333540147015 ) ) ;
#34026=ORIENTED_EDGE ( 'NONE', *, *, #18702, .F. ) ;
#34027=DIRECTION ( 'NONE',  ( 0.9999697198139515519, 0.000000000000000000, 0.007781995580013368816 ) ) ;
#34028=DIRECTION ( 'NONE',  ( -0.5364919789714478471, 0.6444004775717705469, -0.5449076811759709926 ) ) ;
#34029=CARTESIAN_POINT ( 'NONE',  ( -27.06630483948590893, -0.1191753592594197858, 7.295098399573937797 ) ) ;
#34030=DIRECTION ( 'NONE',  ( 0.005961354470445682716, -0.6427876096865404731, -0.7660212471507180654 ) ) ;
#34031=CARTESIAN_POINT ( 'NONE',  ( -15.56555264407546346, 0.000000000000000000, 8.392593093757724887 ) ) ;
#34032=VECTOR ( 'NONE', #53270, 1000.000000000000227 ) ;
#34033=CARTESIAN_POINT ( 'NONE',  ( -16.89925026227929195, -0.1191753592594197858, 13.49466922669627422 ) ) ;
#34035=VECTOR ( 'NONE', #55025, 1000.000000000000227 ) ;
#34036=VERTEX_POINT ( 'NONE', #56158 ) ;
#34038=CARTESIAN_POINT ( 'NONE',  ( -13.40764798327444574, 3.524445264749008988, 7.873522038848314253 ) ) ;
#34039=LINE ( 'NONE', #7625, #10987 ) ;
#34041=LINE ( 'NONE', #54759, #23702 ) ;
#34042=ADVANCED_FACE ( 'NONE', ( #30621 ), #52460, .F. ) ;
#34043=AXIS2_PLACEMENT_3D ( 'NONE', #42531, #42253, #16388 ) ;
#34044=PLANE ( 'NONE',  #22099 ) ;
#34045=PLANE ( 'NONE',  #5082 ) ;
#34046=LINE ( 'NONE', #51371, #218 ) ;
#34047=ORIENTED_EDGE ( 'NONE', *, *, #40064, .F. ) ;
#34048=PLANE ( 'NONE',  #35809 ) ;
#34049=VECTOR ( 'NONE', #32121, 999.9999999999998863 ) ;
#34050=CARTESIAN_POINT ( 'NONE',  ( 2.072287782118878319, 0.000000000000000000, -2.950529333540147015 ) ) ;
#34051=VECTOR ( 'NONE', #19996, 1000.000000000000227 ) ;
#34052=VERTEX_POINT ( 'NONE', #4215 ) ;
#34053=EDGE_LOOP ( 'NONE', ( #40674, #6645, #4364, #45497 ) ) ;
#34054=DIRECTION ( 'NONE',  ( 0.000000000000000000, 0.000000000000000000, 1.000000000000000000 ) ) ;
#34055=VECTOR ( 'NONE', #19203, 1000.000000000000227 ) ;
#34056=EDGE_CURVE ( 'NONE', #28808, #42382, #39107, .T. ) ;
#34057=ORIENTED_EDGE ( 'NONE', *, *, #42752, .T. ) ;
#34058=VECTOR ( 'NONE', #26119, 1000.000000000000227 ) ;
#34059=EDGE_CURVE ( 'NONE', #14066, #34341, #26077, .T. ) ;
#34060=ADVANCED_FACE ( 'NONE', ( #34863 ), #48174, .F. ) ;
#34061=AXIS2_PLACEMENT_3D ( 'NONE', #29140, #42218, #37961 ) ;
#34062=ORIENTED_EDGE ( 'NONE', *, *, #21050, .F. ) ;
#34063=VECTOR ( 'NONE', #41561, 1000.000000000000227 ) ;
#34064=ORIENTED_EDGE ( 'NONE', *, *, #3977, .T. ) ;
#34065=ORIENTED_EDGE ( 'NONE', *, *, #29963, .T. ) ;
#34068=EDGE_CURVE ( 'NONE', #56109, #8019, #16989, .T. ) ;
#34069=DIRECTION ( 'NONE',  ( 0.007781995580012662783, 0.000000000000000000, -0.9999697198139514409 ) ) ;
#34070=EDGE_CURVE ( 'NONE', #40934, #55582, #12714, .T. ) ;
#34071=ORIENTED_EDGE ( 'NONE', *, *, #26061, .T. ) ;
#34072=ORIENTED_EDGE ( 'NONE', *, *, #23256, .F. ) ;
#34073=EDGE_CURVE ( 'NONE', #33398, #20973, #26606, .T. ) ;
#34074=VECTOR ( 'NONE', #10010, 1000.000000000000000 ) ;
#34075=PLANE ( 'NONE',  #5791 ) ;
#34076=PLANE ( 'NONE',  #49048 ) ;
#34078=ORIENTED_EDGE ( 'NONE', *, *, #42450, .F. ) ;
#34079=LINE ( 'NONE', #51657, #43662 ) ;
#34080=CARTESIAN_POINT ( 'NONE',  ( -25.20200914511100265, -0.1191753592594197858, 6.570942640130446932 ) ) ;
#34081=EDGE_LOOP ( 'NONE', ( #38664, #39500, #19474, #36256 ) ) ;
#34082=AXIS2_PLACEMENT_3D ( 'NONE', #4366, #25367, #16549 ) ;
#34083=CARTESIAN_POINT ( 'NONE',  ( -10.66326506071217040, 0.000000000000000000, 1.244108489361323677 ) ) ;
#34085=ORIENTED_EDGE ( 'NONE', *, *, #2822, .T. ) ;
#34086=CARTESIAN_POINT ( 'NONE',  ( -18.66354898467281132, 0.000000000000000000, 14.21960318569776582 ) ) ;
#34087=AXIS2_PLACEMENT_3D ( 'NONE', #6859, #41494, #40917 ) ;
#34088=EDGE_CURVE ( 'NONE', #10254, #55582, #17531, .T. ) ;
#34089=LINE ( 'NONE', #26376, #51767 ) ;
#34090=VECTOR ( 'NONE', #47782, 1000.000000000000227 ) ;
#34091=VERTEX_POINT ( 'NONE', #47641 ) ;
#34092=CARTESIAN_POINT ( 'NONE',  ( -11.20636620717317378, 0.000000000000000000, 11.32298014792380414 ) ) ;
#34093=DIRECTION ( 'NONE',  ( 0.007781995580012663651, 0.000000000000000000, -0.9999697198139515519 ) ) ;
#34094=DIRECTION ( 'NONE',  ( -0.8531650599175529814, -0.4028455766673920135, 0.3313982828793697877 ) ) ;
#34095=DIRECTION ( 'NONE',  ( 0.7660212471507180654, -0.6427876096865404731, 0.005961354470445141482 ) ) ;
#34096=EDGE_LOOP ( 'NONE', ( #25374, #10002, #9834, #46466 ) ) ;
#34097=AXIS2_PLACEMENT_3D ( 'NONE', #52112, #48121, #22312 ) ;
#34098=VECTOR ( 'NONE', #49657, 1000.000000000000000 ) ;
#34099=PLANE ( 'NONE',  #42789 ) ;
#34100=PLANE ( 'NONE',  #52316 ) ;
#34101=LINE ( 'NONE', #43185, #4035 ) ;
#34102=FACE_OUTER_BOUND ( 'NONE', #35574, .T. ) ;
#34103=CARTESIAN_POINT ( 'NONE',  ( -16.99924723426068951, 0.000000000000000000, 13.49389102713827171 ) ) ;
#34104=FACE_OUTER_BOUND ( 'NONE', #52402, .T. ) ;
#34105=VECTOR ( 'NONE', #19304, 999.9999999999998863 ) ;
#34106=AXIS2_PLACEMENT_3D ( 'NONE', #29977, #39055, #52660 ) ;
#34108=ORIENTED_EDGE ( 'NONE', *, *, #53683, .F. ) ;
#34110=ORIENTED_EDGE ( 'NONE', *, *, #10719, .F. ) ;
#34111=LINE ( 'NONE', #21320, #20260 ) ;
#34112=CARTESIAN_POINT ( 'NONE',  ( -19.26121178987789051, 0.000000000000000000, 5.609182117514321497 ) ) ;
#34113=EDGE_CURVE ( 'NONE', #21256, #42731, #497, .T. ) ;
#34114=DIRECTION ( 'NONE',  ( -0.005002170337468016433, -0.7660444431189770143, 0.6427681459581293666 ) ) ;
#34115=EDGE_CURVE ( 'NONE', #37525, #9203, #51879, .T. ) ;
#34116=LINE ( 'NONE', #3997, #36032 ) ;
#34117=LINE ( 'NONE', #4303, #39264 ) ;
#34118=VECTOR ( 'NONE', #49114, 1000.000000000000227 ) ;
#34119=ORIENTED_EDGE ( 'NONE', *, *, #32173, .T. ) ;
#34120=ORIENTED_EDGE ( 'NONE', *, *, #53262, .T. ) ;
#34121=CARTESIAN_POINT ( 'NONE',  ( -17.46532115785441519, 0.000000000000000000, 13.67492996699914265 ) ) ;
#34122=DIRECTION ( 'NONE',  ( -0.8531650599175529814, -0.4028455766673920135, 0.3313982828793697877 ) ) ;
#34123=EDGE_LOOP ( 'NONE', ( #16432, #21873, #28467, #7238 ) ) ;
#34124=AXIS2_PLACEMENT_3D ( 'NONE', #6640, #49539, #32746 ) ;
#34125=ADVANCED_FACE ( 'NONE', ( #43386 ), #13292, .F. ) ;
#34126=ADVANCED_FACE ( 'NONE', ( #17832 ), #35163, .F. ) ;
#34127=EDGE_CURVE ( 'NONE', #3505, #3254, #32294, .T. ) ;
#34128=DIRECTION ( 'NONE',  ( -0.3620778797217457656, 0.000000000000000000, -0.9321478471874539151 ) ) ;
#34129=ORIENTED_EDGE ( 'NONE', *, *, #20665, .T. ) ;
#34130=LINE ( 'NONE', #46906, #15005 ) ;
#34132=ORIENTED_EDGE ( 'NONE', *, *, #21933, .T. ) ;
#34133=DIRECTION ( 'NONE',  ( 0.007781995580012663651, -3.146120232559066537E-19, -0.9999697198139514409 ) ) ;
#34134=ADVANCED_FACE ( 'NONE', ( #41063 ), #6179, .F. ) ;
#34135=AXIS2_PLACEMENT_3D ( 'NONE', #43446, #17055, #261 ) ;
#34136=ORIENTED_EDGE ( 'NONE', *, *, #18421, .T. ) ;
#34138=VERTEX_POINT ( 'NONE', #1618 ) ;
#34139=CARTESIAN_POINT ( 'NONE',  ( -12.31313304499984440, 4.495856970884013037, 1.321329386160589703 ) ) ;
#34140=DIRECTION ( 'NONE',  ( 0.007781995580012663651, 0.000000000000000000, -0.9999697198139515519 ) ) ;
#34141=FACE_OUTER_BOUND ( 'NONE', #22223, .T. ) ;
#34142=VECTOR ( 'NONE', #21139, 999.9999999999998863 ) ;
#34143=VECTOR ( 'NONE', #38117, 1000.000000000000227 ) ;
#34144=CARTESIAN_POINT ( 'NONE',  ( -20.54204810873173415, 0.000000000000000000, 4.860550213503115558 ) ) ;
#34145=EDGE_CURVE ( 'NONE', #17633, #36664, #28022, .T. ) ;
#34146=ORIENTED_EDGE ( 'NONE', *, *, #53096, .T. ) ;
#34147=EDGE_LOOP ( 'NONE', ( #52360, #49431, #13978, #24324 ) ) ;
#34148=VECTOR ( 'NONE', #45356, 1000.000000000000227 ) ;
#34149=EDGE_CURVE ( 'NONE', #608, #50606, #27173, .T. ) ;
#34150=EDGE_LOOP ( 'NONE', ( #35194, #49762, #33507, #1214 ) ) ;
#34151=PLANE ( 'NONE',  #26794 ) ;
#34152=DIRECTION ( 'NONE',  ( 0.9999697198139515519, 0.000000000000000000, 0.007781995580013368816 ) ) ;
#34153=EDGE_CURVE ( 'NONE', #11770, #52378, #53564, .T. ) ;
#34154=ORIENTED_EDGE ( 'NONE', *, *, #49899, .F. ) ;
#34155=CARTESIAN_POINT ( 'NONE',  ( -19.32961685222932147, 0.000000000000000000, 14.39908572644263351 ) ) ;
#34156=ORIENTED_EDGE ( 'NONE', *, *, #36885, .F. ) ;
#34157=CARTESIAN_POINT ( 'NONE',  ( -19.60990026154428278, 0.000000000000000000, 4.498472333781370125 ) ) ;
#34158=CARTESIAN_POINT ( 'NONE',  ( -13.67982092077429890, 0.000000000000000000, 4.913953652214907208 ) ) ;
#34159=EDGE_CURVE ( 'NONE', #51983, #43785, #36526, .T. ) ;
#34160=ORIENTED_EDGE ( 'NONE', *, *, #30344, .T. ) ;
#34161=CARTESIAN_POINT ( 'NONE',  ( -12.18226100520636379, -0.1191753592594183703, 4.456272911837774409 ) ) ;
#34163=AXIS2_PLACEMENT_3D ( 'NONE', #37604, #16571, #33361 ) ;
#34164=CARTESIAN_POINT ( 'NONE',  ( -19.70588832770281584, 2.167151335408493029, 6.911193162818738855 ) ) ;
#34166=VERTEX_POINT ( 'NONE', #14414 ) ;
#34167=FACE_OUTER_BOUND ( 'NONE', #40276, .T. ) ;
#34168=CARTESIAN_POINT ( 'NONE',  ( -13.37456397384763740, 0.7721120973665037690, 1.852432162681123984 ) ) ;
#34169=LINE ( 'NONE', #24777, #22354 ) ;
#34170=CARTESIAN_POINT ( 'NONE',  ( -19.32961685222932147, 0.000000000000000000, 14.39908572644263351 ) ) ;
#34171=AXIS2_PLACEMENT_3D ( 'NONE', #25026, #7990, #4829 ) ;
#34172=ORIENTED_EDGE ( 'NONE', *, *, #52054, .F. ) ;
#34173=DIRECTION ( 'NONE',  ( 0.005961354470445682716, -0.6427876096865404731, -0.7660212471507180654 ) ) ;
#34174=VECTOR ( 'NONE', #4166, 999.9999999999998863 ) ;
#34175=DIRECTION ( 'NONE',  ( 0.005002170337468016433, -0.7660444431189770143, -0.6427681459581293666 ) ) ;
#34176=CARTESIAN_POINT ( 'NONE',  ( -20.54204810873173415, 0.000000000000000000, 4.860550213503115558 ) ) ;
#34177=FACE_OUTER_BOUND ( 'NONE', #29883, .T. ) ;
#34178=CARTESIAN_POINT ( 'NONE',  ( -11.69750573382829550, -0.1191753592594198274, 1.874720900801436940 ) ) ;
#34179=VECTOR ( 'NONE', #38004, 1000.000000000000000 ) ;
#34180=DIRECTION ( 'NONE',  ( 0.6427681459581294776, -0.7660444431189769032, 0.005002170337467562802 ) ) ;
#34181=ORIENTED_EDGE ( 'NONE', *, *, #31356, .F. ) ;
#34182=PLANE ( 'NONE',  #798 ) ;
#34183=DIRECTION ( 'NONE',  ( 0.000000000000000000, -1.000000000000000000, 0.000000000000000000 ) ) ;
#34184=CARTESIAN_POINT ( 'NONE',  ( -13.97961799777601932, -5.051250379848164940, 2.150318164026983947 ) ) ;
#34185=ORIENTED_EDGE ( 'NONE', *, *, #49364, .F. ) ;
#34186=DIRECTION ( 'NONE',  ( 0.007781995580012663651, -3.146120232559066537E-19, -0.9999697198139514409 ) ) ;
#34187=ORIENTED_EDGE ( 'NONE', *, *, #21624, .F. ) ;
#34188=EDGE_CURVE ( 'NONE', #24292, #171, #2150, .T. ) ;
#34189=DIRECTION ( 'NONE',  ( 0.6427681459581294776, -0.7660444431189769032, 0.005002170337467562802 ) ) ;
#34190=DIRECTION ( 'NONE',  ( 0.007781995580012663651, 0.000000000000000000, -0.9999697198139515519 ) ) ;
#34191=VECTOR ( 'NONE', #32604, 999.9999999999998863 ) ;
#34192=EDGE_CURVE ( 'NONE', #19170, #3617, #36832, .T. ) ;
#34193=CARTESIAN_POINT ( 'NONE',  ( -15.79858100839565083, 0.000000000000000000, 4.328126845270309886 ) ) ;
#34194=AXIS2_PLACEMENT_3D ( 'NONE', #49890, #53059, #44515 ) ;
#34197=AXIS2_PLACEMENT_3D ( 'NONE', #22462, #52803, #11039 ) ;
#34198=ORIENTED_EDGE ( 'NONE', *, *, #47024, .F. ) ;
#34200=LINE ( 'NONE', #30769, #55837 ) ;
#34201=PLANE ( 'NONE',  #37775 ) ;
#34202=EDGE_CURVE ( 'NONE', #5703, #37228, #49610, .T. ) ;
#34204=EDGE_CURVE ( 'NONE', #44736, #47582, #18363, .T. ) ;
#34205=FACE_OUTER_BOUND ( 'NONE', #4181, .T. ) ;
#34206=FACE_OUTER_BOUND ( 'NONE', #47176, .T. ) ;
#34207=DIRECTION ( 'NONE',  ( 0.007781995580012662783, 0.000000000000000000, -0.9999697198139514409 ) ) ;
#34208=ORIENTED_EDGE ( 'NONE', *, *, #22722, .T. ) ;
#34209=EDGE_CURVE ( 'NONE', #36112, #39217, #49311, .T. ) ;
#34211=AXIS2_PLACEMENT_3D ( 'NONE', #879, #26728, #44054 ) ;
#34213=ORIENTED_EDGE ( 'NONE', *, *, #12249, .F. ) ;
#34214=DIRECTION ( 'NONE',  ( -0.9999697198139514409, -0.000000000000000000, -0.007781995580013368816 ) ) ;
#34215=FACE_OUTER_BOUND ( 'NONE', #37553, .T. ) ;
#34216=LINE ( 'NONE', #44384, #40204 ) ;
#34218=CARTESIAN_POINT ( 'NONE',  ( -16.64444113932924196, -1.003701604285656579, 4.794443245222647754 ) ) ;
#34219=VECTOR ( 'NONE', #34740, 1000.000000000000000 ) ;
#34220=EDGE_LOOP ( 'NONE', ( #6382, #29680, #35859, #14722 ) ) ;
#34221=EDGE_CURVE ( 'NONE', #32474, #47218, #10127, .T. ) ;
#34222=ADVANCED_FACE ( 'NONE', ( #27754 ), #45074, .F. ) ;
#34223=ORIENTED_EDGE ( 'NONE', *, *, #13867, .F. ) ;
#34224=VECTOR ( 'NONE', #37038, 1000.000000000000227 ) ;
#34225=EDGE_LOOP ( 'NONE', ( #3244, #29398, #9635, #43680 ) ) ;
#34226=EDGE_CURVE ( 'NONE', #27231, #27480, #35701, .T. ) ;
#34227=VERTEX_POINT ( 'NONE', #54144 ) ;
#34228=LINE ( 'NONE', #43304, #22108 ) ;
#34229=EDGE_LOOP ( 'NONE', ( #19302, #46140, #55787, #20654, #19753 ) ) ;
#34230=PLANE ( 'NONE',  #4090 ) ;
#34231=EDGE_CURVE ( 'NONE', #23596, #44456, #1871, .T. ) ;
#34232=AXIS2_PLACEMENT_3D ( 'NONE', #18087, #5325, #9279 ) ;
#34233=VERTEX_POINT ( 'NONE', #10959 ) ;
#34234=LINE ( 'NONE', #29093, #55840 ) ;
#34235=EDGE_LOOP ( 'NONE', ( #5278, #37297, #35472, #51093 ) ) ;
#34236=VERTEX_POINT ( 'NONE', #53017 ) ;
#34237=EDGE_CURVE ( 'NONE', #947, #45223, #28278, .T. ) ;
#34238=FACE_OUTER_BOUND ( 'NONE', #5764, .T. ) ;
#34239=FACE_OUTER_BOUND ( 'NONE', #6285, .T. ) ;
#34240=PLANE ( 'NONE',  #35838 ) ;
#34241=DIRECTION ( 'NONE',  ( -0.5364919789714478471, 0.6444004775717705469, -0.5449076811759709926 ) ) ;
#34242=DIRECTION ( 'NONE',  ( -0.005961354470445682716, -0.6427876096865404731, 0.7660212471507180654 ) ) ;
#34243=VERTEX_POINT ( 'NONE', #36009 ) ;
#34244=EDGE_LOOP ( 'NONE', ( #30651, #30680, #10470, #2019 ) ) ;
#34245=DIRECTION ( 'NONE',  ( -0.3313982828793700652, 0.4028455766673916250, -0.8531650599175529814 ) ) ;
#34246=DIRECTION ( 'NONE',  ( 0.5364919789714477361, 0.6444004775717706579, 0.5449076811759711036 ) ) ;
#34247=DIRECTION ( 'NONE',  ( 0.6246952433987893460, 0.7422098413412802076, -0.2426528472758539279 ) ) ;
#34248=CARTESIAN_POINT ( 'NONE',  ( -20.54049170961573267, 0.000000000000000000, 4.660556269540326646 ) ) ;
#34249=CARTESIAN_POINT ( 'NONE',  ( -14.66887761629205222, 0.000000000000000000, 12.58869632783390990 ) ) ;
#34250=DIRECTION ( 'NONE',  ( 0.000000000000000000, -0.000000000000000000, -1.000000000000000000 ) ) ;
#34251=ORIENTED_EDGE ( 'NONE', *, *, #54124, .F. ) ;
#34252=FACE_OUTER_BOUND ( 'NONE', #54703, .T. ) ;
#34253=PLANE ( 'NONE',  #31322 ) ;
#34254=ORIENTED_EDGE ( 'NONE', *, *, #17615, .F. ) ;
#34255=CARTESIAN_POINT ( 'NONE',  ( -9.342070512798265725, 0.000000000000000000, 10.59882438848031505 ) ) ;
#34256=DIRECTION ( 'NONE',  ( 0.5364919789714477361, 0.6444004775717706579, 0.5449076811759711036 ) ) ;
#34257=DIRECTION ( 'NONE',  ( 0.7660212471507180654, -0.6427876096865404731, 0.005961354470445141482 ) ) ;
#34259=VECTOR ( 'NONE', #23688, 999.9999999999998863 ) ;
#34260=VERTEX_POINT ( 'NONE', #33503 ) ;
#34261=ORIENTED_EDGE ( 'NONE', *, *, #37837, .F. ) ;
#34262=DIRECTION ( 'NONE',  ( 0.5449076811759707706, 0.6444004775717708799, -0.5364919789714476250 ) ) ;
#34263=LINE ( 'NONE', #21173, #28591 ) ;
#34264=DIRECTION ( 'NONE',  ( -0.9999697198139514409, -0.000000000000000000, -0.007781995580013368816 ) ) ;
#34265=ADVANCED_FACE ( 'NONE', ( #33242 ), #29537, .F. ) ;
#34266=VECTOR ( 'NONE', #16767, 1000.000000000000227 ) ;
#34267=CARTESIAN_POINT ( 'NONE',  ( -10.27421835998572064, 0.000000000000000000, 10.96090226820206048 ) ) ;
#34269=EDGE_CURVE ( 'NONE', #22414, #13266, #46852, .T. ) ;
#34270=CARTESIAN_POINT ( 'NONE',  ( -19.28774072249866478, -2.460819163488157546, 8.212568725711509643 ) ) ;
#34271=EDGE_CURVE ( 'NONE', #21088, #8091, #54498, .T. ) ;
#34272=FACE_OUTER_BOUND ( 'NONE', #10307, .T. ) ;
#34273=DIRECTION ( 'NONE',  ( 0.9999697198139515519, 0.000000000000000000, 0.007781995580013368816 ) ) ;
#34274=LINE ( 'NONE', #51579, #14238 ) ;
#34275=CARTESIAN_POINT ( 'NONE',  ( 2.072287782118878319, 0.000000000000000000, -2.950529333540147015 ) ) ;
#34276=ORIENTED_EDGE ( 'NONE', *, *, #2385, .T. ) ;
#34277=PLANE ( 'NONE',  #11390 ) ;
#34278=ORIENTED_EDGE ( 'NONE', *, *, #24515, .T. ) ;
#34279=ORIENTED_EDGE ( 'NONE', *, *, #40264, .T. ) ;
#34280=ORIENTED_EDGE ( 'NONE', *, *, #48695, .F. ) ;
#34281=EDGE_LOOP ( 'NONE', ( #32257, #6746, #31491, #37537 ) ) ;
#34282=VERTEX_POINT ( 'NONE', #24684 ) ;
#34283=ORIENTED_EDGE ( 'NONE', *, *, #35323, .F. ) ;
#34284=CARTESIAN_POINT ( 'NONE',  ( -17.83139810946674686, -0.1191753592594197858, 13.85674710641801788 ) ) ;
#34285=CARTESIAN_POINT ( 'NONE',  ( -16.81793962562570144, -0.1166911823299060097, 3.314285314562989360 ) ) ;
#34286=DIRECTION ( 'NONE',  ( 0.000000000000000000, -0.000000000000000000, -1.000000000000000000 ) ) ;
#34287=ORIENTED_EDGE ( 'NONE', *, *, #16453, .T. ) ;
#34288=CARTESIAN_POINT ( 'NONE',  ( -26.13337879274045505, 0.000000000000000000, 6.833023547870798353 ) ) ;
#34289=ORIENTED_EDGE ( 'NONE', *, *, #31592, .F. ) ;
#34290=LINE ( 'NONE', #51598, #28606 ) ;
#34291=ORIENTED_EDGE ( 'NONE', *, *, #45294, .T. ) ;
#34292=EDGE_CURVE ( 'NONE', #4182, #35810, #28963, .T. ) ;
#34293=DIRECTION ( 'NONE',  ( -0.5449076811759708816, 0.6444004775717707689, 0.5364919789714475140 ) ) ;
#34294=ADVANCED_FACE ( 'NONE', ( #7663 ), #37779, .F. ) ;
#34295=CARTESIAN_POINT ( 'NONE',  ( -25.20123094555300369, 0.000000000000000000, 6.470945668149052032 ) ) ;
#34296=FACE_OUTER_BOUND ( 'NONE', #28239, .T. ) ;
#34297=EDGE_LOOP ( 'NONE', ( #45866, #8792, #48825, #39764 ) ) ;
#34298=DIRECTION ( 'NONE',  ( 0.6427681459581294776, -0.7660444431189769032, 0.005002170337467562802 ) ) ;
#34299=ORIENTED_EDGE ( 'NONE', *, *, #54193, .T. ) ;
#34300=AXIS2_PLACEMENT_3D ( 'NONE', #44701, #48118, #43864 ) ;
#34301=PLANE ( 'NONE',  #11896 ) ;
#34302=EDGE_CURVE ( 'NONE', #6152, #26523, #50250, .T. ) ;
#34303=PLANE ( 'NONE',  #24827 ) ;
#34304=CARTESIAN_POINT ( 'NONE',  ( -9.542064456761055524, 0.000000000000000000, 10.59726798936431180 ) ) ;
#34305=PLANE ( 'NONE',  #26782 ) ;
#34306=CARTESIAN_POINT ( 'NONE',  ( -13.86944162542047287, -3.756034771668159689, 8.233586821798175137 ) ) ;
#34307=CARTESIAN_POINT ( 'NONE',  ( -12.96168924638702968, -0.5179957512181557755, 1.899554624828523108 ) ) ;
#34308=LINE ( 'NONE', #55886, #27548 ) ;
#34309=FACE_OUTER_BOUND ( 'NONE', #29958, .T. ) ;
#34310=ORIENTED_EDGE ( 'NONE', *, *, #29645, .T. ) ;
#34311=DIRECTION ( 'NONE',  ( 0.9999697198139515519, 0.000000000000000000, 0.007781995580013368816 ) ) ;
#34312=EDGE_LOOP ( 'NONE', ( #5811, #29449, #50236, #42367 ) ) ;
#34313=CARTESIAN_POINT ( 'NONE',  ( -17.93139508144814442, 0.000000000000000000, 13.85596890686001537 ) ) ;
#34314=DIRECTION ( 'NONE',  ( 0.007781995580012663651, -3.146120232559066537E-19, -0.9999697198139514409 ) ) ;
#34315=DIRECTION ( 'NONE',  ( 0.9999697198139515519, 0.000000000000000000, 0.007781995580013368816 ) ) ;
#34316=PLANE ( 'NONE',  #39481 ) ;
#34317=DIRECTION ( 'NONE',  ( 0.5449076811759707706, 0.6444004775717708799, -0.5364919789714476250 ) ) ;
#34318=DIRECTION ( 'NONE',  ( -0.6427681459581293666, -0.7660444431189770143, -0.005002170337467561935 ) ) ;
#34320=ORIENTED_EDGE ( 'NONE', *, *, #34558, .F. ) ;
#34321=CARTESIAN_POINT ( 'NONE',  ( -14.01623497886155256, -0.1191753592594197858, 2.226008083469502630 ) ) ;
#34322=CARTESIAN_POINT ( 'NONE',  ( -25.20200914511100265, -0.1191753592594197858, 6.570942640130446932 ) ) ;
#34323=ADVANCED_FACE ( 'NONE', ( #3667 ), #42312, .F. ) ;
#34324=DIRECTION ( 'NONE',  ( -0.005002170337468016433, -0.7660444431189770143, 0.6427681459581293666 ) ) ;
#34325=EDGE_CURVE ( 'NONE', #28099, #1224, #3107, .T. ) ;
#34326=LINE ( 'NONE', #17261, #39112 ) ;
#34328=LINE ( 'NONE', #38280, #5978 ) ;
#34329=ADVANCED_FACE ( 'NONE', ( #51087 ), #11063, .F. ) ;
#34330=EDGE_CURVE ( 'NONE', #41524, #7759, #28388, .T. ) ;
#34331=DIRECTION ( 'NONE',  ( 0.005002170337468016433, -0.7660444431189770143, -0.6427681459581293666 ) ) ;
#34332=EDGE_LOOP ( 'NONE', ( #14713, #8202, #53343, #8585 ) ) ;
#34333=PLANE ( 'NONE',  #19458 ) ;
#34334=LINE ( 'NONE', #54766, #18725 ) ;
#34335=EDGE_LOOP ( 'NONE', ( #28843, #9957, #30264, #27010 ) ) ;
#34336=ORIENTED_EDGE ( 'NONE', *, *, #24515, .F. ) ;
#34337=LINE ( 'NONE', #33486, #29208 ) ;
#34338=AXIS2_PLACEMENT_3D ( 'NONE', #32506, #20252, #19418 ) ;
#34339=ORIENTED_EDGE ( 'NONE', *, *, #55601, .T. ) ;
#34341=VERTEX_POINT ( 'NONE', #25270 ) ;
#34342=EDGE_LOOP ( 'NONE', ( #41700, #14327, #41747, #10950 ) ) ;
#34343=ORIENTED_EDGE ( 'NONE', *, *, #41815, .T. ) ;
#34344=DIRECTION ( 'NONE',  ( -0.5364919789714478471, 0.6444004775717705469, -0.5449076811759709926 ) ) ;
#34346=PLANE ( 'NONE',  #11482 ) ;
#34347=LINE ( 'NONE', #55344, #6761 ) ;
#34348=ORIENTED_EDGE ( 'NONE', *, *, #8100, .F. ) ;
#34349=VERTEX_POINT ( 'NONE', #11361 ) ;
#34350=CARTESIAN_POINT ( 'NONE',  ( -17.77227403482580570, -0.1191753592594188005, 6.259430486910483538 ) ) ;
#34351=DIRECTION ( 'NONE',  ( 0.6427681459581294776, -0.7660444431189769032, 0.005002170337467562802 ) ) ;
#34352=ORIENTED_EDGE ( 'NONE', *, *, #16630, .T. ) ;
#34353=LINE ( 'NONE', #55635, #5571 ) ;
#34354=CARTESIAN_POINT ( 'NONE',  ( -9.280420900666706885, 0.000000000000000000, 3.101530451399800103 ) ) ;
#34356=LINE ( 'NONE', #51660, #11275 ) ;
#34357=ORIENTED_EDGE ( 'NONE', *, *, #2622, .F. ) ;
#34358=FACE_OUTER_BOUND ( 'NONE', #39383, .T. ) ;
#34359=ADVANCED_FACE ( 'NONE', ( #33768 ), #15597, .F. ) ;
#34360=LINE ( 'NONE', #29550, #30893 ) ;
#34361=VERTEX_POINT ( 'NONE', #29228 ) ;
#34362=FACE_OUTER_BOUND ( 'NONE', #42904, .T. ) ;
#34363=CARTESIAN_POINT ( 'NONE',  ( -8.938424887834608867, -0.1191753592594185784, 5.589513403987136364 ) ) ;
#34364=LINE ( 'NONE', #12214, #37520 ) ;
#34365=DIRECTION ( 'NONE',  ( 0.9999697198139515519, 0.000000000000000000, 0.007781995580013368816 ) ) ;
#34366=ORIENTED_EDGE ( 'NONE', *, *, #29944, .T. ) ;
#34367=ADVANCED_FACE ( 'NONE', ( #15897 ), #34075, .F. ) ;
#34368=DIRECTION ( 'NONE',  ( 0.7660212471507180654, -0.6427876096865404731, 0.005961354470445141482 ) ) ;
#34369=LINE ( 'NONE', #25853, #12399 ) ;
#34370=LINE ( 'NONE', #25553, #28512 ) ;
#34371=LINE ( 'NONE', #51676, #4178 ) ;
#34372=CARTESIAN_POINT ( 'NONE',  ( -27.99767448711536133, 0.000000000000000000, 7.557179307314289218 ) ) ;
#34374=PLANE ( 'NONE',  #54829 ) ;
#34375=CARTESIAN_POINT ( 'NONE',  ( -10.22563470401762764, 0.01196729935014182421, 0.6681340434156105568 ) ) ;
#34376=EDGE_CURVE ( 'NONE', #50478, #55289, #12757, .T. ) ;
#34377=DIRECTION ( 'NONE',  ( -0.5364919789714478471, 0.6444004775717705469, -0.5449076811759709926 ) ) ;
#34378=LINE ( 'NONE', #38645, #37692 ) ;
#34379=ORIENTED_EDGE ( 'NONE', *, *, #49247, .T. ) ;
#34381=VERTEX_POINT ( 'NONE', #21278 ) ;
#34382=CARTESIAN_POINT ( 'NONE',  ( -14.00280974873554030, 0.000000000000000000, 12.40921378708904044 ) ) ;
#34383=ADVANCED_FACE ( 'NONE', ( #39451 ), #43156, .F. ) ;
#34384=PLANE ( 'NONE',  #43584 ) ;
#34385=ADVANCED_FACE ( 'NONE', ( #38607 ), #47114, .F. ) ;
#34386=CARTESIAN_POINT ( 'NONE',  ( -9.591484076946107606, 1.593386918697492494, 2.300716907277841727 ) ) ;
#34387=CARTESIAN_POINT ( 'NONE',  ( -16.73935101609895426, 0.000000000000000000, 5.798133834765347494 ) ) ;
#34388=EDGE_CURVE ( 'NONE', #1645, #31141, #51655, .T. ) ;
#34389=CARTESIAN_POINT ( 'NONE',  ( -26.13493519185646008, 0.000000000000000000, 7.033017491833586377 ) ) ;
#34391=ORIENTED_EDGE ( 'NONE', *, *, #54330, .F. ) ;
#34393=DIRECTION ( 'NONE',  ( -0.6427681459581293666, -0.7660444431189770143, -0.005002170337467561935 ) ) ;
#34394=VERTEX_POINT ( 'NONE', #48218 ) ;
#34395=CARTESIAN_POINT ( 'NONE',  ( 2.072287782118878319, 0.000000000000000000, -2.950529333540147015 ) ) ;
#34396=ADVANCED_FACE ( 'NONE', ( #9328 ), #4795, .F. ) ;
#34397=ORIENTED_EDGE ( 'NONE', *, *, #31772, .T. ) ;
#34398=DIRECTION ( 'NONE',  ( 0.000000000000000000, -0.000000000000000000, -1.000000000000000000 ) ) ;
#34400=CARTESIAN_POINT ( 'NONE',  ( -10.00813838035478298, 0.000000000000000000, 10.77830692922518452 ) ) ;
#34401=EDGE_CURVE ( 'NONE', #2695, #33003, #12498, .T. ) ;
#34402=ORIENTED_EDGE ( 'NONE', *, *, #54064, .F. ) ;
#34403=VERTEX_POINT ( 'NONE', #13592 ) ;
#34404=ORIENTED_EDGE ( 'NONE', *, *, #11624, .T. ) ;
#34405=CARTESIAN_POINT ( 'NONE',  ( -17.67305526240241065, 0.000000000000000000, 6.360205658449882726 ) ) ;
#34406=LINE ( 'NONE', #11427, #32326 ) ;
#34407=CARTESIAN_POINT ( 'NONE',  ( 2.072287782118878319, 0.000000000000000000, -2.950529333540147015 ) ) ;
#34408=CARTESIAN_POINT ( 'NONE',  ( -22.40478740399063895, 0.000000000000000000, 5.384712028983816623 ) ) ;
#34409=ORIENTED_EDGE ( 'NONE', *, *, #281, .T. ) ;
#34410=ORIENTED_EDGE ( 'NONE', *, *, #42694, .F. ) ;
#34411=ORIENTED_EDGE ( 'NONE', *, *, #34822, .F. ) ;
#34413=ORIENTED_EDGE ( 'NONE', *, *, #2477, .F. ) ;
#34414=FACE_OUTER_BOUND ( 'NONE', #54451, .T. ) ;
#34415=ORIENTED_EDGE ( 'NONE', *, *, #16540, .F. ) ;
#34416=DIRECTION ( 'NONE',  ( 0.6427681459581294776, -0.7660444431189769032, 0.005002170337467562802 ) ) ;
#34417=DIRECTION ( 'NONE',  ( 0.005961354470445682716, -0.6427876096865404731, -0.7660212471507180654 ) ) ;
#34418=VERTEX_POINT ( 'NONE', #34350 ) ;
#34419=PLANE ( 'NONE',  #28605 ) ;
#34420=EDGE_CURVE ( 'NONE', #8019, #29009, #13340, .T. ) ;
#34422=DIRECTION ( 'NONE',  ( 0.000000000000000000, -0.000000000000000000, -1.000000000000000000 ) ) ;
#34423=LINE ( 'NONE', #8294, #38359 ) ;
#34424=ORIENTED_EDGE ( 'NONE', *, *, #35926, .T. ) ;
#34426=LINE ( 'NONE', #42396, #28436 ) ;
#34427=FACE_OUTER_BOUND ( 'NONE', #25990, .T. ) ;
#34428=ORIENTED_EDGE ( 'NONE', *, *, #44441, .F. ) ;
#34429=LINE ( 'NONE', #34703, #4746 ) ;
#34430=FACE_OUTER_BOUND ( 'NONE', #43215, .T. ) ;
#34431=CARTESIAN_POINT ( 'NONE',  ( -17.73140113748535285, 0.000000000000000000, 13.85752530597602039 ) ) ;
#34432=DIRECTION ( 'NONE',  ( 0.000000000000000000, -0.000000000000000000, -1.000000000000000000 ) ) ;
#34434=ADVANCED_FACE ( 'NONE', ( #9061 ), #43973, .F. ) ;
#34435=VERTEX_POINT ( 'NONE', #808 ) ;
#34436=CARTESIAN_POINT ( 'NONE',  ( -9.342070512798265725, 0.000000000000000000, 10.59882438848031505 ) ) ;
#34437=FACE_OUTER_BOUND ( 'NONE', #10549, .T. ) ;
#34438=DIRECTION ( 'NONE',  ( 0.005961354470445682716, -0.6427876096865404731, -0.7660212471507180654 ) ) ;
#34439=EDGE_LOOP ( 'NONE', ( #19598, #16503, #14733, #27266 ) ) ;
#34440=DIRECTION ( 'NONE',  ( 0.005002170337468016433, -0.7660444431189770143, -0.6427681459581293666 ) ) ;
#34441=DIRECTION ( 'NONE',  ( 0.5449076811759707706, 0.6444004775717708799, -0.5364919789714476250 ) ) ;
#34442=ORIENTED_EDGE ( 'NONE', *, *, #33992, .F. ) ;
#34443=CARTESIAN_POINT ( 'NONE',  ( -27.99923088623136636, 0.000000000000000000, 7.757173251277078130 ) ) ;
#34444=DIRECTION ( 'NONE',  ( -0.5449076811759708816, 0.6444004775717707689, 0.5364919789714475140 ) ) ;
#34445=ADVANCED_FACE ( 'NONE', ( #26366 ), #18128, .F. ) ;
#34446=DIRECTION ( 'NONE',  ( 0.9999697198139515519, 0.000000000000000000, 0.007781995580013368816 ) ) ;
#34449=VERTEX_POINT ( 'NONE', #17284 ) ;
#34451=EDGE_CURVE ( 'NONE', #23008, #12964, #234, .T. ) ;
#34452=FACE_OUTER_BOUND ( 'NONE', #6207, .T. ) ;
#34453=CARTESIAN_POINT ( 'NONE',  ( -20.54049170961573267, 0.000000000000000000, 4.660556269540326646 ) ) ;
#34454=CARTESIAN_POINT ( 'NONE',  ( -12.57759610834895447, 2.553033558614007603, 5.956849598244149391 ) ) ;
#34455=PLANE ( 'NONE',  #46541 ) ;
#34456=EDGE_CURVE ( 'NONE', #36489, #5931, #51925, .T. ) ;
#34458=LINE ( 'NONE', #8924, #12195 ) ;
#34459=ORIENTED_EDGE ( 'NONE', *, *, #4388, .F. ) ;
#34460=CARTESIAN_POINT ( 'NONE',  ( -14.93495759592298988, 0.000000000000000000, 12.77129166681078409 ) ) ;
#34461=ADVANCED_FACE ( 'NONE', ( #14717 ), #28058, .F. ) ;
#34462=CARTESIAN_POINT ( 'NONE',  ( -17.53328333432119379, 2.391131607591508335, 3.416164794119107562 ) ) ;
#34463=ORIENTED_EDGE ( 'NONE', *, *, #43837, .T. ) ;
#34464=PLANE ( 'NONE',  #41979 ) ;
#34465=FACE_OUTER_BOUND ( 'NONE', #43888, .T. ) ;
#34466=CARTESIAN_POINT ( 'NONE',  ( -26.13415699229845757, -0.1191753592594197858, 6.933020519852192365 ) ) ;
#34467=EDGE_LOOP ( 'NONE', ( #44053, #6892, #45683, #13645 ) ) ;
#34468=DIRECTION ( 'NONE',  ( 0.5364919789714477361, 0.6444004775717706579, 0.5449076811759711036 ) ) ;
#34470=VECTOR ( 'NONE', #28576, 999.9999999999998863 ) ;
#34471=ORIENTED_EDGE ( 'NONE', *, *, #12549, .F. ) ;
#34472=ORIENTED_EDGE ( 'NONE', *, *, #51181, .F. ) ;
#34473=VERTEX_POINT ( 'NONE', #10172 ) ;
#34474=DIRECTION ( 'NONE',  ( -0.005961354470445682716, -0.6427876096865404731, 0.7660212471507180654 ) ) ;
#34475=ORIENTED_EDGE ( 'NONE', *, *, #19630, .F. ) ;
#34476=EDGE_CURVE ( 'NONE', #34233, #29943, #1911, .T. ) ;
#34477=DIRECTION ( 'NONE',  ( 0.6427681459581294776, -0.7660444431189769032, 0.005002170337467562802 ) ) ;
#34478=ORIENTED_EDGE ( 'NONE', *, *, #41686, .F. ) ;
#34480=ORIENTED_EDGE ( 'NONE', *, *, #21946, .T. ) ;
#34481=CARTESIAN_POINT ( 'NONE',  ( -24.27063949748155380, 0.000000000000000000, 6.308861732390097288 ) ) ;
#34483=VERTEX_POINT ( 'NONE', #1374 ) ;
#34484=DIRECTION ( 'NONE',  ( 0.005002170337468016433, -0.7660444431189770143, -0.6427681459581293666 ) ) ;
#34485=CARTESIAN_POINT ( 'NONE',  ( -18.39746900504187010, 0.000000000000000000, 14.03700784672088808 ) ) ;
#34486=ADVANCED_FACE ( 'NONE', ( #35747 ), #45365, .F. ) ;
#34487=CARTESIAN_POINT ( 'NONE',  ( -12.07729412577240602, 0.000000000000000000, 3.818428676861645776 ) ) ;
#34488=CARTESIAN_POINT ( 'NONE',  ( -18.39746900504187010, 0.000000000000000000, 14.03700784672088808 ) ) ;
#34489=CARTESIAN_POINT ( 'NONE',  ( -11.17676086714305761, 0.000000000000000000, 7.518757532975309132 ) ) ;
#34490=EDGE_LOOP ( 'NONE', ( #2813, #32536, #40909, #42560 ) ) ;
#34491=EDGE_CURVE ( 'NONE', #6556, #35938, #23521, .T. ) ;
#34492=EDGE_CURVE ( 'NONE', #28751, #31964, #53067, .T. ) ;
#34494=ORIENTED_EDGE ( 'NONE', *, *, #14738, .F. ) ;
#34495=DIRECTION ( 'NONE',  ( 0.000000000000000000, -0.000000000000000000, -1.000000000000000000 ) ) ;
#34496=CARTESIAN_POINT ( 'NONE',  ( -13.53673582514181106, 0.000000000000000000, 12.22817484722816772 ) ) ;
#34497=CARTESIAN_POINT ( 'NONE',  ( -16.81267852042391198, -0.1191753592594197858, 3.312241722634738039 ) ) ;
#34498=LINE ( 'NONE', #22837, #18554 ) ;
#34499=DIRECTION ( 'NONE',  ( -0.5364919789714478471, 0.6444004775717705469, -0.5449076811759709926 ) ) ;
#34500=DIRECTION ( 'NONE',  ( -0.5449076811759708816, 0.6444004775717707689, 0.5364919789714475140 ) ) ;
#34501=ORIENTED_EDGE ( 'NONE', *, *, #29084, .T. ) ;
#34502=DIRECTION ( 'NONE',  ( 0.007781995580012662783, 0.000000000000000000, -0.9999697198139514409 ) ) ;
#34504=ORIENTED_EDGE ( 'NONE', *, *, #47633, .F. ) ;
#34505=DIRECTION ( 'NONE',  ( -0.6427681459581293666, -0.7660444431189770143, -0.005002170337467561935 ) ) ;
#34506=CARTESIAN_POINT ( 'NONE',  ( -11.67244013076689946, 0.000000000000000000, 11.50401908778467863 ) ) ;
#34507=ADVANCED_FACE ( 'NONE', ( #14182 ), #53354, .F. ) ;
#34509=LINE ( 'NONE', #39895, #38687 ) ;
#34510=VECTOR ( 'NONE', #33532, 1000.000000000000114 ) ;
#34511=ADVANCED_FACE ( 'NONE', ( #14450 ), #35451, .F. ) ;
#34512=EDGE_LOOP ( 'NONE', ( #24157, #40611, #52095, #32945 ) ) ;
#34513=ORIENTED_EDGE ( 'NONE', *, *, #2183, .F. ) ;
#34514=ADVANCED_FACE ( 'NONE', ( #5371 ), #31193, .F. ) ;
#34515=CARTESIAN_POINT ( 'NONE',  ( -8.578754870427481194, 0.000000000000000000, 6.230973550731281563 ) ) ;
#34516=CARTESIAN_POINT ( 'NONE',  ( -17.86312967602380652, 2.229229656569006401, 3.549453834752706705 ) ) ;
#34517=DIRECTION ( 'NONE',  ( -0.9999697198139514409, -0.000000000000000000, -0.007781995580013368816 ) ) ;
#34520=DIRECTION ( 'NONE',  ( -0.7660212471507179544, -0.6427876096865405842, -0.005961354470445141482 ) ) ;
#34521=DIRECTION ( 'NONE',  ( -0.005002170337468016433, -0.7660444431189770143, 0.6427681459581293666 ) ) ;
#34522=DIRECTION ( 'NONE',  ( -0.005961354470445682716, -0.6427876096865404731, 0.7660212471507180654 ) ) ;
#34523=EDGE_CURVE ( 'NONE', #38038, #18836, #51863, .T. ) ;
#34525=ORIENTED_EDGE ( 'NONE', *, *, #44838, .F. ) ;
#34526=LINE ( 'NONE', #34813, #33227 ) ;
#34527=LINE ( 'NONE', #35655, #15161 ) ;
#34528=ORIENTED_EDGE ( 'NONE', *, *, #52367, .T. ) ;
#34529=CARTESIAN_POINT ( 'NONE',  ( 2.072287782118878319, 0.000000000000000000, -2.950529333540147015 ) ) ;
#34530=VERTEX_POINT ( 'NONE', #55565 ) ;
#34531=LINE ( 'NONE', #4171, #44921 ) ;
#34532=ORIENTED_EDGE ( 'NONE', *, *, #21644, .F. ) ;
#34533=VECTOR ( 'NONE', #23852, 999.9999999999998863 ) ;
#34535=ORIENTED_EDGE ( 'NONE', *, *, #10794, .F. ) ;
#34536=ORIENTED_EDGE ( 'NONE', *, *, #18085, .T. ) ;
#34537=VERTEX_POINT ( 'NONE', #21208 ) ;
#34538=ORIENTED_EDGE ( 'NONE', *, *, #38593, .F. ) ;
#34539=DIRECTION ( 'NONE',  ( -0.5364919789714478471, 0.6444004775717705469, -0.5449076811759709926 ) ) ;
#34540=FACE_OUTER_BOUND ( 'NONE', #17815, .T. ) ;
#34542=AXIS2_PLACEMENT_3D ( 'NONE', #11077, #50264, #50815 ) ;
#34543=VERTEX_POINT ( 'NONE', #55872 ) ;
#34544=PLANE ( 'NONE',  #40350 ) ;
#34545=VERTEX_POINT ( 'NONE', #30855 ) ;
#34546=PLANE ( 'NONE',  #25907 ) ;
#34547=ORIENTED_EDGE ( 'NONE', *, *, #7928, .T. ) ;
#34548=VECTOR ( 'NONE', #26626, 1000.000000000000000 ) ;
#34549=DIRECTION ( 'NONE',  ( 0.9999697198139515519, 0.000000000000000000, 0.007781995580013368816 ) ) ;
#34550=FACE_OUTER_BOUND ( 'NONE', #1714, .T. ) ;
#34551=EDGE_LOOP ( 'NONE', ( #31274, #5297, #2808, #13206 ) ) ;
#34552=CARTESIAN_POINT ( 'NONE',  ( -11.87243407472968926, 0.000000000000000000, 11.50246268866867361 ) ) ;
#34553=ORIENTED_EDGE ( 'NONE', *, *, #10620, .T. ) ;
#34554=ADVANCED_FACE ( 'NONE', ( #16974 ), #12981, .F. ) ;
#34555=ADVANCED_FACE ( 'NONE', ( #43373 ), #3884, .F. ) ;
#34556=CARTESIAN_POINT ( 'NONE',  ( -11.69649624729248316, 2.067327705546507133, 4.817474438081196908 ) ) ;
#34557=DIRECTION ( 'NONE',  ( -0.7660212471507179544, -0.6427876096865405842, -0.005961354470445141482 ) ) ;
#34558=EDGE_CURVE ( 'NONE', #43904, #13447, #39095, .T. ) ;
#34560=DIRECTION ( 'NONE',  ( 0.9999697198139515519, 0.000000000000000000, 0.007781995580013368816 ) ) ;
#34561=DIRECTION ( 'NONE',  ( 0.005961354470445682716, -0.6427876096865404731, -0.7660212471507180654 ) ) ;
#34562=DIRECTION ( 'NONE',  ( -0.6427681459581293666, -0.7660444431189770143, -0.005002170337467561935 ) ) ;
#34563=CARTESIAN_POINT ( 'NONE',  ( -17.74560456716937296, 0.000000000000000000, 3.774316574337878372 ) ) ;
#34565=EDGE_LOOP ( 'NONE', ( #13583, #47610, #47572, #55713 ) ) ;
#34566=CARTESIAN_POINT ( 'NONE',  ( -12.06579791175127525, 0.000000000000000000, 2.341189863830586582 ) ) ;
#34567=ORIENTED_EDGE ( 'NONE', *, *, #43848, .F. ) ;
#34568=VECTOR ( 'NONE', #35183, 1000.000000000000000 ) ;
#34569=VECTOR ( 'NONE', #43433, 1000.000000000000000 ) ;
#34571=DIRECTION ( 'NONE',  ( -0.5364919789714478471, 0.6444004775717705469, -0.5449076811759709926 ) ) ;
#34572=DIRECTION ( 'NONE',  ( -0.6427681459581293666, -0.7660444431189770143, -0.005002170337467561935 ) ) ;
#34573=CARTESIAN_POINT ( 'NONE',  ( -19.16331067184377801, -0.1191753592594172323, 5.879273048348689024 ) ) ;
#34574=CARTESIAN_POINT ( 'NONE',  ( -18.31888538305858916, 0.000000000000000000, 3.939181184056494089 ) ) ;
#34576=FACE_OUTER_BOUND ( 'NONE', #29815, .T. ) ;
#34578=ORIENTED_EDGE ( 'NONE', *, *, #49239, .F. ) ;
#34579=LINE ( 'NONE', #17549, #25701 ) ;
#34580=DIRECTION ( 'NONE',  ( 0.005961354470445682716, -0.6427876096865404731, -0.7660212471507180654 ) ) ;
#34581=LINE ( 'NONE', #22091, #19139 ) ;
#34582=EDGE_CURVE ( 'NONE', #5827, #35406, #52444, .T. ) ;
#34583=LINE ( 'NONE', #789, #38210 ) ;
#34584=DIRECTION ( 'NONE',  ( -0.5449076811759708816, 0.6444004775717707689, 0.5364919789714475140 ) ) ;
#34585=EDGE_CURVE ( 'NONE', #18526, #36044, #47323, .T. ) ;
#34586=CARTESIAN_POINT ( 'NONE',  ( -29.86274838104827367, -0.1191753592594197858, 8.381332038739175871 ) ) ;
#34587=FACE_OUTER_BOUND ( 'NONE', #969, .T. ) ;
#34588=AXIS2_PLACEMENT_3D ( 'NONE', #55941, #51091, #13047 ) ;
#34589=FACE_OUTER_BOUND ( 'NONE', #43501, .T. ) ;
#34590=LINE ( 'NONE', #212, #35977 ) ;
#34592=ORIENTED_EDGE ( 'NONE', *, *, #48709, .T. ) ;
#34593=LINE ( 'NONE', #13326, #48263 ) ;
#34594=EDGE_CURVE ( 'NONE', #31864, #26534, #56143, .T. ) ;
#34595=ORIENTED_EDGE ( 'NONE', *, *, #33631, .T. ) ;
#34596=ADVANCED_FACE ( 'NONE', ( #30018 ), #17230, .F. ) ;
#34597=ORIENTED_EDGE ( 'NONE', *, *, #3914, .T. ) ;
#34598=EDGE_LOOP ( 'NONE', ( #9976, #48674, #7122, #55217 ) ) ;
#34599=ORIENTED_EDGE ( 'NONE', *, *, #25176, .T. ) ;
#34600=EDGE_LOOP ( 'NONE', ( #29701, #15216, #20686, #11350 ) ) ;
#34601=DIRECTION ( 'NONE',  ( -0.6427681459581293666, -0.7660444431189770143, -0.005002170337467561935 ) ) ;
#34602=LINE ( 'NONE', #18402, #27605 ) ;
#34603=VECTOR ( 'NONE', #12092, 1000.000000000000227 ) ;
#34604=VECTOR ( 'NONE', #55292, 999.9999999999998863 ) ;
#34605=ORIENTED_EDGE ( 'NONE', *, *, #18198, .T. ) ;
#34606=VECTOR ( 'NONE', #4442, 1000.000000000000227 ) ;
#34607=CARTESIAN_POINT ( 'NONE',  ( 2.072287782118878319, 0.000000000000000000, -2.950529333540147015 ) ) ;
#34608=ORIENTED_EDGE ( 'NONE', *, *, #32486, .F. ) ;
#34609=LINE ( 'NONE', #51927, #37294 ) ;
#34610=LINE ( 'NONE', #16743, #34999 ) ;
#34611=ORIENTED_EDGE ( 'NONE', *, *, #29677, .F. ) ;
#34612=CARTESIAN_POINT ( 'NONE',  ( -13.63673279712320507, -0.1191753592594197858, 12.22739664767016521 ) ) ;
#34613=ADVANCED_FACE ( 'NONE', ( #25758 ), #26594, .F. ) ;
#34614=ORIENTED_EDGE ( 'NONE', *, *, #43984, .T. ) ;
#34615=CARTESIAN_POINT ( 'NONE',  ( -19.12962290826653700, 0.000000000000000000, 14.40064212555863854 ) ) ;
#34616=VECTOR ( 'NONE', #43376, 1000.000000000000227 ) ;
#34617=EDGE_CURVE ( 'NONE', #30608, #3673, #48160, .T. ) ;
#34618=EDGE_CURVE ( 'NONE', #19103, #50804, #4199, .T. ) ;
#34619=VECTOR ( 'NONE', #50746, 999.9999999999998863 ) ;
#34620=CARTESIAN_POINT ( 'NONE',  ( -16.76521749764649982, 0.000000000000000000, 9.121921164085227574 ) ) ;
#34622=DIRECTION ( 'NONE',  ( 0.000000000000000000, -0.000000000000000000, -1.000000000000000000 ) ) ;
#34623=CARTESIAN_POINT ( 'NONE',  ( -16.81190032086591302, 0.000000000000000000, 3.212244750653343583 ) ) ;
#34624=CARTESIAN_POINT ( 'NONE',  ( -13.53673582514181106, 0.000000000000000000, 12.22817484722816772 ) ) ;
#34625=LINE ( 'NONE', #38325, #5674 ) ;
#34626=ORIENTED_EDGE ( 'NONE', *, *, #43840, .F. ) ;
#34627=CARTESIAN_POINT ( 'NONE',  ( -15.53549445463335488, 0.000000000000000000, 4.530180301885105010 ) ) ;
#34628=DIRECTION ( 'NONE',  ( 0.9999697198139515519, 0.000000000000000000, 0.007781995580013368816 ) ) ;
#34629=FACE_OUTER_BOUND ( 'NONE', #45202, .T. ) ;
#34630=LINE ( 'NONE', #48241, #2373 ) ;
#34631=DIRECTION ( 'NONE',  ( 0.007781995580012662783, 0.000000000000000000, -0.9999697198139514409 ) ) ;
#34634=ADVANCED_FACE ( 'NONE', ( #35149 ), #8745, .F. ) ;
#34635=CARTESIAN_POINT ( 'NONE',  ( -16.53317331066696383, 0.000000000000000000, 13.31285208727739899 ) ) ;
#34637=ORIENTED_EDGE ( 'NONE', *, *, #21277, .T. ) ;
#34638=CARTESIAN_POINT ( 'NONE',  ( 0.000000000000000000, 0.000000000000000000, 0.000000000000000000 ) ) ;
#34639=LINE ( 'NONE', #26687, #49573 ) ;
#34640=ORIENTED_EDGE ( 'NONE', *, *, #32062, .T. ) ;
#34641=LINE ( 'NONE', #585, #30209 ) ;
#34642=CARTESIAN_POINT ( 'NONE',  ( -12.60458797795435615, 0.000000000000000000, 11.86609696750642229 ) ) ;
#34644=AXIS2_PLACEMENT_3D ( 'NONE', #22694, #39752, #45133 ) ;
#34645=CARTESIAN_POINT ( 'NONE',  ( -14.94760462649100496, 0.000000000000000000, 2.488088991209854051 ) ) ;
#34646=EDGE_CURVE ( 'NONE', #27953, #36809, #38240, .T. ) ;
#34647=CARTESIAN_POINT ( 'NONE',  ( -12.84690689054629154, -1.489407457353159048, 1.823976140470426444 ) ) ;
#34648=DIRECTION ( 'NONE',  ( 0.6427681459581294776, -0.7660444431189769032, 0.005002170337467562802 ) ) ;
#34649=ORIENTED_EDGE ( 'NONE', *, *, #27903, .T. ) ;
#34650=VECTOR ( 'NONE', #9663, 1000.000000000000227 ) ;
#34651=ORIENTED_EDGE ( 'NONE', *, *, #32956, .F. ) ;
#34652=EDGE_CURVE ( 'NONE', #27029, #39457, #16670, .T. ) ;
#34653=FACE_OUTER_BOUND ( 'NONE', #12086, .T. ) ;
#34654=CARTESIAN_POINT ( 'NONE',  ( -12.13851405436063047, 0.000000000000000000, 11.68505802764555135 ) ) ;
#34655=ORIENTED_EDGE ( 'NONE', *, *, #54063, .T. ) ;
#34656=PLANE ( 'NONE',  #1187 ) ;
#34657=EDGE_LOOP ( 'NONE', ( #32104, #43461, #41004, #47685 ) ) ;
#34658=PLANE ( 'NONE',  #54879 ) ;
#34659=ADVANCED_FACE ( 'NONE', ( #39385 ), #12439, .F. ) ;
#34660=AXIS2_PLACEMENT_3D ( 'NONE', #22900, #18081, #30859 ) ;
#34661=ORIENTED_EDGE ( 'NONE', *, *, #3965, .T. ) ;
#34662=LINE ( 'NONE', #13097, #20195 ) ;
#34663=ORIENTED_EDGE ( 'NONE', *, *, #11076, .T. ) ;
#34664=ORIENTED_EDGE ( 'NONE', *, *, #5494, .F. ) ;
#34665=VERTEX_POINT ( 'NONE', #35997 ) ;
#34666=PLANE ( 'NONE',  #49294 ) ;
#34667=DIRECTION ( 'NONE',  ( 0.005961354470445682716, -0.6427876096865404731, -0.7660212471507180654 ) ) ;
#34668=DIRECTION ( 'NONE',  ( 0.005961354470445682716, -0.6427876096865404731, -0.7660212471507180654 ) ) ;
#34669=EDGE_CURVE ( 'NONE', #9132, #28372, #27737, .T. ) ;
#34670=CARTESIAN_POINT ( 'NONE',  ( -17.73140113748535285, 0.000000000000000000, 13.85752530597602039 ) ) ;
#34671=ORIENTED_EDGE ( 'NONE', *, *, #34073, .T. ) ;
#34672=ORIENTED_EDGE ( 'NONE', *, *, #24608, .F. ) ;
#34673=VECTOR ( 'NONE', #40394, 1000.000000000000227 ) ;
#34674=ADVANCED_FACE ( 'NONE', ( #22363 ), #13806, .F. ) ;
#34675=EDGE_CURVE ( 'NONE', #47218, #18585, #53304, .T. ) ;
#34676=ORIENTED_EDGE ( 'NONE', *, *, #47103, .F. ) ;
#34677=CARTESIAN_POINT ( 'NONE',  ( -13.66832470675316635, 0.000000000000000000, 3.436714839183848458 ) ) ;
#34678=VERTEX_POINT ( 'NONE', #49597 ) ;
#34679=AXIS2_PLACEMENT_3D ( 'NONE', #49761, #2026, #49187 ) ;
#34680=CARTESIAN_POINT ( 'NONE',  ( -21.47263955680318404, 0.000000000000000000, 5.022634149262071190 ) ) ;
#34681=EDGE_CURVE ( 'NONE', #2187, #21767, #14940, .T. ) ;
#34682=ORIENTED_EDGE ( 'NONE', *, *, #3906, .F. ) ;
#34683=CARTESIAN_POINT ( 'NONE',  ( -18.72454025655023813, -0.1191753592594158168, 9.206676289436575900 ) ) ;
#34684=CARTESIAN_POINT ( 'NONE',  ( -23.33849165029409889, 0.000000000000000000, 5.946783852668351855 ) ) ;
#34685=VECTOR ( 'NONE', #49052, 999.9999999999998863 ) ;
#34686=AXIS2_PLACEMENT_3D ( 'NONE', #2987, #3296, #29116 ) ;
#34687=EDGE_LOOP ( 'NONE', ( #21444, #36239, #56085, #36935 ) ) ;
#34688=EDGE_CURVE ( 'NONE', #34917, #27150, #31443, .T. ) ;
#34689=DIRECTION ( 'NONE',  ( -0.005002170337468016433, -0.7660444431189770143, 0.6427681459581293666 ) ) ;
#34690=ORIENTED_EDGE ( 'NONE', *, *, #27536, .F. ) ;
#34691=EDGE_CURVE ( 'NONE', #39023, #1495, #53829, .T. ) ;
#34692=VECTOR ( 'NONE', #8793, 1000.000000000000227 ) ;
#34694=VECTOR ( 'NONE', #2514, 999.9999999999998863 ) ;
#34696=LINE ( 'NONE', #30467, #34090 ) ;
#34697=CARTESIAN_POINT ( 'NONE',  ( -23.33693525117809386, 0.000000000000000000, 5.746789908705562944 ) ) ;
#34698=LINE ( 'NONE', #29894, #9236 ) ;
#34699=ORIENTED_EDGE ( 'NONE', *, *, #38991, .F. ) ;
#34700=EDGE_CURVE ( 'NONE', #55928, #17587, #48456, .T. ) ;
#34701=LINE ( 'NONE', #21914, #16606 ) ;
#34702=ADVANCED_FACE ( 'NONE', ( #22625 ), #40524, .F. ) ;
#34703=CARTESIAN_POINT ( 'NONE',  ( -10.00813838035478298, 0.000000000000000000, 10.77830692922518452 ) ) ;
#34704=CARTESIAN_POINT ( 'NONE',  ( -9.908141408373387193, -0.1191753592594197858, 10.77908512878318703 ) ) ;
#34705=DIRECTION ( 'NONE',  ( 0.5449076811759707706, 0.6444004775717708799, -0.5364919789714476250 ) ) ;
#34706=VECTOR ( 'NONE', #16810, 1000.000000000000000 ) ;
#34707=CARTESIAN_POINT ( 'NONE',  ( 2.072287782118878319, 0.000000000000000000, -2.950529333540147015 ) ) ;
#34708=CARTESIAN_POINT ( 'NONE',  ( -24.26908309836554878, 0.000000000000000000, 6.108867788427308376 ) ) ;
#34709=ADVANCED_FACE ( 'NONE', ( #26898 ), #6167, .F. ) ;
#34710=DIRECTION ( 'NONE',  ( 0.5364919789714477361, 0.6444004775717706579, 0.5449076811759711036 ) ) ;
#34712=FACE_OUTER_BOUND ( 'NONE', #33624, .T. ) ;
#34713=LINE ( 'NONE', #52030, #34962 ) ;
#34714=CARTESIAN_POINT ( 'NONE',  ( -27.06552663992790997, 0.000000000000000000, 7.195101427592543786 ) ) ;
#34715=EDGE_LOOP ( 'NONE', ( #53506, #14018, #25172, #37403 ) ) ;
#34716=DIRECTION ( 'NONE',  ( 0.007781995580012662783, 0.000000000000000000, -0.9999697198139514409 ) ) ;
#34717=PLANE ( 'NONE',  #34082 ) ;
#34718=ORIENTED_EDGE ( 'NONE', *, *, #45213, .F. ) ;
#34719=AXIS2_PLACEMENT_3D ( 'NONE', #29761, #10115, #14116 ) ;
#34720=CARTESIAN_POINT ( 'NONE',  ( -17.73140113748535285, 0.000000000000000000, 13.85752530597602039 ) ) ;
#34721=DIRECTION ( 'NONE',  ( 0.9999697198139515519, 0.000000000000000000, 0.007781995580013368816 ) ) ;
#34722=VECTOR ( 'NONE', #38075, 999.9999999999998863 ) ;
#34723=FACE_OUTER_BOUND ( 'NONE', #36846, .T. ) ;
#34725=ORIENTED_EDGE ( 'NONE', *, *, #17283, .F. ) ;
#34726=ORIENTED_EDGE ( 'NONE', *, *, #50958, .T. ) ;
#34727=FACE_OUTER_BOUND ( 'NONE', #9904, .T. ) ;
#34728=DIRECTION ( 'NONE',  ( 0.5449076811759707706, 0.6444004775717708799, -0.5364919789714476250 ) ) ;
#34729=VECTOR ( 'NONE', #4317, 1000.000000000000227 ) ;
#34730=LINE ( 'NONE', #34454, #38666 ) ;
#34731=VECTOR ( 'NONE', #6138, 999.9999999999998863 ) ;
#34732=CARTESIAN_POINT ( 'NONE',  ( -15.96710241509184058, -0.1191753592594218814, 13.13259134697452879 ) ) ;
#34733=AXIS2_PLACEMENT_3D ( 'NONE', #10659, #37034, #11171 ) ;
#34734=FACE_OUTER_BOUND ( 'NONE', #48754, .T. ) ;
#34735=LINE ( 'NONE', #9760, #26709 ) ;
#34736=EDGE_CURVE ( 'NONE', #44414, #49377, #35400, .T. ) ;
#34737=EDGE_LOOP ( 'NONE', ( #45122, #53149, #27855, #46468 ) ) ;
#34739=VECTOR ( 'NONE', #35969, 1000.000000000000114 ) ;
#34740=DIRECTION ( 'NONE',  ( -0.5364919789714478471, 0.6444004775717705469, -0.5449076811759709926 ) ) ;
#34741=VECTOR ( 'NONE', #39257, 1000.000000000000114 ) ;
#34742=VERTEX_POINT ( 'NONE', #9574 ) ;
#34743=DIRECTION ( 'NONE',  ( -0.5364919789714478471, 0.6444004775717705469, -0.5449076811759709926 ) ) ;
#34744=LINE ( 'NONE', #48931, #54035 ) ;
#34745=LINE ( 'NONE', #12884, #53818 ) ;
#34746=ADVANCED_FACE ( 'NONE', ( #44756 ), #18345, .F. ) ;
#34747=VERTEX_POINT ( 'NONE', #48758 ) ;
#34748=CARTESIAN_POINT ( 'NONE',  ( -10.23156040681847045, 0.000000000000000000, 5.479446896259717370 ) ) ;
#34749=VECTOR ( 'NONE', #17594, 1000.000000000000114 ) ;
#34750=ORIENTED_EDGE ( 'NONE', *, *, #26458, .F. ) ;
#34751=ADVANCED_FACE ( 'NONE', ( #9857 ), #52704, .F. ) ;
#34753=EDGE_CURVE ( 'NONE', #883, #49206, #14399, .T. ) ;
#34754=ORIENTED_EDGE ( 'NONE', *, *, #37201, .F. ) ;
#34755=ORIENTED_EDGE ( 'NONE', *, *, #43529, .F. ) ;
#34756=EDGE_LOOP ( 'NONE', ( #40762, #24697, #4913, #53966 ) ) ;
#34758=ORIENTED_EDGE ( 'NONE', *, *, #27351, .F. ) ;
#34759=VECTOR ( 'NONE', #39617, 1000.000000000000227 ) ;
#34761=ORIENTED_EDGE ( 'NONE', *, *, #44278, .T. ) ;
#34762=LINE ( 'NONE', #52918, #33143 ) ;
#34763=ADVANCED_FACE ( 'NONE', ( #22893 ), #44467, .F. ) ;
#34764=ORIENTED_EDGE ( 'NONE', *, *, #6882, .F. ) ;
#34765=FACE_OUTER_BOUND ( 'NONE', #3541, .T. ) ;
#34766=VECTOR ( 'NONE', #36697, 1000.000000000000227 ) ;
#34767=EDGE_LOOP ( 'NONE', ( #55339, #29409, #18603, #5415 ) ) ;
#34768=EDGE_CURVE ( 'NONE', #28225, #12315, #40220, .T. ) ;
#34769=PLANE ( 'NONE',  #49273 ) ;
#34770=CARTESIAN_POINT ( 'NONE',  ( -9.542064456761055524, 0.000000000000000000, 10.59726798936431180 ) ) ;
#34771=DIRECTION ( 'NONE',  ( 0.7660212471507180654, -0.6427876096865404731, 0.005961354470445141482 ) ) ;
#34772=CARTESIAN_POINT ( 'NONE',  ( -22.40634380310664397, 0.000000000000000000, 5.584705972946605534 ) ) ;
#34773=AXIS2_PLACEMENT_3D ( 'NONE', #51776, #25665, #29933 ) ;
#34774=LINE ( 'NONE', #43844, #38305 ) ;
#34775=EDGE_LOOP ( 'NONE', ( #30360, #44319, #37180, #19879 ) ) ;
#34777=EDGE_CURVE ( 'NONE', #46860, #55008, #33634, .T. ) ;
#34778=VECTOR ( 'NONE', #20097, 1000.000000000000227 ) ;
#34779=VERTEX_POINT ( 'NONE', #24850 ) ;
#34780=LINE ( 'NONE', #4963, #8651 ) ;
#34781=PLANE ( 'NONE',  #3994 ) ;
#34782=CARTESIAN_POINT ( 'NONE',  ( -16.53317331066696383, 0.000000000000000000, 13.31285208727739899 ) ) ;
#34783=EDGE_CURVE ( 'NONE', #30486, #9050, #24552, .T. ) ;
#34784=VECTOR ( 'NONE', #17089, 1000.000000000000114 ) ;
#34785=AXIS2_PLACEMENT_3D ( 'NONE', #22089, #13571, #30881 ) ;
#34786=CARTESIAN_POINT ( 'NONE',  ( -11.59541290789961998, 0.000000000000000000, 1.606186369083069332 ) ) ;
#34787=DIRECTION ( 'NONE',  ( 0.007781995580012663651, 0.000000000000000000, -0.9999697198139515519 ) ) ;
#34788=DIRECTION ( 'NONE',  ( 0.000000000000000000, -0.000000000000000000, -1.000000000000000000 ) ) ;
#34789=ORIENTED_EDGE ( 'NONE', *, *, #13393, .F. ) ;
#34790=DIRECTION ( 'NONE',  ( -0.005002170337468016433, -0.7660444431189770143, 0.6427681459581293666 ) ) ;
#34791=DIRECTION ( 'NONE',  ( -0.6427681459581293666, -0.7660444431189770143, -0.005002170337467561935 ) ) ;
#34792=VERTEX_POINT ( 'NONE', #7520 ) ;
#34793=DIRECTION ( 'NONE',  ( 0.7660212471507180654, -0.6427876096865404731, 0.005961354470445141482 ) ) ;
#34794=PLANE ( 'NONE',  #36022 ) ;
#34795=CARTESIAN_POINT ( 'NONE',  ( -14.12433944307840861, 0.000000000000000000, 2.325169817642546821 ) ) ;
#34796=CARTESIAN_POINT ( 'NONE',  ( -17.49039288222042998, 0.1245042932765029059, 3.471821964380750192 ) ) ;
#34797=CARTESIAN_POINT ( 'NONE',  ( 2.072287782118878319, 0.000000000000000000, -2.950529333540147015 ) ) ;
#34798=EDGE_LOOP ( 'NONE', ( #42764, #49261, #45031, #36946 ) ) ;
#34799=VECTOR ( 'NONE', #27569, 1000.000000000000227 ) ;
#34801=FACE_OUTER_BOUND ( 'NONE', #19491, .T. ) ;
#34802=CARTESIAN_POINT ( 'NONE',  ( -16.43317633868556626, -0.1191753592594197858, 13.31363028683540151 ) ) ;
#34803=LINE ( 'NONE', #17780, #7948 ) ;
#34804=EDGE_CURVE ( 'NONE', #25674, #19445, #16063, .T. ) ;
#34805=VECTOR ( 'NONE', #7598, 1000.000000000000000 ) ;
#34806=DIRECTION ( 'NONE',  ( 0.5449076811759707706, 0.6444004775717708799, -0.5364919789714476250 ) ) ;
#34807=LINE ( 'NONE', #52963, #29432 ) ;
#34808=EDGE_CURVE ( 'NONE', #21782, #35835, #50110, .T. ) ;
#34809=VECTOR ( 'NONE', #185, 999.9999999999998863 ) ;
#34810=LINE ( 'NONE', #18615, #54535 ) ;
#34811=LINE ( 'NONE', #52674, #43802 ) ;
#34813=CARTESIAN_POINT ( 'NONE',  ( -17.03126345885748449, 4.010151117816511679, 3.169508026948365309 ) ) ;
#34814=LINE ( 'NONE', #13249, #36930 ) ;
#34815=EDGE_CURVE ( 'NONE', #7643, #43820, #15232, .T. ) ;
#34816=ADVANCED_FACE ( 'NONE', ( #7248 ), #15757, .F. ) ;
#34817=VECTOR ( 'NONE', #52296, 999.9999999999998863 ) ;
#34819=DIRECTION ( 'NONE',  ( -0.9999697198139514409, -0.000000000000000000, -0.007781995580013368816 ) ) ;
#34820=VERTEX_POINT ( 'NONE', #28008 ) ;
#34821=CARTESIAN_POINT ( 'NONE',  ( -18.86354292863559579, 0.000000000000000000, 14.21804678658176080 ) ) ;
#34822=EDGE_CURVE ( 'NONE', #45853, #48933, #11527, .T. ) ;
#34823=ADVANCED_FACE ( 'NONE', ( #10946 ), #28844, .F. ) ;
#34824=CARTESIAN_POINT ( 'NONE',  ( -30.79411802867772607, 0.000000000000000000, 8.643412946479525516 ) ) ;
#34825=EDGE_CURVE ( 'NONE', #50938, #37343, #24297, .T. ) ;
#34826=VECTOR ( 'NONE', #25844, 999.9999999999998863 ) ;
#34827=ORIENTED_EDGE ( 'NONE', *, *, #26977, .F. ) ;
#34828=VERTEX_POINT ( 'NONE', #16315 ) ;
#34829=VECTOR ( 'NONE', #15052, 1000.000000000000114 ) ;
#34830=ORIENTED_EDGE ( 'NONE', *, *, #39394, .T. ) ;
#34831=VERTEX_POINT ( 'NONE', #54379 ) ;
#34833=ORIENTED_EDGE ( 'NONE', *, *, #17019, .T. ) ;
#34834=VERTEX_POINT ( 'NONE', #32545 ) ;
#34835=DIRECTION ( 'NONE',  ( 0.007781995580012663651, 0.000000000000000000, -0.9999697198139515519 ) ) ;
#34836=CARTESIAN_POINT ( 'NONE',  ( -19.26540349777245353, 0.000000000000000000, 6.147807580067062183 ) ) ;
#34837=LINE ( 'NONE', #38826, #6808 ) ;
#34838=EDGE_LOOP ( 'NONE', ( #7164, #56202, #417, #14029 ) ) ;
#34839=DIRECTION ( 'NONE',  ( 0.9999697198139515519, 0.000000000000000000, 0.007781995580013368816 ) ) ;
#34840=EDGE_CURVE ( 'NONE', #5501, #53603, #23725, .T. ) ;
#34841=ORIENTED_EDGE ( 'NONE', *, *, #37121, .T. ) ;
#34842=ORIENTED_EDGE ( 'NONE', *, *, #48806, .T. ) ;
#34843=EDGE_CURVE ( 'NONE', #5277, #27412, #46407, .T. ) ;
#34844=VECTOR ( 'NONE', #49141, 1000.000000000000000 ) ;
#34845=DIRECTION ( 'NONE',  ( 0.9999697198139515519, 0.000000000000000000, 0.007781995580013368816 ) ) ;
#34846=VECTOR ( 'NONE', #19092, 1000.000000000000227 ) ;
#34847=FACE_OUTER_BOUND ( 'NONE', #54395, .T. ) ;
#34848=ADVANCED_FACE ( 'NONE', ( #20607 ), #45578, .F. ) ;
#34849=DIRECTION ( 'NONE',  ( -0.005002170337468016433, -0.7660444431189770143, 0.6427681459581293666 ) ) ;
#34850=ORIENTED_EDGE ( 'NONE', *, *, #46601, .F. ) ;
#34851=DIRECTION ( 'NONE',  ( 0.9321478471874540261, 0.000000000000000000, -0.3620778797217457101 ) ) ;
#34852=VECTOR ( 'NONE', #32207, 999.9999999999998863 ) ;
#34853=EDGE_LOOP ( 'NONE', ( #49673, #47955, #33547, #358 ) ) ;
#34854=EDGE_CURVE ( 'NONE', #14573, #26718, #37919, .T. ) ;
#34855=CARTESIAN_POINT ( 'NONE',  ( -16.30618749709877591, 2.553033558614006271, 7.405161117131130233 ) ) ;
#34856=DIRECTION ( 'NONE',  ( 0.005002170337468016433, -0.7660444431189770143, -0.6427681459581293666 ) ) ;
#34857=AXIS2_PLACEMENT_3D ( 'NONE', #8434, #8162, #13542 ) ;
#34859=DIRECTION ( 'NONE',  ( -0.7660212471507179544, -0.6427876096865405842, -0.005961354470445141482 ) ) ;
#34860=DIRECTION ( 'NONE',  ( -0.005002170337468016433, -0.7660444431189770143, 0.6427681459581293666 ) ) ;
#34861=DIRECTION ( 'NONE',  ( 0.007781995580012662783, 0.000000000000000000, -0.9999697198139514409 ) ) ;
#34863=FACE_OUTER_BOUND ( 'NONE', #22032, .T. ) ;
#34864=VECTOR ( 'NONE', #22111, 1000.000000000000227 ) ;
#34866=ORIENTED_EDGE ( 'NONE', *, *, #42834, .F. ) ;
#34867=CARTESIAN_POINT ( 'NONE',  ( -20.54204810873173415, 0.000000000000000000, 4.860550213503115558 ) ) ;
#34868=VECTOR ( 'NONE', #4214, 1000.000000000000227 ) ;
#34869=LINE ( 'NONE', #52723, #31989 ) ;
#34870=FACE_OUTER_BOUND ( 'NONE', #52059, .T. ) ;
#34871=LINE ( 'NONE', #3910, #25395 ) ;
#34872=DIRECTION ( 'NONE',  ( -0.7660212471507179544, -0.6427876096865405842, -0.005961354470445141482 ) ) ;
#34873=DIRECTION ( 'NONE',  ( -0.9999697198139514409, -0.000000000000000000, -0.007781995580013368816 ) ) ;
#34875=VECTOR ( 'NONE', #35185, 999.9999999999998863 ) ;
#34876=DIRECTION ( 'NONE',  ( 0.007781995580012662783, 0.000000000000000000, -0.9999697198139514409 ) ) ;
#34877=VECTOR ( 'NONE', #3556, 999.9999999999998863 ) ;
#34879=ORIENTED_EDGE ( 'NONE', *, *, #55381, .T. ) ;
#34880=DIRECTION ( 'NONE',  ( 0.6427681459581294776, -0.7660444431189769032, 0.005002170337467562802 ) ) ;
#34881=DIRECTION ( 'NONE',  ( -0.005002170337468016433, -0.7660444431189770143, 0.6427681459581293666 ) ) ;
#34882=CARTESIAN_POINT ( 'NONE',  ( -8.273148203881921958, 0.000000000000000000, 5.694693769082166845 ) ) ;
#34883=LINE ( 'NONE', #47359, #45420 ) ;
#34884=DIRECTION ( 'NONE',  ( 0.000000000000000000, -0.000000000000000000, -1.000000000000000000 ) ) ;
#34885=EDGE_CURVE ( 'NONE', #38344, #1220, #2689, .T. ) ;
#34886=CARTESIAN_POINT ( 'NONE',  ( -13.08934823687588889, -0.1166911823299076612, 1.865973795676008073 ) ) ;
#34887=CARTESIAN_POINT ( 'NONE',  ( -20.18930731220519093, -2.460819163488159766, 4.645020693886293905 ) ) ;
#34888=VECTOR ( 'NONE', #34190, 999.9999999999998863 ) ;
#34889=DIRECTION ( 'NONE',  ( -0.7660212471507179544, -0.6427876096865405842, -0.005961354470445141482 ) ) ;
#34890=EDGE_CURVE ( 'NONE', #9132, #55490, #55228, .T. ) ;
#34891=PLANE ( 'NONE',  #16121 ) ;
#34892=AXIS2_PLACEMENT_3D ( 'NONE', #8510, #38048, #30086 ) ;
#34893=ORIENTED_EDGE ( 'NONE', *, *, #52536, .T. ) ;
#34894=CARTESIAN_POINT ( 'NONE',  ( -14.01545677930355183, 0.000000000000000000, 2.126011111488108174 ) ) ;
#34895=VECTOR ( 'NONE', #16844, 999.9999999999998863 ) ;
#34896=EDGE_CURVE ( 'NONE', #38597, #21963, #2435, .T. ) ;
#34897=EDGE_CURVE ( 'NONE', #2279, #43270, #28548, .T. ) ;
#34898=ADVANCED_FACE ( 'NONE', ( #34238 ), #30537, .F. ) ;
#34899=EDGE_LOOP ( 'NONE', ( #17355, #7879, #13767, #13804 ) ) ;
#34900=AXIS2_PLACEMENT_3D ( 'NONE', #40368, #17667, #31838 ) ;
#34901=ADVANCED_FACE ( 'NONE', ( #47552 ), #4666, .F. ) ;
#34902=ORIENTED_EDGE ( 'NONE', *, *, #12284, .T. ) ;
#34903=ORIENTED_EDGE ( 'NONE', *, *, #41617, .T. ) ;
#34904=VECTOR ( 'NONE', #18946, 999.9999999999998863 ) ;
#34905=ORIENTED_EDGE ( 'NONE', *, *, #41760, .T. ) ;
#34906=VECTOR ( 'NONE', #35144, 999.9999999999998863 ) ;
#34907=ORIENTED_EDGE ( 'NONE', *, *, #21508, .T. ) ;
#34908=CARTESIAN_POINT ( 'NONE',  ( -12.33850799832341849, 0.000000000000000000, 11.68350162852954632 ) ) ;
#34909=FACE_OUTER_BOUND ( 'NONE', #10039, .T. ) ;
#34910=VECTOR ( 'NONE', #27891, 1000.000000000000000 ) ;
#34911=VERTEX_POINT ( 'NONE', #4119 ) ;
#34912=ORIENTED_EDGE ( 'NONE', *, *, #18101, .F. ) ;
#34913=EDGE_CURVE ( 'NONE', #22163, #37012, #46709, .T. ) ;
#34914=VECTOR ( 'NONE', #41230, 999.9999999999998863 ) ;
#34915=VECTOR ( 'NONE', #29105, 999.9999999999998863 ) ;
#34916=DIRECTION ( 'NONE',  ( 0.000000000000000000, -0.000000000000000000, -1.000000000000000000 ) ) ;
#34917=VERTEX_POINT ( 'NONE', #13199 ) ;
#34918=EDGE_CURVE ( 'NONE', #6114, #44308, #25994, .T. ) ;
#34919=DIRECTION ( 'NONE',  ( 0.6427681459581294776, -0.7660444431189769032, 0.005002170337467562802 ) ) ;
#34920=DIRECTION ( 'NONE',  ( 0.9999697198139515519, 0.000000000000000000, 0.007781995580013368816 ) ) ;
#34921=EDGE_LOOP ( 'NONE', ( #42741, #14593, #11049, #31616 ) ) ;
#34922=FACE_OUTER_BOUND ( 'NONE', #6265, .T. ) ;
#34923=ORIENTED_EDGE ( 'NONE', *, *, #2743, .F. ) ;
#34924=ADVANCED_FACE ( 'NONE', ( #52089 ), #8950, .F. ) ;
#34925=DIRECTION ( 'NONE',  ( 0.9999697198139515519, 0.000000000000000000, 0.007781995580013368816 ) ) ;
#34926=EDGE_CURVE ( 'NONE', #24834, #11836, #20860, .T. ) ;
#34927=VECTOR ( 'NONE', #42277, 1000.000000000000227 ) ;
#34928=CARTESIAN_POINT ( 'NONE',  ( -30.79411802867772607, 0.000000000000000000, 8.643412946479525516 ) ) ;
#34929=EDGE_LOOP ( 'NONE', ( #6584, #36347, #36351, #36165 ) ) ;
#34930=LINE ( 'NONE', #26379, #37645 ) ;
#34931=DIRECTION ( 'NONE',  ( 0.007781995580012663651, 0.000000000000000000, -0.9999697198139515519 ) ) ;
#34932=PLANE ( 'NONE',  #23026 ) ;
#34933=VECTOR ( 'NONE', #5567, 1000.000000000000227 ) ;
#34934=VERTEX_POINT ( 'NONE', #39030 ) ;
#34935=LINE ( 'NONE', #254, #10167 ) ;
#34936=ORIENTED_EDGE ( 'NONE', *, *, #35615, .F. ) ;
#34937=VECTOR ( 'NONE', #49676, 1000.000000000000114 ) ;
#34938=PLANE ( 'NONE',  #7450 ) ;
#34939=CARTESIAN_POINT ( 'NONE',  ( -17.36532418587302473, -0.1191753592594177458, 13.67570816655714516 ) ) ;
#34940=LINE ( 'NONE', #43999, #5020 ) ;
#34941=CARTESIAN_POINT ( 'NONE',  ( -30.79411802867772607, 0.000000000000000000, 8.643412946479525516 ) ) ;
#34942=AXIS2_PLACEMENT_3D ( 'NONE', #55730, #51488, #52024 ) ;
#34943=PLANE ( 'NONE',  #24106 ) ;
#34946=CARTESIAN_POINT ( 'NONE',  ( -19.35744109503886889, -4.241740624735664156, 4.265074886081953842 ) ) ;
#34947=VECTOR ( 'NONE', #46498, 999.9999999999998863 ) ;
#34948=VECTOR ( 'NONE', #46350, 999.9999999999998863 ) ;
#34950=VECTOR ( 'NONE', #18825, 999.9999999999998863 ) ;
#34951=PLANE ( 'NONE',  #18721 ) ;
#34952=ORIENTED_EDGE ( 'NONE', *, *, #7814, .T. ) ;
#34953=CARTESIAN_POINT ( 'NONE',  ( -15.87975247367846166, 0.000000000000000000, 2.850166870931599927 ) ) ;
#34954=LINE ( 'NONE', #47994, #975 ) ;
#34955=LINE ( 'NONE', #21866, #14164 ) ;
#34956=AXIS2_PLACEMENT_3D ( 'NONE', #21237, #7616, #194 ) ;
#34957=PLANE ( 'NONE',  #1363 ) ;
#34958=CARTESIAN_POINT ( 'NONE',  ( -13.13452722693079444, -0.1191753592594185784, 7.403518714363871212 ) ) ;
#34959=PLANE ( 'NONE',  #46497 ) ;
#34960=ORIENTED_EDGE ( 'NONE', *, *, #6264, .F. ) ;
#34961=VECTOR ( 'NONE', #49184, 1000.000000000000227 ) ;
#34962=VECTOR ( 'NONE', #39557, 1000.000000000000227 ) ;
#34963=ORIENTED_EDGE ( 'NONE', *, *, #30144, .T. ) ;
#34964=DIRECTION ( 'NONE',  ( 0.6427681459581294776, -0.7660444431189769032, 0.005002170337467562802 ) ) ;
#34965=FACE_OUTER_BOUND ( 'NONE', #1720, .T. ) ;
#34966=VERTEX_POINT ( 'NONE', #3547 ) ;
#34967=LINE ( 'NONE', #39198, #2116 ) ;
#34968=EDGE_CURVE ( 'NONE', #50596, #38457, #8365, .T. ) ;
#34969=ORIENTED_EDGE ( 'NONE', *, *, #55381, .F. ) ;
#34970=CARTESIAN_POINT ( 'NONE',  ( -14.20280369269832832, 0.000000000000000000, 12.40765738797303719 ) ) ;
#34971=ORIENTED_EDGE ( 'NONE', *, *, #40668, .T. ) ;
#34972=FACE_OUTER_BOUND ( 'NONE', #8732, .T. ) ;
#34973=ADVANCED_FACE ( 'NONE', ( #17436 ), #34769, .F. ) ;
#34974=EDGE_CURVE ( 'NONE', #51694, #23998, #55494, .T. ) ;
#34975=AXIS2_PLACEMENT_3D ( 'NONE', #36773, #49558, #1571 ) ;
#34976=ORIENTED_EDGE ( 'NONE', *, *, #12744, .F. ) ;
#34977=ORIENTED_EDGE ( 'NONE', *, *, #15719, .F. ) ;
#34978=VERTEX_POINT ( 'NONE', #43563 ) ;
#34979=VECTOR ( 'NONE', #30951, 999.9999999999998863 ) ;
#34980=LINE ( 'NONE', #33832, #24805 ) ;
#34981=PLANE ( 'NONE',  #20512 ) ;
#34982=VECTOR ( 'NONE', #45075, 1000.000000000000227 ) ;
#34983=CARTESIAN_POINT ( 'NONE',  ( -14.00280974873554030, 0.000000000000000000, 12.40921378708904044 ) ) ;
#34984=PLANE ( 'NONE',  #39293 ) ;
#34985=ORIENTED_EDGE ( 'NONE', *, *, #34456, .T. ) ;
#34986=VECTOR ( 'NONE', #7136, 1000.000000000000227 ) ;
#34987=VERTEX_POINT ( 'NONE', #21137 ) ;
#34988=EDGE_LOOP ( 'NONE', ( #54592, #52447, #29210, #12444 ) ) ;
#34989=VECTOR ( 'NONE', #45186, 999.9999999999998863 ) ;
#34991=CARTESIAN_POINT ( 'NONE',  ( -11.18042193777012017, 0.9340140483890051470, 0.9949873626040346419 ) ) ;
#34992=ORIENTED_EDGE ( 'NONE', *, *, #11075, .T. ) ;
#34993=PLANE ( 'NONE',  #27542 ) ;
#34994=ORIENTED_EDGE ( 'NONE', *, *, #53359, .F. ) ;
#34995=DIRECTION ( 'NONE',  ( -0.005961354470445682716, -0.6427876096865404731, 0.7660212471507180654 ) ) ;
#34996=CARTESIAN_POINT ( 'NONE',  ( -16.46476824831552932, 0.000000000000000000, 4.522948478349086088 ) ) ;
#34997=AXIS2_PLACEMENT_3D ( 'NONE', #12080, #3303, #8389 ) ;
#34998=ORIENTED_EDGE ( 'NONE', *, *, #8027, .T. ) ;
#34999=VECTOR ( 'NONE', #38898, 1000.000000000000227 ) ;
#35000=DIRECTION ( 'NONE',  ( 0.007781995580012663651, 0.000000000000000000, -0.9999697198139515519 ) ) ;
#35001=VECTOR ( 'NONE', #5353, 999.9999999999998863 ) ;
#35002=VERTEX_POINT ( 'NONE', #21980 ) ;
#35003=EDGE_CURVE ( 'NONE', #9247, #49612, #25408, .T. ) ;
#35004=VECTOR ( 'NONE', #35379, 999.9999999999998863 ) ;
#35005=CARTESIAN_POINT ( 'NONE',  ( -27.99845268667336384, -0.1191753592594197858, 7.657176279295684118 ) ) ;
#35006=VECTOR ( 'NONE', #4492, 999.9999999999998863 ) ;
#35007=ORIENTED_EDGE ( 'NONE', *, *, #9900, .F. ) ;
#35008=EDGE_CURVE ( 'NONE', #25831, #19882, #29392, .T. ) ;
#35009=LINE ( 'NONE', #52575, #2374 ) ;
#35010=DIRECTION ( 'NONE',  ( 0.9999697198139515519, 0.000000000000000000, 0.007781995580013368816 ) ) ;
#35011=DIRECTION ( 'NONE',  ( 0.007781995580012662783, 0.000000000000000000, -0.9999697198139514409 ) ) ;
#35012=ORIENTED_EDGE ( 'NONE', *, *, #25394, .F. ) ;
#35013=LINE ( 'NONE', #13960, #30198 ) ;
#35014=DIRECTION ( 'NONE',  ( 0.000000000000000000, -0.000000000000000000, -1.000000000000000000 ) ) ;
#35016=CARTESIAN_POINT ( 'NONE',  ( -14.94760462649100496, 0.000000000000000000, 2.488088991209854051 ) ) ;
#35017=CARTESIAN_POINT ( 'NONE',  ( 2.072287782118878319, 0.000000000000000000, -2.950529333540147015 ) ) ;
#35018=CARTESIAN_POINT ( 'NONE',  ( -13.74590162550491890, -1.975113310420657520, 5.262804166939828221 ) ) ;
#35019=LINE ( 'NONE', #52329, #18858 ) ;
#35020=VECTOR ( 'NONE', #36696, 999.9999999999998863 ) ;
#35022=ORIENTED_EDGE ( 'NONE', *, *, #34968, .T. ) ;
#35023=CARTESIAN_POINT ( 'NONE',  ( -25.20278734466900517, 0.000000000000000000, 6.670939612111840944 ) ) ;
#35024=PLANE ( 'NONE',  #47684 ) ;
#35025=DIRECTION ( 'NONE',  ( 0.007781995580012662783, 0.000000000000000000, -0.9999697198139514409 ) ) ;
#35026=ORIENTED_EDGE ( 'NONE', *, *, #54155, .F. ) ;
#35027=CARTESIAN_POINT ( 'NONE',  ( -22.40556560354864146, -0.1191753592594197858, 5.484709000965211523 ) ) ;
#35028=DIRECTION ( 'NONE',  ( -0.7660212471507179544, -0.6427876096865405842, -0.005961354470445141482 ) ) ;
#35029=AXIS2_PLACEMENT_3D ( 'NONE', #56099, #17452, #34788 ) ;
#35030=EDGE_LOOP ( 'NONE', ( #1859, #19376, #41724, #42634 ) ) ;
#35031=PLANE ( 'NONE',  #14406 ) ;
#35032=CARTESIAN_POINT ( 'NONE',  ( -20.25347771009236908, -0.1191753592594193140, 5.501457046573825060 ) ) ;
#35033=VECTOR ( 'NONE', #11925, 1000.000000000000114 ) ;
#35034=DIRECTION ( 'NONE',  ( 0.9999697198139515519, 0.000000000000000000, 0.007781995580013368816 ) ) ;
#35035=CARTESIAN_POINT ( 'NONE',  ( -16.30304311551386931, -1.165603555308157846, 3.176787860902857918 ) ) ;
#35036=VERTEX_POINT ( 'NONE', #38771 ) ;
#35037=VECTOR ( 'NONE', #24105, 999.9999999999998863 ) ;
#35038=VECTOR ( 'NONE', #32727, 999.9999999999998863 ) ;
#35039=EDGE_LOOP ( 'NONE', ( #17662, #37909, #4002, #37852 ) ) ;
#35040=LINE ( 'NONE', #5471, #44831 ) ;
#35041=LINE ( 'NONE', #39837, #15944 ) ;
#35042=CARTESIAN_POINT ( 'NONE',  ( -15.13495153988577968, 0.000000000000000000, 12.76973526769478084 ) ) ;
#35043=EDGE_CURVE ( 'NONE', #1119, #29692, #400, .T. ) ;
#35046=DIRECTION ( 'NONE',  ( -0.5449076811759708816, 0.6444004775717707689, 0.5364919789714475140 ) ) ;
#35047=AXIS2_PLACEMENT_3D ( 'NONE', #24922, #20921, #21211 ) ;
#35048=CARTESIAN_POINT ( 'NONE',  ( 2.072287782118878319, 0.000000000000000000, -2.950529333540147015 ) ) ;
#35049=CARTESIAN_POINT ( 'NONE',  ( -10.63551161020563995, 0.2864062442990031321, 0.8039877656949352414 ) ) ;
#35050=ORIENTED_EDGE ( 'NONE', *, *, #32641, .T. ) ;
#35051=DIRECTION ( 'NONE',  ( 0.7660212471507180654, -0.6427876096865404731, 0.005961354470445141482 ) ) ;
#35052=EDGE_CURVE ( 'NONE', #2799, #55479, #29702, .T. ) ;
#35053=AXIS2_PLACEMENT_3D ( 'NONE', #27632, #10860, #11123 ) ;
#35054=VECTOR ( 'NONE', #25950, 999.9999999999998863 ) ;
#35055=CARTESIAN_POINT ( 'NONE',  ( -13.90497357559251590, 4.172053068839010947, 1.949985347149532533 ) ) ;
#35056=ORIENTED_EDGE ( 'NONE', *, *, #5023, .F. ) ;
#35058=DIRECTION ( 'NONE',  ( 0.9321478471874540261, 0.000000000000000000, -0.3620778797217457101 ) ) ;
#35059=LINE ( 'NONE', #52363, #29381 ) ;
#35060=ORIENTED_EDGE ( 'NONE', *, *, #13979, .T. ) ;
#35062=DIRECTION ( 'NONE',  ( 0.000000000000000000, 1.000000000000000000, 0.000000000000000000 ) ) ;
#35063=ORIENTED_EDGE ( 'NONE', *, *, #9501, .T. ) ;
#35064=AXIS2_PLACEMENT_3D ( 'NONE', #45291, #10922, #23444 ) ;
#35065=EDGE_CURVE ( 'NONE', #18119, #14885, #17172, .T. ) ;
#35066=VERTEX_POINT ( 'NONE', #47255 ) ;
#35067=ORIENTED_EDGE ( 'NONE', *, *, #36145, .T. ) ;
#35068=ORIENTED_EDGE ( 'NONE', *, *, #48998, .F. ) ;
#35069=FACE_OUTER_BOUND ( 'NONE', #47163, .T. ) ;
#35070=VECTOR ( 'NONE', #14286, 999.9999999999998863 ) ;
#35071=ORIENTED_EDGE ( 'NONE', *, *, #36270, .F. ) ;
#35072=LINE ( 'NONE', #39861, #27688 ) ;
#35073=ORIENTED_EDGE ( 'NONE', *, *, #7955, .F. ) ;
#35074=LINE ( 'NONE', #35332, #48583 ) ;
#35075=AXIS2_PLACEMENT_3D ( 'NONE', #38739, #42976, #56050 ) ;
#35076=ORIENTED_EDGE ( 'NONE', *, *, #27727, .T. ) ;
#35077=CARTESIAN_POINT ( 'NONE',  ( -14.10280672071693431, -0.1191753592594197858, 12.40843558753103792 ) ) ;
#35078=ORIENTED_EDGE ( 'NONE', *, *, #27574, .T. ) ;
#35079=VECTOR ( 'NONE', #41626, 1000.000000000000227 ) ;
#35080=CARTESIAN_POINT ( 'NONE',  ( -9.993945985744899119, -0.4219234865752066743, 1.264602792408272114 ) ) ;
#35081=DIRECTION ( 'NONE',  ( 0.007781995580012662783, 0.000000000000000000, -0.9999697198139514409 ) ) ;
#35082=LINE ( 'NONE', #42718, #43085 ) ;
#35083=DIRECTION ( 'NONE',  ( -0.9999697198139514409, -0.000000000000000000, -0.007781995580013368816 ) ) ;
#35084=CARTESIAN_POINT ( 'NONE',  ( -31.72782227498118601, 0.000000000000000000, 9.205484770164058972 ) ) ;
#35085=VERTEX_POINT ( 'NONE', #30237 ) ;
#35086=ORIENTED_EDGE ( 'NONE', *, *, #54254, .T. ) ;
#35087=VECTOR ( 'NONE', #35083, 1000.000000000000227 ) ;
#35088=CARTESIAN_POINT ( 'NONE',  ( -13.07066190154808361, 0.000000000000000000, 12.04713590736729678 ) ) ;
#35089=ADVANCED_FACE ( 'NONE', ( #48687 ), #53487, .F. ) ;
#35090=FACE_OUTER_BOUND ( 'NONE', #11553, .T. ) ;
#35091=VECTOR ( 'NONE', #17570, 999.9999999999998863 ) ;
#35092=PLANE ( 'NONE',  #35169 ) ;
#35093=AXIS2_PLACEMENT_3D ( 'NONE', #13629, #35790, #27538 ) ;
#35094=LINE ( 'NONE', #52395, #50279 ) ;
#35095=PLANE ( 'NONE',  #44874 ) ;
#35096=CARTESIAN_POINT ( 'NONE',  ( -8.397167190602280229, -10.18620209871003190, 6.480118481491868643 ) ) ;
#35097=EDGE_LOOP ( 'NONE', ( #15588, #50632, #44727, #10226 ) ) ;
#35098=CARTESIAN_POINT ( 'NONE',  ( -11.71762410836527479, -0.1191753592594190225, 4.459888823605786534 ) ) ;
#35099=CARTESIAN_POINT ( 'NONE',  ( -19.60990026154428278, 0.000000000000000000, 4.498472333781370125 ) ) ;
#35100=ORIENTED_EDGE ( 'NONE', *, *, #2556, .F. ) ;
#35101=EDGE_CURVE ( 'NONE', #36934, #20261, #35608, .T. ) ;
#35102=CARTESIAN_POINT ( 'NONE',  ( -16.04002523658126833, -0.8417996532631565332, 4.293958898594414819 ) ) ;
#35103=FACE_OUTER_BOUND ( 'NONE', #25362, .T. ) ;
#35104=LINE ( 'NONE', #52658, #20461 ) ;
#35105=ADVANCED_FACE ( 'NONE', ( #1535 ), #5505, .F. ) ;
#35106=EDGE_CURVE ( 'NONE', #12574, #21773, #14587, .T. ) ;
#35108=AXIS2_PLACEMENT_3D ( 'NONE', #32672, #44916, #49456 ) ;
#35109=CARTESIAN_POINT ( 'NONE',  ( -16.79925329029790149, 0.000000000000000000, 13.49544742625427496 ) ) ;
#35110=ORIENTED_EDGE ( 'NONE', *, *, #37841, .F. ) ;
#35111=ORIENTED_EDGE ( 'NONE', *, *, #1643, .T. ) ;
#35112=CARTESIAN_POINT ( 'NONE',  ( -30.79489622823572859, -0.1191753592594197858, 8.743409918460921304 ) ) ;
#35113=LINE ( 'NONE', #39344, #7717 ) ;
#35114=CARTESIAN_POINT ( 'NONE',  ( -16.08797912965199473, -0.3560938001956556742, 3.119077304627356106 ) ) ;
#35115=ADVANCED_FACE ( 'NONE', ( #30799 ), #35337, .F. ) ;
#35116=CARTESIAN_POINT ( 'NONE',  ( -27.06708303904391144, 0.000000000000000000, 7.395095371555332697 ) ) ;
#35117=EDGE_CURVE ( 'NONE', #31029, #41476, #40143, .T. ) ;
#35118=VECTOR ( 'NONE', #41018, 1000.000000000000000 ) ;
#35119=DIRECTION ( 'NONE',  ( -0.5449076811759708816, 0.6444004775717707689, 0.5364919789714475140 ) ) ;
#35120=DIRECTION ( 'NONE',  ( -0.5449076811759708816, 0.6444004775717707689, 0.5364919789714475140 ) ) ;
#35121=CARTESIAN_POINT ( 'NONE',  ( -8.829027555779365599, 0.000000000000000000, 4.382365521790453577 ) ) ;
#35122=EDGE_CURVE ( 'NONE', #48589, #30223, #35913, .T. ) ;
#35123=ORIENTED_EDGE ( 'NONE', *, *, #41772, .T. ) ;
#35124=DIRECTION ( 'NONE',  ( 0.007781995580012663651, 0.000000000000000000, -0.9999697198139515519 ) ) ;
#35125=AXIS2_PLACEMENT_3D ( 'NONE', #39336, #30817, #43581 ) ;
#35126=CARTESIAN_POINT ( 'NONE',  ( -16.81345671998191449, 0.000000000000000000, 3.412238694616132495 ) ) ;
#35127=ORIENTED_EDGE ( 'NONE', *, *, #45290, .T. ) ;
#35128=DIRECTION ( 'NONE',  ( 0.000000000000000000, -0.000000000000000000, -1.000000000000000000 ) ) ;
#35129=ORIENTED_EDGE ( 'NONE', *, *, #39249, .T. ) ;
#35130=CARTESIAN_POINT ( 'NONE',  ( -15.60102546347950536, 0.000000000000000000, 12.95077420755565356 ) ) ;
#35131=CARTESIAN_POINT ( 'NONE',  ( -19.01105676419016888, -2.137015261443157232, 7.573677912176790095 ) ) ;
#35132=EDGE_CURVE ( 'NONE', #52593, #19873, #27098, .T. ) ;
#35133=ORIENTED_EDGE ( 'NONE', *, *, #45254, .T. ) ;
#35134=VECTOR ( 'NONE', #2506, 1000.000000000000227 ) ;
#35135=ORIENTED_EDGE ( 'NONE', *, *, #8948, .T. ) ;
#35136=EDGE_CURVE ( 'NONE', #53425, #7643, #31902, .T. ) ;
#35137=ORIENTED_EDGE ( 'NONE', *, *, #31713, .F. ) ;
#35138=VECTOR ( 'NONE', #25379, 1000.000000000000227 ) ;
#35139=ORIENTED_EDGE ( 'NONE', *, *, #52405, .F. ) ;
#35140=ORIENTED_EDGE ( 'NONE', *, *, #34808, .T. ) ;
#35141=ORIENTED_EDGE ( 'NONE', *, *, #6062, .F. ) ;
#35142=DIRECTION ( 'NONE',  ( -0.5364919789714478471, 0.6444004775717705469, -0.5449076811759709926 ) ) ;
#35143=CARTESIAN_POINT ( 'NONE',  ( 2.072287782118878319, 0.000000000000000000, -2.950529333540147015 ) ) ;
#35144=DIRECTION ( 'NONE',  ( 0.007781995580012663651, 0.000000000000000000, -0.9999697198139515519 ) ) ;
#35145=ORIENTED_EDGE ( 'NONE', *, *, #26749, .T. ) ;
#35146=CARTESIAN_POINT ( 'NONE',  ( -10.86745071256952144, 0.000000000000000000, 1.781177552798060670 ) ) ;
#35147=EDGE_LOOP ( 'NONE', ( #24061, #27868, #44600, #31699 ) ) ;
#35148=VERTEX_POINT ( 'NONE', #18275 ) ;
#35149=FACE_OUTER_BOUND ( 'NONE', #26871, .T. ) ;
#35150=FACE_OUTER_BOUND ( 'NONE', #55763, .T. ) ;
#35152=VERTEX_POINT ( 'NONE', #22560 ) ;
#35153=DIRECTION ( 'NONE',  ( -0.005961354470445682716, -0.6427876096865404731, 0.7660212471507180654 ) ) ;
#35154=ORIENTED_EDGE ( 'NONE', *, *, #10998, .F. ) ;
#35155=DIRECTION ( 'NONE',  ( 0.005002170337468016433, -0.7660444431189770143, -0.6427681459581293666 ) ) ;
#35156=EDGE_CURVE ( 'NONE', #678, #34349, #31060, .T. ) ;
#35157=CARTESIAN_POINT ( 'NONE',  ( -18.92936932203669542, 0.000000000000000000, 4.134436313103331706 ) ) ;
#35158=DIRECTION ( 'NONE',  ( 0.9999697198139515519, 0.000000000000000000, 0.007781995580013368816 ) ) ;
#35159=VECTOR ( 'NONE', #25721, 1000.000000000000227 ) ;
#35160=FACE_OUTER_BOUND ( 'NONE', #9410, .T. ) ;
#35161=LINE ( 'NONE', #13821, #41349 ) ;
#35163=PLANE ( 'NONE',  #24831 ) ;
#35164=DIRECTION ( 'NONE',  ( 0.5449076811759707706, 0.6444004775717708799, -0.5364919789714476250 ) ) ;
#35165=ORIENTED_EDGE ( 'NONE', *, *, #22632, .F. ) ;
#35166=CARTESIAN_POINT ( 'NONE',  ( -18.32175943656386963, 0.000000000000000000, 4.308490887314260220 ) ) ;
#35167=EDGE_CURVE ( 'NONE', #52074, #37125, #44144, .T. ) ;
#35168=EDGE_CURVE ( 'NONE', #48125, #32400, #5795, .T. ) ;
#35169=AXIS2_PLACEMENT_3D ( 'NONE', #35622, #22836, #1246 ) ;
#35170=LINE ( 'NONE', #18673, #52846 ) ;
#35171=PLANE ( 'NONE',  #31426 ) ;
#35172=FACE_OUTER_BOUND ( 'NONE', #16079, .T. ) ;
#35173=FACE_OUTER_BOUND ( 'NONE', #50161, .T. ) ;
#35174=PLANE ( 'NONE',  #7743 ) ;
#35175=ADVANCED_FACE ( 'NONE', ( #10332 ), #1232, .F. ) ;
#35176=LINE ( 'NONE', #22389, #42242 ) ;
#35179=ORIENTED_EDGE ( 'NONE', *, *, #3492, .F. ) ;
#35180=CARTESIAN_POINT ( 'NONE',  ( -15.48150113315929488, -0.1191753592594177180, 9.231914369774386842 ) ) ;
#35181=DIRECTION ( 'NONE',  ( 0.000000000000000000, -1.000000000000000000, 0.000000000000000000 ) ) ;
#35182=CARTESIAN_POINT ( 'NONE',  ( -20.54126990917373519, -0.1191753592594197858, 4.760553241521720658 ) ) ;
#35183=DIRECTION ( 'NONE',  ( -0.5364919789714478471, 0.6444004775717705469, -0.5449076811759709926 ) ) ;
#35184=ADVANCED_FACE ( 'NONE', ( #23117 ), #27658, .F. ) ;
#35185=DIRECTION ( 'NONE',  ( -0.8531650599175529814, -0.4028455766673920135, 0.3313982828793697877 ) ) ;
#35186=PLANE ( 'NONE',  #25015 ) ;
#35187=LINE ( 'NONE', #53042, #28356 ) ;
#35188=EDGE_CURVE ( 'NONE', #4038, #5849, #32929, .T. ) ;
#35189=DIRECTION ( 'NONE',  ( 0.005002170337468016433, -0.7660444431189770143, -0.6427681459581293666 ) ) ;
#35190=LINE ( 'NONE', #47948, #10219 ) ;
#35191=EDGE_CURVE ( 'NONE', #9106, #7467, #22283, .T. ) ;
#35193=ORIENTED_EDGE ( 'NONE', *, *, #29418, .T. ) ;
#35194=ORIENTED_EDGE ( 'NONE', *, *, #21574, .F. ) ;
#35195=ORIENTED_EDGE ( 'NONE', *, *, #46398, .T. ) ;
#35196=EDGE_LOOP ( 'NONE', ( #52145, #18176, #6747, #50695, #11211 ) ) ;
#35197=FACE_OUTER_BOUND ( 'NONE', #25919, .T. ) ;
#35199=VECTOR ( 'NONE', #3760, 1000.000000000000227 ) ;
#35200=EDGE_LOOP ( 'NONE', ( #8295, #46397, #21523, #7945 ) ) ;
#35201=ORIENTED_EDGE ( 'NONE', *, *, #33611, .F. ) ;
#35202=DIRECTION ( 'NONE',  ( 0.000000000000000000, -1.000000000000000000, 0.000000000000000000 ) ) ;
#35203=ORIENTED_EDGE ( 'NONE', *, *, #21811, .F. ) ;
#35205=DIRECTION ( 'NONE',  ( 0.007781995580012662783, 0.000000000000000000, -0.9999697198139514409 ) ) ;
#35206=VERTEX_POINT ( 'NONE', #696 ) ;
#35207=LINE ( 'NONE', #26372, #14809 ) ;
#35208=EDGE_CURVE ( 'NONE', #47771, #15181, #48378, .T. ) ;
#35209=VERTEX_POINT ( 'NONE', #53751 ) ;
#35210=DIRECTION ( 'NONE',  ( -0.2426528472758541499, 0.7422098413412800966, -0.6246952433987894571 ) ) ;
#35211=ADVANCED_FACE ( 'NONE', ( #36735 ), #49521, .F. ) ;
#35212=CARTESIAN_POINT ( 'NONE',  ( -18.14763197414862717, 0.000000000000000000, 7.633834615750140884 ) ) ;
#35214=ORIENTED_EDGE ( 'NONE', *, *, #37437, .F. ) ;
#35215=DIRECTION ( 'NONE',  ( 0.005002170337468016433, -0.7660444431189770143, -0.6427681459581293666 ) ) ;
#35216=CARTESIAN_POINT ( 'NONE',  ( -20.25783497214359130, 5.629170628041515911, 4.371162778664604787 ) ) ;
#35217=CARTESIAN_POINT ( 'NONE',  ( -16.06709938707323460, 0.000000000000000000, 13.13181314741652628 ) ) ;
#35218=EDGE_CURVE ( 'NONE', #40640, #13570, #15992, .T. ) ;
#35219=ORIENTED_EDGE ( 'NONE', *, *, #47951, .T. ) ;
#35220=DIRECTION ( 'NONE',  ( 0.5364919789714477361, 0.6444004775717706579, 0.5449076811759711036 ) ) ;
#35221=ORIENTED_EDGE ( 'NONE', *, *, #9191, .T. ) ;
#35222=EDGE_CURVE ( 'NONE', #3481, #5914, #2893, .T. ) ;
#35223=EDGE_CURVE ( 'NONE', #14453, #44396, #20222, .T. ) ;
#35224=EDGE_CURVE ( 'NONE', #26864, #41020, #54317, .T. ) ;
#35225=CARTESIAN_POINT ( 'NONE',  ( -9.382943410138716800, -0.1191753592594192307, 3.000729569414776421 ) ) ;
#35226=CARTESIAN_POINT ( 'NONE',  ( -10.74029228357944987, 0.000000000000000000, 11.14194120806293320 ) ) ;
#35227=LINE ( 'NONE', #5123, #53967 ) ;
#35228=CARTESIAN_POINT ( 'NONE',  ( -14.00280974873554030, 0.000000000000000000, 12.40921378708904044 ) ) ;
#35229=CARTESIAN_POINT ( 'NONE',  ( -11.37928600064400086, -0.8417996532631553119, 2.483569499985687656 ) ) ;
#35230=ADVANCED_FACE ( 'NONE', ( #11149 ), #10879, .F. ) ;
#35231=LINE ( 'NONE', #52525, #22212 ) ;
#35232=PLANE ( 'NONE',  #10747 ) ;
#35233=CARTESIAN_POINT ( 'NONE',  ( -14.93495759592298988, 0.000000000000000000, 12.77129166681078409 ) ) ;
#35234=DIRECTION ( 'NONE',  ( 0.7660212471507180654, -0.6427876096865404731, 0.005961354470445141482 ) ) ;
#35235=ORIENTED_EDGE ( 'NONE', *, *, #14700, .T. ) ;
#35236=LINE ( 'NONE', #52533, #2137 ) ;
#35237=CARTESIAN_POINT ( 'NONE',  ( -12.20812748675390758, -0.1191753592594177180, 7.780060241157652712 ) ) ;
#35238=FACE_OUTER_BOUND ( 'NONE', #43895, .T. ) ;
#35239=VECTOR ( 'NONE', #9939, 999.9999999999998863 ) ;
#35240=FACE_OUTER_BOUND ( 'NONE', #30559, .T. ) ;
#35241=ADVANCED_FACE ( 'NONE', ( #3197 ), #24234, .F. ) ;
#35242=LINE ( 'NONE', #40619, #44158 ) ;
#35243=CARTESIAN_POINT ( 'NONE',  ( -16.99924723426068951, 0.000000000000000000, 13.49389102713827171 ) ) ;
#35244=ORIENTED_EDGE ( 'NONE', *, *, #37041, .T. ) ;
#35245=EDGE_CURVE ( 'NONE', #51166, #22994, #54882, .T. ) ;
#35246=ORIENTED_EDGE ( 'NONE', *, *, #17011, .F. ) ;
#35248=DIRECTION ( 'NONE',  ( 0.005002170337468016433, -0.7660444431189770143, -0.6427681459581293666 ) ) ;
#35249=DIRECTION ( 'NONE',  ( 0.005961354470445682716, -0.6427876096865404731, -0.7660212471507180654 ) ) ;
#35250=EDGE_CURVE ( 'NONE', #12574, #3673, #14869, .T. ) ;
#35251=ORIENTED_EDGE ( 'NONE', *, *, #13046, .F. ) ;
#35252=CARTESIAN_POINT ( 'NONE',  ( -29.86352658060627618, 0.000000000000000000, 8.481329010720569883 ) ) ;
#35253=EDGE_LOOP ( 'NONE', ( #11474, #43516, #14321, #14605 ) ) ;
#35254=CARTESIAN_POINT ( 'NONE',  ( -30.79489622823572859, -0.1191753592594197858, 8.743409918460921304 ) ) ;
#35255=EDGE_CURVE ( 'NONE', #54647, #29905, #33020, .T. ) ;
#35256=VERTEX_POINT ( 'NONE', #19950 ) ;
#35258=ORIENTED_EDGE ( 'NONE', *, *, #8901, .F. ) ;
#35259=DIRECTION ( 'NONE',  ( 0.7660212471507180654, -0.6427876096865404731, 0.005961354470445141482 ) ) ;
#35261=CARTESIAN_POINT ( 'NONE',  ( -16.95527162670416033, 0.000000000000000000, 7.843119895900956706 ) ) ;
#35262=CARTESIAN_POINT ( 'NONE',  ( -12.08435988717225129, 0.000000000000000000, 4.726363842672150817 ) ) ;
#35263=EDGE_LOOP ( 'NONE', ( #28872, #55149, #20823, #8561 ) ) ;
#35264=VERTEX_POINT ( 'NONE', #29035 ) ;
#35265=LINE ( 'NONE', #31566, #29997 ) ;
#35266=ORIENTED_EDGE ( 'NONE', *, *, #42934, .F. ) ;
#35267=DIRECTION ( 'NONE',  ( 0.8531650599175527594, 0.4028455766673922356, -0.3313982828793700652 ) ) ;
#35268=VERTEX_POINT ( 'NONE', #32197 ) ;
#35269=FACE_OUTER_BOUND ( 'NONE', #40897, .T. ) ;
#35270=DIRECTION ( 'NONE',  ( 0.000000000000000000, -0.000000000000000000, -1.000000000000000000 ) ) ;
#35271=AXIS2_PLACEMENT_3D ( 'NONE', #342, #43266, #8608 ) ;
#35272=EDGE_LOOP ( 'NONE', ( #17326, #33821, #45134, #10932 ) ) ;
#35273=DIRECTION ( 'NONE',  ( 0.007781995580012663651, -3.146120232559066537E-19, -0.9999697198139514409 ) ) ;
#35274=ORIENTED_EDGE ( 'NONE', *, *, #47787, .T. ) ;
#35275=DIRECTION ( 'NONE',  ( -0.9999697198139514409, -0.000000000000000000, -0.007781995580013368816 ) ) ;
#35276=ORIENTED_EDGE ( 'NONE', *, *, #24588, .T. ) ;
#35277=CARTESIAN_POINT ( 'NONE',  ( -15.55848688267561641, 0.000000000000000000, 7.484657927947219846 ) ) ;
#35278=DIRECTION ( 'NONE',  ( 0.5449076811759707706, 0.6444004775717708799, -0.5364919789714476250 ) ) ;
#35279=LINE ( 'NONE', #43769, #37318 ) ;
#35280=ORIENTED_EDGE ( 'NONE', *, *, #22612, .T. ) ;
#35281=EDGE_CURVE ( 'NONE', #11834, #51473, #28776, .T. ) ;
#35282=ADVANCED_FACE ( 'NONE', ( #27947 ), #7186, .F. ) ;
#35283=DIRECTION ( 'NONE',  ( 0.000000000000000000, -1.000000000000000000, 0.000000000000000000 ) ) ;
#35284=FACE_OUTER_BOUND ( 'NONE', #20064, .T. ) ;
#35287=EDGE_CURVE ( 'NONE', #1004, #50871, #6351, .T. ) ;
#35288=DIRECTION ( 'NONE',  ( 0.007781995580012663651, -3.146120232559066537E-19, -0.9999697198139514409 ) ) ;
#35289=DIRECTION ( 'NONE',  ( 0.005002170337468016433, -0.7660444431189770143, -0.6427681459581293666 ) ) ;
#35290=DIRECTION ( 'NONE',  ( -0.7660212471507179544, -0.6427876096865405842, -0.005961354470445141482 ) ) ;
#35291=EDGE_LOOP ( 'NONE', ( #1931, #56130, #13520, #50541 ) ) ;
#35292=CARTESIAN_POINT ( 'NONE',  ( -19.22961988024793101, -0.1191753592594177458, 14.39986392600063603 ) ) ;
#35293=DIRECTION ( 'NONE',  ( 0.9999697198139515519, 0.000000000000000000, 0.007781995580013368816 ) ) ;
#35294=VERTEX_POINT ( 'NONE', #23652 ) ;
#35295=DIRECTION ( 'NONE',  ( -0.9999697198139514409, -0.000000000000000000, -0.007781995580013368816 ) ) ;
#35296=CARTESIAN_POINT ( 'NONE',  ( -16.06709938707323460, 0.000000000000000000, 13.13181314741652628 ) ) ;
#35298=DIRECTION ( 'NONE',  ( 0.7660212471507180654, -0.6427876096865404731, 0.005961354470445141482 ) ) ;
#35299=CARTESIAN_POINT ( 'NONE',  ( -17.73140113748535285, 0.000000000000000000, 13.85752530597602039 ) ) ;
#35300=DIRECTION ( 'NONE',  ( -0.5449076811759708816, 0.6444004775717707689, 0.5364919789714475140 ) ) ;
#35301=PLANE ( 'NONE',  #16596 ) ;
#35302=ORIENTED_EDGE ( 'NONE', *, *, #50598, .F. ) ;
#35303=ORIENTED_EDGE ( 'NONE', *, *, #45068, .F. ) ;
#35304=LINE ( 'NONE', #31319, #24893 ) ;
#35306=CARTESIAN_POINT ( 'NONE',  ( -19.58586870846074390, -5.536956232915663634, 13.37683675498699998 ) ) ;
#35309=LINE ( 'NONE', #31024, #32820 ) ;
#35310=DIRECTION ( 'NONE',  ( -0.005002170337468016433, -0.7660444431189770143, 0.6427681459581293666 ) ) ;
#35311=ORIENTED_EDGE ( 'NONE', *, *, #51155, .T. ) ;
#35312=LINE ( 'NONE', #48925, #11122 ) ;
#35313=EDGE_CURVE ( 'NONE', #33893, #39017, #41545, .T. ) ;
#35314=CARTESIAN_POINT ( 'NONE',  ( -10.64080840018947605, 0.2864062442990034651, 1.484613903501102117 ) ) ;
#35315=ORIENTED_EDGE ( 'NONE', *, *, #1723, .F. ) ;
#35316=EDGE_CURVE ( 'NONE', #25539, #35767, #2060, .T. ) ;
#35317=CARTESIAN_POINT ( 'NONE',  ( -21.47419595591918906, 0.000000000000000000, 5.222628093224860102 ) ) ;
#35318=CARTESIAN_POINT ( 'NONE',  ( -15.86710544311044302, 0.000000000000000000, 13.13336954653252953 ) ) ;
#35319=ADVANCED_FACE ( 'NONE', ( #45797 ), #37269, .F. ) ;
#35320=CARTESIAN_POINT ( 'NONE',  ( -12.29165833726160884, 0.000000000000000000, 5.663420794034463412 ) ) ;
#35322=DIRECTION ( 'NONE',  ( 0.007781995580012663651, -3.146120232559066537E-19, -0.9999697198139514409 ) ) ;
#35323=EDGE_CURVE ( 'NONE', #32995, #31598, #18139, .T. ) ;
#35324=EDGE_LOOP ( 'NONE', ( #28481, #16117, #39742, #53246 ) ) ;
#35325=VERTEX_POINT ( 'NONE', #50880 ) ;
#35326=ORIENTED_EDGE ( 'NONE', *, *, #22725, .T. ) ;
#35327=EDGE_LOOP ( 'NONE', ( #15788, #20588, #51847, #47427 ) ) ;
#35328=CARTESIAN_POINT ( 'NONE',  ( -27.99767448711536133, 0.000000000000000000, 7.557179307314289218 ) ) ;
#35329=EDGE_LOOP ( 'NONE', ( #12526, #39684, #16364, #53964 ) ) ;
#35330=DIRECTION ( 'NONE',  ( -0.5364919789714478471, 0.6444004775717705469, -0.5449076811759709926 ) ) ;
#35331=ORIENTED_EDGE ( 'NONE', *, *, #32404, .F. ) ;
#35332=CARTESIAN_POINT ( 'NONE',  ( -16.66588516698283584, -3.756034771668160577, 9.319820460963413211 ) ) ;
#35333=EDGE_LOOP ( 'NONE', ( #22888, #48363, #21056, #6439 ) ) ;
#35334=DIRECTION ( 'NONE',  ( -0.005961354470445682716, -0.6427876096865404731, 0.7660212471507180654 ) ) ;
#35335=ORIENTED_EDGE ( 'NONE', *, *, #44801, .F. ) ;
#35336=DIRECTION ( 'NONE',  ( -0.7660212471507179544, -0.6427876096865405842, -0.005961354470445141482 ) ) ;
#35337=PLANE ( 'NONE',  #37465 ) ;
#35339=CARTESIAN_POINT ( 'NONE',  ( -18.70729593551854464, -0.1191753592594171213, 6.990818069889991548 ) ) ;
#35341=LINE ( 'NONE', #17748, #12942 ) ;
#35342=ORIENTED_EDGE ( 'NONE', *, *, #10070, .T. ) ;
#35344=ORIENTED_EDGE ( 'NONE', *, *, #15787, .T. ) ;
#35345=DIRECTION ( 'NONE',  ( 0.007781995580012663651, 0.000000000000000000, -0.9999697198139515519 ) ) ;
#35346=DIRECTION ( 'NONE',  ( 0.000000000000000000, -1.000000000000000000, 0.000000000000000000 ) ) ;
#35347=EDGE_CURVE ( 'NONE', #45853, #32666, #55165, .T. ) ;
#35349=DIRECTION ( 'NONE',  ( 0.5364919789714477361, 0.6444004775717706579, 0.5449076811759711036 ) ) ;
#35350=FACE_OUTER_BOUND ( 'NONE', #45523, .T. ) ;
#35351=CARTESIAN_POINT ( 'NONE',  ( -18.52282235942901778, 1.905425754524006532, 3.816031916019901438 ) ) ;
#35352=DIRECTION ( 'NONE',  ( 0.9999697198139515519, 0.000000000000000000, 0.007781995580013368816 ) ) ;
#35353=ORIENTED_EDGE ( 'NONE', *, *, #46627, .F. ) ;
#35354=CARTESIAN_POINT ( 'NONE',  ( -32.65841372305263235, 0.000000000000000000, 9.367568705923016381 ) ) ;
#35356=ORIENTED_EDGE ( 'NONE', *, *, #23281, .T. ) ;
#35357=CARTESIAN_POINT ( 'NONE',  ( -9.775545670493231754, 0.000000000000000000, 6.590991917801018118 ) ) ;
#35358=LINE ( 'NONE', #9518, #11513 ) ;
#35360=DIRECTION ( 'NONE',  ( 0.7660212471507180654, -0.6427876096865404731, 0.005961354470445141482 ) ) ;
#35361=ADVANCED_FACE ( 'NONE', ( #42649 ), #9339, .F. ) ;
#35363=ORIENTED_EDGE ( 'NONE', *, *, #21527, .F. ) ;
#35364=ORIENTED_EDGE ( 'NONE', *, *, #825, .T. ) ;
#35365=DIRECTION ( 'NONE',  ( 0.005002170337468016433, -0.7660444431189770143, -0.6427681459581293666 ) ) ;
#35366=CARTESIAN_POINT ( 'NONE',  ( -14.94838282604900748, -0.1191753592594197858, 2.588085963191248506 ) ) ;
#35367=CARTESIAN_POINT ( 'NONE',  ( -10.40856192273900049, 0.000000000000000000, 2.523412871081599285 ) ) ;
#35368=CARTESIAN_POINT ( 'NONE',  ( -12.33850799832341849, 0.000000000000000000, 11.68350162852954632 ) ) ;
#35369=DIRECTION ( 'NONE',  ( -0.6427681459581293666, -0.7660444431189770143, -0.005002170337467561935 ) ) ;
#35370=EDGE_LOOP ( 'NONE', ( #6246, #18076, #4719, #26700 ) ) ;
#35371=CARTESIAN_POINT ( 'NONE',  ( -16.53317331066696383, 0.000000000000000000, 13.31285208727739899 ) ) ;
#35372=LINE ( 'NONE', #4162, #22939 ) ;
#35373=VECTOR ( 'NONE', #22873, 1000.000000000000227 ) ;
#35374=LINE ( 'NONE', #22601, #46794 ) ;
#35375=PLANE ( 'NONE',  #6095 ) ;
#35376=ORIENTED_EDGE ( 'NONE', *, *, #47172, .F. ) ;
#35377=DIRECTION ( 'NONE',  ( 0.6427681459581294776, -0.7660444431189769032, 0.005002170337467562802 ) ) ;
#35378=ORIENTED_EDGE ( 'NONE', *, *, #45037, .F. ) ;
#35379=DIRECTION ( 'NONE',  ( 0.9999697198139515519, 0.000000000000000000, 0.007781995580013368816 ) ) ;
#35380=CARTESIAN_POINT ( 'NONE',  ( -15.83462604957504283, 0.000000000000000000, 8.959837228326271941 ) ) ;
#35381=ORIENTED_EDGE ( 'NONE', *, *, #47741, .F. ) ;
#35382=DIRECTION ( 'NONE',  ( -0.6427681459581293666, -0.7660444431189770143, -0.005002170337467561935 ) ) ;
#35383=ADVANCED_FACE ( 'NONE', ( #13878 ), #30918, .F. ) ;
#35384=ORIENTED_EDGE ( 'NONE', *, *, #8880, .F. ) ;
#35385=ORIENTED_EDGE ( 'NONE', *, *, #54873, .F. ) ;
#35386=EDGE_LOOP ( 'NONE', ( #50999, #22750, #54233, #23392 ) ) ;
#35387=LINE ( 'NONE', #1002, #13056 ) ;
#35388=VERTEX_POINT ( 'NONE', #51476 ) ;
#35389=ORIENTED_EDGE ( 'NONE', *, *, #31094, .T. ) ;
#35390=DIRECTION ( 'NONE',  ( 0.007781995580012663651, -3.146120232559066537E-19, -0.9999697198139514409 ) ) ;
#35391=DIRECTION ( 'NONE',  ( 0.6246952433987893460, 0.7422098413412802076, -0.2426528472758539279 ) ) ;
#35392=ORIENTED_EDGE ( 'NONE', *, *, #42686, .F. ) ;
#35393=EDGE_CURVE ( 'NONE', #31757, #40214, #7751, .T. ) ;
#35394=ORIENTED_EDGE ( 'NONE', *, *, #21166, .T. ) ;
#35395=DIRECTION ( 'NONE',  ( 0.007781995580012663651, 0.000000000000000000, -0.9999697198139515519 ) ) ;
#35396=ORIENTED_EDGE ( 'NONE', *, *, #36781, .F. ) ;
#35397=EDGE_CURVE ( 'NONE', #19674, #32400, #12292, .T. ) ;
#35398=ORIENTED_EDGE ( 'NONE', *, *, #56190, .F. ) ;
#35399=EDGE_CURVE ( 'NONE', #38932, #56078, #3744, .T. ) ;
#35400=LINE ( 'NONE', #1017, #51931 ) ;
#35401=CARTESIAN_POINT ( 'NONE',  ( -19.56975256245720729, 0.9340140483890051470, 4.253688280099741981 ) ) ;
#35402=CARTESIAN_POINT ( 'NONE',  ( -20.20936687189512071, 3.848249166794008413, 11.04695801043525094 ) ) ;
#35403=EDGE_CURVE ( 'NONE', #52700, #41193, #51176, .T. ) ;
#35404=ORIENTED_EDGE ( 'NONE', *, *, #17158, .T. ) ;
#35405=DIRECTION ( 'NONE',  ( 0.6246952433987893460, 0.7422098413412802076, -0.2426528472758539279 ) ) ;
#35406=VERTEX_POINT ( 'NONE', #43982 ) ;
#35407=EDGE_CURVE ( 'NONE', #3706, #6183, #34423, .T. ) ;
#35408=LINE ( 'NONE', #52710, #330 ) ;
#35409=EDGE_CURVE ( 'NONE', #34792, #48505, #26663, .T. ) ;
#35410=AXIS2_PLACEMENT_3D ( 'NONE', #52267, #586, #22712 ) ;
#35411=CARTESIAN_POINT ( 'NONE',  ( -21.47419595591918906, 0.000000000000000000, 5.222628093224860102 ) ) ;
#35412=DIRECTION ( 'NONE',  ( -0.005002170337468016433, -0.7660444431189770143, 0.6427681459581293666 ) ) ;
#35413=LINE ( 'NONE', #22636, #21413 ) ;
#35414=FACE_OUTER_BOUND ( 'NONE', #39368, .T. ) ;
#35415=CARTESIAN_POINT ( 'NONE',  ( -11.87243407472968926, 0.000000000000000000, 11.50246268866867361 ) ) ;
#35416=DIRECTION ( 'NONE',  ( 0.007781995580012663651, -3.146120232559066537E-19, -0.9999697198139514409 ) ) ;
#35417=VERTEX_POINT ( 'NONE', #48530 ) ;
#35418=DIRECTION ( 'NONE',  ( 0.7660212471507180654, -0.6427876096865404731, 0.005961354470445141482 ) ) ;
#35419=EDGE_CURVE ( 'NONE', #51697, #530, #46933, .T. ) ;
#35420=CARTESIAN_POINT ( 'NONE',  ( -17.39691609550298068, 0.000000000000000000, 4.885026358070830632 ) ) ;
#35421=CARTESIAN_POINT ( 'NONE',  ( -19.45503627000849889, 0.000000000000000000, 7.556996783084074742 ) ) ;
#35422=CARTESIAN_POINT ( 'NONE',  ( -25.20123094555300369, 0.000000000000000000, 6.470945668149052032 ) ) ;
#35424=CARTESIAN_POINT ( 'NONE',  ( -24.27063949748155380, 0.000000000000000000, 6.308861732390097288 ) ) ;
#35425=DIRECTION ( 'NONE',  ( 0.5449076811759707706, 0.6444004775717708799, -0.5364919789714476250 ) ) ;
#35426=EDGE_CURVE ( 'NONE', #34820, #18978, #42938, .T. ) ;
#35428=VERTEX_POINT ( 'NONE', #42393 ) ;
#35429=FACE_OUTER_BOUND ( 'NONE', #45355, .T. ) ;
#35430=LINE ( 'NONE', #44495, #4967 ) ;
#35431=DIRECTION ( 'NONE',  ( 0.7660212471507180654, -0.6427876096865404731, 0.005961354470445141482 ) ) ;
#35432=DIRECTION ( 'NONE',  ( -0.9999697198139514409, -0.000000000000000000, -0.007781995580013368816 ) ) ;
#35433=CARTESIAN_POINT ( 'NONE',  ( -17.46532115785441519, 0.000000000000000000, 13.67492996699914265 ) ) ;
#35434=LINE ( 'NONE', #52480, #52349 ) ;
#35435=DIRECTION ( 'NONE',  ( 0.007781995580012662783, 0.000000000000000000, -0.9999697198139514409 ) ) ;
#35436=LINE ( 'NONE', #47672, #39611 ) ;
#35437=DIRECTION ( 'NONE',  ( 0.9999697198139515519, 0.000000000000000000, 0.007781995580013368816 ) ) ;
#35438=ORIENTED_EDGE ( 'NONE', *, *, #42416, .F. ) ;
#35439=VECTOR ( 'NONE', #4531, 1000.000000000000227 ) ;
#35440=EDGE_CURVE ( 'NONE', #20635, #31613, #5107, .T. ) ;
#35441=VECTOR ( 'NONE', #13014, 999.9999999999998863 ) ;
#35443=ORIENTED_EDGE ( 'NONE', *, *, #51502, .T. ) ;
#35444=VERTEX_POINT ( 'NONE', #16252 ) ;
#35445=ORIENTED_EDGE ( 'NONE', *, *, #40275, .F. ) ;
#35446=LINE ( 'NONE', #17875, #32371 ) ;
#35447=CARTESIAN_POINT ( 'NONE',  ( 2.072287782118878319, 0.000000000000000000, -2.950529333540147015 ) ) ;
#35448=ORIENTED_EDGE ( 'NONE', *, *, #68, .T. ) ;
#35449=ORIENTED_EDGE ( 'NONE', *, *, #54389, .T. ) ;
#35450=EDGE_CURVE ( 'NONE', #8803, #15287, #56019, .T. ) ;
#35451=PLANE ( 'NONE',  #22930 ) ;
#35452=ORIENTED_EDGE ( 'NONE', *, *, #41091, .T. ) ;
#35453=LINE ( 'NONE', #17884, #42762 ) ;
#35454=DIRECTION ( 'NONE',  ( -0.005961354470445682716, -0.6427876096865404731, 0.7660212471507180654 ) ) ;
#35455=ORIENTED_EDGE ( 'NONE', *, *, #14701, .T. ) ;
#35456=CARTESIAN_POINT ( 'NONE',  ( -18.29747203306047609, -0.1191753592594177458, 14.03778604627889059 ) ) ;
#35457=ORIENTED_EDGE ( 'NONE', *, *, #39523, .T. ) ;
#35458=VECTOR ( 'NONE', #1692, 1000.000000000000227 ) ;
#35459=VECTOR ( 'NONE', #24685, 1000.000000000000000 ) ;
#35460=CARTESIAN_POINT ( 'NONE',  ( -15.71229329214178883, -1.003701604285656579, 4.432365365500901433 ) ) ;
#35462=CARTESIAN_POINT ( 'NONE',  ( -27.06708303904391144, 0.000000000000000000, 7.395095371555332697 ) ) ;
#35463=EDGE_CURVE ( 'NONE', #56189, #6902, #45371, .T. ) ;
#35464=DIRECTION ( 'NONE',  ( 0.7660212471507180654, -0.6427876096865404731, 0.005961354470445141482 ) ) ;
#35465=CARTESIAN_POINT ( 'NONE',  ( -14.01701317841955508, 0.000000000000000000, 2.326005055450897085 ) ) ;
#35466=ORIENTED_EDGE ( 'NONE', *, *, #11212, .F. ) ;
#35467=CARTESIAN_POINT ( 'NONE',  ( -27.06552663992790997, 0.000000000000000000, 7.195101427592543786 ) ) ;
#35468=FACE_OUTER_BOUND ( 'NONE', #20329, .T. ) ;
#35469=DIRECTION ( 'NONE',  ( -0.005002170337468016433, -0.7660444431189770143, 0.6427681459581293666 ) ) ;
#35470=ORIENTED_EDGE ( 'NONE', *, *, #14544, .T. ) ;
#35471=CARTESIAN_POINT ( 'NONE',  ( -11.72624626888112154, -0.1191753592594179401, 5.567817933379076045 ) ) ;
#35472=ORIENTED_EDGE ( 'NONE', *, *, #1015, .T. ) ;
#35473=EDGE_CURVE ( 'NONE', #46599, #5827, #15291, .T. ) ;
#35474=VECTOR ( 'NONE', #9651, 999.9999999999998863 ) ;
#35475=DIRECTION ( 'NONE',  ( 0.5449076811759707706, 0.6444004775717708799, -0.5364919789714476250 ) ) ;
#35476=CARTESIAN_POINT ( 'NONE',  ( -17.49243126037356788, 0.000000000000000000, 3.576280771331394437 ) ) ;
#35478=FACE_OUTER_BOUND ( 'NONE', #1964, .T. ) ;
#35479=DIRECTION ( 'NONE',  ( 0.5449076811759707706, 0.6444004775717708799, -0.5364919789714476250 ) ) ;
#35481=LINE ( 'NONE', #47726, #48808 ) ;
#35482=VECTOR ( 'NONE', #13377, 999.9999999999998863 ) ;
#35483=ADVANCED_FACE ( 'NONE', ( #32350 ), #11009, .F. ) ;
#35484=FACE_OUTER_BOUND ( 'NONE', #49785, .T. ) ;
#35485=CARTESIAN_POINT ( 'NONE',  ( -18.42529324785141398, -4.241740624735664156, 3.902997006360208410 ) ) ;
#35486=VERTEX_POINT ( 'NONE', #15015 ) ;
#35487=DIRECTION ( 'NONE',  ( -0.5364919789714478471, 0.6444004775717705469, -0.5449076811759709926 ) ) ;
#35488=DIRECTION ( 'NONE',  ( 0.007781995580012663651, -3.146120232559066537E-19, -0.9999697198139514409 ) ) ;
#35489=LINE ( 'NONE', #51963, #22719 ) ;
#35490=DIRECTION ( 'NONE',  ( -0.6427681459581293666, -0.7660444431189770143, -0.005002170337467561935 ) ) ;
#35491=CARTESIAN_POINT ( 'NONE',  ( -9.044948166384569888, 0.000000000000000000, 6.427351582926061013 ) ) ;
#35493=DIRECTION ( 'NONE',  ( -0.005961354470445682716, -0.6427876096865404731, 0.7660212471507180654 ) ) ;
#35495=EDGE_LOOP ( 'NONE', ( #35692, #48762, #55980, #47242 ) ) ;
#35496=CARTESIAN_POINT ( 'NONE',  ( -19.70704694140911073, 2.714935509636507316, 8.991879102924601241 ) ) ;
#35497=DIRECTION ( 'NONE',  ( 0.007781995580012663651, 0.000000000000000000, -0.9999697198139515519 ) ) ;
#35498=ADVANCED_FACE ( 'NONE', ( #2208 ), #49368, .F. ) ;
#35500=AXIS2_PLACEMENT_3D ( 'NONE', #34615, #51933, #30381 ) ;
#35501=ORIENTED_EDGE ( 'NONE', *, *, #36421, .T. ) ;
#35502=PLANE ( 'NONE',  #25877 ) ;
#35503=EDGE_CURVE ( 'NONE', #37777, #8893, #49663, .T. ) ;
#35504=ORIENTED_EDGE ( 'NONE', *, *, #23547, .F. ) ;
#35505=CARTESIAN_POINT ( 'NONE',  ( -18.58122884748872039, -3.270328918600660995, 9.266678939965695250 ) ) ;
#35506=ORIENTED_EDGE ( 'NONE', *, *, #47646, .F. ) ;
#35507=ORIENTED_EDGE ( 'NONE', *, *, #44318, .T. ) ;
#35508=ADVANCED_FACE ( 'NONE', ( #53362 ), #23791, .F. ) ;
#35509=VECTOR ( 'NONE', #18877, 999.9999999999998863 ) ;
#35510=VERTEX_POINT ( 'NONE', #41121 ) ;
#35511=EDGE_CURVE ( 'NONE', #43483, #55490, #22967, .T. ) ;
#35513=PLANE ( 'NONE',  #37754 ) ;
#35514=CARTESIAN_POINT ( 'NONE',  ( -23.33693525117809386, 0.000000000000000000, 5.746789908705562944 ) ) ;
#35515=ADVANCED_FACE ( 'NONE', ( #1663 ), #40290, .T. ) ;
#35516=EDGE_CURVE ( 'NONE', #49068, #31601, #10758, .T. ) ;
#35517=ADVANCED_FACE ( 'NONE', ( #28066 ), #19545, .F. ) ;
#35518=FACE_OUTER_BOUND ( 'NONE', #53945, .T. ) ;
#35519=ORIENTED_EDGE ( 'NONE', *, *, #26162, .T. ) ;
#35520=ORIENTED_EDGE ( 'NONE', *, *, #50663, .F. ) ;
#35521=AXIS2_PLACEMENT_3D ( 'NONE', #48596, #35824, #9712 ) ;
#35522=PLANE ( 'NONE',  #47214 ) ;
#35523=ORIENTED_EDGE ( 'NONE', *, *, #21644, .T. ) ;
#35524=PLANE ( 'NONE',  #11914 ) ;
#35525=ORIENTED_EDGE ( 'NONE', *, *, #55046, .T. ) ;
#35526=FACE_OUTER_BOUND ( 'NONE', #22941, .T. ) ;
#35527=CARTESIAN_POINT ( 'NONE',  ( -12.55342723663462046, 0.000000000000000000, 5.292051578124692846 ) ) ;
#35528=EDGE_LOOP ( 'NONE', ( #45269, #47776, #2283, #1299 ) ) ;
#35529=PLANE ( 'NONE',  #18648 ) ;
#35530=ADVANCED_FACE ( 'NONE', ( #39998 ), #48821, .F. ) ;
#35531=ORIENTED_EDGE ( 'NONE', *, *, #37949, .F. ) ;
#35532=EDGE_CURVE ( 'NONE', #9855, #42909, #1920, .T. ) ;
#35533=DIRECTION ( 'NONE',  ( -0.005002170337468016433, -0.7660444431189770143, 0.6427681459581293666 ) ) ;
#35534=ORIENTED_EDGE ( 'NONE', *, *, #56223, .F. ) ;
#35535=PLANE ( 'NONE',  #4085 ) ;
#35536=DIRECTION ( 'NONE',  ( -0.6427681459581293666, -0.7660444431189770143, -0.005002170337467561935 ) ) ;
#35537=ADVANCED_FACE ( 'NONE', ( #23528 ), #19253, .F. ) ;
#35538=CARTESIAN_POINT ( 'NONE',  ( -14.99594886780042025, -0.1191753592594194527, 7.758364770549599498 ) ) ;
#35539=VERTEX_POINT ( 'NONE', #14192 ) ;
#35540=VECTOR ( 'NONE', #8630, 1000.000000000000227 ) ;
#35541=DIRECTION ( 'NONE',  ( -0.9999697198139514409, -0.000000000000000000, -0.007781995580013368816 ) ) ;
#35542=EDGE_CURVE ( 'NONE', #44660, #8547, #27224, .T. ) ;
#35543=VECTOR ( 'NONE', #20801, 1000.000000000000227 ) ;
#35544=FACE_OUTER_BOUND ( 'NONE', #16509, .T. ) ;
#35545=FACE_OUTER_BOUND ( 'NONE', #45560, .T. ) ;
#35547=PLANE ( 'NONE',  #18608 ) ;
#35548=LINE ( 'NONE', #35848, #29734 ) ;
#35549=LINE ( 'NONE', #12854, #29462 ) ;
#35550=AXIS2_PLACEMENT_3D ( 'NONE', #21849, #39171, #258 ) ;
#35551=VERTEX_POINT ( 'NONE', #36307 ) ;
#35552=PLANE ( 'NONE',  #43411 ) ;
#35553=CARTESIAN_POINT ( 'NONE',  ( -15.87975247367846166, 0.000000000000000000, 2.850166870931599927 ) ) ;
#35554=LINE ( 'NONE', #48054, #23261 ) ;
#35555=VERTEX_POINT ( 'NONE', #53618 ) ;
#35556=CARTESIAN_POINT ( 'NONE',  ( -13.93141126051546408, 0.000000000000000000, 3.234661382569052446 ) ) ;
#35557=LINE ( 'NONE', #5204, #44476 ) ;
#35558=ORIENTED_EDGE ( 'NONE', *, *, #4635, .F. ) ;
#35559=LINE ( 'NONE', #18518, #56104 ) ;
#35560=FACE_OUTER_BOUND ( 'NONE', #1291, .T. ) ;
#35561=VECTOR ( 'NONE', #21522, 999.9999999999998863 ) ;
#35563=VECTOR ( 'NONE', #54185, 999.9999999999998863 ) ;
#35564=FACE_OUTER_BOUND ( 'NONE', #1710, .T. ) ;
#35565=VERTEX_POINT ( 'NONE', #15543 ) ;
#35566=ORIENTED_EDGE ( 'NONE', *, *, #50722, .F. ) ;
#35567=LINE ( 'NONE', #31608, #48487 ) ;
#35568=DIRECTION ( 'NONE',  ( -0.9999697198139514409, -0.000000000000000000, -0.007781995580013368816 ) ) ;
#35569=DIRECTION ( 'NONE',  ( 0.9999697198139515519, 0.000000000000000000, 0.007781995580013368816 ) ) ;
#35570=DIRECTION ( 'NONE',  ( -0.5364919789714478471, 0.6444004775717705469, -0.5449076811759709926 ) ) ;
#35571=CARTESIAN_POINT ( 'NONE',  ( -27.06552663992790997, 0.000000000000000000, 7.195101427592543786 ) ) ;
#35572=DIRECTION ( 'NONE',  ( 0.9999697198139515519, 0.000000000000000000, 0.007781995580013368816 ) ) ;
#35573=VECTOR ( 'NONE', #1567, 1000.000000000000227 ) ;
#35574=EDGE_LOOP ( 'NONE', ( #39068, #41185, #53729 ) ) ;
#35575=DIRECTION ( 'NONE',  ( 0.005961354470445682716, -0.6427876096865404731, -0.7660212471507180654 ) ) ;
#35577=ADVANCED_FACE ( 'NONE', ( #50189 ), #7061, .F. ) ;
#35578=ORIENTED_EDGE ( 'NONE', *, *, #46697, .T. ) ;
#35579=DIRECTION ( 'NONE',  ( 0.000000000000000000, -1.000000000000000000, 0.000000000000000000 ) ) ;
#35580=VECTOR ( 'NONE', #51892, 1000.000000000000000 ) ;
#35582=CARTESIAN_POINT ( 'NONE',  ( -9.861950574506215261, -0.1191753592594181482, 4.843662173935586956 ) ) ;
#35583=ADVANCED_FACE ( 'NONE', ( #11298 ), #2503, .F. ) ;
#35584=EDGE_CURVE ( 'NONE', #38157, #34381, #37717, .T. ) ;
#35585=VERTEX_POINT ( 'NONE', #42250 ) ;
#35586=VECTOR ( 'NONE', #33973, 1000.000000000000227 ) ;
#35587=VECTOR ( 'NONE', #31840, 1000.000000000000114 ) ;
#35588=FACE_OUTER_BOUND ( 'NONE', #24903, .T. ) ;
#35589=ORIENTED_EDGE ( 'NONE', *, *, #44687, .T. ) ;
#35590=EDGE_CURVE ( 'NONE', #33592, #10988, #12450, .T. ) ;
#35591=ORIENTED_EDGE ( 'NONE', *, *, #46527, .F. ) ;
#35592=VECTOR ( 'NONE', #35437, 999.9999999999998863 ) ;
#35593=ORIENTED_EDGE ( 'NONE', *, *, #46179, .F. ) ;
#35594=AXIS2_PLACEMENT_3D ( 'NONE', #13828, #53324, #39953 ) ;
#35595=ORIENTED_EDGE ( 'NONE', *, *, #46818, .T. ) ;
#35596=CARTESIAN_POINT ( 'NONE',  ( -18.20244891691826084, -3.917936722690661178, 10.18238268731339247 ) ) ;
#35598=LINE ( 'NONE', #52914, #21311 ) ;
#35599=LINE ( 'NONE', #44667, #27736 ) ;
#35600=ORIENTED_EDGE ( 'NONE', *, *, #2039, .T. ) ;
#35601=CARTESIAN_POINT ( 'NONE',  ( -20.10016216420208579, 4.333955019861511992, 4.351241464568151862 ) ) ;
#35602=EDGE_LOOP ( 'NONE', ( #26035, #10096, #49480, #36741 ) ) ;
#35603=CARTESIAN_POINT ( 'NONE',  ( -13.84799759776688433, -1.003701604285656579, 3.708209606057412344 ) ) ;
#35604=AXIS2_PLACEMENT_3D ( 'NONE', #2973, #29101, #28849 ) ;
#35605=ORIENTED_EDGE ( 'NONE', *, *, #40174, .T. ) ;
#35606=EDGE_CURVE ( 'NONE', #18658, #20294, #45648, .T. ) ;
#35607=CARTESIAN_POINT ( 'NONE',  ( -14.01701317841955508, 0.000000000000000000, 2.326005055450897085 ) ) ;
#35608=LINE ( 'NONE', #52925, #3905 ) ;
#35609=CARTESIAN_POINT ( 'NONE',  ( -24.26908309836554878, 0.000000000000000000, 6.108867788427308376 ) ) ;
#35611=EDGE_CURVE ( 'NONE', #54767, #42246, #6769, .T. ) ;
#35612=CARTESIAN_POINT ( 'NONE',  ( -17.74482636761137044, -0.1191753592594197858, 3.674319602356483916 ) ) ;
#35613=PLANE ( 'NONE',  #14724 ) ;
#35615=EDGE_CURVE ( 'NONE', #43426, #37711, #24089, .T. ) ;
#35616=ORIENTED_EDGE ( 'NONE', *, *, #8540, .F. ) ;
#35617=DIRECTION ( 'NONE',  ( -0.9999697198139514409, -0.000000000000000000, -0.007781995580013368816 ) ) ;
#35619=AXIS2_PLACEMENT_3D ( 'NONE', #590, #26407, #5410 ) ;
#35621=ADVANCED_FACE ( 'NONE', ( #45952 ), #29170, .F. ) ;
#35622=CARTESIAN_POINT ( 'NONE',  ( -13.08486533123210194, 0.000000000000000000, 1.963927175729152541 ) ) ;
#35623=CARTESIAN_POINT ( 'NONE',  ( -13.67251641464773115, 0.000000000000000000, 3.975340301736589588 ) ) ;
#35624=ORIENTED_EDGE ( 'NONE', *, *, #8814, .T. ) ;
#35625=CARTESIAN_POINT ( 'NONE',  ( -20.54049170961573267, 0.000000000000000000, 4.660556269540326646 ) ) ;
#35626=DIRECTION ( 'NONE',  ( 0.7660212471507180654, -0.6427876096865404731, 0.005961354470445141482 ) ) ;
#35627=ORIENTED_EDGE ( 'NONE', *, *, #16576, .T. ) ;
#35628=AXIS2_PLACEMENT_3D ( 'NONE', #22557, #22279, #31055 ) ;
#35629=FACE_OUTER_BOUND ( 'NONE', #45775, .T. ) ;
#35630=CARTESIAN_POINT ( 'NONE',  ( -17.74560456716937296, 0.000000000000000000, 3.774316574337878372 ) ) ;
#35631=VERTEX_POINT ( 'NONE', #24358 ) ;
#35632=VECTOR ( 'NONE', #19793, 1000.000000000000227 ) ;
#35633=VECTOR ( 'NONE', #18094, 1000.000000000000000 ) ;
#35634=LINE ( 'NONE', #4978, #28863 ) ;
#35636=CARTESIAN_POINT ( 'NONE',  ( -19.69569380384165669, -0.1191753592594177458, 14.58090286586150697 ) ) ;
#35637=DIRECTION ( 'NONE',  ( 0.5449076811759707706, 0.6444004775717708799, -0.5364919789714476250 ) ) ;
#35638=DIRECTION ( 'NONE',  ( -0.7660212471507179544, -0.6427876096865405842, -0.005961354470445141482 ) ) ;
#35639=ORIENTED_EDGE ( 'NONE', *, *, #6050, .F. ) ;
#35640=AXIS2_PLACEMENT_3D ( 'NONE', #34275, #10680, #14917 ) ;
#35641=VECTOR ( 'NONE', #54827, 1000.000000000000000 ) ;
#35642=ORIENTED_EDGE ( 'NONE', *, *, #9461, .T. ) ;
#35643=DIRECTION ( 'NONE',  ( -0.7660212471507179544, -0.6427876096865405842, -0.005961354470445141482 ) ) ;
#35644=LINE ( 'NONE', #39061, #13198 ) ;
#35645=PLANE ( 'NONE',  #53280 ) ;
#35647=PLANE ( 'NONE',  #49994 ) ;
#35648=VECTOR ( 'NONE', #42590, 1000.000000000000000 ) ;
#35649=CARTESIAN_POINT ( 'NONE',  ( -13.08408713167412074, -0.1191753592594190225, 1.863930203747756975 ) ) ;
#35650=VERTEX_POINT ( 'NONE', #24929 ) ;
#35651=CARTESIAN_POINT ( 'NONE',  ( -12.74479902008156174, 0.000000000000000000, 4.182566069235397421 ) ) ;
#35652=VECTOR ( 'NONE', #24342, 1000.000000000000000 ) ;
#35653=DIRECTION ( 'NONE',  ( -0.005002170337468016433, -0.7660444431189770143, 0.6427681459581293666 ) ) ;
#35654=DIRECTION ( 'NONE',  ( 0.5364919789714477361, 0.6444004775717706579, 0.5449076811759711036 ) ) ;
#35655=CARTESIAN_POINT ( 'NONE',  ( -16.89925026227929195, -0.1191753592594197858, 13.49466922669627422 ) ) ;
#35657=LINE ( 'NONE', #10091, #23827 ) ;
#35658=ORIENTED_EDGE ( 'NONE', *, *, #26887, .F. ) ;
#35659=CARTESIAN_POINT ( 'NONE',  ( -12.08723394067753176, 0.000000000000000000, 5.095673545929914283 ) ) ;
#35661=DIRECTION ( 'NONE',  ( 0.5449076811759707706, 0.6444004775717708799, -0.5364919789714476250 ) ) ;
#35662=EDGE_CURVE ( 'NONE', #32862, #48142, #41668, .T. ) ;
#35663=ORIENTED_EDGE ( 'NONE', *, *, #18478, .F. ) ;
#35664=DIRECTION ( 'NONE',  ( 0.007781995580012662783, 0.000000000000000000, -0.9999697198139514409 ) ) ;
#35665=AXIS2_PLACEMENT_3D ( 'NONE', #53710, #23617, #10287 ) ;
#35666=EDGE_LOOP ( 'NONE', ( #9546, #2123, #43416, #28024 ) ) ;
#35667=EDGE_CURVE ( 'NONE', #6678, #18137, #12136, .T. ) ;
#35668=EDGE_CURVE ( 'NONE', #931, #25817, #2753, .T. ) ;
#35669=ORIENTED_EDGE ( 'NONE', *, *, #40678, .F. ) ;
#35670=ORIENTED_EDGE ( 'NONE', *, *, #2856, .F. ) ;
#35671=FACE_OUTER_BOUND ( 'NONE', #35333, .T. ) ;
#35673=ORIENTED_EDGE ( 'NONE', *, *, #53089, .T. ) ;
#35674=VECTOR ( 'NONE', #32644, 1000.000000000000114 ) ;
#35675=CARTESIAN_POINT ( 'NONE',  ( -18.86992194539476131, -3.108426967578160838, 4.111864531351901775 ) ) ;
#35676=LINE ( 'NONE', #27153, #54826 ) ;
#35677=ORIENTED_EDGE ( 'NONE', *, *, #45270, .F. ) ;
#35678=VECTOR ( 'NONE', #14370, 1000.000000000000114 ) ;
#35679=VECTOR ( 'NONE', #22576, 1000.000000000000227 ) ;
#35680=EDGE_LOOP ( 'NONE', ( #2947, #55007, #12380, #7658 ) ) ;
#35681=DIRECTION ( 'NONE',  ( 0.5449076811759707706, 0.6444004775717708799, -0.5364919789714476250 ) ) ;
#35682=ORIENTED_EDGE ( 'NONE', *, *, #10070, .F. ) ;
#35683=VERTEX_POINT ( 'NONE', #41416 ) ;
#35684=VECTOR ( 'NONE', #46913, 1000.000000000000000 ) ;
#35685=VECTOR ( 'NONE', #16213, 1000.000000000000227 ) ;
#35686=CARTESIAN_POINT ( 'NONE',  ( -28.92982233430281980, 0.000000000000000000, 7.919257187036034651 ) ) ;
#35687=FACE_OUTER_BOUND ( 'NONE', #54008, .T. ) ;
#35688=CARTESIAN_POINT ( 'NONE',  ( 2.602374448188125350E-16, 0.000000000000000000, -2.125000000000000000 ) ) ;
#35689=DIRECTION ( 'NONE',  ( -0.5364919789714478471, 0.6444004775717705469, -0.5449076811759709926 ) ) ;
#35690=ORIENTED_EDGE ( 'NONE', *, *, #20968, .F. ) ;
#35691=CARTESIAN_POINT ( 'NONE',  ( -13.08408713167409942, -0.1191753592594197858, 1.863930203747758085 ) ) ;
#35692=ORIENTED_EDGE ( 'NONE', *, *, #56223, .T. ) ;
#35693=CARTESIAN_POINT ( 'NONE',  ( -27.99845268667336384, -0.1191753592594197858, 7.657176279295684118 ) ) ;
#35694=EDGE_CURVE ( 'NONE', #43321, #10765, #46793, .T. ) ;
#35695=CARTESIAN_POINT ( 'NONE',  ( -12.27441401622991002, 0.000000000000000000, 3.447562574487877729 ) ) ;
#35696=LINE ( 'NONE', #31456, #24957 ) ;
#35697=CARTESIAN_POINT ( 'NONE',  ( -27.06552663992790997, 0.000000000000000000, 7.195101427592543786 ) ) ;
#35698=VECTOR ( 'NONE', #16896, 1000.000000000000227 ) ;
#35699=ADVANCED_FACE ( 'NONE', ( #20078 ), #54442, .F. ) ;
#35700=LINE ( 'NONE', #53016, #390 ) ;
#35701=LINE ( 'NONE', #23481, #43882 ) ;
#35702=LINE ( 'NONE', #498, #54905 ) ;
#35703=ORIENTED_EDGE ( 'NONE', *, *, #2101, .T. ) ;
#35704=CARTESIAN_POINT ( 'NONE',  ( -10.32083936433673621, -0.1191753592594190225, 4.101426855652049674 ) ) ;
#35705=EDGE_CURVE ( 'NONE', #24424, #23097, #46481, .T. ) ;
#35706=AXIS2_PLACEMENT_3D ( 'NONE', #30313, #17523, #34856 ) ;
#35707=CARTESIAN_POINT ( 'NONE',  ( 2.072287782118878319, 0.000000000000000000, -2.950529333540147015 ) ) ;
#35708=DIRECTION ( 'NONE',  ( 0.000000000000000000, -0.000000000000000000, -1.000000000000000000 ) ) ;
#35709=CARTESIAN_POINT ( 'NONE',  ( -19.12962290826653700, 0.000000000000000000, 14.40064212555863854 ) ) ;
#35710=EDGE_CURVE ( 'NONE', #11776, #1716, #33177, .T. ) ;
#35711=VECTOR ( 'NONE', #41577, 999.9999999999998863 ) ;
#35713=DIRECTION ( 'NONE',  ( -0.6427681459581293666, -0.7660444431189770143, -0.005002170337467561935 ) ) ;
#35714=DIRECTION ( 'NONE',  ( 0.007781995580012663651, 0.000000000000000000, -0.9999697198139515519 ) ) ;
#35716=EDGE_LOOP ( 'NONE', ( #23563, #4513, #35145, #55347 ) ) ;
#35717=AXIS2_PLACEMENT_3D ( 'NONE', #50091, #2946, #2112 ) ;
#35718=CARTESIAN_POINT ( 'NONE',  ( -12.19088316572221231, -0.1191753592594179401, 5.564202021611067472 ) ) ;
#35719=FACE_OUTER_BOUND ( 'NONE', #12496, .T. ) ;
#35720=CARTESIAN_POINT ( 'NONE',  ( -8.875996589204540044, 0.000000000000000000, 10.41778544861944233 ) ) ;
#35721=VECTOR ( 'NONE', #8038, 1000.000000000000227 ) ;
#35722=DIRECTION ( 'NONE',  ( -0.5364919789714478471, 0.6444004775717705469, -0.5449076811759709926 ) ) ;
#35723=FACE_OUTER_BOUND ( 'NONE', #7141, .T. ) ;
#35725=EDGE_CURVE ( 'NONE', #9862, #38231, #28910, .T. ) ;
#35726=PLANE ( 'NONE',  #25603 ) ;
#35727=VECTOR ( 'NONE', #26473, 999.9999999999998863 ) ;
#35728=AXIS2_PLACEMENT_3D ( 'NONE', #9367, #22710, #36081 ) ;
#35730=CARTESIAN_POINT ( 'NONE',  ( -22.40478740399063895, 0.000000000000000000, 5.384712028983816623 ) ) ;
#35731=EDGE_CURVE ( 'NONE', #18997, #24292, #41941, .T. ) ;
#35732=ORIENTED_EDGE ( 'NONE', *, *, #22007, .T. ) ;
#35733=ADVANCED_FACE ( 'NONE', ( #490 ), #34303, .F. ) ;
#35734=EDGE_CURVE ( 'NONE', #42927, #47502, #43919, .T. ) ;
#35735=EDGE_LOOP ( 'NONE', ( #3595, #33780, #11494 ) ) ;
#35736=VERTEX_POINT ( 'NONE', #35157 ) ;
#35737=ORIENTED_EDGE ( 'NONE', *, *, #38943, .T. ) ;
#35739=ORIENTED_EDGE ( 'NONE', *, *, #3863, .T. ) ;
#35740=PLANE ( 'NONE',  #34194 ) ;
#35741=DIRECTION ( 'NONE',  ( 0.005002170337468016433, -0.7660444431189770143, -0.6427681459581293666 ) ) ;
#35742=AXIS2_PLACEMENT_3D ( 'NONE', #1797, #44995, #9802 ) ;
#35743=ORIENTED_EDGE ( 'NONE', *, *, #53944, .T. ) ;
#35744=ORIENTED_EDGE ( 'NONE', *, *, #2956, .F. ) ;
#35745=AXIS2_PLACEMENT_3D ( 'NONE', #24987, #50550, #46257 ) ;
#35746=EDGE_CURVE ( 'NONE', #36489, #25453, #18084, .T. ) ;
#35747=FACE_OUTER_BOUND ( 'NONE', #42883, .T. ) ;
#35748=ORIENTED_EDGE ( 'NONE', *, *, #40815, .T. ) ;
#35749=VECTOR ( 'NONE', #24465, 1000.000000000000114 ) ;
#35750=LINE ( 'NONE', #18717, #45477 ) ;
#35751=LINE ( 'NONE', #5938, #36823 ) ;
#35752=ORIENTED_EDGE ( 'NONE', *, *, #48684, .T. ) ;
#35753=CARTESIAN_POINT ( 'NONE',  ( -15.06798350428698896, 0.000000000000000000, 4.164486510395348340 ) ) ;
#35754=AXIS2_PLACEMENT_3D ( 'NONE', #40656, #18803, #36124 ) ;
#35755=EDGE_LOOP ( 'NONE', ( #17580, #23691, #36230, #50729 ) ) ;
#35756=CARTESIAN_POINT ( 'NONE',  ( -14.10280672071693431, -0.1191753592594197858, 12.40843558753103792 ) ) ;
#35757=DIRECTION ( 'NONE',  ( 0.007781995580012663651, 0.000000000000000000, -0.9999697198139515519 ) ) ;
#35758=AXIS2_PLACEMENT_3D ( 'NONE', #30641, #52204, #34884 ) ;
#35759=LINE ( 'NONE', #36059, #20955 ) ;
#35760=CARTESIAN_POINT ( 'NONE',  ( -26.13493519185646008, 0.000000000000000000, 7.033017491833586377 ) ) ;
#35761=ORIENTED_EDGE ( 'NONE', *, *, #15688, .T. ) ;
#35762=FACE_OUTER_BOUND ( 'NONE', #49763, .T. ) ;
#35763=DIRECTION ( 'NONE',  ( 0.9999697198139515519, 0.000000000000000000, 0.007781995580013368816 ) ) ;
#35766=CARTESIAN_POINT ( 'NONE',  ( -19.60834386242827776, 0.000000000000000000, 4.298478389818581213 ) ) ;
#35767=VERTEX_POINT ( 'NONE', #30025 ) ;
#35768=CARTESIAN_POINT ( 'NONE',  ( -23.33849165029409889, 0.000000000000000000, 5.946783852668351855 ) ) ;
#35769=DIRECTION ( 'NONE',  ( 0.005961354470445682716, -0.6427876096865404731, -0.7660212471507180654 ) ) ;
#35770=LINE ( 'NONE', #5654, #24060 ) ;
#35771=PLANE ( 'NONE',  #48645 ) ;
#35772=EDGE_CURVE ( 'NONE', #55300, #12199, #43633, .T. ) ;
#35773=LINE ( 'NONE', #53095, #21402 ) ;
#35774=DIRECTION ( 'NONE',  ( -0.005961354470445682716, -0.6427876096865404731, 0.7660212471507180654 ) ) ;
#35775=DIRECTION ( 'NONE',  ( 0.000000000000000000, -1.000000000000000000, 0.000000000000000000 ) ) ;
#35776=VECTOR ( 'NONE', #33387, 999.9999999999998863 ) ;
#35777=DIRECTION ( 'NONE',  ( 0.7660212471507180654, -0.6427876096865404731, 0.005961354470445141482 ) ) ;
#35778=( NAMED_UNIT ( * ) PLANE_ANGLE_UNIT ( ) SI_UNIT ( $, .RADIAN. ) );
#35779=VECTOR ( 'NONE', #33776, 999.9999999999998863 ) ;
#35780=CARTESIAN_POINT ( 'NONE',  ( -19.72742537039871280, 2.229229656569007734, 4.273609594196196682 ) ) ;
#35781=ORIENTED_EDGE ( 'NONE', *, *, #12978, .F. ) ;
#35782=CARTESIAN_POINT ( 'NONE',  ( -16.33317936670417225, 0.000000000000000000, 13.31440848639340224 ) ) ;
#35783=FACE_OUTER_BOUND ( 'NONE', #42614, .T. ) ;
#35784=CARTESIAN_POINT ( 'NONE',  ( -16.89925026227929195, -0.1191753592594197858, 13.49466922669627422 ) ) ;
#35785=AXIS2_PLACEMENT_3D ( 'NONE', #52581, #31845, #30992 ) ;
#35786=DIRECTION ( 'NONE',  ( -0.005002170337468016433, -0.7660444431189770143, 0.6427681459581293666 ) ) ;
#35787=EDGE_CURVE ( 'NONE', #5570, #21771, #22065, .T. ) ;
#35788=DIRECTION ( 'NONE',  ( 0.007781995580012663651, -3.146120232559066537E-19, -0.9999697198139514409 ) ) ;
#35789=ADVANCED_FACE ( 'NONE', ( #39395 ), #21526, .F. ) ;
#35790=DIRECTION ( 'NONE',  ( 0.000000000000000000, -1.000000000000000000, 0.000000000000000000 ) ) ;
#35791=EDGE_CURVE ( 'NONE', #3166, #21903, #39687, .T. ) ;
#35792=CARTESIAN_POINT ( 'NONE',  ( -20.51801655564820237, -5.536956232915664522, 13.73891463470874186 ) ) ;
#35793=ORIENTED_EDGE ( 'NONE', *, *, #10484, .T. ) ;
#35795=ORIENTED_EDGE ( 'NONE', *, *, #667, .T. ) ;
#35797=AXIS2_PLACEMENT_3D ( 'NONE', #7358, #229, #805 ) ;
#35798=PLANE ( 'NONE',  #17744 ) ;
#35799=ADVANCED_FACE ( 'NONE', ( #8441 ), #52453, .F. ) ;
#35800=VECTOR ( 'NONE', #23948, 1000.000000000000227 ) ;
#35801=ORIENTED_EDGE ( 'NONE', *, *, #24960, .T. ) ;
#35802=ADVANCED_FACE ( 'NONE', ( #30862 ), #3893, .F. ) ;
#35803=FACE_OUTER_BOUND ( 'NONE', #11962, .T. ) ;
#35804=VERTEX_POINT ( 'NONE', #48167 ) ;
#35805=LINE ( 'NONE', #53401, #51051 ) ;
#35806=EDGE_CURVE ( 'NONE', #41646, #52618, #43380, .T. ) ;
#35807=VECTOR ( 'NONE', #49260, 1000.000000000000000 ) ;
#35808=ORIENTED_EDGE ( 'NONE', *, *, #31364, .F. ) ;
#35809=AXIS2_PLACEMENT_3D ( 'NONE', #8790, #38284, #17266 ) ;
#35810=VERTEX_POINT ( 'NONE', #22371 ) ;
#35811=EDGE_LOOP ( 'NONE', ( #47460, #55813, #7243, #6467 ) ) ;
#35812=DIRECTION ( 'NONE',  ( 0.007781995580012662783, 0.000000000000000000, -0.9999697198139514409 ) ) ;
#35813=LINE ( 'NONE', #5998, #28669 ) ;
#35815=EDGE_CURVE ( 'NONE', #31029, #37945, #35408, .T. ) ;
#35816=CARTESIAN_POINT ( 'NONE',  ( -18.78507867901567252, 0.000000000000000000, 4.135559216251272652 ) ) ;
#35817=EDGE_LOOP ( 'NONE', ( #46310, #7999, #27635, #31493 ) ) ;
#35818=ORIENTED_EDGE ( 'NONE', *, *, #3116, .F. ) ;
#35819=VECTOR ( 'NONE', #11034, 1000.000000000000227 ) ;
#35820=ADVANCED_FACE ( 'NONE', ( #177 ), #52169, .F. ) ;
#35822=VECTOR ( 'NONE', #14110, 999.9999999999998863 ) ;
#35823=ORIENTED_EDGE ( 'NONE', *, *, #18487, .T. ) ;
#35824=DIRECTION ( 'NONE',  ( 0.7660212471507180654, -0.6427876096865404731, 0.005961354470445141482 ) ) ;
#35825=ORIENTED_EDGE ( 'NONE', *, *, #27734, .F. ) ;
#35826=VECTOR ( 'NONE', #14604, 999.9999999999998863 ) ;
#35828=CARTESIAN_POINT ( 'NONE',  ( 2.072287782118878319, 0.000000000000000000, -2.950529333540147015 ) ) ;
#35829=ORIENTED_EDGE ( 'NONE', *, *, #27128, .F. ) ;
#35830=CARTESIAN_POINT ( 'NONE',  ( -18.23978498517217517, -0.1191753592594166911, 6.625124278400236655 ) ) ;
#35831=VECTOR ( 'NONE', #20149, 1000.000000000000114 ) ;
#35832=ORIENTED_EDGE ( 'NONE', *, *, #33158, .T. ) ;
#35833=CARTESIAN_POINT ( 'NONE',  ( -15.44621549711509090, -0.1191753592594185784, 5.908200342492767376 ) ) ;
#35834=AXIS2_PLACEMENT_3D ( 'NONE', #15405, #24476, #28183 ) ;
#35835=VERTEX_POINT ( 'NONE', #8169 ) ;
#35836=DIRECTION ( 'NONE',  ( 0.9999697198139515519, 0.000000000000000000, 0.007781995580013368816 ) ) ;
#35837=CARTESIAN_POINT ( 'NONE',  ( -17.93139508144814442, 0.000000000000000000, 13.85596890686001537 ) ) ;
#35838=AXIS2_PLACEMENT_3D ( 'NONE', #56089, #47847, #102 ) ;
#35840=ORIENTED_EDGE ( 'NONE', *, *, #47318, .F. ) ;
#35841=VECTOR ( 'NONE', #8306, 1000.000000000000114 ) ;
#35842=DIRECTION ( 'NONE',  ( -0.6427681459581293666, -0.7660444431189770143, -0.005002170337467561935 ) ) ;
#35843=CARTESIAN_POINT ( 'NONE',  ( -19.45497020661647269, 1.905425754524007642, 4.178109795741645982 ) ) ;
#35844=ADVANCED_FACE ( 'NONE', ( #42787 ), #21218, .F. ) ;
#35845=EDGE_CURVE ( 'NONE', #32241, #24728, #38549, .T. ) ;
#35847=CARTESIAN_POINT ( 'NONE',  ( -11.66794108741423308, 2.067327705546508021, 1.148197717334086043 ) ) ;
#35848=CARTESIAN_POINT ( 'NONE',  ( -14.66887761629205222, 0.000000000000000000, 12.58869632783390990 ) ) ;
#35849=VECTOR ( 'NONE', #31250, 1000.000000000000000 ) ;
#35850=VECTOR ( 'NONE', #50956, 1000.000000000000114 ) ;
#35852=ORIENTED_EDGE ( 'NONE', *, *, #2381, .F. ) ;
#35853=CARTESIAN_POINT ( 'NONE',  ( -15.86710544311044302, 0.000000000000000000, 13.13336954653252953 ) ) ;
#35854=LINE ( 'NONE', #39821, #10476 ) ;
#35855=PLANE ( 'NONE',  #45035 ) ;
#35856=EDGE_LOOP ( 'NONE', ( #20684, #43995, #42063, #21337 ) ) ;
#35857=CARTESIAN_POINT ( 'NONE',  ( -12.80458192191714595, 0.000000000000000000, 11.86454056839041726 ) ) ;
#35858=DIRECTION ( 'NONE',  ( -0.6427681459581293666, -0.7660444431189770143, -0.005002170337467561935 ) ) ;
#35859=ORIENTED_EDGE ( 'NONE', *, *, #37571, .F. ) ;
#35860=ADVANCED_FACE ( 'NONE', ( #43094 ), #12990, .F. ) ;
#35861=EDGE_CURVE ( 'NONE', #16010, #55867, #48464, .T. ) ;
#35862=DIRECTION ( 'NONE',  ( -0.9321478471874540261, 0.000000000000000000, 0.3620778797217457656 ) ) ;
#35863=CARTESIAN_POINT ( 'NONE',  ( -13.07066190154808361, 0.000000000000000000, 12.04713590736729678 ) ) ;
#35864=DIRECTION ( 'NONE',  ( -0.5449076811759708816, 0.6444004775717707689, 0.5364919789714475140 ) ) ;
#35865=EDGE_CURVE ( 'NONE', #54123, #52222, #49304, .T. ) ;
#35867=VECTOR ( 'NONE', #31092, 1000.000000000000227 ) ;
#35868=VERTEX_POINT ( 'NONE', #53837 ) ;
#35869=ORIENTED_EDGE ( 'NONE', *, *, #16808, .F. ) ;
#35870=VECTOR ( 'NONE', #20008, 999.9999999999998863 ) ;
#35871=CARTESIAN_POINT ( 'NONE',  ( -22.05458030558363092, -5.698858183938162902, 14.60147686105872111 ) ) ;
#35872=DIRECTION ( 'NONE',  ( 0.007781995580012662783, 0.000000000000000000, -0.9999697198139514409 ) ) ;
#35873=CARTESIAN_POINT ( 'NONE',  ( -15.87975247367846166, 0.000000000000000000, 2.850166870931599927 ) ) ;
#35874=VECTOR ( 'NONE', #6712, 999.9999999999998863 ) ;
#35875=LINE ( 'NONE', #53715, #23893 ) ;
#35876=CARTESIAN_POINT ( 'NONE',  ( -18.17048319147368218, 2.553033558614007603, 8.129316876574623763 ) ) ;
#35877=EDGE_CURVE ( 'NONE', #3706, #28890, #6431, .T. ) ;
#35878=DIRECTION ( 'NONE',  ( 0.5449076811759707706, 0.6444004775717708799, -0.5364919789714476250 ) ) ;
#35879=VECTOR ( 'NONE', #20380, 1000.000000000000227 ) ;
#35880=ORIENTED_EDGE ( 'NONE', *, *, #45389, .F. ) ;
#35881=DIRECTION ( 'NONE',  ( -0.9999697198139514409, -0.000000000000000000, -0.007781995580013368816 ) ) ;
#35882=ADVANCED_FACE ( 'NONE', ( #10710 ), #36825, .F. ) ;
#35884=VECTOR ( 'NONE', #35273, 1000.000000000000227 ) ;
#35885=VECTOR ( 'NONE', #23394, 1000.000000000000114 ) ;
#35886=ORIENTED_EDGE ( 'NONE', *, *, #26952, .T. ) ;
#35887=EDGE_CURVE ( 'NONE', #16295, #19155, #6175, .T. ) ;
#35888=LINE ( 'NONE', #27631, #47420 ) ;
#35889=FACE_OUTER_BOUND ( 'NONE', #5735, .T. ) ;
#35890=DIRECTION ( 'NONE',  ( 0.5449076811759707706, 0.6444004775717708799, -0.5364919789714476250 ) ) ;
#35891=VECTOR ( 'NONE', #4227, 1000.000000000000227 ) ;
#35892=ORIENTED_EDGE ( 'NONE', *, *, #32249, .T. ) ;
#35893=ADVANCED_FACE ( 'NONE', ( #41058 ), #53559, .F. ) ;
#35894=VECTOR ( 'NONE', #2346, 1000.000000000000114 ) ;
#35897=AXIS2_PLACEMENT_3D ( 'NONE', #10093, #4714, #44191 ) ;
#35898=ORIENTED_EDGE ( 'NONE', *, *, #24418, .T. ) ;
#35899=VECTOR ( 'NONE', #46652, 999.9999999999998863 ) ;
#35900=ORIENTED_EDGE ( 'NONE', *, *, #48930, .F. ) ;
#35901=EDGE_LOOP ( 'NONE', ( #54739, #14360, #22955, #40885 ) ) ;
#35903=ORIENTED_EDGE ( 'NONE', *, *, #27194, .T. ) ;
#35904=CARTESIAN_POINT ( 'NONE',  ( -10.37421533196711465, -0.1191753592594197858, 10.96012406864405975 ) ) ;
#35905=DIRECTION ( 'NONE',  ( 0.005002170337468016433, -0.7660444431189770143, -0.6427681459581293666 ) ) ;
#35906=EDGE_LOOP ( 'NONE', ( #48277, #54242, #32805, #28145 ) ) ;
#35907=CARTESIAN_POINT ( 'NONE',  ( -12.73749451395499577, 0.000000000000000000, 3.243952718757078912 ) ) ;
#35908=ORIENTED_EDGE ( 'NONE', *, *, #4456, .F. ) ;
#35909=CARTESIAN_POINT ( 'NONE',  ( -10.40724426834971794, 0.000000000000000000, 2.354097111786622065 ) ) ;
#35910=ORIENTED_EDGE ( 'NONE', *, *, #37786, .T. ) ;
#35911=AXIS2_PLACEMENT_3D ( 'NONE', #37518, #54282, #19658 ) ;
#35912=PLANE ( 'NONE',  #31012 ) ;
#35913=LINE ( 'NONE', #52384, #22076 ) ;
#35914=VECTOR ( 'NONE', #23832, 1000.000000000000227 ) ;
#35915=DIRECTION ( 'NONE',  ( 0.005002170337468016433, -0.7660444431189770143, -0.6427681459581293666 ) ) ;
#35916=DIRECTION ( 'NONE',  ( 0.6246952433987893460, 0.7422098413412802076, -0.2426528472758539279 ) ) ;
#35917=DIRECTION ( 'NONE',  ( 0.9999697198139515519, 0.000000000000000000, 0.007781995580013368816 ) ) ;
#35918=DIRECTION ( 'NONE',  ( -0.5449076811759708816, 0.6444004775717707689, 0.5364919789714475140 ) ) ;
#35919=VECTOR ( 'NONE', #29714, 1000.000000000000227 ) ;
#35920=ORIENTED_EDGE ( 'NONE', *, *, #51624, .F. ) ;
#35922=VERTEX_POINT ( 'NONE', #40794 ) ;
#35924=LINE ( 'NONE', #44154, #30310 ) ;
#35925=VECTOR ( 'NONE', #8898, 1000.000000000000114 ) ;
#35926=EDGE_CURVE ( 'NONE', #40269, #24198, #1864, .T. ) ;
#35927=DIRECTION ( 'NONE',  ( -0.5449076811759708816, 0.6444004775717707689, 0.5364919789714475140 ) ) ;
#35928=VECTOR ( 'NONE', #1934, 1000.000000000000114 ) ;
#35929=VECTOR ( 'NONE', #8366, 1000.000000000000227 ) ;
#35930=LINE ( 'NONE', #48962, #21313 ) ;
#35931=ORIENTED_EDGE ( 'NONE', *, *, #5016, .F. ) ;
#35932=DIRECTION ( 'NONE',  ( 0.7660212471507180654, -0.6427876096865404731, 0.005961354470445141482 ) ) ;
#35933=CARTESIAN_POINT ( 'NONE',  ( -16.79925329029790149, 0.000000000000000000, 13.49544742625427496 ) ) ;
#35934=ORIENTED_EDGE ( 'NONE', *, *, #38197, .F. ) ;
#35935=CARTESIAN_POINT ( 'NONE',  ( -13.07066190154808361, 0.000000000000000000, 12.04713590736729678 ) ) ;
#35936=VECTOR ( 'NONE', #15772, 999.9999999999998863 ) ;
#35937=DIRECTION ( 'NONE',  ( 0.005002170337468016433, -0.7660444431189770143, -0.6427681459581293666 ) ) ;
#35938=VERTEX_POINT ( 'NONE', #9585 ) ;
#35939=ADVANCED_FACE ( 'NONE', ( #26906 ), #5324, .F. ) ;
#35940=AXIS2_PLACEMENT_3D ( 'NONE', #42484, #47022, #29122 ) ;
#35941=ADVANCED_FACE ( 'NONE', ( #39940 ), #36258, .F. ) ;
#35942=EDGE_CURVE ( 'NONE', #44182, #44163, #36520, .T. ) ;
#35944=CARTESIAN_POINT ( 'NONE',  ( -9.864824628011497509, -0.1191753592594181482, 5.212971877193351311 ) ) ;
#35945=AXIS2_PLACEMENT_3D ( 'NONE', #42523, #8436, #38242 ) ;
#35946=DIRECTION ( 'NONE',  ( 0.007781995580012663651, -3.146120232559066537E-19, -0.9999697198139514409 ) ) ;
#35947=EDGE_CURVE ( 'NONE', #52744, #38022, #14663, .T. ) ;
#35948=CARTESIAN_POINT ( 'NONE',  ( -17.83139810946674686, -0.1191753592594197858, 13.85674710641801788 ) ) ;
#35950=PLANE ( 'NONE',  #55545 ) ;
#35952=VECTOR ( 'NONE', #7860, 1000.000000000000227 ) ;
#35953=ORIENTED_EDGE ( 'NONE', *, *, #34675, .T. ) ;
#35954=CARTESIAN_POINT ( 'NONE',  ( -16.29483249379484633, 0.000000000000000000, 8.386917669337709214 ) ) ;
#35955=CARTESIAN_POINT ( 'NONE',  ( -14.46888367232926420, 0.000000000000000000, 12.59025272694991315 ) ) ;
#35956=DIRECTION ( 'NONE',  ( -0.7660212471507179544, -0.6427876096865405842, -0.005961354470445141482 ) ) ;
#35957=DIRECTION ( 'NONE',  ( 0.5364919789714477361, 0.6444004775717706579, 0.5449076811759711036 ) ) ;
#35958=CARTESIAN_POINT ( 'NONE',  ( -27.06630483948590893, -0.1191753592594197858, 7.295098399573937797 ) ) ;
#35959=ORIENTED_EDGE ( 'NONE', *, *, #44688, .F. ) ;
#35960=LINE ( 'NONE', #53277, #45503 ) ;
#35961=DIRECTION ( 'NONE',  ( -0.005961354470445682716, -0.6427876096865404731, 0.7660212471507180654 ) ) ;
#35962=EDGE_CURVE ( 'NONE', #6097, #36189, #44475, .T. ) ;
#35963=AXIS2_PLACEMENT_3D ( 'NONE', #45408, #38507, #23831 ) ;
#35964=ADVANCED_FACE ( 'NONE', ( #40227 ), #1314, .F. ) ;
#35965=DIRECTION ( 'NONE',  ( 0.7660212471507180654, -0.6427876096865404731, 0.005961354470445141482 ) ) ;
#35966=PLANE ( 'NONE',  #10631 ) ;
#35967=ORIENTED_EDGE ( 'NONE', *, *, #43866, .F. ) ;
#35968=ADVANCED_FACE ( 'NONE', ( #10123 ), #31986, .F. ) ;
#35969=DIRECTION ( 'NONE',  ( -0.6246952433987894571, 0.7422098413412802076, 0.2426528472758539834 ) ) ;
#35970=ORIENTED_EDGE ( 'NONE', *, *, #41013, .T. ) ;
#35971=CARTESIAN_POINT ( 'NONE',  ( 2.072287782118878319, 0.000000000000000000, -2.950529333540147015 ) ) ;
#35972=VECTOR ( 'NONE', #13076, 999.9999999999998863 ) ;
#35973=CARTESIAN_POINT ( 'NONE',  ( -17.41835212442924430, 0.000000000000000000, 7.639510040170157446 ) ) ;
#35974=ORIENTED_EDGE ( 'NONE', *, *, #51187, .F. ) ;
#35975=ADVANCED_FACE ( 'NONE', ( #45067 ), #7531, .F. ) ;
#35976=DIRECTION ( 'NONE',  ( 0.000000000000000000, -0.000000000000000000, -1.000000000000000000 ) ) ;
#35977=VECTOR ( 'NONE', #13847, 1000.000000000000227 ) ;
#35978=ORIENTED_EDGE ( 'NONE', *, *, #25470, .T. ) ;
#35979=EDGE_CURVE ( 'NONE', #41338, #33009, #50957, .T. ) ;
#35980=VERTEX_POINT ( 'NONE', #46151 ) ;
#35981=VECTOR ( 'NONE', #16082, 1000.000000000000114 ) ;
#35982=ORIENTED_EDGE ( 'NONE', *, *, #38842, .T. ) ;
#35983=CARTESIAN_POINT ( 'NONE',  ( -10.94028622754223967, 0.000000000000000000, 11.14038480894692995 ) ) ;
#35984=ORIENTED_EDGE ( 'NONE', *, *, #56190, .T. ) ;
#35985=ORIENTED_EDGE ( 'NONE', *, *, #30452, .T. ) ;
#35986=CARTESIAN_POINT ( 'NONE',  ( 2.072287782118878319, 0.000000000000000000, -2.950529333540147015 ) ) ;
#35987=DIRECTION ( 'NONE',  ( -0.5449076811759708816, 0.6444004775717707689, 0.5364919789714475140 ) ) ;
#35988=ORIENTED_EDGE ( 'NONE', *, *, #15972, .T. ) ;
#35989=VECTOR ( 'NONE', #28802, 1000.000000000000000 ) ;
#35990=VECTOR ( 'NONE', #42719, 1000.000000000000227 ) ;
#35991=ORIENTED_EDGE ( 'NONE', *, *, #17215, .F. ) ;
#35992=DIRECTION ( 'NONE',  ( 0.2426528472758541499, 0.7422098413412800966, 0.6246952433987894571 ) ) ;
#35994=ORIENTED_EDGE ( 'NONE', *, *, #51623, .F. ) ;
#35995=AXIS2_PLACEMENT_3D ( 'NONE', #50172, #37383, #26052 ) ;
#35996=AXIS2_PLACEMENT_3D ( 'NONE', #13445, #353, #38423 ) ;
#35997=CARTESIAN_POINT ( 'NONE',  ( -16.26321790523673982, 0.000000000000000000, 4.324510933502299537 ) ) ;
#35998=CARTESIAN_POINT ( 'NONE',  ( -14.04166784449981442, 0.4483081953215036219, 3.071331889294571571 ) ) ;
#35999=DIRECTION ( 'NONE',  ( 0.007781995580012663651, -3.146120232559066537E-19, -0.9999697198139514409 ) ) ;
#36000=CARTESIAN_POINT ( 'NONE',  ( -13.63673279712320507, -0.1191753592594197858, 12.22739664767016521 ) ) ;
#36001=VERTEX_POINT ( 'NONE', #3287 ) ;
#36002=DIRECTION ( 'NONE',  ( 0.007781995580012663651, -3.146120232559066537E-19, -0.9999697198139514409 ) ) ;
#36003=ORIENTED_EDGE ( 'NONE', *, *, #41459, .F. ) ;
#36004=DIRECTION ( 'NONE',  ( 0.7660212471507180654, -0.6427876096865404731, 0.005961354470445141482 ) ) ;
#36005=VECTOR ( 'NONE', #37211, 999.9999999999998863 ) ;
#36006=CARTESIAN_POINT ( 'NONE',  ( -26.13337879274045505, 0.000000000000000000, 6.833023547870798353 ) ) ;
#36008=CARTESIAN_POINT ( 'NONE',  ( -15.34987077819697987, 0.000000000000000000, 6.378285217289930031 ) ) ;
#36009=CARTESIAN_POINT ( 'NONE',  ( -15.35849293871282839, 0.000000000000000000, 7.486214327063223095 ) ) ;
#36010=CARTESIAN_POINT ( 'NONE',  ( -19.52717239714547048, 0.000000000000000000, 5.776438364157291616 ) ) ;
#36011=ORIENTED_EDGE ( 'NONE', *, *, #30697, .T. ) ;
#36012=CARTESIAN_POINT ( 'NONE',  ( -18.33038159707971815, 0.000000000000000000, 5.416419997087551508 ) ) ;
#36014=EDGE_CURVE ( 'NONE', #7707, #23956, #28559, .T. ) ;
#36015=CARTESIAN_POINT ( 'NONE',  ( -13.17065887352947762, -0.1191753592594197858, 12.04635770780929427 ) ) ;
#36016=DIRECTION ( 'NONE',  ( 0.5364919789714477361, 0.6444004775717706579, 0.5449076811759711036 ) ) ;
#36017=VECTOR ( 'NONE', #26863, 1000.000000000000227 ) ;
#36018=DIRECTION ( 'NONE',  ( 0.005002170337468016433, -0.7660444431189770143, -0.6427681459581293666 ) ) ;
#36019=FACE_OUTER_BOUND ( 'NONE', #34921, .T. ) ;
#36020=EDGE_CURVE ( 'NONE', #45510, #54842, #37928, .T. ) ;
#36021=LINE ( 'NONE', #28031, #11438 ) ;
#36022=AXIS2_PLACEMENT_3D ( 'NONE', #13503, #13224, #48119 ) ;
#36024=VERTEX_POINT ( 'NONE', #55236 ) ;
#36025=CARTESIAN_POINT ( 'NONE',  ( -16.50344859827348287, 0.000000000000000000, 9.493290379994999029 ) ) ;
#36026=LINE ( 'NONE', #23497, #36747 ) ;
#36027=FACE_OUTER_BOUND ( 'NONE', #50547, .T. ) ;
#36028=VECTOR ( 'NONE', #27441, 999.9999999999998863 ) ;
#36030=FACE_OUTER_BOUND ( 'NONE', #32924, .T. ) ;
#36031=DIRECTION ( 'NONE',  ( 0.6427681459581294776, -0.7660444431189769032, 0.005002170337467562802 ) ) ;
#36032=VECTOR ( 'NONE', #17621, 1000.000000000000114 ) ;
#36033=DIRECTION ( 'NONE',  ( 0.5364919789714477361, 0.6444004775717706579, 0.5449076811759711036 ) ) ;
#36034=FACE_OUTER_BOUND ( 'NONE', #4550, .T. ) ;
#36035=ORIENTED_EDGE ( 'NONE', *, *, #48832, .T. ) ;
#36036=EDGE_CURVE ( 'NONE', #32655, #25448, #54138, .T. ) ;
#36037=ORIENTED_EDGE ( 'NONE', *, *, #52219, .T. ) ;
#36038=ORIENTED_EDGE ( 'NONE', *, *, #39364, .T. ) ;
#36039=ORIENTED_EDGE ( 'NONE', *, *, #55319, .T. ) ;
#36040=EDGE_CURVE ( 'NONE', #17655, #24033, #12066, .T. ) ;
#36041=VERTEX_POINT ( 'NONE', #7842 ) ;
#36042=CARTESIAN_POINT ( 'NONE',  ( -27.06552663992790997, 0.000000000000000000, 7.195101427592543786 ) ) ;
#36043=DIRECTION ( 'NONE',  ( 0.7660212471507180654, -0.6427876096865404731, 0.005961354470445141482 ) ) ;
#36044=VERTEX_POINT ( 'NONE', #11787 ) ;
#36046=ORIENTED_EDGE ( 'NONE', *, *, #22966, .T. ) ;
#36047=ADVANCED_FACE ( 'NONE', ( #7003 ), #41616, .F. ) ;
#36049=AXIS2_PLACEMENT_3D ( 'NONE', #37890, #3517, #7485 ) ;
#36051=LINE ( 'NONE', #10173, #6503 ) ;
#36052=PLANE ( 'NONE',  #9584 ) ;
#36053=ORIENTED_EDGE ( 'NONE', *, *, #47393, .F. ) ;
#36054=PLANE ( 'NONE',  #152 ) ;
#36055=EDGE_LOOP ( 'NONE', ( #12025, #50733, #28235, #14339 ) ) ;
#36056=AXIS2_PLACEMENT_3D ( 'NONE', #36195, #39880, #53497 ) ;
#36057=CARTESIAN_POINT ( 'NONE',  ( -13.53673582514181106, 0.000000000000000000, 12.22817484722816772 ) ) ;
#36058=CARTESIAN_POINT ( 'NONE',  ( -13.95122827149485190, -0.03228989815065406305, 2.299421746729317206 ) ) ;
#36059=CARTESIAN_POINT ( 'NONE',  ( -23.33849165029409889, 0.000000000000000000, 5.946783852668351855 ) ) ;
#36060=DIRECTION ( 'NONE',  ( 0.5364919789714477361, 0.6444004775717706579, 0.5449076811759711036 ) ) ;
#36061=FACE_OUTER_BOUND ( 'NONE', #23483, .T. ) ;
#36062=CARTESIAN_POINT ( 'NONE',  ( -11.95923551588343337, 9.532254668142648768, 1.426999636052985965 ) ) ;
#36063=FACE_OUTER_BOUND ( 'NONE', #51614, .T. ) ;
#36064=ORIENTED_EDGE ( 'NONE', *, *, #23683, .T. ) ;
#36065=PLANE ( 'NONE',  #41010 ) ;
#36066=EDGE_CURVE ( 'NONE', #41646, #38799, #29106, .T. ) ;
#36067=ORIENTED_EDGE ( 'NONE', *, *, #38526, .F. ) ;
#36068=ADVANCED_FACE ( 'NONE', ( #15240 ), #29400, .F. ) ;
#36069=DIRECTION ( 'NONE',  ( -0.005002170337468016433, -0.7660444431189770143, 0.6427681459581293666 ) ) ;
#36070=CARTESIAN_POINT ( 'NONE',  ( -14.46888367232926420, 0.000000000000000000, 12.59025272694991315 ) ) ;
#36072=FACE_OUTER_BOUND ( 'NONE', #14244, .T. ) ;
#36073=CARTESIAN_POINT ( 'NONE',  ( -17.93139508144814442, 0.000000000000000000, 13.85596890686001537 ) ) ;
#36074=CARTESIAN_POINT ( 'NONE',  ( -11.20636620717317378, 0.000000000000000000, 11.32298014792380414 ) ) ;
#36076=ADVANCED_FACE ( 'NONE', ( #45590 ), #6707, .F. ) ;
#36077=DIRECTION ( 'NONE',  ( 0.007781995580012662783, 0.000000000000000000, -0.9999697198139514409 ) ) ;
#36078=DIRECTION ( 'NONE',  ( 0.007781995580012663651, 0.000000000000000000, -0.9999697198139515519 ) ) ;
#36079=PLANE ( 'NONE',  #596 ) ;
#36080=VERTEX_POINT ( 'NONE', #11236 ) ;
#36081=DIRECTION ( 'NONE',  ( 0.6427681459581294776, -0.7660444431189769032, 0.005002170337467562802 ) ) ;
#36082=FACE_OUTER_BOUND ( 'NONE', #10242, .T. ) ;
#36084=DIRECTION ( 'NONE',  ( -0.7660212471507179544, -0.6427876096865405842, -0.005961354470445141482 ) ) ;
#36085=CARTESIAN_POINT ( 'NONE',  ( -15.88130887279446490, 0.000000000000000000, 3.050160814894388839 ) ) ;
#36086=CARTESIAN_POINT ( 'NONE',  ( -9.972665560950739305, 0.000000000000000000, 6.220125815427252292 ) ) ;
#36087=LINE ( 'NONE', #19019, #1114 ) ;
#36088=ADVANCED_FACE ( 'NONE', ( #42177 ), #41358, .F. ) ;
#36089=EDGE_LOOP ( 'NONE', ( #20068, #25053, #37886, #1212 ) ) ;
#36090=VECTOR ( 'NONE', #30501, 999.9999999999998863 ) ;
#36091=ORIENTED_EDGE ( 'NONE', *, *, #56043, .T. ) ;
#36092=CARTESIAN_POINT ( 'NONE',  ( -13.49419724433792034, 0.000000000000000000, 6.762058567619732230 ) ) ;
#36093=FACE_OUTER_BOUND ( 'NONE', #42220, .T. ) ;
#36094=VECTOR ( 'NONE', #22766, 1000.000000000000000 ) ;
#36095=EDGE_LOOP ( 'NONE', ( #48087, #47557, #18455, #48612 ) ) ;
#36097=ORIENTED_EDGE ( 'NONE', *, *, #48184, .F. ) ;
#36098=DIRECTION ( 'NONE',  ( 0.007781995580012662783, 0.000000000000000000, -0.9999697198139514409 ) ) ;
#36099=EDGE_LOOP ( 'NONE', ( #13885, #807, #7491, #7242 ) ) ;
#36100=EDGE_LOOP ( 'NONE', ( #10258, #30650, #27642, #37085 ) ) ;
#36101=EDGE_LOOP ( 'NONE', ( #14629, #12790, #19620, #43066 ) ) ;
#36102=DIRECTION ( 'NONE',  ( 0.2426528472758541499, 0.7422098413412800966, 0.6246952433987894571 ) ) ;
#36103=LINE ( 'NONE', #11056, #34105 ) ;
#36104=FACE_OUTER_BOUND ( 'NONE', #28339, .T. ) ;
#36105=DIRECTION ( 'NONE',  ( 0.6427681459581294776, -0.7660444431189769032, 0.005002170337467562802 ) ) ;
#36106=VERTEX_POINT ( 'NONE', #25163 ) ;
#36107=EDGE_CURVE ( 'NONE', #14388, #39202, #42468, .T. ) ;
#36108=VERTEX_POINT ( 'NONE', #37091 ) ;
#36109=DIRECTION ( 'NONE',  ( -0.6427681459581293666, -0.7660444431189770143, -0.005002170337467561935 ) ) ;
#36110=ORIENTED_EDGE ( 'NONE', *, *, #9960, .T. ) ;
#36111=DIRECTION ( 'NONE',  ( 0.7660212471507180654, -0.6427876096865404731, 0.005961354470445141482 ) ) ;
#36112=VERTEX_POINT ( 'NONE', #20308 ) ;
#36113=PLANE ( 'NONE',  #29676 ) ;
#36114=PLANE ( 'NONE',  #37592 ) ;
#36115=ADVANCED_FACE ( 'NONE', ( #50429 ), #11536, .F. ) ;
#36116=ORIENTED_EDGE ( 'NONE', *, *, #37865, .T. ) ;
#36117=LINE ( 'NONE', #1155, #43133 ) ;
#36118=VERTEX_POINT ( 'NONE', #16071 ) ;
#36119=ADVANCED_FACE ( 'NONE', ( #13210 ), #12383, .F. ) ;
#36120=EDGE_CURVE ( 'NONE', #35683, #28956, #47561, .T. ) ;
#36121=LINE ( 'NONE', #52573, #45398 ) ;
#36122=EDGE_LOOP ( 'NONE', ( #45216, #31072, #50704, #6805 ) ) ;
#36123=CARTESIAN_POINT ( 'NONE',  ( 2.072287782118878319, 0.000000000000000000, -2.950529333540147015 ) ) ;
#36124=DIRECTION ( 'NONE',  ( 0.6427681459581294776, -0.7660444431189769032, 0.005002170337467562802 ) ) ;
#36125=DIRECTION ( 'NONE',  ( 0.007781995580012663651, 0.000000000000000000, -0.9999697198139515519 ) ) ;
#36126=ADVANCED_FACE ( 'NONE', ( #35090 ), #29962, .F. ) ;
#36127=ORIENTED_EDGE ( 'NONE', *, *, #38328, .T. ) ;
#36128=AXIS2_PLACEMENT_3D ( 'NONE', #25173, #46734, #8386 ) ;
#36129=ADVANCED_FACE ( 'NONE', ( #21992 ), #4674, .F. ) ;
#36130=PLANE ( 'NONE',  #31951 ) ;
#36131=LINE ( 'NONE', #9989, #16759 ) ;
#36133=CARTESIAN_POINT ( 'NONE',  ( -15.32819600454399911, 0.000000000000000000, 3.593123350522788417 ) ) ;
#36134=EDGE_CURVE ( 'NONE', #52431, #42836, #8677, .T. ) ;
#36135=DIRECTION ( 'NONE',  ( -0.9999697198139514409, -0.000000000000000000, -0.007781995580013368816 ) ) ;
#36137=EDGE_LOOP ( 'NONE', ( #10169, #18855, #30775 ) ) ;
#36138=LINE ( 'NONE', #49467, #4428 ) ;
#36139=LINE ( 'NONE', #27304, #6863 ) ;
#36141=ORIENTED_EDGE ( 'NONE', *, *, #14953, .T. ) ;
#36143=CARTESIAN_POINT ( 'NONE',  ( -15.00597892355332696, -0.1191753592594181482, 9.047205394761215658 ) ) ;
#36144=EDGE_LOOP ( 'NONE', ( #47231, #35123, #5004, #19956 ) ) ;
#36145=EDGE_CURVE ( 'NONE', #9862, #31, #25417, .T. ) ;
#36146=LINE ( 'NONE', #53707, #45783 ) ;
#36147=CARTESIAN_POINT ( 'NONE',  ( -19.60912206198628027, -0.1191753592594197858, 4.398475361799976113 ) ) ;
#36148=PLANE ( 'NONE',  #25593 ) ;
#36149=EDGE_CURVE ( 'NONE', #19918, #47466, #409, .T. ) ;
#36150=EDGE_LOOP ( 'NONE', ( #13637, #20601, #21758, #52152 ) ) ;
#36153=CARTESIAN_POINT ( 'NONE',  ( -11.67244013076689946, 0.000000000000000000, 11.50401908778467863 ) ) ;
#36154=FACE_OUTER_BOUND ( 'NONE', #36226, .T. ) ;
#36155=FACE_OUTER_BOUND ( 'NONE', #47311, .T. ) ;
#36156=ORIENTED_EDGE ( 'NONE', *, *, #12249, .T. ) ;
#36157=LINE ( 'NONE', #53718, #12240 ) ;
#36158=EDGE_LOOP ( 'NONE', ( #27936, #12592, #49515 ) ) ;
#36159=FACE_OUTER_BOUND ( 'NONE', #50247, .T. ) ;
#36160=DIRECTION ( 'NONE',  ( -0.5449076811759708816, 0.6444004775717707689, 0.5364919789714475140 ) ) ;
#36161=EDGE_LOOP ( 'NONE', ( #21122, #14317, #24667, #5990 ) ) ;
#36162=DIRECTION ( 'NONE',  ( 0.7660212471507180654, -0.6427876096865404731, 0.005961354470445141482 ) ) ;
#36163=CARTESIAN_POINT ( 'NONE',  ( -25.20123094555300369, 0.000000000000000000, 6.470945668149052032 ) ) ;
#36164=CARTESIAN_POINT ( 'NONE',  ( -24.27063949748155380, 0.000000000000000000, 6.308861732390097288 ) ) ;
#36165=ORIENTED_EDGE ( 'NONE', *, *, #28455, .F. ) ;
#36166=AXIS2_PLACEMENT_3D ( 'NONE', #31851, #48629, #48318 ) ;
#36167=PLANE ( 'NONE',  #2951 ) ;
#36168=ADVANCED_FACE ( 'NONE', ( #26527 ), #111, .F. ) ;
#36171=ORIENTED_EDGE ( 'NONE', *, *, #38165, .T. ) ;
#36172=DIRECTION ( 'NONE',  ( 0.005961354470445682716, -0.6427876096865404731, -0.7660212471507180654 ) ) ;
#36173=VERTEX_POINT ( 'NONE', #4131 ) ;
#36174=DIRECTION ( 'NONE',  ( 0.000000000000000000, -1.000000000000000000, 0.000000000000000000 ) ) ;
#36175=ORIENTED_EDGE ( 'NONE', *, *, #2727, .T. ) ;
#36176=DIRECTION ( 'NONE',  ( -0.5449076811759708816, 0.6444004775717707689, 0.5364919789714475140 ) ) ;
#36177=DIRECTION ( 'NONE',  ( 0.000000000000000000, -1.000000000000000000, 0.000000000000000000 ) ) ;
#36178=VERTEX_POINT ( 'NONE', #8958 ) ;
#36179=DIRECTION ( 'NONE',  ( -0.6427681459581293666, -0.7660444431189770143, -0.005002170337467561935 ) ) ;
#36180=ORIENTED_EDGE ( 'NONE', *, *, #33874, .F. ) ;
#36181=EDGE_CURVE ( 'NONE', #40214, #33948, #17180, .T. ) ;
#36182=DIRECTION ( 'NONE',  ( 0.007781995580012663651, -3.146120232559066537E-19, -0.9999697198139514409 ) ) ;
#36183=DIRECTION ( 'NONE',  ( 0.000000000000000000, -0.000000000000000000, -1.000000000000000000 ) ) ;
#36185=LINE ( 'NONE', #14589, #8472 ) ;
#36186=CARTESIAN_POINT ( 'NONE',  ( -13.65781925808015629, 0.000000000000000000, 2.086787245668887625 ) ) ;
#36187=FACE_OUTER_BOUND ( 'NONE', #18972, .T. ) ;
#36188=CARTESIAN_POINT ( 'NONE',  ( -14.26730381667732850, 1.257817950434004128, 4.487519983270500390 ) ) ;
#36189=VERTEX_POINT ( 'NONE', #17753 ) ;
#36190=ORIENTED_EDGE ( 'NONE', *, *, #13098, .T. ) ;
#36191=EDGE_CURVE ( 'NONE', #56078, #36080, #26260, .T. ) ;
#36192=CARTESIAN_POINT ( 'NONE',  ( -13.20943591692264718, 0.000000000000000000, 4.178950157467387960 ) ) ;
#36193=DIRECTION ( 'NONE',  ( 0.9999697198139515519, 0.000000000000000000, 0.007781995580013368816 ) ) ;
#36194=EDGE_CURVE ( 'NONE', #13117, #31769, #30807, .T. ) ;
#36195=CARTESIAN_POINT ( 'NONE',  ( -18.19747506107908563, 0.000000000000000000, 14.03856424583689311 ) ) ;
#36196=CARTESIAN_POINT ( 'NONE',  ( -16.06709938707323460, 0.000000000000000000, 13.13181314741652628 ) ) ;
#36197=ORIENTED_EDGE ( 'NONE', *, *, #44878, .T. ) ;
#36198=FACE_OUTER_BOUND ( 'NONE', #1007, .T. ) ;
#36199=DIRECTION ( 'NONE',  ( 0.9999697198139515519, 0.000000000000000000, 0.007781995580013368816 ) ) ;
#36200=ORIENTED_EDGE ( 'NONE', *, *, #31239, .T. ) ;
#36201=CARTESIAN_POINT ( 'NONE',  ( -11.80115495887297428, 0.000000000000000000, 2.343249376482593682 ) ) ;
#36203=EDGE_LOOP ( 'NONE', ( #21763, #31841, #3881 ) ) ;
#36204=ADVANCED_FACE ( 'NONE', ( #55804 ), #34781, .F. ) ;
#36205=MECHANICAL_DESIGN_GEOMETRIC_PRESENTATION_REPRESENTATION('',(#56136),#11700);
#36206=DIRECTION ( 'NONE',  ( -0.005961354470445682716, -0.6427876096865404731, 0.7660212471507180654 ) ) ;
#36207=PLANE ( 'NONE',  #15165 ) ;
#36208=LINE ( 'NONE', #14610, #16872 ) ;
#36209=CARTESIAN_POINT ( 'NONE',  ( 2.072287782118878319, 0.000000000000000000, -2.950529333540147015 ) ) ;
#36210=PLANE ( 'NONE',  #24694 ) ;
#36211=ADVANCED_FACE ( 'NONE', ( #26006 ), #38187, .F. ) ;
#36212=ORIENTED_EDGE ( 'NONE', *, *, #52340, .F. ) ;
#36213=ORIENTED_EDGE ( 'NONE', *, *, #47121, .T. ) ;
#36214=FACE_OUTER_BOUND ( 'NONE', #37758, .T. ) ;
#36215=CARTESIAN_POINT ( 'NONE',  ( -14.66887761629205222, 0.000000000000000000, 12.58869632783390990 ) ) ;
#36216=PLANE ( 'NONE',  #22465 ) ;
#36217=DIRECTION ( 'NONE',  ( 0.9999697198139515519, 0.000000000000000000, 0.007781995580013368816 ) ) ;
#36218=DIRECTION ( 'NONE',  ( 0.6246952433987893460, 0.7422098413412802076, -0.2426528472758539279 ) ) ;
#36219=ORIENTED_EDGE ( 'NONE', *, *, #36617, .T. ) ;
#36220=DIRECTION ( 'NONE',  ( -0.6427681459581293666, -0.7660444431189770143, -0.005002170337467561935 ) ) ;
#36221=CARTESIAN_POINT ( 'NONE',  ( -16.81267852042393685, -0.1191753592594198830, 3.312241722634738927 ) ) ;
#36222=DIRECTION ( 'NONE',  ( -0.9999697198139514409, -0.000000000000000000, -0.007781995580013368816 ) ) ;
#36224=EDGE_LOOP ( 'NONE', ( #2750, #10795, #21564, #5429 ) ) ;
#36226=EDGE_LOOP ( 'NONE', ( #39467, #1075, #28698, #37685 ) ) ;
#36227=CARTESIAN_POINT ( 'NONE',  ( -16.94221901356702631, 0.000000000000000000, 6.165887138907109488 ) ) ;
#36228=EDGE_CURVE ( 'NONE', #636, #9012, #33942, .T. ) ;
#36229=CARTESIAN_POINT ( 'NONE',  ( -15.60102546347950536, 0.000000000000000000, 12.95077420755565356 ) ) ;
#36230=ORIENTED_EDGE ( 'NONE', *, *, #8144, .T. ) ;
#36231=CARTESIAN_POINT ( 'NONE',  ( -17.90602012812457389, 4.495856970884009485, 3.493796664491064963 ) ) ;
#36233=ORIENTED_EDGE ( 'NONE', *, *, #43077, .F. ) ;
#36234=ORIENTED_EDGE ( 'NONE', *, *, #16891, .T. ) ;
#36235=VERTEX_POINT ( 'NONE', #51550 ) ;
#36236=CARTESIAN_POINT ( 'NONE',  ( -13.99411872359561926, -2.298917212465658721, 2.243764576467674576 ) ) ;
#36237=EDGE_LOOP ( 'NONE', ( #46275, #34415, #25685, #48272 ) ) ;
#36238=EDGE_CURVE ( 'NONE', #42908, #49004, #53249, .T. ) ;
#36239=ORIENTED_EDGE ( 'NONE', *, *, #36947, .T. ) ;
#36240=CARTESIAN_POINT ( 'NONE',  ( -19.60990026154428278, 0.000000000000000000, 4.498472333781370125 ) ) ;
#36241=LINE ( 'NONE', #1846, #21319 ) ;
#36242=ORIENTED_EDGE ( 'NONE', *, *, #50063, .T. ) ;
#36243=ADVANCED_FACE ( 'NONE', ( #10344 ), #14042, .F. ) ;
#36244=EDGE_CURVE ( 'NONE', #3565, #35683, #48697, .T. ) ;
#36245=EDGE_CURVE ( 'NONE', #27257, #12509, #27106, .T. ) ;
#36246=ORIENTED_EDGE ( 'NONE', *, *, #36857, .F. ) ;
#36247=LINE ( 'NONE', #39380, #25845 ) ;
#36248=ORIENTED_EDGE ( 'NONE', *, *, #19999, .T. ) ;
#36249=ORIENTED_EDGE ( 'NONE', *, *, #42840, .T. ) ;
#36250=CARTESIAN_POINT ( 'NONE',  ( -21.55158313111639146, -4.079838673713161334, 5.122519686159045627 ) ) ;
#36252=DIRECTION ( 'NONE',  ( 0.5364919789714477361, 0.6444004775717706579, 0.5449076811759711036 ) ) ;
#36253=DIRECTION ( 'NONE',  ( 0.005002170337468016433, -0.7660444431189770143, -0.6427681459581293666 ) ) ;
#36254=ORIENTED_EDGE ( 'NONE', *, *, #10964, .T. ) ;
#36255=DIRECTION ( 'NONE',  ( -0.5364919789714478471, 0.6444004775717705469, -0.5449076811759709926 ) ) ;
#36256=ORIENTED_EDGE ( 'NONE', *, *, #7096, .T. ) ;
#36257=ADVANCED_FACE ( 'NONE', ( #49229 ), #27956, .F. ) ;
#36258=PLANE ( 'NONE',  #13918 ) ;
#36259=EDGE_CURVE ( 'NONE', #26566, #25938, #10649, .T. ) ;
#36260=CARTESIAN_POINT ( 'NONE',  ( -11.59291107943755605, 0.000000000000000000, 1.284706784507182231 ) ) ;
#36262=CARTESIAN_POINT ( 'NONE',  ( -17.74560456716937296, 0.000000000000000000, 3.774316574337878372 ) ) ;
#36264=ADVANCED_FACE ( 'NONE', ( #36447 ), #18581, .F. ) ;
#36265=DIRECTION ( 'NONE',  ( 0.000000000000000000, -1.000000000000000000, 0.000000000000000000 ) ) ;
#36266=CARTESIAN_POINT ( 'NONE',  ( -13.13049853634656472, 5.467268677019015755, 1.607828781524239803 ) ) ;
#36267=EDGE_LOOP ( 'NONE', ( #31557, #17197, #13402, #21003 ) ) ;
#36268=LINE ( 'NONE', #44233, #17460 ) ;
#36269=VERTEX_POINT ( 'NONE', #53761 ) ;
#36270=EDGE_CURVE ( 'NONE', #51541, #55849, #5514, .T. ) ;
#36271=LINE ( 'NONE', #11544, #17468 ) ;
#36272=CARTESIAN_POINT ( 'NONE',  ( -16.48201256934722636, 0.000000000000000000, 6.738806697895671327 ) ) ;
#36273=LINE ( 'NONE', #28029, #38110 ) ;
#36274=DIRECTION ( 'NONE',  ( 0.6427681459581294776, -0.7660444431189769032, 0.005002170337467562802 ) ) ;
#36275=CARTESIAN_POINT ( 'NONE',  ( -17.46532115785441519, 0.000000000000000000, 13.67492996699914265 ) ) ;
#36277=ORIENTED_EDGE ( 'NONE', *, *, #16292, .F. ) ;
#36279=LINE ( 'NONE', #1635, #33984 ) ;
#36280=DIRECTION ( 'NONE',  ( 0.000000000000000000, -1.000000000000000000, 0.000000000000000000 ) ) ;
#36281=CARTESIAN_POINT ( 'NONE',  ( -19.70178816256107979, -1.327505506330656670, 4.491810339156243614 ) ) ;
#36282=DIRECTION ( 'NONE',  ( 0.7660212471507180654, -0.6427876096865404731, 0.005961354470445141482 ) ) ;
#36283=CARTESIAN_POINT ( 'NONE',  ( -8.509919637592204822, -0.1191753592594197858, 10.23596830920056711 ) ) ;
#36284=DIRECTION ( 'NONE',  ( -0.5449076811759708816, 0.6444004775717707689, 0.5364919789714475140 ) ) ;
#36285=DIRECTION ( 'NONE',  ( -0.5449076811759708816, 0.6444004775717707689, 0.5364919789714475140 ) ) ;
#36286=EDGE_LOOP ( 'NONE', ( #38425, #26948, #4319, #52563 ) ) ;
#36287=VERTEX_POINT ( 'NONE', #14342 ) ;
#36288=ORIENTED_EDGE ( 'NONE', *, *, #12704, .F. ) ;
#36289=ORIENTED_EDGE ( 'NONE', *, *, #12763, .F. ) ;
#36290=ORIENTED_EDGE ( 'NONE', *, *, #47098, .F. ) ;
#36291=FACE_OUTER_BOUND ( 'NONE', #20898, .T. ) ;
#36293=EDGE_CURVE ( 'NONE', #21366, #24619, #45257, .T. ) ;
#36294=EDGE_CURVE ( 'NONE', #29459, #51867, #44685, .T. ) ;
#36295=ORIENTED_EDGE ( 'NONE', *, *, #8153, .T. ) ;
#36296=VERTEX_POINT ( 'NONE', #52936 ) ;
#36297=ORIENTED_EDGE ( 'NONE', *, *, #27384, .T. ) ;
#36298=ADVANCED_FACE ( 'NONE', ( #14880 ), #27366, .F. ) ;
#36299=AXIS2_PLACEMENT_3D ( 'NONE', #30629, #17841, #47931 ) ;
#36300=DIRECTION ( 'NONE',  ( 0.6427681459581294776, -0.7660444431189769032, 0.005002170337467562802 ) ) ;
#36301=CARTESIAN_POINT ( 'NONE',  ( -11.36525859708471486, 0.000000000000000000, 6.039962320828248465 ) ) ;
#36302=DIRECTION ( 'NONE',  ( -0.005002170337468016433, -0.7660444431189770143, 0.6427681459581293666 ) ) ;
#36303=ORIENTED_EDGE ( 'NONE', *, *, #43739, .F. ) ;
#36305=ORIENTED_EDGE ( 'NONE', *, *, #3288, .T. ) ;
#36306=CARTESIAN_POINT ( 'NONE',  ( -22.40478740399063895, 0.000000000000000000, 5.384712028983816623 ) ) ;
#36307=CARTESIAN_POINT ( 'NONE',  ( -15.36843275361795591, 0.000000000000000000, 8.763459196131494267 ) ) ;
#36308=ADVANCED_FACE ( 'NONE', ( #22294 ), #14596, .F. ) ;
#36309=LINE ( 'NONE', #27225, #13707 ) ;
#36310=PLANE ( 'NONE',  #656 ) ;
#36311=CARTESIAN_POINT ( 'NONE',  ( -13.71393590006033492, 0.6102101463440037232, 3.209738356201059073 ) ) ;
#36312=PLANE ( 'NONE',  #54676 ) ;
#36313=LINE ( 'NONE', #6491, #41218 ) ;
#36314=ADVANCED_FACE ( 'NONE', ( #39626 ), #705, .F. ) ;
#36315=EDGE_LOOP ( 'NONE', ( #8935, #32281, #11516, #43797 ) ) ;
#36316=CARTESIAN_POINT ( 'NONE',  ( -21.47341775636118655, -0.1191753592594197858, 5.122631121243466090 ) ) ;
#36317=ORIENTED_EDGE ( 'NONE', *, *, #48328, .T. ) ;
#36318=EDGE_CURVE ( 'NONE', #55206, #16632, #31068, .T. ) ;
#36319=CARTESIAN_POINT ( 'NONE',  ( -8.609916609573598834, 0.000000000000000000, 10.23519010964256637 ) ) ;
#36320=CARTESIAN_POINT ( 'NONE',  ( -18.39746900504187010, 0.000000000000000000, 14.03700784672088808 ) ) ;
#36321=LINE ( 'NONE', #33656, #17701 ) ;
#36322=CARTESIAN_POINT ( 'NONE',  ( -10.00813838035478298, 0.000000000000000000, 10.77830692922518452 ) ) ;
#36323=DIRECTION ( 'NONE',  ( -0.5364919789714478471, 0.6444004775717705469, -0.5449076811759709926 ) ) ;
#36324=EDGE_CURVE ( 'NONE', #5802, #39181, #35924, .T. ) ;
#36325=DIRECTION ( 'NONE',  ( -0.005961354470445682716, -0.6427876096865404731, 0.7660212471507180654 ) ) ;
#36326=DIRECTION ( 'NONE',  ( 0.6427681459581294776, -0.7660444431189769032, 0.005002170337467562802 ) ) ;
#36327=DIRECTION ( 'NONE',  ( 0.000000000000000000, -1.000000000000000000, 0.000000000000000000 ) ) ;
#36329=FACE_OUTER_BOUND ( 'NONE', #22732, .T. ) ;
#36330=EDGE_LOOP ( 'NONE', ( #55357, #43158, #17275, #1706 ) ) ;
#36331=CARTESIAN_POINT ( 'NONE',  ( -17.26532721389163072, 0.000000000000000000, 13.67648636611514590 ) ) ;
#36332=LINE ( 'NONE', #10514, #11320 ) ;
#36333=DIRECTION ( 'NONE',  ( -0.6427681459581293666, -0.7660444431189770143, -0.005002170337467561935 ) ) ;
#36335=FACE_OUTER_BOUND ( 'NONE', #23967, .T. ) ;
#36336=ADVANCED_FACE ( 'NONE', ( #33582 ), #33330, .F. ) ;
#36337=DIRECTION ( 'NONE',  ( -0.5364919789714478471, 0.6444004775717705469, -0.5449076811759709926 ) ) ;
#36338=FACE_OUTER_BOUND ( 'NONE', #38600, .T. ) ;
#36339=DIRECTION ( 'NONE',  ( 0.9999697198139515519, 0.000000000000000000, 0.007781995580013368816 ) ) ;
#36340=EDGE_LOOP ( 'NONE', ( #14918, #14714, #9297, #39786 ) ) ;
#36341=VECTOR ( 'NONE', #23067, 999.9999999999998863 ) ;
#36342=ORIENTED_EDGE ( 'NONE', *, *, #19148, .T. ) ;
#36343=DIRECTION ( 'NONE',  ( 0.5449076811759707706, 0.6444004775717708799, -0.5364919789714476250 ) ) ;
#36344=CARTESIAN_POINT ( 'NONE',  ( -13.84758239767214860, 4.657758921906512306, 1.912196104970483868 ) ) ;
#36345=ORIENTED_EDGE ( 'NONE', *, *, #13030, .F. ) ;
#36346=LINE ( 'NONE', #31552, #16784 ) ;
#36347=ORIENTED_EDGE ( 'NONE', *, *, #46434, .T. ) ;
#36348=DIRECTION ( 'NONE',  ( -0.9999697198139514409, -0.000000000000000000, -0.007781995580013368816 ) ) ;
#36349=ORIENTED_EDGE ( 'NONE', *, *, #19934, .T. ) ;
#36350=ORIENTED_EDGE ( 'NONE', *, *, #41686, .T. ) ;
#36351=ORIENTED_EDGE ( 'NONE', *, *, #12255, .T. ) ;
#36352=DIRECTION ( 'NONE',  ( 0.9999697198139515519, 0.000000000000000000, 0.007781995580013368816 ) ) ;
#36353=FACE_OUTER_BOUND ( 'NONE', #8207, .T. ) ;
#36354=CARTESIAN_POINT ( 'NONE',  ( -16.81190032086591302, 0.000000000000000000, 3.212244750653343583 ) ) ;
#36355=EDGE_CURVE ( 'NONE', #10472, #14361, #2069, .T. ) ;
#36356=AXIS2_PLACEMENT_3D ( 'NONE', #24054, #15799, #19216 ) ;
#36357=ORIENTED_EDGE ( 'NONE', *, *, #11087, .F. ) ;
#36358=ORIENTED_EDGE ( 'NONE', *, *, #36647, .F. ) ;
#36359=EDGE_CURVE ( 'NONE', #7820, #13266, #24244, .T. ) ;
#36360=EDGE_CURVE ( 'NONE', #41032, #40408, #45513, .T. ) ;
#36361=FACE_OUTER_BOUND ( 'NONE', #20448, .T. ) ;
#36362=ORIENTED_EDGE ( 'NONE', *, *, #42059, .F. ) ;
#36363=CARTESIAN_POINT ( 'NONE',  ( -23.33693525117809386, 0.000000000000000000, 5.746789908705562944 ) ) ;
#36364=ORIENTED_EDGE ( 'NONE', *, *, #3677, .F. ) ;
#36365=FACE_OUTER_BOUND ( 'NONE', #16107, .T. ) ;
#36366=CARTESIAN_POINT ( 'NONE',  ( -10.22581229980790418, 0.000000000000000000, 4.740827489744188661 ) ) ;
#36367=ORIENTED_EDGE ( 'NONE', *, *, #8804, .T. ) ;
#36368=VECTOR ( 'NONE', #13669, 1000.000000000000114 ) ;
#36369=CARTESIAN_POINT ( 'NONE',  ( -13.95883414117900934, 0.000000000000000000, 6.758442655851721881 ) ) ;
#36370=ADVANCED_FACE ( 'NONE', ( #54891 ), #41812, .F. ) ;
#36371=VECTOR ( 'NONE', #6793, 1000.000000000000227 ) ;
#36372=LINE ( 'NONE', #1725, #49931 ) ;
#36373=ORIENTED_EDGE ( 'NONE', *, *, #15269, .F. ) ;
#36374=DIRECTION ( 'NONE',  ( -0.005002170337468016433, -0.7660444431189770143, 0.6427681459581293666 ) ) ;
#36375=FACE_OUTER_BOUND ( 'NONE', #51568, .T. ) ;
#36376=CARTESIAN_POINT ( 'NONE',  ( -15.82666044788779303, 3.686347215771511365, 2.711930348772070509 ) ) ;
#36377=EDGE_LOOP ( 'NONE', ( #27651, #33860, #56183, #15331 ) ) ;
#36378=DIRECTION ( 'NONE',  ( 0.5364919789714477361, 0.6444004775717706579, 0.5449076811759711036 ) ) ;
#36379=CARTESIAN_POINT ( 'NONE',  ( -12.56049299803446750, 0.000000000000000000, 6.199986743935199662 ) ) ;
#36380=PLANE ( 'NONE',  #42131 ) ;
#36381=CARTESIAN_POINT ( 'NONE',  ( -14.86511550681891691, 0.000000000000000000, 3.796733206253588122 ) ) ;
#36382=EDGE_CURVE ( 'NONE', #42498, #21366, #6632, .T. ) ;
#36383=CARTESIAN_POINT ( 'NONE',  ( -12.52505892662501097, 0.000000000000000000, 1.646784664228929218 ) ) ;
#36384=DIRECTION ( 'NONE',  ( -0.5449076811759708816, 0.6444004775717707689, 0.5364919789714475140 ) ) ;
#36386=EDGE_LOOP ( 'NONE', ( #50557, #14437, #15632, #53219 ) ) ;
#36387=PLANE ( 'NONE',  #22580 ) ;
#36388=EDGE_CURVE ( 'NONE', #22744, #2049, #19702, .T. ) ;
#36389=DIRECTION ( 'NONE',  ( -0.5364919789714478471, 0.6444004775717705469, -0.5449076811759709926 ) ) ;
#36391=ORIENTED_EDGE ( 'NONE', *, *, #43699, .T. ) ;
#36392=CARTESIAN_POINT ( 'NONE',  ( -18.39746900504187010, 0.000000000000000000, 14.03700784672088808 ) ) ;
#36393=LINE ( 'NONE', #49743, #3657 ) ;
#36394=VECTOR ( 'NONE', #7338, 999.9999999999998863 ) ;
#36395=VECTOR ( 'NONE', #16679, 1000.000000000000227 ) ;
#36396=EDGE_CURVE ( 'NONE', #55993, #37342, #37869, .T. ) ;
#36397=LINE ( 'NONE', #24191, #54867 ) ;
#36398=PLANE ( 'NONE',  #6955 ) ;
#36399=FACE_OUTER_BOUND ( 'NONE', #40963, .T. ) ;
#36400=VERTEX_POINT ( 'NONE', #15693 ) ;
#36401=ORIENTED_EDGE ( 'NONE', *, *, #32908, .T. ) ;
#36402=FACE_OUTER_BOUND ( 'NONE', #16044, .T. ) ;
#36403=DIRECTION ( 'NONE',  ( -0.9999697198139514409, -0.000000000000000000, -0.007781995580013368816 ) ) ;
#36404=ADVANCED_FACE ( 'NONE', ( #7460 ), #23947, .F. ) ;
#36405=LINE ( 'NONE', #15133, #40197 ) ;
#36406=ORIENTED_EDGE ( 'NONE', *, *, #33852, .T. ) ;
#36408=VERTEX_POINT ( 'NONE', #54061 ) ;
#36409=PLANE ( 'NONE',  #27431 ) ;
#36410=ADVANCED_FACE ( 'NONE', ( #15177 ), #24783, .F. ) ;
#36411=AXIS2_PLACEMENT_3D ( 'NONE', #11652, #36656, #11365 ) ;
#36412=VERTEX_POINT ( 'NONE', #11992 ) ;
#36413=CARTESIAN_POINT ( 'NONE',  ( -10.74029228357944987, 0.000000000000000000, 11.14194120806293320 ) ) ;
#36414=ADVANCED_FACE ( 'NONE', ( #37567 ), #45805, .F. ) ;
#36415=LINE ( 'NONE', #10612, #1461 ) ;
#36416=LINE ( 'NONE', #49496, #16690 ) ;
#36417=ORIENTED_EDGE ( 'NONE', *, *, #331, .T. ) ;
#36418=FACE_OUTER_BOUND ( 'NONE', #3221, .T. ) ;
#36419=EDGE_CURVE ( 'NONE', #41178, #4939, #16263, .T. ) ;
#36420=ORIENTED_EDGE ( 'NONE', *, *, #929, .F. ) ;
#36421=EDGE_CURVE ( 'NONE', #48670, #55547, #50350, .T. ) ;
#36422=EDGE_LOOP ( 'NONE', ( #46240, #40265, #47766, #18853 ) ) ;
#36423=ORIENTED_EDGE ( 'NONE', *, *, #51024, .T. ) ;
#36424=FACE_OUTER_BOUND ( 'NONE', #54682, .T. ) ;
#36425=ORIENTED_EDGE ( 'NONE', *, *, #33000, .F. ) ;
#36427=EDGE_LOOP ( 'NONE', ( #26065, #34410, #17497, #5982 ) ) ;
#36428=CARTESIAN_POINT ( 'NONE',  ( -1.299719944060198529, -6.815497196261854462, 3.723228940611872595 ) ) ;
#36429=FACE_OUTER_BOUND ( 'NONE', #41225, .T. ) ;
#36430=EDGE_CURVE ( 'NONE', #30223, #40790, #11462, .T. ) ;
#36431=VECTOR ( 'NONE', #24270, 999.9999999999998863 ) ;
#36432=AXIS2_PLACEMENT_3D ( 'NONE', #23656, #27951, #13549 ) ;
#36433=ORIENTED_EDGE ( 'NONE', *, *, #6366, .F. ) ;
#36434=DIRECTION ( 'NONE',  ( 0.6427681459581294776, -0.7660444431189769032, 0.005002170337467562802 ) ) ;
#36435=ORIENTED_EDGE ( 'NONE', *, *, #30342, .F. ) ;
#36436=EDGE_CURVE ( 'NONE', #42084, #50596, #2902, .T. ) ;
#36437=PLANE ( 'NONE',  #18327 ) ;
#36438=CARTESIAN_POINT ( 'NONE',  ( -12.23851102634202448, -0.1191753592594197858, 11.68427982808754884 ) ) ;
#36439=VECTOR ( 'NONE', #27666, 999.9999999999998863 ) ;
#36440=LINE ( 'NONE', #35609, #47706 ) ;
#36441=LINE ( 'NONE', #53753, #30244 ) ;
#36442=DIRECTION ( 'NONE',  ( 0.7660212471507180654, -0.6427876096865404731, 0.005961354470445141482 ) ) ;
#36443=DIRECTION ( 'NONE',  ( -0.005961354470445682716, -0.6427876096865404731, 0.7660212471507180654 ) ) ;
#36444=ORIENTED_EDGE ( 'NONE', *, *, #33280, .F. ) ;
#36446=CARTESIAN_POINT ( 'NONE',  ( -10.22293824630262193, 0.000000000000000000, 4.371517786486424306 ) ) ;
#36447=FACE_OUTER_BOUND ( 'NONE', #11961, .T. ) ;
#36448=AXIS2_PLACEMENT_3D ( 'NONE', #5036, #34851, #52165 ) ;
#36449=AXIS2_PLACEMENT_3D ( 'NONE', #47325, #42522, #9489 ) ;
#36450=DIRECTION ( 'NONE',  ( -0.9999697198139514409, -0.000000000000000000, -0.007781995580013368816 ) ) ;
#36451=CARTESIAN_POINT ( 'NONE',  ( 0.000000000000000000, -1.000000000000000000, 0.000000000000000000 ) ) ;
#36452=ORIENTED_EDGE ( 'NONE', *, *, #7197, .T. ) ;
#36453=DIRECTION ( 'NONE',  ( -0.6427681459581293666, -0.7660444431189770143, -0.005002170337467561935 ) ) ;
#36455=ORIENTED_EDGE ( 'NONE', *, *, #46821, .F. ) ;
#36456=CARTESIAN_POINT ( 'NONE',  ( -26.13415699229845757, -0.1191753592594197858, 6.933020519852192365 ) ) ;
#36457=FACE_OUTER_BOUND ( 'NONE', #2656, .T. ) ;
#36458=ORIENTED_EDGE ( 'NONE', *, *, #53716, .T. ) ;
#36460=PLANE ( 'NONE',  #26957 ) ;
#36461=EDGE_CURVE ( 'NONE', #5753, #20039, #25092, .T. ) ;
#36462=FACE_OUTER_BOUND ( 'NONE', #53009, .T. ) ;
#36463=CARTESIAN_POINT ( 'NONE',  ( -19.06540955380966551, 0.000000000000000000, 6.149363979183064544 ) ) ;
#36464=FACE_OUTER_BOUND ( 'NONE', #15747, .T. ) ;
#36465=ORIENTED_EDGE ( 'NONE', *, *, #34897, .T. ) ;
#36466=ORIENTED_EDGE ( 'NONE', *, *, #4188, .T. ) ;
#36467=DIRECTION ( 'NONE',  ( 0.000000000000000000, -0.000000000000000000, -1.000000000000000000 ) ) ;
#36468=CARTESIAN_POINT ( 'NONE',  ( -10.24018256733431897, 0.000000000000000000, 6.587376006033009546 ) ) ;
#36469=VECTOR ( 'NONE', #946, 1000.000000000000114 ) ;
#36470=DIRECTION ( 'NONE',  ( 0.007781995580012663651, 0.000000000000000000, -0.9999697198139515519 ) ) ;
#36471=EDGE_CURVE ( 'NONE', #6270, #49012, #38973, .T. ) ;
#36472=AXIS2_PLACEMENT_3D ( 'NONE', #35048, #9172, #30505 ) ;
#36473=AXIS2_PLACEMENT_3D ( 'NONE', #7977, #21002, #50819 ) ;
#36474=CARTESIAN_POINT ( 'NONE',  ( -14.60753831534046476, 0.000000000000000000, 4.706727884716099375 ) ) ;
#36475=LINE ( 'NONE', #41580, #24930 ) ;
#36477=EDGE_CURVE ( 'NONE', #55458, #8286, #8600, .T. ) ;
#36478=PLANE ( 'NONE',  #38324 ) ;
#36479=EDGE_CURVE ( 'NONE', #50963, #52679, #17376, .T. ) ;
#36480=CARTESIAN_POINT ( 'NONE',  ( -18.19747506107908563, 0.000000000000000000, 14.03856424583689311 ) ) ;
#36481=VECTOR ( 'NONE', #17270, 1000.000000000000114 ) ;
#36483=AXIS2_PLACEMENT_3D ( 'NONE', #6855, #50271, #20464 ) ;
#36484=VERTEX_POINT ( 'NONE', #3495 ) ;
#36487=CARTESIAN_POINT ( 'NONE',  ( -13.07066190154808361, 0.000000000000000000, 12.04713590736729678 ) ) ;
#36488=LINE ( 'NONE', #19447, #3956 ) ;
#36489=VERTEX_POINT ( 'NONE', #8304 ) ;
#36490=CARTESIAN_POINT ( 'NONE',  ( -17.88011496776504572, 0.000000000000000000, 7.266584425144382742 ) ) ;
#36491=ADVANCED_FACE ( 'NONE', ( #34430 ), #43258, .F. ) ;
#36492=VECTOR ( 'NONE', #36255, 1000.000000000000000 ) ;
#36493=ORIENTED_EDGE ( 'NONE', *, *, #33426, .T. ) ;
#36494=ADVANCED_FACE ( 'NONE', ( #55729 ), #12582, .F. ) ;
#36495=ORIENTED_EDGE ( 'NONE', *, *, #40950, .T. ) ;
#36496=ORIENTED_EDGE ( 'NONE', *, *, #17978, .T. ) ;
#36497=FACE_OUTER_BOUND ( 'NONE', #10398, .T. ) ;
#36498=ORIENTED_EDGE ( 'NONE', *, *, #53773, .F. ) ;
#36499=ORIENTED_EDGE ( 'NONE', *, *, #10270, .T. ) ;
#36500=DIRECTION ( 'NONE',  ( 0.9999697198139515519, 0.000000000000000000, 0.007781995580013368816 ) ) ;
#36501=FACE_OUTER_BOUND ( 'NONE', #34229, .T. ) ;
#36502=ORIENTED_EDGE ( 'NONE', *, *, #28126, .F. ) ;
#36504=ORIENTED_EDGE ( 'NONE', *, *, #25618, .F. ) ;
#36506=ORIENTED_EDGE ( 'NONE', *, *, #8064, .F. ) ;
#36507=VECTOR ( 'NONE', #31792, 1000.000000000000227 ) ;
#36508=ORIENTED_EDGE ( 'NONE', *, *, #9494, .F. ) ;
#36509=EDGE_CURVE ( 'NONE', #48860, #55206, #29899, .T. ) ;
#36510=DIRECTION ( 'NONE',  ( 0.6427681459581294776, -0.7660444431189769032, 0.005002170337467562802 ) ) ;
#36512=CARTESIAN_POINT ( 'NONE',  ( -16.49195238425235743, 0.000000000000000000, 8.016051566963941610 ) ) ;
#36513=LINE ( 'NONE', #14659, #52298 ) ;
#36514=VECTOR ( 'NONE', #37057, 1000.000000000000227 ) ;
#36515=EDGE_LOOP ( 'NONE', ( #11136, #16678, #13419, #1981 ) ) ;
#36516=LINE ( 'NONE', #23200, #30171 ) ;
#36517=ORIENTED_EDGE ( 'NONE', *, *, #47821, .T. ) ;
#36518=VECTOR ( 'NONE', #24055, 1000.000000000000227 ) ;
#36519=AXIS2_PLACEMENT_3D ( 'NONE', #12147, #41950, #29482 ) ;
#36520=LINE ( 'NONE', #35693, #45646 ) ;
#36521=CARTESIAN_POINT ( 'NONE',  ( -18.05255645404804454, -2.137015261443159009, 3.825365135988253673 ) ) ;
#36522=AXIS2_PLACEMENT_3D ( 'NONE', #18543, #1207, #31030 ) ;
#36523=VECTOR ( 'NONE', #49916, 1000.000000000000114 ) ;
#36524=DIRECTION ( 'NONE',  ( -0.9321478471874540261, 0.000000000000000000, 0.3620778797217457656 ) ) ;
#36525=CARTESIAN_POINT ( 'NONE',  ( -17.73140113748535285, 0.000000000000000000, 13.85752530597602039 ) ) ;
#36526=LINE ( 'NONE', #31724, #335 ) ;
#36527=DIRECTION ( 'NONE',  ( 0.6427681459581294776, -0.7660444431189769032, 0.005002170337467562802 ) ) ;
#36528=EDGE_LOOP ( 'NONE', ( #7633, #26050, #30308, #17349 ) ) ;
#36529=LINE ( 'NONE', #22915, #24703 ) ;
#36530=VERTEX_POINT ( 'NONE', #12849 ) ;
#36531=CARTESIAN_POINT ( 'NONE',  ( -22.57598249675604052, 4.981562823951511731, 13.82619267738939328 ) ) ;
#36532=LINE ( 'NONE', #18953, #41419 ) ;
#36533=PLANE ( 'NONE',  #41708 ) ;
#36534=VECTOR ( 'NONE', #52247, 1000.000000000000227 ) ;
#36535=ADVANCED_FACE ( 'NONE', ( #3757 ), #47488, .F. ) ;
#36536=CARTESIAN_POINT ( 'NONE',  ( -18.86354292863559579, 0.000000000000000000, 14.21804678658176080 ) ) ;
#36537=VECTOR ( 'NONE', #33914, 1000.000000000000114 ) ;
#36538=CARTESIAN_POINT ( 'NONE',  ( -13.27065584551087163, 0.000000000000000000, 12.04557950825129176 ) ) ;
#36539=ADVANCED_FACE ( 'NONE', ( #25931 ), #4355, .F. ) ;
#36540=ORIENTED_EDGE ( 'NONE', *, *, #31276, .F. ) ;
#36541=CARTESIAN_POINT ( 'NONE',  ( -9.959851692540329537, 0.000000000000000000, 4.573571243101220318 ) ) ;
#36542=DIRECTION ( 'NONE',  ( -0.5364919789714478471, 0.6444004775717705469, -0.5449076811759709926 ) ) ;
#36543=DIRECTION ( 'NONE',  ( 0.5364919789714477361, 0.6444004775717706579, 0.5449076811759711036 ) ) ;
#36544=EDGE_CURVE ( 'NONE', #2632, #10808, #13429, .T. ) ;
#36545=VECTOR ( 'NONE', #5316, 999.9999999999998863 ) ;
#36546=EDGE_CURVE ( 'NONE', #23289, #17566, #26201, .T. ) ;
#36547=EDGE_CURVE ( 'NONE', #27982, #7513, #25622, .T. ) ;
#36549=LINE ( 'NONE', #32575, #21239 ) ;
#36550=CIRCLE ( 'NONE', #45617, 2.125000000000000000 ) ;
#36551=CARTESIAN_POINT ( 'NONE',  ( -15.44908955062037492, -0.1191753592594185784, 6.277510045750531731 ) ) ;
#36552=CARTESIAN_POINT ( 'NONE',  ( -10.87607287308537174, 0.000000000000000000, 2.889106662571353290 ) ) ;
#36553=ADVANCED_FACE ( 'NONE', ( #55437 ), #16537, .F. ) ;
#36554=LINE ( 'NONE', #19512, #23309 ) ;
#36555=VECTOR ( 'NONE', #47447, 1000.000000000000227 ) ;
#36556=LINE ( 'NONE', #6461, #24671 ) ;
#36558=VECTOR ( 'NONE', #29178, 1000.000000000000114 ) ;
#36559=VECTOR ( 'NONE', #49390, 1000.000000000000227 ) ;
#36560=ORIENTED_EDGE ( 'NONE', *, *, #39578, .F. ) ;
#36561=EDGE_CURVE ( 'NONE', #41657, #21645, #29639, .T. ) ;
#36563=AXIS2_PLACEMENT_3D ( 'NONE', #20129, #37462, #33231 ) ;
#36564=ORIENTED_EDGE ( 'NONE', *, *, #55992, .T. ) ;
#36565=ORIENTED_EDGE ( 'NONE', *, *, #51811, .T. ) ;
#36567=ORIENTED_EDGE ( 'NONE', *, *, #35136, .F. ) ;
#36568=EDGE_CURVE ( 'NONE', #34678, #44201, #36131, .T. ) ;
#36569=VERTEX_POINT ( 'NONE', #53432 ) ;
#36570=DIRECTION ( 'NONE',  ( -0.8531650599175527594, 0.4028455766673922356, 0.3313982828793700652 ) ) ;
#36571=CARTESIAN_POINT ( 'NONE',  ( -23.33849165029409889, 0.000000000000000000, 5.946783852668351855 ) ) ;
#36572=EDGE_CURVE ( 'NONE', #31757, #10233, #53693, .T. ) ;
#36573=ORIENTED_EDGE ( 'NONE', *, *, #39111, .F. ) ;
#36574=ORIENTED_EDGE ( 'NONE', *, *, #40529, .F. ) ;
#36575=VECTOR ( 'NONE', #51404, 1000.000000000000114 ) ;
#36577=VECTOR ( 'NONE', #42230, 999.9999999999998863 ) ;
#36578=DIRECTION ( 'NONE',  ( 0.5449076811759707706, 0.6444004775717708799, -0.5364919789714476250 ) ) ;
#36579=FACE_OUTER_BOUND ( 'NONE', #7442, .T. ) ;
#36580=DIRECTION ( 'NONE',  ( 0.6427681459581294776, -0.7660444431189769032, 0.005002170337467562802 ) ) ;
#36581=ORIENTED_EDGE ( 'NONE', *, *, #7414, .T. ) ;
#36582=CARTESIAN_POINT ( 'NONE',  ( -21.47341775636118655, -0.1191753592594197858, 5.122631121243466090 ) ) ;
#36583=AXIS2_PLACEMENT_3D ( 'NONE', #54571, #38394, #47189 ) ;
#36584=FACE_OUTER_BOUND ( 'NONE', #6010, .T. ) ;
#36585=CARTESIAN_POINT ( 'NONE',  ( -17.26532721389163072, 0.000000000000000000, 13.67648636611514590 ) ) ;
#36586=VECTOR ( 'NONE', #4082, 1000.000000000000227 ) ;
#36587=CARTESIAN_POINT ( 'NONE',  ( -15.82444748994319283, 0.000000000000000000, 7.651914174590189965 ) ) ;
#36588=FACE_OUTER_BOUND ( 'NONE', #43748, .T. ) ;
#36589=LINE ( 'NONE', #37148, #51262 ) ;
#36590=CARTESIAN_POINT ( 'NONE',  ( -15.91372644746146037, -0.1191753592594204797, 6.273894133982523158 ) ) ;
#36591=DIRECTION ( 'NONE',  ( 0.5364919789714477361, 0.6444004775717706579, 0.5449076811759711036 ) ) ;
#36592=VECTOR ( 'NONE', #18060, 1000.000000000000114 ) ;
#36593=CARTESIAN_POINT ( 'NONE',  ( -10.94028622754223967, 0.000000000000000000, 11.14038480894692995 ) ) ;
#36594=VERTEX_POINT ( 'NONE', #44917 ) ;
#36595=DIRECTION ( 'NONE',  ( 0.5364919789714477361, 0.6444004775717706579, 0.5449076811759711036 ) ) ;
#36596=ORIENTED_EDGE ( 'NONE', *, *, #38548, .F. ) ;
#36597=ADVANCED_FACE ( 'NONE', ( #22762 ), #6032, .F. ) ;
#36598=VECTOR ( 'NONE', #22756, 999.9999999999998863 ) ;
#36600=DIRECTION ( 'NONE',  ( -0.5449076811759708816, 0.6444004775717707689, 0.5364919789714475140 ) ) ;
#36601=DIRECTION ( 'NONE',  ( -0.6427681459581293666, -0.7660444431189770143, -0.005002170337467561935 ) ) ;
#36602=PLANE ( 'NONE',  #21300 ) ;
#36603=DIRECTION ( 'NONE',  ( -0.005002170337468016433, -0.7660444431189770143, 0.6427681459581293666 ) ) ;
#36604=EDGE_CURVE ( 'NONE', #931, #19450, #40663, .T. ) ;
#36605=LINE ( 'NONE', #15851, #25046 ) ;
#36606=DIRECTION ( 'NONE',  ( 0.6427681459581294776, -0.7660444431189769032, 0.005002170337467562802 ) ) ;
#36607=CARTESIAN_POINT ( 'NONE',  ( -12.08591628628825276, 0.000000000000000000, 4.926357786634938840 ) ) ;
#36609=CARTESIAN_POINT ( 'NONE',  ( -23.33693525117809386, 0.000000000000000000, 5.746789908705562944 ) ) ;
#36610=ADVANCED_FACE ( 'NONE', ( #14276 ), #9142, .F. ) ;
#36611=VECTOR ( 'NONE', #6247, 999.9999999999998863 ) ;
#36613=DIRECTION ( 'NONE',  ( 0.005961354470445682716, -0.6427876096865404731, -0.7660212471507180654 ) ) ;
#36614=DIRECTION ( 'NONE',  ( 0.7660212471507180654, -0.6427876096865404731, 0.005961354470445141482 ) ) ;
#36615=CARTESIAN_POINT ( 'NONE',  ( -15.87975247367846166, 0.000000000000000000, 2.850166870931599927 ) ) ;
#36616=DIRECTION ( 'NONE',  ( -0.5449076811759708816, 0.6444004775717707689, 0.5364919789714475140 ) ) ;
#36617=EDGE_CURVE ( 'NONE', #17974, #15806, #44349, .T. ) ;
#36618=LINE ( 'NONE', #45149, #3281 ) ;
#36619=EDGE_CURVE ( 'NONE', #5931, #30283, #5448, .T. ) ;
#36620=EDGE_CURVE ( 'NONE', #38231, #52239, #5192, .T. ) ;
#36621=DIRECTION ( 'NONE',  ( 0.005961354470445682716, -0.6427876096865404731, -0.7660212471507180654 ) ) ;
#36622=CARTESIAN_POINT ( 'NONE',  ( -13.08408713167409942, -0.1191753592594197858, 1.863930203747758085 ) ) ;
#36623=EDGE_CURVE ( 'NONE', #48904, #23765, #9732, .T. ) ;
#36624=PLANE ( 'NONE',  #20467 ) ;
#36625=DIRECTION ( 'NONE',  ( -0.005002170337468016433, -0.7660444431189770143, 0.6427681459581293666 ) ) ;
#36626=ORIENTED_EDGE ( 'NONE', *, *, #12082, .T. ) ;
#36627=ORIENTED_EDGE ( 'NONE', *, *, #9358, .T. ) ;
#36628=AXIS2_PLACEMENT_3D ( 'NONE', #51534, #12625, #30788 ) ;
#36629=CARTESIAN_POINT ( 'NONE',  ( -17.74404816805336793, 0.000000000000000000, 3.574322630375089460 ) ) ;
#36630=CARTESIAN_POINT ( 'NONE',  ( -9.808144436391993182, 0.000000000000000000, 10.77986332834118777 ) ) ;
#36631=VECTOR ( 'NONE', #20376, 1000.000000000000227 ) ;
#36633=CARTESIAN_POINT ( 'NONE',  ( -14.90092180327158999, 0.000000000000000000, 8.397765404641738485 ) ) ;
#36635=ORIENTED_EDGE ( 'NONE', *, *, #53773, .T. ) ;
#36637=ADVANCED_FACE ( 'NONE', ( #35545 ), #26751, .F. ) ;
#36638=ORIENTED_EDGE ( 'NONE', *, *, #929, .T. ) ;
#36639=VERTEX_POINT ( 'NONE', #18501 ) ;
#36640=ORIENTED_EDGE ( 'NONE', *, *, #3670, .F. ) ;
#36641=EDGE_CURVE ( 'NONE', #12052, #50963, #52854, .T. ) ;
#36643=VECTOR ( 'NONE', #22257, 1000.000000000000227 ) ;
#36644=CARTESIAN_POINT ( 'NONE',  ( -18.85266870113162341, 1.743523803501506375, 3.949320956653499692 ) ) ;
#36645=LINE ( 'NONE', #19035, #38497 ) ;
#36646=VECTOR ( 'NONE', #53978, 1000.000000000000227 ) ;
#36647=EDGE_CURVE ( 'NONE', #21379, #47620, #31293, .T. ) ;
#36649=VERTEX_POINT ( 'NONE', #31588 ) ;
#36650=EDGE_LOOP ( 'NONE', ( #32633, #45378, #20730, #1605 ) ) ;
#36651=ADVANCED_FACE ( 'NONE', ( #10267 ), #36380, .F. ) ;
#36652=VECTOR ( 'NONE', #3581, 999.9999999999998863 ) ;
#36653=VECTOR ( 'NONE', #41005, 999.9999999999998863 ) ;
#36654=DIRECTION ( 'NONE',  ( 0.007781995580012663651, -3.146120232559066537E-19, -0.9999697198139514409 ) ) ;
#36655=VERTEX_POINT ( 'NONE', #4891 ) ;
#36656=DIRECTION ( 'NONE',  ( -0.005961354470445682716, -0.6427876096865404731, 0.7660212471507180654 ) ) ;
#36657=ORIENTED_EDGE ( 'NONE', *, *, #38680, .F. ) ;
#36658=PLANE ( 'NONE',  #21252 ) ;
#36659=CARTESIAN_POINT ( 'NONE',  ( -22.40634380310664397, 0.000000000000000000, 5.584705972946605534 ) ) ;
#36660=ORIENTED_EDGE ( 'NONE', *, *, #9383, .T. ) ;
#36661=LINE ( 'NONE', #40067, #34989 ) ;
#36662=DIRECTION ( 'NONE',  ( -0.005002170337468016433, -0.7660444431189770143, 0.6427681459581293666 ) ) ;
#36663=VECTOR ( 'NONE', #13108, 1000.000000000000000 ) ;
#36664=VERTEX_POINT ( 'NONE', #1470 ) ;
#36665=CARTESIAN_POINT ( 'NONE',  ( -14.94760462649100496, 0.000000000000000000, 2.488088991209854051 ) ) ;
#36666=CARTESIAN_POINT ( 'NONE',  ( -20.54204810873173415, 0.000000000000000000, 4.860550213503115558 ) ) ;
#36667=CARTESIAN_POINT ( 'NONE',  ( -17.40266420251354873, 0.000000000000000000, 5.623645764586359341 ) ) ;
#36669=AXIS2_PLACEMENT_3D ( 'NONE', #53312, #31720, #49022 ) ;
#36670=CARTESIAN_POINT ( 'NONE',  ( 2.072287782118878319, 0.000000000000000000, -2.950529333540147015 ) ) ;
#36671=PLANE ( 'NONE',  #35108 ) ;
#36672=DIRECTION ( 'NONE',  ( 0.3313982828793700097, 0.4028455766673915694, 0.8531650599175529814 ) ) ;
#36673=CARTESIAN_POINT ( 'NONE',  ( -15.88130887279446490, 0.000000000000000000, 3.050160814894388839 ) ) ;
#36674=LINE ( 'NONE', #2578, #1367 ) ;
#36675=LINE ( 'NONE', #6861, #20673 ) ;
#36676=CARTESIAN_POINT ( 'NONE',  ( -10.54003869734961718, 0.000000000000000000, 0.8757353956076227020 ) ) ;
#36677=VERTEX_POINT ( 'NONE', #22216 ) ;
#36678=CARTESIAN_POINT ( 'NONE',  ( -16.99924723426068951, 0.000000000000000000, 13.49389102713827171 ) ) ;
#36679=PLANE ( 'NONE',  #5935 ) ;
#36681=VERTEX_POINT ( 'NONE', #39550 ) ;
#36682=VECTOR ( 'NONE', #55087, 999.9999999999998863 ) ;
#36683=CARTESIAN_POINT ( 'NONE',  ( -16.23369548331420020, 0.2864062442990022439, 3.657081181831572714 ) ) ;
#36684=PLANE ( 'NONE',  #27256 ) ;
#36685=VECTOR ( 'NONE', #37569, 1000.000000000000227 ) ;
#36686=ADVANCED_FACE ( 'NONE', ( #11090 ), #6858, .F. ) ;
#36687=DIRECTION ( 'NONE',  ( -0.9999697198139514409, -0.000000000000000000, -0.007781995580013368816 ) ) ;
#36688=EDGE_CURVE ( 'NONE', #35922, #52348, #33263, .T. ) ;
#36689=EDGE_CURVE ( 'NONE', #31243, #6083, #19896, .T. ) ;
#36690=DIRECTION ( 'NONE',  ( -0.8531650599175527594, 0.4028455766673922356, 0.3313982828793700652 ) ) ;
#36692=VERTEX_POINT ( 'NONE', #32673 ) ;
#36693=AXIS2_PLACEMENT_3D ( 'NONE', #52356, #47818, #39582 ) ;
#36694=VECTOR ( 'NONE', #3932, 999.9999999999998863 ) ;
#36695=ORIENTED_EDGE ( 'NONE', *, *, #50355, .T. ) ;
#36696=DIRECTION ( 'NONE',  ( 0.007781995580012663651, 0.000000000000000000, -0.9999697198139515519 ) ) ;
#36697=DIRECTION ( 'NONE',  ( -0.5449076811759708816, 0.6444004775717707689, 0.5364919789714475140 ) ) ;
#36698=ORIENTED_EDGE ( 'NONE', *, *, #24814, .T. ) ;
#36699=DIRECTION ( 'NONE',  ( 0.005961354470445682716, -0.6427876096865404731, -0.7660212471507180654 ) ) ;
#36700=ORIENTED_EDGE ( 'NONE', *, *, #34523, .F. ) ;
#36702=AXIS2_PLACEMENT_3D ( 'NONE', #5903, #31737, #10974 ) ;
#36703=ORIENTED_EDGE ( 'NONE', *, *, #49463, .F. ) ;
#36704=ORIENTED_EDGE ( 'NONE', *, *, #53589, .T. ) ;
#36705=AXIS2_PLACEMENT_3D ( 'NONE', #4037, #3476, #47470 ) ;
#36706=LINE ( 'NONE', #22799, #28364 ) ;
#36707=FACE_OUTER_BOUND ( 'NONE', #39962, .T. ) ;
#36708=VECTOR ( 'NONE', #10577, 1000.000000000000227 ) ;
#36709=LINE ( 'NONE', #2335, #8506 ) ;
#36710=ORIENTED_EDGE ( 'NONE', *, *, #32286, .T. ) ;
#36711=CARTESIAN_POINT ( 'NONE',  ( -13.96015179556829011, 0.000000000000000000, 6.927758415146698212 ) ) ;
#36712=VERTEX_POINT ( 'NONE', #36964 ) ;
#36713=EDGE_CURVE ( 'NONE', #28808, #485, #11667, .T. ) ;
#36715=ORIENTED_EDGE ( 'NONE', *, *, #52340, .T. ) ;
#36716=VECTOR ( 'NONE', #18856, 1000.000000000000114 ) ;
#36717=CARTESIAN_POINT ( 'NONE',  ( -12.57354561117159797, 0.000000000000000000, 7.877219500929045992 ) ) ;
#36718=VECTOR ( 'NONE', #24181, 1000.000000000000114 ) ;
#36719=EDGE_CURVE ( 'NONE', #30987, #26051, #15619, .T. ) ;
#36720=ORIENTED_EDGE ( 'NONE', *, *, #12194, .F. ) ;
#36721=VECTOR ( 'NONE', #30449, 999.9999999999998863 ) ;
#36722=FACE_OUTER_BOUND ( 'NONE', #47832, .T. ) ;
#36723=ADVANCED_FACE ( 'NONE', ( #10828 ), #37212, .F. ) ;
#36724=ORIENTED_EDGE ( 'NONE', *, *, #46594, .T. ) ;
#36727=VECTOR ( 'NONE', #4545, 999.9999999999998863 ) ;
#36728=VERTEX_POINT ( 'NONE', #41493 ) ;
#36729=EDGE_CURVE ( 'NONE', #3193, #1369, #19335, .T. ) ;
#36730=PLANE ( 'NONE',  #521 ) ;
#36731=ORIENTED_EDGE ( 'NONE', *, *, #26730, .F. ) ;
#36733=CARTESIAN_POINT ( 'NONE',  ( -19.60834386242827776, 0.000000000000000000, 4.298478389818581213 ) ) ;
#36734=VECTOR ( 'NONE', #21728, 1000.000000000000000 ) ;
#36735=FACE_OUTER_BOUND ( 'NONE', #5716, .T. ) ;
#36736=PLANE ( 'NONE',  #14160 ) ;
#36737=DIRECTION ( 'NONE',  ( 0.005961354470445682716, -0.6427876096865404731, -0.7660212471507180654 ) ) ;
#36738=DIRECTION ( 'NONE',  ( -0.7660212471507179544, -0.6427876096865405842, -0.005961354470445141482 ) ) ;
#36739=DIRECTION ( 'NONE',  ( -0.9999697198139514409, -0.000000000000000000, -0.007781995580013368816 ) ) ;
#36741=ORIENTED_EDGE ( 'NONE', *, *, #33957, .F. ) ;
#36743=DIRECTION ( 'NONE',  ( 0.6427681459581294776, -0.7660444431189769032, 0.005002170337467562802 ) ) ;
#36744=CARTESIAN_POINT ( 'NONE',  ( -22.52493451062505869, 5.467268677019012202, 14.60348995783060211 ) ) ;
#36746=DIRECTION ( 'NONE',  ( 0.6427681459581294776, -0.7660444431189769032, 0.005002170337467562802 ) ) ;
#36747=VECTOR ( 'NONE', #40813, 1000.000000000000227 ) ;
#36748=LINE ( 'NONE', #1550, #429 ) ;
#36749=ORIENTED_EDGE ( 'NONE', *, *, #36904, .T. ) ;
#36750=VECTOR ( 'NONE', #31972, 999.9999999999998863 ) ;
#36752=DIRECTION ( 'NONE',  ( 0.9999697198139515519, 0.000000000000000000, 0.007781995580013368816 ) ) ;
#36753=EDGE_LOOP ( 'NONE', ( #13417, #10532, #10076, #24369 ) ) ;
#36754=FACE_OUTER_BOUND ( 'NONE', #4383, .T. ) ;
#36755=EDGE_CURVE ( 'NONE', #6150, #8005, #28720, .T. ) ;
#36756=FACE_OUTER_BOUND ( 'NONE', #34235, .T. ) ;
#36757=VECTOR ( 'NONE', #53914, 1000.000000000000227 ) ;
#36758=VERTEX_POINT ( 'NONE', #41204 ) ;
#36759=ADVANCED_FACE ( 'NONE', ( #28137 ), #19634, .F. ) ;
#36760=LINE ( 'NONE', #24798, #37052 ) ;
#36762=VECTOR ( 'NONE', #53622, 1000.000000000000227 ) ;
#36763=DIRECTION ( 'NONE',  ( -0.005961354470445682716, -0.6427876096865404731, 0.7660212471507180654 ) ) ;
#36764=EDGE_CURVE ( 'NONE', #5849, #17764, #45729, .T. ) ;
#36765=DIRECTION ( 'NONE',  ( 0.9999697198139515519, 0.000000000000000000, 0.007781995580013368816 ) ) ;
#36766=CARTESIAN_POINT ( 'NONE',  ( -13.58223596932098154, 4.819660872929010687, 10.06700741326545234 ) ) ;
#36767=ORIENTED_EDGE ( 'NONE', *, *, #47587, .T. ) ;
#36768=VECTOR ( 'NONE', #42935, 1000.000000000000114 ) ;
#36770=VERTEX_POINT ( 'NONE', #45196 ) ;
#36771=VECTOR ( 'NONE', #2014, 1000.000000000000227 ) ;
#36772=CARTESIAN_POINT ( 'NONE',  ( -18.49718515159138477, -1.003701604285657911, 4.034232660979946594 ) ) ;
#36773=CARTESIAN_POINT ( 'NONE',  ( 2.072287782118878319, 0.000000000000000000, -2.950529333540147015 ) ) ;
#36774=FACE_OUTER_BOUND ( 'NONE', #29440, .T. ) ;
#36776=VECTOR ( 'NONE', #46856, 1000.000000000000114 ) ;
#36777=DIRECTION ( 'NONE',  ( -0.005002170337468016433, -0.7660444431189770143, 0.6427681459581293666 ) ) ;
#36778=FACE_OUTER_BOUND ( 'NONE', #35856, .T. ) ;
#36779=ORIENTED_EDGE ( 'NONE', *, *, #48482, .F. ) ;
#36780=DIRECTION ( 'NONE',  ( 0.7660212471507180654, -0.6427876096865404731, 0.005961354470445141482 ) ) ;
#36781=EDGE_CURVE ( 'NONE', #33095, #22624, #32961, .T. ) ;
#36782=VECTOR ( 'NONE', #51979, 1000.000000000000227 ) ;
#36783=DIRECTION ( 'NONE',  ( -0.6427681459581293666, -0.7660444431189770143, -0.005002170337467561935 ) ) ;
#36784=VECTOR ( 'NONE', #6937, 1000.000000000000114 ) ;
#36785=CARTESIAN_POINT ( 'NONE',  ( -16.49925689037891985, 0.000000000000000000, 8.954664917442258343 ) ) ;
#36786=ORIENTED_EDGE ( 'NONE', *, *, #38472, .T. ) ;
#36787=CARTESIAN_POINT ( 'NONE',  ( -11.15221203998479460, 0.000000000000000000, 4.364285962950406272 ) ) ;
#36788=ORIENTED_EDGE ( 'NONE', *, *, #3852, .F. ) ;
#36789=DIRECTION ( 'NONE',  ( 0.6427681459581294776, -0.7660444431189769032, 0.005002170337467562802 ) ) ;
#36790=DIRECTION ( 'NONE',  ( 0.000000000000000000, -0.000000000000000000, -1.000000000000000000 ) ) ;
#36791=ORIENTED_EDGE ( 'NONE', *, *, #35450, .F. ) ;
#36792=DIRECTION ( 'NONE',  ( -0.5364919789714478471, 0.6444004775717705469, -0.5449076811759709926 ) ) ;
#36793=ORIENTED_EDGE ( 'NONE', *, *, #27797, .T. ) ;
#36796=ORIENTED_EDGE ( 'NONE', *, *, #24478, .T. ) ;
#36797=CARTESIAN_POINT ( 'NONE',  ( -14.07714710935361779, 2.714935509636509536, 2.063353073686676531 ) ) ;
#36798=ORIENTED_EDGE ( 'NONE', *, *, #19807, .T. ) ;
#36799=AXIS2_PLACEMENT_3D ( 'NONE', #25147, #20856, #38175 ) ;
#36800=ORIENTED_EDGE ( 'NONE', *, *, #14782, .F. ) ;
#36801=CARTESIAN_POINT ( 'NONE',  ( -20.51915365390780011, -2.298917212465658721, 4.778309734519891272 ) ) ;
#36802=VECTOR ( 'NONE', #41823, 1000.000000000000227 ) ;
#36803=ORIENTED_EDGE ( 'NONE', *, *, #1808, .T. ) ;
#36804=EDGE_LOOP ( 'NONE', ( #46540, #46382, #28248, #27798 ) ) ;
#36806=EDGE_CURVE ( 'NONE', #54647, #13476, #2831, .T. ) ;
#36807=EDGE_LOOP ( 'NONE', ( #1834, #50348, #31651, #6144 ) ) ;
#36808=VECTOR ( 'NONE', #33264, 1000.000000000000227 ) ;
#36809=VERTEX_POINT ( 'NONE', #6297 ) ;
#36810=ORIENTED_EDGE ( 'NONE', *, *, #41490, .F. ) ;
#36811=VECTOR ( 'NONE', #42460, 1000.000000000000227 ) ;
#36812=VECTOR ( 'NONE', #41592, 1000.000000000000227 ) ;
#36813=DIRECTION ( 'NONE',  ( 0.007781995580012663651, 0.000000000000000000, -0.9999697198139515519 ) ) ;
#36814=DIRECTION ( 'NONE',  ( 0.007781995580012662783, 0.000000000000000000, -0.9999697198139514409 ) ) ;
#36816=CARTESIAN_POINT ( 'NONE',  ( -19.60834386242827776, 0.000000000000000000, 4.298478389818581213 ) ) ;
#36817=ORIENTED_EDGE ( 'NONE', *, *, #17574, .T. ) ;
#36819=ORIENTED_EDGE ( 'NONE', *, *, #11928, .F. ) ;
#36820=VECTOR ( 'NONE', #20255, 1000.000000000000227 ) ;
#36821=EDGE_CURVE ( 'NONE', #11634, #25655, #11385, .T. ) ;
#36822=ORIENTED_EDGE ( 'NONE', *, *, #52496, .F. ) ;
#36823=VECTOR ( 'NONE', #53070, 1000.000000000000227 ) ;
#36824=AXIS2_PLACEMENT_3D ( 'NONE', #12477, #17010, #25801 ) ;
#36825=PLANE ( 'NONE',  #54724 ) ;
#36826=EDGE_CURVE ( 'NONE', #40568, #27421, #54814, .T. ) ;
#36827=ADVANCED_FACE ( 'NONE', ( #50273 ), #7135, .F. ) ;
#36828=AXIS2_PLACEMENT_3D ( 'NONE', #41323, #49572, #53804 ) ;
#36829=DIRECTION ( 'NONE',  ( 0.005961354470445682716, -0.6427876096865404731, -0.7660212471507180654 ) ) ;
#36830=AXIS2_PLACEMENT_3D ( 'NONE', #27184, #44491, #40244 ) ;
#36831=CARTESIAN_POINT ( 'NONE',  ( -16.81345671998191449, 0.000000000000000000, 3.412238694616132495 ) ) ;
#36832=LINE ( 'NONE', #19193, #39349 ) ;
#36833=CARTESIAN_POINT ( 'NONE',  ( -20.52784467904771759, 0.000000000000000000, 14.94375894514125491 ) ) ;
#36834=ORIENTED_EDGE ( 'NONE', *, *, #53268, .T. ) ;
#36835=LINE ( 'NONE', #46159, #47412 ) ;
#36836=EDGE_CURVE ( 'NONE', #2309, #17653, #40916, .T. ) ;
#36837=VERTEX_POINT ( 'NONE', #29838 ) ;
#36838=CARTESIAN_POINT ( 'NONE',  ( -14.94916102560700821, 0.000000000000000000, 2.688082935172642962 ) ) ;
#36839=CARTESIAN_POINT ( 'NONE',  ( -24.26908309836554878, 0.000000000000000000, 6.108867788427308376 ) ) ;
#36840=ADVANCED_FACE ( 'NONE', ( #3690 ), #46568, .F. ) ;
#36841=FACE_OUTER_BOUND ( 'NONE', #21265, .T. ) ;
#36842=CARTESIAN_POINT ( 'NONE',  ( -12.47550013608699260, 3.524445264749008988, 7.511444159126568820 ) ) ;
#36843=EDGE_CURVE ( 'NONE', #54306, #1702, #46876, .T. ) ;
#36844=LINE ( 'NONE', #23493, #14170 ) ;
#36845=AXIS2_PLACEMENT_3D ( 'NONE', #42690, #7493, #29363 ) ;
#36846=EDGE_LOOP ( 'NONE', ( #32033, #47439, #238, #42456 ) ) ;
#36848=DIRECTION ( 'NONE',  ( -0.005961354470445682716, -0.6427876096865404731, 0.7660212471507180654 ) ) ;
#36849=FACE_OUTER_BOUND ( 'NONE', #15112, .T. ) ;
#36850=VECTOR ( 'NONE', #22574, 1000.000000000000227 ) ;
#36851=EDGE_CURVE ( 'NONE', #45499, #17332, #47135, .T. ) ;
#36852=CARTESIAN_POINT ( 'NONE',  ( -10.32946152485258295, -0.1191753592594181482, 5.209355965425340962 ) ) ;
#36853=AXIS2_PLACEMENT_3D ( 'NONE', #44295, #22703, #48243 ) ;
#36854=DIRECTION ( 'NONE',  ( -0.9321478471874540261, 0.000000000000000000, 0.3620778797217457656 ) ) ;
#36855=LINE ( 'NONE', #15262, #46394 ) ;
#36856=CARTESIAN_POINT ( 'NONE',  ( -1.086233639165236964, -1.000000000000000000, -2.796443541562362078 ) ) ;
#36857=EDGE_CURVE ( 'NONE', #37024, #41757, #29563, .T. ) ;
#36858=VECTOR ( 'NONE', #4821, 1000.000000000000227 ) ;
#36859=VECTOR ( 'NONE', #56021, 1000.000000000000227 ) ;
#36860=CARTESIAN_POINT ( 'NONE',  ( -16.35723548322975418, 2.067327705546507133, 6.627863836689923183 ) ) ;
#36861=DIRECTION ( 'NONE',  ( -0.5449076811759708816, 0.6444004775717707689, 0.5364919789714475140 ) ) ;
#36862=VECTOR ( 'NONE', #7089, 999.9999999999998863 ) ;
#36863=ORIENTED_EDGE ( 'NONE', *, *, #45821, .T. ) ;
#36864=VECTOR ( 'NONE', #51545, 1000.000000000000227 ) ;
#36865=AXIS2_PLACEMENT_3D ( 'NONE', #17718, #35058, #928 ) ;
#36866=ORIENTED_EDGE ( 'NONE', *, *, #9267, .T. ) ;
#36868=ORIENTED_EDGE ( 'NONE', *, *, #15639, .T. ) ;
#36869=ORIENTED_EDGE ( 'NONE', *, *, #38088, .T. ) ;
#36870=VERTEX_POINT ( 'NONE', #25293 ) ;
#36871=LINE ( 'NONE', #15274, #43232 ) ;
#36872=FACE_OUTER_BOUND ( 'NONE', #35386, .T. ) ;
#36873=VERTEX_POINT ( 'NONE', #55960 ) ;
#36874=DIRECTION ( 'NONE',  ( 0.9999697198139515519, 0.000000000000000000, 0.007781995580013368816 ) ) ;
#36875=ADVANCED_FACE ( 'NONE', ( #12519 ), #8237, .F. ) ;
#36876=ORIENTED_EDGE ( 'NONE', *, *, #48716, .F. ) ;
#36877=VERTEX_POINT ( 'NONE', #50827 ) ;
#36878=VECTOR ( 'NONE', #21302, 999.9999999999998863 ) ;
#36880=CARTESIAN_POINT ( 'NONE',  ( -22.40634380310664397, 0.000000000000000000, 5.584705972946605534 ) ) ;
#36881=CARTESIAN_POINT ( 'NONE',  ( -15.56710904319146671, 0.000000000000000000, 8.592587037720512910 ) ) ;
#36882=ORIENTED_EDGE ( 'NONE', *, *, #34753, .T. ) ;
#36883=VECTOR ( 'NONE', #650, 1000.000000000000114 ) ;
#36885=EDGE_CURVE ( 'NONE', #2328, #18331, #34370, .T. ) ;
#36886=CARTESIAN_POINT ( 'NONE',  ( -25.20200914511100265, -0.1191753592594197858, 6.570942640130446932 ) ) ;
#36887=VECTOR ( 'NONE', #29137, 1000.000000000000227 ) ;
#36888=CARTESIAN_POINT ( 'NONE',  ( -11.87243407472968926, 0.000000000000000000, 11.50246268866867361 ) ) ;
#36889=ADVANCED_FACE ( 'NONE', ( #34629 ), #12779, .F. ) ;
#36890=CARTESIAN_POINT ( 'NONE',  ( 1.086233639165236964, 0.000000000000000000, 2.796443541562362078 ) ) ;
#36891=CARTESIAN_POINT ( 'NONE',  ( -12.15271748404464880, 0.000000000000000000, 1.601849296007406664 ) ) ;
#36892=VECTOR ( 'NONE', #26330, 1000.000000000000227 ) ;
#36893=DIRECTION ( 'NONE',  ( 0.9999697198139515519, 0.000000000000000000, 0.007781995580013368816 ) ) ;
#36894=CARTESIAN_POINT ( 'NONE',  ( -17.41128636302939725, 0.000000000000000000, 6.731574874359651517 ) ) ;
#36895=CARTESIAN_POINT ( 'NONE',  ( 2.072287782118878319, 0.000000000000000000, -2.950529333540147015 ) ) ;
#36896=DIRECTION ( 'NONE',  ( 0.7660212471507180654, -0.6427876096865404731, 0.005961354470445141482 ) ) ;
#36897=EDGE_LOOP ( 'NONE', ( #36067, #28716, #9698, #601 ) ) ;
#36899=VERTEX_POINT ( 'NONE', #11923 ) ;
#36900=AXIS2_PLACEMENT_3D ( 'NONE', #4744, #22068, #29474 ) ;
#36901=DIRECTION ( 'NONE',  ( -0.9999697198139514409, -0.000000000000000000, -0.007781995580013368816 ) ) ;
#36902=CARTESIAN_POINT ( 'NONE',  ( -11.67244013076689946, 0.000000000000000000, 11.50401908778467863 ) ) ;
#36903=PLANE ( 'NONE',  #51257 ) ;
#36904=EDGE_CURVE ( 'NONE', #54774, #1287, #34101, .T. ) ;
#36905=PLANE ( 'NONE',  #33200 ) ;
#36906=CARTESIAN_POINT ( 'NONE',  ( -20.54479086174542957, 3.200641362704010007, 4.560108989559846115 ) ) ;
#36907=FACE_OUTER_BOUND ( 'NONE', #6172, .T. ) ;
#36908=VECTOR ( 'NONE', #25523, 999.9999999999998863 ) ;
#36909=ADVANCED_FACE ( 'NONE', ( #25014 ), #3980, .F. ) ;
#36910=AXIS2_PLACEMENT_3D ( 'NONE', #22160, #589, #52273 ) ;
#36911=LINE ( 'NONE', #19008, #1990 ) ;
#36912=CARTESIAN_POINT ( 'NONE',  ( -12.80458192191714595, 0.000000000000000000, 11.86454056839041726 ) ) ;
#36913=CARTESIAN_POINT ( 'NONE',  ( 2.072287782118878319, 0.000000000000000000, -2.950529333540147015 ) ) ;
#36914=DIRECTION ( 'NONE',  ( 0.005961354470445682716, -0.6427876096865404731, -0.7660212471507180654 ) ) ;
#36915=FACE_OUTER_BOUND ( 'NONE', #30720, .T. ) ;
#36916=CARTESIAN_POINT ( 'NONE',  ( -9.136524801126023831, 0.000000000000000000, 3.471982353925851861 ) ) ;
#36917=EDGE_CURVE ( 'NONE', #22139, #38141, #29252, .T. ) ;
#36918=LINE ( 'NONE', #19016, #51789 ) ;
#36919=FACE_OUTER_BOUND ( 'NONE', #13914, .T. ) ;
#36920=CARTESIAN_POINT ( 'NONE',  ( 2.072287782118878319, 0.000000000000000000, -2.950529333540147015 ) ) ;
#36921=LINE ( 'NONE', #10522, #27470 ) ;
#36922=AXIS2_PLACEMENT_3D ( 'NONE', #9974, #13946, #23036 ) ;
#36923=ORIENTED_EDGE ( 'NONE', *, *, #41430, .F. ) ;
#36924=DIRECTION ( 'NONE',  ( 0.6427681459581294776, -0.7660444431189769032, 0.005002170337467562802 ) ) ;
#36926=CARTESIAN_POINT ( 'NONE',  ( -8.830583954895368848, 0.000000000000000000, 4.582359465753242489 ) ) ;
#36927=CARTESIAN_POINT ( 'NONE',  ( -19.32961685222932147, 0.000000000000000000, 14.39908572644263351 ) ) ;
#36928=EDGE_LOOP ( 'NONE', ( #52984, #42765, #26357, #45583 ) ) ;
#36929=CARTESIAN_POINT ( 'NONE',  ( -20.54204810873173415, 0.000000000000000000, 4.860550213503115558 ) ) ;
#36930=VECTOR ( 'NONE', #47885, 1000.000000000000114 ) ;
#36931=EDGE_LOOP ( 'NONE', ( #28262, #10887, #35591, #4034 ) ) ;
#36932=CARTESIAN_POINT ( 'NONE',  ( -13.92048961155144937, -3.270328918600660995, 7.456289541356968975 ) ) ;
#36933=VECTOR ( 'NONE', #21739, 1000.000000000000114 ) ;
#36934=VERTEX_POINT ( 'NONE', #38637 ) ;
#36935=ORIENTED_EDGE ( 'NONE', *, *, #36145, .F. ) ;
#36936=ORIENTED_EDGE ( 'NONE', *, *, #12533, .F. ) ;
#36937=DIRECTION ( 'NONE',  ( 0.9999697198139515519, 0.000000000000000000, 0.007781995580013368816 ) ) ;
#36938=DIRECTION ( 'NONE',  ( -0.5364919789714478471, 0.6444004775717705469, -0.5449076811759709926 ) ) ;
#36939=CARTESIAN_POINT ( 'NONE',  ( -18.67697421479882181, -0.1191753592594197858, 4.036397482078229793 ) ) ;
#36940=EDGE_CURVE ( 'NONE', #35444, #8247, #43445, .T. ) ;
#36941=AXIS2_PLACEMENT_3D ( 'NONE', #5262, #41280, #6635 ) ;
#36942=ORIENTED_EDGE ( 'NONE', *, *, #41198, .F. ) ;
#36943=EDGE_CURVE ( 'NONE', #39017, #9012, #21851, .T. ) ;
#36944=ORIENTED_EDGE ( 'NONE', *, *, #28803, .F. ) ;
#36945=DIRECTION ( 'NONE',  ( 0.005002170337468016433, -0.7660444431189770143, -0.6427681459581293666 ) ) ;
#36946=ORIENTED_EDGE ( 'NONE', *, *, #12276, .T. ) ;
#36947=EDGE_CURVE ( 'NONE', #27291, #15255, #17054, .T. ) ;
#36948=DIRECTION ( 'NONE',  ( 0.6427681459581294776, -0.7660444431189769032, 0.005002170337467562802 ) ) ;
#36949=EDGE_LOOP ( 'NONE', ( #3396, #8099, #20587, #28543 ) ) ;
#36951=CARTESIAN_POINT ( 'NONE',  ( -18.76354595665420177, -0.1191753592594177458, 14.21882498613976331 ) ) ;
#36952=EDGE_CURVE ( 'NONE', #16268, #43785, #51114, .T. ) ;
#36954=EDGE_CURVE ( 'NONE', #30608, #48670, #8831, .T. ) ;
#36955=VERTEX_POINT ( 'NONE', #49091 ) ;
#36956=DIRECTION ( 'NONE',  ( 0.5449076811759707706, 0.6444004775717708799, -0.5364919789714476250 ) ) ;
#36957=CARTESIAN_POINT ( 'NONE',  ( -17.31051119149000428, -0.1191753592594168992, 6.632356101936254689 ) ) ;
#36958=ORIENTED_EDGE ( 'NONE', *, *, #36191, .T. ) ;
#36959=CARTESIAN_POINT ( 'NONE',  ( -14.46888367232926420, 0.000000000000000000, 12.59025272694991315 ) ) ;
#36960=FACE_OUTER_BOUND ( 'NONE', #43388, .T. ) ;
#36961=ORIENTED_EDGE ( 'NONE', *, *, #47027, .T. ) ;
#36962=FACE_OUTER_BOUND ( 'NONE', #15246, .T. ) ;
#36963=DIRECTION ( 'NONE',  ( 0.007781995580012663651, 0.000000000000000000, -0.9999697198139515519 ) ) ;
#36964=CARTESIAN_POINT ( 'NONE',  ( -9.712109199288757821, 0.000000000000000000, 1.990174743821643055 ) ) ;
#36965=EDGE_CURVE ( 'NONE', #29764, #42740, #44293, .T. ) ;
#36966=FACE_OUTER_BOUND ( 'NONE', #39918, .T. ) ;
#36967=FACE_OUTER_BOUND ( 'NONE', #27496, .T. ) ;
#36968=CARTESIAN_POINT ( 'NONE',  ( -17.87304920636520222, 0.000000000000000000, 6.358649259333880366 ) ) ;
#36969=ADVANCED_FACE ( 'NONE', ( #52785 ), #1098, .F. ) ;
#36970=VECTOR ( 'NONE', #14905, 1000.000000000000227 ) ;
#36972=ORIENTED_EDGE ( 'NONE', *, *, #53482, .F. ) ;
#36973=CARTESIAN_POINT ( 'NONE',  ( -16.21461322262780058, -2.137015261443158565, 6.487444273011554685 ) ) ;
#36976=EDGE_LOOP ( 'NONE', ( #30142, #50505, #50316, #3412 ) ) ;
#36977=DIRECTION ( 'NONE',  ( 0.000000000000000000, -0.000000000000000000, -1.000000000000000000 ) ) ;
#36978=DIRECTION ( 'NONE',  ( -0.5364919789714478471, 0.6444004775717705469, -0.5449076811759709926 ) ) ;
#36979=EDGE_CURVE ( 'NONE', #51394, #42909, #47983, .T. ) ;
#36980=AXIS2_PLACEMENT_3D ( 'NONE', #42661, #12852, #29643 ) ;
#36981=CARTESIAN_POINT ( 'NONE',  ( -24.26986129792355129, -0.1191753592594197858, 6.208864760408702388 ) ) ;
#36982=CARTESIAN_POINT ( 'NONE',  ( -10.44305056480239102, 0.000000000000000000, 6.955129310174771540 ) ) ;
#36983=EDGE_CURVE ( 'NONE', #9162, #42368, #27236, .T. ) ;
#36984=CARTESIAN_POINT ( 'NONE',  ( 0.000000000000000000, -1.000000000000000000, 0.000000000000000000 ) ) ;
#36985=EDGE_LOOP ( 'NONE', ( #14222, #18219, #33567 ) ) ;
#36986=VERTEX_POINT ( 'NONE', #30683 ) ;
#36987=LINE ( 'NONE', #15379, #51297 ) ;
#36988=LINE ( 'NONE', #37823, #11161 ) ;
#36989=EDGE_LOOP ( 'NONE', ( #9257, #17221, #13049, #31357 ) ) ;
#36990=CARTESIAN_POINT ( 'NONE',  ( -17.80242246511569348, -0.1191753592594190225, 10.13343903392645373 ) ) ;
#36991=EDGE_LOOP ( 'NONE', ( #16244, #36417, #25895, #49348, #8557 ) ) ;
#36992=CARTESIAN_POINT ( 'NONE',  ( -11.87243407472968926, 0.000000000000000000, 11.50246268866867361 ) ) ;
#36993=EDGE_LOOP ( 'NONE', ( #46523, #44085, #30812, #36504 ) ) ;
#36994=VERTEX_POINT ( 'NONE', #53092 ) ;
#36995=DIRECTION ( 'NONE',  ( 0.007781995580012663651, -3.146120232559066537E-19, -0.9999697198139514409 ) ) ;
#36996=DIRECTION ( 'NONE',  ( 0.007781995580012662783, 0.000000000000000000, -0.9999697198139514409 ) ) ;
#36997=DIRECTION ( 'NONE',  ( 0.9999697198139515519, 0.000000000000000000, 0.007781995580013368816 ) ) ;
#36999=FACE_OUTER_BOUND ( 'NONE', #36804, .T. ) ;
#37000=ORIENTED_EDGE ( 'NONE', *, *, #49463, .T. ) ;
#37001=ORIENTED_EDGE ( 'NONE', *, *, #38978, .F. ) ;
#37002=ORIENTED_EDGE ( 'NONE', *, *, #4325, .T. ) ;
#37004=EDGE_LOOP ( 'NONE', ( #40641, #22303, #29718, #25284 ) ) ;
#37005=LINE ( 'NONE', #55154, #33908 ) ;
#37006=ORIENTED_EDGE ( 'NONE', *, *, #18527, .T. ) ;
#37007=CARTESIAN_POINT ( 'NONE',  ( -19.63273726619797088, -2.181752617796719029, 7.099516195845842148 ) ) ;
#37010=EDGE_CURVE ( 'NONE', #34036, #22830, #44548, .T. ) ;
#37011=VECTOR ( 'NONE', #29721, 1000.000000000000227 ) ;
#37012=VERTEX_POINT ( 'NONE', #26388 ) ;
#37013=CARTESIAN_POINT ( 'NONE',  ( -18.48776216474505674, 0.000000000000000000, 10.04718611902029934 ) ) ;
#37014=ORIENTED_EDGE ( 'NONE', *, *, #28741, .F. ) ;
#37015=EDGE_CURVE ( 'NONE', #6991, #44267, #35770, .T. ) ;
#37016=LINE ( 'NONE', #50339, #19218 ) ;
#37017=DIRECTION ( 'NONE',  ( -0.7660212471507179544, -0.6427876096865405842, -0.005961354470445141482 ) ) ;
#37018=CARTESIAN_POINT ( 'NONE',  ( -16.81267852042391198, -0.1191753592594197858, 3.312241722634738039 ) ) ;
#37019=FACE_OUTER_BOUND ( 'NONE', #33940, .T. ) ;
#37020=CARTESIAN_POINT ( 'NONE',  ( -14.20280369269832832, 0.000000000000000000, 12.40765738797303719 ) ) ;
#37021=DIRECTION ( 'NONE',  ( 0.000000000000000000, -0.000000000000000000, -1.000000000000000000 ) ) ;
#37022=CARTESIAN_POINT ( 'NONE',  ( -9.908141408373387193, -0.1191753592594197858, 10.77908512878318703 ) ) ;
#37024=VERTEX_POINT ( 'NONE', #9935 ) ;
#37025=DIRECTION ( 'NONE',  ( 0.005961354470445682716, -0.6427876096865404731, -0.7660212471507180654 ) ) ;
#37026=CARTESIAN_POINT ( 'NONE',  ( 2.072287782118878319, 0.000000000000000000, -2.950529333540147015 ) ) ;
#37027=DIRECTION ( 'NONE',  ( 0.007781995580012663651, -3.146120232559066537E-19, -0.9999697198139514409 ) ) ;
#37028=DIRECTION ( 'NONE',  ( -0.005961354470445682716, -0.6427876096865404731, 0.7660212471507180654 ) ) ;
#37029=CARTESIAN_POINT ( 'NONE',  ( -1.602641424070903486, 5.553834702102301790, 3.840893930704793569 ) ) ;
#37030=ORIENTED_EDGE ( 'NONE', *, *, #9128, .T. ) ;
#37031=LINE ( 'NONE', #29052, #34063 ) ;
#37032=FACE_OUTER_BOUND ( 'NONE', #45255, .T. ) ;
#37033=ORIENTED_EDGE ( 'NONE', *, *, #3975, .T. ) ;
#37034=DIRECTION ( 'NONE',  ( -0.005961354470445682716, -0.6427876096865404731, 0.7660212471507180654 ) ) ;
#37035=CARTESIAN_POINT ( 'NONE',  ( -15.86710544311044302, 0.000000000000000000, 13.13336954653252953 ) ) ;
#37036=ORIENTED_EDGE ( 'NONE', *, *, #48033, .F. ) ;
#37037=FACE_OUTER_BOUND ( 'NONE', #17575, .T. ) ;
#37038=DIRECTION ( 'NONE',  ( 0.007781995580012663651, -3.146120232559066537E-19, -0.9999697198139514409 ) ) ;
#37040=LINE ( 'NONE', #28502, #42233 ) ;
#37041=EDGE_CURVE ( 'NONE', #47084, #32426, #31786, .T. ) ;
#37042=CARTESIAN_POINT ( 'NONE',  ( -20.54204810873173415, 0.000000000000000000, 4.860550213503115558 ) ) ;
#37044=ORIENTED_EDGE ( 'NONE', *, *, #45554, .T. ) ;
#37045=EDGE_CURVE ( 'NONE', #54483, #13455, #1395, .T. ) ;
#37046=VERTEX_POINT ( 'NONE', #48547 ) ;
#37047=DIRECTION ( 'NONE',  ( 0.9999697198139515519, 0.000000000000000000, 0.007781995580013368816 ) ) ;
#37048=DIRECTION ( 'NONE',  ( 0.5364919789714477361, 0.6444004775717706579, 0.5449076811759711036 ) ) ;
#37049=LINE ( 'NONE', #38144, #6140 ) ;
#37050=EDGE_CURVE ( 'NONE', #52840, #23668, #30932, .T. ) ;
#37051=CARTESIAN_POINT ( 'NONE',  ( -16.29195844028956230, 0.000000000000000000, 8.017607966079944859 ) ) ;
#37052=VECTOR ( 'NONE', #19972, 1000.000000000000227 ) ;
#37053=CARTESIAN_POINT ( 'NONE',  ( -28.93137873341882127, 0.000000000000000000, 8.119251130998824451 ) ) ;
#37054=EDGE_CURVE ( 'NONE', #20652, #50912, #34940, .T. ) ;
#37055=CARTESIAN_POINT ( 'NONE',  ( -15.88130887279446490, 0.000000000000000000, 3.050160814894388839 ) ) ;
#37056=ORIENTED_EDGE ( 'NONE', *, *, #38227, .F. ) ;
#37057=DIRECTION ( 'NONE',  ( -0.9999697198139514409, -0.000000000000000000, -0.007781995580013368816 ) ) ;
#37058=CARTESIAN_POINT ( 'NONE',  ( -14.94760462649100496, 0.000000000000000000, 2.488088991209854051 ) ) ;
#37059=LINE ( 'NONE', #33614, #16046 ) ;
#37060=ORIENTED_EDGE ( 'NONE', *, *, #51370, .F. ) ;
#37062=DIRECTION ( 'NONE',  ( 0.000000000000000000, -1.000000000000000000, 0.000000000000000000 ) ) ;
#37063=CARTESIAN_POINT ( 'NONE',  ( -9.808144436391993182, 0.000000000000000000, 10.77986332834118777 ) ) ;
#37064=ORIENTED_EDGE ( 'NONE', *, *, #3203, .T. ) ;
#37065=DIRECTION ( 'NONE',  ( 0.5364919789714477361, 0.6444004775717706579, 0.5449076811759711036 ) ) ;
#37066=ORIENTED_EDGE ( 'NONE', *, *, #38407, .T. ) ;
#37068=EDGE_LOOP ( 'NONE', ( #9062, #12192, #26959, #33511 ) ) ;
#37069=EDGE_LOOP ( 'NONE', ( #28106, #12902, #5422, #39080 ) ) ;
#37070=VERTEX_POINT ( 'NONE', #48240 ) ;
#37072=ORIENTED_EDGE ( 'NONE', *, *, #51923, .T. ) ;
#37073=ADVANCED_FACE ( 'NONE', ( #43702 ), #22142, .F. ) ;
#37074=ORIENTED_EDGE ( 'NONE', *, *, #55716, .T. ) ;
#37076=ORIENTED_EDGE ( 'NONE', *, *, #9900, .T. ) ;
#37078=EDGE_CURVE ( 'NONE', #10313, #29764, #35227, .T. ) ;
#37079=EDGE_CURVE ( 'NONE', #49166, #53648, #39756, .T. ) ;
#37081=DIRECTION ( 'NONE',  ( 0.9999697198139515519, 0.000000000000000000, 0.007781995580013368816 ) ) ;
#37082=CARTESIAN_POINT ( 'NONE',  ( -23.33849165029409889, 0.000000000000000000, 5.946783852668351855 ) ) ;
#37084=DIRECTION ( 'NONE',  ( -0.9999697198139514409, -0.000000000000000000, -0.007781995580013368816 ) ) ;
#37085=ORIENTED_EDGE ( 'NONE', *, *, #20903, .F. ) ;
#37086=DIRECTION ( 'NONE',  ( -0.5449076811759708816, 0.6444004775717707689, 0.5364919789714475140 ) ) ;
#37087=ORIENTED_EDGE ( 'NONE', *, *, #30959, .F. ) ;
#37088=AXIS2_PLACEMENT_3D ( 'NONE', #12864, #35298, #17976 ) ;
#37089=ORIENTED_EDGE ( 'NONE', *, *, #11894, .T. ) ;
#37090=CARTESIAN_POINT ( 'NONE',  ( -11.87243407472968926, 0.000000000000000000, 11.50246268866867361 ) ) ;
#37091=CARTESIAN_POINT ( 'NONE',  ( -17.38961158937641471, 0.000000000000000000, 3.946413007592513456 ) ) ;
#37093=EDGE_CURVE ( 'NONE', #37968, #43469, #22701, .T. ) ;
#37094=CARTESIAN_POINT ( 'NONE',  ( 2.602374448188125350E-16, -1.000000000000000000, -2.125000000000000000 ) ) ;
#37095=DIRECTION ( 'NONE',  ( 0.007781995580012663651, -3.146120232559066537E-19, -0.9999697198139514409 ) ) ;
#37096=CARTESIAN_POINT ( 'NONE',  ( -15.32244789753343461, 0.000000000000000000, 2.854503944007263261 ) ) ;
#37097=LINE ( 'NONE', #54394, #13205 ) ;
#37098=ORIENTED_EDGE ( 'NONE', *, *, #27903, .F. ) ;
#37099=DIRECTION ( 'NONE',  ( 0.000000000000000000, -1.000000000000000000, 0.000000000000000000 ) ) ;
#37100=ORIENTED_EDGE ( 'NONE', *, *, #26105, .F. ) ;
#37101=PLANE ( 'NONE',  #14762 ) ;
#37102=DIRECTION ( 'NONE',  ( 0.007781995580012662783, 0.000000000000000000, -0.9999697198139514409 ) ) ;
#37103=CARTESIAN_POINT ( 'NONE',  ( -14.94838282604900748, -0.1191753592594197858, 2.588085963191248506 ) ) ;
#37104=PLANE ( 'NONE',  #53982 ) ;
#37105=LINE ( 'NONE', #14679, #50433 ) ;
#37106=EDGE_LOOP ( 'NONE', ( #36305, #35748, #26668, #35137 ) ) ;
#37108=PLANE ( 'NONE',  #43952 ) ;
#37109=CARTESIAN_POINT ( 'NONE',  ( -16.69548912546022734, -0.5179957512181551094, 4.017145964781438039 ) ) ;
#37110=DIRECTION ( 'NONE',  ( 0.000000000000000000, -0.000000000000000000, -1.000000000000000000 ) ) ;
#37111=EDGE_CURVE ( 'NONE', #40689, #21263, #45384, .T. ) ;
#37112=DIRECTION ( 'NONE',  ( -0.6427681459581293666, -0.7660444431189770143, -0.005002170337467561935 ) ) ;
#37113=LINE ( 'NONE', #41905, #44497 ) ;
#37114=LINE ( 'NONE', #36283, #36518 ) ;
#37115=DIRECTION ( 'NONE',  ( 0.007781995580012662783, 0.000000000000000000, -0.9999697198139514409 ) ) ;
#37116=DIRECTION ( 'NONE',  ( 0.9999697198139515519, 0.000000000000000000, 0.007781995580013368816 ) ) ;
#37117=EDGE_LOOP ( 'NONE', ( #28837, #4847, #2251, #27963 ) ) ;
#37118=ADVANCED_FACE ( 'NONE', ( #1677 ), #36602, .F. ) ;
#37119=EDGE_LOOP ( 'NONE', ( #7346, #2974, #35519, #51073 ) ) ;
#37120=ADVANCED_FACE ( 'NONE', ( #3297 ), #28079, .F. ) ;
#37121=EDGE_CURVE ( 'NONE', #46316, #2289, #29717, .T. ) ;
#37122=VERTEX_POINT ( 'NONE', #51276 ) ;
#37123=ORIENTED_EDGE ( 'NONE', *, *, #32826, .T. ) ;
#37124=ORIENTED_EDGE ( 'NONE', *, *, #10, .T. ) ;
#37125=VERTEX_POINT ( 'NONE', #19003 ) ;
#37126=PLANE ( 'NONE',  #35995 ) ;
#37127=DIRECTION ( 'NONE',  ( -0.5364919789714478471, 0.6444004775717705469, -0.5449076811759709926 ) ) ;
#37128=ADVANCED_FACE ( 'NONE', ( #40603 ), #19565, .F. ) ;
#37129=DIRECTION ( 'NONE',  ( -0.9999697198139514409, -0.000000000000000000, -0.007781995580013368816 ) ) ;
#37130=VERTEX_POINT ( 'NONE', #11023 ) ;
#37131=ADVANCED_FACE ( 'NONE', ( #55243 ), #12392, .F. ) ;
#37132=LINE ( 'NONE', #32860, #19513 ) ;
#37134=VERTEX_POINT ( 'NONE', #7542 ) ;
#37135=EDGE_CURVE ( 'NONE', #52707, #27279, #1935, .T. ) ;
#37137=DIRECTION ( 'NONE',  ( -0.9999697198139514409, -0.000000000000000000, -0.007781995580013368816 ) ) ;
#37138=LINE ( 'NONE', #40837, #30504 ) ;
#37139=ORIENTED_EDGE ( 'NONE', *, *, #37093, .F. ) ;
#37140=CARTESIAN_POINT ( 'NONE',  ( -21.47419595591918906, 0.000000000000000000, 5.222628093224860102 ) ) ;
#37141=ORIENTED_EDGE ( 'NONE', *, *, #23561, .T. ) ;
#37142=EDGE_CURVE ( 'NONE', #21011, #34747, #36321, .T. ) ;
#37143=DIRECTION ( 'NONE',  ( -0.5449076811759708816, 0.6444004775717707689, 0.5364919789714475140 ) ) ;
#37144=DIRECTION ( 'NONE',  ( 0.5449076811759707706, 0.6444004775717708799, -0.5364919789714476250 ) ) ;
#37145=EDGE_CURVE ( 'NONE', #931, #10342, #41138, .T. ) ;
#37146=CARTESIAN_POINT ( 'NONE',  ( -18.79634312187524614, 5.467268677019011314, 13.15517843894362038 ) ) ;
#37147=CARTESIAN_POINT ( 'NONE',  ( -16.27627051837387029, 0.000000000000000000, 6.001743690496146755 ) ) ;
#37148=CARTESIAN_POINT ( 'NONE',  ( -15.88053067323646417, -0.1191753592594197858, 2.950163842912994383 ) ) ;
#37149=DIRECTION ( 'NONE',  ( -0.9999697198139514409, -0.000000000000000000, -0.007781995580013368816 ) ) ;
#37150=DIRECTION ( 'NONE',  ( 0.6427681459581294776, -0.7660444431189769032, 0.005002170337467562802 ) ) ;
#37151=CARTESIAN_POINT ( 'NONE',  ( -10.77685410066197846, -0.1191753592594185784, 2.989881834110746262 ) ) ;
#37152=ORIENTED_EDGE ( 'NONE', *, *, #2456, .T. ) ;
#37154=ORIENTED_EDGE ( 'NONE', *, *, #17735, .T. ) ;
#37156=CARTESIAN_POINT ( 'NONE',  ( -21.20448354515064437, 2.876837460659008361, 4.826687070827041737 ) ) ;
#37157=CARTESIAN_POINT ( 'NONE',  ( -15.55914933374884512, -2.460819163488158878, 6.764257206824528801 ) ) ;
#37158=CARTESIAN_POINT ( 'NONE',  ( -10.84028925556084388, -0.1191753592594197858, 11.14116300850493246 ) ) ;
#37159=CARTESIAN_POINT ( 'NONE',  ( -14.86068505419763142, 0.000000000000000000, 3.227429559033034856 ) ) ;
#37160=DIRECTION ( 'NONE',  ( -0.005002170337468016433, -0.7660444431189770143, 0.6427681459581293666 ) ) ;
#37162=ORIENTED_EDGE ( 'NONE', *, *, #6055, .T. ) ;
#37163=DIRECTION ( 'NONE',  ( -0.7660212471507179544, -0.6427876096865405842, -0.005961354470445141482 ) ) ;
#37164=DIRECTION ( 'NONE',  ( 0.000000000000000000, -1.000000000000000000, 0.000000000000000000 ) ) ;
#37165=CARTESIAN_POINT ( 'NONE',  ( -19.60834386242827776, 0.000000000000000000, 4.298478389818581213 ) ) ;
#37166=DIRECTION ( 'NONE',  ( -0.005961354470445682716, -0.6427876096865404731, 0.7660212471507180654 ) ) ;
#37167=FACE_OUTER_BOUND ( 'NONE', #15951, .T. ) ;
#37168=CARTESIAN_POINT ( 'NONE',  ( -20.54126990917373519, -0.1191753592594197858, 4.760553241521720658 ) ) ;
#37169=EDGE_CURVE ( 'NONE', #4596, #26120, #24867, .T. ) ;
#37170=DIRECTION ( 'NONE',  ( -0.9999697198139514409, -0.000000000000000000, -0.007781995580013368816 ) ) ;
#37171=LINE ( 'NONE', #16156, #48700 ) ;
#37172=PLANE ( 'NONE',  #17491 ) ;
#37173=ORIENTED_EDGE ( 'NONE', *, *, #46483, .F. ) ;
#37174=CARTESIAN_POINT ( 'NONE',  ( -8.609916609573598834, 0.000000000000000000, 10.23519010964256637 ) ) ;
#37175=ORIENTED_EDGE ( 'NONE', *, *, #37894, .T. ) ;
#37176=DIRECTION ( 'NONE',  ( 0.9999697198139515519, 0.000000000000000000, 0.007781995580013368816 ) ) ;
#37177=PLANE ( 'NONE',  #50968 ) ;
#37178=ADVANCED_FACE ( 'NONE', ( #10501 ), #15304, .F. ) ;
#37179=ORIENTED_EDGE ( 'NONE', *, *, #50789, .F. ) ;
#37180=ORIENTED_EDGE ( 'NONE', *, *, #36647, .T. ) ;
#37181=PLANE ( 'NONE',  #51090 ) ;
#37183=VECTOR ( 'NONE', #3301, 1000.000000000000114 ) ;
#37184=EDGE_LOOP ( 'NONE', ( #50238, #36200, #28310, #37656 ) ) ;
#37185=VERTEX_POINT ( 'NONE', #19266 ) ;
#37186=ORIENTED_EDGE ( 'NONE', *, *, #797, .F. ) ;
#37187=CARTESIAN_POINT ( 'NONE',  ( -19.32961685222932147, 0.000000000000000000, 14.39908572644263351 ) ) ;
#37188=DIRECTION ( 'NONE',  ( -0.7660212471507179544, -0.6427876096865405842, -0.005961354470445141482 ) ) ;
#37189=CARTESIAN_POINT ( 'NONE',  ( -18.66354898467281132, 0.000000000000000000, 14.21960318569776582 ) ) ;
#37190=EDGE_CURVE ( 'NONE', #13455, #22275, #20874, .T. ) ;
#37191=EDGE_LOOP ( 'NONE', ( #17928, #17171, #13536, #7255 ) ) ;
#37192=ORIENTED_EDGE ( 'NONE', *, *, #29814, .T. ) ;
#37193=EDGE_CURVE ( 'NONE', #36955, #34381, #6238, .T. ) ;
#37195=DIRECTION ( 'NONE',  ( -0.005961354470445682716, -0.6427876096865404731, 0.7660212471507180654 ) ) ;
#37196=ORIENTED_EDGE ( 'NONE', *, *, #39955, .F. ) ;
#37197=DIRECTION ( 'NONE',  ( 0.9999697198139515519, 0.000000000000000000, 0.007781995580013368816 ) ) ;
#37198=EDGE_LOOP ( 'NONE', ( #55917, #39234, #23112, #47006 ) ) ;
#37199=DIRECTION ( 'NONE',  ( -0.6427681459581293666, -0.7660444431189770143, -0.005002170337467561935 ) ) ;
#37200=CARTESIAN_POINT ( 'NONE',  ( -28.92982233430281980, 0.000000000000000000, 7.919257187036034651 ) ) ;
#37201=EDGE_CURVE ( 'NONE', #23095, #29543, #10770, .T. ) ;
#37202=ORIENTED_EDGE ( 'NONE', *, *, #43715, .T. ) ;
#37203=ADVANCED_FACE ( 'NONE', ( #2223 ), #36903, .F. ) ;
#37204=DIRECTION ( 'NONE',  ( 0.005961354470445682716, -0.6427876096865404731, -0.7660212471507180654 ) ) ;
#37205=ORIENTED_EDGE ( 'NONE', *, *, #47305, .F. ) ;
#37206=LINE ( 'NONE', #10822, #31277 ) ;
#37208=CARTESIAN_POINT ( 'NONE',  ( -10.14636587563368764, 0.2096447517685606221, 0.8722069013983897445 ) ) ;
#37209=ORIENTED_EDGE ( 'NONE', *, *, #56074, .F. ) ;
#37210=CARTESIAN_POINT ( 'NONE',  ( -13.57617169572962190, -0.1191753592594188005, 4.445425176533747802 ) ) ;
#37211=DIRECTION ( 'NONE',  ( 0.007781995580012663651, 0.000000000000000000, -0.9999697198139515519 ) ) ;
#37212=PLANE ( 'NONE',  #24019 ) ;
#37213=DIRECTION ( 'NONE',  ( 0.000000000000000000, -1.000000000000000000, 0.000000000000000000 ) ) ;
#37214=CARTESIAN_POINT ( 'NONE',  ( -20.39737380963304858, -0.1191753592594195638, 5.131005144047771971 ) ) ;
#37215=CARTESIAN_POINT ( 'NONE',  ( -10.90796677398788006, 0.6102101463440047224, 0.8994875641494844976 ) ) ;
#37216=VECTOR ( 'NONE', #45460, 1000.000000000000114 ) ;
#37217=DIRECTION ( 'NONE',  ( 0.000000000000000000, -1.000000000000000000, 0.000000000000000000 ) ) ;
#37218=ORIENTED_EDGE ( 'NONE', *, *, #28711, .T. ) ;
#37219=PLANE ( 'NONE',  #24082 ) ;
#37221=EDGE_LOOP ( 'NONE', ( #11739, #38892, #2748, #16813 ) ) ;
#37222=CARTESIAN_POINT ( 'NONE',  ( -14.01206388602242292, 3.686347215771508257, 8.374006385476546299 ) ) ;
#37223=DIRECTION ( 'NONE',  ( -0.5449076811759708816, 0.6444004775717707689, 0.5364919789714475140 ) ) ;
#37224=LINE ( 'NONE', #41219, #8640 ) ;
#37225=EDGE_CURVE ( 'NONE', #12737, #30623, #43578, .T. ) ;
#37226=DIRECTION ( 'NONE',  ( 0.007781995580012663651, -3.146120232559066537E-19, -0.9999697198139514409 ) ) ;
#37228=VERTEX_POINT ( 'NONE', #21736 ) ;
#37229=EDGE_CURVE ( 'NONE', #37046, #10112, #13499, .T. ) ;
#37230=ORIENTED_EDGE ( 'NONE', *, *, #6851, .T. ) ;
#37232=CARTESIAN_POINT ( 'NONE',  ( -21.03231001138954070, 4.333955019861511992, 4.713319344289897295 ) ) ;
#37233=EDGE_CURVE ( 'NONE', #15067, #52765, #4143, .T. ) ;
#37234=EDGE_CURVE ( 'NONE', #41830, #37629, #4426, .T. ) ;
#37235=EDGE_CURVE ( 'NONE', #38019, #12500, #39046, .T. ) ;
#37236=LINE ( 'NONE', #42618, #19350 ) ;
#37237=CARTESIAN_POINT ( 'NONE',  ( -14.48966086313376600, -0.1191753592594185784, 2.409902774531527569 ) ) ;
#37238=AXIS2_PLACEMENT_3D ( 'NONE', #54245, #15598, #36945 ) ;
#37239=VERTEX_POINT ( 'NONE', #12926 ) ;
#37240=CARTESIAN_POINT ( 'NONE',  ( -11.87243407472968926, 0.000000000000000000, 11.50246268866867361 ) ) ;
#37241=ORIENTED_EDGE ( 'NONE', *, *, #37329, .T. ) ;
#37242=DIRECTION ( 'NONE',  ( 0.005961354470445682716, -0.6427876096865404731, -0.7660212471507180654 ) ) ;
#37243=ORIENTED_EDGE ( 'NONE', *, *, #24319, .F. ) ;
#37244=ORIENTED_EDGE ( 'NONE', *, *, #7547, .F. ) ;
#37245=CARTESIAN_POINT ( 'NONE',  ( -16.33317936670417225, 0.000000000000000000, 13.31440848639340224 ) ) ;
#37246=PLANE ( 'NONE',  #42287 ) ;
#37247=CARTESIAN_POINT ( 'NONE',  ( -19.60834386242827776, 0.000000000000000000, 4.298478389818581213 ) ) ;
#37248=ORIENTED_EDGE ( 'NONE', *, *, #44450, .T. ) ;
#37249=VECTOR ( 'NONE', #27881, 1000.000000000000000 ) ;
#37250=CARTESIAN_POINT ( 'NONE',  ( -16.11636885593316393, -5.375054281893166142, 2.969973721925023291 ) ) ;
#37252=VERTEX_POINT ( 'NONE', #4683 ) ;
#37253=VECTOR ( 'NONE', #1051, 999.9999999999998863 ) ;
#37254=ADVANCED_FACE ( 'NONE', ( #26017 ), #38486, .F. ) ;
#37255=VERTEX_POINT ( 'NONE', #17187 ) ;
#37256=ORIENTED_EDGE ( 'NONE', *, *, #39615, .T. ) ;
#37257=PLANE ( 'NONE',  #14124 ) ;
#37258=EDGE_CURVE ( 'NONE', #52840, #28798, #25425, .T. ) ;
#37259=ORIENTED_EDGE ( 'NONE', *, *, #37646, .F. ) ;
#37260=CARTESIAN_POINT ( 'NONE',  ( -12.26136140309277778, 0.000000000000000000, 1.770329817494030955 ) ) ;
#37261=ORIENTED_EDGE ( 'NONE', *, *, #46582, .F. ) ;
#37262=PLANE ( 'NONE',  #48506 ) ;
#37263=PLANE ( 'NONE',  #25002 ) ;
#37265=ORIENTED_EDGE ( 'NONE', *, *, #20942, .T. ) ;
#37266=FACE_OUTER_BOUND ( 'NONE', #39785, .T. ) ;
#37267=ORIENTED_EDGE ( 'NONE', *, *, #50732, .T. ) ;
#37268=CARTESIAN_POINT ( 'NONE',  ( -15.82531159426634915, 4.172053068839010059, 9.875459425361245991 ) ) ;
#37269=PLANE ( 'NONE',  #36583 ) ;
#37270=DIRECTION ( 'NONE',  ( 0.7660212471507180654, -0.6427876096865404731, 0.005961354470445141482 ) ) ;
#37271=CARTESIAN_POINT ( 'NONE',  ( -15.47205284714705442, -0.1191753592594190225, 9.228244334622088374 ) ) ;
#37272=CARTESIAN_POINT ( 'NONE',  ( -18.42457910756102990, 0.000000000000000000, 3.938358651053141202 ) ) ;
#37273=LINE ( 'NONE', #46639, #50030 ) ;
#37274=ORIENTED_EDGE ( 'NONE', *, *, #28455, .T. ) ;
#37275=VECTOR ( 'NONE', #8194, 1000.000000000000227 ) ;
#37276=ORIENTED_EDGE ( 'NONE', *, *, #25121, .T. ) ;
#37277=VECTOR ( 'NONE', #28908, 1000.000000000000114 ) ;
#37279=DIRECTION ( 'NONE',  ( 0.007781995580012663651, 0.000000000000000000, -0.9999697198139515519 ) ) ;
#37280=CARTESIAN_POINT ( 'NONE',  ( -20.91587874690506155, 3.038739411681507185, 9.992847796181067110 ) ) ;
#37281=CARTESIAN_POINT ( 'NONE',  ( -9.505154610604371612, 0.000000000000000000, 5.854432023937497398 ) ) ;
#37282=CARTESIAN_POINT ( 'NONE',  ( 2.072287782118878319, 0.000000000000000000, -2.950529333540147015 ) ) ;
#37283=VERTEX_POINT ( 'NONE', #712 ) ;
#37284=DIRECTION ( 'NONE',  ( 0.9999697198139515519, 0.000000000000000000, 0.007781995580013368816 ) ) ;
#37285=DIRECTION ( 'NONE',  ( 0.000000000000000000, -1.000000000000000000, 0.000000000000000000 ) ) ;
#37286=ORIENTED_EDGE ( 'NONE', *, *, #26353, .F. ) ;
#37287=DIRECTION ( 'NONE',  ( 0.6427681459581294776, -0.7660444431189769032, 0.005002170337467562802 ) ) ;
#37288=DIRECTION ( 'NONE',  ( -0.005002170337468016433, -0.7660444431189770143, 0.6427681459581293666 ) ) ;
#37289=ORIENTED_EDGE ( 'NONE', *, *, #2448, .F. ) ;
#37291=CARTESIAN_POINT ( 'NONE',  ( -17.33062956602698179, -0.1191753592594162470, 9.217524024740605171 ) ) ;
#37292=DIRECTION ( 'NONE',  ( 0.005961354470445682716, -0.6427876096865404731, -0.7660212471507180654 ) ) ;
#37293=DIRECTION ( 'NONE',  ( 0.000000000000000000, -1.000000000000000000, 0.000000000000000000 ) ) ;
#37294=VECTOR ( 'NONE', #11905, 999.9999999999998863 ) ;
#37295=CARTESIAN_POINT ( 'NONE',  ( -13.27065584551087163, 0.000000000000000000, 12.04557950825129176 ) ) ;
#37296=VERTEX_POINT ( 'NONE', #39332 ) ;
#37297=ORIENTED_EDGE ( 'NONE', *, *, #46164, .F. ) ;
#37298=PLANE ( 'NONE',  #53866 ) ;
#37299=FACE_OUTER_BOUND ( 'NONE', #35817, .T. ) ;
#37300=DIRECTION ( 'NONE',  ( -0.6427681459581293666, -0.7660444431189770143, -0.005002170337467561935 ) ) ;
#37301=EDGE_CURVE ( 'NONE', #23151, #29528, #18033, .T. ) ;
#37302=ADVANCED_FACE ( 'NONE', ( #42733 ), #34253, .F. ) ;
#37303=PLANE ( 'NONE',  #22080 ) ;
#37304=LINE ( 'NONE', #46675, #9275 ) ;
#37305=CARTESIAN_POINT ( 'NONE',  ( -25.20278734466900517, 0.000000000000000000, 6.670939612111840944 ) ) ;
#37306=EDGE_LOOP ( 'NONE', ( #32187, #33545, #51452, #10750 ) ) ;
#37307=EDGE_CURVE ( 'NONE', #37711, #31703, #47864, .T. ) ;
#37308=DIRECTION ( 'NONE',  ( 0.000000000000000000, -1.000000000000000000, 0.000000000000000000 ) ) ;
#37309=DIRECTION ( 'NONE',  ( -0.6246952433987894571, 0.7422098413412802076, 0.2426528472758539834 ) ) ;
#37310=DIRECTION ( 'NONE',  ( 0.005002170337468016433, -0.7660444431189770143, -0.6427681459581293666 ) ) ;
#37311=EDGE_LOOP ( 'NONE', ( #37461, #31523, #21618, #27137 ) ) ;
#37312=CARTESIAN_POINT ( 'NONE',  ( -23.33849165029409889, 0.000000000000000000, 5.946783852668351855 ) ) ;
#37313=PLANE ( 'NONE',  #51286 ) ;
#37314=EDGE_CURVE ( 'NONE', #883, #11534, #26269, .T. ) ;
#37315=CARTESIAN_POINT ( 'NONE',  ( -11.34070976992645363, 0.000000000000000000, 2.885490750803344273 ) ) ;
#37316=ORIENTED_EDGE ( 'NONE', *, *, #52884, .T. ) ;
#37317=VECTOR ( 'NONE', #38577, 1000.000000000000227 ) ;
#37318=VECTOR ( 'NONE', #47784, 999.9999999999998863 ) ;
#37319=DIRECTION ( 'NONE',  ( 0.005961354470445682716, -0.6427876096865404731, -0.7660212471507180654 ) ) ;
#37320=ORIENTED_EDGE ( 'NONE', *, *, #31514, .F. ) ;
#37321=ORIENTED_EDGE ( 'NONE', *, *, #50261, .F. ) ;
#37322=ORIENTED_EDGE ( 'NONE', *, *, #16958, .F. ) ;
#37323=VERTEX_POINT ( 'NONE', #3832 ) ;
#37324=VECTOR ( 'NONE', #2634, 1000.000000000000227 ) ;
#37325=ADVANCED_FACE ( 'NONE', ( #21162 ), #17763, .F. ) ;
#37326=ORIENTED_EDGE ( 'NONE', *, *, #5368, .F. ) ;
#37327=CARTESIAN_POINT ( 'NONE',  ( -12.49980730458054978, 0.2864062442990030766, 1.528143525138426773 ) ) ;
#37328=VERTEX_POINT ( 'NONE', #29971 ) ;
#37329=EDGE_CURVE ( 'NONE', #23582, #31229, #49542, .T. ) ;
#37330=EDGE_LOOP ( 'NONE', ( #54670, #7107, #40643, #30066, #5430 ) ) ;
#37331=LINE ( 'NONE', #6163, #7721 ) ;
#37333=ORIENTED_EDGE ( 'NONE', *, *, #40626, .F. ) ;
#37334=ADVANCED_FACE ( 'NONE', ( #36756 ), #19132, .F. ) ;
#37335=AXIS2_PLACEMENT_3D ( 'NONE', #6622, #24233, #33858 ) ;
#37336=CARTESIAN_POINT ( 'NONE',  ( -27.99767448711536133, 0.000000000000000000, 7.557179307314289218 ) ) ;
#37337=LINE ( 'NONE', #41346, #47563 ) ;
#37338=CARTESIAN_POINT ( 'NONE',  ( -17.18893626679898645, 5.305366725996512933, 3.189429341044820454 ) ) ;
#37339=LINE ( 'NONE', #50113, #15049 ) ;
#37340=ORIENTED_EDGE ( 'NONE', *, *, #52194, .T. ) ;
#37341=LINE ( 'NONE', #41872, #52814 ) ;
#37342=VERTEX_POINT ( 'NONE', #5269 ) ;
#37343=VERTEX_POINT ( 'NONE', #45268 ) ;
#37344=CARTESIAN_POINT ( 'NONE',  ( -16.99924723426068951, 0.000000000000000000, 13.49389102713827171 ) ) ;
#37346=FACE_OUTER_BOUND ( 'NONE', #51643, .T. ) ;
#37347=DIRECTION ( 'NONE',  ( -0.005002170337468016433, -0.7660444431189770143, 0.6427681459581293666 ) ) ;
#37348=LINE ( 'NONE', #50131, #18619 ) ;
#37349=PLANE ( 'NONE',  #37686 ) ;
#37350=ORIENTED_EDGE ( 'NONE', *, *, #4761, .F. ) ;
#37351=CARTESIAN_POINT ( 'NONE',  ( -18.13613576012749817, 0.000000000000000000, 6.156595802719084354 ) ) ;
#37352=ORIENTED_EDGE ( 'NONE', *, *, #20205, .F. ) ;
#37353=AXIS2_PLACEMENT_3D ( 'NONE', #11492, #3241, #20266 ) ;
#37354=VECTOR ( 'NONE', #4474, 1000.000000000000227 ) ;
#37355=LINE ( 'NONE', #19200, #20165 ) ;
#37356=DIRECTION ( 'NONE',  ( 0.000000000000000000, -1.000000000000000000, 0.000000000000000000 ) ) ;
#37357=PLANE ( 'NONE',  #54434 ) ;
#37358=PLANE ( 'NONE',  #31338 ) ;
#37359=DIRECTION ( 'NONE',  ( 0.5364919789714477361, 0.6444004775717706579, 0.5449076811759711036 ) ) ;
#37360=ORIENTED_EDGE ( 'NONE', *, *, #32016, .T. ) ;
#37361=VECTOR ( 'NONE', #25012, 1000.000000000000227 ) ;
#37362=EDGE_LOOP ( 'NONE', ( #27187, #29611, #27388, #38225 ) ) ;
#37363=LINE ( 'NONE', #54683, #21241 ) ;
#37364=DIRECTION ( 'NONE',  ( 0.000000000000000000, -1.000000000000000000, 0.000000000000000000 ) ) ;
#37365=LINE ( 'NONE', #28875, #15207 ) ;
#37366=EDGE_CURVE ( 'NONE', #40739, #14885, #27965, .T. ) ;
#37367=DIRECTION ( 'NONE',  ( 0.000000000000000000, 0.000000000000000000, 1.000000000000000000 ) ) ;
#37368=VECTOR ( 'NONE', #17824, 1000.000000000000227 ) ;
#37369=CARTESIAN_POINT ( 'NONE',  ( 2.072287782118878319, 0.000000000000000000, -2.950529333540147015 ) ) ;
#37371=LINE ( 'NONE', #10450, #11856 ) ;
#37373=FACE_OUTER_BOUND ( 'NONE', #2762, .T. ) ;
#37375=LINE ( 'NONE', #54695, #39192 ) ;
#37376=ORIENTED_EDGE ( 'NONE', *, *, #19542, .F. ) ;
#37377=VECTOR ( 'NONE', #27971, 999.9999999999998863 ) ;
#37378=VERTEX_POINT ( 'NONE', #6119 ) ;
#37379=ORIENTED_EDGE ( 'NONE', *, *, #26913, .T. ) ;
#37380=ORIENTED_EDGE ( 'NONE', *, *, #40793, .F. ) ;
#37381=ORIENTED_EDGE ( 'NONE', *, *, #9979, .T. ) ;
#37382=VECTOR ( 'NONE', #13171, 1000.000000000000227 ) ;
#37383=DIRECTION ( 'NONE',  ( 0.000000000000000000, -1.000000000000000000, 0.000000000000000000 ) ) ;
#37385=LINE ( 'NONE', #15815, #31286 ) ;
#37386=VECTOR ( 'NONE', #22659, 1000.000000000000227 ) ;
#37387=VECTOR ( 'NONE', #23340, 1000.000000000000000 ) ;
#37388=ORIENTED_EDGE ( 'NONE', *, *, #26977, .T. ) ;
#37389=ORIENTED_EDGE ( 'NONE', *, *, #3283, .F. ) ;
#37390=ORIENTED_EDGE ( 'NONE', *, *, #52011, .T. ) ;
#37392=VERTEX_POINT ( 'NONE', #44697 ) ;
#37393=EDGE_CURVE ( 'NONE', #44507, #10018, #48401, .T. ) ;
#37394=AXIS2_PLACEMENT_3D ( 'NONE', #45920, #50990, #29436 ) ;
#37395=AXIS2_PLACEMENT_3D ( 'NONE', #36838, #18952, #15496 ) ;
#37397=EDGE_CURVE ( 'NONE', #23847, #34987, #14891, .T. ) ;
#37398=LINE ( 'NONE', #53887, #17396 ) ;
#37399=FACE_OUTER_BOUND ( 'NONE', #1431, .T. ) ;
#37400=EDGE_CURVE ( 'NONE', #9714, #3202, #23420, .T. ) ;
#37401=ORIENTED_EDGE ( 'NONE', *, *, #4522, .F. ) ;
#37402=LINE ( 'NONE', #41664, #52770 ) ;
#37403=ORIENTED_EDGE ( 'NONE', *, *, #8154, .F. ) ;
#37404=DIRECTION ( 'NONE',  ( 0.9999697198139515519, 0.000000000000000000, 0.007781995580013368816 ) ) ;
#37405=EDGE_CURVE ( 'NONE', #12044, #20122, #32219, .T. ) ;
#37406=VECTOR ( 'NONE', #17440, 999.9999999999998863 ) ;
#37407=DIRECTION ( 'NONE',  ( -0.005961354470445682716, -0.6427876096865404731, 0.7660212471507180654 ) ) ;
#37408=DIRECTION ( 'NONE',  ( 0.000000000000000000, -1.000000000000000000, 0.000000000000000000 ) ) ;
#37409=CARTESIAN_POINT ( 'NONE',  ( -21.10420191512951149, 1.095915999411505526, 4.844554998909636367 ) ) ;
#37410=DIRECTION ( 'NONE',  ( 0.007781995580012662783, 0.000000000000000000, -0.9999697198139514409 ) ) ;
#37411=FACE_OUTER_BOUND ( 'NONE', #27009, .T. ) ;
#37412=DIRECTION ( 'NONE',  ( 0.6427681459581294776, -0.7660444431189769032, 0.005002170337467562802 ) ) ;
#37413=FACE_OUTER_BOUND ( 'NONE', #34853, .T. ) ;
#37414=LINE ( 'NONE', #54199, #20199 ) ;
#37415=ORIENTED_EDGE ( 'NONE', *, *, #24734, .F. ) ;
#37416=CARTESIAN_POINT ( 'NONE',  ( -18.66354898467281132, 0.000000000000000000, 14.21960318569776582 ) ) ;
#37417=ORIENTED_EDGE ( 'NONE', *, *, #36036, .T. ) ;
#37418=VECTOR ( 'NONE', #52160, 1000.000000000000227 ) ;
#37419=CARTESIAN_POINT ( 'NONE',  ( -10.47421230394850866, 0.000000000000000000, 10.95934586908605723 ) ) ;
#37420=CARTESIAN_POINT ( 'NONE',  ( -11.77243710274829525, -0.1191753592594197858, 11.50324088822667612 ) ) ;
#37421=LINE ( 'NONE', #3371, #44096 ) ;
#37422=VECTOR ( 'NONE', #40322, 1000.000000000000114 ) ;
#37423=DIRECTION ( 'NONE',  ( -0.5364919789714478471, 0.6444004775717705469, -0.5449076811759709926 ) ) ;
#37424=CARTESIAN_POINT ( 'NONE',  ( -12.13851405436063047, 0.000000000000000000, 11.68505802764555135 ) ) ;
#37425=ADVANCED_FACE ( 'NONE', ( #9811 ), #40468, .F. ) ;
#37426=CARTESIAN_POINT ( 'NONE',  ( -19.22961988024793101, -0.1191753592594177458, 14.39986392600063603 ) ) ;
#37427=VERTEX_POINT ( 'NONE', #10063 ) ;
#37428=PLANE ( 'NONE',  #17446 ) ;
#37429=AXIS2_PLACEMENT_3D ( 'NONE', #55137, #55991, #38086 ) ;
#37430=FACE_OUTER_BOUND ( 'NONE', #13152, .T. ) ;
#37431=PLANE ( 'NONE',  #25839 ) ;
#37433=DIRECTION ( 'NONE',  ( 0.9999697198139515519, 0.000000000000000000, 0.007781995580013368816 ) ) ;
#37434=DIRECTION ( 'NONE',  ( 0.5364919789714477361, 0.6444004775717706579, 0.5449076811759711036 ) ) ;
#37435=AXIS2_PLACEMENT_3D ( 'NONE', #18314, #15646, #35653 ) ;
#37436=VECTOR ( 'NONE', #28643, 1000.000000000000227 ) ;
#37437=EDGE_CURVE ( 'NONE', #48957, #25894, #44419, .T. ) ;
#37438=DIRECTION ( 'NONE',  ( -0.6427681459581293666, -0.7660444431189770143, -0.005002170337467561935 ) ) ;
#37439=PLANE ( 'NONE',  #2136 ) ;
#37440=FACE_OUTER_BOUND ( 'NONE', #29617, .T. ) ;
#37441=EDGE_CURVE ( 'NONE', #25831, #19083, #52946, .T. ) ;
#37442=PLANE ( 'NONE',  #15615 ) ;
#37443=EDGE_CURVE ( 'NONE', #51780, #30062, #5524, .T. ) ;
#37444=ORIENTED_EDGE ( 'NONE', *, *, #49046, .T. ) ;
#37445=VECTOR ( 'NONE', #30836, 1000.000000000000227 ) ;
#37446=LINE ( 'NONE', #24132, #46649 ) ;
#37447=VECTOR ( 'NONE', #11399, 1000.000000000000227 ) ;
#37448=LINE ( 'NONE', #24964, #50454 ) ;
#37449=ORIENTED_EDGE ( 'NONE', *, *, #55248, .F. ) ;
#37450=CARTESIAN_POINT ( 'NONE',  ( -18.68223532000061482, -0.1166911823299036782, 4.038441074006483333 ) ) ;
#37451=CARTESIAN_POINT ( 'NONE',  ( -29.86274838104827367, -0.1191753592594197858, 8.381332038739175871 ) ) ;
#37452=ORIENTED_EDGE ( 'NONE', *, *, #45910, .T. ) ;
#37454=AXIS2_PLACEMENT_3D ( 'NONE', #1090, #18426, #44833 ) ;
#37455=ORIENTED_EDGE ( 'NONE', *, *, #17648, .F. ) ;
#37456=DIRECTION ( 'NONE',  ( -0.005961354470445682716, -0.6427876096865404731, 0.7660212471507180654 ) ) ;
#37457=VECTOR ( 'NONE', #13799, 1000.000000000000000 ) ;
#37458=ADVANCED_FACE ( 'NONE', ( #1806 ), #22843, .F. ) ;
#37459=ORIENTED_EDGE ( 'NONE', *, *, #5717, .F. ) ;
#37460=ORIENTED_EDGE ( 'NONE', *, *, #10154, .F. ) ;
#37461=ORIENTED_EDGE ( 'NONE', *, *, #55256, .F. ) ;
#37462=DIRECTION ( 'NONE',  ( -0.005961354470445682716, -0.6427876096865404731, 0.7660212471507180654 ) ) ;
#37463=CARTESIAN_POINT ( 'NONE',  ( -13.53673582514181106, 0.000000000000000000, 12.22817484722816772 ) ) ;
#37464=LINE ( 'NONE', #25267, #29423 ) ;
#37465=AXIS2_PLACEMENT_3D ( 'NONE', #19112, #40446, #44674 ) ;
#37466=ORIENTED_EDGE ( 'NONE', *, *, #52111, .F. ) ;
#37467=ORIENTED_EDGE ( 'NONE', *, *, #56007, .F. ) ;
#37468=AXIS2_PLACEMENT_3D ( 'NONE', #666, #39275, #44103 ) ;
#37469=DIRECTION ( 'NONE',  ( 0.000000000000000000, -0.000000000000000000, -1.000000000000000000 ) ) ;
#37470=DIRECTION ( 'NONE',  ( 0.007781995580012663651, 0.000000000000000000, -0.9999697198139515519 ) ) ;
#37471=ORIENTED_EDGE ( 'NONE', *, *, #5596, .T. ) ;
#37473=DIRECTION ( 'NONE',  ( 0.6427681459581294776, -0.7660444431189769032, 0.005002170337467562802 ) ) ;
#37475=DIRECTION ( 'NONE',  ( -0.5364919789714478471, 0.6444004775717705469, -0.5449076811759709926 ) ) ;
#37476=CARTESIAN_POINT ( 'NONE',  ( -18.58927644294745107, 0.000000000000000000, 4.675741077920016586 ) ) ;
#37477=VECTOR ( 'NONE', #23654, 1000.000000000000114 ) ;
#37478=AXIS2_PLACEMENT_3D ( 'NONE', #52399, #30813, #9220 ) ;
#37479=ORIENTED_EDGE ( 'NONE', *, *, #22957, .T. ) ;
#37480=DIRECTION ( 'NONE',  ( -0.7660212471507179544, -0.6427876096865405842, -0.005961354470445141482 ) ) ;
#37481=EDGE_CURVE ( 'NONE', #9006, #32205, #53258, .T. ) ;
#37482=AXIS2_PLACEMENT_3D ( 'NONE', #11055, #24145, #15591 ) ;
#37483=DIRECTION ( 'NONE',  ( -0.005002170337468016433, -0.7660444431189770143, 0.6427681459581293666 ) ) ;
#37484=AXIS2_PLACEMENT_3D ( 'NONE', #1049, #23754, #11257 ) ;
#37485=EDGE_LOOP ( 'NONE', ( #35781, #37479, #27932, #20848 ) ) ;
#37486=CARTESIAN_POINT ( 'NONE',  ( -9.495214795699244092, 0.000000000000000000, 4.577187154869228891 ) ) ;
#37487=DIRECTION ( 'NONE',  ( 0.2426528472758542054, 0.7422098413412800966, 0.6246952433987894571 ) ) ;
#37488=DIRECTION ( 'NONE',  ( -0.8531650599175529814, -0.4028455766673920135, 0.3313982828793697877 ) ) ;
#37489=ORIENTED_EDGE ( 'NONE', *, *, #6975, .F. ) ;
#37490=ADVANCED_FACE ( 'NONE', ( #36457 ), #53771, .F. ) ;
#37491=LINE ( 'NONE', #55655, #31044 ) ;
#37492=PLANE ( 'NONE',  #29625 ) ;
#37493=CARTESIAN_POINT ( 'NONE',  ( -12.16996096287794060, 0.4483081953215045656, 1.394854484504827852 ) ) ;
#37494=CARTESIAN_POINT ( 'NONE',  ( -13.07066190154808361, 0.000000000000000000, 12.04713590736729678 ) ) ;
#37495=ADVANCED_FACE ( 'NONE', ( #55182 ), #28214, .F. ) ;
#37496=CARTESIAN_POINT ( 'NONE',  ( -17.47832216281435436, -2.189961127332303636, 12.64592903418461667 ) ) ;
#37497=DIRECTION ( 'NONE',  ( 0.007781995580012663651, 0.000000000000000000, -0.9999697198139515519 ) ) ;
#37498=ADVANCED_FACE ( 'NONE', ( #7775 ), #11473, .F. ) ;
#37500=AXIS2_PLACEMENT_3D ( 'NONE', #51244, #12360, #4941 ) ;
#37501=ORIENTED_EDGE ( 'NONE', *, *, #44079, .F. ) ;
#37502=CARTESIAN_POINT ( 'NONE',  ( -18.29747203306047609, -0.1191753592594177458, 14.03778604627889059 ) ) ;
#37503=CARTESIAN_POINT ( 'NONE',  ( -18.86354292863559579, 0.000000000000000000, 14.21804678658176080 ) ) ;
#37504=DIRECTION ( 'NONE',  ( 0.000000000000000000, -0.000000000000000000, -1.000000000000000000 ) ) ;
#37505=ORIENTED_EDGE ( 'NONE', *, *, #12597, .T. ) ;
#37506=CARTESIAN_POINT ( 'NONE',  ( -9.542064456761055524, 0.000000000000000000, 10.59726798936431180 ) ) ;
#37507=EDGE_CURVE ( 'NONE', #24035, #19370, #42114, .T. ) ;
#37508=DIRECTION ( 'NONE',  ( -0.5364919789714478471, 0.6444004775717705469, -0.5449076811759709926 ) ) ;
#37509=VECTOR ( 'NONE', #16385, 1000.000000000000227 ) ;
#37510=EDGE_CURVE ( 'NONE', #30294, #16295, #24254, .T. ) ;
#37511=LINE ( 'NONE', #33535, #14070 ) ;
#37512=VECTOR ( 'NONE', #21829, 999.9999999999998863 ) ;
#37513=DIRECTION ( 'NONE',  ( -0.005002170337468016433, -0.7660444431189770143, 0.6427681459581293666 ) ) ;
#37514=EDGE_CURVE ( 'NONE', #23008, #29351, #20553, .T. ) ;
#37516=ORIENTED_EDGE ( 'NONE', *, *, #48619, .T. ) ;
#37517=ORIENTED_EDGE ( 'NONE', *, *, #41880, .T. ) ;
#37518=CARTESIAN_POINT ( 'NONE',  ( 2.072287782118878319, 0.000000000000000000, -2.950529333540147015 ) ) ;
#37519=AXIS2_PLACEMENT_3D ( 'NONE', #41528, #6595, #44956 ) ;
#37520=VECTOR ( 'NONE', #38627, 999.9999999999998863 ) ;
#37521=CARTESIAN_POINT ( 'NONE',  ( -27.99923088623136636, 0.000000000000000000, 7.757173251277078130 ) ) ;
#37522=EDGE_CURVE ( 'NONE', #30961, #32780, #28797, .T. ) ;
#37523=ORIENTED_EDGE ( 'NONE', *, *, #2846, .T. ) ;
#37524=DIRECTION ( 'NONE',  ( 0.007781995580012663651, -3.146120232559066537E-19, -0.9999697198139514409 ) ) ;
#37525=VERTEX_POINT ( 'NONE', #16015 ) ;
#37526=CARTESIAN_POINT ( 'NONE',  ( -16.33317936670417225, 0.000000000000000000, 13.31440848639340224 ) ) ;
#37527=ADVANCED_FACE ( 'NONE', ( #16272 ), #2913, .F. ) ;
#37528=VECTOR ( 'NONE', #53293, 1000.000000000000227 ) ;
#37529=VERTEX_POINT ( 'NONE', #33591 ) ;
#37530=VECTOR ( 'NONE', #21172, 1000.000000000000227 ) ;
#37531=ORIENTED_EDGE ( 'NONE', *, *, #43167, .F. ) ;
#37532=LINE ( 'NONE', #54851, #48299 ) ;
#37533=DIRECTION ( 'NONE',  ( 0.6427681459581294776, -0.7660444431189769032, 0.005002170337467562802 ) ) ;
#37534=LINE ( 'NONE', #42913, #24838 ) ;
#37535=ORIENTED_EDGE ( 'NONE', *, *, #38186, .F. ) ;
#37536=CARTESIAN_POINT ( 'NONE',  ( -15.60102546347950536, 0.000000000000000000, 12.95077420755565356 ) ) ;
#37537=ORIENTED_EDGE ( 'NONE', *, *, #51742, .F. ) ;
#37538=ORIENTED_EDGE ( 'NONE', *, *, #11740, .F. ) ;
#37539=ORIENTED_EDGE ( 'NONE', *, *, #33426, .F. ) ;
#37540=CARTESIAN_POINT ( 'NONE',  ( -12.60458797795435615, 0.000000000000000000, 11.86609696750642229 ) ) ;
#37541=AXIS2_PLACEMENT_3D ( 'NONE', #19932, #32466, #28174 ) ;
#37542=DIRECTION ( 'NONE',  ( -0.3313982828793700652, 0.4028455766673916250, -0.8531650599175529814 ) ) ;
#37543=ORIENTED_EDGE ( 'NONE', *, *, #7293, .T. ) ;
#37544=CARTESIAN_POINT ( 'NONE',  ( -19.60990026154428278, 0.000000000000000000, 4.498472333781370125 ) ) ;
#37545=ORIENTED_EDGE ( 'NONE', *, *, #44136, .F. ) ;
#37546=VECTOR ( 'NONE', #19768, 1000.000000000000227 ) ;
#37547=DIRECTION ( 'NONE',  ( 0.007781995580012662783, 0.000000000000000000, -0.9999697198139514409 ) ) ;
#37548=LINE ( 'NONE', #10629, #43135 ) ;
#37549=ORIENTED_EDGE ( 'NONE', *, *, #19110, .T. ) ;
#37550=DIRECTION ( 'NONE',  ( 0.000000000000000000, -0.000000000000000000, -1.000000000000000000 ) ) ;
#37551=EDGE_CURVE ( 'NONE', #27150, #41291, #29342, .T. ) ;
#37552=AXIS2_PLACEMENT_3D ( 'NONE', #35686, #18650, #45060 ) ;
#37553=EDGE_LOOP ( 'NONE', ( #20111, #25628, #16829, #26508 ) ) ;
#37554=DIRECTION ( 'NONE',  ( 0.000000000000000000, -1.000000000000000000, 0.000000000000000000 ) ) ;
#37555=DIRECTION ( 'NONE',  ( -0.6427681459581293666, -0.7660444431189770143, -0.005002170337467561935 ) ) ;
#37556=DIRECTION ( 'NONE',  ( -0.005961354470445682716, -0.6427876096865404731, 0.7660212471507180654 ) ) ;
#37559=AXIS2_PLACEMENT_3D ( 'NONE', #16368, #29452, #25207 ) ;
#37560=DIRECTION ( 'NONE',  ( -0.005002170337468016433, -0.7660444431189770143, 0.6427681459581293666 ) ) ;
#37561=ORIENTED_EDGE ( 'NONE', *, *, #45231, .F. ) ;
#37562=ADVANCED_FACE ( 'NONE', ( #45816 ), #42414, .F. ) ;
#37563=EDGE_CURVE ( 'NONE', #8639, #51306, #7472, .T. ) ;
#37564=VECTOR ( 'NONE', #24496, 1000.000000000000227 ) ;
#37565=ORIENTED_EDGE ( 'NONE', *, *, #54137, .F. ) ;
#37566=CARTESIAN_POINT ( 'NONE',  ( -18.67619601524082285, 0.000000000000000000, 3.936400510096834893 ) ) ;
#37567=FACE_OUTER_BOUND ( 'NONE', #36089, .T. ) ;
#37568=CARTESIAN_POINT ( 'NONE',  ( -16.76677389676250485, 0.000000000000000000, 9.321915108048015597 ) ) ;
#37569=DIRECTION ( 'NONE',  ( -0.9999697198139514409, -0.000000000000000000, -0.007781995580013368816 ) ) ;
#37570=CARTESIAN_POINT ( 'NONE',  ( -14.76962374716334381, 2.391131607591507446, 6.542598890781153642 ) ) ;
#37571=EDGE_CURVE ( 'NONE', #1588, #24466, #11172, .T. ) ;
#37572=VECTOR ( 'NONE', #41904, 999.9999999999998863 ) ;
#37574=DIRECTION ( 'NONE',  ( 0.007781995580012662783, 0.000000000000000000, -0.9999697198139514409 ) ) ;
#37575=ORIENTED_EDGE ( 'NONE', *, *, #49354, .F. ) ;
#37576=CARTESIAN_POINT ( 'NONE',  ( -9.306717065757585061, 0.000000000000000000, 6.055982367016289558 ) ) ;
#37577=LINE ( 'NONE', #50901, #7822 ) ;
#37578=ORIENTED_EDGE ( 'NONE', *, *, #22396, .T. ) ;
#37579=FACE_OUTER_BOUND ( 'NONE', #51850, .T. ) ;
#37580=DIRECTION ( 'NONE',  ( -0.5449076811759708816, 0.6444004775717707689, 0.5364919789714475140 ) ) ;
#37581=ORIENTED_EDGE ( 'NONE', *, *, #15012, .T. ) ;
#37582=FACE_OUTER_BOUND ( 'NONE', #19586, .T. ) ;
#37583=PLANE ( 'NONE',  #47796 ) ;
#37584=EDGE_CURVE ( 'NONE', #52222, #9654, #38132, .T. ) ;
#37585=CARTESIAN_POINT ( 'NONE',  ( -21.47419595591918906, 0.000000000000000000, 5.222628093224860102 ) ) ;
#37586=LINE ( 'NONE', #16022, #3291 ) ;
#37587=EDGE_CURVE ( 'NONE', #12202, #40957, #46655, .T. ) ;
#37588=DIRECTION ( 'NONE',  ( 0.007781995580012663651, 0.000000000000000000, -0.9999697198139515519 ) ) ;
#37589=VECTOR ( 'NONE', #49436, 1000.000000000000227 ) ;
#37590=ORIENTED_EDGE ( 'NONE', *, *, #50534, .F. ) ;
#37591=ORIENTED_EDGE ( 'NONE', *, *, #4202, .T. ) ;
#37592=AXIS2_PLACEMENT_3D ( 'NONE', #23037, #39532, #27283 ) ;
#37593=EDGE_CURVE ( 'NONE', #47675, #6779, #50645, .T. ) ;
#37595=CARTESIAN_POINT ( 'NONE',  ( -20.53709881633460199, 3.686347215771508257, 10.90855154352876255 ) ) ;
#37596=CARTESIAN_POINT ( 'NONE',  ( -20.54204810873173415, 0.000000000000000000, 4.860550213503115558 ) ) ;
#37597=VECTOR ( 'NONE', #36672, 1000.000000000000000 ) ;
#37598=PLANE ( 'NONE',  #27870 ) ;
#37599=EDGE_CURVE ( 'NONE', #17866, #15410, #19713, .T. ) ;
#37600=CARTESIAN_POINT ( 'NONE',  ( -18.35205637073270069, 0.000000000000000000, 8.201581863854691790 ) ) ;
#37601=CARTESIAN_POINT ( 'NONE',  ( -18.79789254742608406, 0.000000000000000000, 5.782113788577308178 ) ) ;
#37602=ORIENTED_EDGE ( 'NONE', *, *, #2922, .F. ) ;
#37603=CARTESIAN_POINT ( 'NONE',  ( -13.50413705924304963, 0.000000000000000000, 8.039303436688003401 ) ) ;
#37604=CARTESIAN_POINT ( 'NONE',  ( -16.81190032086591302, 0.000000000000000000, 3.212244750653343583 ) ) ;
#37605=DIRECTION ( 'NONE',  ( 0.000000000000000000, -0.000000000000000000, -1.000000000000000000 ) ) ;
#37606=VECTOR ( 'NONE', #6178, 1000.000000000000227 ) ;
#37607=VERTEX_POINT ( 'NONE', #32749 ) ;
#37608=VECTOR ( 'NONE', #26584, 1000.000000000000227 ) ;
#37610=CARTESIAN_POINT ( 'NONE',  ( -16.99924723426068951, 0.000000000000000000, 13.49389102713827171 ) ) ;
#37611=CARTESIAN_POINT ( 'NONE',  ( -33.59133976979808978, -0.1191753592594197858, 9.829643557626155825 ) ) ;
#37612=VECTOR ( 'NONE', #17964, 1000.000000000000000 ) ;
#37613=ORIENTED_EDGE ( 'NONE', *, *, #2880, .T. ) ;
#37614=FACE_OUTER_BOUND ( 'NONE', #29469, .T. ) ;
#37615=ORIENTED_EDGE ( 'NONE', *, *, #54801, .T. ) ;
#37616=AXIS2_PLACEMENT_3D ( 'NONE', #3242, #12338, #4084 ) ;
#37617=ORIENTED_EDGE ( 'NONE', *, *, #22904, .F. ) ;
#37618=VECTOR ( 'NONE', #22573, 1000.000000000000227 ) ;
#37619=EDGE_LOOP ( 'NONE', ( #34879, #14525, #41572, #44466 ) ) ;
#37620=ORIENTED_EDGE ( 'NONE', *, *, #18337, .F. ) ;
#37621=FACE_OUTER_BOUND ( 'NONE', #23743, .T. ) ;
#37622=ORIENTED_EDGE ( 'NONE', *, *, #40133, .F. ) ;
#37623=EDGE_CURVE ( 'NONE', #51697, #55458, #50059, .T. ) ;
#37624=ORIENTED_EDGE ( 'NONE', *, *, #16123, .T. ) ;
#37625=CARTESIAN_POINT ( 'NONE',  ( -15.92694207790892946, 5.467268677019013978, 2.694062420689476767 ) ) ;
#37626=ORIENTED_EDGE ( 'NONE', *, *, #51522, .F. ) ;
#37627=ADVANCED_FACE ( 'NONE', ( #29056 ), #46357, .F. ) ;
#37628=EDGE_CURVE ( 'NONE', #17269, #17866, #8613, .T. ) ;
#37629=VERTEX_POINT ( 'NONE', #12593 ) ;
#37630=VECTOR ( 'NONE', #5972, 999.9999999999998863 ) ;
#37631=DIRECTION ( 'NONE',  ( 0.7660212471507180654, -0.6427876096865404731, 0.005961354470445141482 ) ) ;
#37632=CARTESIAN_POINT ( 'NONE',  ( -11.36876430285300543, 2.229229656569007290, 4.955880904987684410 ) ) ;
#37633=EDGE_CURVE ( 'NONE', #38023, #55289, #12313, .T. ) ;
#37634=DIRECTION ( 'NONE',  ( 0.5449076811759707706, 0.6444004775717708799, -0.5364919789714476250 ) ) ;
#37635=LINE ( 'NONE', #28847, #33211 ) ;
#37637=VECTOR ( 'NONE', #14053, 1000.000000000000227 ) ;
#37639=ADVANCED_FACE ( 'NONE', ( #3768 ), #17130, .F. ) ;
#37640=ADVANCED_FACE ( 'NONE', ( #8316 ), #34717, .F. ) ;
#37641=EDGE_CURVE ( 'NONE', #33817, #18318, #33882, .T. ) ;
#37642=ORIENTED_EDGE ( 'NONE', *, *, #30136, .F. ) ;
#37643=CARTESIAN_POINT ( 'NONE',  ( -16.03306359442184004, 0.000000000000000000, 8.758286885247480669 ) ) ;
#37644=DIRECTION ( 'NONE',  ( 0.005961354470445682716, -0.6427876096865404731, -0.7660212471507180654 ) ) ;
#37645=VECTOR ( 'NONE', #44536, 999.9999999999998863 ) ;
#37646=EDGE_CURVE ( 'NONE', #3673, #16343, #55743, .T. ) ;
#37648=AXIS2_PLACEMENT_3D ( 'NONE', #1222, #5496, #30790 ) ;
#37651=AXIS2_PLACEMENT_3D ( 'NONE', #12909, #30239, #19908 ) ;
#37652=DIRECTION ( 'NONE',  ( 0.007781995580012663651, 0.000000000000000000, -0.9999697198139515519 ) ) ;
#37653=DIRECTION ( 'NONE',  ( 0.7660212471507180654, -0.6427876096865404731, 0.005961354470445141482 ) ) ;
#37654=ORIENTED_EDGE ( 'NONE', *, *, #45221, .F. ) ;
#37655=DIRECTION ( 'NONE',  ( 0.7660212471507180654, -0.6427876096865404731, 0.005961354470445141482 ) ) ;
#37656=ORIENTED_EDGE ( 'NONE', *, *, #42270, .F. ) ;
#37657=VECTOR ( 'NONE', #20393, 999.9999999999998863 ) ;
#37658=LINE ( 'NONE', #44845, #6212 ) ;
#37659=CARTESIAN_POINT ( 'NONE',  ( 2.072287782118878319, 0.000000000000000000, -2.950529333540147015 ) ) ;
#37660=DIRECTION ( 'NONE',  ( -0.6427681459581293666, -0.7660444431189770143, -0.005002170337467561935 ) ) ;
#37661=LINE ( 'NONE', #28866, #2712 ) ;
#37662=EDGE_CURVE ( 'NONE', #2943, #35066, #46954, .T. ) ;
#37663=FACE_OUTER_BOUND ( 'NONE', #22345, .T. ) ;
#37664=LINE ( 'NONE', #42739, #44969 ) ;
#37665=VECTOR ( 'NONE', #27853, 999.9999999999998863 ) ;
#37666=EDGE_CURVE ( 'NONE', #18658, #29145, #21674, .T. ) ;
#37667=EDGE_LOOP ( 'NONE', ( #42506, #48262, #54902, #21568 ) ) ;
#37668=VECTOR ( 'NONE', #11674, 1000.000000000000227 ) ;
#37670=ORIENTED_EDGE ( 'NONE', *, *, #522, .T. ) ;
#37671=EDGE_CURVE ( 'NONE', #8156, #20135, #38418, .T. ) ;
#37672=DIRECTION ( 'NONE',  ( 0.5364919789714477361, 0.6444004775717706579, 0.5449076811759711036 ) ) ;
#37673=CARTESIAN_POINT ( 'NONE',  ( -21.20308440300454933, -1.975113310420657520, 8.159427204713791681 ) ) ;
#37674=DIRECTION ( 'NONE',  ( 0.005002170337468016433, -0.7660444431189770143, -0.6427681459581293666 ) ) ;
#37675=ADVANCED_FACE ( 'NONE', ( #29911 ), #47210, .F. ) ;
#37676=CARTESIAN_POINT ( 'NONE',  ( -14.94838282604900748, -0.1191753592594197858, 2.588085963191248506 ) ) ;
#37677=PLANE ( 'NONE',  #9448 ) ;
#37679=DIRECTION ( 'NONE',  ( 0.9999697198139515519, 0.000000000000000000, 0.007781995580013368816 ) ) ;
#37680=EDGE_CURVE ( 'NONE', #39457, #24901, #38727, .T. ) ;
#37681=AXIS2_PLACEMENT_3D ( 'NONE', #6726, #2469, #7024 ) ;
#37682=CARTESIAN_POINT ( 'NONE',  ( -18.67775241435682432, 0.000000000000000000, 4.136394454059623804 ) ) ;
#37683=VECTOR ( 'NONE', #52630, 1000.000000000000227 ) ;
#37684=LINE ( 'NONE', #55006, #54621 ) ;
#37685=ORIENTED_EDGE ( 'NONE', *, *, #52269, .F. ) ;
#37686=AXIS2_PLACEMENT_3D ( 'NONE', #28279, #49611, #36527 ) ;
#37687=ORIENTED_EDGE ( 'NONE', *, *, #30145, .T. ) ;
#37688=VECTOR ( 'NONE', #27171, 999.9999999999998863 ) ;
#37689=ORIENTED_EDGE ( 'NONE', *, *, #42777, .F. ) ;
#37690=ORIENTED_EDGE ( 'NONE', *, *, #25851, .T. ) ;
#37691=VECTOR ( 'NONE', #30460, 1000.000000000000114 ) ;
#37692=VECTOR ( 'NONE', #43451, 1000.000000000000227 ) ;
#37693=EDGE_LOOP ( 'NONE', ( #1108, #35677, #14634, #38289 ) ) ;
#37694=ORIENTED_EDGE ( 'NONE', *, *, #39261, .T. ) ;
#37695=DIRECTION ( 'NONE',  ( 0.007781995580012663651, 0.000000000000000000, -0.9999697198139515519 ) ) ;
#37697=CARTESIAN_POINT ( 'NONE',  ( -24.27063949748155380, 0.000000000000000000, 6.308861732390097288 ) ) ;
#37698=VECTOR ( 'NONE', #6948, 999.9999999999998863 ) ;
#37699=VECTOR ( 'NONE', #51592, 1000.000000000000227 ) ;
#37700=EDGE_LOOP ( 'NONE', ( #11220, #35985, #29001, #35991 ) ) ;
#37701=LINE ( 'NONE', #28055, #2276 ) ;
#37702=VECTOR ( 'NONE', #3644, 1000.000000000000227 ) ;
#37703=EDGE_LOOP ( 'NONE', ( #47052, #33153, #38734, #32923 ) ) ;
#37706=VECTOR ( 'NONE', #43062, 999.9999999999998863 ) ;
#37707=AXIS2_PLACEMENT_3D ( 'NONE', #42199, #25431, #29726 ) ;
#37709=DIRECTION ( 'NONE',  ( -0.005002170337468016433, -0.7660444431189770143, 0.6427681459581293666 ) ) ;
#37710=CARTESIAN_POINT ( 'NONE',  ( -9.286598691220605772, 0.000000000000000000, 3.470814444211937300 ) ) ;
#37711=VERTEX_POINT ( 'NONE', #17532 ) ;
#37712=PLANE ( 'NONE',  #16496 ) ;
#37713=ORIENTED_EDGE ( 'NONE', *, *, #30885, .F. ) ;
#37714=EDGE_CURVE ( 'NONE', #50596, #47675, #12145, .T. ) ;
#37715=ADVANCED_FACE ( 'NONE', ( #39108 ), #16990, .F. ) ;
#37716=DIRECTION ( 'NONE',  ( 0.007781995580012663651, -3.146120232559066537E-19, -0.9999697198139514409 ) ) ;
#37717=LINE ( 'NONE', #42528, #41118 ) ;
#37718=EDGE_CURVE ( 'NONE', #21088, #31624, #7916, .T. ) ;
#37719=VECTOR ( 'NONE', #45217, 999.9999999999998863 ) ;
#37720=DIRECTION ( 'NONE',  ( 0.6427681459581294776, -0.7660444431189769032, 0.005002170337467562802 ) ) ;
#37721=FACE_OUTER_BOUND ( 'NONE', #44277, .T. ) ;
#37722=FACE_OUTER_BOUND ( 'NONE', #5461, .T. ) ;
#37723=DIRECTION ( 'NONE',  ( -0.7660212471507179544, -0.6427876096865405842, -0.005961354470445141482 ) ) ;
#37724=CARTESIAN_POINT ( 'NONE',  ( -26.13337879274045505, 0.000000000000000000, 6.833023547870798353 ) ) ;
#37725=CARTESIAN_POINT ( 'NONE',  ( -19.71854418059240643, 0.000000000000000000, 4.666952855267993527 ) ) ;
#37726=ORIENTED_EDGE ( 'NONE', *, *, #12521, .T. ) ;
#37727=CARTESIAN_POINT ( 'NONE',  ( -14.15307997813123286, 0.000000000000000000, 6.018266850220190811 ) ) ;
#37728=EDGE_LOOP ( 'NONE', ( #12362, #37812, #22492, #27923 ) ) ;
#37729=VECTOR ( 'NONE', #28794, 1000.000000000000000 ) ;
#37730=PLANE ( 'NONE',  #33803 ) ;
#37731=LINE ( 'NONE', #24942, #19655 ) ;
#37732=LINE ( 'NONE', #54745, #35037 ) ;
#37734=CARTESIAN_POINT ( 'NONE',  ( -8.638865104681501705, 0.000000000000000000, 4.753177479762371149 ) ) ;
#37735=DIRECTION ( 'NONE',  ( -0.8531650599175529814, -0.4028455766673920135, 0.3313982828793697877 ) ) ;
#37736=VECTOR ( 'NONE', #23543, 1000.000000000000227 ) ;
#37737=CARTESIAN_POINT ( 'NONE',  ( -14.41772293100952673, 0.000000000000000000, 6.016207337568184599 ) ) ;
#37738=VECTOR ( 'NONE', #40976, 1000.000000000000227 ) ;
#37740=EDGE_LOOP ( 'NONE', ( #49741, #17805, #20849, #8410 ) ) ;
#37741=CARTESIAN_POINT ( 'NONE',  ( -12.23851102634202448, -0.1191753592594197858, 11.68427982808754884 ) ) ;
#37742=LINE ( 'NONE', #50215, #6697 ) ;
#37743=DIRECTION ( 'NONE',  ( -0.9999697198139514409, -0.000000000000000000, -0.007781995580013368816 ) ) ;
#37744=CARTESIAN_POINT ( 'NONE',  ( -15.80386756661275882, 1.419719901456505395, 5.350082209620479645 ) ) ;
#37745=VECTOR ( 'NONE', #35999, 1000.000000000000227 ) ;
#37746=CARTESIAN_POINT ( 'NONE',  ( -19.89215662524663841, -2.622721114510659035, 8.713053072339743466 ) ) ;
#37747=VECTOR ( 'NONE', #49901, 1000.000000000000227 ) ;
#37748=PLANE ( 'NONE',  #16438 ) ;
#37749=CARTESIAN_POINT ( 'NONE',  ( -26.13493519185646008, 0.000000000000000000, 7.033017491833586377 ) ) ;
#37750=ADVANCED_FACE ( 'NONE', ( #34309 ), #12715, .F. ) ;
#37751=CARTESIAN_POINT ( 'NONE',  ( -19.45503627000849889, -1.000000000000000000, 7.556996783084074742 ) ) ;
#37752=CARTESIAN_POINT ( 'NONE',  ( -11.14514627858494755, 0.000000000000000000, 3.456350797139899900 ) ) ;
#37754=AXIS2_PLACEMENT_3D ( 'NONE', #5425, #1136, #39515 ) ;
#37755=VECTOR ( 'NONE', #35637, 1000.000000000000114 ) ;
#37756=DIRECTION ( 'NONE',  ( 0.6427681459581294776, -0.7660444431189769032, 0.005002170337467562802 ) ) ;
#37757=CARTESIAN_POINT ( 'NONE',  ( -14.46888367232926420, 0.000000000000000000, 12.59025272694991315 ) ) ;
#37758=EDGE_LOOP ( 'NONE', ( #44750, #4854, #24992, #21833, #7646 ) ) ;
#37760=ORIENTED_EDGE ( 'NONE', *, *, #46659, .T. ) ;
#37761=DIRECTION ( 'NONE',  ( -0.005961354470445682716, -0.6427876096865404731, 0.7660212471507180654 ) ) ;
#37762=EDGE_CURVE ( 'NONE', #21477, #2866, #30321, .T. ) ;
#37763=VERTEX_POINT ( 'NONE', #13293 ) ;
#37764=EDGE_CURVE ( 'NONE', #33896, #50554, #55299, .T. ) ;
#37765=EDGE_LOOP ( 'NONE', ( #40123, #10391, #52603, #10597, #31543 ) ) ;
#37766=DIRECTION ( 'NONE',  ( 0.5449076811759707706, 0.6444004775717708799, -0.5364919789714476250 ) ) ;
#37767=AXIS2_PLACEMENT_3D ( 'NONE', #36480, #35965, #36783 ) ;
#37768=ORIENTED_EDGE ( 'NONE', *, *, #56043, .F. ) ;
#37769=ORIENTED_EDGE ( 'NONE', *, *, #52201, .F. ) ;
#37770=VERTEX_POINT ( 'NONE', #51034 ) ;
#37771=FACE_OUTER_BOUND ( 'NONE', #36427, .T. ) ;
#37772=DIRECTION ( 'NONE',  ( 0.9999697198139515519, 0.000000000000000000, 0.007781995580013368816 ) ) ;
#37773=VECTOR ( 'NONE', #13374, 1000.000000000000227 ) ;
#37774=CARTESIAN_POINT ( 'NONE',  ( -12.15116108492864377, 0.000000000000000000, 1.401855352044617975 ) ) ;
#37775=AXIS2_PLACEMENT_3D ( 'NONE', #51512, #12605, #1497 ) ;
#37776=ORIENTED_EDGE ( 'NONE', *, *, #3863, .F. ) ;
#37777=VERTEX_POINT ( 'NONE', #25230 ) ;
#37778=AXIS2_PLACEMENT_3D ( 'NONE', #14138, #27760, #48782 ) ;
#37779=PLANE ( 'NONE',  #35745 ) ;
#37780=PLANE ( 'NONE',  #54452 ) ;
#37781=VERTEX_POINT ( 'NONE', #34023 ) ;
#37782=FACE_OUTER_BOUND ( 'NONE', #27208, .T. ) ;
#37783=EDGE_LOOP ( 'NONE', ( #15377, #28957, #11825, #24339 ) ) ;
#37784=LINE ( 'NONE', #12203, #52057 ) ;
#37786=EDGE_CURVE ( 'NONE', #223, #31183, #51344, .T. ) ;
#37787=ORIENTED_EDGE ( 'NONE', *, *, #9856, .T. ) ;
#37788=VECTOR ( 'NONE', #34241, 1000.000000000000000 ) ;
#37789=DIRECTION ( 'NONE',  ( -0.005002170337468016433, -0.7660444431189770143, 0.6427681459581293666 ) ) ;
#37790=EDGE_CURVE ( 'NONE', #14283, #49510, #21227, .T. ) ;
#37791=EDGE_CURVE ( 'NONE', #16476, #46316, #39694, .T. ) ;
#37792=VECTOR ( 'NONE', #34539, 1000.000000000000000 ) ;
#37793=PLANE ( 'NONE',  #22748 ) ;
#37794=VECTOR ( 'NONE', #45212, 999.9999999999998863 ) ;
#37795=VERTEX_POINT ( 'NONE', #44772 ) ;
#37796=PLANE ( 'NONE',  #14061 ) ;
#37797=CARTESIAN_POINT ( 'NONE',  ( -16.30058060080541082, 0.000000000000000000, 9.125537075853236146 ) ) ;
#37798=ORIENTED_EDGE ( 'NONE', *, *, #30277, .T. ) ;
#37799=DIRECTION ( 'NONE',  ( 0.005002170337468016433, -0.7660444431189770143, -0.6427681459581293666 ) ) ;
#37800=DIRECTION ( 'NONE',  ( 0.000000000000000000, -1.000000000000000000, 0.000000000000000000 ) ) ;
#37801=CARTESIAN_POINT ( 'NONE',  ( -12.24986416390947497, 2.714935509636507316, 6.095256065150636893 ) ) ;
#37802=FACE_OUTER_BOUND ( 'NONE', #8343, .T. ) ;
#37803=DIRECTION ( 'NONE',  ( 0.007781995580012663651, -3.146120232559066537E-19, -0.9999697198139514409 ) ) ;
#37804=DIRECTION ( 'NONE',  ( -0.5449076811759708816, 0.6444004775717707689, 0.5364919789714475140 ) ) ;
#37805=VECTOR ( 'NONE', #31525, 999.9999999999998863 ) ;
#37806=EDGE_CURVE ( 'NONE', #36112, #883, #35702, .T. ) ;
#37807=PLANE ( 'NONE',  #13214 ) ;
#37808=VERTEX_POINT ( 'NONE', #36010 ) ;
#37809=PLANE ( 'NONE',  #832 ) ;
#37810=CARTESIAN_POINT ( 'NONE',  ( -1.086233639165236964, 0.000000000000000000, -2.796443541562362078 ) ) ;
#37812=ORIENTED_EDGE ( 'NONE', *, *, #28827, .F. ) ;
#37813=LINE ( 'NONE', #28730, #11135 ) ;
#37814=CARTESIAN_POINT ( 'NONE',  ( -9.762731802082821986, 0.000000000000000000, 4.944437345474987033 ) ) ;
#37815=AXIS2_PLACEMENT_3D ( 'NONE', #4446, #43600, #44187 ) ;
#37816=CARTESIAN_POINT ( 'NONE',  ( -12.33850799832341849, 0.000000000000000000, 11.68350162852954632 ) ) ;
#37817=CARTESIAN_POINT ( 'NONE',  ( -27.99767448711536133, 0.000000000000000000, 7.557179307314289218 ) ) ;
#37818=PLANE ( 'NONE',  #12961 ) ;
#37819=ORIENTED_EDGE ( 'NONE', *, *, #33961, .F. ) ;
#37820=AXIS2_PLACEMENT_3D ( 'NONE', #44423, #31927, #53777 ) ;
#37821=VERTEX_POINT ( 'NONE', #53019 ) ;
#37822=CARTESIAN_POINT ( 'NONE',  ( -10.84028925556084388, -0.1191753592594197858, 11.14116300850493246 ) ) ;
#37823=CARTESIAN_POINT ( 'NONE',  ( -19.64439698464071427, -1.813211359398158029, 4.454021096977195171 ) ) ;
#37825=ORIENTED_EDGE ( 'NONE', *, *, #34815, .T. ) ;
#37826=DIRECTION ( 'NONE',  ( -0.005961354470445682716, -0.6427876096865404731, 0.7660212471507180654 ) ) ;
#37827=EDGE_CURVE ( 'NONE', #32241, #8639, #9286, .T. ) ;
#37828=VERTEX_POINT ( 'NONE', #27174 ) ;
#37829=LINE ( 'NONE', #29595, #29288 ) ;
#37830=AXIS2_PLACEMENT_3D ( 'NONE', #20760, #45465, #38074 ) ;
#37831=ORIENTED_EDGE ( 'NONE', *, *, #39299, .T. ) ;
#37832=ORIENTED_EDGE ( 'NONE', *, *, #18874, .F. ) ;
#37833=ORIENTED_EDGE ( 'NONE', *, *, #46363, .T. ) ;
#37834=CARTESIAN_POINT ( 'NONE',  ( -9.110551994824897193, -1.000000000000000000, 3.538847790438064411 ) ) ;
#37835=CARTESIAN_POINT ( 'NONE',  ( -12.54899678401333496, 0.000000000000000000, 4.722747930904141356 ) ) ;
#37836=CARTESIAN_POINT ( 'NONE',  ( -10.80508224072880452, -0.1117717739994080611, 7.415434460100314595 ) ) ;
#37837=EDGE_CURVE ( 'NONE', #44124, #29311, #5587, .T. ) ;
#37838=DIRECTION ( 'NONE',  ( 0.5364919789714477361, 0.6444004775717706579, 0.5449076811759711036 ) ) ;
#37839=ORIENTED_EDGE ( 'NONE', *, *, #9176, .T. ) ;
#37840=ADVANCED_FACE ( 'NONE', ( #9872 ), #53319, .F. ) ;
#37841=EDGE_CURVE ( 'NONE', #22744, #51840, #22639, .T. ) ;
#37842=ORIENTED_EDGE ( 'NONE', *, *, #34492, .F. ) ;
#37844=LINE ( 'NONE', #37540, #48564 ) ;
#37845=LINE ( 'NONE', #16818, #5887 ) ;
#37846=ORIENTED_EDGE ( 'NONE', *, *, #42442, .T. ) ;
#37847=PLANE ( 'NONE',  #49310 ) ;
#37848=EDGE_CURVE ( 'NONE', #33592, #53425, #10428, .T. ) ;
#37849=ORIENTED_EDGE ( 'NONE', *, *, #16469, .T. ) ;
#37850=FACE_OUTER_BOUND ( 'NONE', #26705, .T. ) ;
#37851=CARTESIAN_POINT ( 'NONE',  ( -19.12962290826653700, 0.000000000000000000, 14.40064212555863854 ) ) ;
#37852=ORIENTED_EDGE ( 'NONE', *, *, #14215, .F. ) ;
#37853=ADVANCED_FACE ( 'NONE', ( #14133 ), #49028, .F. ) ;
#37854=LINE ( 'NONE', #33317, #22298 ) ;
#37856=EDGE_CURVE ( 'NONE', #20361, #38484, #1619, .T. ) ;
#37857=VECTOR ( 'NONE', #19981, 999.9999999999998863 ) ;
#37858=FACE_OUTER_BOUND ( 'NONE', #6821, .T. ) ;
#37859=DIRECTION ( 'NONE',  ( 0.9999697198139515519, 0.000000000000000000, 0.007781995580013368816 ) ) ;
#37860=CARTESIAN_POINT ( 'NONE',  ( 2.072287782118878319, 0.000000000000000000, -2.950529333540147015 ) ) ;
#37862=DIRECTION ( 'NONE',  ( 0.005961354470445682716, -0.6427876096865404731, -0.7660212471507180654 ) ) ;
#37863=FACE_OUTER_BOUND ( 'NONE', #32806, .T. ) ;
#37864=EDGE_LOOP ( 'NONE', ( #47330, #53670, #24660, #6865 ) ) ;
#37865=EDGE_CURVE ( 'NONE', #18631, #873, #773, .T. ) ;
#37866=VERTEX_POINT ( 'NONE', #27447 ) ;
#37867=AXIS2_PLACEMENT_3D ( 'NONE', #22570, #44412, #48699 ) ;
#37868=CARTESIAN_POINT ( 'NONE',  ( -12.61734217886482057, -3.432230869623162928, 1.672819171754234890 ) ) ;
#37869=LINE ( 'NONE', #46088, #13959 ) ;
#37871=LINE ( 'NONE', #20235, #36685 ) ;
#37872=LINE ( 'NONE', #11730, #15249 ) ;
#37873=EDGE_CURVE ( 'NONE', #21088, #49698, #14668, .T. ) ;
#37874=CARTESIAN_POINT ( 'NONE',  ( -14.66887761629205222, 0.000000000000000000, 12.58869632783390990 ) ) ;
#37875=ORIENTED_EDGE ( 'NONE', *, *, #47487, .T. ) ;
#37876=CARTESIAN_POINT ( 'NONE',  ( -15.06775173312542826, 5.467268677019012202, 11.70686692005663865 ) ) ;
#37877=CARTESIAN_POINT ( 'NONE',  ( -16.53317331066696383, 0.000000000000000000, 13.31285208727739899 ) ) ;
#37879=DIRECTION ( 'NONE',  ( 0.005961354470445682716, -0.6427876096865404731, -0.7660212471507180654 ) ) ;
#37880=ORIENTED_EDGE ( 'NONE', *, *, #526, .T. ) ;
#37882=DIRECTION ( 'NONE',  ( 0.007781995580012663651, -3.146120232559066537E-19, -0.9999697198139514409 ) ) ;
#37883=FACE_OUTER_BOUND ( 'NONE', #42078, .T. ) ;
#37884=DIRECTION ( 'NONE',  ( 0.005002170337468016433, -0.7660444431189770143, -0.6427681459581293666 ) ) ;
#37886=ORIENTED_EDGE ( 'NONE', *, *, #5637, .T. ) ;
#37887=ORIENTED_EDGE ( 'NONE', *, *, #38441, .T. ) ;
#37889=DIRECTION ( 'NONE',  ( -0.5449076811759708816, 0.6444004775717707689, 0.5364919789714475140 ) ) ;
#37890=CARTESIAN_POINT ( 'NONE',  ( -25.20123094555300369, 0.000000000000000000, 6.470945668149052032 ) ) ;
#37891=DIRECTION ( 'NONE',  ( -0.005002170337468016433, -0.7660444431189770143, 0.6427681459581293666 ) ) ;
#37892=CARTESIAN_POINT ( 'NONE',  ( -18.19747506107908563, 0.000000000000000000, 14.03856424583689311 ) ) ;
#37893=FACE_OUTER_BOUND ( 'NONE', #48669, .T. ) ;
#37894=EDGE_CURVE ( 'NONE', #48923, #37770, #23213, .T. ) ;
#37896=LINE ( 'NONE', #50666, #23815 ) ;
#37897=CARTESIAN_POINT ( 'NONE',  ( -20.49657252799461560, -2.784623065533158304, 9.213537418967975512 ) ) ;
#37898=LINE ( 'NONE', #29679, #42350 ) ;
#37899=VERTEX_POINT ( 'NONE', #18092 ) ;
#37900=FACE_OUTER_BOUND ( 'NONE', #43218, .T. ) ;
#37901=PLANE ( 'NONE',  #34773 ) ;
#37902=ORIENTED_EDGE ( 'NONE', *, *, #49650, .T. ) ;
#37903=VECTOR ( 'NONE', #24709, 1000.000000000000227 ) ;
#37904=LINE ( 'NONE', #54632, #36812 ) ;
#37905=ORIENTED_EDGE ( 'NONE', *, *, #33344, .T. ) ;
#37906=EDGE_CURVE ( 'NONE', #40238, #9638, #22073, .T. ) ;
#37907=ORIENTED_EDGE ( 'NONE', *, *, #54240, .F. ) ;
#37908=ORIENTED_EDGE ( 'NONE', *, *, #13920, .T. ) ;
#37909=ORIENTED_EDGE ( 'NONE', *, *, #30902, .F. ) ;
#37910=CARTESIAN_POINT ( 'NONE',  ( -15.40103151951671734, 0.000000000000000000, 12.95233060667165681 ) ) ;
#37911=ORIENTED_EDGE ( 'NONE', *, *, #46611, .T. ) ;
#37912=LINE ( 'NONE', #33627, #38535 ) ;
#37913=VERTEX_POINT ( 'NONE', #5330 ) ;
#37914=DIRECTION ( 'NONE',  ( -0.005002170337468016433, -0.7660444431189770143, 0.6427681459581293666 ) ) ;
#37915=EDGE_CURVE ( 'NONE', #8596, #42084, #52461, .T. ) ;
#37916=ORIENTED_EDGE ( 'NONE', *, *, #39402, .F. ) ;
#37917=ORIENTED_EDGE ( 'NONE', *, *, #27376, .F. ) ;
#37918=ADVANCED_FACE ( 'NONE', ( #26607 ), #30870, .F. ) ;
#37919=LINE ( 'NONE', #19757, #40278 ) ;
#37920=DIRECTION ( 'NONE',  ( -0.5449076811759708816, 0.6444004775717707689, 0.5364919789714475140 ) ) ;
#37921=CARTESIAN_POINT ( 'NONE',  ( -21.34570666360650293, 1.905425754524007198, 8.299846768392162843 ) ) ;
#37922=CARTESIAN_POINT ( 'NONE',  ( -12.53618291560292519, 0.000000000000000000, 3.076193358578107162 ) ) ;
#37923=CARTESIAN_POINT ( 'NONE',  ( -11.67244013076689946, 0.000000000000000000, 11.50401908778467863 ) ) ;
#37924=ORIENTED_EDGE ( 'NONE', *, *, #40433, .F. ) ;
#37925=EDGE_CURVE ( 'NONE', #19938, #27147, #9594, .T. ) ;
#37926=ORIENTED_EDGE ( 'NONE', *, *, #15073, .T. ) ;
#37927=DIRECTION ( 'NONE',  ( 0.6427681459581294776, -0.7660444431189769032, 0.005002170337467562802 ) ) ;
#37928=LINE ( 'NONE', #24858, #17616 ) ;
#37929=CARTESIAN_POINT ( 'NONE',  ( -13.21075357131192618, 0.000000000000000000, 4.348265916762363403 ) ) ;
#37930=ADVANCED_FACE ( 'NONE', ( #18364 ), #37349, .F. ) ;
#37931=PLANE ( 'NONE',  #15822 ) ;
#37932=FACE_OUTER_BOUND ( 'NONE', #28116, .T. ) ;
#37933=CARTESIAN_POINT ( 'NONE',  ( -11.82546504130451304, 0.000000000000000000, 5.467042761839684850 ) ) ;
#37934=ORIENTED_EDGE ( 'NONE', *, *, #19818, .F. ) ;
#37935=DIRECTION ( 'NONE',  ( -0.6427681459581293666, -0.7660444431189770143, -0.005002170337467561935 ) ) ;
#37936=CARTESIAN_POINT ( 'NONE',  ( -13.53673582514181106, 0.000000000000000000, 12.22817484722816772 ) ) ;
#37937=VERTEX_POINT ( 'NONE', #41364 ) ;
#37938=AXIS2_PLACEMENT_3D ( 'NONE', #49680, #15037, #3299 ) ;
#37939=DIRECTION ( 'NONE',  ( -0.7660212471507179544, -0.6427876096865405842, -0.005961354470445141482 ) ) ;
#37940=PLANE ( 'NONE',  #10596 ) ;
#37941=CARTESIAN_POINT ( 'NONE',  ( -29.86197018149027116, 0.000000000000000000, 8.281335066757780083 ) ) ;
#37942=FACE_OUTER_BOUND ( 'NONE', #26302, .T. ) ;
#37943=DIRECTION ( 'NONE',  ( -0.5364919789714478471, 0.6444004775717705469, -0.5449076811759709926 ) ) ;
#37944=ORIENTED_EDGE ( 'NONE', *, *, #38681, .T. ) ;
#37945=VERTEX_POINT ( 'NONE', #32560 ) ;
#37946=CARTESIAN_POINT ( 'NONE',  ( -16.53317331066696383, 0.000000000000000000, 13.31285208727739899 ) ) ;
#37947=LINE ( 'NONE', #16940, #47654 ) ;
#37948=CARTESIAN_POINT ( 'NONE',  ( -16.30213699992141585, 0.000000000000000000, 9.325531019816025946 ) ) ;
#37949=EDGE_CURVE ( 'NONE', #18997, #6417, #53842, .T. ) ;
#37950=CARTESIAN_POINT ( 'NONE',  ( -14.51406764992763776, -0.1191753592594188005, 5.546122462771021056 ) ) ;
#37951=CARTESIAN_POINT ( 'NONE',  ( 2.072287782118878319, 0.000000000000000000, -2.950529333540147015 ) ) ;
#37952=ADVANCED_FACE ( 'NONE', ( #1872 ), #46157, .F. ) ;
#37953=CARTESIAN_POINT ( 'NONE',  ( -11.62259704383644277, 0.000000000000000000, 5.099289457697922856 ) ) ;
#37954=CARTESIAN_POINT ( 'NONE',  ( -15.45705336148688147, -3.432230869623159819, 8.318851767706947342 ) ) ;
#37955=DIRECTION ( 'NONE',  ( 0.000000000000000000, -1.000000000000000000, 0.000000000000000000 ) ) ;
#37956=DIRECTION ( 'NONE',  ( -0.005961354470445682716, -0.6427876096865404731, 0.7660212471507180654 ) ) ;
#37957=EDGE_CURVE ( 'NONE', #16451, #28682, #19488, .T. ) ;
#37958=EDGE_CURVE ( 'NONE', #25675, #39658, #6438, .T. ) ;
#37959=DIRECTION ( 'NONE',  ( 0.005961354470445682716, -0.6427876096865404731, -0.7660212471507180654 ) ) ;
#37960=VERTEX_POINT ( 'NONE', #23740 ) ;
#37961=DIRECTION ( 'NONE',  ( 0.000000000000000000, -0.000000000000000000, -1.000000000000000000 ) ) ;
#37962=EDGE_CURVE ( 'NONE', #3565, #29285, #19774, .T. ) ;
#37963=ADVANCED_FACE ( 'NONE', ( #41621 ), #15492, .F. ) ;
#37964=EDGE_CURVE ( 'NONE', #39202, #10560, #28023, .T. ) ;
#37965=VERTEX_POINT ( 'NONE', #50703 ) ;
#37966=ORIENTED_EDGE ( 'NONE', *, *, #30573, .T. ) ;
#37967=ORIENTED_EDGE ( 'NONE', *, *, #23738, .F. ) ;
#37968=VERTEX_POINT ( 'NONE', #40800 ) ;
#37969=EDGE_LOOP ( 'NONE', ( #25466, #49623, #43941, #51567 ) ) ;
#37970=ORIENTED_EDGE ( 'NONE', *, *, #18874, .T. ) ;
#37971=LINE ( 'NONE', #55277, #45926 ) ;
#37972=DIRECTION ( 'NONE',  ( -0.6246952433987894571, 0.7422098413412802076, 0.2426528472758539834 ) ) ;
#37973=LINE ( 'NONE', #20910, #23065 ) ;
#37974=AXIS2_PLACEMENT_3D ( 'NONE', #13694, #43789, #39828 ) ;
#37975=VERTEX_POINT ( 'NONE', #33119 ) ;
#37976=CARTESIAN_POINT ( 'NONE',  ( 2.072287782118878319, 0.000000000000000000, -2.950529333540147015 ) ) ;
#37977=EDGE_CURVE ( 'NONE', #9624, #51983, #2985, .T. ) ;
#37978=ORIENTED_EDGE ( 'NONE', *, *, #39887, .F. ) ;
#37979=DIRECTION ( 'NONE',  ( 0.005002170337468016433, -0.7660444431189770143, -0.6427681459581293666 ) ) ;
#37980=ORIENTED_EDGE ( 'NONE', *, *, #47125, .F. ) ;
#37981=EDGE_CURVE ( 'NONE', #17653, #18910, #45598, .T. ) ;
#37983=ADVANCED_FACE ( 'NONE', ( #24032 ), #45894, .F. ) ;
#37984=CARTESIAN_POINT ( 'NONE',  ( -24.26908309836554878, 0.000000000000000000, 6.108867788427308376 ) ) ;
#37986=VERTEX_POINT ( 'NONE', #20313 ) ;
#37987=LINE ( 'NONE', #30022, #5640 ) ;
#37988=ORIENTED_EDGE ( 'NONE', *, *, #37397, .F. ) ;
#37989=EDGE_CURVE ( 'NONE', #38023, #22884, #7009, .T. ) ;
#37990=LINE ( 'NONE', #30312, #36395 ) ;
#37991=DIRECTION ( 'NONE',  ( 0.9999697198139515519, 0.000000000000000000, 0.007781995580013368816 ) ) ;
#37992=CARTESIAN_POINT ( 'NONE',  ( -11.35663643656886634, 0.000000000000000000, 4.932033211054954513 ) ) ;
#37993=FACE_OUTER_BOUND ( 'NONE', #15554, .T. ) ;
#37995=DIRECTION ( 'NONE',  ( 0.5364919789714477361, 0.6444004775717706579, 0.5449076811759711036 ) ) ;
#37997=LINE ( 'NONE', #21225, #44782 ) ;
#37999=EDGE_CURVE ( 'NONE', #7373, #49510, #37097, .T. ) ;
#38000=EDGE_LOOP ( 'NONE', ( #28317, #15744, #52944, #18267 ) ) ;
#38001=LINE ( 'NONE', #2218, #37436 ) ;
#38002=VERTEX_POINT ( 'NONE', #28858 ) ;
#38003=PLANE ( 'NONE',  #44662 ) ;
#38004=DIRECTION ( 'NONE',  ( -0.5364919789714478471, 0.6444004775717705469, -0.5449076811759709926 ) ) ;
#38005=PLANE ( 'NONE',  #25953 ) ;
#38006=LINE ( 'NONE', #30044, #557 ) ;
#38007=PLANE ( 'NONE',  #27697 ) ;
#38008=CARTESIAN_POINT ( 'NONE',  ( 2.072287782118878319, 0.000000000000000000, -2.950529333540147015 ) ) ;
#38009=SHAPE_DEFINITION_REPRESENTATION ( #13296, #12294 ) ;
#38010=ORIENTED_EDGE ( 'NONE', *, *, #53864, .T. ) ;
#38011=DIRECTION ( 'NONE',  ( 0.000000000000000000, -1.000000000000000000, 0.000000000000000000 ) ) ;
#38012=FACE_OUTER_BOUND ( 'NONE', #5198, .T. ) ;
#38013=CARTESIAN_POINT ( 'NONE',  ( -9.400187731170413841, -0.1191753592594185784, 5.216587788961361660 ) ) ;
#38014=DIRECTION ( 'NONE',  ( 0.9999697198139515519, 0.000000000000000000, 0.007781995580013368816 ) ) ;
#38016=CARTESIAN_POINT ( 'NONE',  ( -22.40634380310664397, 0.000000000000000000, 5.584705972946605534 ) ) ;
#38017=DIRECTION ( 'NONE',  ( 0.007781995580012663651, 0.000000000000000000, -0.9999697198139515519 ) ) ;
#38018=DIRECTION ( 'NONE',  ( -0.5364919789714478471, 0.6444004775717705469, -0.5449076811759709926 ) ) ;
#38019=VERTEX_POINT ( 'NONE', #11243 ) ;
#38020=CARTESIAN_POINT ( 'NONE',  ( -31.72782227498118601, 0.000000000000000000, 9.205484770164058972 ) ) ;
#38021=DIRECTION ( 'NONE',  ( 0.000000000000000000, -1.000000000000000000, 0.000000000000000000 ) ) ;
#38022=VERTEX_POINT ( 'NONE', #7262 ) ;
#38023=VERTEX_POINT ( 'NONE', #28569 ) ;
#38025=EDGE_CURVE ( 'NONE', #52283, #21986, #24568, .T. ) ;
#38026=EDGE_CURVE ( 'NONE', #29873, #47765, #33397, .T. ) ;
#38027=EDGE_LOOP ( 'NONE', ( #30948, #27790, #19109, #34129 ) ) ;
#38028=ORIENTED_EDGE ( 'NONE', *, *, #41030, .F. ) ;
#38029=CARTESIAN_POINT ( 'NONE',  ( -18.55457632951175384, -0.5179957512181557755, 4.072021903158996814 ) ) ;
#38030=EDGE_CURVE ( 'NONE', #33009, #12251, #6180, .T. ) ;
#38031=EDGE_LOOP ( 'NONE', ( #16056, #28280, #49062, #37173 ) ) ;
#38032=ORIENTED_EDGE ( 'NONE', *, *, #32173, .F. ) ;
#38033=VERTEX_POINT ( 'NONE', #12072 ) ;
#38034=DIRECTION ( 'NONE',  ( 0.9999697198139515519, 0.000000000000000000, 0.007781995580013368816 ) ) ;
#38036=FACE_OUTER_BOUND ( 'NONE', #54948, .T. ) ;
#38038=VERTEX_POINT ( 'NONE', #39043 ) ;
#38039=EDGE_CURVE ( 'NONE', #22163, #50409, #52103, .T. ) ;
#38040=DIRECTION ( 'NONE',  ( 0.000000000000000000, -1.000000000000000000, 0.000000000000000000 ) ) ;
#38041=CARTESIAN_POINT ( 'NONE',  ( -18.11794600974973690, 0.000000000000000000, 3.819251942559406476 ) ) ;
#38042=EDGE_LOOP ( 'NONE', ( #50474, #9791, #14328, #27024 ) ) ;
#38043=ADVANCED_FACE ( 'NONE', ( #12922 ), #8378, .F. ) ;
#38044=CARTESIAN_POINT ( 'NONE',  ( -14.52177580689696335, 1.581621852479005774, 2.272220598678369896 ) ) ;
#38045=CARTESIAN_POINT ( 'NONE',  ( -14.63053074338272808, 0.000000000000000000, 7.661205510778215988 ) ) ;
#38046=ORIENTED_EDGE ( 'NONE', *, *, #4202, .F. ) ;
#38047=DIRECTION ( 'NONE',  ( -0.005002170337468016433, -0.7660444431189770143, 0.6427681459581293666 ) ) ;
#38048=DIRECTION ( 'NONE',  ( 0.005961354470445682716, -0.6427876096865404731, -0.7660212471507180654 ) ) ;
#38049=ORIENTED_EDGE ( 'NONE', *, *, #29960, .T. ) ;
#38050=EDGE_CURVE ( 'NONE', #27352, #39726, #29408, .T. ) ;
#38051=CARTESIAN_POINT ( 'NONE',  ( -20.54049170961573267, 0.000000000000000000, 4.660556269540326646 ) ) ;
#38052=FACE_OUTER_BOUND ( 'NONE', #5264, .T. ) ;
#38053=ORIENTED_EDGE ( 'NONE', *, *, #365, .T. ) ;
#38056=DIRECTION ( 'NONE',  ( 0.005961354470445682716, -0.6427876096865404731, -0.7660212471507180654 ) ) ;
#38057=LINE ( 'NONE', #16196, #20119 ) ;
#38058=EDGE_CURVE ( 'NONE', #26839, #34987, #17184, .T. ) ;
#38059=ORIENTED_EDGE ( 'NONE', *, *, #11804, .F. ) ;
#38060=CARTESIAN_POINT ( 'NONE',  ( -17.40398185690282773, 0.000000000000000000, 5.792961523881334784 ) ) ;
#38061=CARTESIAN_POINT ( 'NONE',  ( -14.13296160359425535, 0.000000000000000000, 3.433098927415837665 ) ) ;
#38062=DIRECTION ( 'NONE',  ( -0.005002170337468016433, -0.7660444431189770143, 0.6427681459581293666 ) ) ;
#38063=CARTESIAN_POINT ( 'NONE',  ( -16.06709938707323460, 0.000000000000000000, 13.13181314741652628 ) ) ;
#38064=PLANE ( 'NONE',  #51232 ) ;
#38065=CARTESIAN_POINT ( 'NONE',  ( 2.072287782118878319, 0.000000000000000000, -2.950529333540147015 ) ) ;
#38066=DIRECTION ( 'NONE',  ( 0.005961354470445682716, -0.6427876096865404731, -0.7660212471507180654 ) ) ;
#38067=EDGE_LOOP ( 'NONE', ( #23517, #54171, #38168, #24401 ) ) ;
#38068=CARTESIAN_POINT ( 'NONE',  ( -1.086233639165236964, 0.000000000000000000, -2.796443541562362078 ) ) ;
#38069=DIRECTION ( 'NONE',  ( 0.8531650599175529814, -0.4028455766673920135, -0.3313982828793697877 ) ) ;
#38070=ORIENTED_EDGE ( 'NONE', *, *, #18641, .T. ) ;
#38071=DIRECTION ( 'NONE',  ( 0.6427681459581294776, -0.7660444431189769032, 0.005002170337467562802 ) ) ;
#38072=CARTESIAN_POINT ( 'NONE',  ( -9.312785598294761158, 0.000000000000000000, 6.835775765571639795 ) ) ;
#38073=DIRECTION ( 'NONE',  ( 0.005961354470445682716, -0.6427876096865404731, -0.7660212471507180654 ) ) ;
#38074=DIRECTION ( 'NONE',  ( 0.6427681459581294776, -0.7660444431189769032, 0.005002170337467562802 ) ) ;
#38075=DIRECTION ( 'NONE',  ( 0.007781995580012663651, 0.000000000000000000, -0.9999697198139515519 ) ) ;
#38076=ORIENTED_EDGE ( 'NONE', *, *, #16304, .T. ) ;
#38077=ORIENTED_EDGE ( 'NONE', *, *, #16381, .T. ) ;
#38079=DIRECTION ( 'NONE',  ( 0.005961354470445682716, -0.6427876096865404731, -0.7660212471507180654 ) ) ;
#38080=ORIENTED_EDGE ( 'NONE', *, *, #1288, .T. ) ;
#38081=LINE ( 'NONE', #37521, #290 ) ;
#38082=ADVANCED_FACE ( 'NONE', ( #25168 ), #29968, .F. ) ;
#38083=ORIENTED_EDGE ( 'NONE', *, *, #46483, .T. ) ;
#38084=DIRECTION ( 'NONE',  ( 0.007781995580012663651, -3.146120232559066537E-19, -0.9999697198139514409 ) ) ;
#38085=ORIENTED_EDGE ( 'NONE', *, *, #42110, .F. ) ;
#38086=DIRECTION ( 'NONE',  ( -0.005002170337468016433, -0.7660444431189770143, 0.6427681459581293666 ) ) ;
#38087=EDGE_CURVE ( 'NONE', #34545, #34911, #20871, .T. ) ;
#38088=EDGE_CURVE ( 'NONE', #50295, #32412, #4140, .T. ) ;
#38089=ORIENTED_EDGE ( 'NONE', *, *, #31929, .F. ) ;
#38090=VERTEX_POINT ( 'NONE', #116 ) ;
#38091=ORIENTED_EDGE ( 'NONE', *, *, #31169, .T. ) ;
#38092=DIRECTION ( 'NONE',  ( -0.5449076811759708816, 0.6444004775717707689, 0.5364919789714475140 ) ) ;
#38093=CARTESIAN_POINT ( 'NONE',  ( -19.12962290826653700, 0.000000000000000000, 14.40064212555863854 ) ) ;
#38094=CARTESIAN_POINT ( 'NONE',  ( -13.68990958973064664, 3.362543313726509719, 1.892274790874030943 ) ) ;
#38095=DIRECTION ( 'NONE',  ( 0.000000000000000000, -1.000000000000000000, 0.000000000000000000 ) ) ;
#38096=EDGE_LOOP ( 'NONE', ( #7415, #7354, #37615, #40749 ) ) ;
#38097=ORIENTED_EDGE ( 'NONE', *, *, #17691, .F. ) ;
#38098=ORIENTED_EDGE ( 'NONE', *, *, #4196, .T. ) ;
#38099=DIRECTION ( 'NONE',  ( 0.9999697198139515519, 0.000000000000000000, 0.007781995580013368816 ) ) ;
#38100=LINE ( 'NONE', #55414, #42710 ) ;
#38101=ORIENTED_EDGE ( 'NONE', *, *, #12474, .T. ) ;
#38102=CARTESIAN_POINT ( 'NONE',  ( -16.89152113916034992, -4.565544526780660917, 10.73600855493934247 ) ) ;
#38103=ORIENTED_EDGE ( 'NONE', *, *, #53909, .F. ) ;
#38104=PLANE ( 'NONE',  #55030 ) ;
#38105=CARTESIAN_POINT ( 'NONE',  ( -11.22714339797767558, -0.1191753592594190225, 1.142630195505416557 ) ) ;
#38106=VERTEX_POINT ( 'NONE', #37933 ) ;
#38107=DIRECTION ( 'NONE',  ( 0.005961354470445682716, -0.6427876096865404731, -0.7660212471507180654 ) ) ;
#38108=ORIENTED_EDGE ( 'NONE', *, *, #8832, .T. ) ;
#38109=ADVANCED_FACE ( 'NONE', ( #4422 ), #21733, .F. ) ;
#38110=VECTOR ( 'NONE', #1628, 1000.000000000000227 ) ;
#38111=DIRECTION ( 'NONE',  ( 0.007781995580012662783, 0.000000000000000000, -0.9999697198139514409 ) ) ;
#38112=CARTESIAN_POINT ( 'NONE',  ( -25.20123094555300369, 0.000000000000000000, 6.470945668149052032 ) ) ;
#38113=ORIENTED_EDGE ( 'NONE', *, *, #9891, .T. ) ;
#38114=ADVANCED_FACE ( 'NONE', ( #20622 ), #29114, .F. ) ;
#38115=FACE_OUTER_BOUND ( 'NONE', #10032, .T. ) ;
#38116=CARTESIAN_POINT ( 'NONE',  ( -11.57295624737693096, 0.2864062442990046309, 1.846691783222848882 ) ) ;
#38117=DIRECTION ( 'NONE',  ( -0.5449076811759708816, 0.6444004775717707689, 0.5364919789714475140 ) ) ;
#38118=DIRECTION ( 'NONE',  ( -0.005002170337468016433, -0.7660444431189770143, 0.6427681459581293666 ) ) ;
#38119=ORIENTED_EDGE ( 'NONE', *, *, #7657, .F. ) ;
#38120=EDGE_LOOP ( 'NONE', ( #46202, #17495, #1555, #23959 ) ) ;
#38122=ADVANCED_FACE ( 'NONE', ( #7539 ), #21158, .F. ) ;
#38123=DIRECTION ( 'NONE',  ( 0.9999697198139515519, 0.000000000000000000, 0.007781995580013368816 ) ) ;
#38124=CARTESIAN_POINT ( 'NONE',  ( -19.53735095677732403, 0.000000000000000000, 7.084361417893372703 ) ) ;
#38125=LINE ( 'NONE', #28789, #12190 ) ;
#38126=FACE_OUTER_BOUND ( 'NONE', #15527, .T. ) ;
#38127=CARTESIAN_POINT ( 'NONE',  ( -10.47421230394850866, 0.000000000000000000, 10.95934586908605723 ) ) ;
#38128=ORIENTED_EDGE ( 'NONE', *, *, #29047, .F. ) ;
#38129=DIRECTION ( 'NONE',  ( 0.6427681459581294776, -0.7660444431189769032, 0.005002170337467562802 ) ) ;
#38130=CARTESIAN_POINT ( 'NONE',  ( -14.41484887750424448, 0.000000000000000000, 5.646897634310420244 ) ) ;
#38131=ORIENTED_EDGE ( 'NONE', *, *, #41517, .T. ) ;
#38132=LINE ( 'NONE', #46099, #5069 ) ;
#38133=ORIENTED_EDGE ( 'NONE', *, *, #42816, .T. ) ;
#38135=LINE ( 'NONE', #46360, #48729 ) ;
#38136=CARTESIAN_POINT ( 'NONE',  ( -15.88053067323646417, -0.1191753592594197858, 2.950163842912994383 ) ) ;
#38137=ADVANCED_FACE ( 'NONE', ( #38786 ), #46728, .F. ) ;
#38138=PLANE ( 'NONE',  #16026 ) ;
#38140=EDGE_LOOP ( 'NONE', ( #36357, #33014, #45404, #12835 ) ) ;
#38141=VERTEX_POINT ( 'NONE', #33947 ) ;
#38143=CARTESIAN_POINT ( 'NONE',  ( -32.65919192261063841, -0.1191753592594197858, 9.467565677904410393 ) ) ;
#38144=CARTESIAN_POINT ( 'NONE',  ( -22.40478740399063895, 0.000000000000000000, 5.384712028983816623 ) ) ;
#38145=EDGE_CURVE ( 'NONE', #30915, #44660, #47012, .T. ) ;
#38146=CARTESIAN_POINT ( 'NONE',  ( -14.66887761629205222, 0.000000000000000000, 12.58869632783390990 ) ) ;
#38147=CARTESIAN_POINT ( 'NONE',  ( -21.47419595591918906, 0.000000000000000000, 5.222628093224860102 ) ) ;
#38149=EDGE_CURVE ( 'NONE', #14066, #53756, #51813, .T. ) ;
#38150=CARTESIAN_POINT ( 'NONE',  ( -22.40634380310664397, 0.000000000000000000, 5.584705972946605534 ) ) ;
#38151=EDGE_LOOP ( 'NONE', ( #51385, #13294, #5955, #56186 ) ) ;
#38152=CARTESIAN_POINT ( 'NONE',  ( -15.88688127818832463, -2.298917212465657833, 6.625850739918041299 ) ) ;
#38153=ADVANCED_FACE ( 'NONE', ( #25422 ), #55812, .F. ) ;
#38154=VECTOR ( 'NONE', #42041, 999.9999999999998863 ) ;
#38155=FACE_OUTER_BOUND ( 'NONE', #7540, .T. ) ;
#38156=CARTESIAN_POINT ( 'NONE',  ( -19.25678133725660501, 0.000000000000000000, 5.039878470293768231 ) ) ;
#38157=VERTEX_POINT ( 'NONE', #47271 ) ;
#38158=DIRECTION ( 'NONE',  ( 0.000000000000000000, -1.000000000000000000, 0.000000000000000000 ) ) ;
#38160=DIRECTION ( 'NONE',  ( 0.007781995580012663651, 0.000000000000000000, -0.9999697198139515519 ) ) ;
#38161=EDGE_CURVE ( 'NONE', #12315, #165, #31074, .T. ) ;
#38162=VERTEX_POINT ( 'NONE', #13496 ) ;
#38163=PLANE ( 'NONE',  #51924 ) ;
#38164=ORIENTED_EDGE ( 'NONE', *, *, #39770, .F. ) ;
#38165=EDGE_CURVE ( 'NONE', #17943, #47842, #4971, .T. ) ;
#38166=ORIENTED_EDGE ( 'NONE', *, *, #45964, .F. ) ;
#38167=ORIENTED_EDGE ( 'NONE', *, *, #635, .F. ) ;
#38168=ORIENTED_EDGE ( 'NONE', *, *, #54064, .T. ) ;
#38169=CARTESIAN_POINT ( 'NONE',  ( -13.17065887352947762, -0.1191753592594197858, 12.04635770780929427 ) ) ;
#38170=ORIENTED_EDGE ( 'NONE', *, *, #29460, .F. ) ;
#38172=VECTOR ( 'NONE', #56177, 1000.000000000000227 ) ;
#38173=VECTOR ( 'NONE', #3108, 1000.000000000000227 ) ;
#38174=ORIENTED_EDGE ( 'NONE', *, *, #25247, .T. ) ;
#38175=DIRECTION ( 'NONE',  ( 0.005002170337468016433, -0.7660444431189770143, -0.6427681459581293666 ) ) ;
#38177=ORIENTED_EDGE ( 'NONE', *, *, #52086, .T. ) ;
#38178=DIRECTION ( 'NONE',  ( 0.6427681459581294776, -0.7660444431189769032, 0.005002170337467562802 ) ) ;
#38179=CARTESIAN_POINT ( 'NONE',  ( -12.15271748404464880, 0.000000000000000000, 1.601849296007406664 ) ) ;
#38180=DIRECTION ( 'NONE',  ( -0.005002170337468016433, -0.7660444431189770143, 0.6427681459581293666 ) ) ;
#38181=FACE_OUTER_BOUND ( 'NONE', #936, .T. ) ;
#38182=ORIENTED_EDGE ( 'NONE', *, *, #30659, .F. ) ;
#38183=EDGE_LOOP ( 'NONE', ( #11512, #24823, #10178, #27799 ) ) ;
#38184=AXIS2_PLACEMENT_3D ( 'NONE', #10759, #15018, #53897 ) ;
#38185=LINE ( 'NONE', #24022, #45796 ) ;
#38186=EDGE_CURVE ( 'NONE', #10812, #3022, #18289, .T. ) ;
#38187=PLANE ( 'NONE',  #42081 ) ;
#38188=VECTOR ( 'NONE', #46229, 999.9999999999998863 ) ;
#38189=CARTESIAN_POINT ( 'NONE',  ( -19.51236138453683822, 1.419719901456505617, 4.215899037920694425 ) ) ;
#38190=DIRECTION ( 'NONE',  ( 0.5364919789714477361, 0.6444004775717706579, 0.5449076811759711036 ) ) ;
#38191=CARTESIAN_POINT ( 'NONE',  ( -17.65425454225471213, 0.000000000000000000, 3.944353494940506355 ) ) ;
#38192=DIRECTION ( 'NONE',  ( 0.9321478471874540261, 0.000000000000000000, -0.3620778797217457101 ) ) ;
#38193=ORIENTED_EDGE ( 'NONE', *, *, #17133, .T. ) ;
#38194=LINE ( 'NONE', #51815, #55556 ) ;
#38196=ORIENTED_EDGE ( 'NONE', *, *, #37393, .F. ) ;
#38197=EDGE_CURVE ( 'NONE', #38808, #42624, #23136, .T. ) ;
#38198=DIRECTION ( 'NONE',  ( -0.005002170337468016433, -0.7660444431189770143, 0.6427681459581293666 ) ) ;
#38199=CARTESIAN_POINT ( 'NONE',  ( -22.40478740399063895, 0.000000000000000000, 5.384712028983816623 ) ) ;
#38200=FACE_OUTER_BOUND ( 'NONE', #50070, .T. ) ;
#38201=FACE_OUTER_BOUND ( 'NONE', #4618, .T. ) ;
#38202=EDGE_CURVE ( 'NONE', #18181, #42292, #39632, .T. ) ;
#38203=EDGE_CURVE ( 'NONE', #24571, #27123, #13217, .T. ) ;
#38204=CARTESIAN_POINT ( 'NONE',  ( -16.74509912310952231, 0.000000000000000000, 6.536753241280876203 ) ) ;
#38205=ORIENTED_EDGE ( 'NONE', *, *, #5515, .F. ) ;
#38206=ORIENTED_EDGE ( 'NONE', *, *, #49562, .T. ) ;
#38207=DIRECTION ( 'NONE',  ( 0.5449076811759707706, 0.6444004775717708799, -0.5364919789714476250 ) ) ;
#38208=LINE ( 'NONE', #51291, #26771 ) ;
#38209=CARTESIAN_POINT ( 'NONE',  ( -21.14151471908257562, 3.848249166794009746, 11.40903589015699815 ) ) ;
#38210=VECTOR ( 'NONE', #21808, 999.9999999999998863 ) ;
#38211=AXIS2_PLACEMENT_3D ( 'NONE', #24624, #15290, #41939 ) ;
#38212=LINE ( 'NONE', #2717, #10133 ) ;
#38213=EDGE_CURVE ( 'NONE', #47771, #54647, #30811, .T. ) ;
#38214=CARTESIAN_POINT ( 'NONE',  ( -17.85293083182822116, 0.000000000000000000, 3.773481336529526775 ) ) ;
#38215=DIRECTION ( 'NONE',  ( 0.000000000000000000, -1.000000000000000000, 0.000000000000000000 ) ) ;
#38216=DIRECTION ( 'NONE',  ( 0.000000000000000000, -0.000000000000000000, -1.000000000000000000 ) ) ;
#38217=EDGE_CURVE ( 'NONE', #6270, #5817, #8962, .T. ) ;
#38218=CARTESIAN_POINT ( 'NONE',  ( -15.88053067323646417, -0.1191753592594197858, 2.950163842912994383 ) ) ;
#38220=CARTESIAN_POINT ( 'NONE',  ( -14.14612558372896878, -4.079838673713159558, 8.872477635332897350 ) ) ;
#38221=ORIENTED_EDGE ( 'NONE', *, *, #25608, .F. ) ;
#38222=LINE ( 'NONE', #8141, #25021 ) ;
#38223=EDGE_CURVE ( 'NONE', #14383, #39021, #48112, .T. ) ;
#38224=ORIENTED_EDGE ( 'NONE', *, *, #52811, .T. ) ;
#38225=ORIENTED_EDGE ( 'NONE', *, *, #38526, .T. ) ;
#38226=VECTOR ( 'NONE', #22488, 1000.000000000000227 ) ;
#38227=EDGE_CURVE ( 'NONE', #1987, #29115, #48398, .T. ) ;
#38228=VERTEX_POINT ( 'NONE', #39884 ) ;
#38229=EDGE_LOOP ( 'NONE', ( #8106, #6094, #30082, #18515 ) ) ;
#38230=ORIENTED_EDGE ( 'NONE', *, *, #3433, .F. ) ;
#38231=VERTEX_POINT ( 'NONE', #1252 ) ;
#38232=PLANE ( 'NONE',  #49595 ) ;
#38233=CARTESIAN_POINT ( 'NONE',  ( -15.88053067323646417, -0.1191753592594197858, 2.950163842912994383 ) ) ;
#38235=ORIENTED_EDGE ( 'NONE', *, *, #24153, .F. ) ;
#38236=FACE_OUTER_BOUND ( 'NONE', #39678, .T. ) ;
#38237=ORIENTED_EDGE ( 'NONE', *, *, #47856, .F. ) ;
#38238=DIRECTION ( 'NONE',  ( -0.005961354470445682716, -0.6427876096865404731, 0.7660212471507180654 ) ) ;
#38239=ORIENTED_EDGE ( 'NONE', *, *, #51013, .T. ) ;
#38240=LINE ( 'NONE', #4469, #39260 ) ;
#38241=CARTESIAN_POINT ( 'NONE',  ( -18.67775241435682432, 0.000000000000000000, 4.136394454059623804 ) ) ;
#38242=DIRECTION ( 'NONE',  ( 0.005002170337468016433, -0.7660444431189770143, -0.6427681459581293666 ) ) ;
#38243=ORIENTED_EDGE ( 'NONE', *, *, #10903, .F. ) ;
#38244=CARTESIAN_POINT ( 'NONE',  ( -27.99767448711536133, 0.000000000000000000, 7.557179307314289218 ) ) ;
#38245=ORIENTED_EDGE ( 'NONE', *, *, #35710, .F. ) ;
#38247=VECTOR ( 'NONE', #35011, 1000.000000000000227 ) ;
#38248=LINE ( 'NONE', #42786, #46388 ) ;
#38249=EDGE_CURVE ( 'NONE', #6678, #21349, #52650, .T. ) ;
#38250=CARTESIAN_POINT ( 'NONE',  ( -16.89925026227929195, -0.1191753592594197858, 13.49466922669627422 ) ) ;
#38251=CARTESIAN_POINT ( 'NONE',  ( -9.933042293644859910, -0.002715256824217495563, 1.421395705359619122 ) ) ;
#38252=AXIS2_PLACEMENT_3D ( 'NONE', #50349, #54890, #3494 ) ;
#38253=DIRECTION ( 'NONE',  ( -0.005961354470445682716, -0.6427876096865404731, 0.7660212471507180654 ) ) ;
#38256=CARTESIAN_POINT ( 'NONE',  ( -18.14188386713806267, 0.000000000000000000, 6.895215209234613063 ) ) ;
#38258=EDGE_LOOP ( 'NONE', ( #36212, #33609, #27992, #22290 ) ) ;
#38260=ORIENTED_EDGE ( 'NONE', *, *, #2850, .T. ) ;
#38261=EDGE_CURVE ( 'NONE', #10471, #31963, #9218, .T. ) ;
#38262=EDGE_CURVE ( 'NONE', #54647, #3649, #31661, .T. ) ;
#38263=ADVANCED_FACE ( 'NONE', ( #44693 ), #9808, .F. ) ;
#38264=DIRECTION ( 'NONE',  ( -0.005961354470445682716, -0.6427876096865404731, 0.7660212471507180654 ) ) ;
#38265=CARTESIAN_POINT ( 'NONE',  ( -29.86197018149027116, 0.000000000000000000, 8.281335066757780083 ) ) ;
#38266=DIRECTION ( 'NONE',  ( 0.5449076811759707706, 0.6444004775717708799, -0.5364919789714476250 ) ) ;
#38267=VECTOR ( 'NONE', #48763, 1000.000000000000227 ) ;
#38268=CARTESIAN_POINT ( 'NONE',  ( -11.15376843910079607, 0.000000000000000000, 4.564279906913194296 ) ) ;
#38269=DIRECTION ( 'NONE',  ( 0.000000000000000000, -1.000000000000000000, 0.000000000000000000 ) ) ;
#38270=VECTOR ( 'NONE', #5794, 1000.000000000000227 ) ;
#38271=EDGE_CURVE ( 'NONE', #41467, #40214, #14050, .T. ) ;
#38272=PLANE ( 'NONE',  #38288 ) ;
#38273=VERTEX_POINT ( 'NONE', #43859 ) ;
#38274=CARTESIAN_POINT ( 'NONE',  ( -12.20953538199096755, -0.1191753592594198830, 7.960971755595982025 ) ) ;
#38275=LINE ( 'NONE', #38574, #34927 ) ;
#38276=LINE ( 'NONE', #51362, #39976 ) ;
#38277=CARTESIAN_POINT ( 'NONE',  ( -15.40103151951671734, 0.000000000000000000, 12.95233060667165681 ) ) ;
#38279=LINE ( 'NONE', #55604, #39366 ) ;
#38280=CARTESIAN_POINT ( 'NONE',  ( -16.81267852042391198, -0.1191753592594197858, 3.312241722634738039 ) ) ;
#38281=DIRECTION ( 'NONE',  ( -0.005002170337468016433, -0.7660444431189770143, 0.6427681459581293666 ) ) ;
#38283=ADVANCED_FACE ( 'NONE', ( #40157 ), #21997, .F. ) ;
#38284=DIRECTION ( 'NONE',  ( -0.005961354470445682716, -0.6427876096865404731, 0.7660212471507180654 ) ) ;
#38285=PLANE ( 'NONE',  #28689 ) ;
#38286=ORIENTED_EDGE ( 'NONE', *, *, #7013, .T. ) ;
#38287=ADVANCED_FACE ( 'NONE', ( #22840 ), #20241, .F. ) ;
#38288=AXIS2_PLACEMENT_3D ( 'NONE', #38008, #11864, #55060 ) ;
#38289=ORIENTED_EDGE ( 'NONE', *, *, #31253, .F. ) ;
#38290=CARTESIAN_POINT ( 'NONE',  ( 0.000000000000000000, 0.000000000000000000, 0.000000000000000000 ) ) ;
#38291=VECTOR ( 'NONE', #50383, 999.9999999999998863 ) ;
#38292=EDGE_CURVE ( 'NONE', #41711, #42294, #27962, .T. ) ;
#38293=VECTOR ( 'NONE', #49087, 999.9999999999998863 ) ;
#38294=EDGE_LOOP ( 'NONE', ( #29584, #50357, #20705, #20526 ) ) ;
#38295=FACE_OUTER_BOUND ( 'NONE', #35680, .T. ) ;
#38296=VECTOR ( 'NONE', #48499, 999.9999999999998863 ) ;
#38297=VERTEX_POINT ( 'NONE', #49235 ) ;
#38298=ORIENTED_EDGE ( 'NONE', *, *, #28128, .F. ) ;
#38299=AXIS2_PLACEMENT_3D ( 'NONE', #13678, #27296, #44609 ) ;
#38300=ORIENTED_EDGE ( 'NONE', *, *, #46289, .F. ) ;
#38301=CARTESIAN_POINT ( 'NONE',  ( -16.33317936670417225, 0.000000000000000000, 13.31440848639340224 ) ) ;
#38303=DIRECTION ( 'NONE',  ( -0.5364919789714478471, 0.6444004775717705469, -0.5449076811759709926 ) ) ;
#38304=VERTEX_POINT ( 'NONE', #27674 ) ;
#38305=VECTOR ( 'NONE', #44148, 1000.000000000000000 ) ;
#38306=ORIENTED_EDGE ( 'NONE', *, *, #45635, .T. ) ;
#38307=CARTESIAN_POINT ( 'NONE',  ( -20.54049170961573267, 0.000000000000000000, 4.660556269540326646 ) ) ;
#38308=FACE_OUTER_BOUND ( 'NONE', #129, .T. ) ;
#38309=EDGE_LOOP ( 'NONE', ( #19467, #37617, #405, #33848 ) ) ;
#38310=CARTESIAN_POINT ( 'NONE',  ( -12.15116108492864377, 0.000000000000000000, 1.401855352044617975 ) ) ;
#38311=DIRECTION ( 'NONE',  ( -0.9999697198139514409, -0.000000000000000000, -0.007781995580013368816 ) ) ;
#38312=EDGE_LOOP ( 'NONE', ( #40071, #47781, #40922, #49280 ) ) ;
#38313=CARTESIAN_POINT ( 'NONE',  ( -1.086233639165236964, 0.000000000000000000, -2.796443541562362078 ) ) ;
#38314=ADVANCED_FACE ( 'NONE', ( #19967 ), #10353, .F. ) ;
#38315=ORIENTED_EDGE ( 'NONE', *, *, #20834, .T. ) ;
#38316=LINE ( 'NONE', #7970, #55435 ) ;
#38317=ADVANCED_FACE ( 'NONE', ( #37032 ), #10897, .F. ) ;
#38318=AXIS2_PLACEMENT_3D ( 'NONE', #35109, #40170, #18299 ) ;
#38319=LINE ( 'NONE', #56207, #27285 ) ;
#38320=EDGE_LOOP ( 'NONE', ( #16362, #3406, #22709, #54099 ) ) ;
#38322=LINE ( 'NONE', #34623, #45606 ) ;
#38324=AXIS2_PLACEMENT_3D ( 'NONE', #41315, #19986, #27984 ) ;
#38325=CARTESIAN_POINT ( 'NONE',  ( -21.39391032317488595, -2.784623065533159636, 5.102598372062590038 ) ) ;
#38326=ORIENTED_EDGE ( 'NONE', *, *, #22568, .T. ) ;
#38327=EDGE_CURVE ( 'NONE', #8024, #1300, #6370, .T. ) ;
#38328=EDGE_CURVE ( 'NONE', #21349, #23457, #24250, .T. ) ;
#38329=ADVANCED_FACE ( 'NONE', ( #10657 ), #7204, .F. ) ;
#38330=VECTOR ( 'NONE', #9042, 1000.000000000000114 ) ;
#38331=VECTOR ( 'NONE', #38560, 1000.000000000000227 ) ;
#38332=CARTESIAN_POINT ( 'NONE',  ( -13.09043773662596166, -2.298917212465658277, 5.539617100752805001 ) ) ;
#38333=DIRECTION ( 'NONE',  ( 0.005002170337468016433, -0.7660444431189770143, -0.6427681459581293666 ) ) ;
#38334=DIRECTION ( 'NONE',  ( 0.5449076811759707706, 0.6444004775717708799, -0.5364919789714476250 ) ) ;
#38336=EDGE_CURVE ( 'NONE', #33080, #36001, #50056, .T. ) ;
#38337=DIRECTION ( 'NONE',  ( 0.005961354470445682716, -0.6427876096865404731, -0.7660212471507180654 ) ) ;
#38338=CARTESIAN_POINT ( 'NONE',  ( -18.67697421479882181, -0.1191753592594197858, 4.036397482078229793 ) ) ;
#38340=CARTESIAN_POINT ( 'NONE',  ( -10.47421230394850866, 0.000000000000000000, 10.95934586908605723 ) ) ;
#38341=VECTOR ( 'NONE', #38563, 1000.000000000000114 ) ;
#38342=ORIENTED_EDGE ( 'NONE', *, *, #11573, .T. ) ;
#38344=VERTEX_POINT ( 'NONE', #45004 ) ;
#38345=DIRECTION ( 'NONE',  ( 0.9999697198139515519, 0.000000000000000000, 0.007781995580013368816 ) ) ;
#38346=CARTESIAN_POINT ( 'NONE',  ( 2.072287782118878319, 0.000000000000000000, -2.950529333540147015 ) ) ;
#38347=CARTESIAN_POINT ( 'NONE',  ( -12.27573167061919079, 0.000000000000000000, 3.616878333782851840 ) ) ;
#38348=VECTOR ( 'NONE', #35763, 999.9999999999998863 ) ;
#38349=VECTOR ( 'NONE', #37127, 1000.000000000000000 ) ;
#38350=CARTESIAN_POINT ( 'NONE',  ( -15.13495153988577968, 0.000000000000000000, 12.76973526769478084 ) ) ;
#38352=CARTESIAN_POINT ( 'NONE',  ( -9.756983695072257490, 0.000000000000000000, 4.205817938959457436 ) ) ;
#38354=VERTEX_POINT ( 'NONE', #46095 ) ;
#38355=EDGE_CURVE ( 'NONE', #3202, #31910, #41820, .T. ) ;
#38356=CARTESIAN_POINT ( 'NONE',  ( -16.06709938707323460, 0.000000000000000000, 13.13181314741652628 ) ) ;
#38357=DIRECTION ( 'NONE',  ( -0.3620778797217457101, 0.000000000000000000, -0.9321478471874540261 ) ) ;
#38358=EDGE_LOOP ( 'NONE', ( #24367, #2152, #19754, #27512 ) ) ;
#38359=VECTOR ( 'NONE', #20531, 1000.000000000000227 ) ;
#38361=ADVANCED_FACE ( 'NONE', ( #2910 ), #53767, .F. ) ;
#38363=CARTESIAN_POINT ( 'NONE',  ( -27.06708303904391144, 0.000000000000000000, 7.395095371555332697 ) ) ;
#38364=VECTOR ( 'NONE', #5211, 999.9999999999998863 ) ;
#38365=EDGE_LOOP ( 'NONE', ( #50507, #46698, #30120, #14382 ) ) ;
#38366=LINE ( 'NONE', #29282, #1147 ) ;
#38367=ADVANCED_FACE ( 'NONE', ( #40993 ), #2076, .F. ) ;
#38368=ORIENTED_EDGE ( 'NONE', *, *, #51587, .T. ) ;
#38369=ORIENTED_EDGE ( 'NONE', *, *, #10263, .T. ) ;
#38370=ORIENTED_EDGE ( 'NONE', *, *, #9491, .F. ) ;
#38372=VECTOR ( 'NONE', #7715, 1000.000000000000227 ) ;
#38373=DIRECTION ( 'NONE',  ( 0.000000000000000000, -0.000000000000000000, -1.000000000000000000 ) ) ;
#38374=DIRECTION ( 'NONE',  ( -0.7660212471507179544, -0.6427876096865405842, -0.005961354470445141482 ) ) ;
#38375=VECTOR ( 'NONE', #16351, 999.9999999999998863 ) ;
#38376=AXIS2_PLACEMENT_3D ( 'NONE', #23957, #41564, #15429 ) ;
#38377=FACE_OUTER_BOUND ( 'NONE', #39927, .T. ) ;
#38378=ORIENTED_EDGE ( 'NONE', *, *, #18032, .T. ) ;
#38379=ORIENTED_EDGE ( 'NONE', *, *, #41798, .F. ) ;
#38380=VECTOR ( 'NONE', #24463, 1000.000000000000000 ) ;
#38381=ORIENTED_EDGE ( 'NONE', *, *, #39120, .F. ) ;
#38382=LINE ( 'NONE', #55353, #27745 ) ;
#38383=VECTOR ( 'NONE', #16081, 999.9999999999998863 ) ;
#38384=FACE_OUTER_BOUND ( 'NONE', #17935, .T. ) ;
#38385=VERTEX_POINT ( 'NONE', #45813 ) ;
#38386=LINE ( 'NONE', #55706, #47476 ) ;
#38387=ORIENTED_EDGE ( 'NONE', *, *, #54692, .F. ) ;
#38388=DIRECTION ( 'NONE',  ( 0.7660212471507180654, -0.6427876096865404731, 0.005961354470445141482 ) ) ;
#38389=DIRECTION ( 'NONE',  ( 0.000000000000000000, -1.000000000000000000, 0.000000000000000000 ) ) ;
#38390=ORIENTED_EDGE ( 'NONE', *, *, #25886, .F. ) ;
#38391=LINE ( 'NONE', #13416, #50374 ) ;
#38392=ORIENTED_EDGE ( 'NONE', *, *, #36620, .F. ) ;
#38393=CARTESIAN_POINT ( 'NONE',  ( -1.086233639165236964, 0.000000000000000000, -2.796443541562362078 ) ) ;
#38394=DIRECTION ( 'NONE',  ( -0.005961354470445682716, -0.6427876096865404731, 0.7660212471507180654 ) ) ;
#38395=ORIENTED_EDGE ( 'NONE', *, *, #34918, .F. ) ;
#38396=FACE_OUTER_BOUND ( 'NONE', #44138, .T. ) ;
#38397=CARTESIAN_POINT ( 'NONE',  ( -25.20200914511100265, -0.1191753592594197858, 6.570942640130446932 ) ) ;
#38398=FACE_OUTER_BOUND ( 'NONE', #12654, .T. ) ;
#38399=CARTESIAN_POINT ( 'NONE',  ( -16.78942516689838271, -5.536956232915662746, 12.29060311582175835 ) ) ;
#38400=VERTEX_POINT ( 'NONE', #40735 ) ;
#38401=AXIS2_PLACEMENT_3D ( 'NONE', #22633, #36004, #53011 ) ;
#38402=EDGE_CURVE ( 'NONE', #48148, #25259, #19710, .T. ) ;
#38404=DIRECTION ( 'NONE',  ( -0.5364919789714478471, 0.6444004775717705469, -0.5449076811759709926 ) ) ;
#38405=AXIS2_PLACEMENT_3D ( 'NONE', #33288, #50592, #7410 ) ;
#38406=CARTESIAN_POINT ( 'NONE',  ( -16.61483718085185046, -4.241740624735661491, 10.09711774140462026 ) ) ;
#38407=EDGE_CURVE ( 'NONE', #40878, #9942, #45265, .T. ) ;
#38408=EDGE_CURVE ( 'NONE', #1901, #30787, #54072, .T. ) ;
#38409=DIRECTION ( 'NONE',  ( 0.007781995580012663651, -3.146120232559066537E-19, -0.9999697198139514409 ) ) ;
#38410=DIRECTION ( 'NONE',  ( -0.6427681459581293666, -0.7660444431189770143, -0.005002170337467561935 ) ) ;
#38411=DIRECTION ( 'NONE',  ( -0.005961354470445682716, -0.6427876096865404731, 0.7660212471507180654 ) ) ;
#38412=ORIENTED_EDGE ( 'NONE', *, *, #42055, .F. ) ;
#38413=DIRECTION ( 'NONE',  ( -0.005961354470445682716, -0.6427876096865404731, 0.7660212471507180654 ) ) ;
#38414=CARTESIAN_POINT ( 'NONE',  ( -16.81345671998191449, 0.000000000000000000, 3.412238694616132495 ) ) ;
#38415=DIRECTION ( 'NONE',  ( 0.5364919789714477361, 0.6444004775717706579, 0.5449076811759711036 ) ) ;
#38416=EDGE_LOOP ( 'NONE', ( #17650, #31124, #19614, #44970 ) ) ;
#38418=LINE ( 'NONE', #51499, #44941 ) ;
#38419=ORIENTED_EDGE ( 'NONE', *, *, #30615, .F. ) ;
#38420=AXIS2_PLACEMENT_3D ( 'NONE', #54211, #45391, #15308 ) ;
#38421=LINE ( 'NONE', #13153, #3519 ) ;
#38422=LINE ( 'NONE', #26991, #27858 ) ;
#38423=DIRECTION ( 'NONE',  ( -0.6427681459581293666, -0.7660444431189770143, -0.005002170337467561935 ) ) ;
#38425=ORIENTED_EDGE ( 'NONE', *, *, #51370, .T. ) ;
#38426=VECTOR ( 'NONE', #13154, 999.9999999999998863 ) ;
#38427=VECTOR ( 'NONE', #3070, 1000.000000000000114 ) ;
#38428=ORIENTED_EDGE ( 'NONE', *, *, #44884, .F. ) ;
#38429=CARTESIAN_POINT ( 'NONE',  ( 2.072287782118878319, 0.000000000000000000, -2.950529333540147015 ) ) ;
#38430=CARTESIAN_POINT ( 'NONE',  ( -18.67619601524082285, 0.000000000000000000, 3.936400510096834893 ) ) ;
#38431=FACE_OUTER_BOUND ( 'NONE', #3068, .T. ) ;
#38432=CARTESIAN_POINT ( 'NONE',  ( -26.13415699229845757, -0.1191753592594197858, 6.933020519852192365 ) ) ;
#38433=CARTESIAN_POINT ( 'NONE',  ( 2.072287782118878319, 0.000000000000000000, -2.950529333540147015 ) ) ;
#38434=LINE ( 'NONE', #16567, #18570 ) ;
#38435=ORIENTED_EDGE ( 'NONE', *, *, #22898, .T. ) ;
#38436=LINE ( 'NONE', #25384, #47369 ) ;
#38439=ORIENTED_EDGE ( 'NONE', *, *, #30492, .F. ) ;
#38440=AXIS2_PLACEMENT_3D ( 'NONE', #25676, #34474, #87 ) ;
#38441=EDGE_CURVE ( 'NONE', #46316, #41332, #42112, .T. ) ;
#38442=DIRECTION ( 'NONE',  ( 0.007781995580012663651, 0.000000000000000000, -0.9999697198139515519 ) ) ;
#38443=CARTESIAN_POINT ( 'NONE',  ( -15.39548367756490777, 5.305366725996510269, 11.56846045315015026 ) ) ;
#38444=EDGE_CURVE ( 'NONE', #51932, #17026, #43163, .T. ) ;
#38445=VECTOR ( 'NONE', #48960, 999.9999999999998863 ) ;
#38446=LINE ( 'NONE', #20841, #8465 ) ;
#38447=ORIENTED_EDGE ( 'NONE', *, *, #34209, .T. ) ;
#38448=LINE ( 'NONE', #29687, #8532 ) ;
#38449=EDGE_CURVE ( 'NONE', #40111, #33095, #33337, .T. ) ;
#38451=EDGE_LOOP ( 'NONE', ( #13263, #39889, #9416, #31305 ) ) ;
#38452=VERTEX_POINT ( 'NONE', #38130 ) ;
#38453=ORIENTED_EDGE ( 'NONE', *, *, #36509, .F. ) ;
#38454=ORIENTED_EDGE ( 'NONE', *, *, #53005, .T. ) ;
#38455=AXIS2_PLACEMENT_3D ( 'NONE', #48869, #48280, #53138 ) ;
#38456=PLANE ( 'NONE',  #38440 ) ;
#38457=VERTEX_POINT ( 'NONE', #30179 ) ;
#38459=ORIENTED_EDGE ( 'NONE', *, *, #25108, .F. ) ;
#38460=LINE ( 'NONE', #16901, #20440 ) ;
#38461=EDGE_LOOP ( 'NONE', ( #27938, #20515, #16841, #45803 ) ) ;
#38462=ORIENTED_EDGE ( 'NONE', *, *, #13981, .F. ) ;
#38463=VECTOR ( 'NONE', #22096, 1000.000000000000227 ) ;
#38464=VECTOR ( 'NONE', #38800, 1000.000000000000227 ) ;
#38465=DIRECTION ( 'NONE',  ( -0.6427681459581293666, -0.7660444431189770143, -0.005002170337467561935 ) ) ;
#38466=DIRECTION ( 'NONE',  ( -0.5364919789714478471, 0.6444004775717705469, -0.5449076811759709926 ) ) ;
#38467=CARTESIAN_POINT ( 'NONE',  ( -15.87975247367846166, 0.000000000000000000, 2.850166870931599927 ) ) ;
#38468=CARTESIAN_POINT ( 'NONE',  ( -20.54126990917373519, -0.1191753592594197858, 4.760553241521720658 ) ) ;
#38469=ADVANCED_FACE ( 'NONE', ( #51748 ), #7469, .F. ) ;
#38470=DIRECTION ( 'NONE',  ( -0.9999697198139514409, -0.000000000000000000, -0.007781995580013368816 ) ) ;
#38471=EDGE_LOOP ( 'NONE', ( #45362, #17889, #6215, #1526 ) ) ;
#38472=EDGE_CURVE ( 'NONE', #5817, #17246, #46952, .T. ) ;
#38473=ORIENTED_EDGE ( 'NONE', *, *, #8250, .F. ) ;
#38474=CARTESIAN_POINT ( 'NONE',  ( 2.072287782118878319, 0.000000000000000000, -2.950529333540147015 ) ) ;
#38475=DIRECTION ( 'NONE',  ( 0.9999697198139515519, 0.000000000000000000, 0.007781995580013368816 ) ) ;
#38476=EDGE_CURVE ( 'NONE', #15150, #6764, #17127, .T. ) ;
#38477=ADVANCED_FACE ( 'NONE', ( #16270 ), #20812, .F. ) ;
#38478=LINE ( 'NONE', #34497, #6148 ) ;
#38479=VECTOR ( 'NONE', #17515, 1000.000000000000114 ) ;
#38480=CARTESIAN_POINT ( 'NONE',  ( -12.30602860478801830, 0.000000000000000000, 7.509969310323286074 ) ) ;
#38481=AXIS2_PLACEMENT_3D ( 'NONE', #18795, #44595, #35270 ) ;
#38482=CARTESIAN_POINT ( 'NONE',  ( -19.32961685222932147, 0.000000000000000000, 14.39908572644263351 ) ) ;
#38483=CARTESIAN_POINT ( 'NONE',  ( -10.84028925556084388, -0.1191753592594197858, 11.14116300850493246 ) ) ;
#38484=VERTEX_POINT ( 'NONE', #3504 ) ;
#38485=CARTESIAN_POINT ( 'NONE',  ( -21.16434561149341675, -4.727446477803162850, 4.951441403346398928 ) ) ;
#38486=PLANE ( 'NONE',  #9563 ) ;
#38487=VECTOR ( 'NONE', #16763, 999.9999999999998863 ) ;
#38488=ORIENTED_EDGE ( 'NONE', *, *, #47741, .T. ) ;
#38489=PLANE ( 'NONE',  #15277 ) ;
#38490=DIRECTION ( 'NONE',  ( 0.6427681459581294776, -0.7660444431189769032, 0.005002170337467562802 ) ) ;
#38491=LINE ( 'NONE', #55249, #28662 ) ;
#38492=LINE ( 'NONE', #11550, #39542 ) ;
#38493=ADVANCED_FACE ( 'NONE', ( #51497 ), #42412, .F. ) ;
#38494=ORIENTED_EDGE ( 'NONE', *, *, #28468, .F. ) ;
#38495=VECTOR ( 'NONE', #54391, 1000.000000000000114 ) ;
#38496=ORIENTED_EDGE ( 'NONE', *, *, #27999, .F. ) ;
#38497=VECTOR ( 'NONE', #11057, 999.9999999999998863 ) ;
#38498=LINE ( 'NONE', #46436, #18525 ) ;
#38499=CARTESIAN_POINT ( 'NONE',  ( -18.86354292863559579, 0.000000000000000000, 14.21804678658176080 ) ) ;
#38500=DIRECTION ( 'NONE',  ( -0.6427681459581293666, -0.7660444431189770143, -0.005002170337467561935 ) ) ;
#38501=VECTOR ( 'NONE', #29773, 999.9999999999998863 ) ;
#38502=DIRECTION ( 'NONE',  ( 0.6427681459581294776, -0.7660444431189769032, 0.005002170337467562802 ) ) ;
#38503=DIRECTION ( 'NONE',  ( 0.005002170337468016433, -0.7660444431189770143, -0.6427681459581293666 ) ) ;
#38504=LINE ( 'NONE', #12674, #50937 ) ;
#38505=CARTESIAN_POINT ( 'NONE',  ( -16.99924723426068951, 0.000000000000000000, 13.49389102713827171 ) ) ;
#38506=VECTOR ( 'NONE', #17989, 999.9999999999998863 ) ;
#38507=DIRECTION ( 'NONE',  ( 0.000000000000000000, -1.000000000000000000, 0.000000000000000000 ) ) ;
#38508=AXIS2_PLACEMENT_3D ( 'NONE', #21099, #50656, #11750 ) ;
#38510=PLANE ( 'NONE',  #51911 ) ;
#38511=EDGE_LOOP ( 'NONE', ( #13958, #42970, #8, #16991 ) ) ;
#38512=DIRECTION ( 'NONE',  ( -0.5449076811759708816, 0.6444004775717707689, 0.5364919789714475140 ) ) ;
#38513=EDGE_LOOP ( 'NONE', ( #18984, #6127, #21888, #15718 ) ) ;
#38514=ADVANCED_FACE ( 'NONE', ( #12591 ), #46653, .F. ) ;
#38515=VERTEX_POINT ( 'NONE', #21085 ) ;
#38516=AXIS2_PLACEMENT_3D ( 'NONE', #15312, #10779, #6507 ) ;
#38517=ORIENTED_EDGE ( 'NONE', *, *, #46948, .F. ) ;
#38518=ORIENTED_EDGE ( 'NONE', *, *, #4003, .F. ) ;
#38519=ORIENTED_EDGE ( 'NONE', *, *, #44656, .F. ) ;
#38520=VECTOR ( 'NONE', #26439, 1000.000000000000227 ) ;
#38521=VERTEX_POINT ( 'NONE', #25365 ) ;
#38522=CARTESIAN_POINT ( 'NONE',  ( -20.06177075545399191, 0.000000000000000000, 14.76272000528038220 ) ) ;
#38523=LINE ( 'NONE', #52149, #14811 ) ;
#38524=DIRECTION ( 'NONE',  ( -0.9999697198139514409, -0.000000000000000000, -0.007781995580013368816 ) ) ;
#38525=VECTOR ( 'NONE', #45007, 1000.000000000000227 ) ;
#38526=EDGE_CURVE ( 'NONE', #46316, #14388, #12859, .T. ) ;
#38527=VERTEX_POINT ( 'NONE', #12311 ) ;
#38528=DIRECTION ( 'NONE',  ( -0.9999697198139514409, -0.000000000000000000, -0.007781995580013368816 ) ) ;
#38529=ORIENTED_EDGE ( 'NONE', *, *, #22753, .F. ) ;
#38530=VECTOR ( 'NONE', #5722, 1000.000000000000227 ) ;
#38531=DIRECTION ( 'NONE',  ( -0.5364919789714478471, 0.6444004775717705469, -0.5449076811759709926 ) ) ;
#38532=EDGE_CURVE ( 'NONE', #50552, #2262, #37577, .T. ) ;
#38533=ORIENTED_EDGE ( 'NONE', *, *, #960, .F. ) ;
#38534=EDGE_CURVE ( 'NONE', #40212, #8731, #29650, .T. ) ;
#38535=VECTOR ( 'NONE', #12898, 1000.000000000000000 ) ;
#38536=VECTOR ( 'NONE', #46033, 1000.000000000000227 ) ;
#38537=DIRECTION ( 'NONE',  ( -0.9999697198139514409, -0.000000000000000000, -0.007781995580013368816 ) ) ;
#38538=VECTOR ( 'NONE', #5404, 1000.000000000000000 ) ;
#38539=VECTOR ( 'NONE', #12692, 1000.000000000000227 ) ;
#38540=DIRECTION ( 'NONE',  ( 0.6427681459581294776, -0.7660444431189769032, 0.005002170337467562802 ) ) ;
#38542=ADVANCED_FACE ( 'NONE', ( #55741 ), #47207, .F. ) ;
#38543=ORIENTED_EDGE ( 'NONE', *, *, #44192, .F. ) ;
#38544=CARTESIAN_POINT ( 'NONE',  ( -14.93495759592298988, 0.000000000000000000, 12.77129166681078409 ) ) ;
#38545=ORIENTED_EDGE ( 'NONE', *, *, #32372, .F. ) ;
#38547=PLANE ( 'NONE',  #19162 ) ;
#38548=EDGE_CURVE ( 'NONE', #1131, #55375, #8610, .T. ) ;
#38549=LINE ( 'NONE', #55879, #47484 ) ;
#38550=EDGE_CURVE ( 'NONE', #10988, #24338, #54901, .T. ) ;
#38551=VECTOR ( 'NONE', #35878, 1000.000000000000114 ) ;
#38552=CARTESIAN_POINT ( 'NONE',  ( -12.70458494993575194, -0.1191753592594197858, 11.86531876794841978 ) ) ;
#38553=AXIS2_PLACEMENT_3D ( 'NONE', #38474, #16916, #29961 ) ;
#38554=LINE ( 'NONE', #47338, #50368 ) ;
#38555=DIRECTION ( 'NONE',  ( 0.9999697198139515519, 0.000000000000000000, 0.007781995580013368816 ) ) ;
#38556=DIRECTION ( 'NONE',  ( 0.9999697198139515519, 0.000000000000000000, 0.007781995580013368816 ) ) ;
#38557=CARTESIAN_POINT ( 'NONE',  ( -20.96692673303604337, 2.553033558614007603, 9.215550515739858284 ) ) ;
#38558=CARTESIAN_POINT ( 'NONE',  ( -10.88568941143365087, -10.49235224760979435, 1.009997871305523320 ) ) ;
#38559=ORIENTED_EDGE ( 'NONE', *, *, #20968, .T. ) ;
#38560=DIRECTION ( 'NONE',  ( -0.5449076811759708816, 0.6444004775717707689, 0.5364919789714475140 ) ) ;
#38561=EDGE_LOOP ( 'NONE', ( #8652, #56191, #40711, #49143 ) ) ;
#38562=EDGE_CURVE ( 'NONE', #10029, #43081, #24791, .T. ) ;
#38563=DIRECTION ( 'NONE',  ( 0.5449076811759707706, 0.6444004775717708799, -0.5364919789714476250 ) ) ;
#38564=CARTESIAN_POINT ( 'NONE',  ( -21.47419595591918906, 0.000000000000000000, 5.222628093224860102 ) ) ;
#38565=CARTESIAN_POINT ( 'NONE',  ( -16.31670919488976779, -1.165603555308156736, 4.932849712129135256 ) ) ;
#38566=DIRECTION ( 'NONE',  ( 0.9999697198139515519, 0.000000000000000000, 0.007781995580013368816 ) ) ;
#38567=DIRECTION ( 'NONE',  ( 0.6427681459581294776, -0.7660444431189769032, 0.005002170337467562802 ) ) ;
#38568=AXIS2_PLACEMENT_3D ( 'NONE', #50914, #55193, #20263 ) ;
#38569=ADVANCED_FACE ( 'NONE', ( #48903 ), #35855, .F. ) ;
#38570=DIRECTION ( 'NONE',  ( 0.6427681459581294776, -0.7660444431189769032, 0.005002170337467562802 ) ) ;
#38571=VECTOR ( 'NONE', #50176, 1000.000000000000000 ) ;
#38573=CARTESIAN_POINT ( 'NONE',  ( -19.60990026154428278, 0.000000000000000000, 4.498472333781370125 ) ) ;
#38574=CARTESIAN_POINT ( 'NONE',  ( -16.06709938707323460, 0.000000000000000000, 13.13181314741652628 ) ) ;
#38575=LINE ( 'NONE', #7088, #47229 ) ;
#38577=DIRECTION ( 'NONE',  ( 0.007781995580012662783, 0.000000000000000000, -0.9999697198139514409 ) ) ;
#38578=VECTOR ( 'NONE', #18945, 1000.000000000000227 ) ;
#38579=FACE_OUTER_BOUND ( 'NONE', #8208, .T. ) ;
#38580=DIRECTION ( 'NONE',  ( 0.005002170337468016433, -0.7660444431189770143, -0.6427681459581293666 ) ) ;
#38581=CARTESIAN_POINT ( 'NONE',  ( -16.97387228093712253, 4.495856970884011261, 3.131718784769318198 ) ) ;
#38582=EDGE_LOOP ( 'NONE', ( #49946, #39679, #48523, #39365, #40299, #1761, #6029, #17777, #55528, #25008, #48803, #40246, #7214, #43476, #16533, #20204, #51859, #26726, #48539, #44968, #17278, #45215, #38996, #24296, #25398, #28540, #10742, #751, #39084, #146, #2040, #51644, #15742, #36039, #21906, #20924, #51277, #11408, #42797, #43740, #33230, #32390, #40134, #19945, #51530, #21333, #55332, #19230, #54187, #8871, #53307, #39191, #22679, #51972, #30843, #50490, #28943, #26218, #41283, #41170, #53121, #13123, #7294, #40087, #7790, #25749, #31700, #13472, #23414, #42623, #42557, #8118, #20242, #51493, #22726, #25327, #52633, #14602, #4949, #45895, #13035, #26597, #54658, #31039, #5024, #36703, #9629, #25402, #54788, #53526, #27084, #53673, #50904, #28390, #11447, #11339, #30156, #3119, #9843, #51098, #47538, #921, #51517 ) ) ;
#38583=DIRECTION ( 'NONE',  ( -0.005961354470445682716, -0.6427876096865404731, 0.7660212471507180654 ) ) ;
#38584=VECTOR ( 'NONE', #9977, 999.9999999999998863 ) ;
#38585=DIRECTION ( 'NONE',  ( -0.5364919789714478471, 0.6444004775717705469, -0.5449076811759709926 ) ) ;
#38587=EDGE_LOOP ( 'NONE', ( #14763, #45319, #14650, #36944 ) ) ;
#38588=ORIENTED_EDGE ( 'NONE', *, *, #8336, .T. ) ;
#38589=CARTESIAN_POINT ( 'NONE',  ( -16.53317331066696383, 0.000000000000000000, 13.31285208727739899 ) ) ;
#38590=VECTOR ( 'NONE', #34873, 1000.000000000000227 ) ;
#38591=ORIENTED_EDGE ( 'NONE', *, *, #12956, .T. ) ;
#38592=VECTOR ( 'NONE', #15400, 1000.000000000000114 ) ;
#38593=EDGE_CURVE ( 'NONE', #4269, #42201, #53178, .T. ) ;
#38594=AXIS2_PLACEMENT_3D ( 'NONE', #23450, #37062, #50090 ) ;
#38595=EDGE_LOOP ( 'NONE', ( #18498, #29827, #44429, #40695 ) ) ;
#38596=AXIS2_PLACEMENT_3D ( 'NONE', #25630, #34183, #47496 ) ;
#38597=VERTEX_POINT ( 'NONE', #903 ) ;
#38598=ORIENTED_EDGE ( 'NONE', *, *, #26493, .F. ) ;
#38599=DIRECTION ( 'NONE',  ( 0.9999697198139515519, 0.000000000000000000, 0.007781995580013368816 ) ) ;
#38600=EDGE_LOOP ( 'NONE', ( #15483, #41500, #11471, #53118 ) ) ;
#38601=CARTESIAN_POINT ( 'NONE',  ( -9.499406503593807116, 0.000000000000000000, 5.115812617421968689 ) ) ;
#38602=DIRECTION ( 'NONE',  ( 0.5364919789714477361, 0.6444004775717706579, 0.5449076811759711036 ) ) ;
#38603=ORIENTED_EDGE ( 'NONE', *, *, #27786, .T. ) ;
#38604=VERTEX_POINT ( 'NONE', #13687 ) ;
#38605=EDGE_CURVE ( 'NONE', #2042, #40517, #26761, .T. ) ;
#38606=AXIS2_PLACEMENT_3D ( 'NONE', #49483, #18831, #31320 ) ;
#38607=FACE_OUTER_BOUND ( 'NONE', #3457, .T. ) ;
#38608=FACE_OUTER_BOUND ( 'NONE', #24069, .T. ) ;
#38609=AXIS2_PLACEMENT_3D ( 'NONE', #27092, #52379, #8944 ) ;
#38610=ORIENTED_EDGE ( 'NONE', *, *, #7137, .T. ) ;
#38611=DIRECTION ( 'NONE',  ( -0.005002170337468016433, -0.7660444431189770143, 0.6427681459581293666 ) ) ;
#38612=CARTESIAN_POINT ( 'NONE',  ( -28.93060053386082231, -0.1191753592594197858, 8.019254159017428663 ) ) ;
#38613=ORIENTED_EDGE ( 'NONE', *, *, #49709, .T. ) ;
#38614=VECTOR ( 'NONE', #12997, 1000.000000000000227 ) ;
#38615=DIRECTION ( 'NONE',  ( 0.000000000000000000, -0.000000000000000000, -1.000000000000000000 ) ) ;
#38616=ORIENTED_EDGE ( 'NONE', *, *, #49135, .T. ) ;
#38617=CARTESIAN_POINT ( 'NONE',  ( 2.072287782118878319, 0.000000000000000000, -2.950529333540147015 ) ) ;
#38618=ADVANCED_FACE ( 'NONE', ( #48320 ), #39558, .F. ) ;
#38619=VECTOR ( 'NONE', #7687, 1000.000000000000227 ) ;
#38620=EDGE_CURVE ( 'NONE', #14391, #45526, #35554, .T. ) ;
#38621=CARTESIAN_POINT ( 'NONE',  ( -12.60458797795435615, 0.000000000000000000, 11.86609696750642229 ) ) ;
#38623=VECTOR ( 'NONE', #6921, 1000.000000000000114 ) ;
#38624=ORIENTED_EDGE ( 'NONE', *, *, #19148, .F. ) ;
#38625=DIRECTION ( 'NONE',  ( -0.6427681459581293666, -0.7660444431189770143, -0.005002170337467561935 ) ) ;
#38626=CARTESIAN_POINT ( 'NONE',  ( -15.60102546347950536, 0.000000000000000000, 12.95077420755565356 ) ) ;
#38627=DIRECTION ( 'NONE',  ( 0.5364919789714477361, 0.6444004775717706579, 0.5449076811759711036 ) ) ;
#38628=EDGE_CURVE ( 'NONE', #23457, #33064, #52864, .T. ) ;
#38629=VECTOR ( 'NONE', #7536, 999.9999999999998863 ) ;
#38630=CARTESIAN_POINT ( 'NONE',  ( -21.47419595591918906, 0.000000000000000000, 5.222628093224860102 ) ) ;
#38631=ORIENTED_EDGE ( 'NONE', *, *, #3653, .T. ) ;
#38632=VECTOR ( 'NONE', #8061, 999.9999999999998863 ) ;
#38633=EDGE_CURVE ( 'NONE', #38231, #48589, #21927, .T. ) ;
#38634=VECTOR ( 'NONE', #20014, 1000.000000000000227 ) ;
#38635=DIRECTION ( 'NONE',  ( 0.5449076811759707706, 0.6444004775717708799, -0.5364919789714476250 ) ) ;
#38636=DIRECTION ( 'NONE',  ( -0.5364919789714478471, 0.6444004775717705469, -0.5449076811759709926 ) ) ;
#38637=CARTESIAN_POINT ( 'NONE',  ( -12.07573772665640099, 0.000000000000000000, 3.618434732898855977 ) ) ;
#38638=FACE_OUTER_BOUND ( 'NONE', #21074, .T. ) ;
#38639=CARTESIAN_POINT ( 'NONE',  ( -13.73672976910459909, 0.000000000000000000, 12.22661844811216270 ) ) ;
#38640=LINE ( 'NONE', #41744, #2501 ) ;
#38641=VECTOR ( 'NONE', #40637, 1000.000000000000000 ) ;
#38642=EDGE_CURVE ( 'NONE', #29025, #18181, #27048, .T. ) ;
#38643=VECTOR ( 'NONE', #44240, 999.9999999999998863 ) ;
#38644=DIRECTION ( 'NONE',  ( 0.000000000000000000, -1.000000000000000000, 0.000000000000000000 ) ) ;
#38645=CARTESIAN_POINT ( 'NONE',  ( -16.81267852042391198, -0.1191753592594197858, 3.312241722634738039 ) ) ;
#38646=ORIENTED_EDGE ( 'NONE', *, *, #34159, .T. ) ;
#38647=CARTESIAN_POINT ( 'NONE',  ( -16.46189419481024885, 0.000000000000000000, 4.153638775091319957 ) ) ;
#38648=ORIENTED_EDGE ( 'NONE', *, *, #36940, .F. ) ;
#38649=PLANE ( 'NONE',  #39283 ) ;
#38650=CARTESIAN_POINT ( 'NONE',  ( 2.072287782118878319, 0.000000000000000000, -2.950529333540147015 ) ) ;
#38651=LINE ( 'NONE', #51127, #53979 ) ;
#38652=DIRECTION ( 'NONE',  ( -0.8531650599175529814, -0.4028455766673920135, 0.3313982828793697877 ) ) ;
#38653=FACE_OUTER_BOUND ( 'NONE', #15135, .T. ) ;
#38654=VECTOR ( 'NONE', #34273, 999.9999999999998863 ) ;
#38655=EDGE_LOOP ( 'NONE', ( #22880, #1001, #46243, #17666 ) ) ;
#38656=ORIENTED_EDGE ( 'NONE', *, *, #29460, .T. ) ;
#38657=PLANE ( 'NONE',  #26814 ) ;
#38658=CARTESIAN_POINT ( 'NONE',  ( -3.941126747678045827, 5.958485271846477360, -1.687506105637922360 ) ) ;
#38659=ORIENTED_EDGE ( 'NONE', *, *, #36359, .F. ) ;
#38660=AXIS2_PLACEMENT_3D ( 'NONE', #33589, #33879, #8054 ) ;
#38661=EDGE_CURVE ( 'NONE', #428, #16370, #13973, .T. ) ;
#38663=CARTESIAN_POINT ( 'NONE',  ( -21.47419595591918906, 0.000000000000000000, 5.222628093224860102 ) ) ;
#38664=ORIENTED_EDGE ( 'NONE', *, *, #43413, .T. ) ;
#38665=LINE ( 'NONE', #288, #18617 ) ;
#38666=VECTOR ( 'NONE', #3780, 1000.000000000000227 ) ;
#38667=EDGE_CURVE ( 'NONE', #13188, #9765, #30482, .T. ) ;
#38668=VERTEX_POINT ( 'NONE', #5457 ) ;
#38669=CARTESIAN_POINT ( 'NONE',  ( -9.965599799550892257, 0.000000000000000000, 5.312190649616747251 ) ) ;
#38670=VECTOR ( 'NONE', #37102, 1000.000000000000227 ) ;
#38671=ORIENTED_EDGE ( 'NONE', *, *, #55505, .T. ) ;
#38672=ORIENTED_EDGE ( 'NONE', *, *, #33372, .F. ) ;
#38673=ORIENTED_EDGE ( 'NONE', *, *, #6738, .T. ) ;
#38674=ADVANCED_FACE ( 'NONE', ( #22771 ), #40091, .F. ) ;
#38675=CARTESIAN_POINT ( 'NONE',  ( -10.69487964927027868, 0.000000000000000000, 5.306515225196732466 ) ) ;
#38676=LINE ( 'NONE', #3724, #29610 ) ;
#38677=LINE ( 'NONE', #38094, #39355 ) ;
#38678=EDGE_CURVE ( 'NONE', #51439, #5375, #21671, .T. ) ;
#38680=EDGE_CURVE ( 'NONE', #55993, #1154, #17386, .T. ) ;
#38681=EDGE_CURVE ( 'NONE', #39497, #16451, #13149, .T. ) ;
#38682=VECTOR ( 'NONE', #47193, 1000.000000000000000 ) ;
#38683=DIRECTION ( 'NONE',  ( -0.005961354470445682716, -0.6427876096865404731, 0.7660212471507180654 ) ) ;
#38684=ORIENTED_EDGE ( 'NONE', *, *, #475, .T. ) ;
#38685=ORIENTED_EDGE ( 'NONE', *, *, #10711, .T. ) ;
#38686=VECTOR ( 'NONE', #42229, 999.9999999999998863 ) ;
#38687=VECTOR ( 'NONE', #26275, 1000.000000000000114 ) ;
#38688=VERTEX_POINT ( 'NONE', #26209 ) ;
#38689=CARTESIAN_POINT ( 'NONE',  ( -15.31350409040604887, -1.651309408375657206, 2.776920739002065819 ) ) ;
#38690=CARTESIAN_POINT ( 'NONE',  ( 2.072287782118878319, 0.000000000000000000, -2.950529333540147015 ) ) ;
#38691=VERTEX_POINT ( 'NONE', #43512 ) ;
#38693=VERTEX_POINT ( 'NONE', #4614 ) ;
#38694=LINE ( 'NONE', #42383, #30566 ) ;
#38695=DIRECTION ( 'NONE',  ( 0.9999697198139515519, 0.000000000000000000, 0.007781995580013368816 ) ) ;
#38696=ORIENTED_EDGE ( 'NONE', *, *, #35043, .T. ) ;
#38697=CARTESIAN_POINT ( 'NONE',  ( -11.47086027511496731, 1.257817950434005461, 3.401286344105265869 ) ) ;
#38698=EDGE_CURVE ( 'NONE', #30522, #42624, #39255, .T. ) ;
#38699=ORIENTED_EDGE ( 'NONE', *, *, #23298, .T. ) ;
#38700=EDGE_CURVE ( 'NONE', #17943, #16783, #52335, .T. ) ;
#38701=VECTOR ( 'NONE', #36963, 999.9999999999998863 ) ;
#38703=DIRECTION ( 'NONE',  ( 0.005002170337468016433, -0.7660444431189770143, -0.6427681459581293666 ) ) ;
#38704=DIRECTION ( 'NONE',  ( -0.5449076811759708816, 0.6444004775717707689, 0.5364919789714475140 ) ) ;
#38705=ORIENTED_EDGE ( 'NONE', *, *, #16183, .T. ) ;
#38706=CARTESIAN_POINT ( 'NONE',  ( -11.22056963685719211, 0.000000000000000000, 1.239771416285661010 ) ) ;
#38707=DIRECTION ( 'NONE',  ( 0.5364919789714477361, 0.6444004775717706579, 0.5449076811759711036 ) ) ;
#38708=EDGE_CURVE ( 'NONE', #37378, #9864, #28993, .T. ) ;
#38709=PLANE ( 'NONE',  #45496 ) ;
#38710=VERTEX_POINT ( 'NONE', #47142 ) ;
#38711=EDGE_CURVE ( 'NONE', #29528, #43061, #51122, .T. ) ;
#38712=DIRECTION ( 'NONE',  ( 0.6427681459581294776, -0.7660444431189769032, 0.005002170337467562802 ) ) ;
#38715=CARTESIAN_POINT ( 'NONE',  ( -26.13337879274045505, 0.000000000000000000, 6.833023547870798353 ) ) ;
#38716=LINE ( 'NONE', #48048, #3102 ) ;
#38717=EDGE_CURVE ( 'NONE', #56109, #55993, #42882, .T. ) ;
#38718=DIRECTION ( 'NONE',  ( 0.007781995580012663651, 0.000000000000000000, -0.9999697198139515519 ) ) ;
#38720=DIRECTION ( 'NONE',  ( -0.6427681459581293666, -0.7660444431189770143, -0.005002170337467561935 ) ) ;
#38721=ORIENTED_EDGE ( 'NONE', *, *, #36066, .F. ) ;
#38722=PLANE ( 'NONE',  #32552 ) ;
#38724=DIRECTION ( 'NONE',  ( 0.007781995580012663651, 0.000000000000000000, -0.9999697198139515519 ) ) ;
#38725=ORIENTED_EDGE ( 'NONE', *, *, #15380, .T. ) ;
#38726=DIRECTION ( 'NONE',  ( 0.007781995580012662783, 0.000000000000000000, -0.9999697198139514409 ) ) ;
#38727=LINE ( 'NONE', #46800, #38614 ) ;
#38728=ORIENTED_EDGE ( 'NONE', *, *, #43846, .T. ) ;
#38729=PLANE ( 'NONE',  #49768 ) ;
#38730=LINE ( 'NONE', #55746, #26037 ) ;
#38731=VECTOR ( 'NONE', #17829, 999.9999999999998863 ) ;
#38732=PLANE ( 'NONE',  #22362 ) ;
#38734=ORIENTED_EDGE ( 'NONE', *, *, #30277, .F. ) ;
#38735=VECTOR ( 'NONE', #17919, 1000.000000000000227 ) ;
#38736=EDGE_LOOP ( 'NONE', ( #30579, #1686, #27142, #47143 ) ) ;
#38737=LINE ( 'NONE', #55460, #12196 ) ;
#38738=DIRECTION ( 'NONE',  ( 0.007781995580012663651, 0.000000000000000000, -0.9999697198139515519 ) ) ;
#38739=CARTESIAN_POINT ( 'NONE',  ( -13.53673582514181106, 0.000000000000000000, 12.22817484722816772 ) ) ;
#38740=CARTESIAN_POINT ( 'NONE',  ( -12.09585610119338028, 0.000000000000000000, 6.203602655703208235 ) ) ;
#38741=DIRECTION ( 'NONE',  ( 0.005002170337468016433, -0.7660444431189770143, -0.6427681459581293666 ) ) ;
#38742=CARTESIAN_POINT ( 'NONE',  ( -26.13493519185646008, 0.000000000000000000, 7.033017491833586377 ) ) ;
#38743=EDGE_LOOP ( 'NONE', ( #51185, #20883, #31308, #38829 ) ) ;
#38744=DIRECTION ( 'NONE',  ( 0.7660212471507180654, -0.6427876096865404731, 0.005961354470445141482 ) ) ;
#38745=VECTOR ( 'NONE', #1150, 999.9999999999998863 ) ;
#38746=CARTESIAN_POINT ( 'NONE',  ( -17.26532721389163072, 0.000000000000000000, 13.67648636611514590 ) ) ;
#38747=ORIENTED_EDGE ( 'NONE', *, *, #24140, .T. ) ;
#38748=FACE_OUTER_BOUND ( 'NONE', #12886, .T. ) ;
#38749=LINE ( 'NONE', #55772, #10524 ) ;
#38750=PLANE ( 'NONE',  #21185 ) ;
#38751=EDGE_CURVE ( 'NONE', #50517, #44961, #46290, .T. ) ;
#38752=ADVANCED_FACE ( 'NONE', ( #2839 ), #46576, .F. ) ;
#38754=CARTESIAN_POINT ( 'NONE',  ( -20.03163450426368541, -1.165603555308156514, 4.625099379789840981 ) ) ;
#38755=VECTOR ( 'NONE', #9462, 1000.000000000000227 ) ;
#38756=ORIENTED_EDGE ( 'NONE', *, *, #6060, .F. ) ;
#38757=ADVANCED_FACE ( 'NONE', ( #8246 ), #25560, .F. ) ;
#38758=EDGE_LOOP ( 'NONE', ( #53213, #2433, #40354, #9068 ) ) ;
#38759=VECTOR ( 'NONE', #40472, 1000.000000000000227 ) ;
#38760=ORIENTED_EDGE ( 'NONE', *, *, #51382, .T. ) ;
#38761=ORIENTED_EDGE ( 'NONE', *, *, #52916, .F. ) ;
#38762=CARTESIAN_POINT ( 'NONE',  ( -16.48077548314530461, 3.848249166794009746, 9.598646491548270987 ) ) ;
#38763=ORIENTED_EDGE ( 'NONE', *, *, #45467, .F. ) ;
#38764=LINE ( 'NONE', #17734, #36716 ) ;
#38765=VECTOR ( 'NONE', #18285, 1000.000000000000227 ) ;
#38766=VERTEX_POINT ( 'NONE', #38647 ) ;
#38769=LINE ( 'NONE', #13196, #31076 ) ;
#38770=ORIENTED_EDGE ( 'NONE', *, *, #480, .F. ) ;
#38771=CARTESIAN_POINT ( 'NONE',  ( -19.63082162219014748, -0.1191753592594168992, 6.244966839838443917 ) ) ;
#38772=LINE ( 'NONE', #43564, #11421 ) ;
#38773=CARTESIAN_POINT ( 'NONE',  ( -19.50285499688518343, 4.657758921906511418, 12.10106822468943655 ) ) ;
#38774=DIRECTION ( 'NONE',  ( 0.000000000000000000, -1.000000000000000000, 0.000000000000000000 ) ) ;
#38775=DIRECTION ( 'NONE',  ( 0.005961354470445682716, -0.6427876096865404731, -0.7660212471507180654 ) ) ;
#38776=ORIENTED_EDGE ( 'NONE', *, *, #34825, .F. ) ;
#38777=ADVANCED_FACE ( 'NONE', ( #55377 ), #16475, .F. ) ;
#38778=VERTEX_POINT ( 'NONE', #29574 ) ;
#38779=CARTESIAN_POINT ( 'NONE',  ( -27.06708303904391144, 0.000000000000000000, 7.395095371555332697 ) ) ;
#38780=DIRECTION ( 'NONE',  ( 0.6427681459581294776, -0.7660444431189769032, 0.005002170337467562802 ) ) ;
#38781=EDGE_CURVE ( 'NONE', #39543, #5013, #15937, .T. ) ;
#38782=PLANE ( 'NONE',  #8857 ) ;
#38783=DIRECTION ( 'NONE',  ( -0.7660212471507179544, -0.6427876096865405842, -0.005961354470445141482 ) ) ;
#38784=EDGE_CURVE ( 'NONE', #35551, #6162, #24443, .T. ) ;
#38785=CARTESIAN_POINT ( 'NONE',  ( 2.072287782118878319, 0.000000000000000000, -2.950529333540147015 ) ) ;
#38786=FACE_OUTER_BOUND ( 'NONE', #52974, .T. ) ;
#38787=VERTEX_POINT ( 'NONE', #11675 ) ;
#38788=LINE ( 'NONE', #38485, #32944 ) ;
#38789=EDGE_CURVE ( 'NONE', #49206, #55415, #16211, .T. ) ;
#38790=CARTESIAN_POINT ( 'NONE',  ( -18.25036719564678123, 1.581621852479005774, 3.720532117565352070 ) ) ;
#38791=ORIENTED_EDGE ( 'NONE', *, *, #17132, .F. ) ;
#38792=DIRECTION ( 'NONE',  ( 0.6427681459581294776, -0.7660444431189769032, 0.005002170337467562802 ) ) ;
#38793=CARTESIAN_POINT ( 'NONE',  ( -10.69619730365955945, 0.000000000000000000, 5.475830984491707909 ) ) ;
#38794=ADVANCED_FACE ( 'NONE', ( #50837 ), #29261, .F. ) ;
#38795=CARTESIAN_POINT ( 'NONE',  ( -18.67775241435682432, 0.000000000000000000, 4.136394454059623804 ) ) ;
#38796=CARTESIAN_POINT ( 'NONE',  ( -17.74404816805336793, 0.000000000000000000, 3.574322630375089460 ) ) ;
#38797=VECTOR ( 'NONE', #52121, 999.9999999999998863 ) ;
#38798=ORIENTED_EDGE ( 'NONE', *, *, #21281, .T. ) ;
#38799=VERTEX_POINT ( 'NONE', #17611 ) ;
#38800=DIRECTION ( 'NONE',  ( -0.5449076811759708816, 0.6444004775717707689, 0.5364919789714475140 ) ) ;
#38801=DIRECTION ( 'NONE',  ( -0.9999697198139514409, -0.000000000000000000, -0.007781995580013368816 ) ) ;
#38802=DIRECTION ( 'NONE',  ( 0.9999697198139515519, 0.000000000000000000, 0.007781995580013368816 ) ) ;
#38803=AXIS2_PLACEMENT_3D ( 'NONE', #40667, #40919, #32433 ) ;
#38804=DIRECTION ( 'NONE',  ( 0.7660212471507180654, -0.6427876096865404731, 0.005961354470445141482 ) ) ;
#38805=PLANE ( 'NONE',  #7661 ) ;
#38806=LINE ( 'NONE', #43349, #25530 ) ;
#38808=VERTEX_POINT ( 'NONE', #38922 ) ;
#38809=DIRECTION ( 'NONE',  ( 0.9999697198139515519, 0.000000000000000000, 0.007781995580013368816 ) ) ;
#38810=LINE ( 'NONE', #17481, #11509 ) ;
#38811=ORIENTED_EDGE ( 'NONE', *, *, #7859, .F. ) ;
#38812=CARTESIAN_POINT ( 'NONE',  ( -16.82487927491429502, -0.1134144341942024126, 3.316980910018160422 ) ) ;
#38813=ORIENTED_EDGE ( 'NONE', *, *, #11205, .F. ) ;
#38815=EDGE_CURVE ( 'NONE', #14388, #4025, #30939, .T. ) ;
#38816=ORIENTED_EDGE ( 'NONE', *, *, #23093, .T. ) ;
#38817=ORIENTED_EDGE ( 'NONE', *, *, #49424, .T. ) ;
#38818=EDGE_CURVE ( 'NONE', #22139, #1353, #40022, .T. ) ;
#38819=EDGE_CURVE ( 'NONE', #8289, #30652, #8535, .T. ) ;
#38820=ORIENTED_EDGE ( 'NONE', *, *, #53779, .T. ) ;
#38821=EDGE_LOOP ( 'NONE', ( #28919, #1648, #32981, #40854 ) ) ;
#38822=ORIENTED_EDGE ( 'NONE', *, *, #1025, .F. ) ;
#38823=ORIENTED_EDGE ( 'NONE', *, *, #54553, .F. ) ;
#38824=LINE ( 'NONE', #38522, #30549 ) ;
#38825=PLANE ( 'NONE',  #19337 ) ;
#38826=CARTESIAN_POINT ( 'NONE',  ( -22.40556560354864146, -0.1191753592594197858, 5.484709000965211523 ) ) ;
#38827=ORIENTED_EDGE ( 'NONE', *, *, #6218, .T. ) ;
#38828=FACE_OUTER_BOUND ( 'NONE', #31793, .T. ) ;
#38829=ORIENTED_EDGE ( 'NONE', *, *, #24306, .F. ) ;
#38830=CARTESIAN_POINT ( 'NONE',  ( -18.62089103150555758, 0.000000000000000000, 8.738147813755425375 ) ) ;
#38831=ORIENTED_EDGE ( 'NONE', *, *, #4133, .F. ) ;
#38833=DIRECTION ( 'NONE',  ( 0.007781995580012663651, 0.000000000000000000, -0.9999697198139515519 ) ) ;
#38834=DIRECTION ( 'NONE',  ( 0.6427681459581294776, -0.7660444431189769032, 0.005002170337467562802 ) ) ;
#38835=DIRECTION ( 'NONE',  ( 0.9999697198139515519, 0.000000000000000000, 0.007781995580013368816 ) ) ;
#38836=ORIENTED_EDGE ( 'NONE', *, *, #10738, .F. ) ;
#38837=FACE_OUTER_BOUND ( 'NONE', #32588, .T. ) ;
#38838=EDGE_LOOP ( 'NONE', ( #28119, #42827, #17967, #11043 ) ) ;
#38839=AXIS2_PLACEMENT_3D ( 'NONE', #8836, #52790, #13619 ) ;
#38840=CARTESIAN_POINT ( 'NONE',  ( -11.82561389535573682, 3.362543313726509719, 1.168119031430539634 ) ) ;
#38841=DIRECTION ( 'NONE',  ( -0.005002170337468016433, -0.7660444431189770143, 0.6427681459581293666 ) ) ;
#38842=EDGE_CURVE ( 'NONE', #39505, #93, #34639, .T. ) ;
#38843=LINE ( 'NONE', #47636, #15134 ) ;
#38844=PLANE ( 'NONE',  #44001 ) ;
#38845=FACE_OUTER_BOUND ( 'NONE', #46525, .T. ) ;
#38846=DIRECTION ( 'NONE',  ( 0.9999697198139515519, 0.000000000000000000, 0.007781995580013368816 ) ) ;
#38847=DIRECTION ( 'NONE',  ( 0.007781995580012662783, 0.000000000000000000, -0.9999697198139514409 ) ) ;
#38849=VERTEX_POINT ( 'NONE', #44299 ) ;
#38850=LINE ( 'NONE', #47927, #38331 ) ;
#38851=ORIENTED_EDGE ( 'NONE', *, *, #54287, .F. ) ;
#38852=CARTESIAN_POINT ( 'NONE',  ( -17.03414339976229996, 4.495856970884009485, 10.87642811861771186 ) ) ;
#38853=LINE ( 'NONE', #56165, #33241 ) ;
#38854=DIRECTION ( 'NONE',  ( 0.000000000000000000, -0.000000000000000000, -1.000000000000000000 ) ) ;
#38855=EDGE_CURVE ( 'NONE', #34418, #10029, #18444, .T. ) ;
#38856=CARTESIAN_POINT ( 'NONE',  ( -20.08582687197957029, 2.067327705546507133, 8.076175355576905801 ) ) ;
#38857=CARTESIAN_POINT ( 'NONE',  ( -14.49969738240122474, -0.1191753592594189115, 3.699573946482198394 ) ) ;
#38858=DIRECTION ( 'NONE',  ( 0.6246952433987894571, -0.7422098413412800966, -0.2426528472758541777 ) ) ;
#38859=DIRECTION ( 'NONE',  ( 0.7660212471507180654, -0.6427876096865404731, 0.005961354470445141482 ) ) ;
#38861=ORIENTED_EDGE ( 'NONE', *, *, #39966, .F. ) ;
#38863=DIRECTION ( 'NONE',  ( -0.9999697198139514409, -0.000000000000000000, -0.007781995580013368816 ) ) ;
#38864=CARTESIAN_POINT ( 'NONE',  ( -11.40636015113596180, 0.000000000000000000, 11.32142374880780089 ) ) ;
#38865=EDGE_CURVE ( 'NONE', #43820, #5084, #39763, .T. ) ;
#38866=CARTESIAN_POINT ( 'NONE',  ( -24.26908309836554878, 0.000000000000000000, 6.108867788427308376 ) ) ;
#38867=DIRECTION ( 'NONE',  ( -0.005002170337468016433, -0.7660444431189770143, 0.6427681459581293666 ) ) ;
#38868=EDGE_CURVE ( 'NONE', #36173, #44387, #31228, .T. ) ;
#38869=DIRECTION ( 'NONE',  ( -0.5364919789714478471, 0.6444004775717705469, -0.5449076811759709926 ) ) ;
#38870=EDGE_CURVE ( 'NONE', #17707, #25181, #13622, .T. ) ;
#38871=CARTESIAN_POINT ( 'NONE',  ( -15.88579177843824830, -0.1166911823299096179, 2.952207434841243927 ) ) ;
#38875=ORIENTED_EDGE ( 'NONE', *, *, #17940, .T. ) ;
#38877=FACE_OUTER_BOUND ( 'NONE', #4724, .T. ) ;
#38878=EDGE_CURVE ( 'NONE', #19762, #20122, #22152, .T. ) ;
#38880=VERTEX_POINT ( 'NONE', #9365 ) ;
#38881=ADVANCED_FACE ( 'NONE', ( #18161 ), #30110, .F. ) ;
#38883=ORIENTED_EDGE ( 'NONE', *, *, #45821, .F. ) ;
#38884=ORIENTED_EDGE ( 'NONE', *, *, #13399, .F. ) ;
#38885=ORIENTED_EDGE ( 'NONE', *, *, #42096, .T. ) ;
#38886=LINE ( 'NONE', #749, #13940 ) ;
#38887=ORIENTED_EDGE ( 'NONE', *, *, #26772, .F. ) ;
#38888=LINE ( 'NONE', #52226, #16919 ) ;
#38889=LINE ( 'NONE', #26112, #3099 ) ;
#38890=ADVANCED_FACE ( 'NONE', ( #842 ), #34951, .F. ) ;
#38891=EDGE_CURVE ( 'NONE', #35565, #26804, #43711, .T. ) ;
#38892=ORIENTED_EDGE ( 'NONE', *, *, #28065, .F. ) ;
#38893=ORIENTED_EDGE ( 'NONE', *, *, #6602, .F. ) ;
#38894=EDGE_CURVE ( 'NONE', #12052, #30300, #26988, .T. ) ;
#38896=ORIENTED_EDGE ( 'NONE', *, *, #16425, .F. ) ;
#38897=DIRECTION ( 'NONE',  ( 0.000000000000000000, -1.000000000000000000, 0.000000000000000000 ) ) ;
#38898=DIRECTION ( 'NONE',  ( -0.9999697198139514409, -0.000000000000000000, -0.007781995580013368816 ) ) ;
#38899=ORIENTED_EDGE ( 'NONE', *, *, #1674, .F. ) ;
#38900=LINE ( 'NONE', #47120, #42127 ) ;
#38901=VERTEX_POINT ( 'NONE', #52531 ) ;
#38902=DIRECTION ( 'NONE',  ( 0.7660212471507180654, -0.6427876096865404731, 0.005961354470445141482 ) ) ;
#38903=DIRECTION ( 'NONE',  ( -0.8531650599175527594, 0.4028455766673922356, 0.3313982828793700652 ) ) ;
#38904=ORIENTED_EDGE ( 'NONE', *, *, #23589, .T. ) ;
#38905=DIRECTION ( 'NONE',  ( 0.000000000000000000, -1.000000000000000000, 0.000000000000000000 ) ) ;
#38906=CARTESIAN_POINT ( 'NONE',  ( -7.148249425445639460, -2.280392264726430529, 8.590678399319719105 ) ) ;
#38907=FACE_OUTER_BOUND ( 'NONE', #31282, .T. ) ;
#38908=CARTESIAN_POINT ( 'NONE',  ( -18.67697421479882181, -0.1191753592594197858, 4.036397482078229793 ) ) ;
#38909=ORIENTED_EDGE ( 'NONE', *, *, #18108, .T. ) ;
#38911=FACE_OUTER_BOUND ( 'NONE', #224, .T. ) ;
#38912=LINE ( 'NONE', #48239, #628 ) ;
#38913=CARTESIAN_POINT ( 'NONE',  ( -20.18792284424153038, 1.095915999411505082, 6.521580794694486372 ) ) ;
#38914=DIRECTION ( 'NONE',  ( 0.000000000000000000, -1.000000000000000000, 0.000000000000000000 ) ) ;
#38915=EDGE_CURVE ( 'NONE', #15160, #42447, #5399, .T. ) ;
#38916=DIRECTION ( 'NONE',  ( 0.2426528472758541499, 0.7422098413412800966, 0.6246952433987894571 ) ) ;
#38917=LINE ( 'NONE', #263, #43091 ) ;
#38918=CARTESIAN_POINT ( 'NONE',  ( -17.28610440469613252, -0.1191753592594162470, 3.496136413696765644 ) ) ;
#38919=CARTESIAN_POINT ( 'NONE',  ( -9.948355478519198769, 0.000000000000000000, 3.096332430070161124 ) ) ;
#38920=LINE ( 'NONE', #51955, #48556 ) ;
#38921=ORIENTED_EDGE ( 'NONE', *, *, #49337, .F. ) ;
#38922=CARTESIAN_POINT ( 'NONE',  ( -13.58479385624546865, -0.1191753592594188005, 5.553354286307040866 ) ) ;
#38923=ORIENTED_EDGE ( 'NONE', *, *, #5060, .T. ) ;
#38924=DIRECTION ( 'NONE',  ( -0.6427681459581293666, -0.7660444431189770143, -0.005002170337467561935 ) ) ;
#38925=DIRECTION ( 'NONE',  ( 0.005002170337468016433, -0.7660444431189770143, -0.6427681459581293666 ) ) ;
#38926=EDGE_CURVE ( 'NONE', #33548, #19751, #25867, .T. ) ;
#38927=CARTESIAN_POINT ( 'NONE',  ( -10.47421230394850866, 0.000000000000000000, 10.95934586908605723 ) ) ;
#38928=ADVANCED_FACE ( 'NONE', ( #43452 ), #17317, .F. ) ;
#38929=LINE ( 'NONE', #13083, #1549 ) ;
#38930=ADVANCED_FACE ( 'NONE', ( #36329 ), #36079, .F. ) ;
#38931=CARTESIAN_POINT ( 'NONE',  ( -26.13493519185646008, 0.000000000000000000, 7.033017491833586377 ) ) ;
#38932=VERTEX_POINT ( 'NONE', #49925 ) ;
#38933=ORIENTED_EDGE ( 'NONE', *, *, #52111, .T. ) ;
#38934=DIRECTION ( 'NONE',  ( 0.007781995580012662783, 0.000000000000000000, -0.9999697198139514409 ) ) ;
#38935=CARTESIAN_POINT ( 'NONE',  ( -28.92982233430281980, 0.000000000000000000, 7.919257187036034651 ) ) ;
#38936=ORIENTED_EDGE ( 'NONE', *, *, #11863, .T. ) ;
#38937=CARTESIAN_POINT ( 'NONE',  ( -17.36532418587302473, -0.1191753592594177458, 13.67570816655714516 ) ) ;
#38938=ORIENTED_EDGE ( 'NONE', *, *, #50766, .T. ) ;
#38939=ADVANCED_FACE ( 'NONE', ( #6790 ), #53638, .F. ) ;
#38940=CARTESIAN_POINT ( 'NONE',  ( -12.00530485164738970, 0.000000000000000000, 7.881641681912517683 ) ) ;
#38941=ORIENTED_EDGE ( 'NONE', *, *, #16428, .F. ) ;
#38942=DIRECTION ( 'NONE',  ( 0.007781995580012663651, 0.000000000000000000, -0.9999697198139515519 ) ) ;
#38943=EDGE_CURVE ( 'NONE', #4182, #36112, #14744, .T. ) ;
#38944=VERTEX_POINT ( 'NONE', #53381 ) ;
#38945=EDGE_LOOP ( 'NONE', ( #16595, #11054, #18255, #5792 ) ) ;
#38946=ORIENTED_EDGE ( 'NONE', *, *, #43705, .T. ) ;
#38947=DIRECTION ( 'NONE',  ( 0.007781995580012662783, 0.000000000000000000, -0.9999697198139514409 ) ) ;
#38948=CARTESIAN_POINT ( 'NONE',  ( -9.027703845352876399, 0.000000000000000000, 4.211493363379472221 ) ) ;
#38949=DIRECTION ( 'NONE',  ( -0.005002170337468016433, -0.7660444431189770143, 0.6427681459581293666 ) ) ;
#38950=EDGE_CURVE ( 'NONE', #19740, #2, #28350, .T. ) ;
#38951=DIRECTION ( 'NONE',  ( 0.005002170337468016433, -0.7660444431189770143, -0.6427681459581293666 ) ) ;
#38952=ORIENTED_EDGE ( 'NONE', *, *, #49754, .F. ) ;
#38953=ORIENTED_EDGE ( 'NONE', *, *, #35167, .T. ) ;
#38954=EDGE_CURVE ( 'NONE', #32592, #31186, #14479, .T. ) ;
#38955=ORIENTED_EDGE ( 'NONE', *, *, #47442, .T. ) ;
#38956=CARTESIAN_POINT ( 'NONE',  ( -14.88523388135589443, 0.000000000000000000, 6.381901129057940381 ) ) ;
#38957=ORIENTED_EDGE ( 'NONE', *, *, #12853, .T. ) ;
#38958=DIRECTION ( 'NONE',  ( -0.5364919789714478471, 0.6444004775717705469, -0.5449076811759709926 ) ) ;
#38959=ORIENTED_EDGE ( 'NONE', *, *, #51560, .T. ) ;
#38961=DIRECTION ( 'NONE',  ( 0.5364919789714477361, 0.6444004775717706579, 0.5449076811759711036 ) ) ;
#38962=ORIENTED_EDGE ( 'NONE', *, *, #52269, .T. ) ;
#38963=CARTESIAN_POINT ( 'NONE',  ( -17.74560456716937296, 0.000000000000000000, 3.774316574337878372 ) ) ;
#38964=ORIENTED_EDGE ( 'NONE', *, *, #6294, .T. ) ;
#38965=DIRECTION ( 'NONE',  ( 0.007781995580012663651, -3.146120232559066537E-19, -0.9999697198139514409 ) ) ;
#38966=ORIENTED_EDGE ( 'NONE', *, *, #44815, .T. ) ;
#38967=FACE_OUTER_BOUND ( 'NONE', #20229, .T. ) ;
#38968=LINE ( 'NONE', #12840, #35721 ) ;
#38969=DIRECTION ( 'NONE',  ( 0.007781995580012663651, -3.146120232559066537E-19, -0.9999697198139514409 ) ) ;
#38970=ORIENTED_EDGE ( 'NONE', *, *, #4952, .F. ) ;
#38971=DIRECTION ( 'NONE',  ( 0.5449076811759707706, 0.6444004775717708799, -0.5364919789714476250 ) ) ;
#38972=CARTESIAN_POINT ( 'NONE',  ( -15.60102546347950536, 0.000000000000000000, 12.95077420755565356 ) ) ;
#38973=LINE ( 'NONE', #334, #12218 ) ;
#38974=EDGE_CURVE ( 'NONE', #2376, #36986, #32077, .T. ) ;
#38975=CARTESIAN_POINT ( 'NONE',  ( -11.98370190339197272, -1.003701604285656579, 2.984053846613921035 ) ) ;
#38976=LINE ( 'NONE', #43, #47588 ) ;
#38977=DIRECTION ( 'NONE',  ( 0.007781995580012663651, 0.000000000000000000, -0.9999697198139515519 ) ) ;
#38978=EDGE_CURVE ( 'NONE', #5370, #1847, #44850, .T. ) ;
#38979=CARTESIAN_POINT ( 'NONE',  ( -16.89925026227929195, -0.1191753592594197858, 13.49466922669627422 ) ) ;
#38980=ORIENTED_EDGE ( 'NONE', *, *, #17428, .T. ) ;
#38981=DIRECTION ( 'NONE',  ( 0.6427681459581294776, -0.7660444431189769032, 0.005002170337467562802 ) ) ;
#38982=ADVANCED_FACE ( 'NONE', ( #32376 ), #24113, .F. ) ;
#38983=LINE ( 'NONE', #29907, #40430 ) ;
#38984=CARTESIAN_POINT ( 'NONE',  ( -20.98837076068963370, 5.305366725996512045, 13.74092773148062285 ) ) ;
#38985=ORIENTED_EDGE ( 'NONE', *, *, #50497, .T. ) ;
#38986=LINE ( 'NONE', #30484, #4828 ) ;
#38987=DIRECTION ( 'NONE',  ( -0.6427681459581293666, -0.7660444431189770143, -0.005002170337467561935 ) ) ;
#38988=ORIENTED_EDGE ( 'NONE', *, *, #41373, .T. ) ;
#38989=ADVANCED_FACE ( 'NONE', ( #10204 ), #19573, .F. ) ;
#38991=EDGE_CURVE ( 'NONE', #45002, #37252, #45674, .T. ) ;
#38992=CARTESIAN_POINT ( 'NONE',  ( -27.06552663992790997, 0.000000000000000000, 7.195101427592543786 ) ) ;
#38993=PLANE ( 'NONE',  #20298 ) ;
#38994=DIRECTION ( 'NONE',  ( -0.6427681459581293666, -0.7660444431189770143, -0.005002170337467561935 ) ) ;
#38996=ORIENTED_EDGE ( 'NONE', *, *, #5627, .F. ) ;
#38997=ORIENTED_EDGE ( 'NONE', *, *, #23296, .T. ) ;
#38998=DIRECTION ( 'NONE',  ( 0.5449076811759707706, 0.6444004775717708799, -0.5364919789714476250 ) ) ;
#38999=CARTESIAN_POINT ( 'NONE',  ( -19.60990026154428278, 0.000000000000000000, 4.498472333781370125 ) ) ;
#39000=DIRECTION ( 'NONE',  ( -0.5449076811759708816, 0.6444004775717707689, 0.5364919789714475140 ) ) ;
#39001=CARTESIAN_POINT ( 'NONE',  ( 2.072287782118878319, 0.000000000000000000, -2.950529333540147015 ) ) ;
#39002=CARTESIAN_POINT ( 'NONE',  ( -18.86354292863559579, 0.000000000000000000, 14.21804678658176080 ) ) ;
#39003=EDGE_CURVE ( 'NONE', #55548, #17566, #48844, .T. ) ;
#39004=CARTESIAN_POINT ( 'NONE',  ( -22.40478740399063895, 0.000000000000000000, 5.384712028983816623 ) ) ;
#39005=ORIENTED_EDGE ( 'NONE', *, *, #6377, .F. ) ;
#39006=PLANE ( 'NONE',  #214 ) ;
#39007=ADVANCED_FACE ( 'NONE', ( #1685 ), #19010, .F. ) ;
#39008=CARTESIAN_POINT ( 'NONE',  ( -13.02668629399155265, 0.000000000000000000, 6.396364776129978225 ) ) ;
#39009=VERTEX_POINT ( 'NONE', #18753 ) ;
#39010=ADVANCED_FACE ( 'NONE', ( #5665 ), #27835, .F. ) ;
#39011=PLANE ( 'NONE',  #49252 ) ;
#39012=FACE_OUTER_BOUND ( 'NONE', #24984, .T. ) ;
#39013=CARTESIAN_POINT ( 'NONE',  ( -27.06708303904391144, 0.000000000000000000, 7.395095371555332697 ) ) ;
#39014=VERTEX_POINT ( 'NONE', #19273 ) ;
#39015=EDGE_CURVE ( 'NONE', #20518, #6678, #23814, .T. ) ;
#39016=CARTESIAN_POINT ( 'NONE',  ( -11.95764949545960754, -3.756034771668162797, 1.406241090487040157 ) ) ;
#39017=VERTEX_POINT ( 'NONE', #39057 ) ;
#39018=VECTOR ( 'NONE', #26923, 1000.000000000000000 ) ;
#39020=ORIENTED_EDGE ( 'NONE', *, *, #40358, .T. ) ;
#39021=VERTEX_POINT ( 'NONE', #42275 ) ;
#39022=PLANE ( 'NONE',  #41158 ) ;
#39023=VERTEX_POINT ( 'NONE', #29193 ) ;
#39025=ORIENTED_EDGE ( 'NONE', *, *, #52139, .T. ) ;
#39026=DIRECTION ( 'NONE',  ( 0.007781995580012662783, 0.000000000000000000, -0.9999697198139514409 ) ) ;
#39027=ORIENTED_EDGE ( 'NONE', *, *, #8618, .T. ) ;
#39028=CARTESIAN_POINT ( 'NONE',  ( -18.19747506107908563, 0.000000000000000000, 14.03856424583689311 ) ) ;
#39029=VERTEX_POINT ( 'NONE', #42549 ) ;
#39030=CARTESIAN_POINT ( 'NONE',  ( -9.498088849204524564, 0.000000000000000000, 4.946496858126993246 ) ) ;
#39031=LINE ( 'NONE', #51543, #18695 ) ;
#39032=CARTESIAN_POINT ( 'NONE',  ( -17.51501930259471962, 2.876837460659008805, 8.406129810387598766 ) ) ;
#39033=LINE ( 'NONE', #34772, #27824 ) ;
#39034=LINE ( 'NONE', #13744, #29225 ) ;
#39035=EDGE_LOOP ( 'NONE', ( #54906, #31119, #51654 ) ) ;
#39037=CARTESIAN_POINT ( 'NONE',  ( -9.935275981939433620, 0.000000000000000000, 1.415645208431519642 ) ) ;
#39038=CARTESIAN_POINT ( 'NONE',  ( -14.82598494076193596, -0.5179957512181571078, 2.623710384272013751 ) ) ;
#39039=EDGE_CURVE ( 'NONE', #50224, #48862, #20697, .T. ) ;
#39040=LINE ( 'NONE', #50959, #26083 ) ;
#39041=LINE ( 'NONE', #30552, #13126 ) ;
#39042=DIRECTION ( 'NONE',  ( -0.7660212471507179544, -0.6427876096865405842, -0.005961354470445141482 ) ) ;
#39043=CARTESIAN_POINT ( 'NONE',  ( -12.76910910251310227, 0.000000000000000000, 7.306359454592487701 ) ) ;
#39044=EDGE_LOOP ( 'NONE', ( #13540, #45826, #49275, #47446 ) ) ;
#39045=DIRECTION ( 'NONE',  ( 0.9999697198139515519, 0.000000000000000000, 0.007781995580013368816 ) ) ;
#39046=LINE ( 'NONE', #4974, #16805 ) ;
#39048=ADVANCED_FACE ( 'NONE', ( #26276 ), #37428, .F. ) ;
#39049=EDGE_CURVE ( 'NONE', #48365, #7041, #41963, .T. ) ;
#39050=EDGE_CURVE ( 'NONE', #37328, #34091, #127, .T. ) ;
#39051=FACE_OUTER_BOUND ( 'NONE', #34929, .T. ) ;
#39052=FACE_OUTER_BOUND ( 'NONE', #31921, .T. ) ;
#39054=ADVANCED_FACE ( 'NONE', ( #46226 ), #13232, .F. ) ;
#39055=DIRECTION ( 'NONE',  ( 0.000000000000000000, -1.000000000000000000, 0.000000000000000000 ) ) ;
#39056=VECTOR ( 'NONE', #41217, 1000.000000000000227 ) ;
#39057=CARTESIAN_POINT ( 'NONE',  ( -19.16043661833849754, -0.1191753592594170102, 5.509963345090925557 ) ) ;
#39058=ORIENTED_EDGE ( 'NONE', *, *, #46253, .F. ) ;
#39059=ORIENTED_EDGE ( 'NONE', *, *, #34897, .F. ) ;
#39060=LINE ( 'NONE', #42742, #38464 ) ;
#39061=CARTESIAN_POINT ( 'NONE',  ( -14.56543180263941828, 4.333955019861509328, 9.651788012545988948 ) ) ;
#39062=DIRECTION ( 'NONE',  ( 0.7660212471507180654, -0.6427876096865404731, 0.005961354470445141482 ) ) ;
#39064=CARTESIAN_POINT ( 'NONE',  ( -28.93060053386082231, -0.1191753592594197858, 8.019254159017428663 ) ) ;
#39065=LINE ( 'NONE', #44437, #16703 ) ;
#39066=PLANE ( 'NONE',  #29173 ) ;
#39067=DIRECTION ( 'NONE',  ( 0.005961354470445682716, -0.6427876096865404731, -0.7660212471507180654 ) ) ;
#39068=ORIENTED_EDGE ( 'NONE', *, *, #37054, .F. ) ;
#39069=ADVANCED_FACE ( 'NONE', ( #33205 ), #15858, .F. ) ;
#39070=LINE ( 'NONE', #21756, #50445 ) ;
#39071=LINE ( 'NONE', #144, #47790 ) ;
#39072=ADVANCED_FACE ( 'NONE', ( #3377 ), #11324, .F. ) ;
#39073=ORIENTED_EDGE ( 'NONE', *, *, #44258, .F. ) ;
#39074=LINE ( 'NONE', #21494, #9280 ) ;
#39075=ORIENTED_EDGE ( 'NONE', *, *, #49948, .T. ) ;
#39076=CARTESIAN_POINT ( 'NONE',  ( -12.13851405436063047, 0.000000000000000000, 11.68505802764555135 ) ) ;
#39077=ORIENTED_EDGE ( 'NONE', *, *, #4196, .F. ) ;
#39078=EDGE_CURVE ( 'NONE', #1003, #441, #47872, .T. ) ;
#39079=VECTOR ( 'NONE', #23579, 1000.000000000000114 ) ;
#39080=ORIENTED_EDGE ( 'NONE', *, *, #34192, .F. ) ;
#39081=EDGE_CURVE ( 'NONE', #54767, #36041, #43585, .T. ) ;
#39082=EDGE_LOOP ( 'NONE', ( #4460, #39676, #49892 ) ) ;
#39083=ORIENTED_EDGE ( 'NONE', *, *, #30236, .T. ) ;
#39084=ORIENTED_EDGE ( 'NONE', *, *, #43124, .T. ) ;
#39085=ORIENTED_EDGE ( 'NONE', *, *, #18074, .T. ) ;
#39086=CARTESIAN_POINT ( 'NONE',  ( -9.110551994824897193, 0.000000000000000000, 3.538847790438064411 ) ) ;
#39087=DIRECTION ( 'NONE',  ( 0.000000000000000000, -0.000000000000000000, -1.000000000000000000 ) ) ;
#39088=CARTESIAN_POINT ( 'NONE',  ( -14.00280974873554030, 0.000000000000000000, 12.40921378708904044 ) ) ;
#39089=VECTOR ( 'NONE', #17045, 1000.000000000000000 ) ;
#39090=ORIENTED_EDGE ( 'NONE', *, *, #19652, .T. ) ;
#39091=CARTESIAN_POINT ( 'NONE',  ( -16.58287145540726826, 2.876837460659006585, 8.044051930665851557 ) ) ;
#39093=VERTEX_POINT ( 'NONE', #15564 ) ;
#39094=VECTOR ( 'NONE', #16152, 1000.000000000000227 ) ;
#39095=LINE ( 'NONE', #30305, #41952 ) ;
#39096=DIRECTION ( 'NONE',  ( 0.000000000000000000, -0.000000000000000000, -1.000000000000000000 ) ) ;
#39097=DIRECTION ( 'NONE',  ( -0.5364919789714478471, 0.6444004775717705469, -0.5449076811759709926 ) ) ;
#39098=ORIENTED_EDGE ( 'NONE', *, *, #37522, .F. ) ;
#39099=DIRECTION ( 'NONE',  ( 0.5449076811759707706, 0.6444004775717708799, -0.5364919789714476250 ) ) ;
#39100=ORIENTED_EDGE ( 'NONE', *, *, #8094, .F. ) ;
#39101=CARTESIAN_POINT ( 'NONE',  ( -17.40972996391339578, 0.000000000000000000, 6.531580930396862605 ) ) ;
#39102=DIRECTION ( 'NONE',  ( -0.005002170337468016433, -0.7660444431189770143, 0.6427681459581293666 ) ) ;
#39103=CARTESIAN_POINT ( 'NONE',  ( -12.80458192191714595, 0.000000000000000000, 11.86454056839041726 ) ) ;
#39104=DIRECTION ( 'NONE',  ( 0.000000000000000000, -1.000000000000000000, 0.000000000000000000 ) ) ;
#39106=CARTESIAN_POINT ( 'NONE',  ( -10.94028622754223967, 0.000000000000000000, 11.14038480894692995 ) ) ;
#39107=LINE ( 'NONE', #5329, #45691 ) ;
#39108=FACE_OUTER_BOUND ( 'NONE', #21272, .T. ) ;
#39109=ORIENTED_EDGE ( 'NONE', *, *, #8841, .T. ) ;
#39111=EDGE_CURVE ( 'NONE', #32474, #41831, #2774, .T. ) ;
#39112=VECTOR ( 'NONE', #30345, 1000.000000000000000 ) ;
#39113=VECTOR ( 'NONE', #53361, 999.9999999999998863 ) ;
#39114=DIRECTION ( 'NONE',  ( 0.9999697198139515519, 0.000000000000000000, 0.007781995580013368816 ) ) ;
#39115=DIRECTION ( 'NONE',  ( 0.6427681459581294776, -0.7660444431189769032, 0.005002170337467562802 ) ) ;
#39116=LINE ( 'NONE', #52725, #14533 ) ;
#39118=LINE ( 'NONE', #42545, #1412 ) ;
#39120=EDGE_CURVE ( 'NONE', #27927, #46187, #45975, .T. ) ;
#39121=LINE ( 'NONE', #21544, #23208 ) ;
#39122=CARTESIAN_POINT ( 'NONE',  ( -17.74482636761137044, -0.1191753592594197858, 3.674319602356483916 ) ) ;
#39125=DIRECTION ( 'NONE',  ( 0.005961354470445682716, -0.6427876096865404731, -0.7660212471507180654 ) ) ;
#39126=DIRECTION ( 'NONE',  ( 0.000000000000000000, -0.000000000000000000, -1.000000000000000000 ) ) ;
#39127=LINE ( 'NONE', #39712, #37253 ) ;
#39128=FACE_OUTER_BOUND ( 'NONE', #42424, .T. ) ;
#39129=DIRECTION ( 'NONE',  ( 0.9999697198139515519, 0.000000000000000000, 0.007781995580013368816 ) ) ;
#39130=DIRECTION ( 'NONE',  ( 0.005961354470445682716, -0.6427876096865404731, -0.7660212471507180654 ) ) ;
#39131=CARTESIAN_POINT ( 'NONE',  ( -15.52718360830426292, 1.095915999411505082, 4.711191396085759209 ) ) ;
#39132=VECTOR ( 'NONE', #49715, 1000.000000000000227 ) ;
#39133=FACE_OUTER_BOUND ( 'NONE', #1838, .T. ) ;
#39134=CARTESIAN_POINT ( 'NONE',  ( -12.50510409456438587, 0.2864062442990034651, 2.208769662944593648 ) ) ;
#39135=EDGE_LOOP ( 'NONE', ( #4984, #41405, #38010, #18211 ) ) ;
#39136=CARTESIAN_POINT ( 'NONE',  ( -16.45746374218896335, 0.000000000000000000, 3.584335127870767135 ) ) ;
#39137=ORIENTED_EDGE ( 'NONE', *, *, #22411, .F. ) ;
#39138=EDGE_CURVE ( 'NONE', #19873, #38484, #46815, .T. ) ;
#39139=ORIENTED_EDGE ( 'NONE', *, *, #39675, .F. ) ;
#39140=ORIENTED_EDGE ( 'NONE', *, *, #53870, .T. ) ;
#39141=ORIENTED_EDGE ( 'NONE', *, *, #31740, .F. ) ;
#39142=ADVANCED_FACE ( 'NONE', ( #3069 ), #7085, .F. ) ;
#39143=ORIENTED_EDGE ( 'NONE', *, *, #53519, .T. ) ;
#39144=DIRECTION ( 'NONE',  ( -0.5364919789714478471, 0.6444004775717705469, -0.5449076811759709926 ) ) ;
#39145=DIRECTION ( 'NONE',  ( -0.6427681459581293666, -0.7660444431189770143, -0.005002170337467561935 ) ) ;
#39146=VECTOR ( 'NONE', #19790, 1000.000000000000227 ) ;
#39147=AXIS2_PLACEMENT_3D ( 'NONE', #37, #17957, #328 ) ;
#39148=ORIENTED_EDGE ( 'NONE', *, *, #2937, .F. ) ;
#39149=EDGE_LOOP ( 'NONE', ( #51599, #23179, #19130, #539, #46612 ) ) ;
#39150=EDGE_CURVE ( 'NONE', #45990, #15181, #7931, .T. ) ;
#39151=VECTOR ( 'NONE', #42099, 999.9999999999998863 ) ;
#39152=CARTESIAN_POINT ( 'NONE',  ( -27.06552663992790997, 0.000000000000000000, 7.195101427592543786 ) ) ;
#39153=EDGE_LOOP ( 'NONE', ( #55694, #7519, #32591, #20933 ) ) ;
#39154=DIRECTION ( 'NONE',  ( 0.6246952433987894571, -0.7422098413412800966, -0.2426528472758541777 ) ) ;
#39156=ORIENTED_EDGE ( 'NONE', *, *, #627, .F. ) ;
#39157=DIRECTION ( 'NONE',  ( 0.000000000000000000, -1.000000000000000000, 0.000000000000000000 ) ) ;
#39158=ORIENTED_EDGE ( 'NONE', *, *, #3280, .F. ) ;
#39159=PLANE ( 'NONE',  #52722 ) ;
#39160=AXIS2_PLACEMENT_3D ( 'NONE', #15288, #11294, #1915 ) ;
#39161=AXIS2_PLACEMENT_3D ( 'NONE', #42648, #16832, #38703 ) ;
#39162=DIRECTION ( 'NONE',  ( 0.5364919789714477361, 0.6444004775717706579, 0.5449076811759711036 ) ) ;
#39163=ORIENTED_EDGE ( 'NONE', *, *, #4275, .T. ) ;
#39164=FACE_OUTER_BOUND ( 'NONE', #5314, .T. ) ;
#39165=CARTESIAN_POINT ( 'NONE',  ( -17.26532721389163072, 0.000000000000000000, 13.67648636611514590 ) ) ;
#39166=LINE ( 'NONE', #25006, #34826 ) ;
#39167=EDGE_LOOP ( 'NONE', ( #38193, #27578, #38671 ) ) ;
#39168=DIRECTION ( 'NONE',  ( 0.9321478471874541372, 0.000000000000000000, -0.3620778797217453771 ) ) ;
#39169=EDGE_CURVE ( 'NONE', #53748, #22074, #55063, .T. ) ;
#39170=VERTEX_POINT ( 'NONE', #41689 ) ;
#39171=DIRECTION ( 'NONE',  ( 0.7660212471507180654, -0.6427876096865404731, 0.005961354470445141482 ) ) ;
#39172=LINE ( 'NONE', #52255, #14230 ) ;
#39173=CARTESIAN_POINT ( 'NONE',  ( -20.54126990917373519, -0.1191753592594197858, 4.760553241521720658 ) ) ;
#39174=DIRECTION ( 'NONE',  ( -0.5449076811759708816, 0.6444004775717707689, 0.5364919789714475140 ) ) ;
#39176=CARTESIAN_POINT ( 'NONE',  ( -20.54049170961573267, 0.000000000000000000, 4.660556269540326646 ) ) ;
#39177=ADVANCED_FACE ( 'NONE', ( #52952 ), #45016, .F. ) ;
#39178=CARTESIAN_POINT ( 'NONE',  ( 1.086233639165236964, 0.000000000000000000, 2.796443541562362078 ) ) ;
#39179=FACE_OUTER_BOUND ( 'NONE', #52487, .T. ) ;
#39180=DIRECTION ( 'NONE',  ( 0.007781995580012662783, 0.000000000000000000, -0.9999697198139514409 ) ) ;
#39181=VERTEX_POINT ( 'NONE', #427 ) ;
#39182=PLANE ( 'NONE',  #1161 ) ;
#39183=DIRECTION ( 'NONE',  ( 0.9999697198139515519, 0.000000000000000000, 0.007781995580013368816 ) ) ;
#39184=FACE_OUTER_BOUND ( 'NONE', #29082, .T. ) ;
#39185=AXIS2_PLACEMENT_3D ( 'NONE', #38290, #55615, #34054 ) ;
#39186=VECTOR ( 'NONE', #44541, 1000.000000000000000 ) ;
#39187=DIRECTION ( 'NONE',  ( 0.007781995580012663651, -3.146120232559066537E-19, -0.9999697198139514409 ) ) ;
#39188=CARTESIAN_POINT ( 'NONE',  ( -10.37421533196711465, -0.1191753592594197858, 10.96012406864405975 ) ) ;
#39189=FACE_OUTER_BOUND ( 'NONE', #25463, .T. ) ;
#39190=ADVANCED_FACE ( 'NONE', ( #26548 ), #52409, .F. ) ;
#39191=ORIENTED_EDGE ( 'NONE', *, *, #21089, .T. ) ;
#39192=VECTOR ( 'NONE', #15805, 999.9999999999998863 ) ;
#39193=VECTOR ( 'NONE', #19632, 999.9999999999998863 ) ;
#39195=CARTESIAN_POINT ( 'NONE',  ( -17.93139508144814442, 0.000000000000000000, 13.85596890686001537 ) ) ;
#39197=ORIENTED_EDGE ( 'NONE', *, *, #38950, .T. ) ;
#39198=CARTESIAN_POINT ( 'NONE',  ( -20.94928162563153862, -3.917936722690662954, 4.893730847070894896 ) ) ;
#39199=ORIENTED_EDGE ( 'NONE', *, *, #19657, .T. ) ;
#39200=CARTESIAN_POINT ( 'NONE',  ( -17.26532721389163072, 0.000000000000000000, 13.67648636611514590 ) ) ;
#39201=VECTOR ( 'NONE', #36002, 1000.000000000000227 ) ;
#39202=VERTEX_POINT ( 'NONE', #1261 ) ;
#39203=CARTESIAN_POINT ( 'NONE',  ( -13.79694961163590072, -1.489407457353155717, 4.485506886498618506 ) ) ;
#39205=ORIENTED_EDGE ( 'NONE', *, *, #44909, .F. ) ;
#39207=CARTESIAN_POINT ( 'NONE',  ( -15.40103151951671734, 0.000000000000000000, 12.95233060667165681 ) ) ;
#39208=FACE_OUTER_BOUND ( 'NONE', #7543, .T. ) ;
#39209=DIRECTION ( 'NONE',  ( -0.005002170337468016433, -0.7660444431189770143, 0.6427681459581293666 ) ) ;
#39210=LINE ( 'NONE', #13653, #14901 ) ;
#39211=ORIENTED_EDGE ( 'NONE', *, *, #8469, .F. ) ;
#39212=EDGE_CURVE ( 'NONE', #42908, #40238, #13507, .T. ) ;
#39213=EDGE_LOOP ( 'NONE', ( #38672, #27687, #4380, #29730 ) ) ;
#39214=VECTOR ( 'NONE', #11747, 999.9999999999998863 ) ;
#39215=ORIENTED_EDGE ( 'NONE', *, *, #4327, .F. ) ;
#39216=DIRECTION ( 'NONE',  ( 0.9999697198139515519, 0.000000000000000000, 0.007781995580013368816 ) ) ;
#39217=VERTEX_POINT ( 'NONE', #14065 ) ;
#39218=VECTOR ( 'NONE', #54544, 999.9999999999998863 ) ;
#39219=DIRECTION ( 'NONE',  ( 0.5449076811759707706, 0.6444004775717708799, -0.5364919789714476250 ) ) ;
#39220=EDGE_LOOP ( 'NONE', ( #43006, #15344, #31257, #13826 ) ) ;
#39221=LINE ( 'NONE', #18485, #46882 ) ;
#39222=DIRECTION ( 'NONE',  ( 0.005002170337468016433, -0.7660444431189770143, -0.6427681459581293666 ) ) ;
#39223=EDGE_CURVE ( 'NONE', #56039, #35922, #39643, .T. ) ;
#39224=AXIS2_PLACEMENT_3D ( 'NONE', #28301, #54413, #28042 ) ;
#39225=VECTOR ( 'NONE', #9025, 999.9999999999998863 ) ;
#39227=DIRECTION ( 'NONE',  ( 0.9999697198139515519, 0.000000000000000000, 0.007781995580013368816 ) ) ;
#39228=EDGE_LOOP ( 'NONE', ( #45949, #24182, #11274, #34789 ) ) ;
#39229=ADVANCED_FACE ( 'NONE', ( #18041 ), #36210, .F. ) ;
#39230=ADVANCED_FACE ( 'NONE', ( #27686 ), #35950, .F. ) ;
#39231=AXIS2_PLACEMENT_3D ( 'NONE', #39285, #372, #4929 ) ;
#39232=DIRECTION ( 'NONE',  ( 0.007781995580012663651, -3.146120232559066537E-19, -0.9999697198139514409 ) ) ;
#39233=VECTOR ( 'NONE', #48181, 1000.000000000000227 ) ;
#39234=ORIENTED_EDGE ( 'NONE', *, *, #6549, .T. ) ;
#39235=CARTESIAN_POINT ( 'NONE',  ( -19.27845611090958755, 0.000000000000000000, 7.825040337060908513 ) ) ;
#39236=LINE ( 'NONE', #56022, #46551 ) ;
#39237=DIRECTION ( 'NONE',  ( 0.005002170337468016433, -0.7660444431189770143, -0.6427681459581293666 ) ) ;
#39238=EDGE_CURVE ( 'NONE', #39979, #29674, #31398, .T. ) ;
#39239=ORIENTED_EDGE ( 'NONE', *, *, #44544, .T. ) ;
#39240=PLANE ( 'NONE',  #32902 ) ;
#39241=EDGE_CURVE ( 'NONE', #42246, #39979, #5276, .T. ) ;
#39242=PLANE ( 'NONE',  #30080 ) ;
#39243=CARTESIAN_POINT ( 'NONE',  ( -20.97491883346917163, 4.819660872929012463, 4.675530102110849739 ) ) ;
#39244=AXIS2_PLACEMENT_3D ( 'NONE', #39165, #25843, #21000 ) ;
#39245=PLANE ( 'NONE',  #5027 ) ;
#39246=VECTOR ( 'NONE', #19675, 1000.000000000000000 ) ;
#39247=CARTESIAN_POINT ( 'NONE',  ( -9.342070512798265725, 0.000000000000000000, 10.59882438848031505 ) ) ;
#39249=EDGE_CURVE ( 'NONE', #27552, #1558, #14613, .T. ) ;
#39251=DIRECTION ( 'NONE',  ( 0.7660212471507180654, -0.6427876096865404731, 0.005961354470445141482 ) ) ;
#39252=ORIENTED_EDGE ( 'NONE', *, *, #36388, .T. ) ;
#39253=PLANE ( 'NONE',  #35271 ) ;
#39255=LINE ( 'NONE', #26464, #54998 ) ;
#39256=ORIENTED_EDGE ( 'NONE', *, *, #42966, .T. ) ;
#39257=DIRECTION ( 'NONE',  ( 0.5449076811759707706, 0.6444004775717708799, -0.5364919789714476250 ) ) ;
#39258=DIRECTION ( 'NONE',  ( 0.9999697198139515519, 0.000000000000000000, 0.007781995580013368816 ) ) ;
#39259=ORIENTED_EDGE ( 'NONE', *, *, #13845, .T. ) ;
#39260=VECTOR ( 'NONE', #21776, 1000.000000000000227 ) ;
#39261=EDGE_CURVE ( 'NONE', #30915, #22464, #30821, .T. ) ;
#39262=DIRECTION ( 'NONE',  ( 0.007781995580012662783, 0.000000000000000000, -0.9999697198139514409 ) ) ;
#39263=DIRECTION ( 'NONE',  ( 0.007781995580012662783, 0.000000000000000000, -0.9999697198139514409 ) ) ;
#39264=VECTOR ( 'NONE', #42353, 999.9999999999998863 ) ;
#39265=LINE ( 'NONE', #21403, #13277 ) ;
#39266=FACE_OUTER_BOUND ( 'NONE', #13928, .T. ) ;
#39267=ADVANCED_FACE ( 'NONE', ( #26849 ), #44172, .F. ) ;
#39268=ORIENTED_EDGE ( 'NONE', *, *, #46909, .T. ) ;
#39269=ORIENTED_EDGE ( 'NONE', *, *, #36419, .F. ) ;
#39270=CARTESIAN_POINT ( 'NONE',  ( -23.33693525117809386, 0.000000000000000000, 5.746789908705562944 ) ) ;
#39271=FACE_OUTER_BOUND ( 'NONE', #40956, .T. ) ;
#39272=VECTOR ( 'NONE', #36098, 1000.000000000000227 ) ;
#39273=DIRECTION ( 'NONE',  ( 0.000000000000000000, -1.000000000000000000, 0.000000000000000000 ) ) ;
#39274=AXIS2_PLACEMENT_3D ( 'NONE', #16138, #7070, #49670 ) ;
#39275=DIRECTION ( 'NONE',  ( 0.7660212471507180654, -0.6427876096865404731, 0.005961354470445141482 ) ) ;
#39276=AXIS2_PLACEMENT_3D ( 'NONE', #56101, #17186, #52652 ) ;
#39277=CARTESIAN_POINT ( 'NONE',  ( -16.67577990931724941, -3.270328918600661439, 3.254419731274814875 ) ) ;
#39278=DIRECTION ( 'NONE',  ( 0.005002170337468016433, -0.7660444431189770143, -0.6427681459581293666 ) ) ;
#39279=ORIENTED_EDGE ( 'NONE', *, *, #21440, .F. ) ;
#39280=CARTESIAN_POINT ( 'NONE',  ( -9.908141408373387193, -0.1191753592594197858, 10.77908512878318703 ) ) ;
#39281=AXIS2_PLACEMENT_3D ( 'NONE', #23019, #19033, #53135 ) ;
#39283=AXIS2_PLACEMENT_3D ( 'NONE', #16777, #13376, #270 ) ;
#39284=ORIENTED_EDGE ( 'NONE', *, *, #51515, .F. ) ;
#39285=CARTESIAN_POINT ( 'NONE',  ( -24.26908309836554878, 0.000000000000000000, 6.108867788427308376 ) ) ;
#39286=CARTESIAN_POINT ( 'NONE',  ( 2.072287782118878319, 0.000000000000000000, -2.950529333540147015 ) ) ;
#39287=CARTESIAN_POINT ( 'NONE',  ( -11.21901323774118708, 0.000000000000000000, 1.039777472322872098 ) ) ;
#39288=ORIENTED_EDGE ( 'NONE', *, *, #1927, .F. ) ;
#39289=DIRECTION ( 'NONE',  ( 0.005002170337468016433, -0.7660444431189770143, -0.6427681459581293666 ) ) ;
#39290=VECTOR ( 'NONE', #14188, 999.9999999999998863 ) ;
#39293=AXIS2_PLACEMENT_3D ( 'NONE', #5165, #44885, #48282 ) ;
#39294=ORIENTED_EDGE ( 'NONE', *, *, #2856, .T. ) ;
#39295=ORIENTED_EDGE ( 'NONE', *, *, #1095, .T. ) ;
#39296=ORIENTED_EDGE ( 'NONE', *, *, #6705, .F. ) ;
#39297=LINE ( 'NONE', #16589, #35698 ) ;
#39298=ORIENTED_EDGE ( 'NONE', *, *, #29686, .T. ) ;
#39299=EDGE_CURVE ( 'NONE', #50871, #50902, #14358, .T. ) ;
#39300=VECTOR ( 'NONE', #8101, 1000.000000000000227 ) ;
#39301=LINE ( 'NONE', #9479, #33113 ) ;
#39302=ADVANCED_FACE ( 'NONE', ( #39339 ), #43870, .F. ) ;
#39304=CARTESIAN_POINT ( 'NONE',  ( -14.13560388593797335, 5.467268677019012202, 11.34478904033489322 ) ) ;
#39305=VERTEX_POINT ( 'NONE', #44428 ) ;
#39306=LINE ( 'NONE', #17432, #36469 ) ;
#39307=VECTOR ( 'NONE', #31868, 1000.000000000000227 ) ;
#39308=ORIENTED_EDGE ( 'NONE', *, *, #51872, .F. ) ;
#39309=EDGE_CURVE ( 'NONE', #21477, #30276, #5534, .T. ) ;
#39310=CARTESIAN_POINT ( 'NONE',  ( -23.33693525117809386, 0.000000000000000000, 5.746789908705562944 ) ) ;
#39311=LINE ( 'NONE', #8951, #6891 ) ;
#39312=DIRECTION ( 'NONE',  ( -0.005961354470445682716, -0.6427876096865404731, 0.7660212471507180654 ) ) ;
#39313=CARTESIAN_POINT ( 'NONE',  ( -21.47263955680318404, 0.000000000000000000, 5.022634149262071190 ) ) ;
#39314=AXIS2_PLACEMENT_3D ( 'NONE', #10026, #17996, #1209 ) ;
#39315=CARTESIAN_POINT ( 'NONE',  ( -26.13337879274045505, 0.000000000000000000, 6.833023547870798353 ) ) ;
#39316=ORIENTED_EDGE ( 'NONE', *, *, #25933, .T. ) ;
#39318=VECTOR ( 'NONE', #784, 1000.000000000000114 ) ;
#39319=ORIENTED_EDGE ( 'NONE', *, *, #51187, .T. ) ;
#39320=EDGE_CURVE ( 'NONE', #12870, #47161, #27386, .T. ) ;
#39321=LINE ( 'NONE', #22293, #47598 ) ;
#39322=DIRECTION ( 'NONE',  ( -0.6427681459581293666, -0.7660444431189770143, -0.005002170337467561935 ) ) ;
#39323=EDGE_CURVE ( 'NONE', #30584, #24781, #46108, .T. ) ;
#39325=AXIS2_PLACEMENT_3D ( 'NONE', #11121, #11696, #20504 ) ;
#39326=AXIS2_PLACEMENT_3D ( 'NONE', #15565, #2233, #41965 ) ;
#39327=CARTESIAN_POINT ( 'NONE',  ( -16.99924723426068951, 0.000000000000000000, 13.49389102713827171 ) ) ;
#39328=DIRECTION ( 'NONE',  ( 0.000000000000000000, -1.000000000000000000, 0.000000000000000000 ) ) ;
#39329=CARTESIAN_POINT ( 'NONE',  ( -32.65841372305263235, 0.000000000000000000, 9.367568705923016381 ) ) ;
#39330=ORIENTED_EDGE ( 'NONE', *, *, #39697, .F. ) ;
#39332=CARTESIAN_POINT ( 'NONE',  ( -16.48907833074707341, 0.000000000000000000, 7.646741863706176368 ) ) ;
#39333=EDGE_LOOP ( 'NONE', ( #56131, #47618, #43418, #10803 ) ) ;
#39335=FACE_OUTER_BOUND ( 'NONE', #43969, .T. ) ;
#39336=CARTESIAN_POINT ( 'NONE',  ( 2.072287782118878319, 0.000000000000000000, -2.950529333540147015 ) ) ;
#39338=DIRECTION ( 'NONE',  ( 0.007781995580012663651, 0.000000000000000000, -0.9999697198139515519 ) ) ;
#39339=FACE_OUTER_BOUND ( 'NONE', #35327, .T. ) ;
#39340=VERTEX_POINT ( 'NONE', #28224 ) ;
#39341=AXIS2_PLACEMENT_3D ( 'NONE', #25399, #21127, #29942 ) ;
#39342=ORIENTED_EDGE ( 'NONE', *, *, #25540, .T. ) ;
#39343=CARTESIAN_POINT ( 'NONE',  ( -13.57904574923490060, -0.1191753592594181482, 4.814734879791510380 ) ) ;
#39344=CARTESIAN_POINT ( 'NONE',  ( -14.75409303702196873, -3.756034771668162797, 2.492474729652275567 ) ) ;
#39345=CARTESIAN_POINT ( 'NONE',  ( -27.99923088623136636, 0.000000000000000000, 7.757173251277078130 ) ) ;
#39346=VECTOR ( 'NONE', #5880, 999.9999999999998863 ) ;
#39347=CARTESIAN_POINT ( 'NONE',  ( -12.63916579227093173, -0.6798977022406551551, 2.707240912800944699 ) ) ;
#39348=CARTESIAN_POINT ( 'NONE',  ( -9.542064456761055524, 0.000000000000000000, 10.59726798936431180 ) ) ;
#39349=VECTOR ( 'NONE', #14667, 999.9999999999998863 ) ;
#39351=CARTESIAN_POINT ( 'NONE',  ( -18.66354898467281132, 0.000000000000000000, 14.21960318569776582 ) ) ;
#39352=VERTEX_POINT ( 'NONE', #15715 ) ;
#39353=FACE_OUTER_BOUND ( 'NONE', #11824, .T. ) ;
#39354=CARTESIAN_POINT ( 'NONE',  ( -12.76048694199725553, 0.000000000000000000, 6.198430344819195525 ) ) ;
#39355=VECTOR ( 'NONE', #24747, 1000.000000000000000 ) ;
#39356=EDGE_LOOP ( 'NONE', ( #33152, #23510, #35063, #17517 ) ) ;
#39357=CARTESIAN_POINT ( 'NONE',  ( -13.95021198066316259, 0.000000000000000000, 5.650513546078428817 ) ) ;
#39359=DIRECTION ( 'NONE',  ( 0.5364919789714477361, 0.6444004775717706579, 0.5449076811759711036 ) ) ;
#39360=EDGE_CURVE ( 'NONE', #48042, #6272, #24513, .T. ) ;
#39361=DIRECTION ( 'NONE',  ( -0.005002170337468016433, -0.7660444431189770143, 0.6427681459581293666 ) ) ;
#39362=VECTOR ( 'NONE', #35278, 1000.000000000000114 ) ;
#39363=ORIENTED_EDGE ( 'NONE', *, *, #48746, .T. ) ;
#39364=EDGE_CURVE ( 'NONE', #21773, #44736, #49811, .T. ) ;
#39365=ORIENTED_EDGE ( 'NONE', *, *, #36238, .T. ) ;
#39366=VECTOR ( 'NONE', #39129, 999.9999999999998863 ) ;
#39367=ORIENTED_EDGE ( 'NONE', *, *, #41847, .T. ) ;
#39368=EDGE_LOOP ( 'NONE', ( #18829, #24340, #35470, #23217 ) ) ;
#39369=VECTOR ( 'NONE', #19208, 999.9999999999998863 ) ;
#39370=ORIENTED_EDGE ( 'NONE', *, *, #18990, .T. ) ;
#39371=EDGE_CURVE ( 'NONE', #14113, #12863, #14898, .T. ) ;
#39372=EDGE_LOOP ( 'NONE', ( #16937, #242, #13275, #11821 ) ) ;
#39373=DIRECTION ( 'NONE',  ( 0.6427681459581294776, -0.7660444431189769032, 0.005002170337467562802 ) ) ;
#39374=CARTESIAN_POINT ( 'NONE',  ( -16.81267852042391198, -0.1191753592594197858, 3.312241722634738039 ) ) ;
#39375=CARTESIAN_POINT ( 'NONE',  ( -16.99924723426068951, 0.000000000000000000, 13.49389102713827171 ) ) ;
#39376=EDGE_CURVE ( 'NONE', #51007, #51066, #28806, .T. ) ;
#39377=EDGE_CURVE ( 'NONE', #12878, #24462, #41829, .T. ) ;
#39378=ADVANCED_FACE ( 'NONE', ( #54914 ), #54604, .F. ) ;
#39379=ORIENTED_EDGE ( 'NONE', *, *, #20470, .F. ) ;
#39380=CARTESIAN_POINT ( 'NONE',  ( -16.20409152483680870, 3.524445264749008988, 8.959755678013548774 ) ) ;
#39381=EDGE_LOOP ( 'NONE', ( #42501, #55475, #36423, #1457 ) ) ;
#39382=ADVANCED_FACE ( 'NONE', ( #36464 ), #29062, .F. ) ;
#39383=EDGE_LOOP ( 'NONE', ( #10538, #41328, #45428, #12 ) ) ;
#39384=VECTOR ( 'NONE', #46408, 1000.000000000000227 ) ;
#39385=FACE_OUTER_BOUND ( 'NONE', #49571, .T. ) ;
#39386=VECTOR ( 'NONE', #40701, 1000.000000000000227 ) ;
#39387=CARTESIAN_POINT ( 'NONE',  ( -11.41981228898398548, 1.743523803501505709, 4.178583624546474695 ) ) ;
#39388=LINE ( 'NONE', #26596, #20508 ) ;
#39389=VERTEX_POINT ( 'NONE', #6381 ) ;
#39390=CARTESIAN_POINT ( 'NONE',  ( -23.33849165029409889, 0.000000000000000000, 5.946783852668351855 ) ) ;
#39392=ORIENTED_EDGE ( 'NONE', *, *, #41729, .T. ) ;
#39394=EDGE_CURVE ( 'NONE', #29873, #38799, #50371, .T. ) ;
#39395=FACE_OUTER_BOUND ( 'NONE', #45737, .T. ) ;
#39396=AXIS2_PLACEMENT_3D ( 'NONE', #47391, #5097, #4523 ) ;
#39397=EDGE_CURVE ( 'NONE', #5309, #24312, #11483, .T. ) ;
#39398=LINE ( 'NONE', #47068, #49627 ) ;
#39399=CARTESIAN_POINT ( 'NONE',  ( -22.35034652457852644, 4.172053068839010059, 12.41000458341346580 ) ) ;
#39400=DIRECTION ( 'NONE',  ( -0.9999697198139514409, -0.000000000000000000, -0.007781995580013368816 ) ) ;
#39401=CARTESIAN_POINT ( 'NONE',  ( 2.072287782118878319, 0.000000000000000000, -2.950529333540147015 ) ) ;
#39402=EDGE_CURVE ( 'NONE', #32587, #6528, #2653, .T. ) ;
#39404=VECTOR ( 'NONE', #29755, 999.9999999999998863 ) ;
#39405=CARTESIAN_POINT ( 'NONE',  ( 1.086233639165236964, 0.000000000000000000, 2.796443541562362078 ) ) ;
#39407=LINE ( 'NONE', #500, #53731 ) ;
#39408=AXIS2_PLACEMENT_3D ( 'NONE', #33452, #37723, #20382 ) ;
#39409=EDGE_CURVE ( 'NONE', #15255, #26117, #54084, .T. ) ;
#39410=LINE ( 'NONE', #13562, #28322 ) ;
#39411=LINE ( 'NONE', #51885, #36892 ) ;
#39412=DIRECTION ( 'NONE',  ( 0.6427681459581294776, -0.7660444431189769032, 0.005002170337467562802 ) ) ;
#39414=CARTESIAN_POINT ( 'NONE',  ( -22.40634380310664397, 0.000000000000000000, 5.584705972946605534 ) ) ;
#39415=EDGE_CURVE ( 'NONE', #50386, #30703, #10666, .T. ) ;
#39416=DIRECTION ( 'NONE',  ( 0.9999697198139515519, 0.000000000000000000, 0.007781995580013368816 ) ) ;
#39417=VECTOR ( 'NONE', #42492, 1000.000000000000114 ) ;
#39418=CARTESIAN_POINT ( 'NONE',  ( -21.09046673295159735, 4.333955019861509328, 12.18633317059820698 ) ) ;
#39419=VECTOR ( 'NONE', #43526, 999.9999999999998863 ) ;
#39420=ORIENTED_EDGE ( 'NONE', *, *, #21354, .T. ) ;
#39423=CARTESIAN_POINT ( 'NONE',  ( -14.13583565709953938, 0.000000000000000000, 3.802408630673602019 ) ) ;
#39424=FACE_OUTER_BOUND ( 'NONE', #54639, .T. ) ;
#39425=DIRECTION ( 'NONE',  ( 0.007781995580012662783, 0.000000000000000000, -0.9999697198139514409 ) ) ;
#39426=FACE_OUTER_BOUND ( 'NONE', #46244, .T. ) ;
#39427=CARTESIAN_POINT ( 'NONE',  ( -15.99725729796916340, 0.000000000000000000, 4.157254686859329418 ) ) ;
#39428=AXIS2_PLACEMENT_3D ( 'NONE', #26339, #52475, #14151 ) ;
#39429=CARTESIAN_POINT ( 'NONE',  ( -15.96710241509184058, -0.1191753592594218814, 13.13259134697452879 ) ) ;
#39430=VECTOR ( 'NONE', #29881, 1000.000000000000227 ) ;
#39431=DIRECTION ( 'NONE',  ( 0.007781995580012663651, -3.146120232559066537E-19, -0.9999697198139514409 ) ) ;
#39432=VECTOR ( 'NONE', #18214, 1000.000000000000114 ) ;
#39435=ORIENTED_EDGE ( 'NONE', *, *, #48503, .T. ) ;
#39436=ORIENTED_EDGE ( 'NONE', *, *, #31142, .T. ) ;
#39437=VECTOR ( 'NONE', #8902, 999.9999999999998863 ) ;
#39438=EDGE_LOOP ( 'NONE', ( #1731, #25157, #15900, #7958 ) ) ;
#39439=VECTOR ( 'NONE', #19172, 1000.000000000000227 ) ;
#39440=ORIENTED_EDGE ( 'NONE', *, *, #26882, .T. ) ;
#39441=LINE ( 'NONE', #4258, #3329 ) ;
#39442=DIRECTION ( 'NONE',  ( 0.9999697198139515519, 0.000000000000000000, 0.007781995580013368816 ) ) ;
#39443=AXIS2_PLACEMENT_3D ( 'NONE', #39176, #38337, #51116 ) ;
#39444=EDGE_CURVE ( 'NONE', #44308, #51416, #19424, .T. ) ;
#39446=VERTEX_POINT ( 'NONE', #48062 ) ;
#39447=ORIENTED_EDGE ( 'NONE', *, *, #13742, .F. ) ;
#39448=EDGE_CURVE ( 'NONE', #46834, #23390, #14296, .T. ) ;
#39449=AXIS2_PLACEMENT_3D ( 'NONE', #21693, #25963, #22245 ) ;
#39450=VECTOR ( 'NONE', #48111, 1000.000000000000000 ) ;
#39451=FACE_OUTER_BOUND ( 'NONE', #8996, .T. ) ;
#39452=ORIENTED_EDGE ( 'NONE', *, *, #22475, .T. ) ;
#39454=DIRECTION ( 'NONE',  ( 0.000000000000000000, -1.000000000000000000, 0.000000000000000000 ) ) ;
#39455=ORIENTED_EDGE ( 'NONE', *, *, #34002, .F. ) ;
#39456=PLANE ( 'NONE',  #32835 ) ;
#39457=VERTEX_POINT ( 'NONE', #912 ) ;
#39458=DIRECTION ( 'NONE',  ( 0.000000000000000000, -1.000000000000000000, 0.000000000000000000 ) ) ;
#39459=VECTOR ( 'NONE', #45832, 999.9999999999998863 ) ;
#39460=CARTESIAN_POINT ( 'NONE',  ( -25.20200914511100265, -0.1191753592594197858, 6.570942640130446932 ) ) ;
#39461=DIRECTION ( 'NONE',  ( -0.005961354470445682716, -0.6427876096865404731, 0.7660212471507180654 ) ) ;
#39462=ORIENTED_EDGE ( 'NONE', *, *, #20753, .T. ) ;
#39463=CARTESIAN_POINT ( 'NONE',  ( -24.27063949748155380, 0.000000000000000000, 6.308861732390097288 ) ) ;
#39464=CARTESIAN_POINT ( 'NONE',  ( -9.636218942796791254, 0.000000000000000000, 6.961408260418826544 ) ) ;
#39465=FACE_OUTER_BOUND ( 'NONE', #13059, .T. ) ;
#39466=VECTOR ( 'NONE', #54713, 1000.000000000000227 ) ;
#39467=ORIENTED_EDGE ( 'NONE', *, *, #20239, .T. ) ;
#39468=LINE ( 'NONE', #568, #2888 ) ;
#39469=ORIENTED_EDGE ( 'NONE', *, *, #54389, .F. ) ;
#39470=VECTOR ( 'NONE', #32068, 1000.000000000000114 ) ;
#39471=DIRECTION ( 'NONE',  ( -0.9999697198139514409, -0.000000000000000000, -0.007781995580013368816 ) ) ;
#39472=LINE ( 'NONE', #22141, #50484 ) ;
#39473=CARTESIAN_POINT ( 'NONE',  ( -28.93137873341882127, 0.000000000000000000, 8.119251130998824451 ) ) ;
#39474=CARTESIAN_POINT ( 'NONE',  ( -9.337105429206005169, -0.06496798097431694119, 2.955599522707465177 ) ) ;
#39475=VECTOR ( 'NONE', #46645, 1000.000000000000227 ) ;
#39476=DIRECTION ( 'NONE',  ( 0.5364919789714477361, 0.6444004775717706579, 0.5449076811759711036 ) ) ;
#39477=EDGE_CURVE ( 'NONE', #12259, #6907, #48912, .T. ) ;
#39478=CARTESIAN_POINT ( 'NONE',  ( -15.09229358671853127, 0.000000000000000000, 7.288279895752441284 ) ) ;
#39479=CARTESIAN_POINT ( 'NONE',  ( -12.33850799832341849, 0.000000000000000000, 11.68350162852954632 ) ) ;
#39480=CARTESIAN_POINT ( 'NONE',  ( -14.95473343100087149, -2.298917212465658277, 6.263772860196296755 ) ) ;
#39481=AXIS2_PLACEMENT_3D ( 'NONE', #51621, #52185, #22646 ) ;
#39482=VECTOR ( 'NONE', #44976, 1000.000000000000114 ) ;
#39483=EDGE_CURVE ( 'NONE', #48148, #8713, #13446, .T. ) ;
#39484=VECTOR ( 'NONE', #29578, 1000.000000000000227 ) ;
#39485=DIRECTION ( 'NONE',  ( 0.5449076811759707706, 0.6444004775717708799, -0.5364919789714476250 ) ) ;
#39486=ORIENTED_EDGE ( 'NONE', *, *, #30304, .T. ) ;
#39487=LINE ( 'NONE', #25869, #32912 ) ;
#39488=PLANE ( 'NONE',  #10031 ) ;
#39489=EDGE_CURVE ( 'NONE', #18842, #9247, #44365, .T. ) ;
#39490=LINE ( 'NONE', #16553, #38632 ) ;
#39491=VECTOR ( 'NONE', #11549, 1000.000000000000227 ) ;
#39492=VECTOR ( 'NONE', #48151, 1000.000000000000114 ) ;
#39493=ADVANCED_FACE ( 'NONE', ( #659 ), #36148, .F. ) ;
#39494=DIRECTION ( 'NONE',  ( -0.005002170337468016433, -0.7660444431189770143, 0.6427681459581293666 ) ) ;
#39495=LINE ( 'NONE', #47736, #18789 ) ;
#39496=DIRECTION ( 'NONE',  ( -0.5449076811759708816, 0.6444004775717707689, 0.5364919789714475140 ) ) ;
#39497=VERTEX_POINT ( 'NONE', #26478 ) ;
#39498=VECTOR ( 'NONE', #33825, 1000.000000000000227 ) ;
#39499=AXIS2_PLACEMENT_3D ( 'NONE', #44415, #5812, #5519 ) ;
#39500=ORIENTED_EDGE ( 'NONE', *, *, #45901, .F. ) ;
#39503=CARTESIAN_POINT ( 'NONE',  ( -14.46888367232926420, 0.000000000000000000, 12.59025272694991315 ) ) ;
#39504=DIRECTION ( 'NONE',  ( 0.7660212471507180654, -0.6427876096865404731, 0.005961354470445141482 ) ) ;
#39505=VERTEX_POINT ( 'NONE', #48334 ) ;
#39506=FACE_OUTER_BOUND ( 'NONE', #4600, .T. ) ;
#39507=ORIENTED_EDGE ( 'NONE', *, *, #8349, .F. ) ;
#39508=CARTESIAN_POINT ( 'NONE',  ( -27.99923088623136636, 0.000000000000000000, 7.757173251277078130 ) ) ;
#39509=VECTOR ( 'NONE', #42358, 1000.000000000000227 ) ;
#39510=VERTEX_POINT ( 'NONE', #43795 ) ;
#39511=ORIENTED_EDGE ( 'NONE', *, *, #397, .T. ) ;
#39512=ORIENTED_EDGE ( 'NONE', *, *, #50301, .F. ) ;
#39513=VECTOR ( 'NONE', #51974, 1000.000000000000227 ) ;
#39514=DIRECTION ( 'NONE',  ( 0.5449076811759707706, 0.6444004775717708799, -0.5364919789714476250 ) ) ;
#39515=DIRECTION ( 'NONE',  ( -0.6427681459581293666, -0.7660444431189770143, -0.005002170337467561935 ) ) ;
#39516=VECTOR ( 'NONE', #35416, 1000.000000000000227 ) ;
#39517=LINE ( 'NONE', #48018, #6724 ) ;
#39518=ADVANCED_FACE ( 'NONE', ( #53448 ), #5752, .F. ) ;
#39519=DIRECTION ( 'NONE',  ( 0.005961354470445682716, -0.6427876096865404731, -0.7660212471507180654 ) ) ;
#39520=ORIENTED_EDGE ( 'NONE', *, *, #12487, .T. ) ;
#39521=VECTOR ( 'NONE', #33522, 999.9999999999998863 ) ;
#39522=ORIENTED_EDGE ( 'NONE', *, *, #34401, .T. ) ;
#39523=EDGE_CURVE ( 'NONE', #52679, #25619, #39569, .T. ) ;
#39524=ADVANCED_FACE ( 'NONE', ( #39266 ), #35301, .F. ) ;
#39525=AXIS2_PLACEMENT_3D ( 'NONE', #24769, #20525, #15409 ) ;
#39526=AXIS2_PLACEMENT_3D ( 'NONE', #33620, #37319, #19451 ) ;
#39527=LINE ( 'NONE', #52306, #31819 ) ;
#39528=EDGE_LOOP ( 'NONE', ( #50527, #55395, #22176, #10619 ) ) ;
#39529=DIRECTION ( 'NONE',  ( 0.7660212471507180654, -0.6427876096865404731, 0.005961354470445141482 ) ) ;
#39530=ORIENTED_EDGE ( 'NONE', *, *, #48019, .F. ) ;
#39531=CARTESIAN_POINT ( 'NONE',  ( -21.96445785857699562, 4.333955019861511992, 5.075397224011642727 ) ) ;
#39532=DIRECTION ( 'NONE',  ( 0.7660212471507180654, -0.6427876096865404731, 0.005961354470445141482 ) ) ;
#39533=VECTOR ( 'NONE', #32757, 999.9999999999998863 ) ;
#39534=ORIENTED_EDGE ( 'NONE', *, *, #37015, .T. ) ;
#39535=VECTOR ( 'NONE', #52446, 999.9999999999998863 ) ;
#39537=VECTOR ( 'NONE', #48195, 999.9999999999998863 ) ;
#39538=ORIENTED_EDGE ( 'NONE', *, *, #27450, .F. ) ;
#39540=VECTOR ( 'NONE', #21188, 999.9999999999998863 ) ;
#39542=VECTOR ( 'NONE', #11254, 1000.000000000000114 ) ;
#39543=VERTEX_POINT ( 'NONE', #31314 ) ;
#39544=PLANE ( 'NONE',  #45876 ) ;
#39545=DIRECTION ( 'NONE',  ( -0.005002170337468016433, -0.7660444431189770143, 0.6427681459581293666 ) ) ;
#39546=CARTESIAN_POINT ( 'NONE',  ( -12.23851102634202448, -0.1191753592594197858, 11.68427982808754884 ) ) ;
#39547=EDGE_LOOP ( 'NONE', ( #30035, #55392, #52350, #55276 ) ) ;
#39548=CARTESIAN_POINT ( 'NONE',  ( -16.79925329029790149, 0.000000000000000000, 13.49544742625427496 ) ) ;
#39549=DIRECTION ( 'NONE',  ( 0.000000000000000000, -1.000000000000000000, 0.000000000000000000 ) ) ;
#39550=CARTESIAN_POINT ( 'NONE',  ( -19.86151716922415034, 0.000000000000000000, 4.496514192825078915 ) ) ;
#39551=DIRECTION ( 'NONE',  ( 0.6427681459581294776, -0.7660444431189769032, 0.005002170337467562802 ) ) ;
#39552=CARTESIAN_POINT ( 'NONE',  ( -15.28175012032331459, 3.038739411681508518, 2.520930751862971331 ) ) ;
#39553=CARTESIAN_POINT ( 'NONE',  ( -25.20278734466900517, 0.000000000000000000, 6.670939612111840944 ) ) ;
#39554=AXIS2_PLACEMENT_3D ( 'NONE', #13248, #18315, #30278 ) ;
#39555=ORIENTED_EDGE ( 'NONE', *, *, #28711, .F. ) ;
#39556=CARTESIAN_POINT ( 'NONE',  ( -15.13495153988577968, 0.000000000000000000, 12.76973526769478084 ) ) ;
#39557=DIRECTION ( 'NONE',  ( -0.5449076811759708816, 0.6444004775717707689, 0.5364919789714475140 ) ) ;
#39558=PLANE ( 'NONE',  #12405 ) ;
#39559=ORIENTED_EDGE ( 'NONE', *, *, #3850, .T. ) ;
#39560=FACE_OUTER_BOUND ( 'NONE', #33028, .T. ) ;
#39562=VECTOR ( 'NONE', #8686, 1000.000000000000000 ) ;
#39563=ORIENTED_EDGE ( 'NONE', *, *, #39713, .T. ) ;
#39564=DIRECTION ( 'NONE',  ( 0.007781995580012663651, -3.146120232559066537E-19, -0.9999697198139514409 ) ) ;
#39565=ADVANCED_FACE ( 'NONE', ( #35564 ), #26770, .F. ) ;
#39566=LINE ( 'NONE', #17393, #28443 ) ;
#39567=VECTOR ( 'NONE', #41140, 1000.000000000000227 ) ;
#39568=CARTESIAN_POINT ( 'NONE',  ( -25.20278734466900517, 0.000000000000000000, 6.670939612111840944 ) ) ;
#39569=LINE ( 'NONE', #10006, #32845 ) ;
#39570=ORIENTED_EDGE ( 'NONE', *, *, #40012, .F. ) ;
#39571=AXIS2_PLACEMENT_3D ( 'NONE', #44950, #1204, #39845 ) ;
#39573=ORIENTED_EDGE ( 'NONE', *, *, #13357, .T. ) ;
#39574=PLANE ( 'NONE',  #18572 ) ;
#39575=CARTESIAN_POINT ( 'NONE',  ( -9.765605855588104234, 0.000000000000000000, 5.313747048732751388 ) ) ;
#39577=VECTOR ( 'NONE', #37634, 1000.000000000000114 ) ;
#39578=EDGE_CURVE ( 'NONE', #29224, #55190, #27318, .T. ) ;
#39580=AXIS2_PLACEMENT_3D ( 'NONE', #54053, #23655, #54321 ) ;
#39581=DIRECTION ( 'NONE',  ( 0.5449076811759707706, 0.6444004775717708799, -0.5364919789714476250 ) ) ;
#39582=DIRECTION ( 'NONE',  ( -0.005002170337468016433, -0.7660444431189770143, 0.6427681459581293666 ) ) ;
#39583=ORIENTED_EDGE ( 'NONE', *, *, #50006, .T. ) ;
#39584=EDGE_CURVE ( 'NONE', #40212, #47084, #8916, .T. ) ;
#39585=DIRECTION ( 'NONE',  ( -0.005002170337468016433, -0.7660444431189770143, 0.6427681459581293666 ) ) ;
#39586=EDGE_CURVE ( 'NONE', #32587, #11776, #21939, .T. ) ;
#39587=AXIS2_PLACEMENT_3D ( 'NONE', #25322, #46058, #38373 ) ;
#39588=AXIS2_PLACEMENT_3D ( 'NONE', #26847, #17195, #44170 ) ;
#39589=CARTESIAN_POINT ( 'NONE',  ( -15.86710544311044302, 0.000000000000000000, 13.13336954653252953 ) ) ;
#39590=EDGE_LOOP ( 'NONE', ( #55146, #17457, #9111, #4582 ) ) ;
#39591=DIRECTION ( 'NONE',  ( 0.5449076811759707706, 0.6444004775717708799, -0.5364919789714476250 ) ) ;
#39592=EDGE_CURVE ( 'NONE', #42084, #5690, #39833, .T. ) ;
#39593=DIRECTION ( 'NONE',  ( 0.9999697198139515519, 0.000000000000000000, 0.007781995580013368816 ) ) ;
#39594=LINE ( 'NONE', #40419, #51987 ) ;
#39596=DIRECTION ( 'NONE',  ( 0.6427681459581294776, -0.7660444431189769032, 0.005002170337467562802 ) ) ;
#39597=ADVANCED_FACE ( 'NONE', ( #18522 ), #10594, .F. ) ;
#39598=ORIENTED_EDGE ( 'NONE', *, *, #32306, .F. ) ;
#39599=EDGE_CURVE ( 'NONE', #47757, #11984, #23895, .T. ) ;
#39600=VECTOR ( 'NONE', #38636, 1000.000000000000000 ) ;
#39601=ORIENTED_EDGE ( 'NONE', *, *, #10376, .F. ) ;
#39602=ORIENTED_EDGE ( 'NONE', *, *, #8635, .F. ) ;
#39603=ORIENTED_EDGE ( 'NONE', *, *, #28741, .T. ) ;
#39604=LINE ( 'NONE', #48088, #46573 ) ;
#39605=VECTOR ( 'NONE', #15310, 1000.000000000000227 ) ;
#39606=VERTEX_POINT ( 'NONE', #27908 ) ;
#39607=CARTESIAN_POINT ( 'NONE',  ( -11.62127938944716377, 0.000000000000000000, 4.929973698402949189 ) ) ;
#39608=EDGE_CURVE ( 'NONE', #8988, #54304, #11108, .T. ) ;
#39609=ORIENTED_EDGE ( 'NONE', *, *, #20775, .T. ) ;
#39610=DIRECTION ( 'NONE',  ( 0.9999697198139515519, 0.000000000000000000, 0.007781995580013368816 ) ) ;
#39611=VECTOR ( 'NONE', #31178, 1000.000000000000227 ) ;
#39612=ORIENTED_EDGE ( 'NONE', *, *, #9713, .F. ) ;
#39613=CARTESIAN_POINT ( 'NONE',  ( -19.79569077582305070, 0.000000000000000000, 14.58012466630350445 ) ) ;
#39614=ORIENTED_EDGE ( 'NONE', *, *, #6738, .F. ) ;
#39615=EDGE_CURVE ( 'NONE', #12878, #35417, #32691, .T. ) ;
#39616=VECTOR ( 'NONE', #49867, 999.9999999999998863 ) ;
#39617=DIRECTION ( 'NONE',  ( -0.9999697198139514409, -0.000000000000000000, -0.007781995580013368816 ) ) ;
#39618=CARTESIAN_POINT ( 'NONE',  ( -9.463279351066496758, -0.1191753592594187727, 2.630772306739904032 ) ) ;
#39619=DIRECTION ( 'NONE',  ( -0.5449076811759708816, 0.6444004775717707689, 0.5364919789714475140 ) ) ;
#39620=DIRECTION ( 'NONE',  ( -0.5449076811759708816, 0.6444004775717707689, 0.5364919789714475140 ) ) ;
#39621=LINE ( 'NONE', #22288, #27456 ) ;
#39623=ORIENTED_EDGE ( 'NONE', *, *, #28296, .F. ) ;
#39624=AXIS2_PLACEMENT_3D ( 'NONE', #34304, #34859, #43097 ) ;
#39625=CARTESIAN_POINT ( 'NONE',  ( -9.397313677665129816, -0.1191753592594181482, 4.847278085703597306 ) ) ;
#39626=FACE_OUTER_BOUND ( 'NONE', #32817, .T. ) ;
#39627=AXIS2_PLACEMENT_3D ( 'NONE', #1649, #22949, #9905 ) ;
#39628=DIRECTION ( 'NONE',  ( 0.5449076811759707706, 0.6444004775717708799, -0.5364919789714476250 ) ) ;
#39629=AXIS2_PLACEMENT_3D ( 'NONE', #37751, #54219, #19852 ) ;
#39630=DIRECTION ( 'NONE',  ( 0.6427681459581294776, -0.7660444431189769032, 0.005002170337467562802 ) ) ;
#39631=DIRECTION ( 'NONE',  ( 0.6427681459581294776, -0.7660444431189769032, 0.005002170337467562802 ) ) ;
#39632=LINE ( 'NONE', #5266, #15949 ) ;
#39633=VERTEX_POINT ( 'NONE', #45750 ) ;
#39634=PLANE ( 'NONE',  #30245 ) ;
#39636=ORIENTED_EDGE ( 'NONE', *, *, #7305, .T. ) ;
#39637=FACE_OUTER_BOUND ( 'NONE', #5180, .T. ) ;
#39638=DIRECTION ( 'NONE',  ( -0.5449076811759708816, 0.6444004775717707689, 0.5364919789714475140 ) ) ;
#39639=EDGE_CURVE ( 'NONE', #23263, #54036, #19073, .T. ) ;
#39640=CARTESIAN_POINT ( 'NONE',  ( -16.33317936670417225, 0.000000000000000000, 13.31440848639340224 ) ) ;
#39641=CARTESIAN_POINT ( 'NONE',  ( -20.54204810873173415, 0.000000000000000000, 4.860550213503115558 ) ) ;
#39643=LINE ( 'NONE', #53511, #49185 ) ;
#39644=ORIENTED_EDGE ( 'NONE', *, *, #55538, .T. ) ;
#39645=ORIENTED_EDGE ( 'NONE', *, *, #4579, .T. ) ;
#39646=CARTESIAN_POINT ( 'NONE',  ( -32.65997012216863737, 0.000000000000000000, 9.567562649885804404 ) ) ;
#39647=CARTESIAN_POINT ( 'NONE',  ( 2.072287782118878319, 0.000000000000000000, -2.950529333540147015 ) ) ;
#39648=PLANE ( 'NONE',  #32434 ) ;
#39649=DIRECTION ( 'NONE',  ( 0.000000000000000000, -0.000000000000000000, -1.000000000000000000 ) ) ;
#39650=VECTOR ( 'NONE', #36033, 999.9999999999998863 ) ;
#39651=LINE ( 'NONE', #5541, #8604 ) ;
#39652=LINE ( 'NONE', #52673, #52730 ) ;
#39653=DIRECTION ( 'NONE',  ( -0.005002170337468016433, -0.7660444431189770143, 0.6427681459581293666 ) ) ;
#39654=EDGE_CURVE ( 'NONE', #45114, #53352, #6052, .T. ) ;
#39655=LINE ( 'NONE', #17480, #545 ) ;
#39656=VECTOR ( 'NONE', #45011, 1000.000000000000227 ) ;
#39657=DIRECTION ( 'NONE',  ( -0.5364919789714478471, 0.6444004775717705469, -0.5449076811759709926 ) ) ;
#39658=VERTEX_POINT ( 'NONE', #6874 ) ;
#39659=DIRECTION ( 'NONE',  ( -0.005002170337468016433, -0.7660444431189770143, 0.6427681459581293666 ) ) ;
#39660=ORIENTED_EDGE ( 'NONE', *, *, #24695, .T. ) ;
#39661=DIRECTION ( 'NONE',  ( 0.007781995580012662783, 0.000000000000000000, -0.9999697198139514409 ) ) ;
#39662=LINE ( 'NONE', #741, #36592 ) ;
#39663=ORIENTED_EDGE ( 'NONE', *, *, #19860, .T. ) ;
#39664=VECTOR ( 'NONE', #55882, 1000.000000000000227 ) ;
#39665=LINE ( 'NONE', #40768, #45364 ) ;
#39667=ORIENTED_EDGE ( 'NONE', *, *, #38476, .T. ) ;
#39668=EDGE_CURVE ( 'NONE', #50804, #16658, #2317, .T. ) ;
#39669=ORIENTED_EDGE ( 'NONE', *, *, #31248, .T. ) ;
#39671=VERTEX_POINT ( 'NONE', #54834 ) ;
#39672=ORIENTED_EDGE ( 'NONE', *, *, #26905, .T. ) ;
#39673=CARTESIAN_POINT ( 'NONE',  ( 1.971453974394196562, 0.000000000000000000, 10.00639841352631088 ) ) ;
#39674=LINE ( 'NONE', #13800, #19487 ) ;
#39675=EDGE_CURVE ( 'NONE', #6706, #45963, #2595, .T. ) ;
#39676=ORIENTED_EDGE ( 'NONE', *, *, #24051, .F. ) ;
#39677=DIRECTION ( 'NONE',  ( 0.5364919789714477361, 0.6444004775717706579, 0.5449076811759711036 ) ) ;
#39678=EDGE_LOOP ( 'NONE', ( #31496, #21585, #5789, #11407 ) ) ;
#39679=ORIENTED_EDGE ( 'NONE', *, *, #37906, .F. ) ;
#39680=ADVANCED_FACE ( 'NONE', ( #45466 ), #28735, .F. ) ;
#39681=DIRECTION ( 'NONE',  ( -0.5364919789714478471, 0.6444004775717705469, -0.5449076811759709926 ) ) ;
#39683=CARTESIAN_POINT ( 'NONE',  ( -28.92982233430281980, 0.000000000000000000, 7.919257187036034651 ) ) ;
#39684=ORIENTED_EDGE ( 'NONE', *, *, #7464, .T. ) ;
#39685=CARTESIAN_POINT ( 'NONE',  ( -25.20278734466900517, 0.000000000000000000, 6.670939612111840944 ) ) ;
#39686=ORIENTED_EDGE ( 'NONE', *, *, #41986, .T. ) ;
#39687=LINE ( 'NONE', #17827, #18459 ) ;
#39688=CARTESIAN_POINT ( 'NONE',  ( -14.89229964275573970, 0.000000000000000000, 7.289836294868443645 ) ) ;
#39689=VECTOR ( 'NONE', #133, 1000.000000000000227 ) ;
#39690=PLANE ( 'NONE',  #45822 ) ;
#39691=DIRECTION ( 'NONE',  ( 0.007781995580012662783, 0.000000000000000000, -0.9999697198139514409 ) ) ;
#39692=CARTESIAN_POINT ( 'NONE',  ( -21.47263955680318404, 0.000000000000000000, 5.022634149262071190 ) ) ;
#39693=DIRECTION ( 'NONE',  ( -0.005961354470445682716, -0.6427876096865404731, 0.7660212471507180654 ) ) ;
#39694=LINE ( 'NONE', #18948, #33145 ) ;
#39695=ORIENTED_EDGE ( 'NONE', *, *, #37790, .F. ) ;
#39696=DIRECTION ( 'NONE',  ( -0.005961354470445682716, -0.6427876096865404731, 0.7660212471507180654 ) ) ;
#39697=EDGE_CURVE ( 'NONE', #41918, #54227, #36550, .T. ) ;
#39698=VECTOR ( 'NONE', #40988, 999.9999999999998863 ) ;
#39700=FACE_OUTER_BOUND ( 'NONE', #38416, .T. ) ;
#39701=PLANE ( 'NONE',  #32646 ) ;
#39702=ADVANCED_FACE ( 'NONE', ( #36399 ), #31862, .F. ) ;
#39704=DIRECTION ( 'NONE',  ( -0.005002170337468016433, -0.7660444431189770143, 0.6427681459581293666 ) ) ;
#39705=DIRECTION ( 'NONE',  ( -0.005002170337468016433, -0.7660444431189770143, 0.6427681459581293666 ) ) ;
#39706=DIRECTION ( 'NONE',  ( -0.5449076811759708816, 0.6444004775717707689, 0.5364919789714475140 ) ) ;
#39707=ADVANCED_FACE ( 'NONE', ( #40682 ), #32154, .F. ) ;
#39708=EDGE_LOOP ( 'NONE', ( #15270, #27563, #40345, #1272 ) ) ;
#39709=EDGE_CURVE ( 'NONE', #44124, #44724, #49748, .T. ) ;
#39711=PLANE ( 'NONE',  #17649 ) ;
#39712=CARTESIAN_POINT ( 'NONE',  ( -14.01701317841955508, 0.000000000000000000, 2.326005055450897085 ) ) ;
#39713=EDGE_CURVE ( 'NONE', #45704, #47757, #16484, .T. ) ;
#39715=EDGE_CURVE ( 'NONE', #17269, #2394, #21024, .T. ) ;
#39716=CARTESIAN_POINT ( 'NONE',  ( -22.40478740399063895, 0.000000000000000000, 5.384712028983816623 ) ) ;
#39717=LINE ( 'NONE', #18111, #1290 ) ;
#39718=DIRECTION ( 'NONE',  ( -0.7660212471507179544, -0.6427876096865405842, -0.005961354470445141482 ) ) ;
#39719=DIRECTION ( 'NONE',  ( -0.8531650599175527594, 0.4028455766673922356, 0.3313982828793700652 ) ) ;
#39720=CYLINDRICAL_SURFACE ( 'NONE', #7869, 6.999999999999999112 ) ;
#39721=DIRECTION ( 'NONE',  ( 0.007781995580012662783, 0.000000000000000000, -0.9999697198139514409 ) ) ;
#39722=EDGE_LOOP ( 'NONE', ( #50867, #43054, #46984, #14973 ) ) ;
#39723=ADVANCED_FACE ( 'NONE', ( #38653 ), #37818, .F. ) ;
#39724=ADVANCED_FACE ( 'NONE', ( #55129 ), #33538, .F. ) ;
#39725=ORIENTED_EDGE ( 'NONE', *, *, #8901, .T. ) ;
#39726=VERTEX_POINT ( 'NONE', #3999 ) ;
#39728=EDGE_CURVE ( 'NONE', #42362, #14988, #34117, .T. ) ;
#39729=ORIENTED_EDGE ( 'NONE', *, *, #50187, .T. ) ;
#39730=PLANE ( 'NONE',  #10607 ) ;
#39732=EDGE_CURVE ( 'NONE', #38932, #42567, #29269, .T. ) ;
#39733=AXIS2_PLACEMENT_3D ( 'NONE', #28417, #41497, #2579 ) ;
#39734=ORIENTED_EDGE ( 'NONE', *, *, #49247, .F. ) ;
#39736=CARTESIAN_POINT ( 'NONE',  ( -12.80458192191714595, 0.000000000000000000, 11.86454056839041726 ) ) ;
#39737=VERTEX_POINT ( 'NONE', #38352 ) ;
#39739=DIRECTION ( 'NONE',  ( 0.000000000000000000, -0.000000000000000000, -1.000000000000000000 ) ) ;
#39740=VERTEX_POINT ( 'NONE', #7404 ) ;
#39741=LINE ( 'NONE', #9643, #32035 ) ;
#39742=ORIENTED_EDGE ( 'NONE', *, *, #46063, .T. ) ;
#39743=CARTESIAN_POINT ( 'NONE',  ( -16.81345671998191449, 0.000000000000000000, 3.412238694616132495 ) ) ;
#39744=DIRECTION ( 'NONE',  ( 0.005961354470445682716, -0.6427876096865404731, -0.7660212471507180654 ) ) ;
#39745=LINE ( 'NONE', #5380, #8274 ) ;
#39746=FACE_OUTER_BOUND ( 'NONE', #6012, .T. ) ;
#39748=CARTESIAN_POINT ( 'NONE',  ( -14.10280672071693431, -0.1191753592594197858, 12.40843558753103792 ) ) ;
#39749=CARTESIAN_POINT ( 'NONE',  ( -14.95573478672749346, -0.1191753592594190225, 2.590941714392399842 ) ) ;
#39750=PLANE ( 'NONE',  #52036 ) ;
#39751=ORIENTED_EDGE ( 'NONE', *, *, #6740, .T. ) ;
#39752=DIRECTION ( 'NONE',  ( -0.005961354470445682716, -0.6427876096865404731, 0.7660212471507180654 ) ) ;
#39753=VERTEX_POINT ( 'NONE', #50588 ) ;
#39754=CARTESIAN_POINT ( 'NONE',  ( -17.74482636761137044, -0.1191753592594197858, 3.674319602356483916 ) ) ;
#39755=LINE ( 'NONE', #35226, #26907 ) ;
#39756=LINE ( 'NONE', #835, #46715 ) ;
#39757=DIRECTION ( 'NONE',  ( 0.000000000000000000, -1.000000000000000000, 0.000000000000000000 ) ) ;
#39758=CARTESIAN_POINT ( 'NONE',  ( -18.94948708026818807, 4.010151117816509903, 10.82328659761999567 ) ) ;
#39759=CARTESIAN_POINT ( 'NONE',  ( -24.27063949748155380, 0.000000000000000000, 6.308861732390097288 ) ) ;
#39760=DIRECTION ( 'NONE',  ( 0.000000000000000000, -0.000000000000000000, -1.000000000000000000 ) ) ;
#39761=PLANE ( 'NONE',  #1198 ) ;
#39763=LINE ( 'NONE', #53104, #4220 ) ;
#39764=ORIENTED_EDGE ( 'NONE', *, *, #38678, .F. ) ;
#39765=DIRECTION ( 'NONE',  ( -0.5364919789714478471, 0.6444004775717705469, -0.5449076811759709926 ) ) ;
#39766=CARTESIAN_POINT ( 'NONE',  ( -17.44252728881015102, 0.6102101463440037232, 4.658049875088040359 ) ) ;
#39767=FACE_OUTER_BOUND ( 'NONE', #42153, .T. ) ;
#39768=LINE ( 'NONE', #13627, #42279 ) ;
#39769=EDGE_CURVE ( 'NONE', #3456, #17353, #29852, .T. ) ;
#39770=EDGE_CURVE ( 'NONE', #47757, #54534, #21617, .T. ) ;
#39771=VECTOR ( 'NONE', #121, 1000.000000000000114 ) ;
#39772=LINE ( 'NONE', #43721, #25866 ) ;
#39773=EDGE_CURVE ( 'NONE', #27291, #9862, #55677, .T. ) ;
#39774=CARTESIAN_POINT ( 'NONE',  ( -26.13337879274045505, 0.000000000000000000, 6.833023547870798353 ) ) ;
#39775=DIRECTION ( 'NONE',  ( 0.5449076811759707706, 0.6444004775717708799, -0.5364919789714476250 ) ) ;
#39776=ORIENTED_EDGE ( 'NONE', *, *, #48325, .T. ) ;
#39777=ORIENTED_EDGE ( 'NONE', *, *, #54210, .T. ) ;
#39778=DIRECTION ( 'NONE',  ( 0.9999697198139515519, 0.000000000000000000, 0.007781995580013368816 ) ) ;
#39779=DIRECTION ( 'NONE',  ( -0.005002170337468016433, -0.7660444431189770143, 0.6427681459581293666 ) ) ;
#39780=EDGE_LOOP ( 'NONE', ( #33167, #50373, #53209, #13538 ) ) ;
#39781=DIRECTION ( 'NONE',  ( 0.007781995580012663651, 0.000000000000000000, -0.9999697198139515519 ) ) ;
#39782=ORIENTED_EDGE ( 'NONE', *, *, #46237, .F. ) ;
#39783=LINE ( 'NONE', #9388, #41089 ) ;
#39784=EDGE_CURVE ( 'NONE', #18005, #41229, #50844, .T. ) ;
#39785=EDGE_LOOP ( 'NONE', ( #13336, #8268, #10814, #3092 ) ) ;
#39786=ORIENTED_EDGE ( 'NONE', *, *, #42198, .F. ) ;
#39787=ORIENTED_EDGE ( 'NONE', *, *, #36688, .F. ) ;
#39788=EDGE_CURVE ( 'NONE', #55101, #35565, #11942, .T. ) ;
#39789=LINE ( 'NONE', #31816, #47462 ) ;
#39790=PLANE ( 'NONE',  #11436 ) ;
#39791=PLANE ( 'NONE',  #21226 ) ;
#39792=ADVANCED_FACE ( 'NONE', ( #47434 ), #3151, .F. ) ;
#39793=CARTESIAN_POINT ( 'NONE',  ( -25.20278734466900517, 0.000000000000000000, 6.670939612111840944 ) ) ;
#39794=EDGE_LOOP ( 'NONE', ( #13471, #36779, #13590, #4923 ) ) ;
#39795=EDGE_LOOP ( 'NONE', ( #41352, #26465, #28254, #50403 ) ) ;
#39796=ADVANCED_FACE ( 'NONE', ( #8546 ), #51130, .F. ) ;
#39797=PLANE ( 'NONE',  #47247 ) ;
#39798=ORIENTED_EDGE ( 'NONE', *, *, #15268, .F. ) ;
#39799=DIRECTION ( 'NONE',  ( -0.5449076811759708816, 0.6444004775717707689, 0.5364919789714475140 ) ) ;
#39801=DIRECTION ( 'NONE',  ( 0.5364919789714477361, 0.6444004775717706579, 0.5449076811759711036 ) ) ;
#39802=CARTESIAN_POINT ( 'NONE',  ( -14.00280974873554030, 0.000000000000000000, 12.40921378708904044 ) ) ;
#39803=VECTOR ( 'NONE', #5206, 1000.000000000000000 ) ;
#39804=ORIENTED_EDGE ( 'NONE', *, *, #7385, .T. ) ;
#39805=FACE_OUTER_BOUND ( 'NONE', #23945, .T. ) ;
#39806=ORIENTED_EDGE ( 'NONE', *, *, #24479, .T. ) ;
#39807=CARTESIAN_POINT ( 'NONE',  ( -16.29351483940556733, 0.000000000000000000, 8.217601910042732882 ) ) ;
#39808=ORIENTED_EDGE ( 'NONE', *, *, #35008, .T. ) ;
#39809=FACE_OUTER_BOUND ( 'NONE', #14346, .T. ) ;
#39810=CARTESIAN_POINT ( 'NONE',  ( -27.06552663992790997, 0.000000000000000000, 7.195101427592543786 ) ) ;
#39811=CARTESIAN_POINT ( 'NONE',  ( -14.13453828727398864, 2.229229656569006401, 2.101142315865724974 ) ) ;
#39812=ORIENTED_EDGE ( 'NONE', *, *, #3395, .F. ) ;
#39813=CARTESIAN_POINT ( 'NONE',  ( -12.07154601876183975, 0.000000000000000000, 3.079809270346117067 ) ) ;
#39814=PLANE ( 'NONE',  #24674 ) ;
#39815=CARTESIAN_POINT ( 'NONE',  ( -15.91580559589089461, -1.813211359398159583, 3.005709578090212997 ) ) ;
#39816=LINE ( 'NONE', #1472, #26828 ) ;
#39817=DIRECTION ( 'NONE',  ( 0.007781995580012662783, 0.000000000000000000, -0.9999697198139514409 ) ) ;
#39818=CARTESIAN_POINT ( 'NONE',  ( -12.10316060731994803, 0.000000000000000000, 7.142216006181524968 ) ) ;
#39819=ORIENTED_EDGE ( 'NONE', *, *, #43530, .F. ) ;
#39820=CARTESIAN_POINT ( 'NONE',  ( -16.18264749718321838, 0.7721120973665051013, 4.434378462272783317 ) ) ;
#39821=CARTESIAN_POINT ( 'NONE',  ( -20.54204810873173415, 0.000000000000000000, 4.860550213503115558 ) ) ;
#39822=CARTESIAN_POINT ( 'NONE',  ( -25.20123094555300369, 0.000000000000000000, 6.470945668149052032 ) ) ;
#39823=ORIENTED_EDGE ( 'NONE', *, *, #14750, .T. ) ;
#39824=FACE_OUTER_BOUND ( 'NONE', #37703, .T. ) ;
#39825=CARTESIAN_POINT ( 'NONE',  ( -13.12877911992022995, -0.1191753592594185784, 6.664899307848342502 ) ) ;
#39826=ORIENTED_EDGE ( 'NONE', *, *, #29109, .F. ) ;
#39828=DIRECTION ( 'NONE',  ( 0.005002170337468016433, -0.7660444431189770143, -0.6427681459581293666 ) ) ;
#39829=CARTESIAN_POINT ( 'NONE',  ( 2.072287782118878319, 0.000000000000000000, -2.950529333540147015 ) ) ;
#39830=EDGE_CURVE ( 'NONE', #50554, #2552, #46895, .T. ) ;
#39831=ADVANCED_FACE ( 'NONE', ( #23001 ), #26696, .F. ) ;
#39832=DIRECTION ( 'NONE',  ( -0.6246952433987893460, -0.7422098413412802076, 0.2426528472758542054 ) ) ;
#39833=LINE ( 'NONE', #40101, #9338 ) ;
#39834=ORIENTED_EDGE ( 'NONE', *, *, #1060, .T. ) ;
#39835=ORIENTED_EDGE ( 'NONE', *, *, #12248, .F. ) ;
#39836=DIRECTION ( 'NONE',  ( 0.005002170337468016433, -0.7660444431189770143, -0.6427681459581293666 ) ) ;
#39837=CARTESIAN_POINT ( 'NONE',  ( -18.01733923308073670, 4.010151117816509903, 10.46120871789824847 ) ) ;
#39839=CARTESIAN_POINT ( 'NONE',  ( -30.79567442779373110, 0.000000000000000000, 8.843406890442315316 ) ) ;
#39840=VECTOR ( 'NONE', #3138, 999.9999999999998863 ) ;
#39841=CARTESIAN_POINT ( 'NONE',  ( -13.03938975049497984, -2.784623065533158304, 6.316914381194012940 ) ) ;
#39842=CARTESIAN_POINT ( 'NONE',  ( -16.00587945848501192, 0.000000000000000000, 5.265183796632624258 ) ) ;
#39843=ORIENTED_EDGE ( 'NONE', *, *, #50814, .T. ) ;
#39844=CARTESIAN_POINT ( 'NONE',  ( -17.73140113748535285, 0.000000000000000000, 13.85752530597602039 ) ) ;
#39845=DIRECTION ( 'NONE',  ( -0.005002170337468016433, -0.7660444431189770143, 0.6427681459581293666 ) ) ;
#39846=ORIENTED_EDGE ( 'NONE', *, *, #44441, .T. ) ;
#39847=DIRECTION ( 'NONE',  ( 0.005002170337468016433, -0.7660444431189770143, -0.6427681459581293666 ) ) ;
#39848=CARTESIAN_POINT ( 'NONE',  ( -13.73672976910459909, 0.000000000000000000, 12.22661844811216270 ) ) ;
#39849=DIRECTION ( 'NONE',  ( 0.9999697198139515519, 0.000000000000000000, 0.007781995580013368816 ) ) ;
#39850=ORIENTED_EDGE ( 'NONE', *, *, #1561, .F. ) ;
#39851=CARTESIAN_POINT ( 'NONE',  ( -9.808144436391993182, 0.000000000000000000, 10.77986332834118777 ) ) ;
#39853=EDGE_CURVE ( 'NONE', #2673, #8988, #44307, .T. ) ;
#39854=EDGE_LOOP ( 'NONE', ( #33719, #51881, #55777, #7105 ) ) ;
#39855=ORIENTED_EDGE ( 'NONE', *, *, #52536, .F. ) ;
#39856=EDGE_CURVE ( 'NONE', #10112, #54371, #30416, .T. ) ;
#39857=ORIENTED_EDGE ( 'NONE', *, *, #2728, .F. ) ;
#39858=CARTESIAN_POINT ( 'NONE',  ( -15.36711509922867869, 0.000000000000000000, 8.594143436836516159 ) ) ;
#39859=ADVANCED_FACE ( 'NONE', ( #30701 ), #4838, .F. ) ;
#39860=ORIENTED_EDGE ( 'NONE', *, *, #29786, .T. ) ;
#39861=CARTESIAN_POINT ( 'NONE',  ( -13.17065887352947762, -0.1191753592594197858, 12.04635770780929427 ) ) ;
#39862=DIRECTION ( 'NONE',  ( -0.005002170337468016433, -0.7660444431189770143, 0.6427681459581293666 ) ) ;
#39863=ORIENTED_EDGE ( 'NONE', *, *, #30338, .T. ) ;
#39864=LINE ( 'NONE', #9787, #12309 ) ;
#39865=EDGE_CURVE ( 'NONE', #2789, #39305, #9377, .T. ) ;
#39866=ORIENTED_EDGE ( 'NONE', *, *, #49709, .F. ) ;
#39867=FACE_OUTER_BOUND ( 'NONE', #31417, .T. ) ;
#39868=ORIENTED_EDGE ( 'NONE', *, *, #25788, .F. ) ;
#39869=CARTESIAN_POINT ( 'NONE',  ( -11.77243710274829525, -0.1191753592594197858, 11.50324088822667612 ) ) ;
#39870=DIRECTION ( 'NONE',  ( 0.007781995580012663651, 0.000000000000000000, -0.9999697198139515519 ) ) ;
#39871=DIRECTION ( 'NONE',  ( 0.6246952433987893460, 0.7422098413412802076, -0.2426528472758539279 ) ) ;
#39872=PLANE ( 'NONE',  #18473 ) ;
#39873=LINE ( 'NONE', #52387, #33251 ) ;
#39874=CARTESIAN_POINT ( 'NONE',  ( -14.12468155607537845, -1.327505506330655782, 4.347100419592131004 ) ) ;
#39875=ORIENTED_EDGE ( 'NONE', *, *, #37999, .F. ) ;
#39876=ORIENTED_EDGE ( 'NONE', *, *, #45, .T. ) ;
#39880=DIRECTION ( 'NONE',  ( 0.7660212471507180654, -0.6427876096865404731, 0.005961354470445141482 ) ) ;
#39881=DIRECTION ( 'NONE',  ( 0.007781995580012662783, 0.000000000000000000, -0.9999697198139514409 ) ) ;
#39882=ORIENTED_EDGE ( 'NONE', *, *, #17490, .T. ) ;
#39883=PLANE ( 'NONE',  #15932 ) ;
#39884=CARTESIAN_POINT ( 'NONE',  ( -10.96739633006137105, 0.000000000000000000, 1.041735613279166195 ) ) ;
#39885=ORIENTED_EDGE ( 'NONE', *, *, #37514, .T. ) ;
#39886=DIRECTION ( 'NONE',  ( 0.007781995580012662783, 0.000000000000000000, -0.9999697198139514409 ) ) ;
#39887=EDGE_CURVE ( 'NONE', #54373, #21014, #47998, .T. ) ;
#39888=DIRECTION ( 'NONE',  ( 0.6427681459581294776, -0.7660444431189769032, 0.005002170337467562802 ) ) ;
#39889=ORIENTED_EDGE ( 'NONE', *, *, #10651, .F. ) ;
#39890=DIRECTION ( 'NONE',  ( 0.9999697198139515519, 0.000000000000000000, 0.007781995580013368816 ) ) ;
#39891=DIRECTION ( 'NONE',  ( 0.000000000000000000, -0.000000000000000000, -1.000000000000000000 ) ) ;
#39892=EDGE_CURVE ( 'NONE', #18488, #1003, #5143, .T. ) ;
#39893=LINE ( 'NONE', #39640, #53152 ) ;
#39894=ADVANCED_FACE ( 'NONE', ( #13630 ), #18170, .F. ) ;
#39895=CARTESIAN_POINT ( 'NONE',  ( -18.30454488918022449, -2.946525016555660237, 8.627788126430976590 ) ) ;
#39896=DIRECTION ( 'NONE',  ( 0.6427681459581294776, -0.7660444431189769032, 0.005002170337467562802 ) ) ;
#39897=EDGE_LOOP ( 'NONE', ( #48113, #23713, #14669, #6271 ) ) ;
#39898=EDGE_LOOP ( 'NONE', ( #6681, #6005, #2348, #6939 ) ) ;
#39899=CARTESIAN_POINT ( 'NONE',  ( -25.20278734466900517, 0.000000000000000000, 6.670939612111840944 ) ) ;
#39900=DIRECTION ( 'NONE',  ( 0.005002170337468016433, -0.7660444431189770143, -0.6427681459581293666 ) ) ;
#39901=CARTESIAN_POINT ( 'NONE',  ( -10.37421533196711465, -0.1191753592594197858, 10.96012406864405975 ) ) ;
#39902=CARTESIAN_POINT ( 'NONE',  ( -21.47419595591918906, 0.000000000000000000, 5.222628093224860102 ) ) ;
#39903=DIRECTION ( 'NONE',  ( -0.5449076811759708816, 0.6444004775717707689, 0.5364919789714475140 ) ) ;
#39904=ORIENTED_EDGE ( 'NONE', *, *, #55792, .F. ) ;
#39906=CARTESIAN_POINT ( 'NONE',  ( -17.66862480978112515, 0.000000000000000000, 5.790902011229328572 ) ) ;
#39907=EDGE_CURVE ( 'NONE', #37913, #27257, #13084, .T. ) ;
#39908=VECTOR ( 'NONE', #53849, 1000.000000000000227 ) ;
#39909=CARTESIAN_POINT ( 'NONE',  ( -19.60912206198628027, -0.1191753592594197858, 4.398475361799976113 ) ) ;
#39910=LINE ( 'NONE', #25734, #16943 ) ;
#39911=ORIENTED_EDGE ( 'NONE', *, *, #26736, .F. ) ;
#39912=PLANE ( 'NONE',  #9316 ) ;
#39913=VERTEX_POINT ( 'NONE', #26152 ) ;
#39914=DIRECTION ( 'NONE',  ( -0.7660212471507179544, -0.6427876096865405842, -0.005961354470445141482 ) ) ;
#39915=CARTESIAN_POINT ( 'NONE',  ( -20.54204810873173415, 0.000000000000000000, 4.860550213503115558 ) ) ;
#39916=ORIENTED_EDGE ( 'NONE', *, *, #6380, .F. ) ;
#39917=LINE ( 'NONE', #45301, #47150 ) ;
#39918=EDGE_LOOP ( 'NONE', ( #2540, #598, #6466, #54301 ) ) ;
#39919=ORIENTED_EDGE ( 'NONE', *, *, #8292, .F. ) ;
#39920=ORIENTED_EDGE ( 'NONE', *, *, #49014, .T. ) ;
#39921=DIRECTION ( 'NONE',  ( -0.9999697198139514409, -0.000000000000000000, -0.007781995580013368816 ) ) ;
#39922=ORIENTED_EDGE ( 'NONE', *, *, #3314, .F. ) ;
#39923=VERTEX_POINT ( 'NONE', #44020 ) ;
#39924=CARTESIAN_POINT ( 'NONE',  ( -10.79122436818839148, -0.1191753592594179401, 4.836430350399566258 ) ) ;
#39925=DIRECTION ( 'NONE',  ( 0.007781995580012663651, 0.000000000000000000, -0.9999697198139515519 ) ) ;
#39926=ORIENTED_EDGE ( 'NONE', *, *, #17916, .T. ) ;
#39927=EDGE_LOOP ( 'NONE', ( #50600, #55098, #56047, #3607 ) ) ;
#39928=LINE ( 'NONE', #43618, #3169 ) ;
#39929=EDGE_CURVE ( 'NONE', #53080, #28729, #14229, .T. ) ;
#39930=ORIENTED_EDGE ( 'NONE', *, *, #21574, .T. ) ;
#39931=ORIENTED_EDGE ( 'NONE', *, *, #5979, .T. ) ;
#39932=DIRECTION ( 'NONE',  ( 0.000000000000000000, -1.000000000000000000, 0.000000000000000000 ) ) ;
#39933=FACE_OUTER_BOUND ( 'NONE', #14466, .T. ) ;
#39934=DIRECTION ( 'NONE',  ( 0.000000000000000000, -0.000000000000000000, -1.000000000000000000 ) ) ;
#39935=DIRECTION ( 'NONE',  ( -0.005002170337468016433, -0.7660444431189770143, 0.6427681459581293666 ) ) ;
#39936=ORIENTED_EDGE ( 'NONE', *, *, #24149, .T. ) ;
#39937=FACE_OUTER_BOUND ( 'NONE', #48580, .T. ) ;
#39938=ORIENTED_EDGE ( 'NONE', *, *, #23705, .F. ) ;
#39939=EDGE_CURVE ( 'NONE', #39023, #43550, #18453, .T. ) ;
#39940=FACE_OUTER_BOUND ( 'NONE', #39987, .T. ) ;
#39941=ADVANCED_FACE ( 'NONE', ( #39189 ), #43460, .F. ) ;
#39942=EDGE_CURVE ( 'NONE', #34091, #10496, #44564, .T. ) ;
#39943=VECTOR ( 'NONE', #17320, 1000.000000000000227 ) ;
#39944=DIRECTION ( 'NONE',  ( 0.7660212471507180654, -0.6427876096865404731, 0.005961354470445141482 ) ) ;
#39945=PLANE ( 'NONE',  #14112 ) ;
#39947=DIRECTION ( 'NONE',  ( 0.007781995580012663651, -3.146120232559066537E-19, -0.9999697198139514409 ) ) ;
#39948=DIRECTION ( 'NONE',  ( 0.000000000000000000, -0.000000000000000000, -1.000000000000000000 ) ) ;
#39949=CARTESIAN_POINT ( 'NONE',  ( -1.450993146028691116, -7.184208846019964234, 3.781988589515998367 ) ) ;
#39950=ORIENTED_EDGE ( 'NONE', *, *, #4425, .F. ) ;
#39951=FACE_OUTER_BOUND ( 'NONE', #54558, .T. ) ;
#39952=ADVANCED_FACE ( 'NONE', ( #51970 ), #31542, .F. ) ;
#39953=DIRECTION ( 'NONE',  ( -0.005002170337468016433, -0.7660444431189770143, 0.6427681459581293666 ) ) ;
#39954=DIRECTION ( 'NONE',  ( 0.005961354470445682716, -0.6427876096865404731, -0.7660212471507180654 ) ) ;
#39955=EDGE_CURVE ( 'NONE', #42246, #23133, #18109, .T. ) ;
#39956=CARTESIAN_POINT ( 'NONE',  ( -17.76652592781524120, -0.1191753592594196748, 5.520811080394955717 ) ) ;
#39958=DIRECTION ( 'NONE',  ( -0.005961354470445682716, -0.6427876096865404731, 0.7660212471507180654 ) ) ;
#39959=ADVANCED_FACE ( 'NONE', ( #17622 ), #34959, .F. ) ;
#39960=DIRECTION ( 'NONE',  ( 0.007781995580012662783, 0.000000000000000000, -0.9999697198139514409 ) ) ;
#39961=CARTESIAN_POINT ( 'NONE',  ( -13.53673582514181106, 0.000000000000000000, 12.22817484722816772 ) ) ;
#39962=EDGE_LOOP ( 'NONE', ( #3152, #3376, #39239, #48208 ) ) ;
#39963=PLANE ( 'NONE',  #37484 ) ;
#39964=CARTESIAN_POINT ( 'NONE',  ( -14.29695817873406405, 0.000000000000000000, 8.771797659027555483 ) ) ;
#39965=CARTESIAN_POINT ( 'NONE',  ( -1.086233639165236964, 0.000000000000000000, -2.796443541562362078 ) ) ;
#39966=EDGE_CURVE ( 'NONE', #7042, #44931, #11040, .T. ) ;
#39967=FACE_OUTER_BOUND ( 'NONE', #21086, .T. ) ;
#39968=LINE ( 'NONE', #35433, #52087 ) ;
#39969=LINE ( 'NONE', #26631, #45098 ) ;
#39970=CARTESIAN_POINT ( 'NONE',  ( -16.02731548741127199, 0.000000000000000000, 8.019667478731950183 ) ) ;
#39971=EDGE_CURVE ( 'NONE', #30096, #20287, #36921, .T. ) ;
#39972=PLANE ( 'NONE',  #600 ) ;
#39973=PLANE ( 'NONE',  #11095 ) ;
#39974=VERTEX_POINT ( 'NONE', #32907 ) ;
#39975=AXIS2_PLACEMENT_3D ( 'NONE', #40364, #6023, #52845 ) ;
#39976=VECTOR ( 'NONE', #50217, 1000.000000000000227 ) ;
#39977=ORIENTED_EDGE ( 'NONE', *, *, #54021, .F. ) ;
#39978=VERTEX_POINT ( 'NONE', #28098 ) ;
#39979=VERTEX_POINT ( 'NONE', #27845 ) ;
#39981=CARTESIAN_POINT ( 'NONE',  ( -16.46033779569424382, 0.000000000000000000, 3.953644831128531489 ) ) ;
#39982=CARTESIAN_POINT ( 'NONE',  ( -11.67244013076689946, 0.000000000000000000, 11.50401908778467863 ) ) ;
#39983=ORIENTED_EDGE ( 'NONE', *, *, #31623, .T. ) ;
#39984=ORIENTED_EDGE ( 'NONE', *, *, #4608, .F. ) ;
#39985=EDGE_CURVE ( 'NONE', #25477, #693, #11334, .T. ) ;
#39986=CARTESIAN_POINT ( 'NONE',  ( 2.072287782118878319, 0.000000000000000000, -2.950529333540147015 ) ) ;
#39987=EDGE_LOOP ( 'NONE', ( #8179, #5369, #16178, #34391 ) ) ;
#39988=CARTESIAN_POINT ( 'NONE',  ( -13.27065584551087163, 0.000000000000000000, 12.04557950825129176 ) ) ;
#39989=CARTESIAN_POINT ( 'NONE',  ( -26.13337879274045505, 0.000000000000000000, 6.833023547870798353 ) ) ;
#39991=DIRECTION ( 'NONE',  ( 0.9999697198139515519, 0.000000000000000000, 0.007781995580013368816 ) ) ;
#39992=EDGE_CURVE ( 'NONE', #14652, #35264, #2532, .T. ) ;
#39993=EDGE_CURVE ( 'NONE', #21352, #31229, #14759, .T. ) ;
#39994=VERTEX_POINT ( 'NONE', #45987 ) ;
#39995=VECTOR ( 'NONE', #18450, 1000.000000000000227 ) ;
#39996=AXIS2_PLACEMENT_3D ( 'NONE', #23327, #37195, #25532 ) ;
#39997=DIRECTION ( 'NONE',  ( -0.9999697198139514409, -0.000000000000000000, -0.007781995580013368816 ) ) ;
#39998=FACE_OUTER_BOUND ( 'NONE', #42301, .T. ) ;
#39999=EDGE_CURVE ( 'NONE', #3951, #42842, #7094, .T. ) ;
#40000=DIRECTION ( 'NONE',  ( 0.007781995580012663651, -3.146120232559066537E-19, -0.9999697198139514409 ) ) ;
#40001=CARTESIAN_POINT ( 'NONE',  ( -10.34383179237899775, -0.1191753592594181482, 7.055904481714163623 ) ) ;
#40002=EDGE_LOOP ( 'NONE', ( #45475, #3028, #1861 ) ) ;
#40003=CARTESIAN_POINT ( 'NONE',  ( -13.21230997042793120, 0.000000000000000000, 4.548259860725153203 ) ) ;
#40004=FACE_OUTER_BOUND ( 'NONE', #15819, .T. ) ;
#40005=LINE ( 'NONE', #48537, #1283 ) ;
#40006=ORIENTED_EDGE ( 'NONE', *, *, #41651, .F. ) ;
#40007=CARTESIAN_POINT ( 'NONE',  ( -13.76383987162373579, 0.000000000000000000, 2.127969252444404713 ) ) ;
#40008=ORIENTED_EDGE ( 'NONE', *, *, #36826, .T. ) ;
#40009=DIRECTION ( 'NONE',  ( -0.005961354470445682716, -0.6427876096865404731, 0.7660212471507180654 ) ) ;
#40010=DIRECTION ( 'NONE',  ( 0.9999697198139515519, 0.000000000000000000, 0.007781995580013368816 ) ) ;
#40011=CARTESIAN_POINT ( 'NONE',  ( -8.975993561185934055, -0.1191753592594197858, 10.41700724906143982 ) ) ;
#40012=EDGE_CURVE ( 'NONE', #21780, #41291, #40621, .T. ) ;
#40013=PLANE ( 'NONE',  #47705 ) ;
#40014=LINE ( 'NONE', #14472, #54062 ) ;
#40016=CARTESIAN_POINT ( 'NONE',  ( -32.65841372305263235, 0.000000000000000000, 9.367568705923016381 ) ) ;
#40017=VECTOR ( 'NONE', #8507, 1000.000000000000000 ) ;
#40018=EDGE_CURVE ( 'NONE', #40865, #5570, #5981, .T. ) ;
#40019=DIRECTION ( 'NONE',  ( 0.9999697198139515519, 0.000000000000000000, 0.007781995580013368816 ) ) ;
#40020=( LENGTH_UNIT ( ) NAMED_UNIT ( * ) SI_UNIT ( .MILLI., .METRE. ) );
#40021=EDGE_CURVE ( 'NONE', #54304, #21718, #54220, .T. ) ;
#40022=LINE ( 'NONE', #35485, #30526 ) ;
#40023=ORIENTED_EDGE ( 'NONE', *, *, #52903, .T. ) ;
#40024=DIRECTION ( 'NONE',  ( 0.005961354470445682716, -0.6427876096865404731, -0.7660212471507180654 ) ) ;
#40025=DIRECTION ( 'NONE',  ( -0.005002170337468016433, -0.7660444431189770143, 0.6427681459581293666 ) ) ;
#40026=LINE ( 'NONE', #43201, #52661 ) ;
#40028=LINE ( 'NONE', #6251, #31285 ) ;
#40029=ADVANCED_FACE ( 'NONE', ( #23825 ), #37172, .F. ) ;
#40030=LINE ( 'NONE', #5141, #19161 ) ;
#40031=DIRECTION ( 'NONE',  ( -0.005002170337468016433, -0.7660444431189770143, 0.6427681459581293666 ) ) ;
#40033=ORIENTED_EDGE ( 'NONE', *, *, #4878, .F. ) ;
#40034=ORIENTED_EDGE ( 'NONE', *, *, #47239, .T. ) ;
#40035=CARTESIAN_POINT ( 'NONE',  ( -21.36715069126009325, 4.657758921906509642, 12.82522398413292741 ) ) ;
#40037=CARTESIAN_POINT ( 'NONE',  ( -16.38985955832367836, -0.1191753592594190225, 7.747517035245570227 ) ) ;
#40038=VECTOR ( 'NONE', #34806, 1000.000000000000114 ) ;
#40039=VECTOR ( 'NONE', #16131, 1000.000000000000227 ) ;
#40040=ORIENTED_EDGE ( 'NONE', *, *, #39999, .T. ) ;
#40041=CARTESIAN_POINT ( 'NONE',  ( -11.77243710274829525, -0.1191753592594197858, 11.50324088822667612 ) ) ;
#40042=VERTEX_POINT ( 'NONE', #18764 ) ;
#40043=LINE ( 'NONE', #17339, #55596 ) ;
#40044=ORIENTED_EDGE ( 'NONE', *, *, #6299, .T. ) ;
#40045=EDGE_LOOP ( 'NONE', ( #8512, #11705, #52368, #37980 ) ) ;
#40046=AXIS2_PLACEMENT_3D ( 'NONE', #33581, #15420, #2368 ) ;
#40049=FACE_OUTER_BOUND ( 'NONE', #42757, .T. ) ;
#40051=EDGE_CURVE ( 'NONE', #35922, #21974, #36087, .T. ) ;
#40052=CARTESIAN_POINT ( 'NONE',  ( -15.60102546347950536, 0.000000000000000000, 12.95077420755565356 ) ) ;
#40053=EDGE_LOOP ( 'NONE', ( #34459, #34339, #39435, #37064 ) ) ;
#40054=EDGE_CURVE ( 'NONE', #14368, #873, #15320, .T. ) ;
#40056=VECTOR ( 'NONE', #18015, 999.9999999999998863 ) ;
#40057=CARTESIAN_POINT ( 'NONE',  ( -24.26908309836554878, 0.000000000000000000, 6.108867788427308376 ) ) ;
#40058=ORIENTED_EDGE ( 'NONE', *, *, #49364, .T. ) ;
#40059=FACE_OUTER_BOUND ( 'NONE', #785, .T. ) ;
#40060=ORIENTED_EDGE ( 'NONE', *, *, #33425, .T. ) ;
#40061=LINE ( 'NONE', #44594, #38745 ) ;
#40062=DIRECTION ( 'NONE',  ( -0.005961354470445682716, -0.6427876096865404731, 0.7660212471507180654 ) ) ;
#40063=EDGE_CURVE ( 'NONE', #52847, #5849, #44859, .T. ) ;
#40064=EDGE_CURVE ( 'NONE', #50295, #26566, #32632, .T. ) ;
#40065=EDGE_CURVE ( 'NONE', #36873, #27011, #45156, .T. ) ;
#40066=ORIENTED_EDGE ( 'NONE', *, *, #35845, .T. ) ;
#40067=CARTESIAN_POINT ( 'NONE',  ( -25.20278734466900517, 0.000000000000000000, 6.670939612111840944 ) ) ;
#40068=ORIENTED_EDGE ( 'NONE', *, *, #19041, .T. ) ;
#40069=ADVANCED_FACE ( 'NONE', ( #23560 ), #40875, .F. ) ;
#40070=PLANE ( 'NONE',  #17302 ) ;
#40071=ORIENTED_EDGE ( 'NONE', *, *, #36623, .F. ) ;
#40072=DIRECTION ( 'NONE',  ( 0.9999697198139515519, 0.000000000000000000, 0.007781995580013368816 ) ) ;
#40073=CARTESIAN_POINT ( 'NONE',  ( -13.57329764222433788, -0.1191753592594185784, 4.076115473275981671 ) ) ;
#40074=LINE ( 'NONE', #40912, #16520 ) ;
#40075=VERTEX_POINT ( 'NONE', #53933 ) ;
#40076=VECTOR ( 'NONE', #28674, 1000.000000000000114 ) ;
#40077=AXIS2_PLACEMENT_3D ( 'NONE', #45442, #1729, #41197 ) ;
#40078=LINE ( 'NONE', #23342, #33757 ) ;
#40079=CARTESIAN_POINT ( 'NONE',  ( -22.40478740399063895, 0.000000000000000000, 5.384712028983816623 ) ) ;
#40080=CARTESIAN_POINT ( 'NONE',  ( -26.13337879274045505, 0.000000000000000000, 6.833023547870798353 ) ) ;
#40081=CARTESIAN_POINT ( 'NONE',  ( -15.60102546347950536, 0.000000000000000000, 12.95077420755565356 ) ) ;
#40082=DIRECTION ( 'NONE',  ( 0.9999697198139515519, 0.000000000000000000, 0.007781995580013368816 ) ) ;
#40083=EDGE_CURVE ( 'NONE', #10299, #530, #15054, .T. ) ;
#40084=ADVANCED_FACE ( 'NONE', ( #7341 ), #33215, .F. ) ;
#40085=LINE ( 'NONE', #41208, #1361 ) ;
#40086=AXIS2_PLACEMENT_3D ( 'NONE', #25930, #34173, #43256 ) ;
#40087=ORIENTED_EDGE ( 'NONE', *, *, #29960, .F. ) ;
#40089=LINE ( 'NONE', #20477, #54881 ) ;
#40090=EDGE_CURVE ( 'NONE', #10456, #25250, #42284, .T. ) ;
#40091=PLANE ( 'NONE',  #51390 ) ;
#40092=ORIENTED_EDGE ( 'NONE', *, *, #46429, .F. ) ;
#40093=PLANE ( 'NONE',  #9364 ) ;
#40094=CARTESIAN_POINT ( 'NONE',  ( -17.43575422274359710, -4.727446477803164626, 3.503129884459415422 ) ) ;
#40095=VERTEX_POINT ( 'NONE', #3645 ) ;
#40096=CARTESIAN_POINT ( 'NONE',  ( -17.46532115785441519, 0.000000000000000000, 13.67492996699914265 ) ) ;
#40097=EDGE_CURVE ( 'NONE', #41167, #44596, #24656, .T. ) ;
#40098=PLANE ( 'NONE',  #55646 ) ;
#40099=CARTESIAN_POINT ( 'NONE',  ( -16.03018954091655601, 0.000000000000000000, 8.388977181989714538 ) ) ;
#40100=EDGE_CURVE ( 'NONE', #20518, #36569, #29507, .T. ) ;
#40101=CARTESIAN_POINT ( 'NONE',  ( -18.76964031537362487, -1.327505506330657781, 4.129732459434496405 ) ) ;
#40102=VERTEX_POINT ( 'NONE', #47363 ) ;
#40103=ORIENTED_EDGE ( 'NONE', *, *, #26257, .F. ) ;
#40104=FACE_OUTER_BOUND ( 'NONE', #51936, .T. ) ;
#40105=CARTESIAN_POINT ( 'NONE',  ( -27.99767448711536133, 0.000000000000000000, 7.557179307314289218 ) ) ;
#40106=LINE ( 'NONE', #917, #8768 ) ;
#40107=PLANE ( 'NONE',  #12095 ) ;
#40108=LINE ( 'NONE', #27622, #21959 ) ;
#40109=PLANE ( 'NONE',  #33079 ) ;
#40110=VECTOR ( 'NONE', #6125, 1000.000000000000114 ) ;
#40111=VERTEX_POINT ( 'NONE', #24389 ) ;
#40112=CARTESIAN_POINT ( 'NONE',  ( -16.92784874604061329, 0.000000000000000000, 4.319338622618287715 ) ) ;
#40113=DIRECTION ( 'NONE',  ( -0.005002170337468016433, -0.7660444431189770143, 0.6427681459581293666 ) ) ;
#40114=ORIENTED_EDGE ( 'NONE', *, *, #48779, .F. ) ;
#40115=CARTESIAN_POINT ( 'NONE',  ( -17.74560456716937296, 0.000000000000000000, 3.774316574337878372 ) ) ;
#40116=AXIS2_PLACEMENT_3D ( 'NONE', #54355, #36780, #36220 ) ;
#40117=CARTESIAN_POINT ( 'NONE',  ( -18.66354898467281132, 0.000000000000000000, 14.21960318569776582 ) ) ;
#40118=CARTESIAN_POINT ( 'NONE',  ( -25.20278734466900517, 0.000000000000000000, 6.670939612111840944 ) ) ;
#40120=VECTOR ( 'NONE', #2784, 1000.000000000000114 ) ;
#40121=VECTOR ( 'NONE', #39168, 1000.000000000000114 ) ;
#40122=DIRECTION ( 'NONE',  ( -0.9999697198139514409, -0.000000000000000000, -0.007781995580013368816 ) ) ;
#40123=ORIENTED_EDGE ( 'NONE', *, *, #849, .F. ) ;
#40124=ORIENTED_EDGE ( 'NONE', *, *, #213, .F. ) ;
#40125=VECTOR ( 'NONE', #41908, 999.9999999999998863 ) ;
#40127=VECTOR ( 'NONE', #19493, 1000.000000000000227 ) ;
#40128=EDGE_LOOP ( 'NONE', ( #13732, #30107, #13408, #20211, #27599 ) ) ;
#40129=DIRECTION ( 'NONE',  ( -0.005002170337468016433, -0.7660444431189770143, 0.6427681459581293666 ) ) ;
#40130=ORIENTED_EDGE ( 'NONE', *, *, #18158, .T. ) ;
#40131=LINE ( 'NONE', #26805, #43082 ) ;
#40132=PLANE ( 'NONE',  #31333 ) ;
#40133=EDGE_CURVE ( 'NONE', #52910, #55300, #20110, .T. ) ;
#40134=ORIENTED_EDGE ( 'NONE', *, *, #1140, .T. ) ;
#40135=DIRECTION ( 'NONE',  ( 0.7660212471507180654, -0.6427876096865404731, 0.005961354470445141482 ) ) ;
#40136=ORIENTED_EDGE ( 'NONE', *, *, #4275, .F. ) ;
#40137=PLANE ( 'NONE',  #11374 ) ;
#40139=VERTEX_POINT ( 'NONE', #46827 ) ;
#40140=EDGE_CURVE ( 'NONE', #5645, #5914, #28942, .T. ) ;
#40141=ADVANCED_FACE ( 'NONE', ( #41977 ), #37442, .F. ) ;
#40142=CARTESIAN_POINT ( 'NONE',  ( -13.08330893211609869, 0.000000000000000000, 1.763933231766363630 ) ) ;
#40143=LINE ( 'NONE', #23400, #2111 ) ;
#40144=LINE ( 'NONE', #14034, #45000 ) ;
#40145=CARTESIAN_POINT ( 'NONE',  ( -16.25746979822617178, 0.000000000000000000, 3.585891526986769051 ) ) ;
#40146=LINE ( 'NONE', #30540, #40516 ) ;
#40147=CARTESIAN_POINT ( 'NONE',  ( -27.06552663992790997, 0.000000000000000000, 7.195101427592543786 ) ) ;
#40148=ORIENTED_EDGE ( 'NONE', *, *, #19223, .F. ) ;
#40149=ORIENTED_EDGE ( 'NONE', *, *, #35008, .F. ) ;
#40150=DIRECTION ( 'NONE',  ( 0.007781995580012663651, 0.000000000000000000, -0.9999697198139515519 ) ) ;
#40151=CARTESIAN_POINT ( 'NONE',  ( -12.80458192191714595, 0.000000000000000000, 11.86454056839041726 ) ) ;
#40152=VECTOR ( 'NONE', #6315, 1000.000000000000114 ) ;
#40154=CARTESIAN_POINT ( 'NONE',  ( -15.03495456790438389, -0.1191753592594197858, 12.77051346725278158 ) ) ;
#40155=ORIENTED_EDGE ( 'NONE', *, *, #53531, .F. ) ;
#40156=LINE ( 'NONE', #48964, #3154 ) ;
#40157=FACE_OUTER_BOUND ( 'NONE', #20422, .T. ) ;
#40158=ORIENTED_EDGE ( 'NONE', *, *, #5733, .F. ) ;
#40159=VECTOR ( 'NONE', #23569, 1000.000000000000114 ) ;
#40161=DIRECTION ( 'NONE',  ( -0.5449076811759708816, 0.6444004775717707689, 0.5364919789714475140 ) ) ;
#40162=ORIENTED_EDGE ( 'NONE', *, *, #24753, .F. ) ;
#40163=VECTOR ( 'NONE', #19260, 1000.000000000000227 ) ;
#40164=AXIS2_PLACEMENT_3D ( 'NONE', #30872, #35418, #40236 ) ;
#40165=LINE ( 'NONE', #14606, #7103 ) ;
#40166=LINE ( 'NONE', #1258, #54156 ) ;
#40167=FACE_OUTER_BOUND ( 'NONE', #21990, .T. ) ;
#40168=EDGE_CURVE ( 'NONE', #7643, #9219, #7632, .T. ) ;
#40169=PLANE ( 'NONE',  #45929 ) ;
#40170=DIRECTION ( 'NONE',  ( 0.7660212471507180654, -0.6427876096865404731, 0.005961354470445141482 ) ) ;
#40171=ORIENTED_EDGE ( 'NONE', *, *, #51796, .T. ) ;
#40172=VECTOR ( 'NONE', #49269, 999.9999999999998863 ) ;
#40173=VECTOR ( 'NONE', #38726, 1000.000000000000227 ) ;
#40174=EDGE_CURVE ( 'NONE', #13341, #13570, #17012, .T. ) ;
#40175=ORIENTED_EDGE ( 'NONE', *, *, #20859, .F. ) ;
#40176=DIRECTION ( 'NONE',  ( -0.5449076811759708816, 0.6444004775717707689, 0.5364919789714475140 ) ) ;
#40178=DIRECTION ( 'NONE',  ( 0.9999697198139515519, 0.000000000000000000, 0.007781995580013368816 ) ) ;
#40179=CARTESIAN_POINT ( 'NONE',  ( -11.67244013076689946, 0.000000000000000000, 11.50401908778467863 ) ) ;
#40180=EDGE_CURVE ( 'NONE', #33398, #54798, #42556, .T. ) ;
#40182=CARTESIAN_POINT ( 'NONE',  ( -13.33648223891196949, 0.000000000000000000, 1.961969034772858667 ) ) ;
#40183=ORIENTED_EDGE ( 'NONE', *, *, #6616, .F. ) ;
#40184=DIRECTION ( 'NONE',  ( -0.6427681459581293666, -0.7660444431189770143, -0.005002170337467561935 ) ) ;
#40185=VECTOR ( 'NONE', #15222, 999.9999999999998863 ) ;
#40186=CARTESIAN_POINT ( 'NONE',  ( -15.81163362153278129, 0.000000000000000000, 6.005359602264157104 ) ) ;
#40187=LINE ( 'NONE', #47597, #54992 ) ;
#40188=DIRECTION ( 'NONE',  ( 0.9999697198139515519, 0.000000000000000000, 0.007781995580013368816 ) ) ;
#40189=ORIENTED_EDGE ( 'NONE', *, *, #29248, .T. ) ;
#40190=CARTESIAN_POINT ( 'NONE',  ( -18.68049516737052329, 3.200641362704010007, 3.835953230116354362 ) ) ;
#40192=CARTESIAN_POINT ( 'NONE',  ( -22.40634380310664397, 0.000000000000000000, 5.584705972946605534 ) ) ;
#40193=VECTOR ( 'NONE', #50625, 1000.000000000000227 ) ;
#40194=DIRECTION ( 'NONE',  ( 0.005961354470445682716, -0.6427876096865404731, -0.7660212471507180654 ) ) ;
#40195=EDGE_LOOP ( 'NONE', ( #14171, #14494, #30068, #26210 ) ) ;
#40196=FACE_OUTER_BOUND ( 'NONE', #4901, .T. ) ;
#40197=VECTOR ( 'NONE', #13995, 999.9999999999998863 ) ;
#40198=VERTEX_POINT ( 'NONE', #37752 ) ;
#40199=ORIENTED_EDGE ( 'NONE', *, *, #47261, .T. ) ;
#40200=ORIENTED_EDGE ( 'NONE', *, *, #41551, .T. ) ;
#40201=DIRECTION ( 'NONE',  ( -0.005961354470445682716, -0.6427876096865404731, 0.7660212471507180654 ) ) ;
#40202=ORIENTED_EDGE ( 'NONE', *, *, #15372, .F. ) ;
#40203=ORIENTED_EDGE ( 'NONE', *, *, #36806, .F. ) ;
#40204=VECTOR ( 'NONE', #23092, 999.9999999999998863 ) ;
#40206=ADVANCED_FACE ( 'NONE', ( #47093 ), #16157, .F. ) ;
#40207=LINE ( 'NONE', #18638, #44864 ) ;
#40208=ORIENTED_EDGE ( 'NONE', *, *, #37234, .T. ) ;
#40209=AXIS2_PLACEMENT_3D ( 'NONE', #3748, #12296, #51479 ) ;
#40210=AXIS2_PLACEMENT_3D ( 'NONE', #21735, #33654, #34790 ) ;
#40211=EDGE_CURVE ( 'NONE', #485, #51780, #34046, .T. ) ;
#40212=VERTEX_POINT ( 'NONE', #55910 ) ;
#40213=CARTESIAN_POINT ( 'NONE',  ( -19.47419960943008732, -2.577107522633557135, 7.507661911811399413 ) ) ;
#40214=VERTEX_POINT ( 'NONE', #50783 ) ;
#40215=ORIENTED_EDGE ( 'NONE', *, *, #54259, .T. ) ;
#40216=ADVANCED_FACE ( 'NONE', ( #11876 ), #55325, .F. ) ;
#40218=VECTOR ( 'NONE', #46607, 1000.000000000000114 ) ;
#40219=VECTOR ( 'NONE', #9884, 1000.000000000000000 ) ;
#40220=LINE ( 'NONE', #23195, #17487 ) ;
#40221=PLANE ( 'NONE',  #14002 ) ;
#40222=LINE ( 'NONE', #18653, #37745 ) ;
#40223=LINE ( 'NONE', #18348, #39535 ) ;
#40224=ORIENTED_EDGE ( 'NONE', *, *, #41453, .F. ) ;
#40225=LINE ( 'NONE', #45065, #2015 ) ;
#40226=ORIENTED_EDGE ( 'NONE', *, *, #7305, .F. ) ;
#40227=FACE_OUTER_BOUND ( 'NONE', #25762, .T. ) ;
#40228=EDGE_CURVE ( 'NONE', #49004, #33246, #19279, .T. ) ;
#40230=CARTESIAN_POINT ( 'NONE',  ( -14.66887761629205222, 0.000000000000000000, 12.58869632783390990 ) ) ;
#40231=LINE ( 'NONE', #17528, #20366 ) ;
#40232=VECTOR ( 'NONE', #17164, 1000.000000000000227 ) ;
#40233=DIRECTION ( 'NONE',  ( 0.5364919789714477361, 0.6444004775717706579, 0.5449076811759711036 ) ) ;
#40234=DIRECTION ( 'NONE',  ( 0.6246952433987894571, -0.7422098413412800966, -0.2426528472758541777 ) ) ;
#40235=ORIENTED_EDGE ( 'NONE', *, *, #43536, .T. ) ;
#40236=DIRECTION ( 'NONE',  ( -0.6427681459581293666, -0.7660444431189770143, -0.005002170337467561935 ) ) ;
#40237=VECTOR ( 'NONE', #35757, 999.9999999999998863 ) ;
#40238=VERTEX_POINT ( 'NONE', #12168 ) ;
#40239=DIRECTION ( 'NONE',  ( -0.3620778797217457656, 0.000000000000000000, -0.9321478471874539151 ) ) ;
#40240=DIRECTION ( 'NONE',  ( -0.005002170337468016433, -0.7660444431189770143, 0.6427681459581293666 ) ) ;
#40241=FACE_OUTER_BOUND ( 'NONE', #22060, .T. ) ;
#40242=AXIS2_PLACEMENT_3D ( 'NONE', #53318, #36265, #39948 ) ;
#40243=FACE_OUTER_BOUND ( 'NONE', #19977, .T. ) ;
#40244=DIRECTION ( 'NONE',  ( 0.000000000000000000, -0.000000000000000000, -1.000000000000000000 ) ) ;
#40246=ORIENTED_EDGE ( 'NONE', *, *, #23665, .F. ) ;
#40247=VECTOR ( 'NONE', #22736, 999.9999999999998863 ) ;
#40248=DIRECTION ( 'NONE',  ( 0.000000000000000000, -0.000000000000000000, -1.000000000000000000 ) ) ;
#40249=CARTESIAN_POINT ( 'NONE',  ( -13.08486533123210194, 0.000000000000000000, 1.963927175729152541 ) ) ;
#40250=DIRECTION ( 'NONE',  ( 0.9999697198139515519, 0.000000000000000000, 0.007781995580013368816 ) ) ;
#40251=VECTOR ( 'NONE', #19889, 1000.000000000000227 ) ;
#40252=CARTESIAN_POINT ( 'NONE',  ( -22.40634380310664397, 0.000000000000000000, 5.584705972946605534 ) ) ;
#40253=EDGE_CURVE ( 'NONE', #10480, #15058, #13846, .T. ) ;
#40254=PLANE ( 'NONE',  #35758 ) ;
#40255=LINE ( 'NONE', #1344, #39537 ) ;
#40256=CARTESIAN_POINT ( 'NONE',  ( -20.67116051404115140, -4.079838673713159558, 11.40702279338511538 ) ) ;
#40257=AXIS2_PLACEMENT_3D ( 'NONE', #25820, #13796, #7652 ) ;
#40258=VECTOR ( 'NONE', #34262, 1000.000000000000114 ) ;
#40260=DIRECTION ( 'NONE',  ( -0.9999697198139514409, -0.000000000000000000, -0.007781995580013368816 ) ) ;
#40261=ADVANCED_FACE ( 'NONE', ( #43950 ), #35726, .F. ) ;
#40262=ORIENTED_EDGE ( 'NONE', *, *, #5016, .T. ) ;
#40263=EDGE_CURVE ( 'NONE', #30962, #3478, #22098, .T. ) ;
#40264=EDGE_CURVE ( 'NONE', #43270, #31194, #13020, .T. ) ;
#40265=ORIENTED_EDGE ( 'NONE', *, *, #3592, .F. ) ;
#40266=ORIENTED_EDGE ( 'NONE', *, *, #42450, .T. ) ;
#40267=VERTEX_POINT ( 'NONE', #22402 ) ;
#40268=AXIS2_PLACEMENT_3D ( 'NONE', #17644, #39519, #44042 ) ;
#40269=VERTEX_POINT ( 'NONE', #30643 ) ;
#40270=DIRECTION ( 'NONE',  ( -0.005002170337468016433, -0.7660444431189770143, 0.6427681459581293666 ) ) ;
#40271=EDGE_CURVE ( 'NONE', #23289, #4032, #35187, .T. ) ;
#40272=LINE ( 'NONE', #15276, #25821 ) ;
#40273=VECTOR ( 'NONE', #24023, 1000.000000000000000 ) ;
#40274=ORIENTED_EDGE ( 'NONE', *, *, #54597, .F. ) ;
#40275=EDGE_CURVE ( 'NONE', #19751, #7777, #793, .T. ) ;
#40276=EDGE_LOOP ( 'NONE', ( #29874, #50213, #15004, #2564 ) ) ;
#40277=ORIENTED_EDGE ( 'NONE', *, *, #5613, .F. ) ;
#40278=VECTOR ( 'NONE', #37081, 999.9999999999998863 ) ;
#40279=ADVANCED_FACE ( 'NONE', ( #13578 ), #21813, .F. ) ;
#40280=CARTESIAN_POINT ( 'NONE',  ( -14.20280369269832832, 0.000000000000000000, 12.40765738797303719 ) ) ;
#40282=CARTESIAN_POINT ( 'NONE',  ( -12.06998961964583650, 0.000000000000000000, 2.879815326383328156 ) ) ;
#40283=DIRECTION ( 'NONE',  ( -0.6427681459581293666, -0.7660444431189770143, -0.005002170337467561935 ) ) ;
#40284=EDGE_LOOP ( 'NONE', ( #6233, #46759, #26178, #44731 ) ) ;
#40285=CARTESIAN_POINT ( 'NONE',  ( -10.00813838035478298, 0.000000000000000000, 10.77830692922518452 ) ) ;
#40286=VECTOR ( 'NONE', #21224, 999.9999999999998863 ) ;
#40287=EDGE_CURVE ( 'NONE', #53425, #31213, #31483, .T. ) ;
#40288=ORIENTED_EDGE ( 'NONE', *, *, #36066, .T. ) ;
#40289=CARTESIAN_POINT ( 'NONE',  ( -10.74029228357944987, 0.000000000000000000, 11.14194120806293320 ) ) ;
#40290=PLANE ( 'NONE',  #32974 ) ;
#40291=EDGE_CURVE ( 'NONE', #44163, #40865, #8477, .T. ) ;
#40292=VECTOR ( 'NONE', #41636, 1000.000000000000114 ) ;
#40293=DIRECTION ( 'NONE',  ( -0.3620778797217457656, 0.000000000000000000, -0.9321478471874539151 ) ) ;
#40294=CARTESIAN_POINT ( 'NONE',  ( -16.99924723426068951, 0.000000000000000000, 13.49389102713827171 ) ) ;
#40295=AXIS2_PLACEMENT_3D ( 'NONE', #48915, #43798, #27321 ) ;
#40296=DIRECTION ( 'NONE',  ( 0.9999697198139515519, 0.000000000000000000, 0.007781995580013368816 ) ) ;
#40297=DIRECTION ( 'NONE',  ( 0.5364919789714477361, 0.6444004775717706579, 0.5449076811759711036 ) ) ;
#40298=DIRECTION ( 'NONE',  ( 0.007781995580012662783, 0.000000000000000000, -0.9999697198139514409 ) ) ;
#40299=ORIENTED_EDGE ( 'NONE', *, *, #42453, .T. ) ;
#40300=CARTESIAN_POINT ( 'NONE',  ( -10.00813838035478298, 0.000000000000000000, 10.77830692922518452 ) ) ;
#40301=VERTEX_POINT ( 'NONE', #39427 ) ;
#40302=DIRECTION ( 'NONE',  ( 0.005002170337468016433, -0.7660444431189770143, -0.6427681459581293666 ) ) ;
#40303=CARTESIAN_POINT ( 'NONE',  ( -19.59569683186026268, 0.000000000000000000, 14.58168106541950948 ) ) ;
#40304=DIRECTION ( 'NONE',  ( 0.007781995580012663651, -3.146120232559066537E-19, -0.9999697198139514409 ) ) ;
#40305=DIRECTION ( 'NONE',  ( 0.000000000000000000, -0.000000000000000000, -1.000000000000000000 ) ) ;
#40306=PLANE ( 'NONE',  #28649 ) ;
#40309=AXIS2_PLACEMENT_3D ( 'NONE', #53676, #14792, #38047 ) ;
#40310=DIRECTION ( 'NONE',  ( -0.7660212471507179544, -0.6427876096865405842, -0.005961354470445141482 ) ) ;
#40311=VECTOR ( 'NONE', #24161, 1000.000000000000227 ) ;
#40312=DIRECTION ( 'NONE',  ( 0.005961354470445682716, -0.6427876096865404731, -0.7660212471507180654 ) ) ;
#40313=ORIENTED_EDGE ( 'NONE', *, *, #44531, .T. ) ;
#40314=CARTESIAN_POINT ( 'NONE',  ( -20.54049170961573267, 0.000000000000000000, 4.660556269540326646 ) ) ;
#40315=LINE ( 'NONE', #13904, #28737 ) ;
#40317=AXIS2_PLACEMENT_3D ( 'NONE', #4820, #52521, #17601 ) ;
#40318=CARTESIAN_POINT ( 'NONE',  ( -13.20081375640679866, 0.000000000000000000, 3.071021047694093564 ) ) ;
#40319=CARTESIAN_POINT ( 'NONE',  ( -11.30636317915456779, -0.1191753592594197858, 11.32220194836580340 ) ) ;
#40321=FACE_OUTER_BOUND ( 'NONE', #2730, .T. ) ;
#40322=DIRECTION ( 'NONE',  ( 0.5449076811759707706, 0.6444004775717708799, -0.5364919789714476250 ) ) ;
#40323=ORIENTED_EDGE ( 'NONE', *, *, #51013, .F. ) ;
#40324=VECTOR ( 'NONE', #46155, 1000.000000000000227 ) ;
#40325=VERTEX_POINT ( 'NONE', #47668 ) ;
#40327=AXIS2_PLACEMENT_3D ( 'NONE', #42306, #29812, #3404 ) ;
#40328=LINE ( 'NONE', #5149, #509 ) ;
#40329=AXIS2_PLACEMENT_3D ( 'NONE', #53170, #48623, #1174 ) ;
#40330=EDGE_LOOP ( 'NONE', ( #37967, #30751, #21143, #20133 ) ) ;
#40331=CARTESIAN_POINT ( 'NONE',  ( -29.93654370153088706, 0.000000000000000000, 22.35628214185738116 ) ) ;
#40332=ORIENTED_EDGE ( 'NONE', *, *, #27794, .F. ) ;
#40333=LINE ( 'NONE', #49121, #18428 ) ;
#40334=ADVANCED_FACE ( 'NONE', ( #34587 ), #4241, .F. ) ;
#40335=AXIS2_PLACEMENT_3D ( 'NONE', #29070, #29673, #42135 ) ;
#40336=ORIENTED_EDGE ( 'NONE', *, *, #49587, .F. ) ;
#40337=VECTOR ( 'NONE', #51553, 1000.000000000000000 ) ;
#40338=ORIENTED_EDGE ( 'NONE', *, *, #37848, .F. ) ;
#40339=ORIENTED_EDGE ( 'NONE', *, *, #39615, .F. ) ;
#40340=CARTESIAN_POINT ( 'NONE',  ( -14.01701317841955508, 0.000000000000000000, 2.326005055450897085 ) ) ;
#40341=DIRECTION ( 'NONE',  ( -0.5449076811759708816, 0.6444004775717707689, 0.5364919789714475140 ) ) ;
#40342=CARTESIAN_POINT ( 'NONE',  ( -16.74378146872023976, 0.000000000000000000, 6.367437481985902537 ) ) ;
#40343=FACE_OUTER_BOUND ( 'NONE', #12061, .T. ) ;
#40344=EDGE_CURVE ( 'NONE', #2394, #31162, #43661, .T. ) ;
#40345=ORIENTED_EDGE ( 'NONE', *, *, #18135, .T. ) ;
#40346=ORIENTED_EDGE ( 'NONE', *, *, #24436, .F. ) ;
#40347=EDGE_CURVE ( 'NONE', #14766, #5010, #30888, .T. ) ;
#40348=VECTOR ( 'NONE', #55902, 999.9999999999998863 ) ;
#40350=AXIS2_PLACEMENT_3D ( 'NONE', #16968, #16664, #8739 ) ;
#40351=ORIENTED_EDGE ( 'NONE', *, *, #25722, .T. ) ;
#40352=EDGE_CURVE ( 'NONE', #38297, #31963, #9308, .T. ) ;
#40353=DIRECTION ( 'NONE',  ( 0.9999697198139515519, 0.000000000000000000, 0.007781995580013368816 ) ) ;
#40354=ORIENTED_EDGE ( 'NONE', *, *, #20109, .T. ) ;
#40355=VECTOR ( 'NONE', #40996, 999.9999999999998863 ) ;
#40356=CARTESIAN_POINT ( 'NONE',  ( 2.072287782118878319, 0.000000000000000000, -2.950529333540147015 ) ) ;
#40357=LINE ( 'NONE', #17658, #26723 ) ;
#40358=EDGE_CURVE ( 'NONE', #23668, #54371, #26099, .T. ) ;
#40361=AXIS2_PLACEMENT_3D ( 'NONE', #7675, #38905, #34622 ) ;
#40362=VERTEX_POINT ( 'NONE', #38871 ) ;
#40363=EDGE_CURVE ( 'NONE', #45114, #8988, #44251, .T. ) ;
#40364=CARTESIAN_POINT ( 'NONE',  ( 2.072287782118878319, 0.000000000000000000, -2.950529333540147015 ) ) ;
#40365=AXIS2_PLACEMENT_3D ( 'NONE', #14861, #2619, #19941 ) ;
#40366=VECTOR ( 'NONE', #3761, 999.9999999999998863 ) ;
#40367=VERTEX_POINT ( 'NONE', #39970 ) ;
#40368=CARTESIAN_POINT ( 'NONE',  ( 2.072287782118878319, 0.000000000000000000, -2.950529333540147015 ) ) ;
#40369=CARTESIAN_POINT ( 'NONE',  ( -13.54170968098099159, -3.917936722690661178, 8.371993288704665304 ) ) ;
#40370=AXIS2_PLACEMENT_3D ( 'NONE', #28153, #10592, #27314 ) ;
#40371=LINE ( 'NONE', #1467, #5624 ) ;
#40372=ORIENTED_EDGE ( 'NONE', *, *, #20523, .F. ) ;
#40373=AXIS2_PLACEMENT_3D ( 'NONE', #18156, #5127, #5395 ) ;
#40374=DIRECTION ( 'NONE',  ( 0.007781995580012662783, 0.000000000000000000, -0.9999697198139514409 ) ) ;
#40375=DIRECTION ( 'NONE',  ( 0.6427681459581294776, -0.7660444431189769032, 0.005002170337467562802 ) ) ;
#40376=CARTESIAN_POINT ( 'NONE',  ( -18.67775241435682432, 0.000000000000000000, 4.136394454059623804 ) ) ;
#40377=CARTESIAN_POINT ( 'NONE',  ( -11.33651806203188883, 0.000000000000000000, 2.346865288250602255 ) ) ;
#40379=VECTOR ( 'NONE', #11415, 999.9999999999998863 ) ;
#40380=AXIS2_PLACEMENT_3D ( 'NONE', #29113, #11242, #55508 ) ;
#40382=VERTEX_POINT ( 'NONE', #56182 ) ;
#40383=CARTESIAN_POINT ( 'NONE',  ( -15.99150919095859713, 0.000000000000000000, 3.418635280343801153 ) ) ;
#40384=CARTESIAN_POINT ( 'NONE',  ( -14.60047255394062127, 0.000000000000000000, 3.798792718905593890 ) ) ;
#40386=ORIENTED_EDGE ( 'NONE', *, *, #2314, .F. ) ;
#40387=DIRECTION ( 'NONE',  ( 0.6427681459581294776, -0.7660444431189769032, 0.005002170337467562802 ) ) ;
#40388=CARTESIAN_POINT ( 'NONE',  ( -19.60834386242827776, 0.000000000000000000, 4.298478389818581213 ) ) ;
#40389=ORIENTED_EDGE ( 'NONE', *, *, #43794, .F. ) ;
#40390=EDGE_CURVE ( 'NONE', #3168, #50762, #17264, .T. ) ;
#40391=LINE ( 'NONE', #36981, #36771 ) ;
#40392=ADVANCED_FACE ( 'NONE', ( #40819 ), #18967, .F. ) ;
#40393=FACE_OUTER_BOUND ( 'NONE', #14239, .T. ) ;
#40394=DIRECTION ( 'NONE',  ( 0.007781995580012662783, 0.000000000000000000, -0.9999697198139514409 ) ) ;
#40395=VECTOR ( 'NONE', #15257, 999.9999999999998863 ) ;
#40397=ORIENTED_EDGE ( 'NONE', *, *, #4292, .T. ) ;
#40398=VECTOR ( 'NONE', #45312, 1000.000000000000227 ) ;
#40399=EDGE_CURVE ( 'NONE', #24834, #44124, #37114, .T. ) ;
#40400=DIRECTION ( 'NONE',  ( 0.6427681459581294776, -0.7660444431189769032, 0.005002170337467562802 ) ) ;
#40401=CARTESIAN_POINT ( 'NONE',  ( -14.40335266348311372, 0.000000000000000000, 4.169658821279362826 ) ) ;
#40402=VECTOR ( 'NONE', #49312, 999.9999999999998863 ) ;
#40403=ADVANCED_FACE ( 'NONE', ( #53585 ), #1891, .F. ) ;
#40404=EDGE_CURVE ( 'NONE', #38944, #27123, #41385, .T. ) ;
#40405=ADVANCED_FACE ( 'NONE', ( #10451 ), #2476, .F. ) ;
#40406=DIRECTION ( 'NONE',  ( -0.005002170337468016433, -0.7660444431189770143, 0.6427681459581293666 ) ) ;
#40407=CARTESIAN_POINT ( 'NONE',  ( -25.20123094555300369, 0.000000000000000000, 6.470945668149052032 ) ) ;
#40408=VERTEX_POINT ( 'NONE', #36552 ) ;
#40409=DIRECTION ( 'NONE',  ( -0.7660212471507179544, -0.6427876096865405842, -0.005961354470445141482 ) ) ;
#40410=VECTOR ( 'NONE', #5046, 1000.000000000000227 ) ;
#40411=VERTEX_POINT ( 'NONE', #53863 ) ;
#40412=DIRECTION ( 'NONE',  ( 0.9999697198139515519, 0.000000000000000000, 0.007781995580013368816 ) ) ;
#40413=DIRECTION ( 'NONE',  ( 0.6427681459581294776, -0.7660444431189769032, 0.005002170337467562802 ) ) ;
#40414=VECTOR ( 'NONE', #28771, 1000.000000000000114 ) ;
#40415=VECTOR ( 'NONE', #28466, 999.9999999999998863 ) ;
#40416=ORIENTED_EDGE ( 'NONE', *, *, #15574, .T. ) ;
#40417=FACE_OUTER_BOUND ( 'NONE', #9287, .T. ) ;
#40418=DIRECTION ( 'NONE',  ( -0.7660212471507179544, -0.6427876096865405842, -0.005961354470445141482 ) ) ;
#40419=CARTESIAN_POINT ( 'NONE',  ( -14.46888367232926420, 0.000000000000000000, 12.59025272694991315 ) ) ;
#40420=AXIS2_PLACEMENT_3D ( 'NONE', #19569, #33464, #36606 ) ;
#40421=ORIENTED_EDGE ( 'NONE', *, *, #55040, .T. ) ;
#40422=VECTOR ( 'NONE', #42923, 1000.000000000000227 ) ;
#40423=PLANE ( 'NONE',  #52060 ) ;
#40424=EDGE_CURVE ( 'NONE', #40269, #1575, #27776, .T. ) ;
#40425=AXIS2_PLACEMENT_3D ( 'NONE', #12167, #43128, #51901 ) ;
#40426=ORIENTED_EDGE ( 'NONE', *, *, #15289, .F. ) ;
#40427=VECTOR ( 'NONE', #55209, 999.9999999999998863 ) ;
#40428=EDGE_CURVE ( 'NONE', #52847, #27231, #23234, .T. ) ;
#40429=ORIENTED_EDGE ( 'NONE', *, *, #14936, .F. ) ;
#40430=VECTOR ( 'NONE', #17385, 999.9999999999998863 ) ;
#40431=ORIENTED_EDGE ( 'NONE', *, *, #10122, .F. ) ;
#40432=LINE ( 'NONE', #1523, #50469 ) ;
#40433=EDGE_CURVE ( 'NONE', #42084, #36986, #14434, .T. ) ;
#40434=ORIENTED_EDGE ( 'NONE', *, *, #9887, .F. ) ;
#40435=DIRECTION ( 'NONE',  ( 0.007781995580012662783, 0.000000000000000000, -0.9999697198139514409 ) ) ;
#40436=ORIENTED_EDGE ( 'NONE', *, *, #5333, .F. ) ;
#40437=CARTESIAN_POINT ( 'NONE',  ( -19.06121784591510249, 0.000000000000000000, 5.610738516630323858 ) ) ;
#40438=DIRECTION ( 'NONE',  ( 0.000000000000000000, -0.000000000000000000, -1.000000000000000000 ) ) ;
#40439=ADVANCED_FACE ( 'NONE', ( #1639 ), #40563, .F. ) ;
#40440=ORIENTED_EDGE ( 'NONE', *, *, #11248, .F. ) ;
#40441=CARTESIAN_POINT ( 'NONE',  ( -18.67619601524082285, 0.000000000000000000, 3.936400510096834893 ) ) ;
#40442=ORIENTED_EDGE ( 'NONE', *, *, #14006, .T. ) ;
#40443=EDGE_CURVE ( 'NONE', #5277, #46034, #49336, .T. ) ;
#40445=PLANE ( 'NONE',  #25543 ) ;
#40446=DIRECTION ( 'NONE',  ( 0.7660212471507180654, -0.6427876096865404731, 0.005961354470445141482 ) ) ;
#40447=VECTOR ( 'NONE', #31246, 999.9999999999998863 ) ;
#40449=LINE ( 'NONE', #10639, #55642 ) ;
#40450=LINE ( 'NONE', #1538, #46822 ) ;
#40451=FACE_OUTER_BOUND ( 'NONE', #31580, .T. ) ;
#40452=CARTESIAN_POINT ( 'NONE',  ( -10.27421835998572064, 0.000000000000000000, 10.96090226820206048 ) ) ;
#40453=AXIS2_PLACEMENT_3D ( 'NONE', #46418, #21466, #34250 ) ;
#40454=ORIENTED_EDGE ( 'NONE', *, *, #17647, .F. ) ;
#40455=ORIENTED_EDGE ( 'NONE', *, *, #5607, .F. ) ;
#40456=LINE ( 'NONE', #54060, #40975 ) ;
#40457=DIRECTION ( 'NONE',  ( 0.007781995580012662783, 0.000000000000000000, -0.9999697198139514409 ) ) ;
#40458=VECTOR ( 'NONE', #25016, 1000.000000000000227 ) ;
#40459=DIRECTION ( 'NONE',  ( -0.5449076811759708816, 0.6444004775717707689, 0.5364919789714475140 ) ) ;
#40460=VECTOR ( 'NONE', #8526, 1000.000000000000227 ) ;
#40461=VECTOR ( 'NONE', #24487, 1000.000000000000227 ) ;
#40463=ORIENTED_EDGE ( 'NONE', *, *, #11909, .F. ) ;
#40464=PLANE ( 'NONE',  #10443 ) ;
#40465=DIRECTION ( 'NONE',  ( 0.007781995580012662783, 0.000000000000000000, -0.9999697198139514409 ) ) ;
#40466=ORIENTED_EDGE ( 'NONE', *, *, #35426, .T. ) ;
#40467=PLANE ( 'NONE',  #5760 ) ;
#40468=PLANE ( 'NONE',  #4081 ) ;
#40469=ORIENTED_EDGE ( 'NONE', *, *, #54420, .T. ) ;
#40470=VECTOR ( 'NONE', #48973, 1000.000000000000000 ) ;
#40472=DIRECTION ( 'NONE',  ( -0.9999697198139514409, -0.000000000000000000, -0.007781995580013368816 ) ) ;
#40473=AXIS2_PLACEMENT_3D ( 'NONE', #22896, #1609, #18934 ) ;
#40474=FACE_OUTER_BOUND ( 'NONE', #18884, .T. ) ;
#40475=CARTESIAN_POINT ( 'NONE',  ( -26.13337879274045505, 0.000000000000000000, 6.833023547870798353 ) ) ;
#40476=VECTOR ( 'NONE', #45768, 999.9999999999998863 ) ;
#40477=DIRECTION ( 'NONE',  ( 0.5449076811759707706, 0.6444004775717708799, -0.5364919789714476250 ) ) ;
#40479=VECTOR ( 'NONE', #53573, 999.9999999999998863 ) ;
#40480=VERTEX_POINT ( 'NONE', #44502 ) ;
#40481=CARTESIAN_POINT ( 'NONE',  ( -10.30646909681032142, -0.1191753592594186895, 2.254878339363226569 ) ) ;
#40482=DIRECTION ( 'NONE',  ( -0.005961354470445682716, -0.6427876096865404731, 0.7660212471507180654 ) ) ;
#40483=LINE ( 'NONE', #6387, #46931 ) ;
#40484=ADVANCED_FACE ( 'NONE', ( #54165 ), #6458, .F. ) ;
#40485=EDGE_CURVE ( 'NONE', #17974, #38400, #32316, .T. ) ;
#40487=CARTESIAN_POINT ( 'NONE',  ( -36.91819796696599099, -1.000000000000000000, 21.84982018086542155 ) ) ;
#40488=EDGE_LOOP ( 'NONE', ( #6471, #46993, #16714, #38518 ) ) ;
#40490=CARTESIAN_POINT ( 'NONE',  ( -10.84028925556084388, -0.1191753592594197858, 11.14116300850493246 ) ) ;
#40491=FACE_OUTER_BOUND ( 'NONE', #14299, .T. ) ;
#40492=AXIS2_PLACEMENT_3D ( 'NONE', #40624, #27002, #19023 ) ;
#40493=DIRECTION ( 'NONE',  ( -0.7660212471507179544, -0.6427876096865405842, -0.005961354470445141482 ) ) ;
#40494=CARTESIAN_POINT ( 'NONE',  ( -22.40634380310664397, 0.000000000000000000, 5.584705972946605534 ) ) ;
#40495=ORIENTED_EDGE ( 'NONE', *, *, #31578, .T. ) ;
#40496=FACE_OUTER_BOUND ( 'NONE', #46309, .T. ) ;
#40497=ORIENTED_EDGE ( 'NONE', *, *, #34926, .T. ) ;
#40498=CARTESIAN_POINT ( 'NONE',  ( -11.82259098779923256, 0.000000000000000000, 5.097733058581920496 ) ) ;
#40499=VECTOR ( 'NONE', #33529, 1000.000000000000114 ) ;
#40500=DIRECTION ( 'NONE',  ( 0.5449076811759707706, 0.6444004775717708799, -0.5364919789714476250 ) ) ;
#40501=ORIENTED_EDGE ( 'NONE', *, *, #5913, .T. ) ;
#40502=CARTESIAN_POINT ( 'NONE',  ( -15.08941953321324725, 0.000000000000000000, 6.918970192494675153 ) ) ;
#40503=VECTOR ( 'NONE', #48497, 999.9999999999998863 ) ;
#40504=ORIENTED_EDGE ( 'NONE', *, *, #16165, .T. ) ;
#40505=EDGE_CURVE ( 'NONE', #53467, #27029, #10152, .T. ) ;
#40507=AXIS2_PLACEMENT_3D ( 'NONE', #17538, #13563, #30874 ) ;
#40508=ORIENTED_EDGE ( 'NONE', *, *, #22760, .F. ) ;
#40509=CARTESIAN_POINT ( 'NONE',  ( -12.13851405436063047, 0.000000000000000000, 11.68505802764555135 ) ) ;
#40510=ORIENTED_EDGE ( 'NONE', *, *, #19449, .T. ) ;
#40513=DIRECTION ( 'NONE',  ( -0.5364919789714478471, 0.6444004775717705469, -0.5449076811759709926 ) ) ;
#40514=ORIENTED_EDGE ( 'NONE', *, *, #36396, .F. ) ;
#40515=EDGE_CURVE ( 'NONE', #291, #10918, #2176, .T. ) ;
#40516=VECTOR ( 'NONE', #47848, 1000.000000000000114 ) ;
#40517=VERTEX_POINT ( 'NONE', #19509 ) ;
#40518=DIRECTION ( 'NONE',  ( -0.5364919789714478471, 0.6444004775717705469, -0.5449076811759709926 ) ) ;
#40520=EDGE_LOOP ( 'NONE', ( #3258, #49202, #37613, #3879 ) ) ;
#40521=EDGE_CURVE ( 'NONE', #19083, #24779, #32577, .T. ) ;
#40522=VECTOR ( 'NONE', #50737, 999.9999999999998863 ) ;
#40523=VECTOR ( 'NONE', #36765, 999.9999999999998863 ) ;
#40524=PLANE ( 'NONE',  #37552 ) ;
#40525=EDGE_CURVE ( 'NONE', #41560, #12666, #2721, .T. ) ;
#40526=LINE ( 'NONE', #35998, #27580 ) ;
#40527=CARTESIAN_POINT ( 'NONE',  ( -26.13493519185646008, 0.000000000000000000, 7.033017491833586377 ) ) ;
#40528=PLANE ( 'NONE',  #40473 ) ;
#40529=EDGE_CURVE ( 'NONE', #52907, #9714, #24890, .T. ) ;
#40530=ORIENTED_EDGE ( 'NONE', *, *, #31402, .F. ) ;
#40531=CARTESIAN_POINT ( 'NONE',  ( -20.53653072179030659, -0.1046794588179832119, 4.772753996012100153 ) ) ;
#40532=EDGE_LOOP ( 'NONE', ( #3096, #4168, #34903, #44837 ) ) ;
#40533=EDGE_CURVE ( 'NONE', #25397, #38228, #50987, .T. ) ;
#40534=CARTESIAN_POINT ( 'NONE',  ( -27.99845268667336384, -0.1191753592594197858, 7.657176279295684118 ) ) ;
#40535=VECTOR ( 'NONE', #12565, 999.9999999999998863 ) ;
#40536=LINE ( 'NONE', #48768, #15214 ) ;
#40537=LINE ( 'NONE', #33032, #52155 ) ;
#40538=CARTESIAN_POINT ( 'NONE',  ( -12.70458494993575194, -0.1191753592594197858, 11.86531876794841978 ) ) ;
#40539=DIRECTION ( 'NONE',  ( -0.9999697198139514409, -0.000000000000000000, -0.007781995580013368816 ) ) ;
#40540=DIRECTION ( 'NONE',  ( -0.9999697198139514409, -0.000000000000000000, -0.007781995580013368816 ) ) ;
#40541=EDGE_LOOP ( 'NONE', ( #34985, #7254, #3104, #46399 ) ) ;
#40542=DIRECTION ( 'NONE',  ( 0.6427681459581294776, -0.7660444431189769032, 0.005002170337467562802 ) ) ;
#40544=EDGE_LOOP ( 'NONE', ( #35335, #33742, #25169, #35832 ) ) ;
#40545=CARTESIAN_POINT ( 'NONE',  ( -22.40634380310664397, 0.000000000000000000, 5.584705972946605534 ) ) ;
#40546=DIRECTION ( 'NONE',  ( 0.005961354470445682716, -0.6427876096865404731, -0.7660212471507180654 ) ) ;
#40547=VECTOR ( 'NONE', #2941, 1000.000000000000227 ) ;
#40548=CARTESIAN_POINT ( 'NONE',  ( -15.41378572042718353, -3.432230869623161595, 2.759052810919471188 ) ) ;
#40549=CARTESIAN_POINT ( 'NONE',  ( -18.43979397367102280, -1.489407457353156827, 3.996443418800899927 ) ) ;
#40550=PLANE ( 'NONE',  #4198 ) ;
#40551=AXIS2_PLACEMENT_3D ( 'NONE', #8387, #56106, #38490 ) ;
#40552=CARTESIAN_POINT ( 'NONE',  ( -10.47421230394850866, 0.000000000000000000, 10.95934586908605723 ) ) ;
#40553=ORIENTED_EDGE ( 'NONE', *, *, #44150, .T. ) ;
#40554=CARTESIAN_POINT ( 'NONE',  ( 2.072287782118878319, 0.000000000000000000, -2.950529333540147015 ) ) ;
#40555=CARTESIAN_POINT ( 'NONE',  ( -18.67775241435682432, 0.000000000000000000, 4.136394454059623804 ) ) ;
#40556=DIRECTION ( 'NONE',  ( -0.5449076811759708816, 0.6444004775717707689, 0.5364919789714475140 ) ) ;
#40557=ADVANCED_FACE ( 'NONE', ( #7562 ), #25192, .F. ) ;
#40558=AXIS2_PLACEMENT_3D ( 'NONE', #5381, #53366, #1922 ) ;
#40559=DIRECTION ( 'NONE',  ( 0.005002170337468016433, -0.7660444431189770143, -0.6427681459581293666 ) ) ;
#40560=LINE ( 'NONE', #14693, #2178 ) ;
#40561=ADVANCED_FACE ( 'NONE', ( #12097 ), #29431, .F. ) ;
#40562=ADVANCED_FACE ( 'NONE', ( #7872 ), #12413, .F. ) ;
#40563=PLANE ( 'NONE',  #44653 ) ;
#40564=VECTOR ( 'NONE', #30415, 1000.000000000000227 ) ;
#40565=DIRECTION ( 'NONE',  ( 0.005002170337468016433, -0.7660444431189770143, -0.6427681459581293666 ) ) ;
#40566=DIRECTION ( 'NONE',  ( 0.000000000000000000, -0.000000000000000000, -1.000000000000000000 ) ) ;
#40567=VERTEX_POINT ( 'NONE', #20892 ) ;
#40568=VERTEX_POINT ( 'NONE', #28880 ) ;
#40569=ORIENTED_EDGE ( 'NONE', *, *, #55222, .F. ) ;
#40570=EDGE_LOOP ( 'NONE', ( #21064, #36246, #21136, #29386 ) ) ;
#40571=ORIENTED_EDGE ( 'NONE', *, *, #11511, .F. ) ;
#40572=CARTESIAN_POINT ( 'NONE',  ( -18.67697421479882181, -0.1191753592594197858, 4.036397482078229793 ) ) ;
#40573=LINE ( 'NONE', #31495, #28523 ) ;
#40575=ORIENTED_EDGE ( 'NONE', *, *, #26345, .T. ) ;
#40576=EDGE_LOOP ( 'NONE', ( #50798, #49452, #52072, #16047, #40833 ) ) ;
#40577=EDGE_LOOP ( 'NONE', ( #21274, #42980, #86, #24251 ) ) ;
#40578=EDGE_CURVE ( 'NONE', #40517, #13439, #28590, .T. ) ;
#40579=VECTOR ( 'NONE', #2399, 1000.000000000000000 ) ;
#40581=EDGE_CURVE ( 'NONE', #54113, #25817, #42210, .T. ) ;
#40582=FACE_OUTER_BOUND ( 'NONE', #54855, .T. ) ;
#40583=FACE_OUTER_BOUND ( 'NONE', #36315, .T. ) ;
#40584=VERTEX_POINT ( 'NONE', #20048 ) ;
#40585=DIRECTION ( 'NONE',  ( 0.007781995580012662783, 0.000000000000000000, -0.9999697198139514409 ) ) ;
#40586=ORIENTED_EDGE ( 'NONE', *, *, #41203, .F. ) ;
#40587=AXIS2_PLACEMENT_3D ( 'NONE', #7260, #2980, #14954 ) ;
#40588=DIRECTION ( 'NONE',  ( -0.6427681459581293666, -0.7660444431189770143, -0.005002170337467561935 ) ) ;
#40589=EDGE_CURVE ( 'NONE', #42375, #40584, #3319, .T. ) ;
#40590=CARTESIAN_POINT ( 'NONE',  ( -12.70458494993575194, -0.1191753592594197858, 11.86531876794841978 ) ) ;
#40591=CARTESIAN_POINT ( 'NONE',  ( -17.16329905896135699, -4.403642575758163424, 3.407630086004865611 ) ) ;
#40592=DIRECTION ( 'NONE',  ( 0.005961354470445682716, -0.6427876096865404731, -0.7660212471507180654 ) ) ;
#40594=CARTESIAN_POINT ( 'NONE',  ( -23.33693525117809386, 0.000000000000000000, 5.746789908705562944 ) ) ;
#40595=DIRECTION ( 'NONE',  ( 0.007781995580012663651, 0.000000000000000000, -0.9999697198139515519 ) ) ;
#40596=VERTEX_POINT ( 'NONE', #20338 ) ;
#40597=DIRECTION ( 'NONE',  ( 0.7660212471507180654, -0.6427876096865404731, 0.005961354470445141482 ) ) ;
#40598=ORIENTED_EDGE ( 'NONE', *, *, #16613, .F. ) ;
#40599=ADVANCED_FACE ( 'NONE', ( #24591 ), #41906, .F. ) ;
#40601=CARTESIAN_POINT ( 'NONE',  ( -18.67775241435682432, 0.000000000000000000, 4.136394454059623804 ) ) ;
#40602=DIRECTION ( 'NONE',  ( 0.7660212471507180654, -0.6427876096865404731, 0.005961354470445141482 ) ) ;
#40603=FACE_OUTER_BOUND ( 'NONE', #2182, .T. ) ;
#40604=DIRECTION ( 'NONE',  ( 0.5449076811759707706, 0.6444004775717708799, -0.5364919789714476250 ) ) ;
#40605=CARTESIAN_POINT ( 'NONE',  ( -27.99845268667336384, -0.1191753592594197858, 7.657176279295684118 ) ) ;
#40606=CARTESIAN_POINT ( 'NONE',  ( -21.47419595591918906, 0.000000000000000000, 5.222628093224860102 ) ) ;
#40607=DIRECTION ( 'NONE',  ( 0.6427681459581294776, -0.7660444431189769032, 0.005002170337467562802 ) ) ;
#40608=EDGE_CURVE ( 'NONE', #33095, #48957, #33419, .T. ) ;
#40609=PLANE ( 'NONE',  #4817 ) ;
#40610=DIRECTION ( 'NONE',  ( -0.005961354470445682716, -0.6427876096865404731, 0.7660212471507180654 ) ) ;
#40611=ORIENTED_EDGE ( 'NONE', *, *, #46878, .T. ) ;
#40612=CARTESIAN_POINT ( 'NONE',  ( -0.6946271361862269567, -5.340650597229416263, 3.488190344995370396 ) ) ;
#40613=PLANE ( 'NONE',  #24900 ) ;
#40614=EDGE_CURVE ( 'NONE', #29543, #17332, #42494, .T. ) ;
#40615=LINE ( 'NONE', #37744, #12785 ) ;
#40616=DIRECTION ( 'NONE',  ( 0.000000000000000000, -0.000000000000000000, -1.000000000000000000 ) ) ;
#40617=EDGE_CURVE ( 'NONE', #32117, #3254, #55261, .T. ) ;
#40618=CARTESIAN_POINT ( 'NONE',  ( -18.67619601524082285, 0.000000000000000000, 3.936400510096834893 ) ) ;
#40619=CARTESIAN_POINT ( 'NONE',  ( -30.79567442779373110, 0.000000000000000000, 8.843406890442315316 ) ) ;
#40620=ADVANCED_FACE ( 'NONE', ( #33677 ), #47035, .F. ) ;
#40621=LINE ( 'NONE', #1694, #2965 ) ;
#40622=ORIENTED_EDGE ( 'NONE', *, *, #54100, .T. ) ;
#40623=EDGE_LOOP ( 'NONE', ( #7289, #43906, #26278, #35404 ) ) ;
#40624=CARTESIAN_POINT ( 'NONE',  ( -15.60102546347950536, 0.000000000000000000, 12.95077420755565356 ) ) ;
#40625=CARTESIAN_POINT ( 'NONE',  ( -18.79370083953152459, 0.000000000000000000, 5.243488326024565715 ) ) ;
#40626=EDGE_CURVE ( 'NONE', #19288, #24739, #42751, .T. ) ;
#40627=VECTOR ( 'NONE', #2001, 1000.000000000000000 ) ;
#40628=ORIENTED_EDGE ( 'NONE', *, *, #51808, .T. ) ;
#40629=CARTESIAN_POINT ( 'NONE',  ( -11.60247866929946525, 0.000000000000000000, 2.514121534893573262 ) ) ;
#40631=PLANE ( 'NONE',  #30195 ) ;
#40632=ADVANCED_FACE ( 'NONE', ( #37373 ), #11264, .F. ) ;
#40633=EDGE_LOOP ( 'NONE', ( #1522, #1216, #28243, #42376, #10627 ) ) ;
#40634=ORIENTED_EDGE ( 'NONE', *, *, #5916, .T. ) ;
#40635=ORIENTED_EDGE ( 'NONE', *, *, #22062, .T. ) ;
#40636=DIRECTION ( 'NONE',  ( 0.007781995580012663651, -3.146120232559066537E-19, -0.9999697198139514409 ) ) ;
#40637=DIRECTION ( 'NONE',  ( -0.5364919789714478471, 0.6444004775717705469, -0.5449076811759709926 ) ) ;
#40638=DIRECTION ( 'NONE',  ( -0.6427681459581293666, -0.7660444431189770143, -0.005002170337467561935 ) ) ;
#40639=DIRECTION ( 'NONE',  ( -0.005002170337468016433, -0.7660444431189770143, 0.6427681459581293666 ) ) ;
#40640=VERTEX_POINT ( 'NONE', #8712 ) ;
#40641=ORIENTED_EDGE ( 'NONE', *, *, #25440, .F. ) ;
#40642=DIRECTION ( 'NONE',  ( 0.5449076811759707706, 0.6444004775717708799, -0.5364919789714476250 ) ) ;
#40643=ORIENTED_EDGE ( 'NONE', *, *, #25404, .F. ) ;
#40644=CARTESIAN_POINT ( 'NONE',  ( -8.782761204222188312, 0.000000000000000000, 4.382725577236319836 ) ) ;
#40645=VERTEX_POINT ( 'NONE', #31103 ) ;
#40646=PLANE ( 'NONE',  #13111 ) ;
#40647=CARTESIAN_POINT ( 'NONE',  ( -23.33771345073609638, -0.1191753592594197858, 5.846786880686956955 ) ) ;
#40648=VERTEX_POINT ( 'NONE', #26561 ) ;
#40649=CARTESIAN_POINT ( 'NONE',  ( -12.55851384766255663, -4.403642575758160760, 8.787212689424128698 ) ) ;
#40650=EDGE_CURVE ( 'NONE', #47105, #31087, #5288, .T. ) ;
#40651=EDGE_LOOP ( 'NONE', ( #10482, #2676, #29634, #47609 ) ) ;
#40652=FACE_OUTER_BOUND ( 'NONE', #55130, .T. ) ;
#40653=ADVANCED_FACE ( 'NONE', ( #47593 ), #29987, .F. ) ;
#40654=ORIENTED_EDGE ( 'NONE', *, *, #9445, .T. ) ;
#40656=CARTESIAN_POINT ( 'NONE',  ( -19.79569077582305070, 0.000000000000000000, 14.58012466630350445 ) ) ;
#40657=CARTESIAN_POINT ( 'NONE',  ( -20.23897083037251576, 0.6102101463440048335, 5.744283514253277545 ) ) ;
#40658=ORIENTED_EDGE ( 'NONE', *, *, #11433, .T. ) ;
#40659=ADVANCED_FACE ( 'NONE', ( #43053 ), #12675, .F. ) ;
#40660=VECTOR ( 'NONE', #27831, 1000.000000000000227 ) ;
#40661=CARTESIAN_POINT ( 'NONE',  ( -21.32662440292010686, -3.756034771668159689, 11.13020985957213860 ) ) ;
#40662=DIRECTION ( 'NONE',  ( -0.5364919789714478471, 0.6444004775717705469, -0.5449076811759709926 ) ) ;
#40663=LINE ( 'NONE', #13679, #11280 ) ;
#40665=EDGE_CURVE ( 'NONE', #40102, #23572, #34811, .T. ) ;
#40666=CARTESIAN_POINT ( 'NONE',  ( -18.35624807862726371, 0.000000000000000000, 8.740207326407432475 ) ) ;
#40667=CARTESIAN_POINT ( 'NONE',  ( -17.74404816805336793, 0.000000000000000000, 3.574322630375089460 ) ) ;
#40668=EDGE_CURVE ( 'NONE', #1004, #4402, #22326, .T. ) ;
#40670=ORIENTED_EDGE ( 'NONE', *, *, #2239, .F. ) ;
#40671=CARTESIAN_POINT ( 'NONE',  ( -10.74029228357944987, 0.000000000000000000, 11.14194120806293320 ) ) ;
#40672=LINE ( 'NONE', #35553, #47637 ) ;
#40674=ORIENTED_EDGE ( 'NONE', *, *, #49469, .T. ) ;
#40675=CARTESIAN_POINT ( 'NONE',  ( -22.12213066651850113, 5.629170628041515023, 5.095318538108095652 ) ) ;
#40676=CARTESIAN_POINT ( 'NONE',  ( -1.086233639165236964, 0.000000000000000000, -2.796443541562362078 ) ) ;
#40677=ORIENTED_EDGE ( 'NONE', *, *, #19102, .F. ) ;
#40678=EDGE_CURVE ( 'NONE', #25320, #38090, #13777, .T. ) ;
#40679=LINE ( 'NONE', #49475, #5923 ) ;
#40680=LINE ( 'NONE', #10286, #32328 ) ;
#40681=ADVANCED_FACE ( 'NONE', ( #17784 ), #9541, .F. ) ;
#40682=FACE_OUTER_BOUND ( 'NONE', #51701, .T. ) ;
#40683=ORIENTED_EDGE ( 'NONE', *, *, #34617, .T. ) ;
#40684=ORIENTED_EDGE ( 'NONE', *, *, #21364, .F. ) ;
#40685=DIRECTION ( 'NONE',  ( -0.7660212471507179544, -0.6427876096865405842, -0.005961354470445141482 ) ) ;
#40686=LINE ( 'NONE', #48917, #54108 ) ;
#40687=CARTESIAN_POINT ( 'NONE',  ( -15.32299166378033739, 3.038739411681507185, 7.820380517850593627 ) ) ;
#40688=ADVANCED_FACE ( 'NONE', ( #30578 ), #8984, .F. ) ;
#40689=VERTEX_POINT ( 'NONE', #35121 ) ;
#40691=ORIENTED_EDGE ( 'NONE', *, *, #19298, .T. ) ;
#40692=CARTESIAN_POINT ( 'NONE',  ( -19.60834386242827776, 0.000000000000000000, 4.298478389818581213 ) ) ;
#40693=ADVANCED_FACE ( 'NONE', ( #21754 ), #52126, .F. ) ;
#40694=PLANE ( 'NONE',  #19687 ) ;
#40695=ORIENTED_EDGE ( 'NONE', *, *, #32558, .T. ) ;
#40696=LINE ( 'NONE', #1767, #5718 ) ;
#40697=DIRECTION ( 'NONE',  ( -0.6427681459581293666, -0.7660444431189770143, -0.005002170337467561935 ) ) ;
#40698=PLANE ( 'NONE',  #49328 ) ;
#40699=ORIENTED_EDGE ( 'NONE', *, *, #9188, .F. ) ;
#40700=VECTOR ( 'NONE', #30480, 999.9999999999998863 ) ;
#40701=DIRECTION ( 'NONE',  ( -0.9999697198139514409, -0.000000000000000000, -0.007781995580013368816 ) ) ;
#40702=ORIENTED_EDGE ( 'NONE', *, *, #10232, .F. ) ;
#40706=ORIENTED_EDGE ( 'NONE', *, *, #782, .F. ) ;
#40708=ORIENTED_EDGE ( 'NONE', *, *, #12634, .F. ) ;
#40709=DIRECTION ( 'NONE',  ( -0.7660212471507179544, -0.6427876096865405842, -0.005961354470445141482 ) ) ;
#40711=ORIENTED_EDGE ( 'NONE', *, *, #41307, .T. ) ;
#40712=CARTESIAN_POINT ( 'NONE',  ( -19.60990026154428278, 0.000000000000000000, 4.498472333781370125 ) ) ;
#40713=EDGE_CURVE ( 'NONE', #27792, #5782, #9241, .T. ) ;
#40714=VERTEX_POINT ( 'NONE', #39906 ) ;
#40715=CARTESIAN_POINT ( 'NONE',  ( -14.93495759592298988, 0.000000000000000000, 12.77129166681078409 ) ) ;
#40716=EDGE_CURVE ( 'NONE', #25279, #28407, #4704, .T. ) ;
#40717=DIRECTION ( 'NONE',  ( -0.9999697198139514409, -0.000000000000000000, -0.007781995580013368816 ) ) ;
#40719=ADVANCED_FACE ( 'NONE', ( #34272 ), #52420, .F. ) ;
#40720=DIRECTION ( 'NONE',  ( 0.9999697198139515519, 0.000000000000000000, 0.007781995580013368816 ) ) ;
#40721=FACE_OUTER_BOUND ( 'NONE', #34220, .T. ) ;
#40722=CARTESIAN_POINT ( 'NONE',  ( -26.13415699229845757, -0.1191753592594197858, 6.933020519852192365 ) ) ;
#40723=CARTESIAN_POINT ( 'NONE',  ( -11.37388075760056161, 0.000000000000000000, 7.147891430601540641 ) ) ;
#40724=ORIENTED_EDGE ( 'NONE', *, *, #2007, .T. ) ;
#40725=ADVANCED_FACE ( 'NONE', ( #30832 ), #12946, .F. ) ;
#40726=EDGE_CURVE ( 'NONE', #15181, #50938, #35372, .T. ) ;
#40727=ADVANCED_FACE ( 'NONE', ( #30275 ), #31946, .F. ) ;
#40728=VERTEX_POINT ( 'NONE', #40186 ) ;
#40729=DIRECTION ( 'NONE',  ( -0.005961354470445682716, -0.6427876096865404731, 0.7660212471507180654 ) ) ;
#40730=CARTESIAN_POINT ( 'NONE',  ( -16.79925329029790149, 0.000000000000000000, 13.49544742625427496 ) ) ;
#40731=CARTESIAN_POINT ( 'NONE',  ( -18.71016998902382511, -0.1191753592594162470, 7.360127773147754127 ) ) ;
#40733=VERTEX_POINT ( 'NONE', #31411 ) ;
#40734=PLANE ( 'NONE',  #20379 ) ;
#40735=CARTESIAN_POINT ( 'NONE',  ( -18.36067853124854921, 0.000000000000000000, 9.309510973627983077 ) ) ;
#40737=DIRECTION ( 'NONE',  ( 0.005961354470445682716, -0.6427876096865404731, -0.7660212471507180654 ) ) ;
#40739=VERTEX_POINT ( 'NONE', #28742 ) ;
#40741=DIRECTION ( 'NONE',  ( -0.7660212471507179544, -0.6427876096865405842, -0.005961354470445141482 ) ) ;
#40742=PLANE ( 'NONE',  #22423 ) ;
#40743=EDGE_CURVE ( 'NONE', #39023, #45704, #19917, .T. ) ;
#40744=DIRECTION ( 'NONE',  ( 0.007781995580012663651, 0.000000000000000000, -0.9999697198139515519 ) ) ;
#40745=FACE_OUTER_BOUND ( 'NONE', #16035, .T. ) ;
#40746=EDGE_CURVE ( 'NONE', #19074, #46703, #18616, .T. ) ;
#40747=DIRECTION ( 'NONE',  ( 0.5364919789714477361, 0.6444004775717706579, 0.5449076811759711036 ) ) ;
#40748=EDGE_LOOP ( 'NONE', ( #19866, #2998, #20153, #17205 ) ) ;
#40749=ORIENTED_EDGE ( 'NONE', *, *, #40063, .T. ) ;
#40750=ADVANCED_FACE ( 'NONE', ( #40491 ), #18907, .F. ) ;
#40751=LINE ( 'NONE', #23433, #10349 ) ;
#40752=CARTESIAN_POINT ( 'NONE',  ( -10.81131361120978696, -0.1191753592594194527, 7.417854936013363876 ) ) ;
#40753=LINE ( 'NONE', #5281, #13385 ) ;
#40754=EDGE_CURVE ( 'NONE', #45599, #39737, #23442, .T. ) ;
#40755=CARTESIAN_POINT ( 'NONE',  ( -12.99507170543344436, 0.000000000000000000, 2.333958040294567660 ) ) ;
#40757=VERTEX_POINT ( 'NONE', #22863 ) ;
#40758=PLANE ( 'NONE',  #15611 ) ;
#40759=DIRECTION ( 'NONE',  ( 0.007781995580012663651, 0.000000000000000000, -0.9999697198139515519 ) ) ;
#40760=FACE_OUTER_BOUND ( 'NONE', #8657, .T. ) ;
#40761=DIRECTION ( 'NONE',  ( 0.007781995580012663651, -3.146120232559066537E-19, -0.9999697198139514409 ) ) ;
#40762=ORIENTED_EDGE ( 'NONE', *, *, #18086, .T. ) ;
#40763=CARTESIAN_POINT ( 'NONE',  ( -12.53462651648692194, 0.000000000000000000, 2.876199414615318251 ) ) ;
#40764=ORIENTED_EDGE ( 'NONE', *, *, #42407, .T. ) ;
#40765=LINE ( 'NONE', #8080, #12343 ) ;
#40766=PLANE ( 'NONE',  #1237 ) ;
#40767=EDGE_LOOP ( 'NONE', ( #32649, #46343, #56071, #5845 ) ) ;
#40768=CARTESIAN_POINT ( 'NONE',  ( -13.17065887352947762, -0.1191753592594197858, 12.04635770780929427 ) ) ;
#40769=VERTEX_POINT ( 'NONE', #36221 ) ;
#40770=ORIENTED_EDGE ( 'NONE', *, *, #37258, .T. ) ;
#40771=ORIENTED_EDGE ( 'NONE', *, *, #22422, .F. ) ;
#40772=DIRECTION ( 'NONE',  ( 0.7660212471507180654, -0.6427876096865404731, 0.005961354470445141482 ) ) ;
#40773=ORIENTED_EDGE ( 'NONE', *, *, #46152, .F. ) ;
#40774=ORIENTED_EDGE ( 'NONE', *, *, #40989, .F. ) ;
#40775=DIRECTION ( 'NONE',  ( 0.007781995580012663651, -3.146120232559066537E-19, -0.9999697198139514409 ) ) ;
#40776=DIRECTION ( 'NONE',  ( -0.005961354470445682716, -0.6427876096865404731, 0.7660212471507180654 ) ) ;
#40777=ORIENTED_EDGE ( 'NONE', *, *, #10402, .F. ) ;
#40778=VERTEX_POINT ( 'NONE', #2859 ) ;
#40779=LINE ( 'NONE', #37625, #31362 ) ;
#40780=ORIENTED_EDGE ( 'NONE', *, *, #49333, .F. ) ;
#40781=EDGE_CURVE ( 'NONE', #47262, #21619, #986, .T. ) ;
#40782=ORIENTED_EDGE ( 'NONE', *, *, #14757, .T. ) ;
#40784=DIRECTION ( 'NONE',  ( 0.7660212471507180654, -0.6427876096865404731, 0.005961354470445141482 ) ) ;
#40785=DIRECTION ( 'NONE',  ( 0.000000000000000000, 0.000000000000000000, 1.000000000000000000 ) ) ;
#40786=CARTESIAN_POINT ( 'NONE',  ( -15.02654820080420706, -4.079838673713164887, 2.587974528106823602 ) ) ;
#40787=CARTESIAN_POINT ( 'NONE',  ( -20.54126990917373519, -0.1191753592594197858, 4.760553241521720658 ) ) ;
#40788=VERTEX_POINT ( 'NONE', #50298 ) ;
#40789=CARTESIAN_POINT ( 'NONE',  ( -21.47263955680318404, 0.000000000000000000, 5.022634149262071190 ) ) ;
#40790=VERTEX_POINT ( 'NONE', #37237 ) ;
#40791=EDGE_CURVE ( 'NONE', #36173, #48176, #53278, .T. ) ;
#40792=ADVANCED_FACE ( 'NONE', ( #11413 ), #54539, .F. ) ;
#40793=EDGE_CURVE ( 'NONE', #3654, #19401, #46050, .T. ) ;
#40794=CARTESIAN_POINT ( 'NONE',  ( -17.29326687045830724, -0.1191753592594164690, 4.416497882389668561 ) ) ;
#40795=EDGE_CURVE ( 'NONE', #52907, #37899, #31682, .T. ) ;
#40797=DIRECTION ( 'NONE',  ( 0.9999697198139515519, 0.000000000000000000, 0.007781995580013368816 ) ) ;
#40798=FACE_OUTER_BOUND ( 'NONE', #16956, .T. ) ;
#40799=CARTESIAN_POINT ( 'NONE',  ( -18.19747506107908563, 0.000000000000000000, 14.03856424583689311 ) ) ;
#40800=CARTESIAN_POINT ( 'NONE',  ( -20.09258446552595245, -0.1191753592594195638, 5.872041224812675431 ) ) ;
#40801=ORIENTED_EDGE ( 'NONE', *, *, #42849, .T. ) ;
#40802=DIRECTION ( 'NONE',  ( 0.000000000000000000, -1.000000000000000000, 0.000000000000000000 ) ) ;
#40803=VERTEX_POINT ( 'NONE', #27399 ) ;
#40804=LINE ( 'NONE', #10722, #5680 ) ;
#40805=LINE ( 'NONE', #53848, #15128 ) ;
#40806=LINE ( 'NONE', #14422, #39018 ) ;
#40807=DIRECTION ( 'NONE',  ( -0.005961354470445682716, -0.6427876096865404731, 0.7660212471507180654 ) ) ;
#40808=DIRECTION ( 'NONE',  ( 0.000000000000000000, -1.000000000000000000, 0.000000000000000000 ) ) ;
#40809=CARTESIAN_POINT ( 'NONE',  ( -12.64977195555273148, -0.1191753592594188005, 4.821966703327531079 ) ) ;
#40810=ORIENTED_EDGE ( 'NONE', *, *, #51310, .T. ) ;
#40811=EDGE_CURVE ( 'NONE', #43546, #14582, #44721, .T. ) ;
#40812=LINE ( 'NONE', #6450, #39369 ) ;
#40813=DIRECTION ( 'NONE',  ( 0.007781995580012662783, 0.000000000000000000, -0.9999697198139514409 ) ) ;
#40815=EDGE_CURVE ( 'NONE', #40825, #6164, #24456, .T. ) ;
#40816=DIRECTION ( 'NONE',  ( 0.007781995580012662783, 0.000000000000000000, -0.9999697198139514409 ) ) ;
#40817=LINE ( 'NONE', #10733, #51145 ) ;
#40818=DIRECTION ( 'NONE',  ( 0.7660212471507180654, -0.6427876096865404731, 0.005961354470445141482 ) ) ;
#40819=FACE_OUTER_BOUND ( 'NONE', #17750, .T. ) ;
#40820=ADVANCED_FACE ( 'NONE', ( #5839 ), #23161, .F. ) ;
#40821=DIRECTION ( 'NONE',  ( -0.6427681459581293666, -0.7660444431189770143, -0.005002170337467561935 ) ) ;
#40822=CARTESIAN_POINT ( 'NONE',  ( -14.81148421494233780, -3.270328918600661439, 2.530263971831323566 ) ) ;
#40823=ORIENTED_EDGE ( 'NONE', *, *, #9121, .T. ) ;
#40824=ORIENTED_EDGE ( 'NONE', *, *, #3462, .F. ) ;
#40825=VERTEX_POINT ( 'NONE', #30471 ) ;
#40826=ORIENTED_EDGE ( 'NONE', *, *, #44878, .F. ) ;
#40827=ORIENTED_EDGE ( 'NONE', *, *, #37405, .T. ) ;
#40828=EDGE_LOOP ( 'NONE', ( #40351, #2824, #48655, #19455 ) ) ;
#40829=LINE ( 'NONE', #40572, #17862 ) ;
#40830=DIRECTION ( 'NONE',  ( -0.5449076811759708816, 0.6444004775717707689, 0.5364919789714475140 ) ) ;
#40831=EDGE_LOOP ( 'NONE', ( #20626, #22572, #38938 ) ) ;
#40832=ORIENTED_EDGE ( 'NONE', *, *, #39654, .F. ) ;
#40833=ORIENTED_EDGE ( 'NONE', *, *, #41738, .F. ) ;
#40834=VECTOR ( 'NONE', #45953, 1000.000000000000227 ) ;
#40836=CARTESIAN_POINT ( 'NONE',  ( -15.50102849149811135, -0.1191753592594197858, 12.95155240711365430 ) ) ;
#40837=CARTESIAN_POINT ( 'NONE',  ( -19.60834386242827776, 0.000000000000000000, 4.298478389818581213 ) ) ;
#40838=ORIENTED_EDGE ( 'NONE', *, *, #20107, .F. ) ;
#40839=DIRECTION ( 'NONE',  ( 0.5449076811759707706, 0.6444004775717708799, -0.5364919789714476250 ) ) ;
#40840=EDGE_CURVE ( 'NONE', #6678, #37427, #8894, .T. ) ;
#40841=ORIENTED_EDGE ( 'NONE', *, *, #5091, .T. ) ;
#40842=FACE_OUTER_BOUND ( 'NONE', #7368, .T. ) ;
#40843=DIRECTION ( 'NONE',  ( -0.005961354470445682716, -0.6427876096865404731, 0.7660212471507180654 ) ) ;
#40844=EDGE_CURVE ( 'NONE', #55993, #32241, #52020, .T. ) ;
#40845=EDGE_CURVE ( 'NONE', #23263, #34917, #892, .T. ) ;
#40846=CARTESIAN_POINT ( 'NONE',  ( -28.92982233430281980, 0.000000000000000000, 7.919257187036034651 ) ) ;
#40847=DIRECTION ( 'NONE',  ( 0.5364919789714477361, 0.6444004775717706579, 0.5449076811759711036 ) ) ;
#40848=LINE ( 'NONE', #44832, #19518 ) ;
#40849=DIRECTION ( 'NONE',  ( 0.007781995580012663651, 0.000000000000000000, -0.9999697198139515519 ) ) ;
#40850=LINE ( 'NONE', #20084, #24841 ) ;
#40851=CARTESIAN_POINT ( 'NONE',  ( -29.86274838104827367, -0.1191753592594197858, 8.381332038739175871 ) ) ;
#40852=ORIENTED_EDGE ( 'NONE', *, *, #27192, .T. ) ;
#40853=LINE ( 'NONE', #44289, #23776 ) ;
#40854=ORIENTED_EDGE ( 'NONE', *, *, #40390, .F. ) ;
#40855=DIRECTION ( 'NONE',  ( 0.9999697198139515519, 0.000000000000000000, 0.007781995580013368816 ) ) ;
#40856=DIRECTION ( 'NONE',  ( -0.6427681459581293666, -0.7660444431189770143, -0.005002170337467561935 ) ) ;
#40857=DIRECTION ( 'NONE',  ( 0.9999697198139515519, 0.000000000000000000, 0.007781995580013368816 ) ) ;
#40858=CARTESIAN_POINT ( 'NONE',  ( -19.60834386242827776, 0.000000000000000000, 4.298478389818581213 ) ) ;
#40860=CARTESIAN_POINT ( 'NONE',  ( -22.12471055240100881, 3.362543313726509719, 10.99381648943753476 ) ) ;
#40861=LINE ( 'NONE', #27240, #5323 ) ;
#40862=CARTESIAN_POINT ( 'NONE',  ( -8.609916609573598834, 0.000000000000000000, 10.23519010964256637 ) ) ;
#40864=CARTESIAN_POINT ( 'NONE',  ( -24.26908309836554878, 0.000000000000000000, 6.108867788427308376 ) ) ;
#40865=VERTEX_POINT ( 'NONE', #18212 ) ;
#40866=DIRECTION ( 'NONE',  ( 0.5449076811759707706, 0.6444004775717708799, -0.5364919789714476250 ) ) ;
#40867=DIRECTION ( 'NONE',  ( -0.5449076811759708816, 0.6444004775717707689, 0.5364919789714475140 ) ) ;
#40869=DIRECTION ( 'NONE',  ( -0.5364919789714478471, 0.6444004775717705469, -0.5449076811759709926 ) ) ;
#40871=DIRECTION ( 'NONE',  ( -0.005002170337468016433, -0.7660444431189770143, 0.6427681459581293666 ) ) ;
#40872=DIRECTION ( 'NONE',  ( 0.005961354470445682716, -0.6427876096865404731, -0.7660212471507180654 ) ) ;
#40873=EDGE_CURVE ( 'NONE', #41466, #49575, #26198, .T. ) ;
#40874=LINE ( 'NONE', #1952, #42325 ) ;
#40875=PLANE ( 'NONE',  #29247 ) ;
#40876=ORIENTED_EDGE ( 'NONE', *, *, #15880, .F. ) ;
#40877=VECTOR ( 'NONE', #11104, 1000.000000000000227 ) ;
#40878=VERTEX_POINT ( 'NONE', #26748 ) ;
#40879=EDGE_CURVE ( 'NONE', #32990, #34138, #22214, .T. ) ;
#40880=CARTESIAN_POINT ( 'NONE',  ( -24.26908309836554878, 0.000000000000000000, 6.108867788427308376 ) ) ;
#40881=LINE ( 'NONE', #20115, #35914 ) ;
#40882=ORIENTED_EDGE ( 'NONE', *, *, #25075, .F. ) ;
#40883=DIRECTION ( 'NONE',  ( -0.005961354470445682716, -0.6427876096865404731, 0.7660212471507180654 ) ) ;
#40884=EDGE_CURVE ( 'NONE', #9862, #17943, #13136, .T. ) ;
#40885=ORIENTED_EDGE ( 'NONE', *, *, #14966, .T. ) ;
#40886=LINE ( 'NONE', #44577, #42911 ) ;
#40887=ORIENTED_EDGE ( 'NONE', *, *, #10054, .F. ) ;
#40888=ORIENTED_EDGE ( 'NONE', *, *, #37764, .T. ) ;
#40889=ORIENTED_EDGE ( 'NONE', *, *, #17035, .F. ) ;
#40890=DIRECTION ( 'NONE',  ( -0.6427681459581293666, -0.7660444431189770143, -0.005002170337467561935 ) ) ;
#40891=DIRECTION ( 'NONE',  ( -0.5364919789714478471, 0.6444004775717705469, -0.5449076811759709926 ) ) ;
#40892=PLANE ( 'NONE',  #5799 ) ;
#40893=VECTOR ( 'NONE', #21279, 999.9999999999998863 ) ;
#40894=ORIENTED_EDGE ( 'NONE', *, *, #32819, .T. ) ;
#40895=ORIENTED_EDGE ( 'NONE', *, *, #11219, .T. ) ;
#40896=FACE_OUTER_BOUND ( 'NONE', #41717, .T. ) ;
#40897=EDGE_LOOP ( 'NONE', ( #13596, #41099, #10943, #30835 ) ) ;
#40898=LINE ( 'NONE', #7118, #32759 ) ;
#40899=EDGE_CURVE ( 'NONE', #34678, #33817, #34701, .T. ) ;
#40900=EDGE_LOOP ( 'NONE', ( #18012, #25670, #36038, #53267 ) ) ;
#40901=LINE ( 'NONE', #41186, #32122 ) ;
#40902=CARTESIAN_POINT ( 'NONE',  ( -11.20636620717317378, 0.000000000000000000, 11.32298014792380414 ) ) ;
#40903=ORIENTED_EDGE ( 'NONE', *, *, #19542, .T. ) ;
#40904=VECTOR ( 'NONE', #23529, 1000.000000000000000 ) ;
#40905=DIRECTION ( 'NONE',  ( 0.007781995580012663651, 0.000000000000000000, -0.9999697198139515519 ) ) ;
#40906=EDGE_CURVE ( 'NONE', #51780, #50886, #4351, .T. ) ;
#40907=VECTOR ( 'NONE', #23555, 999.9999999999998863 ) ;
#40908=CARTESIAN_POINT ( 'NONE',  ( -19.18251504283423259, 1.581621852479005774, 4.082609997287097947 ) ) ;
#40909=ORIENTED_EDGE ( 'NONE', *, *, #53041, .T. ) ;
#40910=DIRECTION ( 'NONE',  ( 0.9999697198139515519, 0.000000000000000000, 0.007781995580013368816 ) ) ;
#40911=CARTESIAN_POINT ( 'NONE',  ( -18.99737516508532309, 0.000000000000000000, 8.735217927174451447 ) ) ;
#40912=CARTESIAN_POINT ( 'NONE',  ( -8.509919637592204822, -0.1191753592594197858, 10.23596830920056711 ) ) ;
#40913=VERTEX_POINT ( 'NONE', #45131 ) ;
#40914=CARTESIAN_POINT ( 'NONE',  ( 2.072287782118878319, 0.000000000000000000, -2.950529333540147015 ) ) ;
#40915=FACE_OUTER_BOUND ( 'NONE', #15472, .T. ) ;
#40916=LINE ( 'NONE', #1997, #37597 ) ;
#40917=DIRECTION ( 'NONE',  ( -0.005002170337468016433, -0.7660444431189770143, 0.6427681459581293666 ) ) ;
#40918=LINE ( 'NONE', #40081, #43968 ) ;
#40919=DIRECTION ( 'NONE',  ( 0.005961354470445682716, -0.6427876096865404731, -0.7660212471507180654 ) ) ;
#40920=ADVANCED_FACE ( 'NONE', ( #637 ), #39240, .F. ) ;
#40922=ORIENTED_EDGE ( 'NONE', *, *, #4687, .T. ) ;
#40923=DIRECTION ( 'NONE',  ( -0.8531650599175527594, 0.4028455766673922356, 0.3313982828793700652 ) ) ;
#40924=LINE ( 'NONE', #16210, #52172 ) ;
#40926=VERTEX_POINT ( 'NONE', #23534 ) ;
#40928=CARTESIAN_POINT ( 'NONE',  ( -29.86197018149027116, 0.000000000000000000, 8.281335066757780083 ) ) ;
#40929=VECTOR ( 'NONE', #28664, 999.9999999999998863 ) ;
#40930=AXIS2_PLACEMENT_3D ( 'NONE', #2565, #37480, #33252 ) ;
#40931=DIRECTION ( 'NONE',  ( 0.007781995580012662783, 0.000000000000000000, -0.9999697198139514409 ) ) ;
#40932=LINE ( 'NONE', #31861, #4277 ) ;
#40933=CARTESIAN_POINT ( 'NONE',  ( 2.072287782118878319, 0.000000000000000000, -2.950529333540147015 ) ) ;
#40934=VERTEX_POINT ( 'NONE', #39813 ) ;
#40935=ORIENTED_EDGE ( 'NONE', *, *, #15645, .T. ) ;
#40936=LINE ( 'NONE', #15131, #7766 ) ;
#40937=DIRECTION ( 'NONE',  ( 0.7660212471507180654, -0.6427876096865404731, 0.005961354470445141482 ) ) ;
#40938=CARTESIAN_POINT ( 'NONE',  ( -25.20278734466900517, 0.000000000000000000, 6.670939612111840944 ) ) ;
#40939=EDGE_LOOP ( 'NONE', ( #25902, #4026, #13395, #15743 ) ) ;
#40940=PLANE ( 'NONE',  #19499 ) ;
#40941=EDGE_CURVE ( 'NONE', #37781, #30111, #332, .T. ) ;
#40942=ORIENTED_EDGE ( 'NONE', *, *, #10407, .T. ) ;
#40943=CARTESIAN_POINT ( 'NONE',  ( -18.58021353734938685, 1.419719901456505617, 3.853821158198948993 ) ) ;
#40944=AXIS2_PLACEMENT_3D ( 'NONE', #38310, #43427, #38611 ) ;
#40945=ORIENTED_EDGE ( 'NONE', *, *, #28292, .T. ) ;
#40946=ORIENTED_EDGE ( 'NONE', *, *, #31371, .T. ) ;
#40947=PLANE ( 'NONE',  #22943 ) ;
#40948=CARTESIAN_POINT ( 'NONE',  ( -25.20278734466900517, 0.000000000000000000, 6.670939612111840944 ) ) ;
#40949=CARTESIAN_POINT ( 'NONE',  ( -26.13415699229845757, -0.1191753592594197858, 6.933020519852192365 ) ) ;
#40950=EDGE_CURVE ( 'NONE', #5490, #25102, #17673, .T. ) ;
#40951=VERTEX_POINT ( 'NONE', #39 ) ;
#40953=VERTEX_POINT ( 'NONE', #52852 ) ;
#40954=EDGE_CURVE ( 'NONE', #14910, #15700, #35013, .T. ) ;
#40955=ADVANCED_FACE ( 'NONE', ( #31291 ), #48618, .F. ) ;
#40956=EDGE_LOOP ( 'NONE', ( #2966, #48667, #45630, #26773 ) ) ;
#40957=VERTEX_POINT ( 'NONE', #12845 ) ;
#40958=CARTESIAN_POINT ( 'NONE',  ( -18.39746900504187010, 0.000000000000000000, 14.03700784672088808 ) ) ;
#40959=VERTEX_POINT ( 'NONE', #30743 ) ;
#40960=FACE_OUTER_BOUND ( 'NONE', #14233, .T. ) ;
#40962=ADVANCED_FACE ( 'NONE', ( #48043 ), #4888, .F. ) ;
#40963=EDGE_LOOP ( 'NONE', ( #42025, #11523, #39342, #40235 ) ) ;
#40964=CARTESIAN_POINT ( 'NONE',  ( -19.05391333978853652, 0.000000000000000000, 4.672125166152008013 ) ) ;
#40965=LINE ( 'NONE', #28184, #2288 ) ;
#40966=VECTOR ( 'NONE', #44498, 1000.000000000000227 ) ;
#40967=AXIS2_PLACEMENT_3D ( 'NONE', #21524, #55878, #12706 ) ;
#40968=VERTEX_POINT ( 'NONE', #48307 ) ;
#40969=EDGE_CURVE ( 'NONE', #3673, #44736, #9422, .T. ) ;
#40971=ORIENTED_EDGE ( 'NONE', *, *, #26573, .T. ) ;
#40972=EDGE_CURVE ( 'NONE', #16295, #6087, #43255, .T. ) ;
#40973=DIRECTION ( 'NONE',  ( 0.5449076811759707706, 0.6444004775717708799, -0.5364919789714476250 ) ) ;
#40974=CARTESIAN_POINT ( 'NONE',  ( -22.40556560354864146, -0.1191753592594197858, 5.484709000965211523 ) ) ;
#40975=VECTOR ( 'NONE', #22831, 1000.000000000000227 ) ;
#40976=DIRECTION ( 'NONE',  ( -0.5449076811759708816, 0.6444004775717707689, 0.5364919789714475140 ) ) ;
#40977=FACE_OUTER_BOUND ( 'NONE', #12579, .T. ) ;
#40978=CARTESIAN_POINT ( 'NONE',  ( -9.075990533167328067, 0.000000000000000000, 10.41622904950343909 ) ) ;
#40979=CARTESIAN_POINT ( 'NONE',  ( -32.65997012216863737, 0.000000000000000000, 9.567562649885804404 ) ) ;
#40980=ORIENTED_EDGE ( 'NONE', *, *, #544, .F. ) ;
#40981=ADVANCED_FACE ( 'NONE', ( #42257 ), #11309, .F. ) ;
#40982=ORIENTED_EDGE ( 'NONE', *, *, #44838, .T. ) ;
#40985=VECTOR ( 'NONE', #54439, 999.9999999999998863 ) ;
#40986=LINE ( 'NONE', #17529, #15795 ) ;
#40987=VECTOR ( 'NONE', #40973, 1000.000000000000114 ) ;
#40988=DIRECTION ( 'NONE',  ( 0.5364919789714477361, 0.6444004775717706579, 0.5449076811759711036 ) ) ;
#40989=EDGE_CURVE ( 'NONE', #15522, #53467, #37414, .T. ) ;
#40990=DIRECTION ( 'NONE',  ( 0.007781995580012663651, -3.146120232559066537E-19, -0.9999697198139514409 ) ) ;
#40992=DIRECTION ( 'NONE',  ( -0.005002170337468016433, -0.7660444431189770143, 0.6427681459581293666 ) ) ;
#40993=FACE_OUTER_BOUND ( 'NONE', #32111, .T. ) ;
#40994=ORIENTED_EDGE ( 'NONE', *, *, #555, .T. ) ;
#40995=FACE_OUTER_BOUND ( 'NONE', #41849, .T. ) ;
#40996=DIRECTION ( 'NONE',  ( 0.9999697198139515519, 0.000000000000000000, 0.007781995580013368816 ) ) ;
#40997=ORIENTED_EDGE ( 'NONE', *, *, #48403, .F. ) ;
#40999=DIRECTION ( 'NONE',  ( 0.007781995580012662783, 0.000000000000000000, -0.9999697198139514409 ) ) ;
#41000=LINE ( 'NONE', #11179, #27744 ) ;
#41001=DIRECTION ( 'NONE',  ( -0.005961354470445682716, -0.6427876096865404731, 0.7660212471507180654 ) ) ;
#41002=CARTESIAN_POINT ( 'NONE',  ( -9.110551994824897193, -1.000000000000000000, 3.538847790438064411 ) ) ;
#41003=ORIENTED_EDGE ( 'NONE', *, *, #51275, .F. ) ;
#41004=ORIENTED_EDGE ( 'NONE', *, *, #41298, .T. ) ;
#41005=DIRECTION ( 'NONE',  ( 0.007781995580012663651, 0.000000000000000000, -0.9999697198139515519 ) ) ;
#41006=DIRECTION ( 'NONE',  ( -0.7660212471507179544, -0.6427876096865405842, -0.005961354470445141482 ) ) ;
#41008=LINE ( 'NONE', #31405, #34259 ) ;
#41009=VECTOR ( 'NONE', #51766, 1000.000000000000227 ) ;
#41010=AXIS2_PLACEMENT_3D ( 'NONE', #22444, #53626, #44836 ) ;
#41011=CARTESIAN_POINT ( 'NONE',  ( -28.93137873341882127, 0.000000000000000000, 8.119251130998824451 ) ) ;
#41012=DIRECTION ( 'NONE',  ( 0.5364919789714477361, 0.6444004775717706579, 0.5449076811759711036 ) ) ;
#41013=EDGE_CURVE ( 'NONE', #5645, #40951, #24633, .T. ) ;
#41014=EDGE_LOOP ( 'NONE', ( #30450, #20139, #11659, #51049 ) ) ;
#41015=FACE_OUTER_BOUND ( 'NONE', #52381, .T. ) ;
#41017=AXIS2_PLACEMENT_3D ( 'NONE', #34529, #4169, #35128 ) ;
#41018=DIRECTION ( 'NONE',  ( -0.5364919789714478471, 0.6444004775717705469, -0.5449076811759709926 ) ) ;
#41019=VECTOR ( 'NONE', #36378, 999.9999999999998863 ) ;
#41020=VERTEX_POINT ( 'NONE', #28918 ) ;
#41021=LINE ( 'NONE', #54101, #53736 ) ;
#41023=DIRECTION ( 'NONE',  ( 0.007781995580012663651, 0.000000000000000000, -0.9999697198139515519 ) ) ;
#41024=ADVANCED_FACE ( 'NONE', ( #7318 ), #50504, .F. ) ;
#41025=DIRECTION ( 'NONE',  ( 0.000000000000000000, -1.000000000000000000, 0.000000000000000000 ) ) ;
#41026=ORIENTED_EDGE ( 'NONE', *, *, #4952, .T. ) ;
#41027=CARTESIAN_POINT ( 'NONE',  ( -20.93202838136840427, 2.553033558614008047, 4.731187272372491037 ) ) ;
#41029=VERTEX_POINT ( 'NONE', #2761 ) ;
#41030=EDGE_CURVE ( 'NONE', #8484, #30283, #49912, .T. ) ;
#41031=EDGE_LOOP ( 'NONE', ( #24221, #43034, #47056, #22758 ) ) ;
#41032=VERTEX_POINT ( 'NONE', #37151 ) ;
#41033=DIRECTION ( 'NONE',  ( -0.5364919789714478471, 0.6444004775717705469, -0.5449076811759709926 ) ) ;
#41034=VERTEX_POINT ( 'NONE', #45960 ) ;
#41035=ORIENTED_EDGE ( 'NONE', *, *, #27339, .F. ) ;
#41036=LINE ( 'NONE', #1297, #32920 ) ;
#41037=EDGE_LOOP ( 'NONE', ( #54951, #53555, #15066, #37642 ) ) ;
#41038=ORIENTED_EDGE ( 'NONE', *, *, #47082, .T. ) ;
#41040=ADVANCED_FACE ( 'NONE', ( #28072 ), #3364, .F. ) ;
#41041=EDGE_LOOP ( 'NONE', ( #28726, #52104, #24337, #461 ) ) ;
#41042=VECTOR ( 'NONE', #50518, 1000.000000000000227 ) ;
#41043=ORIENTED_EDGE ( 'NONE', *, *, #20888, .T. ) ;
#41044=EDGE_CURVE ( 'NONE', #2953, #20314, #32881, .T. ) ;
#41045=EDGE_LOOP ( 'NONE', ( #52389, #670, #8956, #2669 ) ) ;
#41046=CARTESIAN_POINT ( 'NONE',  ( -16.73601541380021374, 1.419719901456506728, 5.712160089342227742 ) ) ;
#41048=CARTESIAN_POINT ( 'NONE',  ( -11.79352356370524646, 0.000000000000000000, 1.362631486225394761 ) ) ;
#41049=LINE ( 'NONE', #40787, #9625 ) ;
#41050=VECTOR ( 'NONE', #27329, 1000.000000000000227 ) ;
#41052=CARTESIAN_POINT ( 'NONE',  ( -10.33808368536842970, -0.1191753592594177180, 6.317285075198634026 ) ) ;
#41053=ORIENTED_EDGE ( 'NONE', *, *, #18991, .T. ) ;
#41054=VECTOR ( 'NONE', #4504, 999.9999999999998863 ) ;
#41055=ADVANCED_FACE ( 'NONE', ( #11016 ), #19555, .F. ) ;
#41056=VECTOR ( 'NONE', #39045, 999.9999999999998863 ) ;
#41057=ORIENTED_EDGE ( 'NONE', *, *, #39169, .T. ) ;
#41058=FACE_OUTER_BOUND ( 'NONE', #45625, .T. ) ;
#41059=CARTESIAN_POINT ( 'NONE',  ( 1.086233639165236964, 0.000000000000000000, 2.796443541562362078 ) ) ;
#41060=VECTOR ( 'NONE', #7498, 999.9999999999998863 ) ;
#41062=CARTESIAN_POINT ( 'NONE',  ( -12.56779750416103347, 0.000000000000000000, 7.138600094413515507 ) ) ;
#41063=FACE_OUTER_BOUND ( 'NONE', #19097, .T. ) ;
#41064=DIRECTION ( 'NONE',  ( -0.5449076811759708816, 0.6444004775717707689, 0.5364919789714475140 ) ) ;
#41065=VERTEX_POINT ( 'NONE', #37725 ) ;
#41066=PLANE ( 'NONE',  #23821 ) ;
#41067=ORIENTED_EDGE ( 'NONE', *, *, #9982, .F. ) ;
#41068=CARTESIAN_POINT ( 'NONE',  ( -27.99767448711536133, 0.000000000000000000, 7.557179307314289218 ) ) ;
#41069=DIRECTION ( 'NONE',  ( 0.007781995580012662783, 0.000000000000000000, -0.9999697198139514409 ) ) ;
#41070=CARTESIAN_POINT ( 'NONE',  ( -18.86354292863559579, 0.000000000000000000, 14.21804678658176080 ) ) ;
#41071=VECTOR ( 'NONE', #47339, 999.9999999999998863 ) ;
#41073=AXIS2_PLACEMENT_3D ( 'NONE', #20909, #23322, #40639 ) ;
#41074=LINE ( 'NONE', #36275, #32292 ) ;
#41075=ORIENTED_EDGE ( 'NONE', *, *, #55532, .T. ) ;
#41076=DIRECTION ( 'NONE',  ( -0.9999697198139514409, -0.000000000000000000, -0.007781995580013368816 ) ) ;
#41077=LINE ( 'NONE', #24047, #22187 ) ;
#41078=DIRECTION ( 'NONE',  ( 0.007781995580012663651, -3.146120232559066537E-19, -0.9999697198139514409 ) ) ;
#41079=EDGE_CURVE ( 'NONE', #20591, #54534, #10764, .T. ) ;
#41080=AXIS2_PLACEMENT_3D ( 'NONE', #44402, #31646, #26518 ) ;
#41081=CARTESIAN_POINT ( 'NONE',  ( -9.758301349461536489, 0.000000000000000000, 4.375133698254432879 ) ) ;
#41082=CARTESIAN_POINT ( 'NONE',  ( -17.42697428494509282, 0.000000000000000000, 8.747439149943453174 ) ) ;
#41083=EDGE_CURVE ( 'NONE', #28433, #32707, #24366, .T. ) ;
#41084=VECTOR ( 'NONE', #45214, 1000.000000000000000 ) ;
#41085=LINE ( 'NONE', #33139, #43607 ) ;
#41087=PLANE ( 'NONE',  #32392 ) ;
#41088=EDGE_CURVE ( 'NONE', #5802, #20904, #6778, .T. ) ;
#41089=VECTOR ( 'NONE', #30958, 999.9999999999998863 ) ;
#41090=LINE ( 'NONE', #10156, #18358 ) ;
#41091=EDGE_CURVE ( 'NONE', #5706, #661, #20384, .T. ) ;
#41092=EDGE_CURVE ( 'NONE', #11344, #4466, #19830, .T. ) ;
#41093=ADVANCED_FACE ( 'NONE', ( #46489 ), #15551, .F. ) ;
#41094=VECTOR ( 'NONE', #7157, 1000.000000000000227 ) ;
#41095=VECTOR ( 'NONE', #14603, 1000.000000000000000 ) ;
#41096=EDGE_LOOP ( 'NONE', ( #18061, #28871, #42944, #46717, #47236 ) ) ;
#41097=VECTOR ( 'NONE', #4855, 999.9999999999998863 ) ;
#41098=ORIENTED_EDGE ( 'NONE', *, *, #33018, .F. ) ;
#41099=ORIENTED_EDGE ( 'NONE', *, *, #12120, .F. ) ;
#41100=AXIS2_PLACEMENT_3D ( 'NONE', #23612, #31306, #10280 ) ;
#41101=ORIENTED_EDGE ( 'NONE', *, *, #15688, .F. ) ;
#41102=ORIENTED_EDGE ( 'NONE', *, *, #17979, .T. ) ;
#41103=DIRECTION ( 'NONE',  ( 0.5364919789714477361, 0.6444004775717706579, 0.5449076811759711036 ) ) ;
#41104=CARTESIAN_POINT ( 'NONE',  ( -11.22056963685719211, 0.000000000000000000, 1.239771416285661010 ) ) ;
#41105=EDGE_LOOP ( 'NONE', ( #31473, #36277, #36698, #81 ) ) ;
#41106=ORIENTED_EDGE ( 'NONE', *, *, #40097, .T. ) ;
#41107=ADVANCED_FACE ( 'NONE', ( #50200 ), #20086, .F. ) ;
#41108=VERTEX_POINT ( 'NONE', #52927 ) ;
#41109=AXIS2_PLACEMENT_3D ( 'NONE', #37910, #2424, #15746 ) ;
#41110=ORIENTED_EDGE ( 'NONE', *, *, #28830, .T. ) ;
#41111=EDGE_CURVE ( 'NONE', #3615, #8086, #1789, .T. ) ;
#41114=CARTESIAN_POINT ( 'NONE',  ( -32.65919192261063841, -0.1191753592594197858, 9.467565677904410393 ) ) ;
#41115=PLANE ( 'NONE',  #44058 ) ;
#41116=ORIENTED_EDGE ( 'NONE', *, *, #48385, .F. ) ;
#41117=DIRECTION ( 'NONE',  ( -0.6246952433987893460, -0.7422098413412802076, 0.2426528472758542054 ) ) ;
#41118=VECTOR ( 'NONE', #37991, 999.9999999999998863 ) ;
#41119=EDGE_CURVE ( 'NONE', #56078, #42377, #36441, .T. ) ;
#41120=CARTESIAN_POINT ( 'NONE',  ( -10.00813838035478298, 0.000000000000000000, 10.77830692922518452 ) ) ;
#41121=CARTESIAN_POINT ( 'NONE',  ( -13.23242834496490872, 0.000000000000000000, 7.133427783529502797 ) ) ;
#41122=VECTOR ( 'NONE', #35046, 1000.000000000000227 ) ;
#41123=EDGE_CURVE ( 'NONE', #49125, #8091, #49523, .T. ) ;
#41124=CARTESIAN_POINT ( 'NONE',  ( -16.81345671998191449, 0.000000000000000000, 3.412238694616132495 ) ) ;
#41125=DIRECTION ( 'NONE',  ( -0.005961354470445682716, -0.6427876096865404731, 0.7660212471507180654 ) ) ;
#41126=LINE ( 'NONE', #49667, #9520 ) ;
#41127=CARTESIAN_POINT ( 'NONE',  ( -11.87243407472968926, 0.000000000000000000, 11.50246268866867361 ) ) ;
#41128=CARTESIAN_POINT ( 'NONE',  ( -14.66887761629205222, 0.000000000000000000, 12.58869632783390990 ) ) ;
#41129=VECTOR ( 'NONE', #28526, 1000.000000000000114 ) ;
#41130=DIRECTION ( 'NONE',  ( -0.005961354470445682716, -0.6427876096865404731, 0.7660212471507180654 ) ) ;
#41131=ORIENTED_EDGE ( 'NONE', *, *, #1013, .F. ) ;
#41132=LINE ( 'NONE', #11311, #44700 ) ;
#41133=VERTEX_POINT ( 'NONE', #32199 ) ;
#41134=VECTOR ( 'NONE', #9796, 1000.000000000000227 ) ;
#41135=VECTOR ( 'NONE', #43560, 1000.000000000000227 ) ;
#41136=CARTESIAN_POINT ( 'NONE',  ( -14.93495759592298988, 0.000000000000000000, 12.77129166681078409 ) ) ;
#41137=CARTESIAN_POINT ( 'NONE',  ( -12.55917534364518495, 0.000000000000000000, 6.030670984640223331 ) ) ;
#41138=LINE ( 'NONE', #3567, #39470 ) ;
#41139=PLANE ( 'NONE',  #25050 ) ;
#41140=DIRECTION ( 'NONE',  ( 0.6246952433987894571, -0.7422098413412800966, -0.2426528472758541777 ) ) ;
#41141=DIRECTION ( 'NONE',  ( 0.007781995580012663651, -3.146120232559066537E-19, -0.9999697198139514409 ) ) ;
#41142=VECTOR ( 'NONE', #52039, 1000.000000000000000 ) ;
#41144=AXIS2_PLACEMENT_3D ( 'NONE', #26093, #20698, #3639 ) ;
#41146=DIRECTION ( 'NONE',  ( -0.9999697198139514409, -0.000000000000000000, -0.007781995580013368816 ) ) ;
#41147=PLANE ( 'NONE',  #39326 ) ;
#41148=LINE ( 'NONE', #32080, #47607 ) ;
#41149=PLANE ( 'NONE',  #50866 ) ;
#41150=PLANE ( 'NONE',  #11475 ) ;
#41151=DIRECTION ( 'NONE',  ( 0.9999697198139515519, 0.000000000000000000, 0.007781995580013368816 ) ) ;
#41152=DIRECTION ( 'NONE',  ( -0.005002170337468016433, -0.7660444431189770143, 0.6427681459581293666 ) ) ;
#41153=FACE_OUTER_BOUND ( 'NONE', #38294, .T. ) ;
#41154=CARTESIAN_POINT ( 'NONE',  ( -22.40634380310664397, 0.000000000000000000, 5.584705972946605534 ) ) ;
#41155=ORIENTED_EDGE ( 'NONE', *, *, #35861, .F. ) ;
#41156=CARTESIAN_POINT ( 'NONE',  ( -11.77243710274829525, -0.1191753592594197858, 11.50324088822667612 ) ) ;
#41157=ORIENTED_EDGE ( 'NONE', *, *, #21705, .T. ) ;
#41158=AXIS2_PLACEMENT_3D ( 'NONE', #52373, #42999, #30225 ) ;
#41159=DIRECTION ( 'NONE',  ( 0.007781995580012663651, -3.146120232559066537E-19, -0.9999697198139514409 ) ) ;
#41160=DIRECTION ( 'NONE',  ( -0.7660212471507179544, -0.6427876096865405842, -0.005961354470445141482 ) ) ;
#41161=AXIS2_PLACEMENT_3D ( 'NONE', #32048, #45125, #18727 ) ;
#41162=ADVANCED_FACE ( 'NONE', ( #1537 ), #6102, .F. ) ;
#41163=EDGE_CURVE ( 'NONE', #37134, #45757, #10046, .T. ) ;
#41164=ORIENTED_EDGE ( 'NONE', *, *, #2743, .T. ) ;
#41165=DIRECTION ( 'NONE',  ( -0.000000000000000000, -1.000000000000000000, 0.000000000000000000 ) ) ;
#41166=AXIS2_PLACEMENT_3D ( 'NONE', #46799, #11308, #32880 ) ;
#41167=VERTEX_POINT ( 'NONE', #40145 ) ;
#41168=DIRECTION ( 'NONE',  ( -0.005002170337468016433, -0.7660444431189770143, 0.6427681459581293666 ) ) ;
#41169=EDGE_CURVE ( 'NONE', #33959, #18846, #40449, .T. ) ;
#41170=ORIENTED_EDGE ( 'NONE', *, *, #40589, .T. ) ;
#41171=ORIENTED_EDGE ( 'NONE', *, *, #49205, .T. ) ;
#41172=EDGE_LOOP ( 'NONE', ( #49658, #50439, #17340, #44327 ) ) ;
#41174=VECTOR ( 'NONE', #50862, 1000.000000000000227 ) ;
#41175=DIRECTION ( 'NONE',  ( 0.000000000000000000, -1.000000000000000000, 0.000000000000000000 ) ) ;
#41176=DIRECTION ( 'NONE',  ( 0.9999697198139515519, 0.000000000000000000, 0.007781995580013368816 ) ) ;
#41177=AXIS2_PLACEMENT_3D ( 'NONE', #43439, #38056, #8825 ) ;
#41178=VERTEX_POINT ( 'NONE', #22825 ) ;
#41179=ORIENTED_EDGE ( 'NONE', *, *, #42511, .T. ) ;
#41180=VECTOR ( 'NONE', #36854, 1000.000000000000000 ) ;
#41181=VECTOR ( 'NONE', #10729, 1000.000000000000114 ) ;
#41182=DIRECTION ( 'NONE',  ( 0.007781995580012663651, -3.146120232559066537E-19, -0.9999697198139514409 ) ) ;
#41183=ORIENTED_EDGE ( 'NONE', *, *, #30299, .F. ) ;
#41184=DIRECTION ( 'NONE',  ( -0.005961354470445682716, -0.6427876096865404731, 0.7660212471507180654 ) ) ;
#41185=ORIENTED_EDGE ( 'NONE', *, *, #43247, .T. ) ;
#41186=CARTESIAN_POINT ( 'NONE',  ( -28.93137873341882127, 0.000000000000000000, 8.119251130998824451 ) ) ;
#41187=DIRECTION ( 'NONE',  ( 0.007781995580012663651, -3.146120232559066537E-19, -0.9999697198139514409 ) ) ;
#41188=EDGE_LOOP ( 'NONE', ( #37289, #9151, #47370 ) ) ;
#41189=LINE ( 'NONE', #20734, #26415 ) ;
#41190=EDGE_CURVE ( 'NONE', #47896, #33095, #26819, .T. ) ;
#41191=AXIS2_PLACEMENT_3D ( 'NONE', #23583, #6013, #10815 ) ;
#41192=DIRECTION ( 'NONE',  ( -0.6427681459581293666, -0.7660444431189770143, -0.005002170337467561935 ) ) ;
#41193=VERTEX_POINT ( 'NONE', #53489 ) ;
#41195=FACE_OUTER_BOUND ( 'NONE', #26296, .T. ) ;
#41196=LINE ( 'NONE', #41734, #32109 ) ;
#41197=DIRECTION ( 'NONE',  ( -0.6427681459581293666, -0.7660444431189770143, -0.005002170337467561935 ) ) ;
#41198=EDGE_CURVE ( 'NONE', #49377, #8607, #36185, .T. ) ;
#41199=ORIENTED_EDGE ( 'NONE', *, *, #7927, .T. ) ;
#41200=AXIS2_PLACEMENT_3D ( 'NONE', #29709, #43020, #17445 ) ;
#41201=LINE ( 'NONE', #28135, #55527 ) ;
#41202=DIRECTION ( 'NONE',  ( 0.007781995580012662783, 0.000000000000000000, -0.9999697198139514409 ) ) ;
#41203=EDGE_CURVE ( 'NONE', #5052, #39740, #27100, .T. ) ;
#41204=CARTESIAN_POINT ( 'NONE',  ( -10.79697247519895420, -0.1191753592594185784, 5.575049756915096744 ) ) ;
#41205=CARTESIAN_POINT ( 'NONE',  ( -12.15116108492864377, 0.000000000000000000, 1.401855352044617975 ) ) ;
#41207=LINE ( 'NONE', #45734, #12495 ) ;
#41208=CARTESIAN_POINT ( 'NONE',  ( -9.808144436391993182, 0.000000000000000000, 10.77986332834118777 ) ) ;
#41210=VERTEX_POINT ( 'NONE', #35339 ) ;
#41211=CARTESIAN_POINT ( 'NONE',  ( -16.89925026227929195, -0.1191753592594197858, 13.49466922669627422 ) ) ;
#41212=LINE ( 'NONE', #36973, #31400 ) ;
#41214=ORIENTED_EDGE ( 'NONE', *, *, #35393, .F. ) ;
#41215=VECTOR ( 'NONE', #31188, 1000.000000000000227 ) ;
#41216=PLANE ( 'NONE',  #15668 ) ;
#41217=DIRECTION ( 'NONE',  ( -0.5449076811759708816, 0.6444004775717707689, 0.5364919789714475140 ) ) ;
#41218=VECTOR ( 'NONE', #49911, 999.9999999999998863 ) ;
#41219=CARTESIAN_POINT ( 'NONE',  ( -9.542064456761055524, 0.000000000000000000, 10.59726798936431180 ) ) ;
#41222=ORIENTED_EDGE ( 'NONE', *, *, #44122, .F. ) ;
#41223=AXIS2_PLACEMENT_3D ( 'NONE', #39348, #4702, #437 ) ;
#41224=VECTOR ( 'NONE', #31017, 999.9999999999998863 ) ;
#41225=EDGE_LOOP ( 'NONE', ( #5205, #23172, #26970, #33313 ) ) ;
#41226=FACE_OUTER_BOUND ( 'NONE', #21579, .T. ) ;
#41229=VERTEX_POINT ( 'NONE', #23402 ) ;
#41230=DIRECTION ( 'NONE',  ( 0.007781995580012663651, 0.000000000000000000, -0.9999697198139515519 ) ) ;
#41231=ORIENTED_EDGE ( 'NONE', *, *, #7980, .T. ) ;
#41232=LINE ( 'NONE', #23906, #19274 ) ;
#41233=EDGE_CURVE ( 'NONE', #9162, #48014, #52639, .T. ) ;
#41234=EDGE_CURVE ( 'NONE', #19170, #8089, #31648, .T. ) ;
#41235=VECTOR ( 'NONE', #19503, 999.9999999999998863 ) ;
#41237=ORIENTED_EDGE ( 'NONE', *, *, #54619, .T. ) ;
#41238=VECTOR ( 'NONE', #49964, 1000.000000000000000 ) ;
#41239=CARTESIAN_POINT ( 'NONE',  ( -17.46397131646373779, 3.362543313726509719, 9.183427090828809369 ) ) ;
#41240=CARTESIAN_POINT ( 'NONE',  ( -14.66887761629205222, 0.000000000000000000, 12.58869632783390990 ) ) ;
#41241=AXIS2_PLACEMENT_3D ( 'NONE', #21381, #30473, #30170 ) ;
#41242=DIRECTION ( 'NONE',  ( 0.005961354470445682716, -0.6427876096865404731, -0.7660212471507180654 ) ) ;
#41244=DIRECTION ( 'NONE',  ( 0.5364919789714477361, 0.6444004775717706579, 0.5449076811759711036 ) ) ;
#41245=AXIS2_PLACEMENT_3D ( 'NONE', #36665, #3422, #55650 ) ;
#41246=ORIENTED_EDGE ( 'NONE', *, *, #19176, .T. ) ;
#41247=EDGE_CURVE ( 'NONE', #3660, #41644, #44146, .T. ) ;
#41248=ORIENTED_EDGE ( 'NONE', *, *, #29596, .T. ) ;
#41249=ORIENTED_EDGE ( 'NONE', *, *, #25328, .F. ) ;
#41250=AXIS2_PLACEMENT_3D ( 'NONE', #15162, #5790, #49214 ) ;
#41251=LINE ( 'NONE', #50023, #35894 ) ;
#41252=AXIS2_PLACEMENT_3D ( 'NONE', #28492, #2073, #2375 ) ;
#41253=VERTEX_POINT ( 'NONE', #22562 ) ;
#41254=AXIS2_PLACEMENT_3D ( 'NONE', #20302, #12057, #29394 ) ;
#41255=VECTOR ( 'NONE', #52694, 1000.000000000000227 ) ;
#41256=PLANE ( 'NONE',  #48413 ) ;
#41258=ORIENTED_EDGE ( 'NONE', *, *, #38818, .T. ) ;
#41259=LINE ( 'NONE', #44975, #46723 ) ;
#41260=PLANE ( 'NONE',  #15915 ) ;
#41261=VECTOR ( 'NONE', #15361, 999.9999999999998863 ) ;
#41262=ORIENTED_EDGE ( 'NONE', *, *, #34292, .F. ) ;
#41263=FACE_OUTER_BOUND ( 'NONE', #46109, .T. ) ;
#41264=ORIENTED_EDGE ( 'NONE', *, *, #5579, .T. ) ;
#41265=CIRCLE ( 'NONE', #43971, 6.999999999999999112 ) ;
#41266=CARTESIAN_POINT ( 'NONE',  ( -19.61438316718806973, -0.1166911823299058987, 4.400518953728226990 ) ) ;
#41267=VECTOR ( 'NONE', #21157, 1000.000000000000000 ) ;
#41268=CARTESIAN_POINT ( 'NONE',  ( -11.14243809316658052, -10.74105472484483670, 1.109727778512525687 ) ) ;
#41269=CARTESIAN_POINT ( 'NONE',  ( -11.20636620717317378, 0.000000000000000000, 11.32298014792380414 ) ) ;
#41270=DIRECTION ( 'NONE',  ( 0.9999697198139515519, 0.000000000000000000, 0.007781995580013368816 ) ) ;
#41271=PLANE ( 'NONE',  #12381 ) ;
#41272=LINE ( 'NONE', #489, #4700 ) ;
#41274=EDGE_LOOP ( 'NONE', ( #29152, #42901, #34026, #13332 ) ) ;
#41275=EDGE_LOOP ( 'NONE', ( #16494, #15946, #2957, #19777 ) ) ;
#41276=LINE ( 'NONE', #41553, #37324 ) ;
#41277=ADVANCED_FACE ( 'NONE', ( #24776 ), #39872, .F. ) ;
#41278=DIRECTION ( 'NONE',  ( 0.000000000000000000, -1.000000000000000000, 0.000000000000000000 ) ) ;
#41279=LINE ( 'NONE', #10891, #4050 ) ;
#41280=DIRECTION ( 'NONE',  ( -0.7660212471507179544, -0.6427876096865405842, -0.005961354470445141482 ) ) ;
#41281=VECTOR ( 'NONE', #43343, 1000.000000000000227 ) ;
#41283=ORIENTED_EDGE ( 'NONE', *, *, #15032, .F. ) ;
#41284=VECTOR ( 'NONE', #21772, 1000.000000000000227 ) ;
#41285=DIRECTION ( 'NONE',  ( 0.007781995580012662783, 0.000000000000000000, -0.9999697198139514409 ) ) ;
#41286=CARTESIAN_POINT ( 'NONE',  ( -22.40634380310664397, 0.000000000000000000, 5.584705972946605534 ) ) ;
#41287=ORIENTED_EDGE ( 'NONE', *, *, #5860, .T. ) ;
#41288=LINE ( 'NONE', #36456, #55602 ) ;
#41289=DIRECTION ( 'NONE',  ( 0.9999697198139515519, 0.000000000000000000, 0.007781995580013368816 ) ) ;
#41290=VECTOR ( 'NONE', #26537, 1000.000000000000114 ) ;
#41291=VERTEX_POINT ( 'NONE', #23939 ) ;
#41292=EDGE_CURVE ( 'NONE', #37937, #53290, #29037, .T. ) ;
#41294=DIRECTION ( 'NONE',  ( 0.7660212471507180654, -0.6427876096865404731, 0.005961354470445141482 ) ) ;
#41295=VECTOR ( 'NONE', #19257, 1000.000000000000227 ) ;
#41296=CARTESIAN_POINT ( 'NONE',  ( -13.94865558154716112, 0.000000000000000000, 5.450519602115640794 ) ) ;
#41297=EDGE_CURVE ( 'NONE', #43180, #43341, #46082, .T. ) ;
#41298=EDGE_CURVE ( 'NONE', #39217, #39457, #42091, .T. ) ;
#41299=FACE_OUTER_BOUND ( 'NONE', #32447, .T. ) ;
#41300=ORIENTED_EDGE ( 'NONE', *, *, #30659, .T. ) ;
#41301=VECTOR ( 'NONE', #44336, 999.9999999999998863 ) ;
#41302=VECTOR ( 'NONE', #21606, 999.9999999999998863 ) ;
#41303=ORIENTED_EDGE ( 'NONE', *, *, #17724, .F. ) ;
#41304=DIRECTION ( 'NONE',  ( 0.9999697198139515519, 0.000000000000000000, 0.007781995580013368816 ) ) ;
#41305=CARTESIAN_POINT ( 'NONE',  ( -12.23851102634202448, -0.1191753592594197858, 11.68427982808754884 ) ) ;
#41306=CARTESIAN_POINT ( 'NONE',  ( -20.26176469941677993, 0.000000000000000000, 14.76116360616437895 ) ) ;
#41307=EDGE_CURVE ( 'NONE', #42825, #10301, #45799, .T. ) ;
#41308=VECTOR ( 'NONE', #30331, 1000.000000000000000 ) ;
#41310=VECTOR ( 'NONE', #28762, 1000.000000000000114 ) ;
#41311=DIRECTION ( 'NONE',  ( -0.5364919789714478471, 0.6444004775717705469, -0.5449076811759709926 ) ) ;
#41312=EDGE_CURVE ( 'NONE', #35388, #48977, #54319, .T. ) ;
#41313=DIRECTION ( 'NONE',  ( 0.9999697198139515519, 0.000000000000000000, 0.007781995580013368816 ) ) ;
#41314=ORIENTED_EDGE ( 'NONE', *, *, #44317, .T. ) ;
#41315=CARTESIAN_POINT ( 'NONE',  ( -21.47419595591918906, 0.000000000000000000, 5.222628093224860102 ) ) ;
#41316=ADVANCED_FACE ( 'NONE', ( #2361 ), #11721, .F. ) ;
#41317=VECTOR ( 'NONE', #12883, 1000.000000000000227 ) ;
#41318=DIRECTION ( 'NONE',  ( 0.7660212471507180654, -0.6427876096865404731, 0.005961354470445141482 ) ) ;
#41319=VECTOR ( 'NONE', #30047, 999.9999999999998863 ) ;
#41321=ORIENTED_EDGE ( 'NONE', *, *, #51283, .T. ) ;
#41322=CARTESIAN_POINT ( 'NONE',  ( -10.74029228357944987, 0.000000000000000000, 11.14194120806293320 ) ) ;
#41323=CARTESIAN_POINT ( 'NONE',  ( -12.60458797795435615, 0.000000000000000000, 11.86609696750642229 ) ) ;
#41324=CARTESIAN_POINT ( 'NONE',  ( -16.83725213413307031, -0.1191753592594191197, 5.528042903930973750 ) ) ;
#41325=ADVANCED_FACE ( 'NONE', ( #37019 ), #50883, .F. ) ;
#41326=ORIENTED_EDGE ( 'NONE', *, *, #4209, .F. ) ;
#41327=DIRECTION ( 'NONE',  ( 0.007781995580012662783, 0.000000000000000000, -0.9999697198139514409 ) ) ;
#41328=ORIENTED_EDGE ( 'NONE', *, *, #50258, .F. ) ;
#41329=VECTOR ( 'NONE', #38738, 999.9999999999998863 ) ;
#41330=ADVANCED_FACE ( 'NONE', ( #32485 ), #19952, .F. ) ;
#41331=VERTEX_POINT ( 'NONE', #7188 ) ;
#41332=VERTEX_POINT ( 'NONE', #24488 ) ;
#41333=EDGE_LOOP ( 'NONE', ( #6877, #52010, #38083, #38997 ) ) ;
#41334=AXIS2_PLACEMENT_3D ( 'NONE', #48002, #5987, #14493 ) ;
#41335=EDGE_LOOP ( 'NONE', ( #18300, #41688, #55418, #49076 ) ) ;
#41336=CARTESIAN_POINT ( 'NONE',  ( -23.33693525117809386, 0.000000000000000000, 5.746789908705562944 ) ) ;
#41337=AXIS2_PLACEMENT_3D ( 'NONE', #20932, #12457, #30034 ) ;
#41338=VERTEX_POINT ( 'NONE', #37271 ) ;
#41339=ORIENTED_EDGE ( 'NONE', *, *, #30736, .T. ) ;
#41340=FACE_OUTER_BOUND ( 'NONE', #32470, .T. ) ;
#41341=ORIENTED_EDGE ( 'NONE', *, *, #41669, .T. ) ;
#41342=AXIS2_PLACEMENT_3D ( 'NONE', #17057, #55962, #21007 ) ;
#41343=ORIENTED_EDGE ( 'NONE', *, *, #45917, .T. ) ;
#41344=EDGE_LOOP ( 'NONE', ( #11653, #32264, #3097, #18413 ) ) ;
#41345=DIRECTION ( 'NONE',  ( -0.5364919789714478471, 0.6444004775717705469, -0.5449076811759709926 ) ) ;
#41346=CARTESIAN_POINT ( 'NONE',  ( -18.67619601524082285, 0.000000000000000000, 3.936400510096834893 ) ) ;
#41347=LINE ( 'NONE', #37338, #10559 ) ;
#41348=DIRECTION ( 'NONE',  ( -0.9999697198139514409, -0.000000000000000000, -0.007781995580013368816 ) ) ;
#41349=VECTOR ( 'NONE', #18089, 1000.000000000000114 ) ;
#41350=ORIENTED_EDGE ( 'NONE', *, *, #48541, .F. ) ;
#41351=FACE_OUTER_BOUND ( 'NONE', #44390, .T. ) ;
#41352=ORIENTED_EDGE ( 'NONE', *, *, #48568, .F. ) ;
#41353=AXIS2_PLACEMENT_3D ( 'NONE', #13378, #46660, #55187 ) ;
#41354=ORIENTED_EDGE ( 'NONE', *, *, #26987, .T. ) ;
#41355=AXIS2_PLACEMENT_3D ( 'NONE', #10479, #22428, #40283 ) ;
#41356=CARTESIAN_POINT ( 'NONE',  ( -18.07819366188567400, 3.038739411681509850, 3.607164391028207628 ) ) ;
#41357=EDGE_CURVE ( 'NONE', #5052, #22227, #33022, .T. ) ;
#41358=PLANE ( 'NONE',  #14906 ) ;
#41359=AXIS2_PLACEMENT_3D ( 'NONE', #24146, #23574, #23318 ) ;
#41361=VECTOR ( 'NONE', #25715, 1000.000000000000000 ) ;
#41362=DIRECTION ( 'NONE',  ( -0.3620778797217461542, -0.000000000000000000, -0.9321478471874538041 ) ) ;
#41364=CARTESIAN_POINT ( 'NONE',  ( -11.70900194784942805, -0.1191753592594185784, 3.351959713832490362 ) ) ;
#41365=ORIENTED_EDGE ( 'NONE', *, *, #51624, .T. ) ;
#41366=CARTESIAN_POINT ( 'NONE',  ( -24.27063949748155380, 0.000000000000000000, 6.308861732390097288 ) ) ;
#41367=ORIENTED_EDGE ( 'NONE', *, *, #17618, .T. ) ;
#41368=EDGE_CURVE ( 'NONE', #49949, #33064, #2896, .T. ) ;
#41369=CARTESIAN_POINT ( 'NONE',  ( -9.542064456761055524, 0.000000000000000000, 10.59726798936431180 ) ) ;
#41370=FACE_OUTER_BOUND ( 'NONE', #49813, .T. ) ;
#41371=DIRECTION ( 'NONE',  ( 0.007781995580012663651, 0.000000000000000000, -0.9999697198139515519 ) ) ;
#41372=PLANE ( 'NONE',  #29518 ) ;
#41373=EDGE_CURVE ( 'NONE', #42922, #13439, #50628, .T. ) ;
#41374=CARTESIAN_POINT ( 'NONE',  ( -15.99857495235844418, 0.000000000000000000, 4.326570446154306637 ) ) ;
#41375=AXIS2_PLACEMENT_3D ( 'NONE', #3585, #19593, #4165 ) ;
#41376=ORIENTED_EDGE ( 'NONE', *, *, #31629, .F. ) ;
#41377=LINE ( 'NONE', #2166, #41181 ) ;
#41378=CARTESIAN_POINT ( 'NONE',  ( -11.35508003745286310, 0.000000000000000000, 4.732039267092165602 ) ) ;
#41379=LINE ( 'NONE', #23229, #14612 ) ;
#41380=AXIS2_PLACEMENT_3D ( 'NONE', #35933, #35626, #13756 ) ;
#41381=CARTESIAN_POINT ( 'NONE',  ( -15.05936134377114044, 0.000000000000000000, 3.056557400622056608 ) ) ;
#41382=ADVANCED_FACE ( 'NONE', ( #40977 ), #2062, .F. ) ;
#41383=FACE_OUTER_BOUND ( 'NONE', #46131, .T. ) ;
#41384=DIRECTION ( 'NONE',  ( -0.005961354470445682716, -0.6427876096865404731, 0.7660212471507180654 ) ) ;
#41385=LINE ( 'NONE', #49882, #14754 ) ;
#41386=EDGE_CURVE ( 'NONE', #41034, #4870, #25616, .T. ) ;
#41387=AXIS2_PLACEMENT_3D ( 'NONE', #30100, #4288, #22449 ) ;
#41389=DIRECTION ( 'NONE',  ( 0.005961354470445682716, -0.6427876096865404731, -0.7660212471507180654 ) ) ;
#41390=VECTOR ( 'NONE', #14485, 1000.000000000000227 ) ;
#41391=EDGE_CURVE ( 'NONE', #27257, #41560, #8891, .T. ) ;
#41392=ORIENTED_EDGE ( 'NONE', *, *, #49306, .T. ) ;
#41393=AXIS2_PLACEMENT_3D ( 'NONE', #27101, #5256, #52092 ) ;
#41394=VECTOR ( 'NONE', #33154, 1000.000000000000227 ) ;
#41395=EDGE_CURVE ( 'NONE', #3168, #7513, #55429, .T. ) ;
#41396=VERTEX_POINT ( 'NONE', #51180 ) ;
#41397=VECTOR ( 'NONE', #48332, 1000.000000000000227 ) ;
#41398=ORIENTED_EDGE ( 'NONE', *, *, #22648, .T. ) ;
#41399=ORIENTED_EDGE ( 'NONE', *, *, #28749, .T. ) ;
#41400=ORIENTED_EDGE ( 'NONE', *, *, #53243, .F. ) ;
#41401=CARTESIAN_POINT ( 'NONE',  ( -10.84028925556084388, -0.1191753592594197858, 11.14116300850493246 ) ) ;
#41402=DIRECTION ( 'NONE',  ( -0.7660212471507179544, -0.6427876096865405842, -0.005961354470445141482 ) ) ;
#41403=ORIENTED_EDGE ( 'NONE', *, *, #52598, .T. ) ;
#41404=CARTESIAN_POINT ( 'NONE',  ( -16.75880829507524439, 3.686347215771511365, 3.074008228493816386 ) ) ;
#41405=ORIENTED_EDGE ( 'NONE', *, *, #22722, .F. ) ;
#41406=ORIENTED_EDGE ( 'NONE', *, *, #45527, .T. ) ;
#41407=AXIS2_PLACEMENT_3D ( 'NONE', #9354, #4819, #43998 ) ;
#41409=FACE_OUTER_BOUND ( 'NONE', #39794, .T. ) ;
#41410=CARTESIAN_POINT ( 'NONE',  ( -9.975539614456023330, 0.000000000000000000, 6.589435518685016646 ) ) ;
#41411=EDGE_LOOP ( 'NONE', ( #13170, #36297, #50675, #48829 ) ) ;
#41412=LINE ( 'NONE', #36582, #20134 ) ;
#41413=LINE ( 'NONE', #20077, #8302 ) ;
#41414=VECTOR ( 'NONE', #37115, 1000.000000000000227 ) ;
#41415=EDGE_CURVE ( 'NONE', #47873, #7239, #12576, .T. ) ;
#41416=CARTESIAN_POINT ( 'NONE',  ( -11.73723008791625766, -0.1117717739994089354, 7.777512339822061804 ) ) ;
#41417=DIRECTION ( 'NONE',  ( 0.9321478471874541372, 0.000000000000000000, -0.3620778797217453771 ) ) ;
#41418=CARTESIAN_POINT ( 'NONE',  ( -17.73140113748535285, 0.000000000000000000, 13.85752530597602039 ) ) ;
#41419=VECTOR ( 'NONE', #14965, 1000.000000000000227 ) ;
#41420=ADVANCED_FACE ( 'NONE', ( #16530 ), #42942, .F. ) ;
#41421=CARTESIAN_POINT ( 'NONE',  ( -9.342070512798265725, 0.000000000000000000, 10.59882438848031505 ) ) ;
#41422=DIRECTION ( 'NONE',  ( 0.000000000000000000, -0.000000000000000000, -1.000000000000000000 ) ) ;
#41423=LINE ( 'NONE', #50502, #54785 ) ;
#41424=ADVANCED_FACE ( 'NONE', ( #47480 ), #47783, .F. ) ;
#41425=CARTESIAN_POINT ( 'NONE',  ( -9.115871106642465804, 2.779451633208005923, 3.525154055174515744 ) ) ;
#41426=ORIENTED_EDGE ( 'NONE', *, *, #29406, .T. ) ;
#41428=ORIENTED_EDGE ( 'NONE', *, *, #27472, .T. ) ;
#41429=EDGE_CURVE ( 'NONE', #43064, #1437, #29892, .T. ) ;
#41430=EDGE_CURVE ( 'NONE', #33602, #33755, #4046, .T. ) ;
#41431=ADVANCED_FACE ( 'NONE', ( #43499 ), #29630, .F. ) ;
#41432=AXIS2_PLACEMENT_3D ( 'NONE', #4477, #21787, #26321 ) ;
#41433=FACE_OUTER_BOUND ( 'NONE', #53087, .T. ) ;
#41434=CARTESIAN_POINT ( 'NONE',  ( -11.77243710274829525, -0.1191753592594197858, 11.50324088822667612 ) ) ;
#41435=LINE ( 'NONE', #42543, #24154 ) ;
#41436=DIRECTION ( 'NONE',  ( -0.5364919789714478471, 0.6444004775717705469, -0.5449076811759709926 ) ) ;
#41437=DIRECTION ( 'NONE',  ( 0.8531650599175529814, -0.4028455766673920135, -0.3313982828793697877 ) ) ;
#41438=VECTOR ( 'NONE', #17287, 999.9999999999998863 ) ;
#41439=VECTOR ( 'NONE', #47997, 999.9999999999998863 ) ;
#41440=FACE_OUTER_BOUND ( 'NONE', #22860, .T. ) ;
#41442=DIRECTION ( 'NONE',  ( -0.005002170337468016433, -0.7660444431189770143, 0.6427681459581293666 ) ) ;
#41443=CARTESIAN_POINT ( 'NONE',  ( -11.14933798647950880, 0.000000000000000000, 3.994976259692639697 ) ) ;
#41444=FACE_OUTER_BOUND ( 'NONE', #30708, .T. ) ;
#41445=DIRECTION ( 'NONE',  ( 0.000000000000000000, -1.000000000000000000, 0.000000000000000000 ) ) ;
#41446=FACE_OUTER_BOUND ( 'NONE', #22542, .T. ) ;
#41447=CARTESIAN_POINT ( 'NONE',  ( -18.66354898467281132, 0.000000000000000000, 14.21960318569776582 ) ) ;
#41448=ADVANCED_FACE ( 'NONE', ( #4347 ), #13421, .F. ) ;
#41449=CARTESIAN_POINT ( 'NONE',  ( -25.20123094555300369, 0.000000000000000000, 6.470945668149052032 ) ) ;
#41450=CARTESIAN_POINT ( 'NONE',  ( -18.67775241435682432, 0.000000000000000000, 4.136394454059623804 ) ) ;
#41451=CARTESIAN_POINT ( 'NONE',  ( -17.74560456716937296, 0.000000000000000000, 3.774316574337878372 ) ) ;
#41452=ORIENTED_EDGE ( 'NONE', *, *, #17932, .T. ) ;
#41453=EDGE_CURVE ( 'NONE', #29528, #1645, #25082, .T. ) ;
#41454=DIRECTION ( 'NONE',  ( -0.7660212471507179544, -0.6427876096865405842, -0.005961354470445141482 ) ) ;
#41455=VERTEX_POINT ( 'NONE', #4598 ) ;
#41456=EDGE_CURVE ( 'NONE', #12052, #23033, #34426, .T. ) ;
#41457=LINE ( 'NONE', #54769, #15811 ) ;
#41458=DIRECTION ( 'NONE',  ( -0.005002170337468016433, -0.7660444431189770143, 0.6427681459581293666 ) ) ;
#41459=EDGE_CURVE ( 'NONE', #3819, #26525, #39236, .T. ) ;
#41460=ORIENTED_EDGE ( 'NONE', *, *, #44499, .F. ) ;
#41461=VECTOR ( 'NONE', #673, 999.9999999999998863 ) ;
#41462=EDGE_LOOP ( 'NONE', ( #15389, #24045, #22211, #51136 ) ) ;
#41463=CARTESIAN_POINT ( 'NONE',  ( -9.945481425013914745, 0.000000000000000000, 2.727022726812396769 ) ) ;
#41464=VECTOR ( 'NONE', #30561, 1000.000000000000227 ) ;
#41465=ORIENTED_EDGE ( 'NONE', *, *, #41429, .F. ) ;
#41466=VERTEX_POINT ( 'NONE', #327 ) ;
#41467=VERTEX_POINT ( 'NONE', #3487 ) ;
#41468=DIRECTION ( 'NONE',  ( -0.5364919789714478471, 0.6444004775717705469, -0.5449076811759709926 ) ) ;
#41469=DIRECTION ( 'NONE',  ( 0.000000000000000000, -0.000000000000000000, -1.000000000000000000 ) ) ;
#41470=LINE ( 'NONE', #19305, #17581 ) ;
#41471=VECTOR ( 'NONE', #51265, 999.9999999999998863 ) ;
#41472=ORIENTED_EDGE ( 'NONE', *, *, #22760, .T. ) ;
#41473=ORIENTED_EDGE ( 'NONE', *, *, #54763, .T. ) ;
#41475=DIRECTION ( 'NONE',  ( 0.007781995580012663651, 0.000000000000000000, -0.9999697198139515519 ) ) ;
#41476=VERTEX_POINT ( 'NONE', #25925 ) ;
#41478=ORIENTED_EDGE ( 'NONE', *, *, #46989, .F. ) ;
#41479=PLANE ( 'NONE',  #16972 ) ;
#41480=DIRECTION ( 'NONE',  ( 0.007781995580012662783, 0.000000000000000000, -0.9999697198139514409 ) ) ;
#41481=ORIENTED_EDGE ( 'NONE', *, *, #46398, .F. ) ;
#41482=PLANE ( 'NONE',  #40930 ) ;
#41483=CARTESIAN_POINT ( 'NONE',  ( -17.46532115785441519, 0.000000000000000000, 13.67492996699914265 ) ) ;
#41484=ORIENTED_EDGE ( 'NONE', *, *, #5208, .F. ) ;
#41485=DIRECTION ( 'NONE',  ( -0.6427681459581293666, -0.7660444431189770143, -0.005002170337467561935 ) ) ;
#41486=LINE ( 'NONE', #16195, #6729 ) ;
#41487=LINE ( 'NONE', #15612, #44608 ) ;
#41488=VERTEX_POINT ( 'NONE', #51732 ) ;
#41489=EDGE_CURVE ( 'NONE', #1853, #6537, #38968, .T. ) ;
#41490=EDGE_CURVE ( 'NONE', #51521, #14570, #25349, .T. ) ;
#41491=CARTESIAN_POINT ( 'NONE',  ( -21.87999231953709867, -4.403642575758159872, 12.40799148664158125 ) ) ;
#41492=CARTESIAN_POINT ( 'NONE',  ( -25.20123094555300369, 0.000000000000000000, 6.470945668149052032 ) ) ;
#41493=CARTESIAN_POINT ( 'NONE',  ( -10.90481340813819600, 0.000000000000000000, 6.582203695148996836 ) ) ;
#41494=DIRECTION ( 'NONE',  ( 0.005961354470445682716, -0.6427876096865404731, -0.7660212471507180654 ) ) ;
#41495=ADVANCED_FACE ( 'NONE', ( #36 ), #17367, .F. ) ;
#41496=PLANE ( 'NONE',  #2255 ) ;
#41497=DIRECTION ( 'NONE',  ( -0.7660212471507179544, -0.6427876096865405842, -0.005961354470445141482 ) ) ;
#41498=VECTOR ( 'NONE', #16091, 999.9999999999998863 ) ;
#41499=DIRECTION ( 'NONE',  ( 0.9999697198139515519, 0.000000000000000000, 0.007781995580013368816 ) ) ;
#41500=ORIENTED_EDGE ( 'NONE', *, *, #47849, .F. ) ;
#41501=DIRECTION ( 'NONE',  ( -0.9999697198139514409, -0.000000000000000000, -0.007781995580013368816 ) ) ;
#41502=PLANE ( 'NONE',  #12345 ) ;
#41504=ORIENTED_EDGE ( 'NONE', *, *, #7641, .F. ) ;
#41505=CARTESIAN_POINT ( 'NONE',  ( -8.509919637592204822, -0.1191753592594197858, 10.23596830920056711 ) ) ;
#41506=CARTESIAN_POINT ( 'NONE',  ( -17.74834732018306482, 3.200641362704010451, 3.473875350394609374 ) ) ;
#41507=AXIS2_PLACEMENT_3D ( 'NONE', #22219, #17380, #9145 ) ;
#41508=CARTESIAN_POINT ( 'NONE',  ( -18.39746900504187010, 0.000000000000000000, 14.03700784672088808 ) ) ;
#41509=CARTESIAN_POINT ( 'NONE',  ( -12.70458494993575194, -0.1191753592594197858, 11.86531876794841978 ) ) ;
#41510=ADVANCED_FACE ( 'NONE', ( #44908 ), #14523, .F. ) ;
#41512=ORIENTED_EDGE ( 'NONE', *, *, #33013, .F. ) ;
#41513=ORIENTED_EDGE ( 'NONE', *, *, #50317, .F. ) ;
#41514=EDGE_CURVE ( 'NONE', #25391, #27823, #13672, .T. ) ;
#41516=CARTESIAN_POINT ( 'NONE',  ( -12.78178805287288178, 0.6102101463440037232, 2.847660476479313640 ) ) ;
#41517=EDGE_CURVE ( 'NONE', #14924, #3628, #31284, .T. ) ;
#41518=ORIENTED_EDGE ( 'NONE', *, *, #17610, .T. ) ;
#41519=PLANE ( 'NONE',  #26756 ) ;
#41521=ORIENTED_EDGE ( 'NONE', *, *, #15911, .F. ) ;
#41522=DIRECTION ( 'NONE',  ( 0.007781995580012662783, 0.000000000000000000, -0.9999697198139514409 ) ) ;
#41523=EDGE_CURVE ( 'NONE', #42201, #49088, #4883, .T. ) ;
#41524=VERTEX_POINT ( 'NONE', #17956 ) ;
#41525=ORIENTED_EDGE ( 'NONE', *, *, #25540, .F. ) ;
#41526=LINE ( 'NONE', #42370, #46470 ) ;
#41527=PLANE ( 'NONE',  #35053 ) ;
#41528=CARTESIAN_POINT ( 'NONE',  ( -22.40634380310664397, 0.000000000000000000, 5.584705972946605534 ) ) ;
#41529=EDGE_LOOP ( 'NONE', ( #36958, #50246, #50167, #22620 ) ) ;
#41533=ORIENTED_EDGE ( 'NONE', *, *, #3499, .T. ) ;
#41534=CARTESIAN_POINT ( 'NONE',  ( -27.99923088623136636, 0.000000000000000000, 7.757173251277078130 ) ) ;
#41535=ORIENTED_EDGE ( 'NONE', *, *, #24223, .T. ) ;
#41536=DIRECTION ( 'NONE',  ( 0.007781995580012663651, -3.146120232559066537E-19, -0.9999697198139514409 ) ) ;
#41537=ORIENTED_EDGE ( 'NONE', *, *, #9586, .T. ) ;
#41538=LINE ( 'NONE', #45493, #18601 ) ;
#41539=LINE ( 'NONE', #15984, #33151 ) ;
#41540=VECTOR ( 'NONE', #32754, 1000.000000000000114 ) ;
#41541=VERTEX_POINT ( 'NONE', #5186 ) ;
#41543=ORIENTED_EDGE ( 'NONE', *, *, #1643, .F. ) ;
#41544=DIRECTION ( 'NONE',  ( -0.9999697198139514409, -0.000000000000000000, -0.007781995580013368816 ) ) ;
#41545=LINE ( 'NONE', #40974, #33866 ) ;
#41546=CARTESIAN_POINT ( 'NONE',  ( -18.60807716309514959, 0.000000000000000000, 7.091593241429392513 ) ) ;
#41547=CARTESIAN_POINT ( 'NONE',  ( -20.43000850590469497, 4.172053068839010947, 4.484530505201751005 ) ) ;
#41548=DIRECTION ( 'NONE',  ( 0.6427681459581294776, -0.7660444431189769032, 0.005002170337467562802 ) ) ;
#41549=PLANE ( 'NONE',  #48213 ) ;
#41550=EDGE_LOOP ( 'NONE', ( #19662, #19314, #51308, #34726 ) ) ;
#41551=EDGE_CURVE ( 'NONE', #17246, #33621, #52849, .T. ) ;
#41552=ORIENTED_EDGE ( 'NONE', *, *, #5182, .F. ) ;
#41553=CARTESIAN_POINT ( 'NONE',  ( -29.86274838104827367, -0.1191753592594197858, 8.381332038739175871 ) ) ;
#41554=CARTESIAN_POINT ( 'NONE',  ( -15.86710544311044302, 0.000000000000000000, 13.13336954653252953 ) ) ;
#41555=EDGE_CURVE ( 'NONE', #12878, #14361, #30985, .T. ) ;
#41556=EDGE_CURVE ( 'NONE', #10765, #12832, #27034, .T. ) ;
#41557=LINE ( 'NONE', #33584, #32150 ) ;
#41558=DIRECTION ( 'NONE',  ( -0.5449076811759708816, 0.6444004775717707689, 0.5364919789714475140 ) ) ;
#41559=DIRECTION ( 'NONE',  ( -0.3620778797217457656, 0.000000000000000000, -0.9321478471874539151 ) ) ;
#41560=VERTEX_POINT ( 'NONE', #40073 ) ;
#41561=DIRECTION ( 'NONE',  ( -0.9999697198139514409, -0.000000000000000000, -0.007781995580013368816 ) ) ;
#41562=CARTESIAN_POINT ( 'NONE',  ( -13.07066190154808361, 0.000000000000000000, 12.04713590736729678 ) ) ;
#41563=ORIENTED_EDGE ( 'NONE', *, *, #8155, .T. ) ;
#41564=DIRECTION ( 'NONE',  ( 0.7660212471507180654, -0.6427876096865404731, 0.005961354470445141482 ) ) ;
#41565=DIRECTION ( 'NONE',  ( 0.005961354470445682716, -0.6427876096865404731, -0.7660212471507180654 ) ) ;
#41566=EDGE_LOOP ( 'NONE', ( #8822, #31388, #55090, #55570 ) ) ;
#41568=CARTESIAN_POINT ( 'NONE',  ( -13.73672976910459909, 0.000000000000000000, 12.22661844811216270 ) ) ;
#41569=CARTESIAN_POINT ( 'NONE',  ( -19.81657051840181794, -0.3560938001956556742, 4.567388823514338725 ) ) ;
#41570=LINE ( 'NONE', #11481, #28709 ) ;
#41571=CARTESIAN_POINT ( 'NONE',  ( -18.67697421479882181, -0.1191753592594197858, 4.036397482078229793 ) ) ;
#41572=ORIENTED_EDGE ( 'NONE', *, *, #11645, .T. ) ;
#41573=ORIENTED_EDGE ( 'NONE', *, *, #18813, .T. ) ;
#41574=CARTESIAN_POINT ( 'NONE',  ( -14.17319835266821393, 0.000000000000000000, 8.603434773024542181 ) ) ;
#41575=LINE ( 'NONE', #55461, #21339 ) ;
#41576=CARTESIAN_POINT ( 'NONE',  ( -15.03495456790438389, -0.1191753592594197858, 12.77051346725278158 ) ) ;
#41577=DIRECTION ( 'NONE',  ( 0.9999697198139515519, 0.000000000000000000, 0.007781995580013368816 ) ) ;
#41579=PLANE ( 'NONE',  #26499 ) ;
#41580=CARTESIAN_POINT ( 'NONE',  ( -13.20239044008653195, 2.229229656569007734, 1.739064436143978432 ) ) ;
#41581=ORIENTED_EDGE ( 'NONE', *, *, #39309, .F. ) ;
#41582=DIRECTION ( 'NONE',  ( 0.005002170337468016433, -0.7660444431189770143, -0.6427681459581293666 ) ) ;
#41583=ADVANCED_FACE ( 'NONE', ( #36375 ), #6027, .F. ) ;
#41584=CARTESIAN_POINT ( 'NONE',  ( -27.99767448711536133, 0.000000000000000000, 7.557179307314289218 ) ) ;
#41585=DIRECTION ( 'NONE',  ( -0.005002170337468016433, -0.7660444431189770143, 0.6427681459581293666 ) ) ;
#41586=ORIENTED_EDGE ( 'NONE', *, *, #13030, .T. ) ;
#41587=EDGE_CURVE ( 'NONE', #50902, #53298, #5723, .T. ) ;
#41589=CARTESIAN_POINT ( 'NONE',  ( -19.45503627000849889, -1.000000000000000000, 7.556996783084074742 ) ) ;
#41590=LINE ( 'NONE', #27991, #32984 ) ;
#41591=ORIENTED_EDGE ( 'NONE', *, *, #11075, .F. ) ;
#41592=DIRECTION ( 'NONE',  ( -0.5449076811759708816, 0.6444004775717707689, 0.5364919789714475140 ) ) ;
#41593=EDGE_CURVE ( 'NONE', #45628, #1080, #53427, .T. ) ;
#41594=EDGE_LOOP ( 'NONE', ( #50177, #15857, #3609, #15731 ) ) ;
#41595=ORIENTED_EDGE ( 'NONE', *, *, #9736, .T. ) ;
#41596=EDGE_LOOP ( 'NONE', ( #46390, #4330, #16491, #35331 ) ) ;
#41597=ORIENTED_EDGE ( 'NONE', *, *, #21404, .T. ) ;
#41598=ORIENTED_EDGE ( 'NONE', *, *, #19929, .F. ) ;
#41599=CARTESIAN_POINT ( 'NONE',  ( -22.40556560354864146, -0.1191753592594197858, 5.484709000965211523 ) ) ;
#41600=VERTEX_POINT ( 'NONE', #48304 ) ;
#41601=ORIENTED_EDGE ( 'NONE', *, *, #55949, .F. ) ;
#41602=CARTESIAN_POINT ( 'NONE',  ( -16.96273579891908412, -0.8417996532631562001, 3.443365942170054428 ) ) ;
#41603=ORIENTED_EDGE ( 'NONE', *, *, #15121, .F. ) ;
#41604=ORIENTED_EDGE ( 'NONE', *, *, #38711, .T. ) ;
#41605=EDGE_CURVE ( 'NONE', #6097, #4731, #53163, .T. ) ;
#41606=DIRECTION ( 'NONE',  ( 0.007781995580012663651, -3.146120232559066537E-19, -0.9999697198139514409 ) ) ;
#41607=PLANE ( 'NONE',  #28505 ) ;
#41608=FACE_OUTER_BOUND ( 'NONE', #47802, .T. ) ;
#41609=CARTESIAN_POINT ( 'NONE',  ( -8.837649716295214120, 0.000000000000000000, 5.490294631563745753 ) ) ;
#41610=EDGE_CURVE ( 'NONE', #19103, #7637, #22500, .T. ) ;
#41611=FACE_OUTER_BOUND ( 'NONE', #1746, .T. ) ;
#41612=VERTEX_POINT ( 'NONE', #26446 ) ;
#41613=ORIENTED_EDGE ( 'NONE', *, *, #37233, .F. ) ;
#41614=EDGE_CURVE ( 'NONE', #13117, #41065, #22208, .T. ) ;
#41615=DIRECTION ( 'NONE',  ( 0.007781995580012662783, 0.000000000000000000, -0.9999697198139514409 ) ) ;
#41616=PLANE ( 'NONE',  #54771 ) ;
#41617=EDGE_CURVE ( 'NONE', #37343, #42852, #26742, .T. ) ;
#41618=PLANE ( 'NONE',  #52377 ) ;
#41619=LINE ( 'NONE', #49860, #28659 ) ;
#41620=LINE ( 'NONE', #24567, #7706 ) ;
#41621=FACE_OUTER_BOUND ( 'NONE', #9320, .T. ) ;
#41622=ORIENTED_EDGE ( 'NONE', *, *, #14012, .T. ) ;
#41623=CARTESIAN_POINT ( 'NONE',  ( -17.89379923316518273, 2.229229656569005957, 7.490426063039901550 ) ) ;
#41624=ORIENTED_EDGE ( 'NONE', *, *, #46929, .F. ) ;
#41625=PLANE ( 'NONE',  #41932 ) ;
#41626=DIRECTION ( 'NONE',  ( -0.5449076811759708816, 0.6444004775717707689, 0.5364919789714475140 ) ) ;
#41627=LINE ( 'NONE', #2708, #12747 ) ;
#41628=LINE ( 'NONE', #7018, #22258 ) ;
#41629=CARTESIAN_POINT ( 'NONE',  ( -17.26082817053895724, 2.067327705546508021, 3.320664995664557750 ) ) ;
#41630=ADVANCED_FACE ( 'NONE', ( #14803 ), #48890, .F. ) ;
#41631=ORIENTED_EDGE ( 'NONE', *, *, #32964, .F. ) ;
#41632=DIRECTION ( 'NONE',  ( 0.5364919789714477361, 0.6444004775717706579, 0.5449076811759711036 ) ) ;
#41633=FACE_OUTER_BOUND ( 'NONE', #34838, .T. ) ;
#41634=PLANE ( 'NONE',  #20633 ) ;
#41635=DIRECTION ( 'NONE',  ( 0.5449076811759707706, 0.6444004775717708799, -0.5364919789714476250 ) ) ;
#41636=DIRECTION ( 'NONE',  ( 0.5449076811759707706, 0.6444004775717708799, -0.5364919789714476250 ) ) ;
#41637=DIRECTION ( 'NONE',  ( 0.007781995580012663651, 0.000000000000000000, -0.9999697198139515519 ) ) ;
#41638=DIRECTION ( 'NONE',  ( -0.5449076811759708816, 0.6444004775717707689, 0.5364919789714475140 ) ) ;
#41639=DIRECTION ( 'NONE',  ( 0.5364919789714477361, 0.6444004775717706579, 0.5449076811759711036 ) ) ;
#41640=CARTESIAN_POINT ( 'NONE',  ( -9.029021499742155399, 0.000000000000000000, 4.380809122674449441 ) ) ;
#41642=ORIENTED_EDGE ( 'NONE', *, *, #46255, .F. ) ;
#41643=EDGE_CURVE ( 'NONE', #25831, #53959, #49149, .T. ) ;
#41644=VERTEX_POINT ( 'NONE', #53685 ) ;
#41645=ORIENTED_EDGE ( 'NONE', *, *, #25874, .T. ) ;
#41646=VERTEX_POINT ( 'NONE', #43768 ) ;
#41647=VERTEX_POINT ( 'NONE', #52576 ) ;
#41648=FACE_OUTER_BOUND ( 'NONE', #34798, .T. ) ;
#41649=LINE ( 'NONE', #20062, #16585 ) ;
#41650=CARTESIAN_POINT ( 'NONE',  ( -25.20278734466900517, 0.000000000000000000, 6.670939612111840944 ) ) ;
#41651=EDGE_CURVE ( 'NONE', #41524, #21438, #9418, .T. ) ;
#41652=ORIENTED_EDGE ( 'NONE', *, *, #42512, .F. ) ;
#41653=ORIENTED_EDGE ( 'NONE', *, *, #46297, .T. ) ;
#41654=ORIENTED_EDGE ( 'NONE', *, *, #39709, .T. ) ;
#41656=EDGE_CURVE ( 'NONE', #41786, #14819, #54511, .T. ) ;
#41657=VERTEX_POINT ( 'NONE', #32954 ) ;
#41658=EDGE_CURVE ( 'NONE', #16476, #50946, #41196, .T. ) ;
#41660=DIRECTION ( 'NONE',  ( 0.007781995580012663651, -3.146120232559066537E-19, -0.9999697198139514409 ) ) ;
#41661=CARTESIAN_POINT ( 'NONE',  ( -15.59709573620632383, 5.629170628041512359, 2.560773380055879844 ) ) ;
#41662=EDGE_CURVE ( 'NONE', #44744, #30955, #1989, .T. ) ;
#41663=VERTEX_POINT ( 'NONE', #33258 ) ;
#41664=CARTESIAN_POINT ( 'NONE',  ( -19.75917934048144531, -0.8417996532631562001, 4.529599581335290281 ) ) ;
#41665=ORIENTED_EDGE ( 'NONE', *, *, #40253, .T. ) ;
#41666=LINE ( 'NONE', #11844, #14636 ) ;
#41667=EDGE_CURVE ( 'NONE', #2799, #43546, #41486, .T. ) ;
#41668=LINE ( 'NONE', #19823, #33911 ) ;
#41669=EDGE_CURVE ( 'NONE', #39352, #46530, #2569, .T. ) ;
#41670=DIRECTION ( 'NONE',  ( 0.9999697198139515519, 0.000000000000000000, 0.007781995580013368816 ) ) ;
#41671=CARTESIAN_POINT ( 'NONE',  ( -13.44920839603113905, -1.651309408375657206, 2.052764979558574510 ) ) ;
#41673=CARTESIAN_POINT ( 'NONE',  ( -11.74061653640753455, -0.1191753592594181482, 7.414366449667899595 ) ) ;
#41674=DIRECTION ( 'NONE',  ( 0.9321478471874540261, 0.000000000000000000, -0.3620778797217457101 ) ) ;
#41675=PLANE ( 'NONE',  #33915 ) ;
#41676=CARTESIAN_POINT ( 'NONE',  ( -14.46888367232926420, 0.000000000000000000, 12.59025272694991315 ) ) ;
#41677=ORIENTED_EDGE ( 'NONE', *, *, #24596, .T. ) ;
#41678=DIRECTION ( 'NONE',  ( -0.5364919789714478471, 0.6444004775717705469, -0.5449076811759709926 ) ) ;
#41679=VERTEX_POINT ( 'NONE', #40911 ) ;
#41680=EDGE_CURVE ( 'NONE', #47084, #12623, #7381, .T. ) ;
#41682=LINE ( 'NONE', #20091, #43220 ) ;
#41683=DIRECTION ( 'NONE',  ( -0.5449076811759708816, 0.6444004775717707689, 0.5364919789714475140 ) ) ;
#41684=DIRECTION ( 'NONE',  ( 0.5364919789714477361, 0.6444004775717706579, 0.5449076811759711036 ) ) ;
#41685=DIRECTION ( 'NONE',  ( 0.6427681459581294776, -0.7660444431189769032, 0.005002170337467562802 ) ) ;
#41686=EDGE_CURVE ( 'NONE', #30915, #31264, #50565, .T. ) ;
#41687=DIRECTION ( 'NONE',  ( -0.9999697198139514409, -0.000000000000000000, -0.007781995580013368816 ) ) ;
#41688=ORIENTED_EDGE ( 'NONE', *, *, #49333, .T. ) ;
#41689=CARTESIAN_POINT ( 'NONE',  ( -15.53836850813863890, 0.000000000000000000, 4.899490005142868476 ) ) ;
#41690=FACE_OUTER_BOUND ( 'NONE', #42713, .T. ) ;
#41691=DIRECTION ( 'NONE',  ( 0.005961354470445682716, -0.6427876096865404731, -0.7660212471507180654 ) ) ;
#41692=CARTESIAN_POINT ( 'NONE',  ( -13.27065584551087163, 0.000000000000000000, 12.04557950825129176 ) ) ;
#41693=FACE_OUTER_BOUND ( 'NONE', #27756, .T. ) ;
#41694=DIRECTION ( 'NONE',  ( -0.005002170337468016433, -0.7660444431189770143, 0.6427681459581293666 ) ) ;
#41695=CARTESIAN_POINT ( 'NONE',  ( -11.61265722893131525, 0.000000000000000000, 3.822044588629654349 ) ) ;
#41696=LINE ( 'NONE', #33214, #9709 ) ;
#41697=DIRECTION ( 'NONE',  ( 0.007781995580012663651, 0.000000000000000000, -0.9999697198139515519 ) ) ;
#41698=VERTEX_POINT ( 'NONE', #49449 ) ;
#41699=CARTESIAN_POINT ( 'NONE',  ( -19.32961685222932147, 0.000000000000000000, 14.39908572644263351 ) ) ;
#41700=ORIENTED_EDGE ( 'NONE', *, *, #49426, .F. ) ;
#41701=FACE_OUTER_BOUND ( 'NONE', #24278, .T. ) ;
#41704=EDGE_LOOP ( 'NONE', ( #44965, #34397, #10847, #4881 ) ) ;
#41705=ADVANCED_FACE ( 'NONE', ( #54258 ), #28131, .F. ) ;
#41706=ORIENTED_EDGE ( 'NONE', *, *, #21748, .T. ) ;
#41707=DIRECTION ( 'NONE',  ( 0.9999697198139515519, 0.000000000000000000, 0.007781995580013368816 ) ) ;
#41708=AXIS2_PLACEMENT_3D ( 'NONE', #48479, #2158, #6444 ) ;
#41709=EDGE_LOOP ( 'NONE', ( #45695, #6493, #51705, #17028 ) ) ;
#41710=ORIENTED_EDGE ( 'NONE', *, *, #25278, .T. ) ;
#41711=VERTEX_POINT ( 'NONE', #32668 ) ;
#41712=DIRECTION ( 'NONE',  ( 0.6246952433987893460, 0.7422098413412802076, -0.2426528472758539279 ) ) ;
#41713=LINE ( 'NONE', #3403, #27832 ) ;
#41714=LINE ( 'NONE', #3948, #14019 ) ;
#41715=EDGE_CURVE ( 'NONE', #5277, #32587, #20457, .T. ) ;
#41716=ADVANCED_FACE ( 'NONE', ( #11080 ), #28409, .F. ) ;
#41717=EDGE_LOOP ( 'NONE', ( #45741, #48966, #23695, #35531 ) ) ;
#41718=ORIENTED_EDGE ( 'NONE', *, *, #21867, .F. ) ;
#41719=EDGE_CURVE ( 'NONE', #34036, #2679, #7127, .T. ) ;
#41720=CARTESIAN_POINT ( 'NONE',  ( 2.072287782118878319, 0.000000000000000000, -2.950529333540147015 ) ) ;
#41722=ORIENTED_EDGE ( 'NONE', *, *, #40180, .F. ) ;
#41723=CARTESIAN_POINT ( 'NONE',  ( -17.93139508144814442, 0.000000000000000000, 13.85596890686001537 ) ) ;
#41724=ORIENTED_EDGE ( 'NONE', *, *, #34681, .F. ) ;
#41725=DIRECTION ( 'NONE',  ( -0.005002170337468016433, -0.7660444431189770143, 0.6427681459581293666 ) ) ;
#41726=DIRECTION ( 'NONE',  ( -0.6427681459581293666, -0.7660444431189770143, -0.005002170337467561935 ) ) ;
#41727=ORIENTED_EDGE ( 'NONE', *, *, #35222, .F. ) ;
#41728=DIRECTION ( 'NONE',  ( -0.5449076811759708816, 0.6444004775717707689, 0.5364919789714475140 ) ) ;
#41729=EDGE_CURVE ( 'NONE', #12359, #2867, #6553, .T. ) ;
#41730=ADVANCED_FACE ( 'NONE', ( #38907 ), #17049, .F. ) ;
#41731=DIRECTION ( 'NONE',  ( 0.5449076811759707706, 0.6444004775717708799, -0.5364919789714476250 ) ) ;
#41732=ORIENTED_EDGE ( 'NONE', *, *, #41234, .F. ) ;
#41733=DIRECTION ( 'NONE',  ( 0.000000000000000000, -0.000000000000000000, -1.000000000000000000 ) ) ;
#41734=CARTESIAN_POINT ( 'NONE',  ( -13.64977165607341192, -5.213152330870665097, 2.017029123393386580 ) ) ;
#41735=EDGE_CURVE ( 'NONE', #37427, #14766, #29556, .T. ) ;
#41736=DIRECTION ( 'NONE',  ( 0.9999697198139515519, 0.000000000000000000, 0.007781995580013368816 ) ) ;
#41737=EDGE_LOOP ( 'NONE', ( #10357, #44761, #49944, #48205 ) ) ;
#41738=EDGE_CURVE ( 'NONE', #4032, #17566, #51939, .T. ) ;
#41739=CARTESIAN_POINT ( 'NONE',  ( -10.27421835998572064, 0.000000000000000000, 10.96090226820206048 ) ) ;
#41740=DIRECTION ( 'NONE',  ( 0.005961354470445682716, -0.6427876096865404731, -0.7660212471507180654 ) ) ;
#41741=DIRECTION ( 'NONE',  ( 0.007781995580012663651, -3.146120232559066537E-19, -0.9999697198139514409 ) ) ;
#41742=CARTESIAN_POINT ( 'NONE',  ( -8.887694952903760992, -0.1191753592594182315, 4.112579916844113725 ) ) ;
#41743=LINE ( 'NONE', #28416, #33123 ) ;
#41744=CARTESIAN_POINT ( 'NONE',  ( -19.77953895519367933, 4.981562823951511731, 12.73995903822415876 ) ) ;
#41745=AXIS2_PLACEMENT_3D ( 'NONE', #53109, #22155, #38925 ) ;
#41746=PLANE ( 'NONE',  #12227 ) ;
#41747=ORIENTED_EDGE ( 'NONE', *, *, #46152, .T. ) ;
#41748=PLANE ( 'NONE',  #15348 ) ;
#41751=ORIENTED_EDGE ( 'NONE', *, *, #15202, .F. ) ;
#41752=DIRECTION ( 'NONE',  ( -0.005961354470445682716, -0.6427876096865404731, 0.7660212471507180654 ) ) ;
#41754=CARTESIAN_POINT ( 'NONE',  ( -26.13415699229845757, -0.1191753592594197858, 6.933020519852192365 ) ) ;
#41755=PLANE ( 'NONE',  #37830 ) ;
#41756=CARTESIAN_POINT ( 'NONE',  ( -12.48602183387798803, -2.137015261443155900, 5.039132754124569402 ) ) ;
#41757=VERTEX_POINT ( 'NONE', #13062 ) ;
#41758=ORIENTED_EDGE ( 'NONE', *, *, #19119, .F. ) ;
#41759=FACE_OUTER_BOUND ( 'NONE', #42961, .T. ) ;
#41760=EDGE_CURVE ( 'NONE', #54483, #8121, #42864, .T. ) ;
#41761=FACE_OUTER_BOUND ( 'NONE', #5294, .T. ) ;
#41762=CARTESIAN_POINT ( 'NONE',  ( -15.59967562208883329, 3.362543313726507499, 8.459271331385316728 ) ) ;
#41763=AXIS2_PLACEMENT_3D ( 'NONE', #51088, #28964, #50806 ) ;
#41764=ORIENTED_EDGE ( 'NONE', *, *, #48779, .T. ) ;
#41765=DIRECTION ( 'NONE',  ( 0.007781995580012663651, 0.000000000000000000, -0.9999697198139515519 ) ) ;
#41767=ORIENTED_EDGE ( 'NONE', *, *, #33640, .T. ) ;
#41768=PLANE ( 'NONE',  #43800 ) ;
#41769=EDGE_CURVE ( 'NONE', #30649, #41455, #30387, .T. ) ;
#41770=VERTEX_POINT ( 'NONE', #55652 ) ;
#41771=EDGE_LOOP ( 'NONE', ( #22484, #43153, #51843, #10064, #28196 ) ) ;
#41772=EDGE_CURVE ( 'NONE', #44308, #30922, #34364, .T. ) ;
#41773=DIRECTION ( 'NONE',  ( -0.3620778797217457101, 0.000000000000000000, -0.9321478471874540261 ) ) ;
#41774=DIRECTION ( 'NONE',  ( -0.9999697198139514409, -0.000000000000000000, -0.007781995580013368816 ) ) ;
#41775=FACE_OUTER_BOUND ( 'NONE', #28889, .T. ) ;
#41776=ADVANCED_FACE ( 'NONE', ( #25548 ), #30094, .F. ) ;
#41777=EDGE_CURVE ( 'NONE', #55993, #42993, #39166, .T. ) ;
#41778=EDGE_CURVE ( 'NONE', #2289, #37965, #46563, .T. ) ;
#41779=ORIENTED_EDGE ( 'NONE', *, *, #42688, .F. ) ;
#41780=VECTOR ( 'NONE', #9980, 1000.000000000000227 ) ;
#41781=DIRECTION ( 'NONE',  ( 0.5449076811759707706, 0.6444004775717708799, -0.5364919789714476250 ) ) ;
#41783=EDGE_CURVE ( 'NONE', #35736, #2493, #42591, .T. ) ;
#41784=AXIS2_PLACEMENT_3D ( 'NONE', #49626, #28035, #27465 ) ;
#41785=EDGE_LOOP ( 'NONE', ( #42087, #39098, #23570, #9961 ) ) ;
#41786=VERTEX_POINT ( 'NONE', #21843 ) ;
#41788=CARTESIAN_POINT ( 'NONE',  ( -18.19747506107908563, 0.000000000000000000, 14.03856424583689311 ) ) ;
#41789=ORIENTED_EDGE ( 'NONE', *, *, #34113, .F. ) ;
#41790=LINE ( 'NONE', #42079, #2149 ) ;
#41791=ORIENTED_EDGE ( 'NONE', *, *, #34153, .F. ) ;
#41792=LINE ( 'NONE', #24225, #14067 ) ;
#41793=LINE ( 'NONE', #2885, #524 ) ;
#41794=ORIENTED_EDGE ( 'NONE', *, *, #54485, .F. ) ;
#41795=LINE ( 'NONE', #20217, #4136 ) ;
#41796=ORIENTED_EDGE ( 'NONE', *, *, #18039, .T. ) ;
#41797=EDGE_CURVE ( 'NONE', #44507, #15829, #3972, .T. ) ;
#41798=EDGE_CURVE ( 'NONE', #48603, #41838, #16755, .T. ) ;
#41799=LINE ( 'NONE', #2892, #27368 ) ;
#41800=DIRECTION ( 'NONE',  ( 0.005961354470445682716, -0.6427876096865404731, -0.7660212471507180654 ) ) ;
#41801=DIRECTION ( 'NONE',  ( -0.9999697198139514409, -0.000000000000000000, -0.007781995580013368816 ) ) ;
#41802=CARTESIAN_POINT ( 'NONE',  ( -29.86197018149027116, 0.000000000000000000, 8.281335066757780083 ) ) ;
#41803=EDGE_CURVE ( 'NONE', #28180, #37125, #21296, .T. ) ;
#41804=DIRECTION ( 'NONE',  ( -0.5364919789714478471, 0.6444004775717705469, -0.5449076811759709926 ) ) ;
#41805=LINE ( 'NONE', #51481, #7401 ) ;
#41806=ORIENTED_EDGE ( 'NONE', *, *, #17300, .F. ) ;
#41807=AXIS2_PLACEMENT_3D ( 'NONE', #45679, #9947, #27251 ) ;
#41808=ADVANCED_FACE ( 'NONE', ( #50818 ), #11918, .F. ) ;
#41809=VERTEX_POINT ( 'NONE', #8520 ) ;
#41810=AXIS2_PLACEMENT_3D ( 'NONE', #38617, #243, #4273 ) ;
#41811=FACE_OUTER_BOUND ( 'NONE', #25864, .T. ) ;
#41812=PLANE ( 'NONE',  #23928 ) ;
#41813=DIRECTION ( 'NONE',  ( 0.007781995580012663651, 0.000000000000000000, -0.9999697198139515519 ) ) ;
#41814=CARTESIAN_POINT ( 'NONE',  ( -14.54259203834542902, -0.1159828484229813300, 8.867210191861607527 ) ) ;
#41815=EDGE_CURVE ( 'NONE', #17943, #33865, #33787, .T. ) ;
#41816=CARTESIAN_POINT ( 'NONE',  ( -15.98433325582929498, 4.981562823951513508, 2.731851662868523434 ) ) ;
#41817=CARTESIAN_POINT ( 'NONE',  ( -14.94916102560700821, 0.000000000000000000, 2.688082935172642962 ) ) ;
#41818=VERTEX_POINT ( 'NONE', #4281 ) ;
#41819=LINE ( 'NONE', #37876, #4154 ) ;
#41820=LINE ( 'NONE', #54335, #552 ) ;
#41822=CARTESIAN_POINT ( 'NONE',  ( -19.27558205740430353, 0.000000000000000000, 7.455730633803142382 ) ) ;
#41823=DIRECTION ( 'NONE',  ( -0.5449076811759708816, 0.6444004775717707689, 0.5364919789714475140 ) ) ;
#41824=ORIENTED_EDGE ( 'NONE', *, *, #24220, .F. ) ;
#41825=DIRECTION ( 'NONE',  ( 0.005002170337468016433, -0.7660444431189770143, -0.6427681459581293666 ) ) ;
#41828=FACE_OUTER_BOUND ( 'NONE', #49779, .T. ) ;
#41829=LINE ( 'NONE', #23965, #20146 ) ;
#41830=VERTEX_POINT ( 'NONE', #12512 ) ;
#41831=VERTEX_POINT ( 'NONE', #46870 ) ;
#41832=DIRECTION ( 'NONE',  ( 0.007781995580012663651, -3.146120232559066537E-19, -0.9999697198139514409 ) ) ;
#41833=PLANE ( 'NONE',  #38568 ) ;
#41834=CARTESIAN_POINT ( 'NONE',  ( -17.84862895020420481, 4.981562823951512620, 3.456007422312016519 ) ) ;
#41835=FACE_OUTER_BOUND ( 'NONE', #13195, .T. ) ;
#41836=LINE ( 'NONE', #11191, #36431 ) ;
#41837=CARTESIAN_POINT ( 'NONE',  ( -20.54204810873173415, 0.000000000000000000, 4.860550213503115558 ) ) ;
#41838=VERTEX_POINT ( 'NONE', #29830 ) ;
#41841=CARTESIAN_POINT ( 'NONE',  ( -13.70125694970055541, 0.000000000000000000, 7.668437334314234022 ) ) ;
#41842=DIRECTION ( 'NONE',  ( 0.007781995580012662783, 0.000000000000000000, -0.9999697198139514409 ) ) ;
#41843=ORIENTED_EDGE ( 'NONE', *, *, #38025, .T. ) ;
#41845=CARTESIAN_POINT ( 'NONE',  ( -15.86710544311044302, 0.000000000000000000, 13.13336954653252953 ) ) ;
#41846=DIRECTION ( 'NONE',  ( 0.007781995580012663651, -3.146120232559066537E-19, -0.9999697198139514409 ) ) ;
#41847=EDGE_CURVE ( 'NONE', #12635, #17790, #47130, .T. ) ;
#41848=EDGE_CURVE ( 'NONE', #55458, #22074, #22691, .T. ) ;
#41849=EDGE_LOOP ( 'NONE', ( #28004, #20180, #37267, #45931 ) ) ;
#41850=VECTOR ( 'NONE', #35957, 999.9999999999998863 ) ;
#41851=AXIS2_PLACEMENT_3D ( 'NONE', #54322, #14874, #45507 ) ;
#41852=DIRECTION ( 'NONE',  ( -0.9999697198139514409, -0.000000000000000000, -0.007781995580013368816 ) ) ;
#41853=ORIENTED_EDGE ( 'NONE', *, *, #41456, .T. ) ;
#41854=ADVANCED_FACE ( 'NONE', ( #10187 ), #39750, .F. ) ;
#41855=ORIENTED_EDGE ( 'NONE', *, *, #22904, .T. ) ;
#41856=ORIENTED_EDGE ( 'NONE', *, *, #52056, .F. ) ;
#41857=ORIENTED_EDGE ( 'NONE', *, *, #13209, .T. ) ;
#41858=VECTOR ( 'NONE', #43596, 999.9999999999998863 ) ;
#41859=ORIENTED_EDGE ( 'NONE', *, *, #4635, .T. ) ;
#41860=LINE ( 'NONE', #38169, #55617 ) ;
#41861=ORIENTED_EDGE ( 'NONE', *, *, #1932, .F. ) ;
#41862=ORIENTED_EDGE ( 'NONE', *, *, #31751, .T. ) ;
#41863=CARTESIAN_POINT ( 'NONE',  ( -30.79411802867772607, 0.000000000000000000, 8.643412946479525516 ) ) ;
#41864=ORIENTED_EDGE ( 'NONE', *, *, #46237, .T. ) ;
#41865=VECTOR ( 'NONE', #52238, 999.9999999999998863 ) ;
#41866=ORIENTED_EDGE ( 'NONE', *, *, #1932, .T. ) ;
#41867=VECTOR ( 'NONE', #41660, 1000.000000000000227 ) ;
#41868=CARTESIAN_POINT ( 'NONE',  ( -12.13851405436063047, 0.000000000000000000, 11.68505802764555135 ) ) ;
#41869=CARTESIAN_POINT ( 'NONE',  ( -22.25877225010755822, -3.756034771668159689, 11.49228773929388581 ) ) ;
#41871=PLANE ( 'NONE',  #52253 ) ;
#41872=CARTESIAN_POINT ( 'NONE',  ( -23.33771345073609638, -0.1191753592594197858, 5.846786880686956955 ) ) ;
#41873=ORIENTED_EDGE ( 'NONE', *, *, #7725, .T. ) ;
#41874=VERTEX_POINT ( 'NONE', #48234 ) ;
#41875=DIRECTION ( 'NONE',  ( 0.007781995580012662783, 0.000000000000000000, -0.9999697198139514409 ) ) ;
#41876=DIRECTION ( 'NONE',  ( -0.005002170337468016433, -0.7660444431189770143, 0.6427681459581293666 ) ) ;
#41879=CARTESIAN_POINT ( 'NONE',  ( -16.81345671998191449, 0.000000000000000000, 3.412238694616132495 ) ) ;
#41880=EDGE_CURVE ( 'NONE', #30486, #16959, #13356, .T. ) ;
#41881=CARTESIAN_POINT ( 'NONE',  ( -13.68688668217414239, 0.000000000000000000, 5.821888818025412249 ) ) ;
#41882=CARTESIAN_POINT ( 'NONE',  ( -20.54204810873173415, 0.000000000000000000, 4.860550213503115558 ) ) ;
#41883=EDGE_LOOP ( 'NONE', ( #2480, #50043, #28002, #16877 ) ) ;
#41884=FACE_OUTER_BOUND ( 'NONE', #51548, .T. ) ;
#41885=EDGE_CURVE ( 'NONE', #39979, #49529, #40005, .T. ) ;
#41886=ORIENTED_EDGE ( 'NONE', *, *, #37050, .F. ) ;
#41887=VECTOR ( 'NONE', #7348, 999.9999999999998863 ) ;
#41888=AXIS2_PLACEMENT_3D ( 'NONE', #1930, #32059, #15026 ) ;
#41890=LINE ( 'NONE', #52, #34741 ) ;
#41891=FACE_OUTER_BOUND ( 'NONE', #25475, .T. ) ;
#41892=FACE_OUTER_BOUND ( 'NONE', #14574, .T. ) ;
#41893=ADVANCED_FACE ( 'NONE', ( #53083 ), #27510, .F. ) ;
#41894=CARTESIAN_POINT ( 'NONE',  ( -27.99923088623136636, 0.000000000000000000, 7.757173251277078130 ) ) ;
#41895=DIRECTION ( 'NONE',  ( -0.9999697198139514409, -0.000000000000000000, -0.007781995580013368816 ) ) ;
#41896=EDGE_LOOP ( 'NONE', ( #35022, #32647, #51605, #6609 ) ) ;
#41897=AXIS2_PLACEMENT_3D ( 'NONE', #16761, #51112, #30392 ) ;
#41898=ORIENTED_EDGE ( 'NONE', *, *, #13718, .F. ) ;
#41900=CARTESIAN_POINT ( 'NONE',  ( -10.27421835998572064, 0.000000000000000000, 10.96090226820206048 ) ) ;
#41902=DIRECTION ( 'NONE',  ( 0.000000000000000000, -1.000000000000000000, 0.000000000000000000 ) ) ;
#41903=VECTOR ( 'NONE', #46145, 1000.000000000000114 ) ;
#41904=DIRECTION ( 'NONE',  ( 0.9999697198139515519, 0.000000000000000000, 0.007781995580013368816 ) ) ;
#41905=CARTESIAN_POINT ( 'NONE',  ( -16.33317936670417225, 0.000000000000000000, 13.31440848639340224 ) ) ;
#41906=PLANE ( 'NONE',  #11085 ) ;
#41907=PLANE ( 'NONE',  #8802 ) ;
#41908=DIRECTION ( 'NONE',  ( 0.9999697198139515519, 0.000000000000000000, 0.007781995580013368816 ) ) ;
#41909=EDGE_CURVE ( 'NONE', #15326, #44124, #43695, .T. ) ;
#41910=EDGE_CURVE ( 'NONE', #41600, #36024, #30925, .T. ) ;
#41911=ORIENTED_EDGE ( 'NONE', *, *, #43531, .F. ) ;
#41912=VECTOR ( 'NONE', #27243, 1000.000000000000227 ) ;
#41913=EDGE_CURVE ( 'NONE', #1495, #3681, #9657, .T. ) ;
#41914=ADVANCED_FACE ( 'NONE', ( #44538 ), #22136, .F. ) ;
#41915=EDGE_LOOP ( 'NONE', ( #37274, #54059, #44149, #2605 ) ) ;
#41916=ORIENTED_EDGE ( 'NONE', *, *, #6839, .T. ) ;
#41917=ORIENTED_EDGE ( 'NONE', *, *, #3593, .F. ) ;
#41918=VERTEX_POINT ( 'NONE', #9076 ) ;
#41919=AXIS2_PLACEMENT_3D ( 'NONE', #8926, #31027, #22793 ) ;
#41920=CARTESIAN_POINT ( 'NONE',  ( -11.27310558606116686, -0.1191753592594168437, 7.048672658178141148 ) ) ;
#41922=DIRECTION ( 'NONE',  ( 0.6246952433987893460, 0.7422098413412802076, -0.2426528472758539279 ) ) ;
#41923=AXIS2_PLACEMENT_3D ( 'NONE', #29738, #51296, #3584 ) ;
#41924=VECTOR ( 'NONE', #12999, 1000.000000000000114 ) ;
#41925=ORIENTED_EDGE ( 'NONE', *, *, #30978, .F. ) ;
#41926=VERTEX_POINT ( 'NONE', #48828 ) ;
#41927=ORIENTED_EDGE ( 'NONE', *, *, #24751, .T. ) ;
#41928=FACE_OUTER_BOUND ( 'NONE', #50857, .T. ) ;
#41929=ORIENTED_EDGE ( 'NONE', *, *, #29606, .F. ) ;
#41930=ADVANCED_FACE ( 'NONE', ( #36063 ), #17595, .F. ) ;
#41931=VECTOR ( 'NONE', #19514, 999.9999999999998863 ) ;
#41932=AXIS2_PLACEMENT_3D ( 'NONE', #53569, #2706, #15780 ) ;
#41934=LINE ( 'NONE', #55032, #40056 ) ;
#41935=CARTESIAN_POINT ( 'NONE',  ( -21.93882065073936261, -3.432230869623161595, 5.293597968971688772 ) ) ;
#41936=ORIENTED_EDGE ( 'NONE', *, *, #54416, .F. ) ;
#41937=LINE ( 'NONE', #7307, #35561 ) ;
#41939=DIRECTION ( 'NONE',  ( 0.6427681459581294776, -0.7660444431189769032, 0.005002170337467562802 ) ) ;
#41940=VECTOR ( 'NONE', #7525, 999.9999999999998863 ) ;
#41941=LINE ( 'NONE', #3046, #36631 ) ;
#41942=VECTOR ( 'NONE', #30783, 1000.000000000000227 ) ;
#41943=LINE ( 'NONE', #3048, #45965 ) ;
#41944=CARTESIAN_POINT ( 'NONE',  ( -8.377443272075408842, 0.000000000000000000, 6.063214190552308480 ) ) ;
#41945=CARTESIAN_POINT ( 'NONE',  ( -12.23851102634202448, -0.1191753592594197858, 11.68427982808754884 ) ) ;
#41947=LINE ( 'NONE', #34022, #22968 ) ;
#41948=CARTESIAN_POINT ( 'NONE',  ( 2.072287782118878319, 0.000000000000000000, -2.950529333540147015 ) ) ;
#41949=VERTEX_POINT ( 'NONE', #52779 ) ;
#41950=DIRECTION ( 'NONE',  ( 0.000000000000000000, -1.000000000000000000, 0.000000000000000000 ) ) ;
#41951=ORIENTED_EDGE ( 'NONE', *, *, #51920, .T. ) ;
#41952=VECTOR ( 'NONE', #34549, 999.9999999999998863 ) ;
#41953=CARTESIAN_POINT ( 'NONE',  ( -18.34762591811141164, 0.000000000000000000, 7.632278216634138523 ) ) ;
#41954=LINE ( 'NONE', #55305, #51397 ) ;
#41955=CARTESIAN_POINT ( 'NONE',  ( 2.072287782118878319, 0.000000000000000000, -2.950529333540147015 ) ) ;
#41956=ADVANCED_FACE ( 'NONE', ( #566 ), #26973, .F. ) ;
#41957=VECTOR ( 'NONE', #24128, 1000.000000000000000 ) ;
#41958=DIRECTION ( 'NONE',  ( 0.7660212471507180654, -0.6427876096865404731, 0.005961354470445141482 ) ) ;
#41959=PLANE ( 'NONE',  #55817 ) ;
#41960=CARTESIAN_POINT ( 'NONE',  ( -18.31051089201068294, -5.213152330870664208, 3.827418522002113299 ) ) ;
#41962=ORIENTED_EDGE ( 'NONE', *, *, #8559, .F. ) ;
#41963=LINE ( 'NONE', #4434, #22889 ) ;
#41964=VECTOR ( 'NONE', #5418, 1000.000000000000227 ) ;
#41965=DIRECTION ( 'NONE',  ( 0.000000000000000000, -0.000000000000000000, -1.000000000000000000 ) ) ;
#41966=CARTESIAN_POINT ( 'NONE',  ( -10.00813838035478298, 0.000000000000000000, 10.77830692922518452 ) ) ;
#41969=ADVANCED_FACE ( 'NONE', ( #23272 ), #34932, .F. ) ;
#41970=AXIS2_PLACEMENT_3D ( 'NONE', #41948, #32608, #33187 ) ;
#41971=AXIS2_PLACEMENT_3D ( 'NONE', #52528, #38644, #266 ) ;
#41972=CARTESIAN_POINT ( 'NONE',  ( -10.89044314061178298, 0.000000000000000000, 4.735655178860175063 ) ) ;
#41973=CARTESIAN_POINT ( 'NONE',  ( -11.13496771895309756, 0.000000000000000000, 2.148427743403817480 ) ) ;
#41974=ADVANCED_FACE ( 'NONE', ( #39465 ), #9929, .F. ) ;
#41975=PLANE ( 'NONE',  #16960 ) ;
#41976=ADVANCED_FACE ( 'NONE', ( #19259 ), #15297, .F. ) ;
#41977=FACE_OUTER_BOUND ( 'NONE', #39898, .T. ) ;
#41978=ORIENTED_EDGE ( 'NONE', *, *, #39409, .T. ) ;
#41979=AXIS2_PLACEMENT_3D ( 'NONE', #17154, #51774, #30211 ) ;
#41980=PLANE ( 'NONE',  #32157 ) ;
#41981=AXIS2_PLACEMENT_3D ( 'NONE', #2588, #46578, #45743 ) ;
#41982=LINE ( 'NONE', #7941, #6929 ) ;
#41983=ORIENTED_EDGE ( 'NONE', *, *, #13535, .T. ) ;
#41984=LINE ( 'NONE', #3087, #43157 ) ;
#41985=CARTESIAN_POINT ( 'NONE',  ( -17.04466509755329184, -3.108426967578160394, 8.404116713615717771 ) ) ;
#41986=EDGE_CURVE ( 'NONE', #33755, #8726, #19829, .T. ) ;
#41987=ORIENTED_EDGE ( 'NONE', *, *, #35503, .F. ) ;
#41988=EDGE_CURVE ( 'NONE', #10050, #3022, #40850, .T. ) ;
#41989=VECTOR ( 'NONE', #37149, 1000.000000000000227 ) ;
#41990=ORIENTED_EDGE ( 'NONE', *, *, #33280, .T. ) ;
#41991=CARTESIAN_POINT ( 'NONE',  ( -19.99049163959727693, 0.000000000000000000, 5.603506693094304936 ) ) ;
#41992=AXIS2_PLACEMENT_3D ( 'NONE', #40052, #1141, #36105 ) ;
#41993=EDGE_CURVE ( 'NONE', #17849, #4586, #1926, .T. ) ;
#41994=VERTEX_POINT ( 'NONE', #32607 ) ;
#41995=ORIENTED_EDGE ( 'NONE', *, *, #10844, .F. ) ;
#41996=ORIENTED_EDGE ( 'NONE', *, *, #8153, .F. ) ;
#41997=CARTESIAN_POINT ( 'NONE',  ( 2.072287782118878319, 0.000000000000000000, -2.950529333540147015 ) ) ;
#41998=DIRECTION ( 'NONE',  ( 0.007781995580012663651, 0.000000000000000000, -0.9999697198139515519 ) ) ;
#41999=CARTESIAN_POINT ( 'NONE',  ( -20.41887202388666012, -0.5179957512181557755, 4.796177662602485903 ) ) ;
#42000=VECTOR ( 'NONE', #21450, 1000.000000000000227 ) ;
#42001=ADVANCED_FACE ( 'NONE', ( #53903 ), #53624, .F. ) ;
#42002=ORIENTED_EDGE ( 'NONE', *, *, #39448, .T. ) ;
#42003=ORIENTED_EDGE ( 'NONE', *, *, #37841, .T. ) ;
#42004=VECTOR ( 'NONE', #9758, 1000.000000000000227 ) ;
#42005=EDGE_CURVE ( 'NONE', #38778, #33081, #24095, .T. ) ;
#42006=CARTESIAN_POINT ( 'NONE',  ( -13.73672976910459909, 0.000000000000000000, 12.22661844811216270 ) ) ;
#42007=LINE ( 'NONE', #20439, #22737 ) ;
#42008=ORIENTED_EDGE ( 'NONE', *, *, #32024, .F. ) ;
#42010=DIRECTION ( 'NONE',  ( 0.005961354470445682716, -0.6427876096865404731, -0.7660212471507180654 ) ) ;
#42011=ORIENTED_EDGE ( 'NONE', *, *, #23422, .T. ) ;
#42012=FACE_OUTER_BOUND ( 'NONE', #25255, .T. ) ;
#42013=DIRECTION ( 'NONE',  ( -0.7660212471507179544, -0.6427876096865405842, -0.005961354470445141482 ) ) ;
#42014=VECTOR ( 'NONE', #13130, 1000.000000000000227 ) ;
#42016=ORIENTED_EDGE ( 'NONE', *, *, #10930, .T. ) ;
#42017=PLANE ( 'NONE',  #2806 ) ;
#42018=VECTOR ( 'NONE', #38092, 1000.000000000000227 ) ;
#42019=CARTESIAN_POINT ( 'NONE',  ( 2.072287782118878319, 0.000000000000000000, -2.950529333540147015 ) ) ;
#42020=VECTOR ( 'NONE', #22393, 999.9999999999998863 ) ;
#42021=ORIENTED_EDGE ( 'NONE', *, *, #30730, .T. ) ;
#42022=DIRECTION ( 'NONE',  ( -0.6427681459581293666, -0.7660444431189770143, -0.005002170337467561935 ) ) ;
#42024=LINE ( 'NONE', #19891, #18354 ) ;
#42025=ORIENTED_EDGE ( 'NONE', *, *, #14912, .F. ) ;
#42027=PLANE ( 'NONE',  #26023 ) ;
#42028=CARTESIAN_POINT ( 'NONE',  ( -1.086233639165236964, 0.000000000000000000, -2.796443541562362078 ) ) ;
#42029=EDGE_CURVE ( 'NONE', #41467, #34435, #36313, .T. ) ;
#42030=CARTESIAN_POINT ( 'NONE',  ( -12.13851405436063047, 0.000000000000000000, 11.68505802764555135 ) ) ;
#42031=DIRECTION ( 'NONE',  ( -0.005961354470445682716, -0.6427876096865404731, 0.7660212471507180654 ) ) ;
#42032=DIRECTION ( 'NONE',  ( 0.000000000000000000, -1.000000000000000000, 0.000000000000000000 ) ) ;
#42034=VECTOR ( 'NONE', #40435, 1000.000000000000227 ) ;
#42035=VERTEX_POINT ( 'NONE', #54733 ) ;
#42036=DIRECTION ( 'NONE',  ( -0.6427681459581293666, -0.7660444431189770143, -0.005002170337467561935 ) ) ;
#42037=DIRECTION ( 'NONE',  ( 0.000000000000000000, -1.000000000000000000, 0.000000000000000000 ) ) ;
#42038=CARTESIAN_POINT ( 'NONE',  ( -15.60102546347950536, 0.000000000000000000, 12.95077420755565356 ) ) ;
#42039=EDGE_LOOP ( 'NONE', ( #12528, #54525, #42227, #49060 ) ) ;
#42040=PLANE ( 'NONE',  #45629 ) ;
#42041=DIRECTION ( 'NONE',  ( 0.9999697198139515519, 0.000000000000000000, 0.007781995580013368816 ) ) ;
#42042=VECTOR ( 'NONE', #47918, 1000.000000000000000 ) ;
#42043=CARTESIAN_POINT ( 'NONE',  ( -16.81190032086591302, 0.000000000000000000, 3.212244750653343583 ) ) ;
#42044=VECTOR ( 'NONE', #13824, 999.9999999999998863 ) ;
#42045=PLANE ( 'NONE',  #26940 ) ;
#42046=EDGE_CURVE ( 'NONE', #46955, #47606, #23797, .T. ) ;
#42048=ORIENTED_EDGE ( 'NONE', *, *, #46781, .F. ) ;
#42049=ORIENTED_EDGE ( 'NONE', *, *, #21812, .T. ) ;
#42050=PLANE ( 'NONE',  #23224 ) ;
#42051=AXIS2_PLACEMENT_3D ( 'NONE', #20197, #53465, #14566 ) ;
#42052=AXIS2_PLACEMENT_3D ( 'NONE', #10492, #6777, #37150 ) ;
#42053=DIRECTION ( 'NONE',  ( -0.5449076811759708816, 0.6444004775717707689, 0.5364919789714475140 ) ) ;
#42054=EDGE_LOOP ( 'NONE', ( #33763, #16771, #52623, #16161 ) ) ;
#42055=EDGE_CURVE ( 'NONE', #25116, #235, #28638, .T. ) ;
#42056=FACE_OUTER_BOUND ( 'NONE', #800, .T. ) ;
#42058=CARTESIAN_POINT ( 'NONE',  ( -19.06210475032114360, -1.651309408375657428, 6.796380631735580380 ) ) ;
#42059=EDGE_CURVE ( 'NONE', #34091, #32088, #19552, .T. ) ;
#42060=VECTOR ( 'NONE', #47807, 1000.000000000000000 ) ;
#42062=VECTOR ( 'NONE', #41832, 1000.000000000000227 ) ;
#42063=ORIENTED_EDGE ( 'NONE', *, *, #6380, .T. ) ;
#42064=ORIENTED_EDGE ( 'NONE', *, *, #7271, .T. ) ;
#42065=LINE ( 'NONE', #24744, #4826 ) ;
#42066=CARTESIAN_POINT ( 'NONE',  ( -24.26908309836554878, 0.000000000000000000, 6.108867788427308376 ) ) ;
#42067=CARTESIAN_POINT ( 'NONE',  ( -14.66887761629205222, 0.000000000000000000, 12.58869632783390990 ) ) ;
#42068=EDGE_CURVE ( 'NONE', #37968, #16268, #49669, .T. ) ;
#42069=PLANE ( 'NONE',  #371 ) ;
#42070=ORIENTED_EDGE ( 'NONE', *, *, #9501, .F. ) ;
#42071=ORIENTED_EDGE ( 'NONE', *, *, #33192, .T. ) ;
#42072=AXIS2_PLACEMENT_3D ( 'NONE', #23857, #54503, #41725 ) ;
#42073=ADVANCED_FACE ( 'NONE', ( #28071 ), #54198, .F. ) ;
#42074=ORIENTED_EDGE ( 'NONE', *, *, #48875, .F. ) ;
#42075=FACE_OUTER_BOUND ( 'NONE', #6289, .T. ) ;
#42077=DIRECTION ( 'NONE',  ( -0.7660212471507179544, -0.6427876096865405842, -0.005961354470445141482 ) ) ;
#42078=EDGE_LOOP ( 'NONE', ( #37286, #14384, #39866, #42973 ) ) ;
#42079=CARTESIAN_POINT ( 'NONE',  ( -20.54049170961573267, 0.000000000000000000, 4.660556269540326646 ) ) ;
#42080=ORIENTED_EDGE ( 'NONE', *, *, #11788, .T. ) ;
#42081=AXIS2_PLACEMENT_3D ( 'NONE', #55503, #21460, #16611 ) ;
#42082=DIRECTION ( 'NONE',  ( 0.9999697198139515519, 0.000000000000000000, 0.007781995580013368816 ) ) ;
#42084=VERTEX_POINT ( 'NONE', #45655 ) ;
#42085=DIRECTION ( 'NONE',  ( 0.7660212471507180654, -0.6427876096865404731, 0.005961354470445141482 ) ) ;
#42086=AXIS2_PLACEMENT_3D ( 'NONE', #17820, #3611, #43084 ) ;
#42087=ORIENTED_EDGE ( 'NONE', *, *, #52736, .T. ) ;
#42089=DIRECTION ( 'NONE',  ( 0.9999697198139515519, 0.000000000000000000, 0.007781995580013368816 ) ) ;
#42090=CARTESIAN_POINT ( 'NONE',  ( -24.26986129792355129, -0.1191753592594197858, 6.208864760408702388 ) ) ;
#42091=LINE ( 'NONE', #41547, #10294 ) ;
#42092=DIRECTION ( 'NONE',  ( -0.5449076811759708816, 0.6444004775717707689, 0.5364919789714475140 ) ) ;
#42093=AXIS2_PLACEMENT_3D ( 'NONE', #16731, #2804, #12494 ) ;
#42094=CARTESIAN_POINT ( 'NONE',  ( -19.06828360731494953, 0.000000000000000000, 6.518673682440828898 ) ) ;
#42095=ORIENTED_EDGE ( 'NONE', *, *, #15953, .F. ) ;
#42096=EDGE_CURVE ( 'NONE', #9862, #37828, #41423, .T. ) ;
#42097=VECTOR ( 'NONE', #46090, 1000.000000000000227 ) ;
#42098=ORIENTED_EDGE ( 'NONE', *, *, #20395, .T. ) ;
#42099=DIRECTION ( 'NONE',  ( 0.9999697198139515519, 0.000000000000000000, 0.007781995580013368816 ) ) ;
#42100=CARTESIAN_POINT ( 'NONE',  ( -25.20278734466900517, 0.000000000000000000, 6.670939612111840944 ) ) ;
#42101=ADVANCED_FACE ( 'NONE', ( #14730 ), #11597, .F. ) ;
#42102=LINE ( 'NONE', #40230, #39475 ) ;
#42103=LINE ( 'NONE', #25094, #25825 ) ;
#42104=PLANE ( 'NONE',  #36980 ) ;
#42105=AXIS2_PLACEMENT_3D ( 'NONE', #44248, #31481, #44500 ) ;
#42106=VECTOR ( 'NONE', #8919, 999.9999999999998863 ) ;
#42107=EDGE_CURVE ( 'NONE', #54123, #11442, #15549, .T. ) ;
#42108=DIRECTION ( 'NONE',  ( -0.7660212471507179544, -0.6427876096865405842, -0.005961354470445141482 ) ) ;
#42109=ORIENTED_EDGE ( 'NONE', *, *, #53010, .T. ) ;
#42110=EDGE_CURVE ( 'NONE', #33688, #5158, #11306, .T. ) ;
#42111=PLANE ( 'NONE',  #28621 ) ;
#42112=LINE ( 'NONE', #34184, #44088 ) ;
#42113=ORIENTED_EDGE ( 'NONE', *, *, #45563, .F. ) ;
#42114=LINE ( 'NONE', #15430, #27678 ) ;
#42115=ORIENTED_EDGE ( 'NONE', *, *, #30412, .F. ) ;
#42116=ADVANCED_FACE ( 'NONE', ( #1669 ), #18996, .F. ) ;
#42117=EDGE_CURVE ( 'NONE', #31264, #40953, #50758, .T. ) ;
#42118=EDGE_CURVE ( 'NONE', #16969, #27886, #43101, .T. ) ;
#42119=CARTESIAN_POINT ( 'NONE',  ( -15.86710544311044302, 0.000000000000000000, 13.13336954653252953 ) ) ;
#42120=DIRECTION ( 'NONE',  ( 0.007781995580012662783, 0.000000000000000000, -0.9999697198139514409 ) ) ;
#42121=CARTESIAN_POINT ( 'NONE',  ( -21.62239062191499528, 2.229229656569007290, 8.938737581926881504 ) ) ;
#42122=DIRECTION ( 'NONE',  ( 0.000000000000000000, -0.000000000000000000, -1.000000000000000000 ) ) ;
#42124=AXIS2_PLACEMENT_3D ( 'NONE', #47660, #30340, #787 ) ;
#42125=ORIENTED_EDGE ( 'NONE', *, *, #24140, .F. ) ;
#42127=VECTOR ( 'NONE', #55944, 1000.000000000000227 ) ;
#42128=LINE ( 'NONE', #39270, #39419 ) ;
#42129=DIRECTION ( 'NONE',  ( 0.7660212471507180654, -0.6427876096865404731, 0.005961354470445141482 ) ) ;
#42130=CARTESIAN_POINT ( 'NONE',  ( -12.75186478148140523, 0.000000000000000000, 5.090501235045900685 ) ) ;
#42131=AXIS2_PLACEMENT_3D ( 'NONE', #43773, #48894, #40375 ) ;
#42132=CARTESIAN_POINT ( 'NONE',  ( -28.93137873341882127, 0.000000000000000000, 8.119251130998824451 ) ) ;
#42133=CARTESIAN_POINT ( 'NONE',  ( -18.81094516056321808, 0.000000000000000000, 7.459346545571152731 ) ) ;
#42134=ADVANCED_FACE ( 'NONE', ( #25773 ), #7914, .F. ) ;
#42135=DIRECTION ( 'NONE',  ( 0.005002170337468016433, -0.7660444431189770143, -0.6427681459581293666 ) ) ;
#42136=VECTOR ( 'NONE', #9074, 1000.000000000000000 ) ;
#42137=VERTEX_POINT ( 'NONE', #3362 ) ;
#42138=CARTESIAN_POINT ( 'NONE',  ( 2.072287782118878319, 0.000000000000000000, -2.950529333540147015 ) ) ;
#42139=EDGE_CURVE ( 'NONE', #38521, #7991, #25484, .T. ) ;
#42140=LINE ( 'NONE', #50668, #20575 ) ;
#42141=CARTESIAN_POINT ( 'NONE',  ( 2.072287782118878319, 0.000000000000000000, -2.950529333540147015 ) ) ;
#42142=AXIS2_PLACEMENT_3D ( 'NONE', #41879, #4138, #3562 ) ;
#42143=ORIENTED_EDGE ( 'NONE', *, *, #28012, .F. ) ;
#42144=EDGE_CURVE ( 'NONE', #27017, #38106, #21532, .T. ) ;
#42145=AXIS2_PLACEMENT_3D ( 'NONE', #18924, #23463, #24472 ) ;
#42148=DIRECTION ( 'NONE',  ( 0.6427681459581294776, -0.7660444431189769032, 0.005002170337467562802 ) ) ;
#42149=AXIS2_PLACEMENT_3D ( 'NONE', #14474, #35774, #17907 ) ;
#42150=ORIENTED_EDGE ( 'NONE', *, *, #47303, .T. ) ;
#42151=EDGE_CURVE ( 'NONE', #24739, #4654, #7603, .T. ) ;
#42152=CARTESIAN_POINT ( 'NONE',  ( -16.96676784072528932, 0.000000000000000000, 9.320358708932014125 ) ) ;
#42153=EDGE_LOOP ( 'NONE', ( #46236, #11717, #22816, #3869 ) ) ;
#42154=VECTOR ( 'NONE', #44945, 1000.000000000000227 ) ;
#42155=EDGE_LOOP ( 'NONE', ( #6992, #8010, #30767, #37415 ) ) ;
#42157=ORIENTED_EDGE ( 'NONE', *, *, #32062, .F. ) ;
#42158=EDGE_LOOP ( 'NONE', ( #13783, #47468, #8098, #22379, #3454 ) ) ;
#42159=CARTESIAN_POINT ( 'NONE',  ( -20.54126990917373519, -0.1191753592594197858, 4.760553241521720658 ) ) ;
#42160=EDGE_LOOP ( 'NONE', ( #8451, #3027, #30065, #18507 ) ) ;
#42162=EDGE_LOOP ( 'NONE', ( #12340, #24840, #51201, #26127 ) ) ;
#42164=ORIENTED_EDGE ( 'NONE', *, *, #37981, .T. ) ;
#42165=ORIENTED_EDGE ( 'NONE', *, *, #960, .T. ) ;
#42166=VECTOR ( 'NONE', #53515, 1000.000000000000227 ) ;
#42167=CARTESIAN_POINT ( 'NONE',  ( -19.39493078104614909, -2.774784975051975966, 7.711734769794177602 ) ) ;
#42171=LINE ( 'NONE', #34488, #36864 ) ;
#42173=VECTOR ( 'NONE', #51816, 1000.000000000000227 ) ;
#42174=ORIENTED_EDGE ( 'NONE', *, *, #42192, .F. ) ;
#42175=ORIENTED_EDGE ( 'NONE', *, *, #37366, .T. ) ;
#42176=LINE ( 'NONE', #16322, #35850 ) ;
#42177=FACE_OUTER_BOUND ( 'NONE', #12175, .T. ) ;
#42178=VECTOR ( 'NONE', #8601, 1000.000000000000227 ) ;
#42180=FACE_OUTER_BOUND ( 'NONE', #45328, .T. ) ;
#42181=VECTOR ( 'NONE', #21542, 1000.000000000000227 ) ;
#42182=VECTOR ( 'NONE', #32742, 999.9999999999998863 ) ;
#42183=CARTESIAN_POINT ( 'NONE',  ( -11.67244013076689946, 0.000000000000000000, 11.50401908778467863 ) ) ;
#42184=VECTOR ( 'NONE', #36687, 1000.000000000000227 ) ;
#42185=CARTESIAN_POINT ( 'NONE',  ( -23.33849165029409889, 0.000000000000000000, 5.946783852668351855 ) ) ;
#42186=DIRECTION ( 'NONE',  ( 0.7660212471507180654, -0.6427876096865404731, 0.005961354470445141482 ) ) ;
#42187=ORIENTED_EDGE ( 'NONE', *, *, #14705, .T. ) ;
#42189=CARTESIAN_POINT ( 'NONE',  ( -21.57134263578401701, 2.714935509636507316, 9.716034862368092107 ) ) ;
#42190=ORIENTED_EDGE ( 'NONE', *, *, #44959, .F. ) ;
#42191=VECTOR ( 'NONE', #22388, 1000.000000000000227 ) ;
#42192=EDGE_CURVE ( 'NONE', #41253, #52332, #56157, .T. ) ;
#42193=EDGE_CURVE ( 'NONE', #11442, #49751, #29478, .T. ) ;
#42194=CARTESIAN_POINT ( 'NONE',  ( -20.26176469941677993, 0.000000000000000000, 14.76116360616437895 ) ) ;
#42195=DIRECTION ( 'NONE',  ( 0.007781995580012662783, 0.000000000000000000, -0.9999697198139514409 ) ) ;
#42196=CARTESIAN_POINT ( 'NONE',  ( -14.66887761629205222, 0.000000000000000000, 12.58869632783390990 ) ) ;
#42197=LINE ( 'NONE', #38795, #50424 ) ;
#42198=EDGE_CURVE ( 'NONE', #5857, #16502, #3898, .T. ) ;
#42199=CARTESIAN_POINT ( 'NONE',  ( -16.81190032086591302, 0.000000000000000000, 3.212244750653343583 ) ) ;
#42200=AXIS2_PLACEMENT_3D ( 'NONE', #1961, #27547, #53126 ) ;
#42201=VERTEX_POINT ( 'NONE', #12995 ) ;
#42202=AXIS2_PLACEMENT_3D ( 'NONE', #4613, #43267, #48053 ) ;
#42203=ORIENTED_EDGE ( 'NONE', *, *, #9094, .F. ) ;
#42204=FACE_OUTER_BOUND ( 'NONE', #26762, .T. ) ;
#42206=PLANE ( 'NONE',  #21529 ) ;
#42207=LINE ( 'NONE', #50152, #18265 ) ;
#42208=DIRECTION ( 'NONE',  ( 0.5364919789714477361, 0.6444004775717706579, 0.5449076811759711036 ) ) ;
#42209=DIRECTION ( 'NONE',  ( 0.005961354470445682716, -0.6427876096865404731, -0.7660212471507180654 ) ) ;
#42210=LINE ( 'NONE', #29136, #49195 ) ;
#42211=VECTOR ( 'NONE', #52413, 1000.000000000000227 ) ;
#42212=LINE ( 'NONE', #49695, #9636 ) ;
#42214=VECTOR ( 'NONE', #30705, 1000.000000000000000 ) ;
#42216=DIRECTION ( 'NONE',  ( -0.005002170337468016433, -0.7660444431189770143, 0.6427681459581293666 ) ) ;
#42217=ORIENTED_EDGE ( 'NONE', *, *, #1429, .T. ) ;
#42218=DIRECTION ( 'NONE',  ( 0.000000000000000000, -1.000000000000000000, 0.000000000000000000 ) ) ;
#42219=VECTOR ( 'NONE', #50363, 1000.000000000000227 ) ;
#42220=EDGE_LOOP ( 'NONE', ( #45830, #18121, #41222 ) ) ;
#42221=ADVANCED_FACE ( 'NONE', ( #17241 ), #8175, .F. ) ;
#42222=VECTOR ( 'NONE', #8527, 999.9999999999998863 ) ;
#42223=ORIENTED_EDGE ( 'NONE', *, *, #51726, .T. ) ;
#42227=ORIENTED_EDGE ( 'NONE', *, *, #17435, .F. ) ;
#42229=DIRECTION ( 'NONE',  ( 0.5364919789714477361, 0.6444004775717706579, 0.5449076811759711036 ) ) ;
#42230=DIRECTION ( 'NONE',  ( 0.9999697198139515519, 0.000000000000000000, 0.007781995580013368816 ) ) ;
#42231=ADVANCED_FACE ( 'NONE', ( #16988 ), #30318, .F. ) ;
#42233=VECTOR ( 'NONE', #45013, 1000.000000000000000 ) ;
#42234=VECTOR ( 'NONE', #38311, 1000.000000000000227 ) ;
#42236=FACE_OUTER_BOUND ( 'NONE', #53611, .T. ) ;
#42237=VECTOR ( 'NONE', #38869, 1000.000000000000000 ) ;
#42238=EDGE_LOOP ( 'NONE', ( #12073, #48155, #47182, #23711 ) ) ;
#42240=VERTEX_POINT ( 'NONE', #20680 ) ;
#42241=VECTOR ( 'NONE', #51524, 1000.000000000000227 ) ;
#42242=VECTOR ( 'NONE', #35425, 1000.000000000000114 ) ;
#42244=FACE_OUTER_BOUND ( 'NONE', #42162, .T. ) ;
#42245=CARTESIAN_POINT ( 'NONE',  ( -18.25702930620386866, -0.1191753592594153865, 8.840982497946823671 ) ) ;
#42246=VERTEX_POINT ( 'NONE', #8759 ) ;
#42247=FACE_OUTER_BOUND ( 'NONE', #24609, .T. ) ;
#42248=ORIENTED_EDGE ( 'NONE', *, *, #13321, .T. ) ;
#42249=CARTESIAN_POINT ( 'NONE',  ( -22.40478740399063895, 0.000000000000000000, 5.384712028983816623 ) ) ;
#42250=CARTESIAN_POINT ( 'NONE',  ( -13.10291263837268616, -0.1191753592594188005, 3.341111978528461535 ) ) ;
#42251=AXIS2_PLACEMENT_3D ( 'NONE', #10291, #32160, #53451 ) ;
#42252=DIRECTION ( 'NONE',  ( -0.5364919789714478471, 0.6444004775717705469, -0.5449076811759709926 ) ) ;
#42253=DIRECTION ( 'NONE',  ( -0.005961354470445682716, -0.6427876096865404731, 0.7660212471507180654 ) ) ;
#42255=LINE ( 'NONE', #34307, #14024 ) ;
#42256=DIRECTION ( 'NONE',  ( -0.9999697198139514409, -0.000000000000000000, -0.007781995580013368816 ) ) ;
#42257=FACE_OUTER_BOUND ( 'NONE', #6630, .T. ) ;
#42258=ORIENTED_EDGE ( 'NONE', *, *, #45773, .T. ) ;
#42259=FACE_OUTER_BOUND ( 'NONE', #21108, .T. ) ;
#42261=VECTOR ( 'NONE', #10060, 999.9999999999998863 ) ;
#42263=CARTESIAN_POINT ( 'NONE',  ( -19.51337669467617530, -3.270328918600659218, 9.628756819687440682 ) ) ;
#42264=LINE ( 'NONE', #45967, #48685 ) ;
#42265=DIRECTION ( 'NONE',  ( -0.6427681459581293666, -0.7660444431189770143, -0.005002170337467561935 ) ) ;
#42266=VECTOR ( 'NONE', #6500, 1000.000000000000114 ) ;
#42267=PLANE ( 'NONE',  #50321 ) ;
#42268=PLANE ( 'NONE',  #24970 ) ;
#42269=EDGE_CURVE ( 'NONE', #42663, #48737, #3051, .T. ) ;
#42270=EDGE_CURVE ( 'NONE', #18631, #28691, #42255, .T. ) ;
#42271=VECTOR ( 'NONE', #45383, 1000.000000000000114 ) ;
#42272=DIRECTION ( 'NONE',  ( 0.9999697198139515519, 0.000000000000000000, 0.007781995580013368816 ) ) ;
#42273=VECTOR ( 'NONE', #28475, 1000.000000000000227 ) ;
#42274=ORIENTED_EDGE ( 'NONE', *, *, #13487, .T. ) ;
#42275=CARTESIAN_POINT ( 'NONE',  ( -15.92522266148258936, -0.1191753592594200495, 7.751132947013579688 ) ) ;
#42276=FACE_OUTER_BOUND ( 'NONE', #15097, .T. ) ;
#42277=DIRECTION ( 'NONE',  ( 0.007781995580012662783, 0.000000000000000000, -0.9999697198139514409 ) ) ;
#42278=LINE ( 'NONE', #20700, #54475 ) ;
#42279=VECTOR ( 'NONE', #10210, 1000.000000000000227 ) ;
#42280=VECTOR ( 'NONE', #54186, 1000.000000000000000 ) ;
#42281=PLANE ( 'NONE',  #46341 ) ;
#42282=DIRECTION ( 'NONE',  ( -0.005961354470445682716, -0.6427876096865404731, 0.7660212471507180654 ) ) ;
#42283=PLANE ( 'NONE',  #39629 ) ;
#42284=LINE ( 'NONE', #50526, #18353 ) ;
#42285=EDGE_CURVE ( 'NONE', #4739, #43397, #55297, .T. ) ;
#42286=VERTEX_POINT ( 'NONE', #51032 ) ;
#42287=AXIS2_PLACEMENT_3D ( 'NONE', #50016, #54550, #44649 ) ;
#42288=VECTOR ( 'NONE', #35034, 999.9999999999998863 ) ;
#42289=CARTESIAN_POINT ( 'NONE',  ( -10.82076189722203452, -0.1191753592594203132, 7.421524971165663231 ) ) ;
#42290=CARTESIAN_POINT ( 'NONE',  ( -9.968473853056176281, 0.000000000000000000, 5.681500352874511606 ) ) ;
#42291=ORIENTED_EDGE ( 'NONE', *, *, #43627, .F. ) ;
#42292=VERTEX_POINT ( 'NONE', #4481 ) ;
#42293=DIRECTION ( 'NONE',  ( -0.9999697198139514409, -0.000000000000000000, -0.007781995580013368816 ) ) ;
#42294=VERTEX_POINT ( 'NONE', #26324 ) ;
#42295=ORIENTED_EDGE ( 'NONE', *, *, #48482, .T. ) ;
#42296=CARTESIAN_POINT ( 'NONE',  ( -9.938176918887348776, 0.000000000000000000, 1.788409376334078926 ) ) ;
#42297=EDGE_CURVE ( 'NONE', #32592, #20518, #26912, .T. ) ;
#42298=VECTOR ( 'NONE', #55539, 1000.000000000000227 ) ;
#42299=EDGE_LOOP ( 'NONE', ( #55051, #40463, #9699, #41403 ) ) ;
#42300=ORIENTED_EDGE ( 'NONE', *, *, #14777, .F. ) ;
#42301=EDGE_LOOP ( 'NONE', ( #11714, #13657, #45923, #5166 ) ) ;
#42302=EDGE_CURVE ( 'NONE', #24756, #34349, #10650, .T. ) ;
#42303=LINE ( 'NONE', #47108, #52938 ) ;
#42304=FACE_OUTER_BOUND ( 'NONE', #30998, .T. ) ;
#42305=VECTOR ( 'NONE', #20478, 999.9999999999998863 ) ;
#42306=CARTESIAN_POINT ( 'NONE',  ( -14.94760462649100496, 0.000000000000000000, 2.488088991209854051 ) ) ;
#42307=VECTOR ( 'NONE', #17267, 1000.000000000000227 ) ;
#42308=ORIENTED_EDGE ( 'NONE', *, *, #39138, .T. ) ;
#42309=EDGE_CURVE ( 'NONE', #9132, #35388, #40986, .T. ) ;
#42310=EDGE_LOOP ( 'NONE', ( #7119, #19689, #12367, #14014 ) ) ;
#42311=AXIS2_PLACEMENT_3D ( 'NONE', #9027, #4223, #26613 ) ;
#42312=PLANE ( 'NONE',  #25728 ) ;
#42313=CARTESIAN_POINT ( 'NONE',  ( -15.48665731996427475, -0.1941918491731561003, 3.016177271524973946 ) ) ;
#42314=ORIENTED_EDGE ( 'NONE', *, *, #14279, .T. ) ;
#42315=DIRECTION ( 'NONE',  ( -0.005002170337468016433, -0.7660444431189770143, 0.6427681459581293666 ) ) ;
#42317=LINE ( 'NONE', #3413, #38479 ) ;
#42318=DIRECTION ( 'NONE',  ( -0.5449076811759708816, 0.6444004775717707689, 0.5364919789714475140 ) ) ;
#42319=ORIENTED_EDGE ( 'NONE', *, *, #3144, .F. ) ;
#42320=VECTOR ( 'NONE', #2063, 1000.000000000000227 ) ;
#42321=DIRECTION ( 'NONE',  ( 0.005961354470445682716, -0.6427876096865404731, -0.7660212471507180654 ) ) ;
#42322=EDGE_CURVE ( 'NONE', #26568, #13781, #19405, .T. ) ;
#42323=VECTOR ( 'NONE', #31494, 999.9999999999998863 ) ;
#42324=CARTESIAN_POINT ( 'NONE',  ( -14.59185039342477275, 0.000000000000000000, 2.690863609132300827 ) ) ;
#42325=VECTOR ( 'NONE', #9375, 999.9999999999998863 ) ;
#42326=VERTEX_POINT ( 'NONE', #21790 ) ;
#42327=CARTESIAN_POINT ( 'NONE',  ( -14.00280974873554030, 0.000000000000000000, 12.40921378708904044 ) ) ;
#42328=DIRECTION ( 'NONE',  ( 0.000000000000000000, -0.000000000000000000, -1.000000000000000000 ) ) ;
#42329=CARTESIAN_POINT ( 'NONE',  ( -14.37176155590648285, -4.889348428825662118, 10.28866572930882839 ) ) ;
#42330=LINE ( 'NONE', #37208, #12929 ) ;
#42332=VERTEX_POINT ( 'NONE', #47923 ) ;
#42333=EDGE_CURVE ( 'NONE', #21510, #41396, #5328, .T. ) ;
#42334=DIRECTION ( 'NONE',  ( 0.000000000000000000, -0.000000000000000000, -1.000000000000000000 ) ) ;
#42335=PLANE ( 'NONE',  #47779 ) ;
#42337=CARTESIAN_POINT ( 'NONE',  ( -16.81190032086591302, 0.000000000000000000, 3.212244750653343583 ) ) ;
#42338=FACE_OUTER_BOUND ( 'NONE', #18780, .T. ) ;
#42340=LINE ( 'NONE', #20749, #50619 ) ;
#42341=VECTOR ( 'NONE', #32960, 999.9999999999998863 ) ;
#42342=CARTESIAN_POINT ( 'NONE',  ( -14.94760462649100496, 0.000000000000000000, 2.488088991209854051 ) ) ;
#42343=ORIENTED_EDGE ( 'NONE', *, *, #35734, .F. ) ;
#42344=LINE ( 'NONE', #41211, #28046 ) ;
#42346=EDGE_LOOP ( 'NONE', ( #7583, #2133, #44565, #4785 ) ) ;
#42347=DIRECTION ( 'NONE',  ( -0.9999697198139514409, -0.000000000000000000, -0.007781995580013368816 ) ) ;
#42348=DIRECTION ( 'NONE',  ( -0.5449076811759708816, 0.6444004775717707689, 0.5364919789714475140 ) ) ;
#42349=ADVANCED_FACE ( 'NONE', ( #35414 ), #52175, .F. ) ;
#42350=VECTOR ( 'NONE', #28520, 999.9999999999998863 ) ;
#42351=LINE ( 'NONE', #7148, #13176 ) ;
#42352=DIRECTION ( 'NONE',  ( 0.005961354470445682716, -0.6427876096865404731, -0.7660212471507180654 ) ) ;
#42353=DIRECTION ( 'NONE',  ( 0.9999697198139515519, 0.000000000000000000, 0.007781995580013368816 ) ) ;
#42354=EDGE_CURVE ( 'NONE', #38710, #20039, #13291, .T. ) ;
#42356=AXIS2_PLACEMENT_3D ( 'NONE', #46735, #25428, #42736 ) ;
#42357=ORIENTED_EDGE ( 'NONE', *, *, #923, .F. ) ;
#42358=DIRECTION ( 'NONE',  ( 0.007781995580012663651, -3.146120232559066537E-19, -0.9999697198139514409 ) ) ;
#42359=DIRECTION ( 'NONE',  ( 0.5364919789714477361, 0.6444004775717706579, 0.5449076811759711036 ) ) ;
#42360=DIRECTION ( 'NONE',  ( 0.000000000000000000, -1.000000000000000000, 0.000000000000000000 ) ) ;
#42361=VECTOR ( 'NONE', #49666, 1000.000000000000227 ) ;
#42362=VERTEX_POINT ( 'NONE', #15178 ) ;
#42363=DIRECTION ( 'NONE',  ( 0.9999697198139515519, 0.000000000000000000, 0.007781995580013368816 ) ) ;
#42364=VERTEX_POINT ( 'NONE', #43924 ) ;
#42365=DIRECTION ( 'NONE',  ( -0.5449076811759708816, 0.6444004775717707689, 0.5364919789714475140 ) ) ;
#42366=VECTOR ( 'NONE', #50916, 999.9999999999998863 ) ;
#42367=ORIENTED_EDGE ( 'NONE', *, *, #51587, .F. ) ;
#42368=VERTEX_POINT ( 'NONE', #30620 ) ;
#42369=ORIENTED_EDGE ( 'NONE', *, *, #26528, .T. ) ;
#42370=CARTESIAN_POINT ( 'NONE',  ( -15.05218540864184540, 4.981562823951512620, 2.369773783146779778 ) ) ;
#42371=DIRECTION ( 'NONE',  ( 0.005002170337468016433, -0.7660444431189770143, -0.6427681459581293666 ) ) ;
#42372=DIRECTION ( 'NONE',  ( 0.9999697198139515519, 0.000000000000000000, 0.007781995580013368816 ) ) ;
#42373=LINE ( 'NONE', #46916, #36663 ) ;
#42374=ADVANCED_FACE ( 'NONE', ( #48772 ), #184, .F. ) ;
#42375=VERTEX_POINT ( 'NONE', #52715 ) ;
#42376=ORIENTED_EDGE ( 'NONE', *, *, #32616, .T. ) ;
#42377=VERTEX_POINT ( 'NONE', #32495 ) ;
#42378=DIRECTION ( 'NONE',  ( -0.9999697198139514409, 0.000000000000000000, -0.007781995580013368816 ) ) ;
#42379=PLANE ( 'NONE',  #431 ) ;
#42380=VERTEX_POINT ( 'NONE', #49797 ) ;
#42381=DIRECTION ( 'NONE',  ( 0.000000000000000000, -0.000000000000000000, -1.000000000000000000 ) ) ;
#42382=VERTEX_POINT ( 'NONE', #26076 ) ;
#42383=CARTESIAN_POINT ( 'NONE',  ( -13.63673279712320507, -0.1191753592594197858, 12.22739664767016521 ) ) ;
#42384=CARTESIAN_POINT ( 'NONE',  ( -29.86197018149027116, 0.000000000000000000, 8.281335066757780083 ) ) ;
#42386=EDGE_LOOP ( 'NONE', ( #43265, #20524, #31127, #31249 ) ) ;
#42387=CARTESIAN_POINT ( 'NONE',  ( 2.072287782118878319, 0.000000000000000000, -2.950529333540147015 ) ) ;
#42388=ORIENTED_EDGE ( 'NONE', *, *, #15269, .T. ) ;
#42389=EDGE_CURVE ( 'NONE', #621, #2726, #35700, .T. ) ;
#42390=EDGE_CURVE ( 'NONE', #29543, #24756, #50896, .T. ) ;
#42392=DIRECTION ( 'NONE',  ( 0.007781995580012662783, 0.000000000000000000, -0.9999697198139514409 ) ) ;
#42393=CARTESIAN_POINT ( 'NONE',  ( -14.89517369626102195, 0.000000000000000000, 7.659145998126207999 ) ) ;
#42396=CARTESIAN_POINT ( 'NONE',  ( -20.50465292808819839, -5.051250379848164052, 4.684863322079202419 ) ) ;
#42397=DIRECTION ( 'NONE',  ( 0.6427681459581294776, -0.7660444431189769032, 0.005002170337467562802 ) ) ;
#42398=CARTESIAN_POINT ( 'NONE',  ( -12.33850799832341849, 0.000000000000000000, 11.68350162852954632 ) ) ;
#42399=ORIENTED_EDGE ( 'NONE', *, *, #39993, .T. ) ;
#42400=ORIENTED_EDGE ( 'NONE', *, *, #51642, .T. ) ;
#42401=AXIS2_PLACEMENT_3D ( 'NONE', #45260, #16006, #27958 ) ;
#42402=EDGE_CURVE ( 'NONE', #39510, #42731, #16542, .T. ) ;
#42403=CARTESIAN_POINT ( 'NONE',  ( -16.89925026227929195, -0.1191753592594197858, 13.49466922669627422 ) ) ;
#42404=DIRECTION ( 'NONE',  ( -0.9999697198139514409, -0.000000000000000000, -0.007781995580013368816 ) ) ;
#42405=LINE ( 'NONE', #20806, #3268 ) ;
#42406=LINE ( 'NONE', #2636, #18562 ) ;
#42407=EDGE_CURVE ( 'NONE', #17347, #13812, #29333, .T. ) ;
#42408=DIRECTION ( 'NONE',  ( 0.6427681459581294776, -0.7660444431189769032, 0.005002170337467562802 ) ) ;
#42409=DIRECTION ( 'NONE',  ( -0.005002170337468016433, -0.7660444431189770143, 0.6427681459581293666 ) ) ;
#42410=ORIENTED_EDGE ( 'NONE', *, *, #25149, .T. ) ;
#42411=CARTESIAN_POINT ( 'NONE',  ( -9.001607178914184715, -0.02746274897879631693, 3.819319703528829546 ) ) ;
#42412=PLANE ( 'NONE',  #6925 ) ;
#42413=EDGE_LOOP ( 'NONE', ( #51995, #21931, #18851, #4514 ) ) ;
#42414=PLANE ( 'NONE',  #514 ) ;
#42415=EDGE_LOOP ( 'NONE', ( #19958, #46319, #42008, #44389 ) ) ;
#42416=EDGE_CURVE ( 'NONE', #3628, #37763, #28487, .T. ) ;
#42417=DIRECTION ( 'NONE',  ( 0.005002170337468016433, -0.7660444431189770143, -0.6427681459581293666 ) ) ;
#42418=LINE ( 'NONE', #23961, #19690 ) ;
#42419=LINE ( 'NONE', #37585, #48601 ) ;
#42420=DIRECTION ( 'NONE',  ( 0.000000000000000000, -0.000000000000000000, -1.000000000000000000 ) ) ;
#42422=EDGE_CURVE ( 'NONE', #873, #18658, #41557, .T. ) ;
#42423=ORIENTED_EDGE ( 'NONE', *, *, #13934, .F. ) ;
#42424=EDGE_LOOP ( 'NONE', ( #23050, #23526, #26498, #24208 ) ) ;
#42425=CARTESIAN_POINT ( 'NONE',  ( -11.23574289049249231, -0.1191753592594189115, 2.247646515827207647 ) ) ;
#42426=LINE ( 'NONE', #20568, #29490 ) ;
#42427=CARTESIAN_POINT ( 'NONE',  ( 1.971453974394196562, 0.000000000000000000, 10.00639841352631088 ) ) ;
#42428=DIRECTION ( 'NONE',  ( 0.6427681459581294776, -0.7660444431189769032, 0.005002170337467562802 ) ) ;
#42429=DIRECTION ( 'NONE',  ( 0.9999697198139515519, 0.000000000000000000, 0.007781995580013368816 ) ) ;
#42430=CARTESIAN_POINT ( 'NONE',  ( -19.61647402266476803, -0.1191753592594171213, 4.401331113001130113 ) ) ;
#42431=ORIENTED_EDGE ( 'NONE', *, *, #41909, .T. ) ;
#42432=LINE ( 'NONE', #38152, #22897 ) ;
#42433=LINE ( 'NONE', #46974, #55923 ) ;
#42434=DIRECTION ( 'NONE',  ( -0.005961354470445682716, -0.6427876096865404731, 0.7660212471507180654 ) ) ;
#42435=ORIENTED_EDGE ( 'NONE', *, *, #40399, .T. ) ;
#42436=CARTESIAN_POINT ( 'NONE',  ( 2.072287782118878319, 0.000000000000000000, -2.950529333540147015 ) ) ;
#42437=DIRECTION ( 'NONE',  ( 0.000000000000000000, -1.000000000000000000, 0.000000000000000000 ) ) ;
#42438=CARTESIAN_POINT ( 'NONE',  ( -8.875996589204540044, 0.000000000000000000, 10.41778544861944233 ) ) ;
#42439=ORIENTED_EDGE ( 'NONE', *, *, #1583, .F. ) ;
#42440=VECTOR ( 'NONE', #27892, 999.9999999999998863 ) ;
#42441=CARTESIAN_POINT ( 'NONE',  ( 2.072287782118878319, 0.000000000000000000, -2.950529333540147015 ) ) ;
#42442=EDGE_CURVE ( 'NONE', #13455, #18918, #7764, .T. ) ;
#42443=ORIENTED_EDGE ( 'NONE', *, *, #20107, .T. ) ;
#42444=ORIENTED_EDGE ( 'NONE', *, *, #43595, .F. ) ;
#42445=EDGE_CURVE ( 'NONE', #19751, #46912, #41279, .T. ) ;
#42446=EDGE_LOOP ( 'NONE', ( #43136, #7353, #47113, #29087 ) ) ;
#42447=VERTEX_POINT ( 'NONE', #55439 ) ;
#42448=LINE ( 'NONE', #24839, #9374 ) ;
#42449=ORIENTED_EDGE ( 'NONE', *, *, #32861, .F. ) ;
#42450=EDGE_CURVE ( 'NONE', #3308, #56226, #42103, .T. ) ;
#42451=LINE ( 'NONE', #55486, #30401 ) ;
#42452=EDGE_CURVE ( 'NONE', #16370, #22478, #42406, .T. ) ;
#42453=EDGE_CURVE ( 'NONE', #49004, #51932, #3497, .T. ) ;
#42454=ORIENTED_EDGE ( 'NONE', *, *, #44960, .F. ) ;
#42456=ORIENTED_EDGE ( 'NONE', *, *, #9761, .F. ) ;
#42458=ADVANCED_FACE ( 'NONE', ( #20807 ), #15696, .F. ) ;
#42459=CARTESIAN_POINT ( 'NONE',  ( -19.60990026154428278, 0.000000000000000000, 4.498472333781370125 ) ) ;
#42460=DIRECTION ( 'NONE',  ( -0.5449076811759708816, 0.6444004775717707689, 0.5364919789714475140 ) ) ;
#42461=DIRECTION ( 'NONE',  ( 0.6427681459581294776, -0.7660444431189769032, 0.005002170337467562802 ) ) ;
#42462=LINE ( 'NONE', #3277, #44104 ) ;
#42464=ORIENTED_EDGE ( 'NONE', *, *, #2381, .T. ) ;
#42465=EDGE_LOOP ( 'NONE', ( #8581, #42761, #22926, #54030 ) ) ;
#42466=EDGE_CURVE ( 'NONE', #37629, #39029, #38125, .T. ) ;
#42468=LINE ( 'NONE', #15486, #37546 ) ;
#42469=EDGE_CURVE ( 'NONE', #35036, #4830, #54329, .T. ) ;
#42470=DIRECTION ( 'NONE',  ( 0.000000000000000000, -0.000000000000000000, -1.000000000000000000 ) ) ;
#42471=CARTESIAN_POINT ( 'NONE',  ( -11.32823801451301726, -1.327505506330656893, 3.260866780426896483 ) ) ;
#42472=EDGE_CURVE ( 'NONE', #56189, #27265, #15422, .T. ) ;
#42473=DIRECTION ( 'NONE',  ( -0.3620778797217456546, 0.000000000000000000, -0.9321478471874540261 ) ) ;
#42474=CARTESIAN_POINT ( 'NONE',  ( -16.28710523641237273, -4.403642575758160760, 10.23552420831110865 ) ) ;
#42475=ORIENTED_EDGE ( 'NONE', *, *, #54140, .F. ) ;
#42476=CARTESIAN_POINT ( 'NONE',  ( -19.94369481285463408, 1.574118978153236093, 6.298974588870400737 ) ) ;
#42477=CARTESIAN_POINT ( 'NONE',  ( -15.86710544311044302, 0.000000000000000000, 13.13336954653252953 ) ) ;
#42478=ORIENTED_EDGE ( 'NONE', *, *, #34149, .T. ) ;
#42480=VECTOR ( 'NONE', #13897, 1000.000000000000114 ) ;
#42481=FACE_OUTER_BOUND ( 'NONE', #30058, .T. ) ;
#42482=DIRECTION ( 'NONE',  ( -0.6427681459581293666, -0.7660444431189770143, -0.005002170337467561935 ) ) ;
#42483=PLANE ( 'NONE',  #25432 ) ;
#42484=CARTESIAN_POINT ( 'NONE',  ( 2.072287782118878319, 0.000000000000000000, -2.950529333540147015 ) ) ;
#42485=CARTESIAN_POINT ( 'NONE',  ( -11.30636317915456779, -0.1191753592594197858, 11.32220194836580340 ) ) ;
#42486=ORIENTED_EDGE ( 'NONE', *, *, #50106, .T. ) ;
#42487=ORIENTED_EDGE ( 'NONE', *, *, #20903, .T. ) ;
#42488=LINE ( 'NONE', #8130, #50212 ) ;
#42489=DIRECTION ( 'NONE',  ( 0.9999697198139515519, 0.000000000000000000, 0.007781995580013368816 ) ) ;
#42490=DIRECTION ( 'NONE',  ( -0.5449076811759708816, 0.6444004775717707689, 0.5364919789714475140 ) ) ;
#42491=CARTESIAN_POINT ( 'NONE',  ( -15.88130887279446490, 0.000000000000000000, 3.050160814894388839 ) ) ;
#42492=DIRECTION ( 'NONE',  ( -0.6246952433987893460, -0.7422098413412802076, 0.2426528472758542054 ) ) ;
#42493=PLANE ( 'NONE',  #50002 ) ;
#42494=LINE ( 'NONE', #11816, #51055 ) ;
#42495=LINE ( 'NONE', #10792, #27801 ) ;
#42497=LINE ( 'NONE', #3013, #15625 ) ;
#42498=VERTEX_POINT ( 'NONE', #45515 ) ;
#42499=FACE_OUTER_BOUND ( 'NONE', #52230, .T. ) ;
#42500=EDGE_CURVE ( 'NONE', #6162, #56100, #7463, .T. ) ;
#42501=ORIENTED_EDGE ( 'NONE', *, *, #33434, .F. ) ;
#42502=EDGE_CURVE ( 'NONE', #34236, #25655, #19961, .T. ) ;
#42503=ORIENTED_EDGE ( 'NONE', *, *, #46840, .T. ) ;
#42504=VERTEX_POINT ( 'NONE', #41814 ) ;
#42505=ORIENTED_EDGE ( 'NONE', *, *, #47303, .F. ) ;
#42506=ORIENTED_EDGE ( 'NONE', *, *, #29966, .T. ) ;
#42507=ORIENTED_EDGE ( 'NONE', *, *, #54541, .F. ) ;
#42508=CARTESIAN_POINT ( 'NONE',  ( -19.02759475333626327, -4.403642575758163424, 4.131785845448357364 ) ) ;
#42509=DIRECTION ( 'NONE',  ( 0.007781995580012663651, -3.146120232559066537E-19, -0.9999697198139514409 ) ) ;
#42510=DIRECTION ( 'NONE',  ( -0.6427681459581293666, -0.7660444431189770143, -0.005002170337467561935 ) ) ;
#42511=EDGE_CURVE ( 'NONE', #46187, #28751, #37871, .T. ) ;
#42512=EDGE_CURVE ( 'NONE', #38880, #5158, #54893, .T. ) ;
#42513=ADVANCED_FACE ( 'NONE', ( #8602 ), #46946, .F. ) ;
#42514=AXIS2_PLACEMENT_3D ( 'NONE', #11476, #10662, #24507 ) ;
#42515=ORIENTED_EDGE ( 'NONE', *, *, #45403, .T. ) ;
#42516=DIRECTION ( 'NONE',  ( 0.8531650599175527594, 0.4028455766673922356, -0.3313982828793700652 ) ) ;
#42517=ORIENTED_EDGE ( 'NONE', *, *, #50726, .T. ) ;
#42519=ADVANCED_FACE ( 'NONE', ( #30475 ), #43260, .F. ) ;
#42522=DIRECTION ( 'NONE',  ( -0.005961354470445682716, -0.6427876096865404731, 0.7660212471507180654 ) ) ;
#42523=CARTESIAN_POINT ( 'NONE',  ( -28.93137873341882127, 0.000000000000000000, 8.119251130998824451 ) ) ;
#42524=ORIENTED_EDGE ( 'NONE', *, *, #22730, .T. ) ;
#42525=DIRECTION ( 'NONE',  ( -0.6427681459581293666, -0.7660444431189770143, -0.005002170337467561935 ) ) ;
#42526=ORIENTED_EDGE ( 'NONE', *, *, #32921, .F. ) ;
#42527=DIRECTION ( 'NONE',  ( -0.005961354470445682716, -0.6427876096865404731, 0.7660212471507180654 ) ) ;
#42528=CARTESIAN_POINT ( 'NONE',  ( -20.54204810873173415, 0.000000000000000000, 4.860550213503115558 ) ) ;
#42529=EDGE_CURVE ( 'NONE', #3673, #36934, #25934, .T. ) ;
#42530=LINE ( 'NONE', #12451, #29659 ) ;
#42531=CARTESIAN_POINT ( 'NONE',  ( -13.08486533123210194, 0.000000000000000000, 1.963927175729152541 ) ) ;
#42532=CARTESIAN_POINT ( 'NONE',  ( -16.89925026227929195, -0.1191753592594197858, 13.49466922669627422 ) ) ;
#42534=ADVANCED_FACE ( 'NONE', ( #9144 ), #30173, .F. ) ;
#42535=CARTESIAN_POINT ( 'NONE',  ( -18.66354898467281132, 0.000000000000000000, 14.21960318569776582 ) ) ;
#42537=EDGE_LOOP ( 'NONE', ( #37620, #19231, #37030, #19616 ) ) ;
#42539=ORIENTED_EDGE ( 'NONE', *, *, #53904, .F. ) ;
#42540=ADVANCED_FACE ( 'NONE', ( #21383 ), #52328, .F. ) ;
#42541=CARTESIAN_POINT ( 'NONE',  ( -23.33849165029409889, 0.000000000000000000, 5.946783852668351855 ) ) ;
#42542=CARTESIAN_POINT ( 'NONE',  ( -14.99479423072147455, 5.467268677019013978, 2.331984540967731334 ) ) ;
#42543=CARTESIAN_POINT ( 'NONE',  ( -14.00280974873554030, 0.000000000000000000, 12.40921378708904044 ) ) ;
#42544=LINE ( 'NONE', #11861, #42181 ) ;
#42545=CARTESIAN_POINT ( 'NONE',  ( -12.83240616472669338, -4.241740624735664156, 1.730529728029736036 ) ) ;
#42546=EDGE_CURVE ( 'NONE', #43321, #26517, #38716, .T. ) ;
#42547=CARTESIAN_POINT ( 'NONE',  ( -11.21979143729918960, -0.1191753592594197858, 1.139774444304266554 ) ) ;
#42548=ORIENTED_EDGE ( 'NONE', *, *, #50856, .F. ) ;
#42549=CARTESIAN_POINT ( 'NONE',  ( -17.85712253972278418, 0.000000000000000000, 4.312106799082268793 ) ) ;
#42551=LINE ( 'NONE', #7933, #7672 ) ;
#42552=DIRECTION ( 'NONE',  ( 0.5449076811759707706, 0.6444004775717708799, -0.5364919789714476250 ) ) ;
#42553=DIRECTION ( 'NONE',  ( 0.000000000000000000, -0.000000000000000000, -1.000000000000000000 ) ) ;
#42554=CARTESIAN_POINT ( 'NONE',  ( -16.06709938707323460, 0.000000000000000000, 13.13181314741652628 ) ) ;
#42555=DIRECTION ( 'NONE',  ( -0.9999697198139514409, -0.000000000000000000, -0.007781995580013368816 ) ) ;
#42556=LINE ( 'NONE', #46235, #55555 ) ;
#42557=ORIENTED_EDGE ( 'NONE', *, *, #35791, .F. ) ;
#42558=DIRECTION ( 'NONE',  ( 0.000000000000000000, -1.000000000000000000, 0.000000000000000000 ) ) ;
#42559=DIRECTION ( 'NONE',  ( -0.5364919789714478471, 0.6444004775717705469, -0.5449076811759709926 ) ) ;
#42560=ORIENTED_EDGE ( 'NONE', *, *, #22172, .T. ) ;
#42561=ORIENTED_EDGE ( 'NONE', *, *, #40713, .F. ) ;
#42562=LINE ( 'NONE', #24662, #7440 ) ;
#42563=ORIENTED_EDGE ( 'NONE', *, *, #34302, .T. ) ;
#42564=LINE ( 'NONE', #50795, #17498 ) ;
#42565=VERTEX_POINT ( 'NONE', #42660 ) ;
#42566=ORIENTED_EDGE ( 'NONE', *, *, #27915, .T. ) ;
#42567=VERTEX_POINT ( 'NONE', #29901 ) ;
#42568=DIRECTION ( 'NONE',  ( -0.005961354470445682716, -0.6427876096865404731, 0.7660212471507180654 ) ) ;
#42570=DIRECTION ( 'NONE',  ( 0.5364919789714477361, 0.6444004775717706579, 0.5449076811759711036 ) ) ;
#42571=EDGE_CURVE ( 'NONE', #33755, #11370, #55731, .T. ) ;
#42572=ORIENTED_EDGE ( 'NONE', *, *, #7329, .F. ) ;
#42574=ADVANCED_FACE ( 'NONE', ( #34177 ), #52025, .F. ) ;
#42575=EDGE_CURVE ( 'NONE', #44124, #38604, #16846, .T. ) ;
#42576=DIRECTION ( 'NONE',  ( 0.000000000000000000, -0.000000000000000000, -1.000000000000000000 ) ) ;
#42577=DIRECTION ( 'NONE',  ( 0.000000000000000000, -0.000000000000000000, -1.000000000000000000 ) ) ;
#42578=ORIENTED_EDGE ( 'NONE', *, *, #52422, .T. ) ;
#42579=PLANE ( 'NONE',  #40944 ) ;
#42580=CARTESIAN_POINT ( 'NONE',  ( -8.975993561185934055, -0.1191753592594197858, 10.41700724906143982 ) ) ;
#42582=DIRECTION ( 'NONE',  ( 0.000000000000000000, -1.000000000000000000, 0.000000000000000000 ) ) ;
#42583=CARTESIAN_POINT ( 'NONE',  ( -12.73174640694442772, 0.000000000000000000, 2.505333312241550647 ) ) ;
#42586=CARTESIAN_POINT ( 'NONE',  ( -15.96710241509184058, -0.1191753592594218814, 13.13259134697452879 ) ) ;
#42587=LINE ( 'NONE', #34928, #70 ) ;
#42588=ORIENTED_EDGE ( 'NONE', *, *, #14681, .F. ) ;
#42589=CARTESIAN_POINT ( 'NONE',  ( -21.47419595591918906, 0.000000000000000000, 5.222628093224860102 ) ) ;
#42590=DIRECTION ( 'NONE',  ( -0.5364919789714478471, 0.6444004775717705469, -0.5449076811759709926 ) ) ;
#42591=LINE ( 'NONE', #26130, #54740 ) ;
#42592=CARTESIAN_POINT ( 'NONE',  ( -26.13493519185646008, 0.000000000000000000, 7.033017491833586377 ) ) ;
#42593=ORIENTED_EDGE ( 'NONE', *, *, #44122, .T. ) ;
#42595=CARTESIAN_POINT ( 'NONE',  ( -20.06177075545399191, 0.000000000000000000, 14.76272000528038220 ) ) ;
#42596=DIRECTION ( 'NONE',  ( 0.005961354470445682716, -0.6427876096865404731, -0.7660212471507180654 ) ) ;
#42597=PLANE ( 'NONE',  #41342 ) ;
#42598=EDGE_CURVE ( 'NONE', #36178, #29020, #17119, .T. ) ;
#42599=CARTESIAN_POINT ( 'NONE',  ( -17.26532721389163072, 0.000000000000000000, 13.67648636611514590 ) ) ;
#42600=DIRECTION ( 'NONE',  ( 0.000000000000000000, -0.000000000000000000, -1.000000000000000000 ) ) ;
#42601=CARTESIAN_POINT ( 'NONE',  ( -21.60897430903675698, -3.594132820645662196, 5.160308928338091405 ) ) ;
#42602=ORIENTED_EDGE ( 'NONE', *, *, #55119, .T. ) ;
#42603=EDGE_CURVE ( 'NONE', #3706, #46700, #4357, .T. ) ;
#42605=EDGE_LOOP ( 'NONE', ( #41350, #50997, #34595, #25943 ) ) ;
#42606=DIRECTION ( 'NONE',  ( -0.6427681459581293666, -0.7660444431189770143, -0.005002170337467561935 ) ) ;
#42608=EDGE_CURVE ( 'NONE', #329, #3917, #38976, .T. ) ;
#42609=CARTESIAN_POINT ( 'NONE',  ( -27.99767448711536133, 0.000000000000000000, 7.557179307314289218 ) ) ;
#42610=PLANE ( 'NONE',  #31485 ) ;
#42611=DIRECTION ( 'NONE',  ( -0.5449076811759708816, 0.6444004775717707689, 0.5364919789714475140 ) ) ;
#42612=EDGE_LOOP ( 'NONE', ( #39570, #14938, #54556, #874 ) ) ;
#42613=VECTOR ( 'NONE', #44487, 1000.000000000000227 ) ;
#42614=EDGE_LOOP ( 'NONE', ( #26244, #36345, #10217, #25613, #27618 ) ) ;
#42615=CARTESIAN_POINT ( 'NONE',  ( -14.01623497886155256, -0.1191753592594197858, 2.226008083469502630 ) ) ;
#42616=DIRECTION ( 'NONE',  ( 0.5449076811759707706, 0.6444004775717708799, -0.5364919789714476250 ) ) ;
#42618=CARTESIAN_POINT ( 'NONE',  ( -23.33849165029409889, 0.000000000000000000, 5.946783852668351855 ) ) ;
#42619=ORIENTED_EDGE ( 'NONE', *, *, #7955, .T. ) ;
#42620=DIRECTION ( 'NONE',  ( 0.005002170337468016433, -0.7660444431189770143, -0.6427681459581293666 ) ) ;
#42621=ORIENTED_EDGE ( 'NONE', *, *, #14260, .T. ) ;
#42622=LINE ( 'NONE', #42058, #11170 ) ;
#42623=ORIENTED_EDGE ( 'NONE', *, *, #25404, .T. ) ;
#42624=VERTEX_POINT ( 'NONE', #30747 ) ;
#42625=ORIENTED_EDGE ( 'NONE', *, *, #4792, .F. ) ;
#42626=CARTESIAN_POINT ( 'NONE',  ( 0.000000000000000000, -1.000000000000000000, 2.125000000000000000 ) ) ;
#42627=ADVANCED_FACE ( 'NONE', ( #643 ), #17378, .F. ) ;
#42628=CARTESIAN_POINT ( 'NONE',  ( 2.072287782118878319, 0.000000000000000000, -2.950529333540147015 ) ) ;
#42629=CARTESIAN_POINT ( 'NONE',  ( -23.33849165029409889, 0.000000000000000000, 5.946783852668351855 ) ) ;
#42630=ADVANCED_FACE ( 'NONE', ( #43777 ), #21919, .F. ) ;
#42631=PLANE ( 'NONE',  #7638 ) ;
#42632=VERTEX_POINT ( 'NONE', #17677 ) ;
#42633=EDGE_CURVE ( 'NONE', #40102, #10235, #337, .T. ) ;
#42634=ORIENTED_EDGE ( 'NONE', *, *, #1060, .F. ) ;
#42635=ORIENTED_EDGE ( 'NONE', *, *, #55593, .F. ) ;
#42636=CARTESIAN_POINT ( 'NONE',  ( -19.39010111284826365, -0.1191753592594167188, 7.724168461730136492 ) ) ;
#42637=LINE ( 'NONE', #7736, #52118 ) ;
#42639=DIRECTION ( 'NONE',  ( -0.6427681459581293666, -0.7660444431189770143, -0.005002170337467561935 ) ) ;
#42640=ORIENTED_EDGE ( 'NONE', *, *, #21168, .T. ) ;
#42642=LINE ( 'NONE', #8584, #5872 ) ;
#42643=ORIENTED_EDGE ( 'NONE', *, *, #55028, .F. ) ;
#42644=FACE_OUTER_BOUND ( 'NONE', #17220, .T. ) ;
#42645=ORIENTED_EDGE ( 'NONE', *, *, #23052, .F. ) ;
#42646=ADVANCED_FACE ( 'NONE', ( #29642 ), #35547, .F. ) ;
#42647=VECTOR ( 'NONE', #20481, 1000.000000000000000 ) ;
#42648=CARTESIAN_POINT ( 'NONE',  ( -17.74560456716937296, 0.000000000000000000, 3.774316574337878372 ) ) ;
#42649=FACE_OUTER_BOUND ( 'NONE', #20769, .T. ) ;
#42650=EDGE_LOOP ( 'NONE', ( #7740, #54794, #7621, #20852 ) ) ;
#42651=DIRECTION ( 'NONE',  ( -0.7660212471507179544, -0.6427876096865405842, -0.005961354470445141482 ) ) ;
#42652=CARTESIAN_POINT ( 'NONE',  ( -28.93137873341882127, 0.000000000000000000, 8.119251130998824451 ) ) ;
#42653=CARTESIAN_POINT ( 'NONE',  ( -10.47421230394850866, 0.000000000000000000, 10.95934586908605723 ) ) ;
#42654=FACE_OUTER_BOUND ( 'NONE', #31054, .T. ) ;
#42655=ORIENTED_EDGE ( 'NONE', *, *, #1045, .F. ) ;
#42656=VERTEX_POINT ( 'NONE', #36133 ) ;
#42657=DIRECTION ( 'NONE',  ( -0.9999697198139514409, -0.000000000000000000, -0.007781995580013368816 ) ) ;
#42659=CARTESIAN_POINT ( 'NONE',  ( -16.33317936670417225, 0.000000000000000000, 13.31440848639340224 ) ) ;
#42660=CARTESIAN_POINT ( 'NONE',  ( -13.02956034749683667, 0.000000000000000000, 6.765674479387740803 ) ) ;
#42661=CARTESIAN_POINT ( 'NONE',  ( -13.53673582514181106, 0.000000000000000000, 12.22817484722816772 ) ) ;
#42662=LINE ( 'NONE', #38127, #5921 ) ;
#42663=VERTEX_POINT ( 'NONE', #53434 ) ;
#42665=DIRECTION ( 'NONE',  ( -0.005002170337468016433, -0.7660444431189770143, 0.6427681459581293666 ) ) ;
#42666=CARTESIAN_POINT ( 'NONE',  ( -9.908141408373387193, -0.1191753592594197858, 10.77908512878318703 ) ) ;
#42667=VERTEX_POINT ( 'NONE', #40666 ) ;
#42668=DIRECTION ( 'NONE',  ( 0.7660212471507180654, -0.6427876096865404731, 0.005961354470445141482 ) ) ;
#42669=VERTEX_POINT ( 'NONE', #36383 ) ;
#42670=CARTESIAN_POINT ( 'NONE',  ( -12.60458797795435615, 0.000000000000000000, 11.86609696750642229 ) ) ;
#42671=CARTESIAN_POINT ( 'NONE',  ( -15.86710544311044302, 0.000000000000000000, 13.13336954653252953 ) ) ;
#42672=ADVANCED_FACE ( 'NONE', ( #52858 ), #23602, .F. ) ;
#42673=DIRECTION ( 'NONE',  ( 0.007781995580012663651, 0.000000000000000000, -0.9999697198139515519 ) ) ;
#42675=ORIENTED_EDGE ( 'NONE', *, *, #4907, .T. ) ;
#42676=ORIENTED_EDGE ( 'NONE', *, *, #13986, .T. ) ;
#42677=PLANE ( 'NONE',  #27617 ) ;
#42678=CARTESIAN_POINT ( 'NONE',  ( -26.13493519185646008, 0.000000000000000000, 7.033017491833586377 ) ) ;
#42679=LINE ( 'NONE', #17986, #1615 ) ;
#42680=ADVANCED_FACE ( 'NONE', ( #49158 ), #1737, .F. ) ;
#42682=CARTESIAN_POINT ( 'NONE',  ( -9.873446788527346030, -0.1191753592594185784, 6.320900986966644375 ) ) ;
#42684=CARTESIAN_POINT ( 'NONE',  ( -8.470622023031074477, -0.1191753592594188838, 5.186309231652734830 ) ) ;
#42685=ORIENTED_EDGE ( 'NONE', *, *, #37235, .T. ) ;
#42686=EDGE_CURVE ( 'NONE', #55206, #49405, #53695, .T. ) ;
#42687=LINE ( 'NONE', #55764, #55551 ) ;
#42688=EDGE_CURVE ( 'NONE', #48572, #308, #31295, .T. ) ;
#42689=VECTOR ( 'NONE', #26095, 1000.000000000000227 ) ;
#42690=CARTESIAN_POINT ( 'NONE',  ( -26.13337879274045505, 0.000000000000000000, 6.833023547870798353 ) ) ;
#42691=DIRECTION ( 'NONE',  ( -0.9999697198139514409, -0.000000000000000000, -0.007781995580013368816 ) ) ;
#42692=ORIENTED_EDGE ( 'NONE', *, *, #31628, .F. ) ;
#42693=FACE_OUTER_BOUND ( 'NONE', #45424, .T. ) ;
#42694=EDGE_CURVE ( 'NONE', #37130, #44870, #40918, .T. ) ;
#42695=CARTESIAN_POINT ( 'NONE',  ( -32.65997012216863737, 0.000000000000000000, 9.567562649885804404 ) ) ;
#42696=PLANE ( 'NONE',  #13011 ) ;
#42697=ORIENTED_EDGE ( 'NONE', *, *, #40954, .F. ) ;
#42698=PLANE ( 'NONE',  #32124 ) ;
#42699=ADVANCED_FACE ( 'NONE', ( #32139 ), #30994, .F. ) ;
#42700=ORIENTED_EDGE ( 'NONE', *, *, #8487, .F. ) ;
#42701=EDGE_CURVE ( 'NONE', #7637, #38457, #10272, .T. ) ;
#42702=ORIENTED_EDGE ( 'NONE', *, *, #26869, .T. ) ;
#42703=EDGE_LOOP ( 'NONE', ( #35589, #55854, #52878, #2454 ) ) ;
#42704=ORIENTED_EDGE ( 'NONE', *, *, #30602, .F. ) ;
#42705=CARTESIAN_POINT ( 'NONE',  ( -26.13493519185646008, 0.000000000000000000, 7.033017491833586377 ) ) ;
#42706=ORIENTED_EDGE ( 'NONE', *, *, #29211, .T. ) ;
#42708=EDGE_CURVE ( 'NONE', #883, #22818, #10579, .T. ) ;
#42709=VECTOR ( 'NONE', #9038, 1000.000000000000227 ) ;
#42710=VECTOR ( 'NONE', #33845, 1000.000000000000227 ) ;
#42711=VERTEX_POINT ( 'NONE', #9427 ) ;
#42712=DIRECTION ( 'NONE',  ( -0.005961354470445682716, -0.6427876096865404731, 0.7660212471507180654 ) ) ;
#42713=EDGE_LOOP ( 'NONE', ( #8883, #24255, #33390, #13261 ) ) ;
#42714=EDGE_LOOP ( 'NONE', ( #46554, #46854, #40691, #38473 ) ) ;
#42715=ADVANCED_FACE ( 'NONE', ( #14278 ), #26753, .F. ) ;
#42716=DIRECTION ( 'NONE',  ( 0.9321478471874541372, 0.000000000000000000, -0.3620778797217453771 ) ) ;
#42717=DIRECTION ( 'NONE',  ( 0.9999697198139515519, 0.000000000000000000, 0.007781995580013368816 ) ) ;
#42718=CARTESIAN_POINT ( 'NONE',  ( -14.10280672071693431, -0.1191753592594197858, 12.40843558753103792 ) ) ;
#42719=DIRECTION ( 'NONE',  ( -0.9999697198139514409, -0.000000000000000000, -0.007781995580013368816 ) ) ;
#42720=EDGE_LOOP ( 'NONE', ( #27175, #47450, #14177, #39787 ) ) ;
#42721=ORIENTED_EDGE ( 'NONE', *, *, #47202, .T. ) ;
#42722=VECTOR ( 'NONE', #48823, 999.9999999999998863 ) ;
#42726=VECTOR ( 'NONE', #810, 1000.000000000000227 ) ;
#42727=CARTESIAN_POINT ( 'NONE',  ( -18.15912818816975616, 0.000000000000000000, 9.111073428781198302 ) ) ;
#42728=FACE_OUTER_BOUND ( 'NONE', #39167, .T. ) ;
#42729=LINE ( 'NONE', #34249, #2263 ) ;
#42730=CARTESIAN_POINT ( 'NONE',  ( -20.05622291350217523, 5.305366725996512045, 13.37884985175888097 ) ) ;
#42731=VERTEX_POINT ( 'NONE', #5731 ) ;
#42732=LINE ( 'NONE', #33949, #6599 ) ;
#42733=FACE_OUTER_BOUND ( 'NONE', #51289, .T. ) ;
#42734=VERTEX_POINT ( 'NONE', #9991 ) ;
#42735=DIRECTION ( 'NONE',  ( 0.6427681459581294776, -0.7660444431189769032, 0.005002170337467562802 ) ) ;
#42736=DIRECTION ( 'NONE',  ( 0.000000000000000000, -0.000000000000000000, -1.000000000000000000 ) ) ;
#42737=ADVANCED_FACE ( 'NONE', ( #27299 ), #27595, .F. ) ;
#42738=PLANE ( 'NONE',  #34997 ) ;
#42739=CARTESIAN_POINT ( 'NONE',  ( -13.27065584551087163, 0.000000000000000000, 12.04557950825129176 ) ) ;
#42740=VERTEX_POINT ( 'NONE', #40377 ) ;
#42741=ORIENTED_EDGE ( 'NONE', *, *, #53268, .F. ) ;
#42742=CARTESIAN_POINT ( 'NONE',  ( -13.61183992779837304, 1.581621852479004442, 4.764332917083475394 ) ) ;
#42744=LINE ( 'NONE', #17200, #35159 ) ;
#42745=ADVANCED_FACE ( 'NONE', ( #44613 ), #5194, .F. ) ;
#42746=VECTOR ( 'NONE', #11560, 1000.000000000000227 ) ;
#42747=VECTOR ( 'NONE', #2502, 999.9999999999998863 ) ;
#42748=DIRECTION ( 'NONE',  ( 0.007781995580012662783, 0.000000000000000000, -0.9999697198139514409 ) ) ;
#42749=DIRECTION ( 'NONE',  ( -0.005961354470445682716, -0.6427876096865404731, 0.7660212471507180654 ) ) ;
#42750=LINE ( 'NONE', #139, #19206 ) ;
#42751=LINE ( 'NONE', #3856, #27476 ) ;
#42752=EDGE_CURVE ( 'NONE', #51326, #12359, #2000, .T. ) ;
#42754=DIRECTION ( 'NONE',  ( 0.007781995580012662783, 0.000000000000000000, -0.9999697198139514409 ) ) ;
#42755=VECTOR ( 'NONE', #16001, 999.9999999999998863 ) ;
#42756=LINE ( 'NONE', #2723, #47378 ) ;
#42757=EDGE_LOOP ( 'NONE', ( #48693, #31041, #25396, #48819 ) ) ;
#42758=LINE ( 'NONE', #49945, #20425 ) ;
#42759=ORIENTED_EDGE ( 'NONE', *, *, #50126, .T. ) ;
#42760=EDGE_CURVE ( 'NONE', #54234, #26894, #52583, .T. ) ;
#42761=ORIENTED_EDGE ( 'NONE', *, *, #26611, .T. ) ;
#42762=VECTOR ( 'NONE', #22959, 1000.000000000000227 ) ;
#42763=ADVANCED_FACE ( 'NONE', ( #897 ), #55114, .F. ) ;
#42764=ORIENTED_EDGE ( 'NONE', *, *, #52400, .F. ) ;
#42765=ORIENTED_EDGE ( 'NONE', *, *, #53265, .T. ) ;
#42766=ORIENTED_EDGE ( 'NONE', *, *, #43866, .T. ) ;
#42767=VERTEX_POINT ( 'NONE', #37214 ) ;
#42768=CARTESIAN_POINT ( 'NONE',  ( -19.41128072241421165, -4.241740624735661491, 11.18335138056985834 ) ) ;
#42769=FACE_OUTER_BOUND ( 'NONE', #13923, .T. ) ;
#42770=CARTESIAN_POINT ( 'NONE',  ( -20.54049170961573267, 0.000000000000000000, 4.660556269540326646 ) ) ;
#42771=ADVANCED_FACE ( 'NONE', ( #36967 ), #15928, .F. ) ;
#42772=ORIENTED_EDGE ( 'NONE', *, *, #19666, .F. ) ;
#42773=DIRECTION ( 'NONE',  ( 0.9999697198139515519, 0.000000000000000000, 0.007781995580013368816 ) ) ;
#42774=EDGE_LOOP ( 'NONE', ( #39876, #21912, #54844, #53492 ) ) ;
#42775=DIRECTION ( 'NONE',  ( 0.005961354470445682716, -0.6427876096865404731, -0.7660212471507180654 ) ) ;
#42776=ORIENTED_EDGE ( 'NONE', *, *, #44688, .T. ) ;
#42777=EDGE_CURVE ( 'NONE', #21762, #17219, #10831, .T. ) ;
#42779=PLANE ( 'NONE',  #50824 ) ;
#42780=CARTESIAN_POINT ( 'NONE',  ( -19.60990026154428278, 0.000000000000000000, 4.498472333781370125 ) ) ;
#42782=PLANE ( 'NONE',  #54582 ) ;
#42783=ORIENTED_EDGE ( 'NONE', *, *, #6754, .T. ) ;
#42784=VECTOR ( 'NONE', #13453, 999.9999999999998863 ) ;
#42785=VECTOR ( 'NONE', #10824, 999.9999999999998863 ) ;
#42786=CARTESIAN_POINT ( 'NONE',  ( -18.67619601524082285, 0.000000000000000000, 3.936400510096834893 ) ) ;
#42787=FACE_OUTER_BOUND ( 'NONE', #16171, .T. ) ;
#42788=CARTESIAN_POINT ( 'NONE',  ( -18.39746900504187010, 0.000000000000000000, 14.03700784672088808 ) ) ;
#42789=AXIS2_PLACEMENT_3D ( 'NONE', #4285, #42870, #42334 ) ;
#42790=CARTESIAN_POINT ( 'NONE',  ( -18.25128119919330416, -0.1191753592594153865, 8.102363091431291409 ) ) ;
#42791=CARTESIAN_POINT ( 'NONE',  ( -10.89619124762234392, 0.000000000000000000, 5.474274585375703772 ) ) ;
#42792=CARTESIAN_POINT ( 'NONE',  ( -10.27421835998572064, 0.000000000000000000, 10.96090226820206048 ) ) ;
#42793=CARTESIAN_POINT ( 'NONE',  ( -14.87505532172404443, 0.000000000000000000, 5.073978075321856629 ) ) ;
#42797=ORIENTED_EDGE ( 'NONE', *, *, #20200, .F. ) ;
#42798=ADVANCED_FACE ( 'NONE', ( #19898 ), #29254, .F. ) ;
#42799=CARTESIAN_POINT ( 'NONE',  ( -15.13495153988577968, 0.000000000000000000, 12.76973526769478084 ) ) ;
#42800=LINE ( 'NONE', #46495, #16008 ) ;
#42801=PLANE ( 'NONE',  #54405 ) ;
#42802=VECTOR ( 'NONE', #5577, 1000.000000000000227 ) ;
#42803=EDGE_CURVE ( 'NONE', #45114, #26051, #46281, .T. ) ;
#42804=CARTESIAN_POINT ( 'NONE',  ( -18.68432617547731311, -0.1191753592594153865, 4.039253233279383792 ) ) ;
#42805=CARTESIAN_POINT ( 'NONE',  ( 2.072287782118878319, 0.000000000000000000, -2.950529333540147015 ) ) ;
#42806=AXIS2_PLACEMENT_3D ( 'NONE', #33442, #35336, #38834 ) ;
#42807=LINE ( 'NONE', #43650, #45663 ) ;
#42809=ORIENTED_EDGE ( 'NONE', *, *, #47724, .F. ) ;
#42810=ADVANCED_FACE ( 'NONE', ( #54519 ), #41496, .F. ) ;
#42811=CARTESIAN_POINT ( 'NONE',  ( -11.64271541837342028, 0.000000000000000000, 7.684457380502274226 ) ) ;
#42812=DIRECTION ( 'NONE',  ( 0.5364919789714477361, 0.6444004775717706579, 0.5449076811759711036 ) ) ;
#42813=LINE ( 'NONE', #41692, #49939 ) ;
#42814=EDGE_CURVE ( 'NONE', #45339, #46146, #16205, .T. ) ;
#42815=EDGE_CURVE ( 'NONE', #53717, #37763, #32676, .T. ) ;
#42816=EDGE_CURVE ( 'NONE', #3505, #22811, #20469, .T. ) ;
#42818=PLANE ( 'NONE',  #29352 ) ;
#42819=VECTOR ( 'NONE', #7622, 999.9999999999998863 ) ;
#42820=FACE_OUTER_BOUND ( 'NONE', #40195, .T. ) ;
#42822=EDGE_LOOP ( 'NONE', ( #54496, #19118, #32658, #12594 ) ) ;
#42823=CARTESIAN_POINT ( 'NONE',  ( -26.13493519185646008, 0.000000000000000000, 7.033017491833586377 ) ) ;
#42824=PLANE ( 'NONE',  #4224 ) ;
#42825=VERTEX_POINT ( 'NONE', #6563 ) ;
#42826=VECTOR ( 'NONE', #7802, 1000.000000000000227 ) ;
#42827=ORIENTED_EDGE ( 'NONE', *, *, #16103, .F. ) ;
#42828=DIRECTION ( 'NONE',  ( 0.005002170337468016433, -0.7660444431189770143, -0.6427681459581293666 ) ) ;
#42829=VECTOR ( 'NONE', #25802, 999.9999999999998863 ) ;
#42831=AXIS2_PLACEMENT_3D ( 'NONE', #28714, #6850, #7128 ) ;
#42832=ORIENTED_EDGE ( 'NONE', *, *, #12093, .F. ) ;
#42833=ADVANCED_FACE ( 'NONE', ( #42338 ), #23877, .F. ) ;
#42834=EDGE_CURVE ( 'NONE', #41663, #15067, #36674, .T. ) ;
#42835=VECTOR ( 'NONE', #20710, 1000.000000000000227 ) ;
#42836=VERTEX_POINT ( 'NONE', #11669 ) ;
#42837=VERTEX_POINT ( 'NONE', #32963 ) ;
#42838=VECTOR ( 'NONE', #17537, 1000.000000000000227 ) ;
#42840=EDGE_CURVE ( 'NONE', #30427, #54774, #32432, .T. ) ;
#42841=CARTESIAN_POINT ( 'NONE',  ( -16.46071592345537127, -2.460819163488160655, 3.196709174999311731 ) ) ;
#42842=VERTEX_POINT ( 'NONE', #2833 ) ;
#42843=DIRECTION ( 'NONE',  ( -0.005961354470445682716, -0.6427876096865404731, 0.7660212471507180654 ) ) ;
#42844=CARTESIAN_POINT ( 'NONE',  ( -22.40634380310664397, 0.000000000000000000, 5.584705972946605534 ) ) ;
#42846=ORIENTED_EDGE ( 'NONE', *, *, #40665, .T. ) ;
#42847=AXIS2_PLACEMENT_3D ( 'NONE', #4125, #48383, #17176 ) ;
#42848=ORIENTED_EDGE ( 'NONE', *, *, #18039, .F. ) ;
#42849=EDGE_CURVE ( 'NONE', #15326, #18261, #41743, .T. ) ;
#42851=CARTESIAN_POINT ( 'NONE',  ( -17.86419527468779123, 5.467268677019012202, 12.79310055922187495 ) ) ;
#42852=VERTEX_POINT ( 'NONE', #20161 ) ;
#42853=LINE ( 'NONE', #30083, #14654 ) ;
#42854=LINE ( 'NONE', #17040, #34058 ) ;
#42855=EDGE_LOOP ( 'NONE', ( #38756, #14011, #12514, #26153 ) ) ;
#42856=LINE ( 'NONE', #20992, #4031 ) ;
#42857=ORIENTED_EDGE ( 'NONE', *, *, #10154, .T. ) ;
#42858=CARTESIAN_POINT ( 'NONE',  ( -14.20280369269832832, 0.000000000000000000, 12.40765738797303719 ) ) ;
#42860=DIRECTION ( 'NONE',  ( -0.5449076811759708816, 0.6444004775717707689, 0.5364919789714475140 ) ) ;
#42861=EDGE_LOOP ( 'NONE', ( #36749, #35274, #27059, #46110 ) ) ;
#42862=CARTESIAN_POINT ( 'NONE',  ( -12.13851405436063047, 0.000000000000000000, 11.68505802764555135 ) ) ;
#42863=CARTESIAN_POINT ( 'NONE',  ( -13.08408713167409942, -0.1191753592594197858, 1.863930203747758085 ) ) ;
#42864=LINE ( 'NONE', #12773, #52977 ) ;
#42865=VECTOR ( 'NONE', #35881, 1000.000000000000227 ) ;
#42866=CARTESIAN_POINT ( 'NONE',  ( -13.59275766711197519, -3.432230869623159819, 7.594696008263455589 ) ) ;
#42867=ORIENTED_EDGE ( 'NONE', *, *, #37079, .T. ) ;
#42868=VECTOR ( 'NONE', #52323, 1000.000000000000227 ) ;
#42869=VECTOR ( 'NONE', #34311, 999.9999999999998863 ) ;
#42870=DIRECTION ( 'NONE',  ( 0.000000000000000000, -1.000000000000000000, 0.000000000000000000 ) ) ;
#42871=DIRECTION ( 'NONE',  ( 0.7660212471507180654, -0.6427876096865404731, 0.005961354470445141482 ) ) ;
#42872=CARTESIAN_POINT ( 'NONE',  ( -12.28182988935405895, -4.079838673713161334, 8.148321875889408261 ) ) ;
#42873=DIRECTION ( 'NONE',  ( 0.5449076811759707706, 0.6444004775717708799, -0.5364919789714476250 ) ) ;
#42874=LINE ( 'NONE', #3983, #4100 ) ;
#42875=CARTESIAN_POINT ( 'NONE',  ( 2.072287782118878319, 0.000000000000000000, -2.950529333540147015 ) ) ;
#42876=VECTOR ( 'NONE', #15210, 1000.000000000000000 ) ;
#42877=DIRECTION ( 'NONE',  ( -0.5449076811759708816, 0.6444004775717707689, 0.5364919789714475140 ) ) ;
#42878=DIRECTION ( 'NONE',  ( 0.007781995580012663651, 0.000000000000000000, -0.9999697198139515519 ) ) ;
#42879=VECTOR ( 'NONE', #19906, 1000.000000000000227 ) ;
#42880=EDGE_LOOP ( 'NONE', ( #14599, #8426, #774, #20179 ) ) ;
#42882=LINE ( 'NONE', #7396, #20536 ) ;
#42883=EDGE_LOOP ( 'NONE', ( #7827, #28891, #34136, #42894 ) ) ;
#42884=LINE ( 'NONE', #25302, #14800 ) ;
#42885=CARTESIAN_POINT ( 'NONE',  ( -12.77198315601838630, 0.000000000000000000, 7.675669157850252944 ) ) ;
#42886=EDGE_CURVE ( 'NONE', #34831, #26641, #50275, .T. ) ;
#42887=EDGE_CURVE ( 'NONE', #29025, #1604, #50574, .T. ) ;
#42888=DIRECTION ( 'NONE',  ( 0.005961354470445682716, -0.6427876096865404731, -0.7660212471507180654 ) ) ;
#42889=VECTOR ( 'NONE', #49668, 999.9999999999998863 ) ;
#42890=ADVANCED_FACE ( 'NONE', ( #55963 ), #34374, .F. ) ;
#42892=DIRECTION ( 'NONE',  ( -0.005961354470445682716, -0.6427876096865404731, 0.7660212471507180654 ) ) ;
#42894=ORIENTED_EDGE ( 'NONE', *, *, #34388, .T. ) ;
#42895=ORIENTED_EDGE ( 'NONE', *, *, #45115, .F. ) ;
#42896=LINE ( 'NONE', #21331, #54007 ) ;
#42897=FACE_OUTER_BOUND ( 'NONE', #52265, .T. ) ;
#42898=EDGE_LOOP ( 'NONE', ( #21198, #46129, #53658, #48731 ) ) ;
#42899=VECTOR ( 'NONE', #41606, 1000.000000000000227 ) ;
#42900=DIRECTION ( 'NONE',  ( 0.007781995580012663651, 0.000000000000000000, -0.9999697198139515519 ) ) ;
#42901=ORIENTED_EDGE ( 'NONE', *, *, #16202, .F. ) ;
#42902=PLANE ( 'NONE',  #15886 ) ;
#42903=AXIS2_PLACEMENT_3D ( 'NONE', #45219, #49181, #49486 ) ;
#42904=EDGE_LOOP ( 'NONE', ( #32609, #6473, #53711, #6224 ) ) ;
#42906=EDGE_CURVE ( 'NONE', #30294, #35325, #29840, .T. ) ;
#42907=ORIENTED_EDGE ( 'NONE', *, *, #49440, .F. ) ;
#42908=VERTEX_POINT ( 'NONE', #26139 ) ;
#42909=VERTEX_POINT ( 'NONE', #29567 ) ;
#42910=LINE ( 'NONE', #34139, #35684 ) ;
#42911=VECTOR ( 'NONE', #23013, 1000.000000000000000 ) ;
#42912=DIRECTION ( 'NONE',  ( 0.000000000000000000, -1.000000000000000000, 0.000000000000000000 ) ) ;
#42913=CARTESIAN_POINT ( 'NONE',  ( -16.43317633868556626, -0.1191753592594197858, 13.31363028683540151 ) ) ;
#42914=VECTOR ( 'NONE', #32987, 999.9999999999998863 ) ;
#42915=AXIS2_PLACEMENT_3D ( 'NONE', #12925, #21468, #21160 ) ;
#42916=EDGE_CURVE ( 'NONE', #14453, #38228, #43448, .T. ) ;
#42917=FACE_OUTER_BOUND ( 'NONE', #1794, .T. ) ;
#42918=VERTEX_POINT ( 'NONE', #8528 ) ;
#42919=VERTEX_POINT ( 'NONE', #51678 ) ;
#42920=EDGE_CURVE ( 'NONE', #11836, #54577, #21008, .T. ) ;
#42921=AXIS2_PLACEMENT_3D ( 'NONE', #5424, #22734, #18469 ) ;
#42922=VERTEX_POINT ( 'NONE', #7985 ) ;
#42923=DIRECTION ( 'NONE',  ( 0.007781995580012663651, -3.146120232559066537E-19, -0.9999697198139514409 ) ) ;
#42924=AXIS2_PLACEMENT_3D ( 'NONE', #11615, #28934, #46504 ) ;
#42926=DIRECTION ( 'NONE',  ( -0.6427681459581293666, -0.7660444431189770143, -0.005002170337467561935 ) ) ;
#42927=VERTEX_POINT ( 'NONE', #12782 ) ;
#42928=DIRECTION ( 'NONE',  ( 0.005961354470445682716, -0.6427876096865404731, -0.7660212471507180654 ) ) ;
#42929=ADVANCED_FACE ( 'NONE', ( #8240 ), #47986, .F. ) ;
#42930=ORIENTED_EDGE ( 'NONE', *, *, #4194, .F. ) ;
#42931=CARTESIAN_POINT ( 'NONE',  ( -18.28212116572951373, -0.1941918491731542684, 3.976522104704446114 ) ) ;
#42932=PLANE ( 'NONE',  #13114 ) ;
#42933=ORIENTED_EDGE ( 'NONE', *, *, #11182, .F. ) ;
#42934=EDGE_CURVE ( 'NONE', #19674, #44901, #17309, .T. ) ;
#42935=DIRECTION ( 'NONE',  ( 0.5449076811759707706, 0.6444004775717708799, -0.5364919789714476250 ) ) ;
#42937=FACE_OUTER_BOUND ( 'NONE', #2921, .T. ) ;
#42938=LINE ( 'NONE', #26967, #21175 ) ;
#42939=VECTOR ( 'NONE', #39219, 1000.000000000000114 ) ;
#42940=ORIENTED_EDGE ( 'NONE', *, *, #45776, .T. ) ;
#42941=CARTESIAN_POINT ( 'NONE',  ( -18.69774841163365764, -4.565544526780663581, 3.998496804814759109 ) ) ;
#42942=PLANE ( 'NONE',  #40209 ) ;
#42943=DIRECTION ( 'NONE',  ( 0.007781995580012662783, 0.000000000000000000, -0.9999697198139514409 ) ) ;
#42944=ORIENTED_EDGE ( 'NONE', *, *, #2818, .F. ) ;
#42945=VECTOR ( 'NONE', #1084, 1000.000000000000227 ) ;
#42946=DIRECTION ( 'NONE',  ( -0.7660212471507179544, -0.6427876096865405842, -0.005961354470445141482 ) ) ;
#42948=VECTOR ( 'NONE', #18833, 1000.000000000000000 ) ;
#42949=CARTESIAN_POINT ( 'NONE',  ( -36.91819796696599099, -1.000000000000000000, 21.84982018086542155 ) ) ;
#42950=CARTESIAN_POINT ( 'NONE',  ( -17.74404816805336793, 0.000000000000000000, 3.574322630375089460 ) ) ;
#42952=LINE ( 'NONE', #9430, #10462 ) ;
#42954=DIRECTION ( 'NONE',  ( 0.007781995580012663651, 0.000000000000000000, -0.9999697198139515519 ) ) ;
#42955=FACE_OUTER_BOUND ( 'NONE', #1190, .T. ) ;
#42956=DIRECTION ( 'NONE',  ( -0.6427681459581293666, -0.7660444431189770143, -0.005002170337467561935 ) ) ;
#42957=ORIENTED_EDGE ( 'NONE', *, *, #39971, .F. ) ;
#42958=VECTOR ( 'NONE', #50537, 1000.000000000000227 ) ;
#42959=CARTESIAN_POINT ( 'NONE',  ( -9.951229532024482793, 0.000000000000000000, 3.465642133327924146 ) ) ;
#42960=DIRECTION ( 'NONE',  ( 0.000000000000000000, -1.000000000000000000, 0.000000000000000000 ) ) ;
#42961=EDGE_LOOP ( 'NONE', ( #23148, #50996, #55285, #55283 ) ) ;
#42962=VECTOR ( 'NONE', #21658, 1000.000000000000000 ) ;
#42963=EDGE_CURVE ( 'NONE', #22414, #50687, #17605, .T. ) ;
#42965=DIRECTION ( 'NONE',  ( 0.005961354470445682716, -0.6427876096865404731, -0.7660212471507180654 ) ) ;
#42966=EDGE_CURVE ( 'NONE', #41657, #53717, #42874, .T. ) ;
#42967=ADVANCED_FACE ( 'NONE', ( #13370 ), #47418, .F. ) ;
#42968=DIRECTION ( 'NONE',  ( 0.7660212471507180654, -0.6427876096865404731, 0.005961354470445141482 ) ) ;
#42970=ORIENTED_EDGE ( 'NONE', *, *, #24806, .F. ) ;
#42971=VECTOR ( 'NONE', #7339, 1000.000000000000227 ) ;
#42972=VECTOR ( 'NONE', #7623, 999.9999999999998863 ) ;
#42973=ORIENTED_EDGE ( 'NONE', *, *, #37010, .F. ) ;
#42975=PLANE ( 'NONE',  #32258 ) ;
#42976=DIRECTION ( 'NONE',  ( 0.7660212471507180654, -0.6427876096865404731, 0.005961354470445141482 ) ) ;
#42977=DIRECTION ( 'NONE',  ( -0.7660212471507179544, -0.6427876096865405842, -0.005961354470445141482 ) ) ;
#42978=CARTESIAN_POINT ( 'NONE',  ( -22.40478740399063895, 0.000000000000000000, 5.384712028983816623 ) ) ;
#42979=CARTESIAN_POINT ( 'NONE',  ( -13.46964841717965911, 0.000000000000000000, 3.607586997594828038 ) ) ;
#42980=ORIENTED_EDGE ( 'NONE', *, *, #18388, .T. ) ;
#42981=PLANE ( 'NONE',  #5667 ) ;
#42982=EDGE_CURVE ( 'NONE', #25199, #6556, #38917, .T. ) ;
#42983=CARTESIAN_POINT ( 'NONE',  ( -17.46139143058123011, 5.629170628041515023, 3.284929139499369377 ) ) ;
#42984=ORIENTED_EDGE ( 'NONE', *, *, #28483, .F. ) ;
#42985=VECTOR ( 'NONE', #51157, 999.9999999999998863 ) ;
#42986=FACE_OUTER_BOUND ( 'NONE', #47248, .T. ) ;
#42988=AXIS2_PLACEMENT_3D ( 'NONE', #18024, #35346, #52645 ) ;
#42989=DIRECTION ( 'NONE',  ( 0.007781995580012663651, 0.000000000000000000, -0.9999697198139515519 ) ) ;
#42990=ORIENTED_EDGE ( 'NONE', *, *, #51483, .F. ) ;
#42991=CARTESIAN_POINT ( 'NONE',  ( -10.23443446032375270, 0.000000000000000000, 5.848756599517480836 ) ) ;
#42992=VECTOR ( 'NONE', #21791, 1000.000000000000114 ) ;
#42993=VERTEX_POINT ( 'NONE', #52259 ) ;
#42994=ADVANCED_FACE ( 'NONE', ( #3692 ), #8835, .F. ) ;
#42995=EDGE_LOOP ( 'NONE', ( #27409, #37670, #29813, #50631 ) ) ;
#42996=EDGE_LOOP ( 'NONE', ( #3536, #7695, #28572, #26176 ) ) ;
#42997=ORIENTED_EDGE ( 'NONE', *, *, #17056, .F. ) ;
#42998=AXIS2_PLACEMENT_3D ( 'NONE', #37247, #41242, #32461 ) ;
#42999=DIRECTION ( 'NONE',  ( -0.005961354470445682716, -0.6427876096865404731, 0.7660212471507180654 ) ) ;
#43000=ORIENTED_EDGE ( 'NONE', *, *, #23298, .F. ) ;
#43003=ORIENTED_EDGE ( 'NONE', *, *, #9277, .T. ) ;
#43005=ADVANCED_FACE ( 'NONE', ( #20748 ), #38064, .F. ) ;
#43006=ORIENTED_EDGE ( 'NONE', *, *, #32491, .T. ) ;
#43007=CARTESIAN_POINT ( 'NONE',  ( -11.20636620717317378, 0.000000000000000000, 11.32298014792380414 ) ) ;
#43008=ORIENTED_EDGE ( 'NONE', *, *, #5494, .T. ) ;
#43009=AXIS2_PLACEMENT_3D ( 'NONE', #29198, #12166, #29503 ) ;
#43010=VECTOR ( 'NONE', #50448, 1000.000000000000227 ) ;
#43011=DIRECTION ( 'NONE',  ( 0.2426528472758542054, 0.7422098413412800966, 0.6246952433987894571 ) ) ;
#43012=CARTESIAN_POINT ( 'NONE',  ( -15.34831437908097840, 0.000000000000000000, 6.178291273327141120 ) ) ;
#43014=CARTESIAN_POINT ( 'NONE',  ( 2.072287782118878319, 0.000000000000000000, -2.950529333540147015 ) ) ;
#43015=CARTESIAN_POINT ( 'NONE',  ( -9.342070512798265725, 0.000000000000000000, 10.59882438848031505 ) ) ;
#43016=ORIENTED_EDGE ( 'NONE', *, *, #44966, .T. ) ;
#43017=EDGE_CURVE ( 'NONE', #2042, #2367, #25295, .T. ) ;
#43018=ORIENTED_EDGE ( 'NONE', *, *, #38217, .F. ) ;
#43019=LINE ( 'NONE', #48107, #4107 ) ;
#43020=DIRECTION ( 'NONE',  ( 0.005961354470445682716, -0.6427876096865404731, -0.7660212471507180654 ) ) ;
#43021=EDGE_CURVE ( 'NONE', #294, #26160, #16766, .T. ) ;
#43022=ADVANCED_FACE ( 'NONE', ( #12522 ), #49386, .F. ) ;
#43023=DIRECTION ( 'NONE',  ( 0.5449076811759707706, 0.6444004775717708799, -0.5364919789714476250 ) ) ;
#43024=VECTOR ( 'NONE', #3815, 1000.000000000000114 ) ;
#43025=CARTESIAN_POINT ( 'NONE',  ( -15.52818994850678891, 0.000000000000000000, 3.591566951406786057 ) ) ;
#43026=AXIS2_PLACEMENT_3D ( 'NONE', #13050, #8224, #38615 ) ;
#43027=CARTESIAN_POINT ( 'NONE',  ( -17.74482636761137044, -0.1191753592594197858, 3.674319602356483916 ) ) ;
#43028=CARTESIAN_POINT ( 'NONE',  ( -14.77973024485960529, 4.657758921906512306, 2.274273984692230410 ) ) ;
#43029=ORIENTED_EDGE ( 'NONE', *, *, #27384, .F. ) ;
#43030=FACE_OUTER_BOUND ( 'NONE', #44300, .T. ) ;
#43031=ADVANCED_FACE ( 'NONE', ( #14213 ), #13896, .F. ) ;
#43033=VECTOR ( 'NONE', #26453, 1000.000000000000227 ) ;
#43034=ORIENTED_EDGE ( 'NONE', *, *, #18897, .T. ) ;
#43036=DIRECTION ( 'NONE',  ( 0.5449076811759707706, 0.6444004775717708799, -0.5364919789714476250 ) ) ;
#43037=ADVANCED_FACE ( 'NONE', ( #48839 ), #14741, .F. ) ;
#43038=DIRECTION ( 'NONE',  ( 0.007781995580012663651, 0.000000000000000000, -0.9999697198139515519 ) ) ;
#43039=EDGE_CURVE ( 'NONE', #47891, #36269, #53633, .T. ) ;
#43040=CARTESIAN_POINT ( 'NONE',  ( -11.50282600055954951, -2.622721114510657703, 5.454352154844033684 ) ) ;
#43041=ORIENTED_EDGE ( 'NONE', *, *, #8680, .F. ) ;
#43042=VECTOR ( 'NONE', #43326, 999.9999999999998863 ) ;
#43043=ORIENTED_EDGE ( 'NONE', *, *, #34523, .T. ) ;
#43044=VECTOR ( 'NONE', #37129, 1000.000000000000227 ) ;
#43045=PLANE ( 'NONE',  #45708 ) ;
#43046=DIRECTION ( 'NONE',  ( 0.000000000000000000, -1.000000000000000000, 0.000000000000000000 ) ) ;
#43047=DIRECTION ( 'NONE',  ( 0.007781995580012663651, 0.000000000000000000, -0.9999697198139515519 ) ) ;
#43048=VECTOR ( 'NONE', #6364, 1000.000000000000227 ) ;
#43049=EDGE_CURVE ( 'NONE', #19374, #48095, #27239, .T. ) ;
#43050=DIRECTION ( 'NONE',  ( 0.9999697198139515519, 0.000000000000000000, 0.007781995580013368816 ) ) ;
#43051=FACE_OUTER_BOUND ( 'NONE', #37068, .T. ) ;
#43052=CARTESIAN_POINT ( 'NONE',  ( -19.72849096906270105, 5.467268677019012202, 13.51725631866536759 ) ) ;
#43053=FACE_OUTER_BOUND ( 'NONE', #23518, .T. ) ;
#43054=ORIENTED_EDGE ( 'NONE', *, *, #41656, .T. ) ;
#43055=EDGE_CURVE ( 'NONE', #42382, #2545, #32071, .T. ) ;
#43056=AXIS2_PLACEMENT_3D ( 'NONE', #9457, #52052, #52891 ) ;
#43057=DIRECTION ( 'NONE',  ( 0.6427681459581294776, -0.7660444431189769032, 0.005002170337467562802 ) ) ;
#43058=AXIS2_PLACEMENT_3D ( 'NONE', #4505, #42558, #47945 ) ;
#43059=FACE_OUTER_BOUND ( 'NONE', #30724, .T. ) ;
#43060=CARTESIAN_POINT ( 'NONE',  ( -14.98365774870343969, -1.813211359398158029, 2.643631698368467564 ) ) ;
#43061=VERTEX_POINT ( 'NONE', #4823 ) ;
#43062=DIRECTION ( 'NONE',  ( 0.5364919789714477361, 0.6444004775717706579, 0.5449076811759711036 ) ) ;
#43063=ORIENTED_EDGE ( 'NONE', *, *, #41556, .F. ) ;
#43064=VERTEX_POINT ( 'NONE', #23283 ) ;
#43065=AXIS2_PLACEMENT_3D ( 'NONE', #19846, #45147, #7087 ) ;
#43066=ORIENTED_EDGE ( 'NONE', *, *, #27602, .F. ) ;
#43067=ORIENTED_EDGE ( 'NONE', *, *, #35806, .F. ) ;
#43068=ORIENTED_EDGE ( 'NONE', *, *, #1850, .F. ) ;
#43069=VECTOR ( 'NONE', #35992, 1000.000000000000114 ) ;
#43070=ORIENTED_EDGE ( 'NONE', *, *, #43536, .F. ) ;
#43071=CARTESIAN_POINT ( 'NONE',  ( -27.06552663992790997, 0.000000000000000000, 7.195101427592543786 ) ) ;
#43072=DIRECTION ( 'NONE',  ( -0.9999697198139514409, -0.000000000000000000, -0.007781995580013368816 ) ) ;
#43074=AXIS2_PLACEMENT_3D ( 'NONE', #18591, #18886, #35937 ) ;
#43075=ORIENTED_EDGE ( 'NONE', *, *, #41614, .T. ) ;
#43076=LINE ( 'NONE', #46777, #52146 ) ;
#43077=EDGE_CURVE ( 'NONE', #21645, #46158, #22987, .T. ) ;
#43078=ORIENTED_EDGE ( 'NONE', *, *, #4520, .T. ) ;
#43079=VECTOR ( 'NONE', #26669, 999.9999999999998863 ) ;
#43080=DIRECTION ( 'NONE',  ( 0.7660212471507180654, -0.6427876096865404731, 0.005961354470445141482 ) ) ;
#43081=VERTEX_POINT ( 'NONE', #44551 ) ;
#43082=VECTOR ( 'NONE', #31637, 1000.000000000000114 ) ;
#43083=COLOUR_RGB ( '', 0.31764706, 0.68627451, 0.89019608) ;
#43084=DIRECTION ( 'NONE',  ( -0.6427681459581293666, -0.7660444431189770143, -0.005002170337467561935 ) ) ;
#43085=VECTOR ( 'NONE', #13483, 1000.000000000000227 ) ;
#43086=DIRECTION ( 'NONE',  ( 0.007781995580012662783, 0.000000000000000000, -0.9999697198139514409 ) ) ;
#43087=CARTESIAN_POINT ( 'NONE',  ( -25.20123094555300369, 0.000000000000000000, 6.470945668149052032 ) ) ;
#43088=ORIENTED_EDGE ( 'NONE', *, *, #36318, .T. ) ;
#43089=DIRECTION ( 'NONE',  ( -0.6427681459581293666, -0.7660444431189770143, -0.005002170337467561935 ) ) ;
#43090=ORIENTED_EDGE ( 'NONE', *, *, #40363, .F. ) ;
#43091=VECTOR ( 'NONE', #51951, 999.9999999999998863 ) ;
#43092=ADVANCED_FACE ( 'NONE', ( #44844 ), #31789, .F. ) ;
#43093=DIRECTION ( 'NONE',  ( -0.5449076811759708816, 0.6444004775717707689, 0.5364919789714475140 ) ) ;
#43094=FACE_OUTER_BOUND ( 'NONE', #13480, .T. ) ;
#43095=ADVANCED_FACE ( 'NONE', ( #18439 ), #5963, .F. ) ;
#43096=AXIS2_PLACEMENT_3D ( 'NONE', #7713, #54542, #32989 ) ;
#43097=DIRECTION ( 'NONE',  ( 0.6427681459581294776, -0.7660444431189769032, 0.005002170337467562802 ) ) ;
#43098=AXIS2_PLACEMENT_3D ( 'NONE', #3821, #52644, #34495 ) ;
#43099=CARTESIAN_POINT ( 'NONE',  ( -17.78089619534165067, -0.1191753592594179401, 7.367359596683773937 ) ) ;
#43100=CARTESIAN_POINT ( 'NONE',  ( -17.29258214062169330, -0.6798977022406558213, 3.576654982803652238 ) ) ;
#43101=LINE ( 'NONE', #34021, #34868 ) ;
#43103=CARTESIAN_POINT ( 'NONE',  ( -19.11315273645212898, -1.165603555308155626, 6.019083351294370665 ) ) ;
#43104=VERTEX_POINT ( 'NONE', #39478 ) ;
#43105=DIRECTION ( 'NONE',  ( -0.9999697198139514409, -0.000000000000000000, -0.007781995580013368816 ) ) ;
#43106=ORIENTED_EDGE ( 'NONE', *, *, #49035, .T. ) ;
#43107=DIRECTION ( 'NONE',  ( 0.005002170337468016433, -0.7660444431189770143, -0.6427681459581293666 ) ) ;
#43108=DIRECTION ( 'NONE',  ( -0.3620778797217455991, 0.000000000000000000, -0.9321478471874540261 ) ) ;
#43109=ADVANCED_FACE ( 'NONE', ( #5659 ), #22145, .F. ) ;
#43110=CARTESIAN_POINT ( 'NONE',  ( -20.63393600974853470, -1.327505506330657781, 4.853888218877987271 ) ) ;
#43111=LINE ( 'NONE', #25786, #7828 ) ;
#43112=CARTESIAN_POINT ( 'NONE',  ( -16.65536346919183686, 5.143464774974010112, 11.79213186596540730 ) ) ;
#43113=EDGE_CURVE ( 'NONE', #8976, #41711, #35231, .T. ) ;
#43114=LINE ( 'NONE', #17845, #55871 ) ;
#43115=VECTOR ( 'NONE', #2925, 1000.000000000000227 ) ;
#43116=LINE ( 'NONE', #34033, #3830 ) ;
#43118=VECTOR ( 'NONE', #31353, 999.9999999999998863 ) ;
#43119=ORIENTED_EDGE ( 'NONE', *, *, #15073, .F. ) ;
#43120=CARTESIAN_POINT ( 'NONE',  ( -12.13851405436063047, 0.000000000000000000, 11.68505802764555135 ) ) ;
#43121=CARTESIAN_POINT ( 'NONE',  ( -30.79411802867772607, 0.000000000000000000, 8.643412946479525516 ) ) ;
#43122=DIRECTION ( 'NONE',  ( -0.9999697198139514409, -0.000000000000000000, -0.007781995580013368816 ) ) ;
#43123=VECTOR ( 'NONE', #24311, 1000.000000000000114 ) ;
#43124=EDGE_CURVE ( 'NONE', #5501, #48505, #48244, .T. ) ;
#43125=CARTESIAN_POINT ( 'NONE',  ( -9.670752905330047611, 1.395709466279072997, 2.096644049295062651 ) ) ;
#43126=AXIS2_PLACEMENT_3D ( 'NONE', #47069, #51609, #25771 ) ;
#43127=CARTESIAN_POINT ( 'NONE',  ( -10.84028925556084388, -0.1191753592594197858, 11.14116300850493246 ) ) ;
#43128=DIRECTION ( 'NONE',  ( -0.7660212471507179544, -0.6427876096865405842, -0.005961354470445141482 ) ) ;
#43129=CARTESIAN_POINT ( 'NONE',  ( 2.072287782118878319, 0.000000000000000000, -2.950529333540147015 ) ) ;
#43132=DIRECTION ( 'NONE',  ( 0.005002170337468016433, -0.7660444431189770143, -0.6427681459581293666 ) ) ;
#43133=VECTOR ( 'NONE', #27028, 999.9999999999998863 ) ;
#43134=LINE ( 'NONE', #8482, #3316 ) ;
#43135=VECTOR ( 'NONE', #32189, 999.9999999999998863 ) ;
#43136=ORIENTED_EDGE ( 'NONE', *, *, #12047, .T. ) ;
#43137=ORIENTED_EDGE ( 'NONE', *, *, #13046, .T. ) ;
#43138=LINE ( 'NONE', #4776, #31042 ) ;
#43139=AXIS2_PLACEMENT_3D ( 'NONE', #13834, #9294, #18372 ) ;
#43140=ORIENTED_EDGE ( 'NONE', *, *, #39856, .F. ) ;
#43141=AXIS2_PLACEMENT_3D ( 'NONE', #25595, #8282, #16816 ) ;
#43142=VECTOR ( 'NONE', #13523, 1000.000000000000114 ) ;
#43143=ORIENTED_EDGE ( 'NONE', *, *, #52415, .F. ) ;
#43144=AXIS2_PLACEMENT_3D ( 'NONE', #48630, #44356, #18509 ) ;
#43146=ORIENTED_EDGE ( 'NONE', *, *, #49922, .T. ) ;
#43147=CARTESIAN_POINT ( 'NONE',  ( -11.16083420050063957, 0.000000000000000000, 5.472215072723697560 ) ) ;
#43148=EDGE_LOOP ( 'NONE', ( #29281, #5495, #14562, #12892 ) ) ;
#43149=DIRECTION ( 'NONE',  ( -0.5449076811759708816, 0.6444004775717707689, 0.5364919789714475140 ) ) ;
#43150=LINE ( 'NONE', #1066, #2201 ) ;
#43151=EDGE_LOOP ( 'NONE', ( #647, #22331, #42410, #11543 ) ) ;
#43152=ADVANCED_FACE ( 'NONE', ( #1102 ), #1400, .F. ) ;
#43153=ORIENTED_EDGE ( 'NONE', *, *, #36544, .F. ) ;
#43154=VECTOR ( 'NONE', #35568, 1000.000000000000227 ) ;
#43155=ADVANCED_FACE ( 'NONE', ( #48551 ), #9938, .F. ) ;
#43156=PLANE ( 'NONE',  #13042 ) ;
#43157=VECTOR ( 'NONE', #6520, 999.9999999999998863 ) ;
#43158=ORIENTED_EDGE ( 'NONE', *, *, #50780, .T. ) ;
#43159=ADVANCED_FACE ( 'NONE', ( #32891 ), #55057, .F. ) ;
#43160=DIRECTION ( 'NONE',  ( -0.9999697198139514409, -0.000000000000000000, -0.007781995580013368816 ) ) ;
#43161=CARTESIAN_POINT ( 'NONE',  ( -19.12962290826653700, 0.000000000000000000, 14.40064212555863854 ) ) ;
#43162=ORIENTED_EDGE ( 'NONE', *, *, #22220, .T. ) ;
#43163=CIRCLE ( 'NONE', #18685, 1.000000000000000222 ) ;
#43164=CARTESIAN_POINT ( 'NONE',  ( -13.27065584551087163, 0.000000000000000000, 12.04557950825129176 ) ) ;
#43165=ADVANCED_FACE ( 'NONE', ( #23545 ), #11318, .F. ) ;
#43166=EDGE_CURVE ( 'NONE', #37821, #55875, #50513, .T. ) ;
#43167=EDGE_CURVE ( 'NONE', #16382, #38901, #32618, .T. ) ;
#43168=ORIENTED_EDGE ( 'NONE', *, *, #42297, .F. ) ;
#43169=FACE_OUTER_BOUND ( 'NONE', #7456, .T. ) ;
#43170=VECTOR ( 'NONE', #31221, 1000.000000000000227 ) ;
#43171=LINE ( 'NONE', #12769, #44508 ) ;
#43172=VECTOR ( 'NONE', #10500, 1000.000000000000227 ) ;
#43173=VECTOR ( 'NONE', #42717, 999.9999999999998863 ) ;
#43174=ORIENTED_EDGE ( 'NONE', *, *, #14231, .T. ) ;
#43175=CARTESIAN_POINT ( 'NONE',  ( -12.30315455128273783, 0.000000000000000000, 7.140659607065521719 ) ) ;
#43176=DIRECTION ( 'NONE',  ( -0.9999697198139514409, -0.000000000000000000, -0.007781995580013368816 ) ) ;
#43177=DIRECTION ( 'NONE',  ( 0.5449076811759707706, 0.6444004775717708799, -0.5364919789714476250 ) ) ;
#43178=AXIS2_PLACEMENT_3D ( 'NONE', #16074, #16922, #21156 ) ;
#43179=DIRECTION ( 'NONE',  ( -0.6427681459581293666, -0.7660444431189770143, -0.005002170337467561935 ) ) ;
#43180=VERTEX_POINT ( 'NONE', #15307 ) ;
#43181=VECTOR ( 'NONE', #27382, 1000.000000000000227 ) ;
#43182=VECTOR ( 'NONE', #48459, 1000.000000000000227 ) ;
#43183=CARTESIAN_POINT ( 'NONE',  ( -14.95364393125079694, -0.1166911823299087991, 2.590129555119498495 ) ) ;
#43184=FACE_OUTER_BOUND ( 'NONE', #7095, .T. ) ;
#43185=CARTESIAN_POINT ( 'NONE',  ( -12.33287787548504078, -3.594132820645661308, 7.371024595448199435 ) ) ;
#43186=EDGE_CURVE ( 'NONE', #8862, #50596, #53917, .T. ) ;
#43187=CARTESIAN_POINT ( 'NONE',  ( -14.86355910770291366, 0.000000000000000000, 3.596739262290799211 ) ) ;
#43188=DIRECTION ( 'NONE',  ( 0.9999697198139515519, 0.000000000000000000, 0.007781995580013368816 ) ) ;
#43190=LINE ( 'NONE', #44552, #22543 ) ;
#43191=AXIS2_PLACEMENT_3D ( 'NONE', #48868, #23021, #49128 ) ;
#43192=ADVANCED_FACE ( 'NONE', ( #23810 ), #15036, .F. ) ;
#43193=AXIS2_PLACEMENT_3D ( 'NONE', #14425, #31733, #49037 ) ;
#43194=DIRECTION ( 'NONE',  ( 0.7660212471507180654, -0.6427876096865404731, 0.005961354470445141482 ) ) ;
#43195=CARTESIAN_POINT ( 'NONE',  ( -15.09097593232924872, 0.000000000000000000, 7.118964136457464065 ) ) ;
#43196=VERTEX_POINT ( 'NONE', #37159 ) ;
#43197=EDGE_CURVE ( 'NONE', #40269, #52695, #6786, .T. ) ;
#43198=DIRECTION ( 'NONE',  ( -0.9999697198139514409, -0.000000000000000000, -0.007781995580013368816 ) ) ;
#43199=ORIENTED_EDGE ( 'NONE', *, *, #48385, .T. ) ;
#43200=PLANE ( 'NONE',  #51956 ) ;
#43201=CARTESIAN_POINT ( 'NONE',  ( -17.74404816805336793, 0.000000000000000000, 3.574322630375089460 ) ) ;
#43202=ADVANCED_FACE ( 'NONE', ( #7081 ), #41959, .F. ) ;
#43203=ADVANCED_FACE ( 'NONE', ( #45971 ), #50772, .F. ) ;
#43205=DIRECTION ( 'NONE',  ( -0.9321478471874540261, 0.000000000000000000, 0.3620778797217457656 ) ) ;
#43206=DIRECTION ( 'NONE',  ( -0.005002170337468016433, -0.7660444431189770143, 0.6427681459581293666 ) ) ;
#43209=ORIENTED_EDGE ( 'NONE', *, *, #43166, .F. ) ;
#43210=FACE_OUTER_BOUND ( 'NONE', #19416, .T. ) ;
#43211=FACE_OUTER_BOUND ( 'NONE', #20965, .T. ) ;
#43212=ORIENTED_EDGE ( 'NONE', *, *, #9168, .F. ) ;
#43213=VECTOR ( 'NONE', #9434, 1000.000000000000227 ) ;
#43214=DIRECTION ( 'NONE',  ( 0.000000000000000000, -1.000000000000000000, 0.000000000000000000 ) ) ;
#43215=EDGE_LOOP ( 'NONE', ( #11748, #37970, #30841, #44140 ) ) ;
#43216=DIRECTION ( 'NONE',  ( -0.005002170337468016433, -0.7660444431189770143, 0.6427681459581293666 ) ) ;
#43217=VECTOR ( 'NONE', #53867, 1000.000000000000227 ) ;
#43218=EDGE_LOOP ( 'NONE', ( #37839, #38988, #1612, #9192 ) ) ;
#43219=DIRECTION ( 'NONE',  ( 0.6427681459581294776, -0.7660444431189769032, 0.005002170337467562802 ) ) ;
#43220=VECTOR ( 'NONE', #24638, 1000.000000000000227 ) ;
#43221=ORIENTED_EDGE ( 'NONE', *, *, #32052, .T. ) ;
#43223=ORIENTED_EDGE ( 'NONE', *, *, #56176, .T. ) ;
#43225=DIRECTION ( 'NONE',  ( -0.005961354470445682716, -0.6427876096865404731, 0.7660212471507180654 ) ) ;
#43226=FACE_OUTER_BOUND ( 'NONE', #7939, .T. ) ;
#43227=VECTOR ( 'NONE', #27535, 1000.000000000000114 ) ;
#43228=VECTOR ( 'NONE', #21723, 1000.000000000000000 ) ;
#43229=PLANE ( 'NONE',  #17609 ) ;
#43230=ORIENTED_EDGE ( 'NONE', *, *, #47449, .F. ) ;
#43231=ORIENTED_EDGE ( 'NONE', *, *, #25850, .F. ) ;
#43232=VECTOR ( 'NONE', #41103, 999.9999999999998863 ) ;
#43233=AXIS2_PLACEMENT_3D ( 'NONE', #25640, #26475, #38994 ) ;
#43234=ORIENTED_EDGE ( 'NONE', *, *, #38441, .F. ) ;
#43235=EDGE_CURVE ( 'NONE', #48860, #29778, #24375, .T. ) ;
#43236=LINE ( 'NONE', #46921, #14957 ) ;
#43237=VERTEX_POINT ( 'NONE', #6241 ) ;
#43238=CARTESIAN_POINT ( 'NONE',  ( -16.81190032086591302, 0.000000000000000000, 3.212244750653343583 ) ) ;
#43239=ORIENTED_EDGE ( 'NONE', *, *, #24447, .T. ) ;
#43240=FACE_OUTER_BOUND ( 'NONE', #27909, .T. ) ;
#43241=CARTESIAN_POINT ( 'NONE',  ( -16.03593764792711340, 0.000000000000000000, 9.127596588505243247 ) ) ;
#43242=EDGE_CURVE ( 'NONE', #18181, #1604, #10774, .T. ) ;
#43243=EDGE_CURVE ( 'NONE', #45359, #38901, #24109, .T. ) ;
#43244=EDGE_LOOP ( 'NONE', ( #40162, #13864, #22125, #49302, #28994 ) ) ;
#43245=LINE ( 'NONE', #4039, #12272 ) ;
#43246=ORIENTED_EDGE ( 'NONE', *, *, #54517, .T. ) ;
#43247=EDGE_CURVE ( 'NONE', #20652, #37968, #19270, .T. ) ;
#43248=VECTOR ( 'NONE', #42082, 999.9999999999998863 ) ;
#43249=DIRECTION ( 'NONE',  ( -0.6427681459581293666, -0.7660444431189770143, -0.005002170337467561935 ) ) ;
#43250=ORIENTED_EDGE ( 'NONE', *, *, #30905, .F. ) ;
#43251=LINE ( 'NONE', #12295, #51313 ) ;
#43252=CARTESIAN_POINT ( 'NONE',  ( -17.16054654051782080, 0.2864062442990030766, 3.338532923747152381 ) ) ;
#43253=DIRECTION ( 'NONE',  ( 0.9999697198139515519, 0.000000000000000000, 0.007781995580013368816 ) ) ;
#43254=VERTEX_POINT ( 'NONE', #6501 ) ;
#43255=LINE ( 'NONE', #24097, #33836 ) ;
#43256=DIRECTION ( 'NONE',  ( -0.005002170337468016433, -0.7660444431189770143, 0.6427681459581293666 ) ) ;
#43257=VECTOR ( 'NONE', #54934, 999.9999999999998863 ) ;
#43258=PLANE ( 'NONE',  #47571 ) ;
#43259=LINE ( 'NONE', #38715, #3175 ) ;
#43260=PLANE ( 'NONE',  #8553 ) ;
#43261=CARTESIAN_POINT ( 'NONE',  ( -17.74482636761137044, -0.1191753592594197858, 3.674319602356483916 ) ) ;
#43262=ADVANCED_FACE ( 'NONE', ( #36907 ), #54209, .F. ) ;
#43263=VECTOR ( 'NONE', #10359, 999.9999999999998863 ) ;
#43264=LINE ( 'NONE', #9738, #27689 ) ;
#43265=ORIENTED_EDGE ( 'NONE', *, *, #38943, .F. ) ;
#43266=DIRECTION ( 'NONE',  ( 0.000000000000000000, -1.000000000000000000, 0.000000000000000000 ) ) ;
#43267=DIRECTION ( 'NONE',  ( -0.005961354470445682716, -0.6427876096865404731, 0.7660212471507180654 ) ) ;
#43268=ADVANCED_FACE ( 'NONE', ( #2770 ), #20095, .F. ) ;
#43269=DIRECTION ( 'NONE',  ( 0.005961354470445682716, -0.6427876096865404731, -0.7660212471507180654 ) ) ;
#43270=VERTEX_POINT ( 'NONE', #38857 ) ;
#43272=DIRECTION ( 'NONE',  ( 0.005002170337468016433, -0.7660444431189770143, -0.6427681459581293666 ) ) ;
#43273=ORIENTED_EDGE ( 'NONE', *, *, #30032, .T. ) ;
#43274=FACE_OUTER_BOUND ( 'NONE', #29380, .T. ) ;
#43275=ADVANCED_FACE ( 'NONE', ( #17252 ), #42268, .F. ) ;
#43276=VECTOR ( 'NONE', #36060, 999.9999999999998863 ) ;
#43277=DIRECTION ( 'NONE',  ( 0.7660212471507180654, -0.6427876096865404731, 0.005961354470445141482 ) ) ;
#43278=CARTESIAN_POINT ( 'NONE',  ( -16.81190032086591302, 0.000000000000000000, 3.212244750653343583 ) ) ;
#43279=EDGE_CURVE ( 'NONE', #35486, #36692, #12154, .T. ) ;
#43282=AXIS2_PLACEMENT_3D ( 'NONE', #38350, #43722, #30118 ) ;
#43283=VERTEX_POINT ( 'NONE', #51622 ) ;
#43284=FACE_OUTER_BOUND ( 'NONE', #11749, .T. ) ;
#43285=DIRECTION ( 'NONE',  ( 0.5364919789714477361, 0.6444004775717706579, 0.5449076811759711036 ) ) ;
#43286=LINE ( 'NONE', #26221, #47752 ) ;
#43287=PLANE ( 'NONE',  #31157 ) ;
#43288=DIRECTION ( 'NONE',  ( -0.2426528472758542054, 0.7422098413412800966, -0.6246952433987894571 ) ) ;
#43289=PLANE ( 'NONE',  #39449 ) ;
#43290=ORIENTED_EDGE ( 'NONE', *, *, #38667, .F. ) ;
#43291=PLANE ( 'NONE',  #41919 ) ;
#43292=DIRECTION ( 'NONE',  ( 0.007781995580012663651, -3.146120232559066537E-19, -0.9999697198139514409 ) ) ;
#43293=ORIENTED_EDGE ( 'NONE', *, *, #15966, .F. ) ;
#43294=PLANE ( 'NONE',  #29256 ) ;
#43295=DIRECTION ( 'NONE',  ( 0.000000000000000000, -1.000000000000000000, 0.000000000000000000 ) ) ;
#43296=DIRECTION ( 'NONE',  ( -0.005961354470445682716, -0.6427876096865404731, 0.7660212471507180654 ) ) ;
#43297=ORIENTED_EDGE ( 'NONE', *, *, #49047, .F. ) ;
#43298=DIRECTION ( 'NONE',  ( 0.000000000000000000, -0.000000000000000000, -1.000000000000000000 ) ) ;
#43299=ORIENTED_EDGE ( 'NONE', *, *, #14087, .T. ) ;
#43300=VERTEX_POINT ( 'NONE', #3913 ) ;
#43301=VECTOR ( 'NONE', #50982, 1000.000000000000114 ) ;
#43302=ORIENTED_EDGE ( 'NONE', *, *, #43420, .F. ) ;
#43303=VERTEX_POINT ( 'NONE', #34574 ) ;
#43304=CARTESIAN_POINT ( 'NONE',  ( -18.56571281152978514, 4.172053068839010947, 3.760374745758259252 ) ) ;
#43305=ORIENTED_EDGE ( 'NONE', *, *, #24550, .T. ) ;
#43307=EDGE_CURVE ( 'NONE', #13391, #48888, #39118, .T. ) ;
#43308=AXIS2_PLACEMENT_3D ( 'NONE', #32291, #36829, #20309 ) ;
#43309=ORIENTED_EDGE ( 'NONE', *, *, #37190, .F. ) ;
#43310=CARTESIAN_POINT ( 'NONE',  ( -14.87218126821876218, 0.000000000000000000, 4.704668372064093163 ) ) ;
#43311=VERTEX_POINT ( 'NONE', #51889 ) ;
#43312=DIRECTION ( 'NONE',  ( 0.007781995580012662783, 0.000000000000000000, -0.9999697198139514409 ) ) ;
#43313=ORIENTED_EDGE ( 'NONE', *, *, #11519, .F. ) ;
#43314=EDGE_CURVE ( 'NONE', #33246, #17026, #13006, .T. ) ;
#43315=EDGE_CURVE ( 'NONE', #48572, #47834, #17000, .T. ) ;
#43316=DIRECTION ( 'NONE',  ( -0.9999697198139514409, -0.000000000000000000, -0.007781995580013368816 ) ) ;
#43317=DIRECTION ( 'NONE',  ( 0.007781995580012662783, 0.000000000000000000, -0.9999697198139514409 ) ) ;
#43318=CARTESIAN_POINT ( 'NONE',  ( -22.40478740399063895, 0.000000000000000000, 5.384712028983816623 ) ) ;
#43319=DIRECTION ( 'NONE',  ( 0.6427681459581294776, -0.7660444431189769032, 0.005002170337467562802 ) ) ;
#43320=DIRECTION ( 'NONE',  ( 0.6427681459581294776, -0.7660444431189769032, 0.005002170337467562802 ) ) ;
#43321=VERTEX_POINT ( 'NONE', #26088 ) ;
#43322=ORIENTED_EDGE ( 'NONE', *, *, #49776, .F. ) ;
#43323=CARTESIAN_POINT ( 'NONE',  ( -17.42853068406109784, 0.000000000000000000, 8.947433093906241197 ) ) ;
#43324=CARTESIAN_POINT ( 'NONE',  ( -19.32961685222932147, 0.000000000000000000, 14.39908572644263351 ) ) ;
#43326=DIRECTION ( 'NONE',  ( 0.9999697198139515519, 0.000000000000000000, 0.007781995580013368816 ) ) ;
#43327=LINE ( 'NONE', #4421, #5900 ) ;
#43328=CARTESIAN_POINT ( 'NONE',  ( -1.602641424070903486, 5.553834702102301790, 3.840893930704793569 ) ) ;
#43329=VERTEX_POINT ( 'NONE', #46499 ) ;
#43330=LINE ( 'NONE', #4424, #27477 ) ;
#43331=DIRECTION ( 'NONE',  ( 0.9999697198139515519, 0.000000000000000000, 0.007781995580013368816 ) ) ;
#43332=ORIENTED_EDGE ( 'NONE', *, *, #51854, .F. ) ;
#43333=CARTESIAN_POINT ( 'NONE',  ( -25.20123094555300369, 0.000000000000000000, 6.470945668149052032 ) ) ;
#43334=LINE ( 'NONE', #5272, #44186 ) ;
#43336=EDGE_CURVE ( 'NONE', #8803, #42565, #30045, .T. ) ;
#43337=PLANE ( 'NONE',  #8789 ) ;
#43339=ORIENTED_EDGE ( 'NONE', *, *, #13986, .F. ) ;
#43340=EDGE_CURVE ( 'NONE', #31630, #40301, #3373, .T. ) ;
#43341=VERTEX_POINT ( 'NONE', #34031 ) ;
#43342=CARTESIAN_POINT ( 'NONE',  ( -10.66901316772273489, 0.000000000000000000, 1.982727895876851942 ) ) ;
#43343=DIRECTION ( 'NONE',  ( 0.007781995580012662783, 0.000000000000000000, -0.9999697198139514409 ) ) ;
#43344=FACE_OUTER_BOUND ( 'NONE', #36897, .T. ) ;
#43345=VECTOR ( 'NONE', #21920, 999.9999999999998863 ) ;
#43347=ADVANCED_FACE ( 'NONE', ( #20944 ), #51045, .F. ) ;
#43348=CARTESIAN_POINT ( 'NONE',  ( -15.35406248609154112, 0.000000000000000000, 6.916910679842669829 ) ) ;
#43349=CARTESIAN_POINT ( 'NONE',  ( 1.971453974394196562, 0.000000000000000000, 10.00639841352631088 ) ) ;
#43350=CARTESIAN_POINT ( 'NONE',  ( -15.40103151951671734, 0.000000000000000000, 12.95233060667165681 ) ) ;
#43351=VERTEX_POINT ( 'NONE', #47651 ) ;
#43352=CARTESIAN_POINT ( 'NONE',  ( -10.47421230394850866, 0.000000000000000000, 10.95934586908605723 ) ) ;
#43353=DIRECTION ( 'NONE',  ( 0.005961354470445682716, -0.6427876096865404731, -0.7660212471507180654 ) ) ;
#43354=ORIENTED_EDGE ( 'NONE', *, *, #9761, .T. ) ;
#43355=DIRECTION ( 'NONE',  ( 0.9999697198139515519, 0.000000000000000000, 0.007781995580013368816 ) ) ;
#43356=ORIENTED_EDGE ( 'NONE', *, *, #10474, .T. ) ;
#43357=DIRECTION ( 'NONE',  ( -0.5364919789714478471, 0.6444004775717705469, -0.5449076811759709926 ) ) ;
#43358=EDGE_LOOP ( 'NONE', ( #13598, #43239, #16088, #8574 ) ) ;
#43359=ORIENTED_EDGE ( 'NONE', *, *, #44643, .F. ) ;
#43360=EDGE_LOOP ( 'NONE', ( #32611, #2986, #24453, #41038 ) ) ;
#43361=ORIENTED_EDGE ( 'NONE', *, *, #51998, .F. ) ;
#43362=ORIENTED_EDGE ( 'NONE', *, *, #322, .F. ) ;
#43363=ORIENTED_EDGE ( 'NONE', *, *, #6770, .F. ) ;
#43364=LINE ( 'NONE', #3872, #32238 ) ;
#43365=DIRECTION ( 'NONE',  ( 0.007781995580012663651, -3.146120232559066537E-19, -0.9999697198139514409 ) ) ;
#43366=EDGE_CURVE ( 'NONE', #41874, #20696, #12466, .T. ) ;
#43367=LINE ( 'NONE', #39088, #34906 ) ;
#43368=EDGE_LOOP ( 'NONE', ( #7458, #11224, #48085, #15647 ) ) ;
#43369=DIRECTION ( 'NONE',  ( -0.5449076811759708816, 0.6444004775717707689, 0.5364919789714475140 ) ) ;
#43370=ORIENTED_EDGE ( 'NONE', *, *, #29719, .T. ) ;
#43371=ORIENTED_EDGE ( 'NONE', *, *, #15376, .T. ) ;
#43372=ADVANCED_FACE ( 'NONE', ( #29784 ), #8771, .F. ) ;
#43373=FACE_OUTER_BOUND ( 'NONE', #19756, .T. ) ;
#43374=CARTESIAN_POINT ( 'NONE',  ( -15.32464057242408195, 5.305366725996512933, 2.465273581601329145 ) ) ;
#43375=VERTEX_POINT ( 'NONE', #4491 ) ;
#43376=DIRECTION ( 'NONE',  ( 0.007781995580012663651, -3.146120232559066537E-19, -0.9999697198139514409 ) ) ;
#43377=ORIENTED_EDGE ( 'NONE', *, *, #36382, .F. ) ;
#43378=AXIS2_PLACEMENT_3D ( 'NONE', #51680, #3984, #12783 ) ;
#43379=FACE_OUTER_BOUND ( 'NONE', #30786, .T. ) ;
#43380=LINE ( 'NONE', #12707, #12132 ) ;
#43381=EDGE_CURVE ( 'NONE', #8547, #35585, #21799, .T. ) ;
#43382=PLANE ( 'NONE',  #41432 ) ;
#43383=FACE_OUTER_BOUND ( 'NONE', #49777, .T. ) ;
#43384=CARTESIAN_POINT ( 'NONE',  ( -18.71879214953967008, -0.1191753592594166911, 8.468056882921050743 ) ) ;
#43386=FACE_OUTER_BOUND ( 'NONE', #29481, .T. ) ;
#43388=EDGE_LOOP ( 'NONE', ( #32100, #41075, #17958, #46762 ) ) ;
#43390=DIRECTION ( 'NONE',  ( 0.9999697198139515519, 0.000000000000000000, 0.007781995580013368816 ) ) ;
#43391=DIRECTION ( 'NONE',  ( -0.005961354470445682716, -0.6427876096865404731, 0.7660212471507180654 ) ) ;
#43392=CARTESIAN_POINT ( 'NONE',  ( -17.87879731337576317, 0.000000000000000000, 7.097268665849407299 ) ) ;
#43394=CARTESIAN_POINT ( 'NONE',  ( -17.64908100030126548, -3.270328918600660995, 8.904601060243949817 ) ) ;
#43395=LINE ( 'NONE', #783, #18705 ) ;
#43396=CARTESIAN_POINT ( 'NONE',  ( -9.042074112879289416, 0.000000000000000000, 6.058041879668295771 ) ) ;
#43397=VERTEX_POINT ( 'NONE', #24945 ) ;
#43398=LINE ( 'NONE', #34321, #50169 ) ;
#43399=PLANE ( 'NONE',  #42124 ) ;
#43400=PLANE ( 'NONE',  #25469 ) ;
#43401=LINE ( 'NONE', #9302, #24585 ) ;
#43402=EDGE_CURVE ( 'NONE', #38162, #27809, #11862, .T. ) ;
#43403=DIRECTION ( 'NONE',  ( 0.005961354470445682716, -0.6427876096865404731, -0.7660212471507180654 ) ) ;
#43404=CARTESIAN_POINT ( 'NONE',  ( -16.32868032335150232, 2.067327705546508021, 2.958587115942813206 ) ) ;
#43405=CARTESIAN_POINT ( 'NONE',  ( -15.83583329205734103, -2.784623065533159636, 7.403148020359251014 ) ) ;
#43406=LINE ( 'NONE', #30645, #13102 ) ;
#43407=CARTESIAN_POINT ( 'NONE',  ( -15.35118843258626065, 0.000000000000000000, 6.547600976584903698 ) ) ;
#43408=ORIENTED_EDGE ( 'NONE', *, *, #54402, .F. ) ;
#43409=CARTESIAN_POINT ( 'NONE',  ( -28.93137873341882127, 0.000000000000000000, 8.119251130998824451 ) ) ;
#43410=ADVANCED_FACE ( 'NONE', ( #8187 ), #38007, .F. ) ;
#43411=AXIS2_PLACEMENT_3D ( 'NONE', #44355, #22769, #44618 ) ;
#43412=ORIENTED_EDGE ( 'NONE', *, *, #5992, .T. ) ;
#43413=EDGE_CURVE ( 'NONE', #46599, #3531, #55897, .T. ) ;
#43414=ADVANCED_FACE ( 'NONE', ( #21543 ), #1043, .F. ) ;
#43415=ORIENTED_EDGE ( 'NONE', *, *, #41719, .T. ) ;
#43416=ORIENTED_EDGE ( 'NONE', *, *, #32701, .F. ) ;
#43417=ORIENTED_EDGE ( 'NONE', *, *, #15465, .T. ) ;
#43418=ORIENTED_EDGE ( 'NONE', *, *, #54418, .T. ) ;
#43419=CARTESIAN_POINT ( 'NONE',  ( -17.21261007345589178, 0.000000000000000000, 6.902447032770631097 ) ) ;
#43420=EDGE_CURVE ( 'NONE', #14352, #49950, #48186, .T. ) ;
#43421=PLANE ( 'NONE',  #26702 ) ;
#43422=ADVANCED_FACE ( 'NONE', ( #36019 ), #44239, .F. ) ;
#43423=ORIENTED_EDGE ( 'NONE', *, *, #9046, .T. ) ;
#43424=ADVANCED_FACE ( 'NONE', ( #18955 ), #30877, .F. ) ;
#43425=CARTESIAN_POINT ( 'NONE',  ( 2.072287782118878319, 0.000000000000000000, -2.950529333540147015 ) ) ;
#43426=VERTEX_POINT ( 'NONE', #31732 ) ;
#43427=DIRECTION ( 'NONE',  ( 0.005961354470445682716, -0.6427876096865404731, -0.7660212471507180654 ) ) ;
#43428=LINE ( 'NONE', #29820, #17768 ) ;
#43430=DIRECTION ( 'NONE',  ( -0.6427681459581293666, -0.7660444431189770143, -0.005002170337467561935 ) ) ;
#43431=EDGE_CURVE ( 'NONE', #45114, #6152, #27457, .T. ) ;
#43432=ORIENTED_EDGE ( 'NONE', *, *, #41368, .T. ) ;
#43433=DIRECTION ( 'NONE',  ( -0.5364919789714478471, 0.6444004775717705469, -0.5449076811759709926 ) ) ;
#43434=ADVANCED_FACE ( 'NONE', ( #14423 ), #1333, .F. ) ;
#43435=LINE ( 'NONE', #247, #31830 ) ;
#43436=EDGE_LOOP ( 'NONE', ( #28451, #40274, #26797, #25136 ) ) ;
#43437=DIRECTION ( 'NONE',  ( 0.6427681459581294776, -0.7660444431189769032, 0.005002170337467562802 ) ) ;
#43438=CARTESIAN_POINT ( 'NONE',  ( -19.45503627000849889, 0.000000000000000000, 7.556996783084074742 ) ) ;
#43439=CARTESIAN_POINT ( 'NONE',  ( -19.60834386242827776, 0.000000000000000000, 4.298478389818581213 ) ) ;
#43440=CARTESIAN_POINT ( 'NONE',  ( -12.74036856746027802, 0.000000000000000000, 3.613262422014844155 ) ) ;
#43441=VERTEX_POINT ( 'NONE', #53027 ) ;
#43442=VECTOR ( 'NONE', #55118, 1000.000000000000114 ) ;
#43444=CARTESIAN_POINT ( 'NONE',  ( -23.33693525117809386, 0.000000000000000000, 5.746789908705562944 ) ) ;
#43445=LINE ( 'NONE', #42872, #32174 ) ;
#43446=CARTESIAN_POINT ( 'NONE',  ( -11.20636620717317378, 0.000000000000000000, 11.32298014792380414 ) ) ;
#43448=LINE ( 'NONE', #13070, #36727 ) ;
#43450=PLANE ( 'NONE',  #41971 ) ;
#43451=DIRECTION ( 'NONE',  ( -0.9999697198139514409, -0.000000000000000000, -0.007781995580013368816 ) ) ;
#43452=FACE_OUTER_BOUND ( 'NONE', #21898, .T. ) ;
#43453=ORIENTED_EDGE ( 'NONE', *, *, #33931, .T. ) ;
#43454=PLANE ( 'NONE',  #17513 ) ;
#43455=LINE ( 'NONE', #9370, #935 ) ;
#43456=DIRECTION ( 'NONE',  ( 0.005961354470445682716, -0.6427876096865404731, -0.7660212471507180654 ) ) ;
#43457=LINE ( 'NONE', #48565, #1917 ) ;
#43458=ADVANCED_FACE ( 'NONE', ( #781 ), #22082, .F. ) ;
#43459=DIRECTION ( 'NONE',  ( 0.000000000000000000, -0.000000000000000000, -1.000000000000000000 ) ) ;
#43460=PLANE ( 'NONE',  #8412 ) ;
#43461=ORIENTED_EDGE ( 'NONE', *, *, #27381, .F. ) ;
#43462=EDGE_LOOP ( 'NONE', ( #24001, #4581, #37578, #6259 ) ) ;
#43463=CARTESIAN_POINT ( 'NONE',  ( -12.20933787556949213, -1.813211359398156919, 4.400241940589850742 ) ) ;
#43464=DIRECTION ( 'NONE',  ( 0.7660212471507180654, -0.6427876096865404731, 0.005961354470445141482 ) ) ;
#43465=EDGE_LOOP ( 'NONE', ( #42655, #30512, #30070, #38533 ) ) ;
#43466=EDGE_CURVE ( 'NONE', #25808, #46628, #44783, .T. ) ;
#43467=ADVANCED_FACE ( 'NONE', ( #4760 ), #18676, .F. ) ;
#43468=DIRECTION ( 'NONE',  ( 0.5364919789714477361, 0.6444004775717706579, 0.5449076811759711036 ) ) ;
#43469=VERTEX_POINT ( 'NONE', #5896 ) ;
#43470=CARTESIAN_POINT ( 'NONE',  ( -17.46532115785441519, 0.000000000000000000, 13.67492996699914265 ) ) ;
#43471=EDGE_LOOP ( 'NONE', ( #15894, #24557, #53816, #3539 ) ) ;
#43472=DIRECTION ( 'NONE',  ( 0.9999697198139515519, 0.000000000000000000, 0.007781995580013368816 ) ) ;
#43473=EDGE_CURVE ( 'NONE', #36189, #10560, #31159, .T. ) ;
#43474=EDGE_LOOP ( 'NONE', ( #17169, #13701, #46631, #49844 ) ) ;
#43476=ORIENTED_EDGE ( 'NONE', *, *, #41233, .F. ) ;
#43477=LINE ( 'NONE', #12814, #41097 ) ;
#43478=DIRECTION ( 'NONE',  ( -0.7660212471507179544, -0.6427876096865405842, -0.005961354470445141482 ) ) ;
#43479=DIRECTION ( 'NONE',  ( -0.6427681459581293666, -0.7660444431189770143, -0.005002170337467561935 ) ) ;
#43480=FACE_OUTER_BOUND ( 'NONE', #53287, .T. ) ;
#43481=EDGE_CURVE ( 'NONE', #44308, #39505, #27183, .T. ) ;
#43482=ORIENTED_EDGE ( 'NONE', *, *, #37135, .F. ) ;
#43483=VERTEX_POINT ( 'NONE', #23222 ) ;
#43484=EDGE_CURVE ( 'NONE', #54767, #7497, #505, .T. ) ;
#43485=EDGE_LOOP ( 'NONE', ( #34699, #26793, #21572, #49419 ) ) ;
#43488=CARTESIAN_POINT ( 'NONE',  ( 2.072287782118878319, 0.000000000000000000, -2.950529333540147015 ) ) ;
#43489=EDGE_LOOP ( 'NONE', ( #17492, #51761, #35455, #47904 ) ) ;
#43490=DIRECTION ( 'NONE',  ( -0.7660212471507179544, -0.6427876096865405842, -0.005961354470445141482 ) ) ;
#43491=CARTESIAN_POINT ( 'NONE',  ( -18.23205287539565589, -0.6798977022406563764, 4.879708191131419071 ) ) ;
#43492=EDGE_CURVE ( 'NONE', #34678, #45226, #5598, .T. ) ;
#43493=ORIENTED_EDGE ( 'NONE', *, *, #19554, .F. ) ;
#43494=CARTESIAN_POINT ( 'NONE',  ( -18.67619601524082285, 0.000000000000000000, 3.936400510096834893 ) ) ;
#43495=EDGE_LOOP ( 'NONE', ( #7407, #52433, #36425, #5270 ) ) ;
#43496=CARTESIAN_POINT ( 'NONE',  ( -17.19979620504548024, 0.000000000000000000, 5.255892460444599124 ) ) ;
#43497=ORIENTED_EDGE ( 'NONE', *, *, #41715, .T. ) ;
#43498=PLANE ( 'NONE',  #5111 ) ;
#43499=FACE_OUTER_BOUND ( 'NONE', #36095, .T. ) ;
#43500=CARTESIAN_POINT ( 'NONE',  ( -10.72382211176504008, -1.165603555308156736, 2.760382433798663993 ) ) ;
#43501=EDGE_LOOP ( 'NONE', ( #12193, #52672, #32267 ) ) ;
#43502=DIRECTION ( 'NONE',  ( 0.5449076811759707706, 0.6444004775717708799, -0.5364919789714476250 ) ) ;
#43504=DIRECTION ( 'NONE',  ( 0.005961354470445682716, -0.6427876096865404731, -0.7660212471507180654 ) ) ;
#43505=DIRECTION ( 'NONE',  ( 0.000000000000000000, -1.000000000000000000, 0.000000000000000000 ) ) ;
#43506=DIRECTION ( 'NONE',  ( 0.000000000000000000, -0.000000000000000000, -1.000000000000000000 ) ) ;
#43507=LINE ( 'NONE', #44352, #26113 ) ;
#43508=DIRECTION ( 'NONE',  ( -0.005961354470445682716, -0.6427876096865404731, 0.7660212471507180654 ) ) ;
#43509=ORIENTED_EDGE ( 'NONE', *, *, #29371, .T. ) ;
#43510=DIRECTION ( 'NONE',  ( 0.000000000000000000, -0.000000000000000000, -1.000000000000000000 ) ) ;
#43511=DIRECTION ( 'NONE',  ( 0.007781995580012663651, -3.146120232559066537E-19, -0.9999697198139514409 ) ) ;
#43512=CARTESIAN_POINT ( 'NONE',  ( -16.26764835785802532, 0.000000000000000000, 4.893814580722853691 ) ) ;
#43513=ORIENTED_EDGE ( 'NONE', *, *, #16953, .F. ) ;
#43514=CARTESIAN_POINT ( 'NONE',  ( -15.60102546347950536, 0.000000000000000000, 12.95077420755565356 ) ) ;
#43515=CARTESIAN_POINT ( 'NONE',  ( -16.53317331066696383, 0.000000000000000000, 13.31285208727739899 ) ) ;
#43516=ORIENTED_EDGE ( 'NONE', *, *, #30015, .F. ) ;
#43517=ADVANCED_FACE ( 'NONE', ( #40243 ), #52186, .F. ) ;
#43518=DIRECTION ( 'NONE',  ( -0.5364919789714478471, 0.6444004775717705469, -0.5449076811759709926 ) ) ;
#43519=DIRECTION ( 'NONE',  ( 0.007781995580012663651, 0.000000000000000000, -0.9999697198139515519 ) ) ;
#43520=ADVANCED_FACE ( 'NONE', ( #17844 ), #35174, .F. ) ;
#43521=LINE ( 'NONE', #8321, #16921 ) ;
#43522=DIRECTION ( 'NONE',  ( 0.9999697198139515519, 0.000000000000000000, 0.007781995580013368816 ) ) ;
#43523=EDGE_LOOP ( 'NONE', ( #11990, #50447, #17887, #28411, #29821 ) ) ;
#43524=ORIENTED_EDGE ( 'NONE', *, *, #12901, .T. ) ;
#43525=EDGE_CURVE ( 'NONE', #51710, #52991, #50443, .T. ) ;
#43526=DIRECTION ( 'NONE',  ( 0.9999697198139515519, 0.000000000000000000, 0.007781995580013368816 ) ) ;
#43527=FACE_OUTER_BOUND ( 'NONE', #18925, .T. ) ;
#43528=DIRECTION ( 'NONE',  ( 0.9999697198139515519, 0.000000000000000000, 0.007781995580013368816 ) ) ;
#43529=EDGE_CURVE ( 'NONE', #55216, #56100, #6188, .T. ) ;
#43530=EDGE_CURVE ( 'NONE', #21707, #39029, #2463, .T. ) ;
#43531=EDGE_CURVE ( 'NONE', #47622, #50731, #10726, .T. ) ;
#43532=CARTESIAN_POINT ( 'NONE',  ( -21.12145515939264584, -2.460819163488159766, 5.007098573608039338 ) ) ;
#43533=CARTESIAN_POINT ( 'NONE',  ( -14.92626657078307417, -2.298917212465660054, 2.605842456189420009 ) ) ;
#43534=CARTESIAN_POINT ( 'NONE',  ( -24.26908309836554878, 0.000000000000000000, 6.108867788427308376 ) ) ;
#43535=EDGE_LOOP ( 'NONE', ( #32528, #20520, #2819, #25826 ) ) ;
#43536=EDGE_CURVE ( 'NONE', #41476, #35980, #41628, .T. ) ;
#43537=LINE ( 'NONE', #21696, #12924 ) ;
#43538=DIRECTION ( 'NONE',  ( 0.7660212471507180654, -0.6427876096865404731, 0.005961354470445141482 ) ) ;
#43539=VERTEX_POINT ( 'NONE', #11253 ) ;
#43540=DIRECTION ( 'NONE',  ( 0.005002170337468016433, -0.7660444431189770143, -0.6427681459581293666 ) ) ;
#43541=LINE ( 'NONE', #14312, #53119 ) ;
#43542=DIRECTION ( 'NONE',  ( 0.007781995580012663651, 0.000000000000000000, -0.9999697198139515519 ) ) ;
#43543=ORIENTED_EDGE ( 'NONE', *, *, #41233, .T. ) ;
#43544=LINE ( 'NONE', #47237, #36537 ) ;
#43545=ADVANCED_FACE ( 'NONE', ( #24576 ), #37104, .F. ) ;
#43546=VERTEX_POINT ( 'NONE', #6445 ) ;
#43547=VECTOR ( 'NONE', #13564, 1000.000000000000227 ) ;
#43548=ADVANCED_FACE ( 'NONE', ( #14968 ), #41372, .F. ) ;
#43549=ORIENTED_EDGE ( 'NONE', *, *, #24551, .F. ) ;
#43550=VERTEX_POINT ( 'NONE', #49323 ) ;
#43552=ORIENTED_EDGE ( 'NONE', *, *, #20205, .T. ) ;
#43553=LINE ( 'NONE', #13473, #4880 ) ;
#43554=ORIENTED_EDGE ( 'NONE', *, *, #4103, .T. ) ;
#43555=CARTESIAN_POINT ( 'NONE',  ( -11.64139776398414128, 0.000000000000000000, 7.515141621207298783 ) ) ;
#43556=EDGE_CURVE ( 'NONE', #14263, #10825, #6721, .T. ) ;
#43557=ORIENTED_EDGE ( 'NONE', *, *, #16928, .T. ) ;
#43558=FACE_OUTER_BOUND ( 'NONE', #47509, .T. ) ;
#43559=ORIENTED_EDGE ( 'NONE', *, *, #20347, .T. ) ;
#43560=DIRECTION ( 'NONE',  ( -0.9999697198139514409, -0.000000000000000000, -0.007781995580013368816 ) ) ;
#43561=VERTEX_POINT ( 'NONE', #24041 ) ;
#43562=EDGE_CURVE ( 'NONE', #38932, #42767, #46166, .T. ) ;
#43563=CARTESIAN_POINT ( 'NONE',  ( -14.88810793486117667, 0.000000000000000000, 6.751210832315702959 ) ) ;
#43564=CARTESIAN_POINT ( 'NONE',  ( -15.49681410618518562, 3.848249166794011522, 2.578641308138473143 ) ) ;
#43565=LINE ( 'NONE', #55797, #15877 ) ;
#43566=DIRECTION ( 'NONE',  ( -0.005961354470445682716, -0.6427876096865404731, 0.7660212471507180654 ) ) ;
#43567=DIRECTION ( 'NONE',  ( -0.5449076811759708816, 0.6444004775717707689, 0.5364919789714475140 ) ) ;
#43568=ORIENTED_EDGE ( 'NONE', *, *, #48145, .T. ) ;
#43569=ORIENTED_EDGE ( 'NONE', *, *, #40795, .T. ) ;
#43570=DIRECTION ( 'NONE',  ( 0.007781995580012663651, 0.000000000000000000, -0.9999697198139515519 ) ) ;
#43571=CARTESIAN_POINT ( 'NONE',  ( -16.46169322245890498, -5.698858183938163791, 12.42900958272824852 ) ) ;
#43572=CARTESIAN_POINT ( 'NONE',  ( -12.08879033979353324, 0.000000000000000000, 5.295667489892703195 ) ) ;
#43573=DIRECTION ( 'NONE',  ( 0.000000000000000000, -1.000000000000000000, 0.000000000000000000 ) ) ;
#43574=DIRECTION ( 'NONE',  ( -0.9999697198139514409, -0.000000000000000000, -0.007781995580013368816 ) ) ;
#43575=CARTESIAN_POINT ( 'NONE',  ( -26.13415699229845757, -0.1191753592594197858, 6.933020519852192365 ) ) ;
#43577=CARTESIAN_POINT ( 'NONE',  ( -18.14475792064334314, 0.000000000000000000, 7.264524912492376529 ) ) ;
#43578=LINE ( 'NONE', #8382, #32220 ) ;
#43579=ORIENTED_EDGE ( 'NONE', *, *, #49848, .T. ) ;
#43580=DIRECTION ( 'NONE',  ( 0.007781995580012663651, 0.000000000000000000, -0.9999697198139515519 ) ) ;
#43581=DIRECTION ( 'NONE',  ( 0.000000000000000000, -0.000000000000000000, -1.000000000000000000 ) ) ;
#43582=DIRECTION ( 'NONE',  ( 0.007781995580012663651, 0.000000000000000000, -0.9999697198139515519 ) ) ;
#43583=PLANE ( 'NONE',  #15096 ) ;
#43584=AXIS2_PLACEMENT_3D ( 'NONE', #38346, #55380, #46889 ) ;
#43585=LINE ( 'NONE', #50775, #26529 ) ;
#43586=ORIENTED_EDGE ( 'NONE', *, *, #24767, .T. ) ;
#43587=ORIENTED_EDGE ( 'NONE', *, *, #49689, .T. ) ;
#43588=CARTESIAN_POINT ( 'NONE',  ( -15.99989958031287962, 5.467268677019012202, 12.06894479977838408 ) ) ;
#43589=FACE_OUTER_BOUND ( 'NONE', #7296, .T. ) ;
#43590=DIRECTION ( 'NONE',  ( -0.005961354470445682716, -0.6427876096865404731, 0.7660212471507180654 ) ) ;
#43591=ADVANCED_FACE ( 'NONE', ( #20036 ), #15499, .F. ) ;
#43592=ADVANCED_FACE ( 'NONE', ( #32825 ), #28030, .F. ) ;
#43594=DIRECTION ( 'NONE',  ( 0.9999697198139515519, 0.000000000000000000, 0.007781995580013368816 ) ) ;
#43595=EDGE_CURVE ( 'NONE', #28974, #21716, #53572, .T. ) ;
#43596=DIRECTION ( 'NONE',  ( 0.5364919789714477361, 0.6444004775717706579, 0.5449076811759711036 ) ) ;
#43597=CARTESIAN_POINT ( 'NONE',  ( -27.99923088623136636, 0.000000000000000000, 7.757173251277078130 ) ) ;
#43598=ORIENTED_EDGE ( 'NONE', *, *, #25108, .T. ) ;
#43599=DIRECTION ( 'NONE',  ( 0.005961354470445682716, -0.6427876096865404731, -0.7660212471507180654 ) ) ;
#43600=DIRECTION ( 'NONE',  ( 0.000000000000000000, -1.000000000000000000, 0.000000000000000000 ) ) ;
#43601=ORIENTED_EDGE ( 'NONE', *, *, #42511, .F. ) ;
#43602=CARTESIAN_POINT ( 'NONE',  ( -15.33107005804928313, 0.000000000000000000, 3.962433053780552328 ) ) ;
#43603=ORIENTED_EDGE ( 'NONE', *, *, #54320, .F. ) ;
#43604=CARTESIAN_POINT ( 'NONE',  ( -15.38456134770231110, -1.165603555308156736, 4.570771832407389823 ) ) ;
#43605=LINE ( 'NONE', #24974, #2972 ) ;
#43606=ORIENTED_EDGE ( 'NONE', *, *, #45332, .F. ) ;
#43607=VECTOR ( 'NONE', #10980, 1000.000000000000227 ) ;
#43609=ORIENTED_EDGE ( 'NONE', *, *, #50485, .F. ) ;
#43610=ORIENTED_EDGE ( 'NONE', *, *, #51560, .F. ) ;
#43611=ORIENTED_EDGE ( 'NONE', *, *, #10080, .F. ) ;
#43612=ORIENTED_EDGE ( 'NONE', *, *, #20343, .F. ) ;
#43613=LINE ( 'NONE', #34284, #37699 ) ;
#43614=CARTESIAN_POINT ( 'NONE',  ( -14.01623497886155256, -0.1191753592594197858, 2.226008083469502630 ) ) ;
#43615=CARTESIAN_POINT ( 'NONE',  ( -14.00280974873554030, 0.000000000000000000, 12.40921378708904044 ) ) ;
#43616=VECTOR ( 'NONE', #45719, 999.9999999999998863 ) ;
#43617=ORIENTED_EDGE ( 'NONE', *, *, #14377, .F. ) ;
#43618=CARTESIAN_POINT ( 'NONE',  ( -25.20123094555300369, 0.000000000000000000, 6.470945668149052032 ) ) ;
#43619=ORIENTED_EDGE ( 'NONE', *, *, #43942, .T. ) ;
#43620=ORIENTED_EDGE ( 'NONE', *, *, #4251, .T. ) ;
#43621=ADVANCED_FACE ( 'NONE', ( #27762 ), #37358, .F. ) ;
#43622=AXIS2_PLACEMENT_3D ( 'NONE', #12730, #35431, #47358 ) ;
#43623=CARTESIAN_POINT ( 'NONE',  ( -12.80458192191714595, 0.000000000000000000, 11.86454056839041726 ) ) ;
#43624=EDGE_CURVE ( 'NONE', #54774, #17288, #23750, .T. ) ;
#43625=CARTESIAN_POINT ( 'NONE',  ( -16.81345671998191449, 0.000000000000000000, 3.412238694616132495 ) ) ;
#43626=PLANE ( 'NONE',  #7796 ) ;
#43627=EDGE_CURVE ( 'NONE', #6097, #5412, #28577, .T. ) ;
#43629=CARTESIAN_POINT ( 'NONE',  ( -13.63673279712320507, -0.1191753592594197858, 12.22739664767016521 ) ) ;
#43630=ORIENTED_EDGE ( 'NONE', *, *, #51818, .F. ) ;
#43631=CARTESIAN_POINT ( 'NONE',  ( -10.84028925556084388, -0.1191753592594197858, 11.14116300850493246 ) ) ;
#43632=EDGE_CURVE ( 'NONE', #54969, #55411, #33956, .T. ) ;
#43633=LINE ( 'NONE', #13286, #7595 ) ;
#43634=PLANE ( 'NONE',  #36900 ) ;
#43635=LINE ( 'NONE', #39399, #49443 ) ;
#43637=CARTESIAN_POINT ( 'NONE',  ( -21.47263955680318404, 0.000000000000000000, 5.022634149262071190 ) ) ;
#43638=CARTESIAN_POINT ( 'NONE',  ( 2.072287782118878319, 0.000000000000000000, -2.950529333540147015 ) ) ;
#43640=ORIENTED_EDGE ( 'NONE', *, *, #17855, .T. ) ;
#43641=LINE ( 'NONE', #4753, #49196 ) ;
#43642=VECTOR ( 'NONE', #26096, 1000.000000000000227 ) ;
#43643=VECTOR ( 'NONE', #52769, 999.9999999999998863 ) ;
#43644=DIRECTION ( 'NONE',  ( 0.9999697198139515519, 0.000000000000000000, 0.007781995580013368816 ) ) ;
#43645=CARTESIAN_POINT ( 'NONE',  ( -14.15152357901523139, 0.000000000000000000, 5.818272906257401900 ) ) ;
#43646=CARTESIAN_POINT ( 'NONE',  ( -10.74029228357944987, 0.000000000000000000, 11.14194120806293320 ) ) ;
#43648=DIRECTION ( 'NONE',  ( 0.5449076811759707706, 0.6444004775717708799, -0.5364919789714476250 ) ) ;
#43650=CARTESIAN_POINT ( 'NONE',  ( -18.76354595665420177, -0.1191753592594177458, 14.21882498613976331 ) ) ;
#43651=ORIENTED_EDGE ( 'NONE', *, *, #24483, .F. ) ;
#43652=CARTESIAN_POINT ( 'NONE',  ( -28.93060053386082231, -0.1191753592594197858, 8.019254159017428663 ) ) ;
#43653=PLANE ( 'NONE',  #39428 ) ;
#43654=FACE_OUTER_BOUND ( 'NONE', #51247, .T. ) ;
#43655=ADVANCED_FACE ( 'NONE', ( #16934 ), #42738, .F. ) ;
#43657=DIRECTION ( 'NONE',  ( 0.005002170337468016433, -0.7660444431189770143, -0.6427681459581293666 ) ) ;
#43658=LINE ( 'NONE', #49051, #23204 ) ;
#43659=EDGE_CURVE ( 'NONE', #41210, #27927, #7858, .T. ) ;
#43660=ADVANCED_FACE ( 'NONE', ( #29724 ), #17193, .F. ) ;
#43661=LINE ( 'NONE', #18113, #8384 ) ;
#43662=VECTOR ( 'NONE', #51401, 999.9999999999998863 ) ;
#43664=ORIENTED_EDGE ( 'NONE', *, *, #14564, .F. ) ;
#43665=LINE ( 'NONE', #4249, #55526 ) ;
#43667=ORIENTED_EDGE ( 'NONE', *, *, #38620, .F. ) ;
#43668=EDGE_CURVE ( 'NONE', #21619, #43550, #42197, .T. ) ;
#43670=VERTEX_POINT ( 'NONE', #20631 ) ;
#43671=ORIENTED_EDGE ( 'NONE', *, *, #40617, .T. ) ;
#43672=ORIENTED_EDGE ( 'NONE', *, *, #11613, .T. ) ;
#43673=CARTESIAN_POINT ( 'NONE',  ( -21.47419595591918906, 0.000000000000000000, 5.222628093224860102 ) ) ;
#43674=PLANE ( 'NONE',  #24878 ) ;
#43675=AXIS2_PLACEMENT_3D ( 'NONE', #11261, #50983, #2473 ) ;
#43676=AXIS2_PLACEMENT_3D ( 'NONE', #6924, #33025, #3490 ) ;
#43678=ORIENTED_EDGE ( 'NONE', *, *, #30907, .T. ) ;
#43680=ORIENTED_EDGE ( 'NONE', *, *, #13722, .F. ) ;
#43682=LINE ( 'NONE', #51928, #17722 ) ;
#43683=EDGE_LOOP ( 'NONE', ( #52117, #25833, #23897, #25489 ) ) ;
#43684=DIRECTION ( 'NONE',  ( -0.005002170337468016433, -0.7660444431189770143, 0.6427681459581293666 ) ) ;
#43685=ORIENTED_EDGE ( 'NONE', *, *, #12638, .T. ) ;
#43686=CARTESIAN_POINT ( 'NONE',  ( -14.19717356985994705, -3.594132820645661308, 8.095180354891688523 ) ) ;
#43687=ADVANCED_FACE ( 'NONE', ( #37942 ), #29419, .F. ) ;
#43688=VECTOR ( 'NONE', #27497, 1000.000000000000227 ) ;
#43689=VECTOR ( 'NONE', #7903, 1000.000000000000227 ) ;
#43690=DIRECTION ( 'NONE',  ( -0.9999697198139514409, -0.000000000000000000, -0.007781995580013368816 ) ) ;
#43692=ORIENTED_EDGE ( 'NONE', *, *, #7614, .T. ) ;
#43693=LINE ( 'NONE', #39748, #32178 ) ;
#43694=LINE ( 'NONE', #53082, #47431 ) ;
#43695=LINE ( 'NONE', #13608, #25739 ) ;
#43696=ORIENTED_EDGE ( 'NONE', *, *, #26683, .F. ) ;
#43697=CARTESIAN_POINT ( 'NONE',  ( 1.969897575278193980, 0.000000000000000000, 10.20639235748909890 ) ) ;
#43699=EDGE_CURVE ( 'NONE', #35428, #52435, #38491, .T. ) ;
#43700=CARTESIAN_POINT ( 'NONE',  ( -15.36998915273395738, 0.000000000000000000, 8.963453140094282290 ) ) ;
#43701=CARTESIAN_POINT ( 'NONE',  ( -27.06708303904391144, 0.000000000000000000, 7.395095371555332697 ) ) ;
#43702=FACE_OUTER_BOUND ( 'NONE', #44417, .T. ) ;
#43703=LINE ( 'NONE', #47722, #7830 ) ;
#43704=CARTESIAN_POINT ( 'NONE',  ( -12.62965358101575397, -0.1191753592594188005, 2.236798780523178820 ) ) ;
#43705=EDGE_CURVE ( 'NONE', #2028, #12064, #25712, .T. ) ;
#43706=DIRECTION ( 'NONE',  ( 0.005002170337468016433, -0.7660444431189770143, -0.6427681459581293666 ) ) ;
#43707=CARTESIAN_POINT ( 'NONE',  ( -14.12003756145438871, 4.981562823951513508, 2.007695903425033901 ) ) ;
#43708=ADVANCED_FACE ( 'NONE', ( #38201 ), #46428, .F. ) ;
#43709=CARTESIAN_POINT ( 'NONE',  ( -25.20200914511100265, -0.1191753592594197858, 6.570942640130446932 ) ) ;
#43711=LINE ( 'NONE', #56228, #37773 ) ;
#43712=EDGE_LOOP ( 'NONE', ( #2441, #14584, #44669, #7896 ) ) ;
#43713=VECTOR ( 'NONE', #395, 999.9999999999998863 ) ;
#43715=EDGE_CURVE ( 'NONE', #46599, #41809, #21167, .T. ) ;
#43716=LINE ( 'NONE', #52534, #32712 ) ;
#43717=DIRECTION ( 'NONE',  ( 0.5449076811759707706, 0.6444004775717708799, -0.5364919789714476250 ) ) ;
#43718=VECTOR ( 'NONE', #33901, 1000.000000000000114 ) ;
#43719=VECTOR ( 'NONE', #30095, 1000.000000000000000 ) ;
#43720=EDGE_CURVE ( 'NONE', #42927, #54093, #8698, .T. ) ;
#43721=CARTESIAN_POINT ( 'NONE',  ( -12.60956183379353845, -3.917936722690661178, 8.009915408982919871 ) ) ;
#43722=DIRECTION ( 'NONE',  ( -0.7660212471507179544, -0.6427876096865405842, -0.005961354470445141482 ) ) ;
#43723=EDGE_CURVE ( 'NONE', #44901, #26765, #16627, .T. ) ;
#43724=CARTESIAN_POINT ( 'NONE',  ( -3.638205267667341758, -7.220147766006030032, -1.805171095730843112 ) ) ;
#43725=ORIENTED_EDGE ( 'NONE', *, *, #9572, .T. ) ;
#43726=VECTOR ( 'NONE', #30282, 999.9999999999998863 ) ;
#43727=AXIS2_PLACEMENT_3D ( 'NONE', #28412, #32959, #37799 ) ;
#43728=ORIENTED_EDGE ( 'NONE', *, *, #9960, .F. ) ;
#43729=CARTESIAN_POINT ( 'NONE',  ( -14.93495759592298988, 0.000000000000000000, 12.77129166681078409 ) ) ;
#43730=LINE ( 'NONE', #4843, #40447 ) ;
#43731=EDGE_LOOP ( 'NONE', ( #28226, #26132, #41398, #44213 ) ) ;
#43732=PLANE ( 'NONE',  #18420 ) ;
#43734=ORIENTED_EDGE ( 'NONE', *, *, #16891, .F. ) ;
#43735=LINE ( 'NONE', #13638, #22267 ) ;
#43737=ORIENTED_EDGE ( 'NONE', *, *, #43917, .T. ) ;
#43738=LINE ( 'NONE', #39508, #7524 ) ;
#43739=EDGE_CURVE ( 'NONE', #41032, #29707, #12932, .T. ) ;
#43740=ORIENTED_EDGE ( 'NONE', *, *, #817, .T. ) ;
#43741=ORIENTED_EDGE ( 'NONE', *, *, #31553, .F. ) ;
#43742=ORIENTED_EDGE ( 'NONE', *, *, #32299, .F. ) ;
#43743=CARTESIAN_POINT ( 'NONE',  ( -13.58962795970950843, 1.581621852479004664, 1.910142718956624908 ) ) ;
#43744=PLANE ( 'NONE',  #15094 ) ;
#43745=DIRECTION ( 'NONE',  ( -0.5364919789714478471, 0.6444004775717705469, -0.5449076811759709926 ) ) ;
#43746=DIRECTION ( 'NONE',  ( 0.007781995580012663651, -3.146120232559066537E-19, -0.9999697198139514409 ) ) ;
#43747=EDGE_LOOP ( 'NONE', ( #29980, #11693, #56213, #44366, #53302 ) ) ;
#43748=EDGE_LOOP ( 'NONE', ( #42300, #34198, #9007, #472 ) ) ;
#43749=AXIS2_PLACEMENT_3D ( 'NONE', #40864, #36613, #5969 ) ;
#43750=LINE ( 'NONE', #34991, #16399 ) ;
#43751=ORIENTED_EDGE ( 'NONE', *, *, #39713, .F. ) ;
#43752=AXIS2_PLACEMENT_3D ( 'NONE', #922, #5478, #4381 ) ;
#43753=CARTESIAN_POINT ( 'NONE',  ( -10.21874653840805891, 0.000000000000000000, 3.832892323933682732 ) ) ;
#43754=EDGE_LOOP ( 'NONE', ( #47740, #32530, #1436, #18951 ) ) ;
#43755=LINE ( 'NONE', #26183, #24216 ) ;
#43756=CARTESIAN_POINT ( 'NONE',  ( -17.74560456716937296, 0.000000000000000000, 3.774316574337878372 ) ) ;
#43757=AXIS2_PLACEMENT_3D ( 'NONE', #25506, #29200, #34331 ) ;
#43759=ORIENTED_EDGE ( 'NONE', *, *, #31657, .F. ) ;
#43760=FACE_OUTER_BOUND ( 'NONE', #5151, .T. ) ;
#43761=EDGE_CURVE ( 'NONE', #27148, #31034, #20325, .T. ) ;
#43762=VERTEX_POINT ( 'NONE', #7549 ) ;
#43763=AXIS2_PLACEMENT_3D ( 'NONE', #50860, #32704, #16232 ) ;
#43764=DIRECTION ( 'NONE',  ( -0.9321478471874540261, 0.000000000000000000, 0.3620778797217457656 ) ) ;
#43765=VECTOR ( 'NONE', #5652, 1000.000000000000000 ) ;
#43766=ORIENTED_EDGE ( 'NONE', *, *, #39081, .T. ) ;
#43767=LINE ( 'NONE', #27584, #38530 ) ;
#43768=CARTESIAN_POINT ( 'NONE',  ( -16.26034385173145580, 0.000000000000000000, 3.955201230244533850 ) ) ;
#43769=CARTESIAN_POINT ( 'NONE',  ( -15.75813278794938732, -0.5179957512181557755, 2.985788263993758296 ) ) ;
#43770=ORIENTED_EDGE ( 'NONE', *, *, #53471, .F. ) ;
#43771=DIRECTION ( 'NONE',  ( 0.9999697198139515519, 0.000000000000000000, 0.007781995580013368816 ) ) ;
#43772=LINE ( 'NONE', #55728, #24628 ) ;
#43773=CARTESIAN_POINT ( 'NONE',  ( -12.33850799832341849, 0.000000000000000000, 11.68350162852954632 ) ) ;
#43774=VECTOR ( 'NONE', #6776, 1000.000000000000227 ) ;
#43775=DIRECTION ( 'NONE',  ( 0.007781995580012662783, 0.000000000000000000, -0.9999697198139514409 ) ) ;
#43776=VECTOR ( 'NONE', #22483, 1000.000000000000227 ) ;
#43777=FACE_OUTER_BOUND ( 'NONE', #53602, .T. ) ;
#43778=CARTESIAN_POINT ( 'NONE',  ( -17.29901497746887173, -0.1191753592594167882, 5.155117288905197270 ) ) ;
#43780=( LENGTH_UNIT ( ) NAMED_UNIT ( * ) SI_UNIT ( .MILLI., .METRE. ) );
#43781=ORIENTED_EDGE ( 'NONE', *, *, #52802, .F. ) ;
#43782=PLANE ( 'NONE',  #20742 ) ;
#43783=PLANE ( 'NONE',  #38596 ) ;
#43784=CARTESIAN_POINT ( 'NONE',  ( -14.20280369269832832, 0.000000000000000000, 12.40765738797303719 ) ) ;
#43785=VERTEX_POINT ( 'NONE', #47576 ) ;
#43786=CARTESIAN_POINT ( 'NONE',  ( -20.28958894222632736, -4.241740624735664156, 4.627152765803700163 ) ) ;
#43787=ORIENTED_EDGE ( 'NONE', *, *, #2534, .F. ) ;
#43788=VECTOR ( 'NONE', #44215, 999.9999999999998863 ) ;
#43789=DIRECTION ( 'NONE',  ( -0.005961354470445682716, -0.6427876096865404731, 0.7660212471507180654 ) ) ;
#43790=ADVANCED_FACE ( 'NONE', ( #37663 ), #1259, .F. ) ;
#43791=CARTESIAN_POINT ( 'NONE',  ( -11.47013034581549462, -2.622721114510659479, 1.253030735756987424 ) ) ;
#43792=AXIS2_PLACEMENT_3D ( 'NONE', #2017, #32446, #49478 ) ;
#43793=PLANE ( 'NONE',  #26897 ) ;
#43794=EDGE_CURVE ( 'NONE', #329, #38597, #17771, .T. ) ;
#43795=CARTESIAN_POINT ( 'NONE',  ( -10.42005813676012949, 0.000000000000000000, 4.000651684112655815 ) ) ;
#43796=ORIENTED_EDGE ( 'NONE', *, *, #4691, .T. ) ;
#43797=ORIENTED_EDGE ( 'NONE', *, *, #2621, .F. ) ;
#43798=DIRECTION ( 'NONE',  ( 0.7660212471507180654, -0.6427876096865404731, 0.005961354470445141482 ) ) ;
#43800=AXIS2_PLACEMENT_3D ( 'NONE', #3455, #25581, #8265 ) ;
#43801=CARTESIAN_POINT ( 'NONE',  ( -26.13337879274045505, 0.000000000000000000, 6.833023547870798353 ) ) ;
#43802=VECTOR ( 'NONE', #44184, 1000.000000000000227 ) ;
#43803=DIRECTION ( 'NONE',  ( 0.5364919789714477361, 0.6444004775717706579, 0.5449076811759711036 ) ) ;
#43804=ADVANCED_FACE ( 'NONE', ( #22847 ), #44169, .F. ) ;
#43806=DIRECTION ( 'NONE',  ( 0.5364919789714477361, 0.6444004775717706579, 0.5449076811759711036 ) ) ;
#43807=DIRECTION ( 'NONE',  ( 0.9999697198139515519, 0.000000000000000000, 0.007781995580013368816 ) ) ;
#43808=ORIENTED_EDGE ( 'NONE', *, *, #49248, .F. ) ;
#43810=ADVANCED_FACE ( 'NONE', ( #40167 ), #9815, .F. ) ;
#43811=VECTOR ( 'NONE', #51388, 999.9999999999998863 ) ;
#43813=VECTOR ( 'NONE', #2156, 999.9999999999998863 ) ;
#43814=VERTEX_POINT ( 'NONE', #5274 ) ;
#43816=PLANE ( 'NONE',  #32290 ) ;
#43817=PLANE ( 'NONE',  #32057 ) ;
#43818=ORIENTED_EDGE ( 'NONE', *, *, #33888, .T. ) ;
#43819=CARTESIAN_POINT ( 'NONE',  ( -14.46888367232926420, 0.000000000000000000, 12.59025272694991315 ) ) ;
#43820=VERTEX_POINT ( 'NONE', #22008 ) ;
#43821=VECTOR ( 'NONE', #35390, 1000.000000000000227 ) ;
#43822=ORIENTED_EDGE ( 'NONE', *, *, #36983, .T. ) ;
#43823=ORIENTED_EDGE ( 'NONE', *, *, #13380, .F. ) ;
#43824=VERTEX_POINT ( 'NONE', #34795 ) ;
#43825=CARTESIAN_POINT ( 'NONE',  ( -16.60113548713373888, 2.391131607591508335, 3.054086914397361685 ) ) ;
#43826=EDGE_LOOP ( 'NONE', ( #6425, #10741, #8864, #35994 ) ) ;
#43828=AXIS2_PLACEMENT_3D ( 'NONE', #45502, #11453, #37555 ) ;
#43829=CARTESIAN_POINT ( 'NONE',  ( -11.77243710274829525, -0.1191753592594197858, 11.50324088822667612 ) ) ;
#43830=ORIENTED_EDGE ( 'NONE', *, *, #39985, .F. ) ;
#43831=DIRECTION ( 'NONE',  ( 0.5449076811759707706, 0.6444004775717708799, -0.5364919789714476250 ) ) ;
#43832=VERTEX_POINT ( 'NONE', #9225 ) ;
#43833=DIRECTION ( 'NONE',  ( -0.7660212471507179544, -0.6427876096865405842, -0.005961354470445141482 ) ) ;
#43834=EDGE_CURVE ( 'NONE', #20287, #26373, #18597, .T. ) ;
#43835=VECTOR ( 'NONE', #33542, 999.9999999999998863 ) ;
#43836=VERTEX_POINT ( 'NONE', #22583 ) ;
#43837=EDGE_CURVE ( 'NONE', #55008, #17361, #4981, .T. ) ;
#43838=DIRECTION ( 'NONE',  ( 0.9999697198139515519, 0.000000000000000000, 0.007781995580013368816 ) ) ;
#43840=EDGE_CURVE ( 'NONE', #30649, #29572, #425, .T. ) ;
#43841=LINE ( 'NONE', #39032, #24967 ) ;
#43842=DIRECTION ( 'NONE',  ( 0.5449076811759707706, 0.6444004775717708799, -0.5364919789714476250 ) ) ;
#43843=VECTOR ( 'NONE', #40500, 1000.000000000000114 ) ;
#43844=CARTESIAN_POINT ( 'NONE',  ( -15.39653247616405096, 2.067327705546508021, 2.596509236221068218 ) ) ;
#43845=ORIENTED_EDGE ( 'NONE', *, *, #15372, .T. ) ;
#43846=EDGE_CURVE ( 'NONE', #49012, #17901, #53263, .T. ) ;
#43847=EDGE_CURVE ( 'NONE', #43483, #13988, #39893, .T. ) ;
#43848=EDGE_CURVE ( 'NONE', #1080, #13383, #35104, .T. ) ;
#43849=VECTOR ( 'NONE', #18496, 999.9999999999998863 ) ;
#43850=AXIS2_PLACEMENT_3D ( 'NONE', #40552, #14146, #23494 ) ;
#43851=ORIENTED_EDGE ( 'NONE', *, *, #32980, .F. ) ;
#43852=LINE ( 'NONE', #25696, #49418 ) ;
#43853=CARTESIAN_POINT ( 'NONE',  ( -18.67619601524082285, 0.000000000000000000, 3.936400510096834893 ) ) ;
#43854=LINE ( 'NONE', #31377, #46008 ) ;
#43855=AXIS2_PLACEMENT_3D ( 'NONE', #5855, #9845, #19457 ) ;
#43856=VECTOR ( 'NONE', #17258, 999.9999999999998863 ) ;
#43857=CARTESIAN_POINT ( 'NONE',  ( -14.94421173320987428, 3.686347215771509145, 8.736084265198291732 ) ) ;
#43858=FACE_OUTER_BOUND ( 'NONE', #4782, .T. ) ;
#43859=CARTESIAN_POINT ( 'NONE',  ( -19.49503486152984166, 0.000000000000000000, 7.454022801337932158 ) ) ;
#43860=ORIENTED_EDGE ( 'NONE', *, *, #52572, .T. ) ;
#43861=DIRECTION ( 'NONE',  ( -0.8531650599175527594, 0.4028455766673922356, 0.3313982828793700652 ) ) ;
#43863=ORIENTED_EDGE ( 'NONE', *, *, #33366, .T. ) ;
#43864=DIRECTION ( 'NONE',  ( 0.6427681459581294776, -0.7660444431189769032, 0.005002170337467562802 ) ) ;
#43865=PLANE ( 'NONE',  #35125 ) ;
#43866=EDGE_CURVE ( 'NONE', #5703, #55216, #48408, .T. ) ;
#43867=DIRECTION ( 'NONE',  ( 0.9999697198139515519, 0.000000000000000000, 0.007781995580013368816 ) ) ;
#43868=DIRECTION ( 'NONE',  ( -0.005961354470445682716, -0.6427876096865404731, 0.7660212471507180654 ) ) ;
#43869=EDGE_CURVE ( 'NONE', #12359, #13117, #30818, .T. ) ;
#43870=PLANE ( 'NONE',  #21092 ) ;
#43871=ORIENTED_EDGE ( 'NONE', *, *, #11788, .F. ) ;
#43872=VECTOR ( 'NONE', #10322, 999.9999999999998863 ) ;
#43873=ORIENTED_EDGE ( 'NONE', *, *, #38698, .T. ) ;
#43874=ADVANCED_FACE ( 'NONE', ( #13504 ), #4432, .F. ) ;
#43875=LINE ( 'NONE', #30825, #357 ) ;
#43876=DIRECTION ( 'NONE',  ( -0.005961354470445682716, -0.6427876096865404731, 0.7660212471507180654 ) ) ;
#43877=CARTESIAN_POINT ( 'NONE',  ( -9.939733318003350249, 0.000000000000000000, 1.988403320296867616 ) ) ;
#43878=AXIS2_PLACEMENT_3D ( 'NONE', #47335, #8752, #25768 ) ;
#43880=DIRECTION ( 'NONE',  ( -0.7660212471507179544, -0.6427876096865405842, -0.005961354470445141482 ) ) ;
#43881=CARTESIAN_POINT ( 'NONE',  ( -10.76754721030951245, -0.6798977022406572646, 1.042109824751433989 ) ) ;
#43882=VECTOR ( 'NONE', #31459, 1000.000000000000000 ) ;
#43884=DIRECTION ( 'NONE',  ( 0.000000000000000000, -0.000000000000000000, -1.000000000000000000 ) ) ;
#43885=CARTESIAN_POINT ( 'NONE',  ( -18.39746900504187010, 0.000000000000000000, 14.03700784672088808 ) ) ;
#43886=DIRECTION ( 'NONE',  ( 0.000000000000000000, -0.000000000000000000, -1.000000000000000000 ) ) ;
#43888=EDGE_LOOP ( 'NONE', ( #1511, #11157, #44190, #30521 ) ) ;
#43889=CARTESIAN_POINT ( 'NONE',  ( -21.47263955680318404, 0.000000000000000000, 5.022634149262071190 ) ) ;
#43890=ORIENTED_EDGE ( 'NONE', *, *, #5466, .F. ) ;
#43891=PLANE ( 'NONE',  #46782 ) ;
#43892=DIRECTION ( 'NONE',  ( -0.7660212471507179544, -0.6427876096865405842, -0.005961354470445141482 ) ) ;
#43893=VECTOR ( 'NONE', #23339, 1000.000000000000114 ) ;
#43894=ORIENTED_EDGE ( 'NONE', *, *, #17022, .F. ) ;
#43895=EDGE_LOOP ( 'NONE', ( #50020, #16219, #6441, #46532 ) ) ;
#43896=AXIS2_PLACEMENT_3D ( 'NONE', #7029, #49878, #24053 ) ;
#43897=VERTEX_POINT ( 'NONE', #13227 ) ;
#43898=ORIENTED_EDGE ( 'NONE', *, *, #3306, .F. ) ;
#43899=VECTOR ( 'NONE', #24582, 1000.000000000000000 ) ;
#43900=ORIENTED_EDGE ( 'NONE', *, *, #39675, .T. ) ;
#43901=ORIENTED_EDGE ( 'NONE', *, *, #17503, .F. ) ;
#43902=LINE ( 'NONE', #13268, #46528 ) ;
#43904=VERTEX_POINT ( 'NONE', #47869 ) ;
#43905=CARTESIAN_POINT ( 'NONE',  ( -12.23851102634202448, -0.1191753592594197858, 11.68427982808754884 ) ) ;
#43906=ORIENTED_EDGE ( 'NONE', *, *, #14710, .F. ) ;
#43907=ORIENTED_EDGE ( 'NONE', *, *, #38550, .F. ) ;
#43908=VECTOR ( 'NONE', #7967, 1000.000000000000114 ) ;
#43909=DIRECTION ( 'NONE',  ( -0.7660212471507179544, -0.6427876096865405842, -0.005961354470445141482 ) ) ;
#43910=VECTOR ( 'NONE', #45772, 999.9999999999998863 ) ;
#43911=LINE ( 'NONE', #31136, #5870 ) ;
#43912=LINE ( 'NONE', #9577, #25961 ) ;
#43913=VERTEX_POINT ( 'NONE', #8970 ) ;
#43914=PLANE ( 'NONE',  #18325 ) ;
#43915=VECTOR ( 'NONE', #49531, 1000.000000000000114 ) ;
#43916=VERTEX_POINT ( 'NONE', #49809 ) ;
#43917=EDGE_CURVE ( 'NONE', #14283, #36681, #41000, .T. ) ;
#43918=ADVANCED_FACE ( 'NONE', ( #50369 ), #6123, .F. ) ;
#43919=LINE ( 'NONE', #9016, #3042 ) ;
#43920=EDGE_CURVE ( 'NONE', #13117, #11647, #19137, .T. ) ;
#43921=CARTESIAN_POINT ( 'NONE',  ( -13.48689273821135259, 0.000000000000000000, 5.823445217141414609 ) ) ;
#43922=DIRECTION ( 'NONE',  ( 0.005961354470445682716, -0.6427876096865404731, -0.7660212471507180654 ) ) ;
#43923=LINE ( 'NONE', #5047, #52116 ) ;
#43924=CARTESIAN_POINT ( 'NONE',  ( -9.312465172768151334, 0.000000000000000000, 6.794601773531817379 ) ) ;
#43925=DIRECTION ( 'NONE',  ( 0.000000000000000000, -0.000000000000000000, -1.000000000000000000 ) ) ;
#43926=VECTOR ( 'NONE', #4789, 1000.000000000000227 ) ;
#43927=DIRECTION ( 'NONE',  ( -0.005961354470445682716, -0.6427876096865404731, 0.7660212471507180654 ) ) ;
#43928=ORIENTED_EDGE ( 'NONE', *, *, #37142, .F. ) ;
#43929=CARTESIAN_POINT ( 'NONE',  ( -10.47421230394850866, 0.000000000000000000, 10.95934586908605723 ) ) ;
#43930=AXIS2_PLACEMENT_3D ( 'NONE', #15022, #46209, #37412 ) ;
#43931=DIRECTION ( 'NONE',  ( 0.007781995580012663651, -3.146120232559066537E-19, -0.9999697198139514409 ) ) ;
#43932=CARTESIAN_POINT ( 'NONE',  ( -9.480844528172831076, 0.000000000000000000, 2.730638638580407118 ) ) ;
#43933=PLANE ( 'NONE',  #36299 ) ;
#43936=ADVANCED_FACE ( 'NONE', ( #36462 ), #23427, .F. ) ;
#43937=DIRECTION ( 'NONE',  ( -0.6246952433987893460, -0.7422098413412802076, 0.2426528472758542054 ) ) ;
#43938=AXIS2_PLACEMENT_3D ( 'NONE', #23625, #45222, #23082 ) ;
#43939=CARTESIAN_POINT ( 'NONE',  ( -9.808144436391993182, 0.000000000000000000, 10.77986332834118777 ) ) ;
#43940=VECTOR ( 'NONE', #20262, 999.9999999999998863 ) ;
#43941=ORIENTED_EDGE ( 'NONE', *, *, #20121, .T. ) ;
#43942=EDGE_CURVE ( 'NONE', #17442, #52077, #54081, .T. ) ;
#43943=LINE ( 'NONE', #48790, #40219 ) ;
#43944=CARTESIAN_POINT ( 'NONE',  ( -25.20123094555300369, 0.000000000000000000, 6.470945668149052032 ) ) ;
#43945=DIRECTION ( 'NONE',  ( 0.9999697198139515519, 0.000000000000000000, 0.007781995580013368816 ) ) ;
#43946=EDGE_CURVE ( 'NONE', #31801, #5857, #53778, .T. ) ;
#43947=CARTESIAN_POINT ( 'NONE',  ( -12.80458192191714595, 0.000000000000000000, 11.86454056839041726 ) ) ;
#43948=LINE ( 'NONE', #17859, #34875 ) ;
#43949=DIRECTION ( 'NONE',  ( 0.7660212471507180654, -0.6427876096865404731, 0.005961354470445141482 ) ) ;
#43950=FACE_OUTER_BOUND ( 'NONE', #26852, .T. ) ;
#43951=EDGE_CURVE ( 'NONE', #12635, #17633, #36208, .T. ) ;
#43952=AXIS2_PLACEMENT_3D ( 'NONE', #10446, #53857, #54408 ) ;
#43954=VECTOR ( 'NONE', #3738, 1000.000000000000227 ) ;
#43955=CARTESIAN_POINT ( 'NONE',  ( -9.442067484779661513, -0.1191753592594197858, 10.59804618892231254 ) ) ;
#43957=ORIENTED_EDGE ( 'NONE', *, *, #5299, .F. ) ;
#43958=VECTOR ( 'NONE', #19888, 999.9999999999998863 ) ;
#43959=ORIENTED_EDGE ( 'NONE', *, *, #11402, .T. ) ;
#43960=VERTEX_POINT ( 'NONE', #1811 ) ;
#43961=VECTOR ( 'NONE', #21236, 1000.000000000000114 ) ;
#43962=VECTOR ( 'NONE', #45809, 1000.000000000000227 ) ;
#43963=ORIENTED_EDGE ( 'NONE', *, *, #1623, .F. ) ;
#43964=VECTOR ( 'NONE', #34152, 999.9999999999998863 ) ;
#43965=EDGE_LOOP ( 'NONE', ( #27874, #28075, #9962, #7891 ) ) ;
#43966=FACE_OUTER_BOUND ( 'NONE', #42995, .T. ) ;
#43967=DIRECTION ( 'NONE',  ( 0.007781995580012663651, 0.000000000000000000, -0.9999697198139515519 ) ) ;
#43968=VECTOR ( 'NONE', #27042, 1000.000000000000227 ) ;
#43969=EDGE_LOOP ( 'NONE', ( #49553, #26258, #29308, #23997 ) ) ;
#43970=ORIENTED_EDGE ( 'NONE', *, *, #18533, .F. ) ;
#43971=AXIS2_PLACEMENT_3D ( 'NONE', #40331, #41165, #18461 ) ;
#43972=VECTOR ( 'NONE', #47011, 999.9999999999998863 ) ;
#43973=PLANE ( 'NONE',  #39396 ) ;
#43975=DIRECTION ( 'NONE',  ( 0.000000000000000000, -0.000000000000000000, -1.000000000000000000 ) ) ;
#43976=LINE ( 'NONE', #41661, #27784 ) ;
#43977=ORIENTED_EDGE ( 'NONE', *, *, #40404, .T. ) ;
#43978=DIRECTION ( 'NONE',  ( 0.007781995580012663651, 0.000000000000000000, -0.9999697198139515519 ) ) ;
#43979=ADVANCED_FACE ( 'NONE', ( #32225 ), #10664, .F. ) ;
#43980=ORIENTED_EDGE ( 'NONE', *, *, #27906, .T. ) ;
#43981=LINE ( 'NONE', #35460, #30040 ) ;
#43982=CARTESIAN_POINT ( 'NONE',  ( -12.77066550162910730, 0.000000000000000000, 7.506353398555276613 ) ) ;
#43983=ADVANCED_FACE ( 'NONE', ( #40474 ), #45276, .F. ) ;
#43984=EDGE_CURVE ( 'NONE', #51541, #38019, #6650, .T. ) ;
#43985=AXIS2_PLACEMENT_3D ( 'NONE', #4697, #14073, #4438 ) ;
#43986=DIRECTION ( 'NONE',  ( 0.5364919789714477361, 0.6444004775717706579, 0.5449076811759711036 ) ) ;
#43987=DIRECTION ( 'NONE',  ( -0.9999697198139514409, -0.000000000000000000, -0.007781995580013368816 ) ) ;
#43988=VERTEX_POINT ( 'NONE', #41296 ) ;
#43989=DIRECTION ( 'NONE',  ( 0.000000000000000000, -0.000000000000000000, -1.000000000000000000 ) ) ;
#43990=LINE ( 'NONE', #44537, #13865 ) ;
#43991=DIRECTION ( 'NONE',  ( 0.007781995580012663651, 0.000000000000000000, -0.9999697198139515519 ) ) ;
#43992=VECTOR ( 'NONE', #5865, 1000.000000000000000 ) ;
#43993=VERTEX_POINT ( 'NONE', #23679 ) ;
#43994=LINE ( 'NONE', #38908, #21060 ) ;
#43995=ORIENTED_EDGE ( 'NONE', *, *, #40275, .T. ) ;
#43996=AXIS2_PLACEMENT_3D ( 'NONE', #20625, #33950, #27827 ) ;
#43997=PLANE ( 'NONE',  #14716 ) ;
#43998=DIRECTION ( 'NONE',  ( -0.005002170337468016433, -0.7660444431189770143, 0.6427681459581293666 ) ) ;
#43999=CARTESIAN_POINT ( 'NONE',  ( -17.62617585138765008, -3.117730071725258956, 12.26528855537868701 ) ) ;
#44000=LINE ( 'NONE', #34941, #23235 ) ;
#44001=AXIS2_PLACEMENT_3D ( 'NONE', #34019, #46796, #46207 ) ;
#44002=DIRECTION ( 'NONE',  ( -0.7660212471507179544, -0.6427876096865405842, -0.005961354470445141482 ) ) ;
#44003=DIRECTION ( 'NONE',  ( 0.005002170337468016433, -0.7660444431189770143, -0.6427681459581293666 ) ) ;
#44005=DIRECTION ( 'NONE',  ( 0.000000000000000000, -0.000000000000000000, -1.000000000000000000 ) ) ;
#44006=AXIS2_PLACEMENT_3D ( 'NONE', #51171, #42085, #12287 ) ;
#44007=VECTOR ( 'NONE', #12525, 1000.000000000000227 ) ;
#44008=AXIS2_PLACEMENT_3D ( 'NONE', #8103, #39312, #25410 ) ;
#44009=CARTESIAN_POINT ( 'NONE',  ( -13.53673582514181106, 0.000000000000000000, 12.22817484722816772 ) ) ;
#44010=ORIENTED_EDGE ( 'NONE', *, *, #23577, .T. ) ;
#44011=CARTESIAN_POINT ( 'NONE',  ( -16.26609195874202385, 0.000000000000000000, 4.693820636760064779 ) ) ;
#44012=CARTESIAN_POINT ( 'NONE',  ( -14.20280369269832832, 0.000000000000000000, 12.40765738797303719 ) ) ;
#44013=LINE ( 'NONE', #18448, #39943 ) ;
#44014=LINE ( 'NONE', #18449, #14205 ) ;
#44015=VECTOR ( 'NONE', #19783, 999.9999999999998863 ) ;
#44016=AXIS2_PLACEMENT_3D ( 'NONE', #18412, #35454, #22960 ) ;
#44017=DIRECTION ( 'NONE',  ( 0.005961354470445682716, -0.6427876096865404731, -0.7660212471507180654 ) ) ;
#44018=EDGE_CURVE ( 'NONE', #9219, #46158, #2389, .T. ) ;
#44019=DIRECTION ( 'NONE',  ( -0.005002170337468016433, -0.7660444431189770143, 0.6427681459581293666 ) ) ;
#44020=CARTESIAN_POINT ( 'NONE',  ( -10.41586642886556824, 0.000000000000000000, 3.462026221559915129 ) ) ;
#44021=ORIENTED_EDGE ( 'NONE', *, *, #25804, .F. ) ;
#44022=AXIS2_PLACEMENT_3D ( 'NONE', #35252, #30426, #26161 ) ;
#44024=ORIENTED_EDGE ( 'NONE', *, *, #47449, .T. ) ;
#44025=EDGE_CURVE ( 'NONE', #33489, #22565, #37040, .T. ) ;
#44026=LINE ( 'NONE', #35496, #15990 ) ;
#44027=LINE ( 'NONE', #53396, #24989 ) ;
#44028=ORIENTED_EDGE ( 'NONE', *, *, #18134, .F. ) ;
#44030=EDGE_CURVE ( 'NONE', #11534, #32995, #54343, .T. ) ;
#44031=EDGE_LOOP ( 'NONE', ( #1338, #50684, #31048, #34187 ) ) ;
#44032=DIRECTION ( 'NONE',  ( 0.9999697198139515519, 0.000000000000000000, 0.007781995580013368816 ) ) ;
#44033=VECTOR ( 'NONE', #39778, 999.9999999999998863 ) ;
#44034=ORIENTED_EDGE ( 'NONE', *, *, #30414, .T. ) ;
#44035=ORIENTED_EDGE ( 'NONE', *, *, #24727, .F. ) ;
#44036=ORIENTED_EDGE ( 'NONE', *, *, #16582, .F. ) ;
#44038=DIRECTION ( 'NONE',  ( -0.5364919789714478471, 0.6444004775717705469, -0.5449076811759709926 ) ) ;
#44039=CARTESIAN_POINT ( 'NONE',  ( -6.777710503706796175, -6.513112611849074085, -0.5856806440065189800 ) ) ;
#44040=AXIS2_PLACEMENT_3D ( 'NONE', #56159, #4216, #51613 ) ;
#44041=DIRECTION ( 'NONE',  ( 0.9999697198139515519, 0.000000000000000000, 0.007781995580013368816 ) ) ;
#44042=DIRECTION ( 'NONE',  ( -0.005002170337468016433, -0.7660444431189770143, 0.6427681459581293666 ) ) ;
#44043=ORIENTED_EDGE ( 'NONE', *, *, #26490, .F. ) ;
#44044=VECTOR ( 'NONE', #2577, 1000.000000000000227 ) ;
#44045=ORIENTED_EDGE ( 'NONE', *, *, #28296, .T. ) ;
#44046=EDGE_CURVE ( 'NONE', #24636, #39671, #49246, .T. ) ;
#44047=VECTOR ( 'NONE', #13129, 1000.000000000000227 ) ;
#44048=VECTOR ( 'NONE', #41327, 1000.000000000000227 ) ;
#44049=LINE ( 'NONE', #40057, #7323 ) ;
#44050=ORIENTED_EDGE ( 'NONE', *, *, #13746, .T. ) ;
#44051=FACE_OUTER_BOUND ( 'NONE', #39381, .T. ) ;
#44052=ADVANCED_FACE ( 'NONE', ( #19974 ), #24259, .F. ) ;
#44053=ORIENTED_EDGE ( 'NONE', *, *, #28812, .F. ) ;
#44054=DIRECTION ( 'NONE',  ( 0.000000000000000000, -0.000000000000000000, -1.000000000000000000 ) ) ;
#44055=DIRECTION ( 'NONE',  ( -0.9999697198139514409, -0.000000000000000000, -0.007781995580013368816 ) ) ;
#44056=VECTOR ( 'NONE', #24801, 1000.000000000000114 ) ;
#44057=VERTEX_POINT ( 'NONE', #15712 ) ;
#44058=AXIS2_PLACEMENT_3D ( 'NONE', #55033, #53888, #36580 ) ;
#44059=EDGE_CURVE ( 'NONE', #36108, #27112, #33049, .T. ) ;
#44060=LINE ( 'NONE', #53679, #10509 ) ;
#44061=VECTOR ( 'NONE', #23824, 1000.000000000000227 ) ;
#44062=ORIENTED_EDGE ( 'NONE', *, *, #14006, .F. ) ;
#44063=EDGE_CURVE ( 'NONE', #31769, #23301, #5820, .T. ) ;
#44064=VECTOR ( 'NONE', #25389, 1000.000000000000227 ) ;
#44065=FACE_OUTER_BOUND ( 'NONE', #38320, .T. ) ;
#44066=VECTOR ( 'NONE', #50282, 1000.000000000000227 ) ;
#44067=EDGE_LOOP ( 'NONE', ( #8548, #12042, #11882, #120, #18700 ) ) ;
#44068=PLANE ( 'NONE',  #34900 ) ;
#44069=DIRECTION ( 'NONE',  ( 0.005002170337468016433, -0.7660444431189770143, -0.6427681459581293666 ) ) ;
#44070=FACE_OUTER_BOUND ( 'NONE', #14232, .T. ) ;
#44071=ORIENTED_EDGE ( 'NONE', *, *, #18306, .F. ) ;
#44072=DIRECTION ( 'NONE',  ( -0.6246952433987893460, -0.7422098413412802076, 0.2426528472758542054 ) ) ;
#44073=FACE_OUTER_BOUND ( 'NONE', #17883, .T. ) ;
#44074=DIRECTION ( 'NONE',  ( -0.005002170337468016433, -0.7660444431189770143, 0.6427681459581293666 ) ) ;
#44076=CARTESIAN_POINT ( 'NONE',  ( -12.13851405436063047, 0.000000000000000000, 11.68505802764555135 ) ) ;
#44077=DIRECTION ( 'NONE',  ( -0.6246952433987894571, 0.7422098413412802076, 0.2426528472758539834 ) ) ;
#44078=VECTOR ( 'NONE', #36343, 1000.000000000000114 ) ;
#44079=EDGE_CURVE ( 'NONE', #93, #49846, #7476, .T. ) ;
#44081=EDGE_LOOP ( 'NONE', ( #52156, #35639, #43078, #19831 ) ) ;
#44082=DIRECTION ( 'NONE',  ( 0.000000000000000000, -0.000000000000000000, -1.000000000000000000 ) ) ;
#44083=DIRECTION ( 'NONE',  ( -0.005961354470445682716, -0.6427876096865404731, 0.7660212471507180654 ) ) ;
#44084=CARTESIAN_POINT ( 'NONE',  ( -16.33317936670417225, 0.000000000000000000, 13.31440848639340224 ) ) ;
#44085=ORIENTED_EDGE ( 'NONE', *, *, #5531, .F. ) ;
#44086=DIRECTION ( 'NONE',  ( -0.005961354470445682716, -0.6427876096865404731, 0.7660212471507180654 ) ) ;
#44087=DIRECTION ( 'NONE',  ( 0.9999697198139515519, 0.000000000000000000, 0.007781995580013368816 ) ) ;
#44088=VECTOR ( 'NONE', #12002, 999.9999999999998863 ) ;
#44089=EDGE_LOOP ( 'NONE', ( #54505, #40841, #543, #31829 ) ) ;
#44091=DIRECTION ( 'NONE',  ( -0.6246952433987893460, -0.7422098413412802076, 0.2426528472758542054 ) ) ;
#44092=AXIS2_PLACEMENT_3D ( 'NONE', #11608, #28928, #24641 ) ;
#44093=CARTESIAN_POINT ( 'NONE',  ( -13.63673279712320507, -0.1191753592594197858, 12.22739664767016521 ) ) ;
#44094=CARTESIAN_POINT ( 'NONE',  ( -15.86710544311044302, 0.000000000000000000, 13.13336954653252953 ) ) ;
#44095=ORIENTED_EDGE ( 'NONE', *, *, #3961, .T. ) ;
#44096=VECTOR ( 'NONE', #50770, 999.9999999999998863 ) ;
#44097=AXIS2_PLACEMENT_3D ( 'NONE', #23592, #15354, #41733 ) ;
#44098=VERTEX_POINT ( 'NONE', #47995 ) ;
#44100=DIRECTION ( 'NONE',  ( 0.9999697198139515519, 0.000000000000000000, 0.007781995580013368816 ) ) ;
#44102=AXIS2_PLACEMENT_3D ( 'NONE', #6700, #50691, #24015 ) ;
#44103=DIRECTION ( 'NONE',  ( -0.6427681459581293666, -0.7660444431189770143, -0.005002170337467561935 ) ) ;
#44104=VECTOR ( 'NONE', #47000, 1000.000000000000114 ) ;
#44105=DIRECTION ( 'NONE',  ( 0.5449076811759707706, 0.6444004775717708799, -0.5364919789714476250 ) ) ;
#44106=DIRECTION ( 'NONE',  ( 0.005961354470445682716, -0.6427876096865404731, -0.7660212471507180654 ) ) ;
#44107=EDGE_CURVE ( 'NONE', #55375, #38787, #12321, .T. ) ;
#44108=ORIENTED_EDGE ( 'NONE', *, *, #1013, .T. ) ;
#44109=DIRECTION ( 'NONE',  ( 0.7660212471507180654, -0.6427876096865404731, 0.005961354470445141482 ) ) ;
#44110=VECTOR ( 'NONE', #13106, 999.9999999999998863 ) ;
#44111=AXIS2_PLACEMENT_3D ( 'NONE', #33890, #20560, #32758 ) ;
#44112=LINE ( 'NONE', #55765, #12448 ) ;
#44113=ORIENTED_EDGE ( 'NONE', *, *, #39323, .F. ) ;
#44114=DIRECTION ( 'NONE',  ( -0.3620778797217456546, 0.000000000000000000, -0.9321478471874540261 ) ) ;
#44115=LINE ( 'NONE', #48662, #31343 ) ;
#44116=DIRECTION ( 'NONE',  ( 0.6427681459581294776, -0.7660444431189769032, 0.005002170337467562802 ) ) ;
#44117=EDGE_CURVE ( 'NONE', #55206, #26525, #52268, .T. ) ;
#44118=ORIENTED_EDGE ( 'NONE', *, *, #11973, .F. ) ;
#44119=DIRECTION ( 'NONE',  ( 0.9999697198139515519, 0.000000000000000000, 0.007781995580013368816 ) ) ;
#44120=ORIENTED_EDGE ( 'NONE', *, *, #43402, .T. ) ;
#44121=EDGE_CURVE ( 'NONE', #48671, #52431, #46362, .T. ) ;
#44122=EDGE_CURVE ( 'NONE', #51697, #15737, #55452, .T. ) ;
#44123=VECTOR ( 'NONE', #17053, 999.9999999999998863 ) ;
#44124=VERTEX_POINT ( 'NONE', #24510 ) ;
#44125=ORIENTED_EDGE ( 'NONE', *, *, #47268, .F. ) ;
#44126=ORIENTED_EDGE ( 'NONE', *, *, #28786, .T. ) ;
#44127=CARTESIAN_POINT ( 'NONE',  ( -13.95596008767372709, 0.000000000000000000, 6.389132952593959303 ) ) ;
#44129=ADVANCED_FACE ( 'NONE', ( #37883 ), #25109, .F. ) ;
#44130=VECTOR ( 'NONE', #22515, 1000.000000000000114 ) ;
#44131=VERTEX_POINT ( 'NONE', #16276 ) ;
#44134=ORIENTED_EDGE ( 'NONE', *, *, #41993, .F. ) ;
#44135=LINE ( 'NONE', #18010, #24096 ) ;
#44136=EDGE_CURVE ( 'NONE', #1292, #31910, #42419, .T. ) ;
#44137=VECTOR ( 'NONE', #7226, 1000.000000000000114 ) ;
#44138=EDGE_LOOP ( 'NONE', ( #54887, #11356, #9073, #3867, #46304 ) ) ;
#44139=DIRECTION ( 'NONE',  ( 0.005002170337468016433, -0.7660444431189770143, -0.6427681459581293666 ) ) ;
#44140=ORIENTED_EDGE ( 'NONE', *, *, #42803, .F. ) ;
#44142=VECTOR ( 'NONE', #32565, 999.9999999999998863 ) ;
#44143=DIRECTION ( 'NONE',  ( 0.007781995580012662783, 0.000000000000000000, -0.9999697198139514409 ) ) ;
#44144=LINE ( 'NONE', #31361, #28384 ) ;
#44145=CARTESIAN_POINT ( 'NONE',  ( 3.004435629306332345, -1.000000000000000000, -3.312607213261892003 ) ) ;
#44146=LINE ( 'NONE', #5255, #31167 ) ;
#44147=LINE ( 'NONE', #13743, #45053 ) ;
#44148=DIRECTION ( 'NONE',  ( -0.5364919789714478471, 0.6444004775717705469, -0.5449076811759709926 ) ) ;
#44149=ORIENTED_EDGE ( 'NONE', *, *, #32131, .F. ) ;
#44150=EDGE_CURVE ( 'NONE', #26242, #52494, #4833, .T. ) ;
#44152=VECTOR ( 'NONE', #14410, 1000.000000000000227 ) ;
#44153=DIRECTION ( 'NONE',  ( -0.6427681459581293666, -0.7660444431189770143, -0.005002170337467561935 ) ) ;
#44154=CARTESIAN_POINT ( 'NONE',  ( -25.20123094555300369, 0.000000000000000000, 6.470945668149052032 ) ) ;
#44155=VECTOR ( 'NONE', #43149, 1000.000000000000227 ) ;
#44156=DIRECTION ( 'NONE',  ( 0.005002170337468016433, -0.7660444431189770143, -0.6427681459581293666 ) ) ;
#44157=EDGE_CURVE ( 'NONE', #38693, #10700, #39490, .T. ) ;
#44158=VECTOR ( 'NONE', #850, 999.9999999999998863 ) ;
#44159=CARTESIAN_POINT ( 'NONE',  ( -18.59945500257930107, 0.000000000000000000, 5.983664131656099450 ) ) ;
#44161=CARTESIAN_POINT ( 'NONE',  ( -11.20636620717317378, 0.000000000000000000, 11.32298014792380414 ) ) ;
#44162=CARTESIAN_POINT ( 'NONE',  ( -25.20278734466900517, 0.000000000000000000, 6.670939612111840944 ) ) ;
#44163=VERTEX_POINT ( 'NONE', #26148 ) ;
#44164=LINE ( 'NONE', #48114, #41095 ) ;
#44165=CARTESIAN_POINT ( 'NONE',  ( -22.40478740399063895, 0.000000000000000000, 5.384712028983816623 ) ) ;
#44166=EDGE_LOOP ( 'NONE', ( #109, #47244, #12031, #29540 ) ) ;
#44168=DIRECTION ( 'NONE',  ( 0.007781995580012663651, 0.000000000000000000, -0.9999697198139515519 ) ) ;
#44169=PLANE ( 'NONE',  #25009 ) ;
#44170=DIRECTION ( 'NONE',  ( -0.6427681459581293666, -0.7660444431189770143, -0.005002170337467561935 ) ) ;
#44171=AXIS2_PLACEMENT_3D ( 'NONE', #52311, #34995, #13413 ) ;
#44172=PLANE ( 'NONE',  #13843 ) ;
#44173=ORIENTED_EDGE ( 'NONE', *, *, #15089, .F. ) ;
#44174=ORIENTED_EDGE ( 'NONE', *, *, #54315, .T. ) ;
#44175=CARTESIAN_POINT ( 'NONE',  ( -12.63252763452103800, -0.1191753592594188005, 2.606108483780943619 ) ) ;
#44176=FACE_OUTER_BOUND ( 'NONE', #2293, .T. ) ;
#44177=CARTESIAN_POINT ( 'NONE',  ( -23.33849165029409889, 0.000000000000000000, 5.946783852668351855 ) ) ;
#44178=CARTESIAN_POINT ( 'NONE',  ( -12.54037462349748822, 0.000000000000000000, 3.614818821130846072 ) ) ;
#44179=AXIS2_PLACEMENT_3D ( 'NONE', #52895, #49188, #48659 ) ;
#44180=CARTESIAN_POINT ( 'NONE',  ( -16.85449645516476380, -0.1191753592594192307, 7.743901123477560766 ) ) ;
#44181=ADVANCED_FACE ( 'NONE', ( #35238 ), #29060, .F. ) ;
#44182=VERTEX_POINT ( 'NONE', #7211 ) ;
#44184=DIRECTION ( 'NONE',  ( -0.9999697198139514409, -0.000000000000000000, -0.007781995580013368816 ) ) ;
#44185=FACE_OUTER_BOUND ( 'NONE', #27413, .T. ) ;
#44186=VECTOR ( 'NONE', #4979, 1000.000000000000114 ) ;
#44187=DIRECTION ( 'NONE',  ( 0.000000000000000000, -0.000000000000000000, -1.000000000000000000 ) ) ;
#44188=ORIENTED_EDGE ( 'NONE', *, *, #6603, .T. ) ;
#44189=FACE_OUTER_BOUND ( 'NONE', #32097, .T. ) ;
#44190=ORIENTED_EDGE ( 'NONE', *, *, #17735, .F. ) ;
#44191=DIRECTION ( 'NONE',  ( 0.6427681459581294776, -0.7660444431189769032, 0.005002170337467562802 ) ) ;
#44192=EDGE_CURVE ( 'NONE', #20216, #40878, #34955, .T. ) ;
#44193=ADVANCED_FACE ( 'NONE', ( #39184 ), #12009, .F. ) ;
#44194=PLANE ( 'NONE',  #4856 ) ;
#44195=EDGE_CURVE ( 'NONE', #24619, #16314, #29348, .T. ) ;
#44196=ORIENTED_EDGE ( 'NONE', *, *, #25394, .T. ) ;
#44197=VECTOR ( 'NONE', #15179, 1000.000000000000000 ) ;
#44198=DIRECTION ( 'NONE',  ( 0.9999697198139515519, 0.000000000000000000, 0.007781995580013368816 ) ) ;
#44200=EDGE_CURVE ( 'NONE', #29572, #1220, #17914, .T. ) ;
#44201=VERTEX_POINT ( 'NONE', #46104 ) ;
#44202=ORIENTED_EDGE ( 'NONE', *, *, #49637, .T. ) ;
#44203=LINE ( 'NONE', #52689, #15755 ) ;
#44204=ORIENTED_EDGE ( 'NONE', *, *, #29286, .F. ) ;
#44206=CARTESIAN_POINT ( 'NONE',  ( -15.00457102831626699, -0.1191753592594181482, 8.866293880322892562 ) ) ;
#44207=DIRECTION ( 'NONE',  ( -0.5364919789714478471, 0.6444004775717705469, -0.5449076811759709926 ) ) ;
#44208=ORIENTED_EDGE ( 'NONE', *, *, #49122, .T. ) ;
#44209=ORIENTED_EDGE ( 'NONE', *, *, #9060, .F. ) ;
#44210=DIRECTION ( 'NONE',  ( 0.9999697198139515519, 0.000000000000000000, 0.007781995580013368816 ) ) ;
#44211=ADVANCED_FACE ( 'NONE', ( #2917 ), #54911, .F. ) ;
#44212=ORIENTED_EDGE ( 'NONE', *, *, #41079, .T. ) ;
#44213=ORIENTED_EDGE ( 'NONE', *, *, #48767, .F. ) ;
#44214=ADVANCED_FACE ( 'NONE', ( #36335 ), #5974, .F. ) ;
#44215=DIRECTION ( 'NONE',  ( 0.9999697198139515519, 0.000000000000000000, 0.007781995580013368816 ) ) ;
#44217=ADVANCED_FACE ( 'NONE', ( #1690 ), #13906, .F. ) ;
#44218=DIRECTION ( 'NONE',  ( 0.5364919789714477361, 0.6444004775717706579, 0.5449076811759711036 ) ) ;
#44219=LINE ( 'NONE', #5319, #38634 ) ;
#44220=VERTEX_POINT ( 'NONE', #48253 ) ;
#44221=CARTESIAN_POINT ( 'NONE',  ( -14.32071356977549925, -5.375054281893163477, 11.06596300975003544 ) ) ;
#44223=EDGE_CURVE ( 'NONE', #15160, #14352, #19015, .T. ) ;
#44224=DIRECTION ( 'NONE',  ( -0.7660212471507179544, -0.6427876096865405842, -0.005961354470445141482 ) ) ;
#44225=PLANE ( 'NONE',  #30625 ) ;
#44226=VECTOR ( 'NONE', #34264, 1000.000000000000227 ) ;
#44227=PLANE ( 'NONE',  #54910 ) ;
#44228=DIRECTION ( 'NONE',  ( 0.9999697198139515519, 0.000000000000000000, 0.007781995580013368816 ) ) ;
#44230=CARTESIAN_POINT ( 'NONE',  ( -5.059434328074208231, -6.953069894654446692, 5.183629687800835661 ) ) ;
#44231=DIRECTION ( 'NONE',  ( 0.007781995580012663651, -3.146120232559066537E-19, -0.9999697198139514409 ) ) ;
#44232=ORIENTED_EDGE ( 'NONE', *, *, #40668, .F. ) ;
#44233=CARTESIAN_POINT ( 'NONE',  ( -16.99924723426068951, 0.000000000000000000, 13.49389102713827171 ) ) ;
#44234=VECTOR ( 'NONE', #44920, 1000.000000000000000 ) ;
#44235=DIRECTION ( 'NONE',  ( 0.000000000000000000, -1.000000000000000000, 0.000000000000000000 ) ) ;
#44236=DIRECTION ( 'NONE',  ( 0.005002170337468016433, -0.7660444431189770143, -0.6427681459581293666 ) ) ;
#44237=DIRECTION ( 'NONE',  ( 0.007781995580012663651, 0.000000000000000000, -0.9999697198139515519 ) ) ;
#44239=PLANE ( 'NONE',  #47631 ) ;
#44240=DIRECTION ( 'NONE',  ( 0.007781995580012663651, 0.000000000000000000, -0.9999697198139515519 ) ) ;
#44241=DIRECTION ( 'NONE',  ( 0.007781995580012663651, 0.000000000000000000, -0.9999697198139515519 ) ) ;
#44243=LINE ( 'NONE', #26624, #8481 ) ;
#44244=CARTESIAN_POINT ( 'NONE',  ( -18.19297601772640860, 2.067327705546506689, 3.682742875386304515 ) ) ;
#44245=CARTESIAN_POINT ( 'NONE',  ( -18.36880263084326259, 0.000000000000000000, 10.35344032464643149 ) ) ;
#44246=EDGE_CURVE ( 'NONE', #43064, #32693, #36618, .T. ) ;
#44248=CARTESIAN_POINT ( 'NONE',  ( -8.875996589204540044, 0.000000000000000000, 10.41778544861944233 ) ) ;
#44249=EDGE_CURVE ( 'NONE', #24292, #33398, #27840, .T. ) ;
#44250=CARTESIAN_POINT ( 'NONE',  ( -18.12906999872765113, 0.000000000000000000, 5.248660636908578425 ) ) ;
#44251=LINE ( 'NONE', #5354, #37386 ) ;
#44253=LINE ( 'NONE', #9311, #2940 ) ;
#44254=EDGE_CURVE ( 'NONE', #33081, #23263, #32082, .T. ) ;
#44256=EDGE_CURVE ( 'NONE', #38231, #40790, #44856, .T. ) ;
#44257=EDGE_LOOP ( 'NONE', ( #8358, #8291, #47343, #54202, #26883 ) ) ;
#44258=EDGE_CURVE ( 'NONE', #37328, #37239, #40028, .T. ) ;
#44259=ORIENTED_EDGE ( 'NONE', *, *, #36917, .F. ) ;
#44261=VERTEX_POINT ( 'NONE', #23556 ) ;
#44262=ORIENTED_EDGE ( 'NONE', *, *, #10021, .F. ) ;
#44263=CARTESIAN_POINT ( 'NONE',  ( -14.85649334630307017, 0.000000000000000000, 2.688804096480295502 ) ) ;
#44264=CARTESIAN_POINT ( 'NONE',  ( -19.71722652620312743, 0.000000000000000000, 4.497637095973019861 ) ) ;
#44265=VECTOR ( 'NONE', #39890, 999.9999999999998863 ) ;
#44266=ORIENTED_EDGE ( 'NONE', *, *, #22498, .T. ) ;
#44267=VERTEX_POINT ( 'NONE', #40318 ) ;
#44268=EDGE_CURVE ( 'NONE', #25423, #33543, #9946, .T. ) ;
#44269=EDGE_CURVE ( 'NONE', #41178, #50871, #39768, .T. ) ;
#44271=ORIENTED_EDGE ( 'NONE', *, *, #9586, .F. ) ;
#44272=EDGE_CURVE ( 'NONE', #22478, #27583, #44560, .T. ) ;
#44273=CARTESIAN_POINT ( 'NONE',  ( -29.86352658060627618, 0.000000000000000000, 8.481329010720569883 ) ) ;
#44274=CARTESIAN_POINT ( 'NONE',  ( -14.42347103802009300, 0.000000000000000000, 6.754826744083713308 ) ) ;
#44275=VERTEX_POINT ( 'NONE', #30943 ) ;
#44276=CARTESIAN_POINT ( 'NONE',  ( -10.90349575374891700, 0.000000000000000000, 6.412887935854022281 ) ) ;
#44277=EDGE_LOOP ( 'NONE', ( #55029, #46135, #44991, #39926 ) ) ;
#44278=EDGE_CURVE ( 'NONE', #52907, #33376, #44014, .T. ) ;
#44279=PLANE ( 'NONE',  #49995 ) ;
#44280=CARTESIAN_POINT ( 'NONE',  ( -23.33693525117809386, 0.000000000000000000, 5.746789908705562944 ) ) ;
#44281=ADVANCED_FACE ( 'NONE', ( #31235 ), #22460, .F. ) ;
#44282=CARTESIAN_POINT ( 'NONE',  ( -13.19638330378551316, 0.000000000000000000, 2.501717400473541186 ) ) ;
#44283=LINE ( 'NONE', #14194, #2426 ) ;
#44284=ORIENTED_EDGE ( 'NONE', *, *, #22365, .F. ) ;
#44285=LINE ( 'NONE', #5113, #53930 ) ;
#44286=DIRECTION ( 'NONE',  ( -0.5364919789714478471, 0.6444004775717705469, -0.5449076811759709926 ) ) ;
#44287=DIRECTION ( 'NONE',  ( 0.6427681459581294776, -0.7660444431189769032, 0.005002170337467562802 ) ) ;
#44288=EDGE_LOOP ( 'NONE', ( #4802, #26850, #20398, #48958 ) ) ;
#44289=CARTESIAN_POINT ( 'NONE',  ( -16.33317936670417225, 0.000000000000000000, 13.31440848639340224 ) ) ;
#44290=EDGE_LOOP ( 'NONE', ( #29022, #1822, #17165, #36715 ) ) ;
#44291=CARTESIAN_POINT ( 'NONE',  ( -16.27052241136330579, 0.000000000000000000, 5.263124283980618046 ) ) ;
#44292=LINE ( 'NONE', #834, #6968 ) ;
#44293=LINE ( 'NONE', #13615, #8582 ) ;
#44294=FACE_OUTER_BOUND ( 'NONE', #7246, .T. ) ;
#44295=CARTESIAN_POINT ( 'NONE',  ( -14.00280974873554030, 0.000000000000000000, 12.40921378708904044 ) ) ;
#44297=FACE_OUTER_BOUND ( 'NONE', #11827, .T. ) ;
#44298=DIRECTION ( 'NONE',  ( 0.007781995580012663651, 0.000000000000000000, -0.9999697198139515519 ) ) ;
#44299=CARTESIAN_POINT ( 'NONE',  ( -10.70481946417540797, 0.000000000000000000, 6.583760094264999196 ) ) ;
#44300=EDGE_LOOP ( 'NONE', ( #49957, #21434, #38610, #14933 ) ) ;
#44301=LINE ( 'NONE', #26689, #16656 ) ;
#44303=DIRECTION ( 'NONE',  ( 0.5364919789714477361, 0.6444004775717706579, 0.5449076811759711036 ) ) ;
#44304=CARTESIAN_POINT ( 'NONE',  ( -13.10210881006539552, 0.4483081953215033444, 1.756932364226573728 ) ) ;
#44305=FACE_OUTER_BOUND ( 'NONE', #35097, .T. ) ;
#44306=PLANE ( 'NONE',  #47811 ) ;
#44307=LINE ( 'NONE', #8849, #51934 ) ;
#44308=VERTEX_POINT ( 'NONE', #18166 ) ;
#44309=ORIENTED_EDGE ( 'NONE', *, *, #35419, .F. ) ;
#44310=CARTESIAN_POINT ( 'NONE',  ( -12.65748011252205352, 1.581621852479007106, 1.548064839234879031 ) ) ;
#44311=CARTESIAN_POINT ( 'NONE',  ( -20.17480658638558921, -5.213152330870665097, 4.551574281445605052 ) ) ;
#44312=EDGE_CURVE ( 'NONE', #23289, #39974, #52798, .T. ) ;
#44313=EDGE_LOOP ( 'NONE', ( #35600, #46953, #21668, #37218 ) ) ;
#44314=CARTESIAN_POINT ( 'NONE',  ( -30.79567442779373110, 0.000000000000000000, 8.843406890442315316 ) ) ;
#44315=ORIENTED_EDGE ( 'NONE', *, *, #15614, .F. ) ;
#44316=CARTESIAN_POINT ( 'NONE',  ( -7.167951541316091024, 2.571841242220739510, 8.539956480301096775 ) ) ;
#44317=EDGE_CURVE ( 'NONE', #18631, #49377, #9678, .T. ) ;
#44318=EDGE_CURVE ( 'NONE', #24756, #53854, #22713, .T. ) ;
#44319=ORIENTED_EDGE ( 'NONE', *, *, #52923, .F. ) ;
#44320=EDGE_LOOP ( 'NONE', ( #457, #723, #40155, #46369 ) ) ;
#44321=EDGE_LOOP ( 'NONE', ( #26043, #51466, #2889, #5433 ) ) ;
#44322=LINE ( 'NONE', #48867, #23863 ) ;
#44324=LINE ( 'NONE', #52823, #52971 ) ;
#44325=CARTESIAN_POINT ( 'NONE',  ( -13.53673582514181106, 0.000000000000000000, 12.22817484722816772 ) ) ;
#44327=ORIENTED_EDGE ( 'NONE', *, *, #20124, .F. ) ;
#44329=ORIENTED_EDGE ( 'NONE', *, *, #13028, .T. ) ;
#44330=CARTESIAN_POINT ( 'NONE',  ( -16.94090135917774376, 0.000000000000000000, 5.996571379612134045 ) ) ;
#44331=EDGE_LOOP ( 'NONE', ( #23611, #11773, #55234, #11709 ) ) ;
#44332=PLANE ( 'NONE',  #55965 ) ;
#44333=CARTESIAN_POINT ( 'NONE',  ( -9.293664452620451044, 0.000000000000000000, 4.378749610022443228 ) ) ;
#44335=ORIENTED_EDGE ( 'NONE', *, *, #45500, .T. ) ;
#44336=DIRECTION ( 'NONE',  ( 0.5364919789714477361, 0.6444004775717706579, 0.5449076811759711036 ) ) ;
#44337=ORIENTED_EDGE ( 'NONE', *, *, #45705, .F. ) ;
#44339=FACE_OUTER_BOUND ( 'NONE', #9047, .T. ) ;
#44340=ORIENTED_EDGE ( 'NONE', *, *, #22336, .F. ) ;
#44341=EDGE_CURVE ( 'NONE', #34349, #661, #20404, .T. ) ;
#44342=DIRECTION ( 'NONE',  ( 0.9999697198139515519, 0.000000000000000000, 0.007781995580013368816 ) ) ;
#44343=CARTESIAN_POINT ( 'NONE',  ( -25.20123094555300369, 0.000000000000000000, 6.470945668149052032 ) ) ;
#44344=LINE ( 'NONE', #49150, #42785 ) ;
#44345=ADVANCED_FACE ( 'NONE', ( #7336 ), #6509, .F. ) ;
#44346=ORIENTED_EDGE ( 'NONE', *, *, #19994, .T. ) ;
#44347=DIRECTION ( 'NONE',  ( 0.7660212471507180654, -0.6427876096865404731, 0.005961354470445141482 ) ) ;
#44348=EDGE_CURVE ( 'NONE', #35486, #26517, #28937, .T. ) ;
#44349=LINE ( 'NONE', #9424, #4975 ) ;
#44350=PLANE ( 'NONE',  #22295 ) ;
#44351=DIRECTION ( 'NONE',  ( 0.005002170337468016433, -0.7660444431189770143, -0.6427681459581293666 ) ) ;
#44352=CARTESIAN_POINT ( 'NONE',  ( -28.92982233430281980, 0.000000000000000000, 7.919257187036034651 ) ) ;
#44354=EDGE_LOOP ( 'NONE', ( #10168, #7966, #18975, #49704 ) ) ;
#44355=CARTESIAN_POINT ( 'NONE',  ( 2.072287782118878319, 0.000000000000000000, -2.950529333540147015 ) ) ;
#44356=DIRECTION ( 'NONE',  ( -0.005961354470445682716, -0.6427876096865404731, 0.7660212471507180654 ) ) ;
#44357=DIRECTION ( 'NONE',  ( 0.000000000000000000, 1.000000000000000000, 0.000000000000000000 ) ) ;
#44359=LINE ( 'NONE', #49742, #26593 ) ;
#44360=FACE_OUTER_BOUND ( 'NONE', #47937, .T. ) ;
#44361=ORIENTED_EDGE ( 'NONE', *, *, #32372, .T. ) ;
#44362=DIRECTION ( 'NONE',  ( -0.7660212471507179544, -0.6427876096865405842, -0.005961354470445141482 ) ) ;
#44363=CARTESIAN_POINT ( 'NONE',  ( 2.072287782118878319, 0.000000000000000000, -2.950529333540147015 ) ) ;
#44364=CARTESIAN_POINT ( 'NONE',  ( -18.67775241435682432, 0.000000000000000000, 4.136394454059623804 ) ) ;
#44365=LINE ( 'NONE', #18235, #50065 ) ;
#44366=ORIENTED_EDGE ( 'NONE', *, *, #24806, .T. ) ;
#44367=ORIENTED_EDGE ( 'NONE', *, *, #26869, .F. ) ;
#44368=DIRECTION ( 'NONE',  ( 0.5449076811759707706, 0.6444004775717708799, -0.5364919789714476250 ) ) ;
#44369=FACE_OUTER_BOUND ( 'NONE', #16510, .T. ) ;
#44370=CARTESIAN_POINT ( 'NONE',  ( -23.33771345073609638, -0.1191753592594197858, 5.846786880686956955 ) ) ;
#44371=ADVANCED_FACE ( 'NONE', ( #41693 ), #15046, .F. ) ;
#44372=LINE ( 'NONE', #2021, #16639 ) ;
#44374=LINE ( 'NONE', #31870, #174 ) ;
#44375=FACE_OUTER_BOUND ( 'NONE', #44906, .T. ) ;
#44376=EDGE_LOOP ( 'NONE', ( #30091, #42602, #11216, #8022 ) ) ;
#44377=LINE ( 'NONE', #52893, #42865 ) ;
#44378=EDGE_CURVE ( 'NONE', #2867, #11380, #16153, .T. ) ;
#44379=EDGE_CURVE ( 'NONE', #30096, #26810, #15314, .T. ) ;
#44380=FACE_OUTER_BOUND ( 'NONE', #30443, .T. ) ;
#44382=DIRECTION ( 'NONE',  ( -0.005961354470445682716, -0.6427876096865404731, 0.7660212471507180654 ) ) ;
#44383=DIRECTION ( 'NONE',  ( 0.000000000000000000, -0.000000000000000000, -1.000000000000000000 ) ) ;
#44384=CARTESIAN_POINT ( 'NONE',  ( -12.13851405436063047, 0.000000000000000000, 11.68505802764555135 ) ) ;
#44385=VERTEX_POINT ( 'NONE', #36916 ) ;
#44386=CARTESIAN_POINT ( 'NONE',  ( -16.99924723426068951, 0.000000000000000000, 13.49389102713827171 ) ) ;
#44387=VERTEX_POINT ( 'NONE', #32901 ) ;
#44388=EDGE_CURVE ( 'NONE', #27005, #11058, #54216, .T. ) ;
#44389=ORIENTED_EDGE ( 'NONE', *, *, #1165, .T. ) ;
#44390=EDGE_LOOP ( 'NONE', ( #34827, #18579, #23861, #29515 ) ) ;
#44391=ORIENTED_EDGE ( 'NONE', *, *, #12001, .F. ) ;
#44392=CARTESIAN_POINT ( 'NONE',  ( -16.56028341318607389, 0.000000000000000000, 3.214202891609632129 ) ) ;
#44393=EDGE_LOOP ( 'NONE', ( #4192, #52768, #23440, #15727 ) ) ;
#44395=CARTESIAN_POINT ( 'NONE',  ( -9.958295293424326289, 0.000000000000000000, 4.373577299138431407 ) ) ;
#44396=VERTEX_POINT ( 'NONE', #20103 ) ;
#44397=CARTESIAN_POINT ( 'NONE',  ( -10.89199953972778623, 0.000000000000000000, 4.935649122822963974 ) ) ;
#44398=ORIENTED_EDGE ( 'NONE', *, *, #47969, .F. ) ;
#44399=CARTESIAN_POINT ( 'NONE',  ( -22.40478740399063895, 0.000000000000000000, 5.384712028983816623 ) ) ;
#44401=CARTESIAN_POINT ( 'NONE',  ( -15.36268464660739141, 0.000000000000000000, 8.024839789615963781 ) ) ;
#44402=CARTESIAN_POINT ( 'NONE',  ( -26.13493519185646008, 0.000000000000000000, 7.033017491833586377 ) ) ;
#44403=DIRECTION ( 'NONE',  ( 0.005961354470445682716, -0.6427876096865404731, -0.7660212471507180654 ) ) ;
#44405=LINE ( 'NONE', #31063, #31435 ) ;
#44406=LINE ( 'NONE', #40147, #6577 ) ;
#44407=ORIENTED_EDGE ( 'NONE', *, *, #30229, .T. ) ;
#44408=ORIENTED_EDGE ( 'NONE', *, *, #49905, .F. ) ;
#44410=ADVANCED_FACE ( 'NONE', ( #53927 ), #11036, .F. ) ;
#44411=CARTESIAN_POINT ( 'NONE',  ( -18.67619601524082285, 0.000000000000000000, 3.936400510096834893 ) ) ;
#44412=DIRECTION ( 'NONE',  ( 0.005961354470445682716, -0.6427876096865404731, -0.7660212471507180654 ) ) ;
#44413=DIRECTION ( 'NONE',  ( -0.5449076811759708816, 0.6444004775717707689, 0.5364919789714475140 ) ) ;
#44414=VERTEX_POINT ( 'NONE', #24383 ) ;
#44415=CARTESIAN_POINT ( 'NONE',  ( -10.74029228357944987, 0.000000000000000000, 11.14194120806293320 ) ) ;
#44417=EDGE_LOOP ( 'NONE', ( #22443, #3730, #15137, #49069 ) ) ;
#44418=CARTESIAN_POINT ( 'NONE',  ( -25.20278734466900517, 0.000000000000000000, 6.670939612111840944 ) ) ;
#44419=LINE ( 'NONE', #35630, #35826 ) ;
#44420=ORIENTED_EDGE ( 'NONE', *, *, #37790, .T. ) ;
#44421=EDGE_CURVE ( 'NONE', #16077, #15628, #28355, .T. ) ;
#44423=CARTESIAN_POINT ( 'NONE',  ( -15.13495153988577968, 0.000000000000000000, 12.76973526769478084 ) ) ;
#44424=CARTESIAN_POINT ( 'NONE',  ( -10.47421230394850866, 0.000000000000000000, 10.95934586908605723 ) ) ;
#44425=ADVANCED_FACE ( 'NONE', ( #37167 ), #41150, .F. ) ;
#44426=ADVANCED_FACE ( 'NONE', ( #41446 ), #19848, .F. ) ;
#44427=FACE_OUTER_BOUND ( 'NONE', #53146, .T. ) ;
#44428=CARTESIAN_POINT ( 'NONE',  ( -17.87436686075448122, 0.000000000000000000, 6.527965018628854033 ) ) ;
#44429=ORIENTED_EDGE ( 'NONE', *, *, #25247, .F. ) ;
#44430=ORIENTED_EDGE ( 'NONE', *, *, #15089, .T. ) ;
#44431=PLANE ( 'NONE',  #55692 ) ;
#44432=DIRECTION ( 'NONE',  ( -0.6427681459581293666, -0.7660444431189770143, -0.005002170337467561935 ) ) ;
#44433=LINE ( 'NONE', #10369, #18814 ) ;
#44434=ADVANCED_FACE ( 'NONE', ( #49599 ), #31977, .F. ) ;
#44435=FACE_OUTER_BOUND ( 'NONE', #30784, .T. ) ;
#44437=CARTESIAN_POINT ( 'NONE',  ( -19.58350694149355675, 0.9340140483890049250, 6.021096448066252549 ) ) ;
#44438=ORIENTED_EDGE ( 'NONE', *, *, #32406, .F. ) ;
#44440=DIRECTION ( 'NONE',  ( 0.5364919789714477361, 0.6444004775717706579, 0.5449076811759711036 ) ) ;
#44441=EDGE_CURVE ( 'NONE', #23769, #26810, #27164, .T. ) ;
#44442=VECTOR ( 'NONE', #1879, 999.9999999999998863 ) ;
#44443=CARTESIAN_POINT ( 'NONE',  ( -16.45458968868368288, 0.000000000000000000, 3.215025424613001892 ) ) ;
#44444=FACE_OUTER_BOUND ( 'NONE', #34657, .T. ) ;
#44446=LINE ( 'NONE', #19154, #50128 ) ;
#44447=ORIENTED_EDGE ( 'NONE', *, *, #6963, .F. ) ;
#44448=DIRECTION ( 'NONE',  ( 0.7660212471507180654, -0.6427876096865404731, 0.005961354470445141482 ) ) ;
#44449=DIRECTION ( 'NONE',  ( 0.000000000000000000, -0.000000000000000000, -1.000000000000000000 ) ) ;
#44450=EDGE_CURVE ( 'NONE', #27927, #36106, #28010, .T. ) ;
#44451=ORIENTED_EDGE ( 'NONE', *, *, #6453, .F. ) ;
#44452=LINE ( 'NONE', #5556, #35373 ) ;
#44453=ORIENTED_EDGE ( 'NONE', *, *, #16540, .T. ) ;
#44454=EDGE_CURVE ( 'NONE', #6528, #29959, #14658, .T. ) ;
#44455=ORIENTED_EDGE ( 'NONE', *, *, #23438, .T. ) ;
#44456=VERTEX_POINT ( 'NONE', #6169 ) ;
#44460=FACE_OUTER_BOUND ( 'NONE', #13859, .T. ) ;
#44461=LINE ( 'NONE', #1006, #53941 ) ;
#44462=ORIENTED_EDGE ( 'NONE', *, *, #31513, .T. ) ;
#44463=EDGE_LOOP ( 'NONE', ( #50655, #6748, #14305 ) ) ;
#44464=LINE ( 'NONE', #48156, #34933 ) ;
#44465=ORIENTED_EDGE ( 'NONE', *, *, #29411, .T. ) ;
#44466=ORIENTED_EDGE ( 'NONE', *, *, #52216, .F. ) ;
#44467=PLANE ( 'NONE',  #20324 ) ;
#44468=CARTESIAN_POINT ( 'NONE',  ( -11.20636620717317378, 0.000000000000000000, 11.32298014792380414 ) ) ;
#44469=DIRECTION ( 'NONE',  ( 0.007781995580012663651, -3.146120232559066537E-19, -0.9999697198139514409 ) ) ;
#44470=CARTESIAN_POINT ( 'NONE',  ( 1.710209902397132220, -1.000000000000000000, -3.882677180727601041 ) ) ;
#44471=ORIENTED_EDGE ( 'NONE', *, *, #55712, .F. ) ;
#44472=LINE ( 'NONE', #35691, #24640 ) ;
#44473=EDGE_LOOP ( 'NONE', ( #41791, #20066, #35129, #55387 ) ) ;
#44474=ADVANCED_FACE ( 'NONE', ( #9576 ), #23727, .F. ) ;
#44475=LINE ( 'NONE', #22905, #28427 ) ;
#44476=VECTOR ( 'NONE', #39258, 999.9999999999998863 ) ;
#44477=LINE ( 'NONE', #48169, #55987 ) ;
#44478=LINE ( 'NONE', #26603, #18645 ) ;
#44479=PLANE ( 'NONE',  #2199 ) ;
#44480=CARTESIAN_POINT ( 'NONE',  ( -9.676870672209137325, -1.212633296248882164, 2.080894224339388199 ) ) ;
#44481=DIRECTION ( 'NONE',  ( -0.9999697198139514409, -0.000000000000000000, -0.007781995580013368816 ) ) ;
#44482=ORIENTED_EDGE ( 'NONE', *, *, #4134, .F. ) ;
#44483=CARTESIAN_POINT ( 'NONE',  ( -14.62633903548816328, 0.000000000000000000, 7.122580048225473526 ) ) ;
#44484=ORIENTED_EDGE ( 'NONE', *, *, #28198, .F. ) ;
#44485=DIRECTION ( 'NONE',  ( -0.9999697198139514409, -0.000000000000000000, -0.007781995580013368816 ) ) ;
#44486=LINE ( 'NONE', #27179, #7875 ) ;
#44487=DIRECTION ( 'NONE',  ( 0.007781995580012663651, -3.146120232559066537E-19, -0.9999697198139514409 ) ) ;
#44490=EDGE_CURVE ( 'NONE', #11209, #8418, #31445, .T. ) ;
#44491=DIRECTION ( 'NONE',  ( 0.000000000000000000, -1.000000000000000000, 0.000000000000000000 ) ) ;
#44493=VERTEX_POINT ( 'NONE', #36512 ) ;
#44494=FACE_OUTER_BOUND ( 'NONE', #25779, .T. ) ;
#44495=CARTESIAN_POINT ( 'NONE',  ( -10.27421835998572064, 0.000000000000000000, 10.96090226820206048 ) ) ;
#44496=LINE ( 'NONE', #28295, #31834 ) ;
#44497=VECTOR ( 'NONE', #41637, 999.9999999999998863 ) ;
#44498=DIRECTION ( 'NONE',  ( 0.007781995580012662783, 0.000000000000000000, -0.9999697198139514409 ) ) ;
#44499=EDGE_CURVE ( 'NONE', #5827, #27227, #26900, .T. ) ;
#44500=DIRECTION ( 'NONE',  ( -0.6427681459581293666, -0.7660444431189770143, -0.005002170337467561935 ) ) ;
#44502=CARTESIAN_POINT ( 'NONE',  ( -9.299412559631017317, 0.000000000000000000, 5.117369016537971937 ) ) ;
#44503=ADVANCED_FACE ( 'NONE', ( #5318 ), #45317, .F. ) ;
#44504=PLANE ( 'NONE',  #48639 ) ;
#44505=PLANE ( 'NONE',  #17467 ) ;
#44506=EDGE_CURVE ( 'NONE', #37427, #36569, #31714, .T. ) ;
#44507=VERTEX_POINT ( 'NONE', #18347 ) ;
#44508=VECTOR ( 'NONE', #21591, 1000.000000000000227 ) ;
#44509=VECTOR ( 'NONE', #13573, 1000.000000000000000 ) ;
#44510=EDGE_CURVE ( 'NONE', #14416, #10323, #53831, .T. ) ;
#44511=VERTEX_POINT ( 'NONE', #5574 ) ;
#44512=ORIENTED_EDGE ( 'NONE', *, *, #7425, .T. ) ;
#44513=VERTEX_POINT ( 'NONE', #14401 ) ;
#44514=VERTEX_POINT ( 'NONE', #41048 ) ;
#44515=DIRECTION ( 'NONE',  ( 0.6427681459581294776, -0.7660444431189769032, 0.005002170337467562802 ) ) ;
#44516=CARTESIAN_POINT ( 'NONE',  ( -19.32961685222932147, 0.000000000000000000, 14.39908572644263351 ) ) ;
#44517=ORIENTED_EDGE ( 'NONE', *, *, #33852, .F. ) ;
#44518=ORIENTED_EDGE ( 'NONE', *, *, #10609, .F. ) ;
#44519=VERTEX_POINT ( 'NONE', #35688 ) ;
#44520=DIRECTION ( 'NONE',  ( -0.6427681459581293666, -0.7660444431189770143, -0.005002170337467561935 ) ) ;
#44521=EDGE_LOOP ( 'NONE', ( #23629, #20583, #34994, #32307 ) ) ;
#44522=CARTESIAN_POINT ( 'NONE',  ( -17.86287064673334868, 0.000000000000000000, 5.050726205597795726 ) ) ;
#44523=LINE ( 'NONE', #39989, #24076 ) ;
#44524=VERTEX_POINT ( 'NONE', #10412 ) ;
#44525=LINE ( 'NONE', #13597, #41865 ) ;
#44526=EDGE_CURVE ( 'NONE', #18734, #52995, #2140, .T. ) ;
#44527=ORIENTED_EDGE ( 'NONE', *, *, #18004, .T. ) ;
#44528=VECTOR ( 'NONE', #35432, 1000.000000000000227 ) ;
#44529=VECTOR ( 'NONE', #47400, 1000.000000000000114 ) ;
#44530=DIRECTION ( 'NONE',  ( -0.6427681459581293666, -0.7660444431189770143, -0.005002170337467561935 ) ) ;
#44531=EDGE_CURVE ( 'NONE', #13033, #33148, #40222, .T. ) ;
#44532=DIRECTION ( 'NONE',  ( 0.005961354470445682716, -0.6427876096865404731, -0.7660212471507180654 ) ) ;
#44533=CARTESIAN_POINT ( 'NONE',  ( -14.18665187206895517, 4.981562823951511731, 10.56749175989368617 ) ) ;
#44534=DIRECTION ( 'NONE',  ( 0.5449076811759707706, 0.6444004775717708799, -0.5364919789714476250 ) ) ;
#44535=ORIENTED_EDGE ( 'NONE', *, *, #25158, .F. ) ;
#44536=DIRECTION ( 'NONE',  ( 0.9999697198139515519, 0.000000000000000000, 0.007781995580013368816 ) ) ;
#44537=CARTESIAN_POINT ( 'NONE',  ( -11.20636620717317378, 0.000000000000000000, 11.32298014792380414 ) ) ;
#44538=FACE_OUTER_BOUND ( 'NONE', #26122, .T. ) ;
#44540=VERTEX_POINT ( 'NONE', #19183 ) ;
#44541=DIRECTION ( 'NONE',  ( -0.5364919789714478471, 0.6444004775717705469, -0.5449076811759709926 ) ) ;
#44542=ORIENTED_EDGE ( 'NONE', *, *, #23718, .F. ) ;
#44543=ADVANCED_FACE ( 'NONE', ( #10117 ), #23197, .F. ) ;
#44544=EDGE_CURVE ( 'NONE', #37239, #48873, #2970, .T. ) ;
#44546=LINE ( 'NONE', #14208, #53699 ) ;
#44547=DIRECTION ( 'NONE',  ( -0.005002170337468016433, -0.7660444431189770143, 0.6427681459581293666 ) ) ;
#44548=LINE ( 'NONE', #18436, #24955 ) ;
#44550=DIRECTION ( 'NONE',  ( -0.5449076811759708816, 0.6444004775717707689, 0.5364919789714475140 ) ) ;
#44551=CARTESIAN_POINT ( 'NONE',  ( -17.87017515285991820, 0.000000000000000000, 5.989339556076115123 ) ) ;
#44552=CARTESIAN_POINT ( 'NONE',  ( -15.96710241509184058, -0.1191753592594218814, 13.13259134697452879 ) ) ;
#44553=AXIS2_PLACEMENT_3D ( 'NONE', #20442, #45712, #6280 ) ;
#44555=DIRECTION ( 'NONE',  ( 0.6427681459581294776, -0.7660444431189769032, 0.005002170337467562802 ) ) ;
#44556=ORIENTED_EDGE ( 'NONE', *, *, #28292, .F. ) ;
#44557=FACE_OUTER_BOUND ( 'NONE', #6208, .T. ) ;
#44558=CARTESIAN_POINT ( 'NONE',  ( -17.74404816805336793, 0.000000000000000000, 3.574322630375089460 ) ) ;
#44559=CARTESIAN_POINT ( 'NONE',  ( -9.342070512798265725, 0.000000000000000000, 10.59882438848031505 ) ) ;
#44560=LINE ( 'NONE', #26693, #43227 ) ;
#44561=DIRECTION ( 'NONE',  ( 0.9999697198139515519, 0.000000000000000000, 0.007781995580013368816 ) ) ;
#44562=EDGE_CURVE ( 'NONE', #52307, #9050, #41347, .T. ) ;
#44563=LINE ( 'NONE', #48854, #55951 ) ;
#44564=LINE ( 'NONE', #48567, #54646 ) ;
#44565=ORIENTED_EDGE ( 'NONE', *, *, #14381, .F. ) ;
#44566=ADVANCED_FACE ( 'NONE', ( #46143 ), #6996, .F. ) ;
#44567=ORIENTED_EDGE ( 'NONE', *, *, #18520, .T. ) ;
#44569=CARTESIAN_POINT ( 'NONE',  ( -18.57070714969772496, 4.657758921906509642, 11.73899034496769112 ) ) ;
#44570=DIRECTION ( 'NONE',  ( -0.9999697198139514409, -0.000000000000000000, -0.007781995580013368816 ) ) ;
#44571=VECTOR ( 'NONE', #28586, 999.9999999999998863 ) ;
#44572=EDGE_CURVE ( 'NONE', #55458, #27295, #3549, .T. ) ;
#44573=VECTOR ( 'NONE', #30741, 999.9999999999998863 ) ;
#44574=ORIENTED_EDGE ( 'NONE', *, *, #34149, .F. ) ;
#44575=DIRECTION ( 'NONE',  ( 0.005002170337468016433, -0.7660444431189770143, -0.6427681459581293666 ) ) ;
#44576=ORIENTED_EDGE ( 'NONE', *, *, #37329, .F. ) ;
#44577=CARTESIAN_POINT ( 'NONE',  ( -19.39757902869610717, 2.391131607591508335, 4.140320553562598427 ) ) ;
#44578=EDGE_CURVE ( 'NONE', #34394, #17707, #54650, .T. ) ;
#44579=ORIENTED_EDGE ( 'NONE', *, *, #31753, .T. ) ;
#44580=ORIENTED_EDGE ( 'NONE', *, *, #12205, .F. ) ;
#44581=VECTOR ( 'NONE', #21075, 1000.000000000000227 ) ;
#44582=EDGE_LOOP ( 'NONE', ( #18009, #1673, #51321, #35244 ) ) ;
#44583=CARTESIAN_POINT ( 'NONE',  ( -20.54204810873173415, 0.000000000000000000, 4.860550213503115558 ) ) ;
#44584=CARTESIAN_POINT ( 'NONE',  ( -19.62507351517958298, -0.1191753592594172323, 5.506347433322916096 ) ) ;
#44585=PLANE ( 'NONE',  #38455 ) ;
#44586=PLANE ( 'NONE',  #40268 ) ;
#44587=VERTEX_POINT ( 'NONE', #55496 ) ;
#44589=VECTOR ( 'NONE', #23936, 1000.000000000000227 ) ;
#44590=LINE ( 'NONE', #52560, #52684 ) ;
#44591=ORIENTED_EDGE ( 'NONE', *, *, #42920, .T. ) ;
#44592=CARTESIAN_POINT ( 'NONE',  ( -18.67697421479882181, -0.1191753592594197858, 4.036397482078229793 ) ) ;
#44593=EDGE_LOOP ( 'NONE', ( #19602, #13559, #46803, #26359 ) ) ;
#44594=CARTESIAN_POINT ( 'NONE',  ( -18.67775241435682432, 0.000000000000000000, 4.136394454059623804 ) ) ;
#44595=DIRECTION ( 'NONE',  ( 0.000000000000000000, -1.000000000000000000, 0.000000000000000000 ) ) ;
#44596=VERTEX_POINT ( 'NONE', #24299 ) ;
#44597=CARTESIAN_POINT ( 'NONE',  ( -24.26986129792355129, -0.1191753592594197858, 6.208864760408702388 ) ) ;
#44598=ORIENTED_EDGE ( 'NONE', *, *, #24580, .T. ) ;
#44599=DIRECTION ( 'NONE',  ( 0.005002170337468016433, -0.7660444431189770143, -0.6427681459581293666 ) ) ;
#44600=ORIENTED_EDGE ( 'NONE', *, *, #11679, .F. ) ;
#44601=CARTESIAN_POINT ( 'NONE',  ( -15.40103151951671734, 0.000000000000000000, 12.95233060667165681 ) ) ;
#44602=CARTESIAN_POINT ( 'NONE',  ( -27.06708303904391144, 0.000000000000000000, 7.395095371555332697 ) ) ;
#44603=LINE ( 'NONE', #1991, #3836 ) ;
#44604=ORIENTED_EDGE ( 'NONE', *, *, #43021, .T. ) ;
#44605=EDGE_CURVE ( 'NONE', #34911, #17803, #7522, .T. ) ;
#44607=AXIS2_PLACEMENT_3D ( 'NONE', #14554, #9759, #41458 ) ;
#44608=VECTOR ( 'NONE', #20740, 999.9999999999998863 ) ;
#44609=DIRECTION ( 'NONE',  ( -0.005002170337468016433, -0.7660444431189770143, 0.6427681459581293666 ) ) ;
#44610=CARTESIAN_POINT ( 'NONE',  ( 2.072287782118878319, 0.000000000000000000, -2.950529333540147015 ) ) ;
#44611=DIRECTION ( 'NONE',  ( -0.7660212471507179544, -0.6427876096865405842, -0.005961354470445141482 ) ) ;
#44612=EDGE_CURVE ( 'NONE', #25423, #5277, #16317, .T. ) ;
#44613=FACE_OUTER_BOUND ( 'NONE', #32166, .T. ) ;
#44614=CARTESIAN_POINT ( 'NONE',  ( -17.78664430235221516, -0.1191753592594194527, 8.105979003199307087 ) ) ;
#44616=VECTOR ( 'NONE', #6030, 999.9999999999998863 ) ;
#44617=VERTEX_POINT ( 'NONE', #33636 ) ;
#44618=DIRECTION ( 'NONE',  ( 0.000000000000000000, -0.000000000000000000, -1.000000000000000000 ) ) ;
#44619=CARTESIAN_POINT ( 'NONE',  ( -8.364753971622430839, 6.050419986852017651, 0.03078093515494761956 ) ) ;
#44620=DIRECTION ( 'NONE',  ( -0.005002170337468016433, -0.7660444431189770143, 0.6427681459581293666 ) ) ;
#44621=ORIENTED_EDGE ( 'NONE', *, *, #8948, .F. ) ;
#44623=DIRECTION ( 'NONE',  ( -0.7660212471507179544, -0.6427876096865405842, -0.005961354470445141482 ) ) ;
#44624=EDGE_LOOP ( 'NONE', ( #3846, #32842, #48757, #7384 ) ) ;
#44625=CARTESIAN_POINT ( 'NONE',  ( -16.22839869333036589, 0.2864062442990018553, 2.976455044025407837 ) ) ;
#44626=PLANE ( 'NONE',  #40370 ) ;
#44627=AXIS2_PLACEMENT_3D ( 'NONE', #4204, #50491, #34298 ) ;
#44628=CARTESIAN_POINT ( 'NONE',  ( -24.27063949748155380, 0.000000000000000000, 6.308861732390097288 ) ) ;
#44629=ADVANCED_FACE ( 'NONE', ( #41608 ), #50950, .F. ) ;
#44630=CARTESIAN_POINT ( 'NONE',  ( -29.86197018149027116, 0.000000000000000000, 8.281335066757780083 ) ) ;
#44631=ORIENTED_EDGE ( 'NONE', *, *, #33536, .T. ) ;
#44632=ORIENTED_EDGE ( 'NONE', *, *, #19860, .F. ) ;
#44633=DIRECTION ( 'NONE',  ( 0.000000000000000000, -1.000000000000000000, 0.000000000000000000 ) ) ;
#44634=FACE_OUTER_BOUND ( 'NONE', #18227, .T. ) ;
#44635=DIRECTION ( 'NONE',  ( 0.7660212471507180654, -0.6427876096865404731, 0.005961354470445141482 ) ) ;
#44637=FACE_OUTER_BOUND ( 'NONE', #12742, .T. ) ;
#44638=ORIENTED_EDGE ( 'NONE', *, *, #49744, .T. ) ;
#44639=DIRECTION ( 'NONE',  ( 0.007781995580012663651, -3.146120232559066537E-19, -0.9999697198139514409 ) ) ;
#44640=VECTOR ( 'NONE', #37588, 999.9999999999998863 ) ;
#44641=ORIENTED_EDGE ( 'NONE', *, *, #26619, .T. ) ;
#44642=DIRECTION ( 'NONE',  ( -0.005961354470445682716, -0.6427876096865404731, 0.7660212471507180654 ) ) ;
#44643=EDGE_CURVE ( 'NONE', #49209, #6017, #33388, .T. ) ;
#44644=CARTESIAN_POINT ( 'NONE',  ( -16.38698550481839433, -0.1191753592594179401, 7.378207331987803208 ) ) ;
#44645=EDGE_LOOP ( 'NONE', ( #17639, #7813, #43234, #54181 ) ) ;
#44646=ADVANCED_FACE ( 'NONE', ( #16065 ), #45580, .F. ) ;
#44647=DIRECTION ( 'NONE',  ( -0.005961354470445682716, -0.6427876096865404731, 0.7660212471507180654 ) ) ;
#44648=VECTOR ( 'NONE', #9763, 1000.000000000000114 ) ;
#44649=DIRECTION ( 'NONE',  ( -0.005002170337468016433, -0.7660444431189770143, 0.6427681459581293666 ) ) ;
#44651=CARTESIAN_POINT ( 'NONE',  ( -15.50102849149811135, -0.1191753592594197858, 12.95155240711365430 ) ) ;
#44652=ORIENTED_EDGE ( 'NONE', *, *, #18806, .F. ) ;
#44653=AXIS2_PLACEMENT_3D ( 'NONE', #45346, #1346, #27198 ) ;
#44654=VECTOR ( 'NONE', #8826, 999.9999999999998863 ) ;
#44655=DIRECTION ( 'NONE',  ( 0.007781995580012662783, 0.000000000000000000, -0.9999697198139514409 ) ) ;
#44656=EDGE_CURVE ( 'NONE', #3804, #39510, #54381, .T. ) ;
#44657=ORIENTED_EDGE ( 'NONE', *, *, #47755, .F. ) ;
#44658=ORIENTED_EDGE ( 'NONE', *, *, #52477, .F. ) ;
#44659=VECTOR ( 'NONE', #1893, 1000.000000000000000 ) ;
#44660=VERTEX_POINT ( 'NONE', #52386 ) ;
#44661=LINE ( 'NONE', #23101, #4148 ) ;
#44662=AXIS2_PLACEMENT_3D ( 'NONE', #26084, #38264, #43107 ) ;
#44663=ORIENTED_EDGE ( 'NONE', *, *, #13850, .F. ) ;
#44664=CARTESIAN_POINT ( 'NONE',  ( -10.27421835998572064, 0.000000000000000000, 10.96090226820206048 ) ) ;
#44665=EDGE_LOOP ( 'NONE', ( #19228, #17659, #23576, #22270 ) ) ;
#44666=CARTESIAN_POINT ( 'NONE',  ( -12.33850799832341849, 0.000000000000000000, 11.68350162852954632 ) ) ;
#44667=CARTESIAN_POINT ( 'NONE',  ( -11.40636015113596180, 0.000000000000000000, 11.32142374880780089 ) ) ;
#44668=ORIENTED_EDGE ( 'NONE', *, *, #36245, .F. ) ;
#44669=ORIENTED_EDGE ( 'NONE', *, *, #47250, .T. ) ;
#44670=FACE_OUTER_BOUND ( 'NONE', #53733, .T. ) ;
#44671=VECTOR ( 'NONE', #44762, 999.9999999999998863 ) ;
#44672=ORIENTED_EDGE ( 'NONE', *, *, #9369, .F. ) ;
#44673=CARTESIAN_POINT ( 'NONE',  ( -10.24461301995560447, 0.000000000000000000, 7.156679653253562812 ) ) ;
#44674=DIRECTION ( 'NONE',  ( -0.6427681459581293666, -0.7660444431189770143, -0.005002170337467561935 ) ) ;
#44675=PLANE ( 'NONE',  #33202 ) ;
#44677=PLANE ( 'NONE',  #41393 ) ;
#44678=CARTESIAN_POINT ( 'NONE',  ( -17.74560456716937296, 0.000000000000000000, 3.774316574337878372 ) ) ;
#44679=FACE_OUTER_BOUND ( 'NONE', #55079, .T. ) ;
#44680=ORIENTED_EDGE ( 'NONE', *, *, #25838, .F. ) ;
#44681=AXIS2_PLACEMENT_3D ( 'NONE', #18077, #52999, #23469 ) ;
#44682=EDGE_CURVE ( 'NONE', #44124, #45158, #52091, .T. ) ;
#44684=PLANE ( 'NONE',  #14682 ) ;
#44685=LINE ( 'NONE', #18878, #38445 ) ;
#44686=VECTOR ( 'NONE', #15126, 1000.000000000000227 ) ;
#44687=EDGE_CURVE ( 'NONE', #33244, #28164, #21722, .T. ) ;
#44688=EDGE_CURVE ( 'NONE', #14263, #14113, #8952, .T. ) ;
#44689=CARTESIAN_POINT ( 'NONE',  ( -16.73317108723761137, -2.784623065533160524, 3.292208973453862431 ) ) ;
#44690=FACE_OUTER_BOUND ( 'NONE', #755, .T. ) ;
#44691=EDGE_LOOP ( 'NONE', ( #40774, #23351, #32849, #48011 ) ) ;
#44693=FACE_OUTER_BOUND ( 'NONE', #40488, .T. ) ;
#44694=ORIENTED_EDGE ( 'NONE', *, *, #55520, .T. ) ;
#44695=VECTOR ( 'NONE', #50855, 1000.000000000000114 ) ;
#44696=CARTESIAN_POINT ( 'NONE',  ( -21.47263955680318404, 0.000000000000000000, 5.022634149262071190 ) ) ;
#44697=CARTESIAN_POINT ( 'NONE',  ( -17.41703447003996175, 0.000000000000000000, 7.470194280875182002 ) ) ;
#44698=ORIENTED_EDGE ( 'NONE', *, *, #42270, .T. ) ;
#44699=AXIS2_PLACEMENT_3D ( 'NONE', #39548, #30989, #30168 ) ;
#44700=VECTOR ( 'NONE', #33189, 1000.000000000000227 ) ;
#44701=CARTESIAN_POINT ( 'NONE',  ( -13.27065584551087163, 0.000000000000000000, 12.04557950825129176 ) ) ;
#44702=DIRECTION ( 'NONE',  ( 0.000000000000000000, 1.000000000000000000, 0.000000000000000000 ) ) ;
#44703=DIRECTION ( 'NONE',  ( -0.5364919789714478471, 0.6444004775717705469, -0.5449076811759709926 ) ) ;
#44704=CARTESIAN_POINT ( 'NONE',  ( -25.20278734466900517, 0.000000000000000000, 6.670939612111840944 ) ) ;
#44705=EDGE_CURVE ( 'NONE', #35804, #23263, #35082, .T. ) ;
#44706=CARTESIAN_POINT ( 'NONE',  ( -9.075990533167328067, 0.000000000000000000, 10.41622904950343909 ) ) ;
#44707=ORIENTED_EDGE ( 'NONE', *, *, #28472, .F. ) ;
#44709=AXIS2_PLACEMENT_3D ( 'NONE', #37659, #54987, #48056 ) ;
#44711=CARTESIAN_POINT ( 'NONE',  ( -17.70820938652583365, -5.051250379848164052, 3.598629682913965677 ) ) ;
#44712=CARTESIAN_POINT ( 'NONE',  ( -20.36148084596629459, -1.003701604285656579, 4.758388420423439236 ) ) ;
#44713=CARTESIAN_POINT ( 'NONE',  ( -3.336033939804074588, 4.483638672814038273, -1.922544701254425004 ) ) ;
#44714=DIRECTION ( 'NONE',  ( 0.7660212471507180654, -0.6427876096865404731, 0.005961354470445141482 ) ) ;
#44715=VECTOR ( 'NONE', #38555, 999.9999999999998863 ) ;
#44716=DIRECTION ( 'NONE',  ( 0.9999697198139515519, 0.000000000000000000, 0.007781995580013368816 ) ) ;
#44717=ORIENTED_EDGE ( 'NONE', *, *, #33462, .F. ) ;
#44720=EDGE_CURVE ( 'NONE', #13585, #1119, #25996, .T. ) ;
#44721=LINE ( 'NONE', #1274, #35678 ) ;
#44722=PLANE ( 'NONE',  #54048 ) ;
#44724=VERTEX_POINT ( 'NONE', #30801 ) ;
#44725=EDGE_CURVE ( 'NONE', #13033, #32707, #4668, .T. ) ;
#44726=CARTESIAN_POINT ( 'NONE',  ( -18.19747506107908563, 0.000000000000000000, 14.03856424583689311 ) ) ;
#44727=ORIENTED_EDGE ( 'NONE', *, *, #25998, .T. ) ;
#44728=DIRECTION ( 'NONE',  ( 0.6427681459581294776, -0.7660444431189769032, 0.005002170337467562802 ) ) ;
#44730=LINE ( 'NONE', #36229, #28435 ) ;
#44731=ORIENTED_EDGE ( 'NONE', *, *, #52503, .F. ) ;
#44732=CARTESIAN_POINT ( 'NONE',  ( -10.96535795190825091, 0.1245042932765017124, 0.9372768063285339402 ) ) ;
#44733=ADVANCED_FACE ( 'NONE', ( #16600 ), #3816, .F. ) ;
#44734=VECTOR ( 'NONE', #25042, 999.9999999999998863 ) ;
#44736=VERTEX_POINT ( 'NONE', #34487 ) ;
#44737=EDGE_LOOP ( 'NONE', ( #37036, #31573, #45711, #22616 ) ) ;
#44739=ORIENTED_EDGE ( 'NONE', *, *, #45527, .F. ) ;
#44740=ORIENTED_EDGE ( 'NONE', *, *, #47091, .F. ) ;
#44741=VECTOR ( 'NONE', #55773, 1000.000000000000114 ) ;
#44742=LINE ( 'NONE', #35675, #40185 ) ;
#44743=DIRECTION ( 'NONE',  ( 0.5364919789714477361, 0.6444004775717706579, 0.5449076811759711036 ) ) ;
#44744=VERTEX_POINT ( 'NONE', #26520 ) ;
#44745=EDGE_CURVE ( 'NONE', #30192, #45238, #12375, .T. ) ;
#44746=VECTOR ( 'NONE', #41270, 999.9999999999998863 ) ;
#44747=AXIS2_PLACEMENT_3D ( 'NONE', #22842, #9810, #26536 ) ;
#44748=ORIENTED_EDGE ( 'NONE', *, *, #20725, .F. ) ;
#44749=CARTESIAN_POINT ( 'NONE',  ( -20.89189044771117665, -4.403642575758161648, 4.855941604891849117 ) ) ;
#44750=ORIENTED_EDGE ( 'NONE', *, *, #53860, .T. ) ;
#44751=EDGE_CURVE ( 'NONE', #53425, #40325, #43841, .T. ) ;
#44752=ORIENTED_EDGE ( 'NONE', *, *, #46076, .T. ) ;
#44753=ADVANCED_FACE ( 'NONE', ( #4409 ), #4957, .F. ) ;
#44754=VECTOR ( 'NONE', #36937, 999.9999999999998863 ) ;
#44756=FACE_OUTER_BOUND ( 'NONE', #7145, .T. ) ;
#44757=DIRECTION ( 'NONE',  ( -0.5364919789714478471, 0.6444004775717705469, -0.5449076811759709926 ) ) ;
#44760=EDGE_CURVE ( 'NONE', #5490, #931, #22286, .T. ) ;
#44761=ORIENTED_EDGE ( 'NONE', *, *, #44760, .F. ) ;
#44762=DIRECTION ( 'NONE',  ( 0.9999697198139515519, 0.000000000000000000, 0.007781995580013368816 ) ) ;
#44763=ORIENTED_EDGE ( 'NONE', *, *, #8464, .F. ) ;
#44764=ADVANCED_FACE ( 'NONE', ( #33936 ), #34240, .F. ) ;
#44765=DIRECTION ( 'NONE',  ( -0.9999697198139514409, -0.000000000000000000, -0.007781995580013368816 ) ) ;
#44766=ADVANCED_FACE ( 'NONE', ( #17438 ), #51254, .F. ) ;
#44767=DIRECTION ( 'NONE',  ( 0.5449076811759707706, 0.6444004775717708799, -0.5364919789714476250 ) ) ;
#44768=LINE ( 'NONE', #49308, #7727 ) ;
#44769=PLANE ( 'NONE',  #14017 ) ;
#44770=VECTOR ( 'NONE', #46323, 999.9999999999998863 ) ;
#44771=CARTESIAN_POINT ( 'NONE',  ( -17.73140113748535285, 0.000000000000000000, 13.85752530597602039 ) ) ;
#44772=CARTESIAN_POINT ( 'NONE',  ( -13.48557508382207359, 0.000000000000000000, 5.654129457846438278 ) ) ;
#44773=ORIENTED_EDGE ( 'NONE', *, *, #13260, .F. ) ;
#44774=CARTESIAN_POINT ( 'NONE',  ( -14.39317410385126372, 0.000000000000000000, 2.861735767543279518 ) ) ;
#44775=AXIS2_PLACEMENT_3D ( 'NONE', #34014, #3356, #33448 ) ;
#44776=ORIENTED_EDGE ( 'NONE', *, *, #16983, .F. ) ;
#44777=EDGE_CURVE ( 'NONE', #52307, #51848, #43565, .T. ) ;
#44778=LINE ( 'NONE', #31729, #39233 ) ;
#44779=CARTESIAN_POINT ( 'NONE',  ( -13.47539652419022360, 0.000000000000000000, 4.346206404110358079 ) ) ;
#44780=ADVANCED_FACE ( 'NONE', ( #51544 ), #21452, .F. ) ;
#44782=VECTOR ( 'NONE', #7069, 1000.000000000000227 ) ;
#44783=LINE ( 'NONE', #31468, #33157 ) ;
#44784=CARTESIAN_POINT ( 'NONE',  ( -16.02312377951670896, 0.000000000000000000, 7.481042016179210385 ) ) ;
#44785=ADVANCED_FACE ( 'NONE', ( #29955 ), #51799, .F. ) ;
#44786=CARTESIAN_POINT ( 'NONE',  ( -13.53673582514181106, 0.000000000000000000, 12.22817484722816772 ) ) ;
#44787=ORIENTED_EDGE ( 'NONE', *, *, #11286, .T. ) ;
#44788=AXIS2_PLACEMENT_3D ( 'NONE', #47762, #34668, #39209 ) ;
#44789=DIRECTION ( 'NONE',  ( 0.9321478471874541372, 0.000000000000000000, -0.3620778797217453771 ) ) ;
#44790=DIRECTION ( 'NONE',  ( -0.005961354470445682716, -0.6427876096865404731, 0.7660212471507180654 ) ) ;
#44791=CARTESIAN_POINT ( 'NONE',  ( -13.70441031555024480, 0.6102101463440035012, 1.985721203314722016 ) ) ;
#44792=VECTOR ( 'NONE', #3684, 999.9999999999998863 ) ;
#44793=FACE_OUTER_BOUND ( 'NONE', #48149, .T. ) ;
#44794=DIRECTION ( 'NONE',  ( 0.5449076811759707706, 0.6444004775717708799, -0.5364919789714476250 ) ) ;
#44795=DIRECTION ( 'NONE',  ( 0.9321478471874541372, 0.000000000000000000, -0.3620778797217453771 ) ) ;
#44796=VECTOR ( 'NONE', #48060, 999.9999999999998863 ) ;
#44797=VECTOR ( 'NONE', #53787, 999.9999999999998863 ) ;
#44798=CARTESIAN_POINT ( 'NONE',  ( -11.40636015113596180, 0.000000000000000000, 11.32142374880780089 ) ) ;
#44799=LINE ( 'NONE', #49884, #28321 ) ;
#44800=ORIENTED_EDGE ( 'NONE', *, *, #17615, .T. ) ;
#44801=EDGE_CURVE ( 'NONE', #43375, #51735, #6049, .T. ) ;
#44802=EDGE_LOOP ( 'NONE', ( #20987, #29126, #37911, #1653 ) ) ;
#44803=ORIENTED_EDGE ( 'NONE', *, *, #26268, .T. ) ;
#44804=ORIENTED_EDGE ( 'NONE', *, *, #10214, .F. ) ;
#44805=ORIENTED_EDGE ( 'NONE', *, *, #44195, .T. ) ;
#44806=DIRECTION ( 'NONE',  ( 0.005961354470445682716, -0.6427876096865404731, -0.7660212471507180654 ) ) ;
#44807=CARTESIAN_POINT ( 'NONE',  ( 2.072287782118878319, 0.000000000000000000, -2.950529333540147015 ) ) ;
#44808=VECTOR ( 'NONE', #42404, 1000.000000000000227 ) ;
#44809=EDGE_CURVE ( 'NONE', #41560, #3665, #10842, .T. ) ;
#44810=VERTEX_POINT ( 'NONE', #28428 ) ;
#44811=EDGE_LOOP ( 'NONE', ( #26964, #9568, #6612, #11417 ) ) ;
#44812=ORIENTED_EDGE ( 'NONE', *, *, #8881, .T. ) ;
#44813=AXIS2_PLACEMENT_3D ( 'NONE', #21518, #17514, #47625 ) ;
#44814=EDGE_CURVE ( 'NONE', #34831, #25201, #50289, .T. ) ;
#44815=EDGE_CURVE ( 'NONE', #54486, #44201, #37224, .T. ) ;
#44817=AXIS2_PLACEMENT_3D ( 'NONE', #11830, #15526, #8152 ) ;
#44818=CARTESIAN_POINT ( 'NONE',  ( -13.73672976910459909, 0.000000000000000000, 12.22661844811216270 ) ) ;
#44819=DIRECTION ( 'NONE',  ( 0.5364919789714477361, 0.6444004775717706579, 0.5449076811759711036 ) ) ;
#44820=ORIENTED_EDGE ( 'NONE', *, *, #8816, .F. ) ;
#44822=VECTOR ( 'NONE', #47340, 999.9999999999998863 ) ;
#44824=LINE ( 'NONE', #48529, #9198 ) ;
#44825=EDGE_CURVE ( 'NONE', #50536, #18340, #45211, .T. ) ;
#44826=DIRECTION ( 'NONE',  ( 0.5364919789714477361, 0.6444004775717706579, 0.5449076811759711036 ) ) ;
#44828=VECTOR ( 'NONE', #517, 1000.000000000000114 ) ;
#44829=CARTESIAN_POINT ( 'NONE',  ( -15.71187809204705665, 4.657758921906512306, 2.636351864413973622 ) ) ;
#44830=DIRECTION ( 'NONE',  ( 0.005002170337468016433, -0.7660444431189770143, -0.6427681459581293666 ) ) ;
#44831=VECTOR ( 'NONE', #30768, 1000.000000000000000 ) ;
#44832=CARTESIAN_POINT ( 'NONE',  ( -14.21625583054634845, 1.743523803501505709, 5.264817263711710105 ) ) ;
#44833=DIRECTION ( 'NONE',  ( -0.3620778797217456546, 0.000000000000000000, -0.9321478471874540261 ) ) ;
#44834=DIRECTION ( 'NONE',  ( 0.005002170337468016433, -0.7660444431189770143, -0.6427681459581293666 ) ) ;
#44835=EDGE_LOOP ( 'NONE', ( #11449, #34251, #31120, #29064 ) ) ;
#44836=DIRECTION ( 'NONE',  ( -0.005002170337468016433, -0.7660444431189770143, 0.6427681459581293666 ) ) ;
#44837=ORIENTED_EDGE ( 'NONE', *, *, #46327, .T. ) ;
#44838=EDGE_CURVE ( 'NONE', #30294, #50472, #32688, .T. ) ;
#44839=LINE ( 'NONE', #31524, #1073 ) ;
#44840=DIRECTION ( 'NONE',  ( 0.007781995580012663651, 0.000000000000000000, -0.9999697198139515519 ) ) ;
#44842=CARTESIAN_POINT ( 'NONE',  ( -13.95308603416844484, 0.000000000000000000, 6.019823249336194948 ) ) ;
#44844=FACE_OUTER_BOUND ( 'NONE', #35735, .T. ) ;
#44845=CARTESIAN_POINT ( 'NONE',  ( -17.02012697683945319, -0.3560938001956556742, 3.481155184349101539 ) ) ;
#44846=VECTOR ( 'NONE', #32415, 1000.000000000000114 ) ;
#44847=EDGE_CURVE ( 'NONE', #12550, #41644, #32444, .T. ) ;
#44848=PLANE ( 'NONE',  #13809 ) ;
#44849=VECTOR ( 'NONE', #44055, 1000.000000000000227 ) ;
#44850=LINE ( 'NONE', #49100, #36507 ) ;
#44851=ORIENTED_EDGE ( 'NONE', *, *, #25149, .F. ) ;
#44852=PLANE ( 'NONE',  #29353 ) ;
#44853=CARTESIAN_POINT ( 'NONE',  ( -28.92982233430281980, 0.000000000000000000, 7.919257187036034651 ) ) ;
#44854=FACE_OUTER_BOUND ( 'NONE', #8201, .T. ) ;
#44855=AXIS2_PLACEMENT_3D ( 'NONE', #4541, #13067, #20745 ) ;
#44856=LINE ( 'NONE', #48850, #41390 ) ;
#44857=CARTESIAN_POINT ( 'NONE',  ( -14.10280672071693431, -0.1191753592594197858, 12.40843558753103792 ) ) ;
#44858=CARTESIAN_POINT ( 'NONE',  ( -16.81190032086591302, 0.000000000000000000, 3.212244750653343583 ) ) ;
#44859=LINE ( 'NONE', #32087, #47374 ) ;
#44860=ORIENTED_EDGE ( 'NONE', *, *, #39728, .T. ) ;
#44861=VECTOR ( 'NONE', #27445, 1000.000000000000227 ) ;
#44862=VERTEX_POINT ( 'NONE', #54530 ) ;
#44864=VECTOR ( 'NONE', #35987, 1000.000000000000227 ) ;
#44865=FACE_OUTER_BOUND ( 'NONE', #19047, .T. ) ;
#44866=VECTOR ( 'NONE', #28140, 999.9999999999998863 ) ;
#44867=ORIENTED_EDGE ( 'NONE', *, *, #36572, .F. ) ;
#44868=LINE ( 'NONE', #40041, #51239 ) ;
#44869=ADVANCED_FACE ( 'NONE', ( #6576 ), #44626, .F. ) ;
#44870=VERTEX_POINT ( 'NONE', #11106 ) ;
#44871=CARTESIAN_POINT ( 'NONE',  ( -10.21719013929205566, 0.000000000000000000, 3.632898379970893821 ) ) ;
#44872=VECTOR ( 'NONE', #44716, 999.9999999999998863 ) ;
#44873=ORIENTED_EDGE ( 'NONE', *, *, #49746, .T. ) ;
#44874=AXIS2_PLACEMENT_3D ( 'NONE', #21732, #39042, #39631 ) ;
#44875=EDGE_LOOP ( 'NONE', ( #21194, #45928, #42002, #54617 ) ) ;
#44876=EDGE_CURVE ( 'NONE', #45468, #34418, #40391, .T. ) ;
#44877=ORIENTED_EDGE ( 'NONE', *, *, #9982, .T. ) ;
#44878=EDGE_CURVE ( 'NONE', #11770, #11704, #1489, .T. ) ;
#44879=DIRECTION ( 'NONE',  ( -0.5449076811759708816, 0.6444004775717707689, 0.5364919789714475140 ) ) ;
#44880=CARTESIAN_POINT ( 'NONE',  ( -25.20200914511100265, -0.1191753592594197858, 6.570942640130446932 ) ) ;
#44881=CARTESIAN_POINT ( 'NONE',  ( -12.55761894452918170, 0.000000000000000000, 5.830677040677434420 ) ) ;
#44882=ADVANCED_FACE ( 'NONE', ( #19349, #15637 ), #6872, .F. ) ;
#44883=EDGE_CURVE ( 'NONE', #29528, #14368, #36146, .T. ) ;
#44884=EDGE_CURVE ( 'NONE', #31703, #10496, #54277, .T. ) ;
#44885=DIRECTION ( 'NONE',  ( 0.005961354470445682716, -0.6427876096865404731, -0.7660212471507180654 ) ) ;
#44886=ORIENTED_EDGE ( 'NONE', *, *, #36477, .F. ) ;
#44887=ORIENTED_EDGE ( 'NONE', *, *, #11419, .F. ) ;
#44888=AXIS2_PLACEMENT_3D ( 'NONE', #20950, #24649, #51361 ) ;
#44889=CARTESIAN_POINT ( 'NONE',  ( -14.42478869240937378, 0.000000000000000000, 6.924142503378688751 ) ) ;
#44890=AXIS2_PLACEMENT_3D ( 'NONE', #11832, #33162, #16115 ) ;
#44891=ORIENTED_EDGE ( 'NONE', *, *, #47714, .T. ) ;
#44892=PLANE ( 'NONE',  #3034 ) ;
#44893=ORIENTED_EDGE ( 'NONE', *, *, #51691, .F. ) ;
#44894=AXIS2_PLACEMENT_3D ( 'NONE', #37035, #2645, #6941 ) ;
#44895=FACE_OUTER_BOUND ( 'NONE', #33689, .T. ) ;
#44896=CARTESIAN_POINT ( 'NONE',  ( 2.072287782118878319, 0.000000000000000000, -2.950529333540147015 ) ) ;
#44897=ORIENTED_EDGE ( 'NONE', *, *, #38223, .F. ) ;
#44898=DIRECTION ( 'NONE',  ( 0.9999697198139515519, 0.000000000000000000, 0.007781995580013368816 ) ) ;
#44899=EDGE_CURVE ( 'NONE', #47831, #15979, #36397, .T. ) ;
#44900=VECTOR ( 'NONE', #30739, 999.9999999999998863 ) ;
#44901=VERTEX_POINT ( 'NONE', #31860 ) ;
#44902=EDGE_CURVE ( 'NONE', #18997, #6604, #49171, .T. ) ;
#44903=CARTESIAN_POINT ( 'NONE',  ( -18.59370689556874012, 0.000000000000000000, 5.245044725140569852 ) ) ;
#44904=VECTOR ( 'NONE', #37547, 1000.000000000000227 ) ;
#44905=AXIS2_PLACEMENT_3D ( 'NONE', #36451, #54332, #18584 ) ;
#44906=EDGE_LOOP ( 'NONE', ( #22844, #34424, #8998, #31488 ) ) ;
#44907=DIRECTION ( 'NONE',  ( 0.000000000000000000, -1.000000000000000000, 0.000000000000000000 ) ) ;
#44908=FACE_OUTER_BOUND ( 'NONE', #44875, .T. ) ;
#44909=EDGE_CURVE ( 'NONE', #23765, #1914, #40679, .T. ) ;
#44910=VECTOR ( 'NONE', #2313, 1000.000000000000227 ) ;
#44911=CARTESIAN_POINT ( 'NONE',  ( -18.86354292863559579, 0.000000000000000000, 14.21804678658176080 ) ) ;
#44912=ORIENTED_EDGE ( 'NONE', *, *, #27211, .T. ) ;
#44913=AXIS2_PLACEMENT_3D ( 'NONE', #37424, #12723, #56168 ) ;
#44914=EDGE_CURVE ( 'NONE', #28441, #6152, #15123, .T. ) ;
#44915=DIRECTION ( 'NONE',  ( 0.9321478471874540261, 0.000000000000000000, -0.3620778797217456546 ) ) ;
#44916=DIRECTION ( 'NONE',  ( 0.005961354470445682716, -0.6427876096865404731, -0.7660212471507180654 ) ) ;
#44917=CARTESIAN_POINT ( 'NONE',  ( -17.70211622298184651, 0.000000000000000000, 10.09447668306734514 ) ) ;
#44919=DIRECTION ( 'NONE',  ( -0.6427681459581293666, -0.7660444431189770143, -0.005002170337467561935 ) ) ;
#44920=DIRECTION ( 'NONE',  ( -0.5364919789714478471, 0.6444004775717705469, -0.5449076811759709926 ) ) ;
#44921=VECTOR ( 'NONE', #17213, 1000.000000000000114 ) ;
#44922=VECTOR ( 'NONE', #3216, 1000.000000000000227 ) ;
#44924=ORIENTED_EDGE ( 'NONE', *, *, #52505, .F. ) ;
#44925=FACE_OUTER_BOUND ( 'NONE', #9558, .T. ) ;
#44926=CARTESIAN_POINT ( 'NONE',  ( -14.88080342873461248, 0.000000000000000000, 5.812597481837387114 ) ) ;
#44928=ORIENTED_EDGE ( 'NONE', *, *, #32084, .F. ) ;
#44929=DIRECTION ( 'NONE',  ( 0.9999697198139515519, 0.000000000000000000, 0.007781995580013368816 ) ) ;
#44931=VERTEX_POINT ( 'NONE', #12534 ) ;
#44932=CARTESIAN_POINT ( 'NONE',  ( -25.20123094555300369, 0.000000000000000000, 6.470945668149052032 ) ) ;
#44933=PLANE ( 'NONE',  #21502 ) ;
#44934=DIRECTION ( 'NONE',  ( -0.7660212471507179544, -0.6427876096865405842, -0.005961354470445141482 ) ) ;
#44935=VECTOR ( 'NONE', #34728, 1000.000000000000114 ) ;
#44936=ORIENTED_EDGE ( 'NONE', *, *, #26913, .F. ) ;
#44937=VERTEX_POINT ( 'NONE', #28733 ) ;
#44938=VECTOR ( 'NONE', #24293, 1000.000000000000114 ) ;
#44939=LINE ( 'NONE', #19355, #34074 ) ;
#44940=PLANE ( 'NONE',  #14191 ) ;
#44941=VECTOR ( 'NONE', #56038, 999.9999999999998863 ) ;
#44942=PLANE ( 'NONE',  #11206 ) ;
#44943=CARTESIAN_POINT ( 'NONE',  ( -15.08810187882396825, 0.000000000000000000, 6.749654433199698822 ) ) ;
#44944=EDGE_LOOP ( 'NONE', ( #28507, #51250, #18708, #47535 ) ) ;
#44945=DIRECTION ( 'NONE',  ( 0.007781995580012663651, -3.146120232559066537E-19, -0.9999697198139514409 ) ) ;
#44946=VECTOR ( 'NONE', #46089, 1000.000000000000114 ) ;
#44947=ADVANCED_FACE ( 'NONE', ( #33812 ), #7995, .F. ) ;
#44948=EDGE_LOOP ( 'NONE', ( #38032, #41155, #7152, #15068 ) ) ;
#44949=DIRECTION ( 'NONE',  ( -0.5449076811759708816, 0.6444004775717707689, 0.5364919789714475140 ) ) ;
#44950=CARTESIAN_POINT ( 'NONE',  ( -27.99767448711536133, 0.000000000000000000, 7.557179307314289218 ) ) ;
#44951=VECTOR ( 'NONE', #29312, 999.9999999999998863 ) ;
#44952=VECTOR ( 'NONE', #25558, 999.9999999999998863 ) ;
#44953=ORIENTED_EDGE ( 'NONE', *, *, #7882, .F. ) ;
#44954=DIRECTION ( 'NONE',  ( -0.5449076811759708816, 0.6444004775717707689, 0.5364919789714475140 ) ) ;
#44955=CARTESIAN_POINT ( 'NONE',  ( -14.85162214859956897, 1.419719901456505617, 2.405509639311967263 ) ) ;
#44956=DIRECTION ( 'NONE',  ( 0.005002170337468016433, -0.7660444431189770143, -0.6427681459581293666 ) ) ;
#44957=EDGE_CURVE ( 'NONE', #23998, #2328, #46042, .T. ) ;
#44958=VECTOR ( 'NONE', #33662, 999.9999999999998863 ) ;
#44959=EDGE_CURVE ( 'NONE', #44744, #55546, #50586, .T. ) ;
#44960=EDGE_CURVE ( 'NONE', #21098, #27295, #33281, .T. ) ;
#44961=VERTEX_POINT ( 'NONE', #11403 ) ;
#44962=VECTOR ( 'NONE', #46617, 999.9999999999998863 ) ;
#44963=CARTESIAN_POINT ( 'NONE',  ( -31.72704407542318350, -0.1191753592594197858, 9.105487798182664960 ) ) ;
#44964=VECTOR ( 'NONE', #9892, 1000.000000000000000 ) ;
#44965=ORIENTED_EDGE ( 'NONE', *, *, #3134, .F. ) ;
#44966=EDGE_CURVE ( 'NONE', #9919, #50834, #42351, .T. ) ;
#44967=VECTOR ( 'NONE', #29683, 999.9999999999998863 ) ;
#44968=ORIENTED_EDGE ( 'NONE', *, *, #18053, .T. ) ;
#44969=VECTOR ( 'NONE', #55823, 1000.000000000000227 ) ;
#44970=ORIENTED_EDGE ( 'NONE', *, *, #9058, .F. ) ;
#44971=DIRECTION ( 'NONE',  ( 0.5364919789714477361, 0.6444004775717706579, 0.5449076811759711036 ) ) ;
#44972=ORIENTED_EDGE ( 'NONE', *, *, #27786, .F. ) ;
#44973=LINE ( 'NONE', #10035, #9415 ) ;
#44974=VERTEX_POINT ( 'NONE', #38347 ) ;
#44975=CARTESIAN_POINT ( 'NONE',  ( -27.99845268667336384, -0.1191753592594197858, 7.657176279295684118 ) ) ;
#44976=DIRECTION ( 'NONE',  ( 0.2426528472758542054, 0.7422098413412800966, 0.6246952433987894571 ) ) ;
#44977=ORIENTED_EDGE ( 'NONE', *, *, #19061, .T. ) ;
#44978=DIRECTION ( 'NONE',  ( 0.5364919789714477361, 0.6444004775717706579, 0.5449076811759711036 ) ) ;
#44979=ORIENTED_EDGE ( 'NONE', *, *, #12090, .T. ) ;
#44980=EDGE_CURVE ( 'NONE', #39202, #10472, #51433, .T. ) ;
#44981=AXIS2_PLACEMENT_3D ( 'NONE', #38356, #47437, #34964 ) ;
#44983=CARTESIAN_POINT ( 'NONE',  ( -24.26986129792355129, -0.1191753592594197858, 6.208864760408702388 ) ) ;
#44986=ADVANCED_FACE ( 'NONE', ( #29850 ), #20759, .F. ) ;
#44988=DIRECTION ( 'NONE',  ( -0.005961354470445682716, -0.6427876096865404731, 0.7660212471507180654 ) ) ;
#44989=DIRECTION ( 'NONE',  ( 0.000000000000000000, -0.000000000000000000, -1.000000000000000000 ) ) ;
#44990=VECTOR ( 'NONE', #12389, 999.9999999999998863 ) ;
#44991=ORIENTED_EDGE ( 'NONE', *, *, #5228, .T. ) ;
#44992=ADVANCED_FACE ( 'NONE', ( #25566 ), #15941, .F. ) ;
#44993=ORIENTED_EDGE ( 'NONE', *, *, #4348, .T. ) ;
#44995=DIRECTION ( 'NONE',  ( 0.000000000000000000, -1.000000000000000000, 0.000000000000000000 ) ) ;
#44996=VECTOR ( 'NONE', #6033, 999.9999999999998863 ) ;
#44997=EDGE_CURVE ( 'NONE', #13033, #47531, #38651, .T. ) ;
#44998=CARTESIAN_POINT ( 'NONE',  ( -19.60834386242827776, 0.000000000000000000, 4.298478389818581213 ) ) ;
#44999=VECTOR ( 'NONE', #23805, 1000.000000000000227 ) ;
#45000=VECTOR ( 'NONE', #14588, 1000.000000000000227 ) ;
#45001=LINE ( 'NONE', #6113, #30403 ) ;
#45002=VERTEX_POINT ( 'NONE', #7402 ) ;
#45003=CARTESIAN_POINT ( 'NONE',  ( -12.26998356360862452, 0.000000000000000000, 2.878258927267324463 ) ) ;
#45004=CARTESIAN_POINT ( 'NONE',  ( -11.62834515084701081, 0.000000000000000000, 5.837908864213453342 ) ) ;
#45005=ORIENTED_EDGE ( 'NONE', *, *, #7507, .T. ) ;
#45006=CARTESIAN_POINT ( 'NONE',  ( 2.072287782118878319, 0.000000000000000000, -2.950529333540147015 ) ) ;
#45007=DIRECTION ( 'NONE',  ( -0.5449076811759708816, 0.6444004775717707689, 0.5364919789714475140 ) ) ;
#45008=ORIENTED_EDGE ( 'NONE', *, *, #27070, .F. ) ;
#45009=VECTOR ( 'NONE', #32278, 999.9999999999998863 ) ;
#45011=DIRECTION ( 'NONE',  ( 0.007781995580012663651, -3.146120232559066537E-19, -0.9999697198139514409 ) ) ;
#45012=VECTOR ( 'NONE', #48816, 1000.000000000000227 ) ;
#45013=DIRECTION ( 'NONE',  ( -0.5364919789714478471, 0.6444004775717705469, -0.5449076811759709926 ) ) ;
#45014=LINE ( 'NONE', #10665, #52262 ) ;
#45015=VECTOR ( 'NONE', #45481, 1000.000000000000227 ) ;
#45016=PLANE ( 'NONE',  #48285 ) ;
#45017=EDGE_LOOP ( 'NONE', ( #284, #37654, #20411, #35673 ) ) ;
#45018=VECTOR ( 'NONE', #16863, 1000.000000000000227 ) ;
#45020=CARTESIAN_POINT ( 'NONE',  ( -14.89098198836645892, 0.000000000000000000, 7.120520535573467313 ) ) ;
#45021=PLANE ( 'NONE',  #49428 ) ;
#45022=LINE ( 'NONE', #6130, #48769 ) ;
#45024=DIRECTION ( 'NONE',  ( 0.5449076811759707706, 0.6444004775717708799, -0.5364919789714476250 ) ) ;
#45025=EDGE_LOOP ( 'NONE', ( #37322, #32583, #9971, #3786 ) ) ;
#45026=PLANE ( 'NONE',  #40116 ) ;
#45027=DIRECTION ( 'NONE',  ( 0.000000000000000000, -1.000000000000000000, 0.000000000000000000 ) ) ;
#45028=VECTOR ( 'NONE', #10527, 999.9999999999998863 ) ;
#45029=CARTESIAN_POINT ( 'NONE',  ( -14.52556386394876853, -0.1191753592594177180, 7.023361275802077586 ) ) ;
#45031=ORIENTED_EDGE ( 'NONE', *, *, #35516, .T. ) ;
#45032=CARTESIAN_POINT ( 'NONE',  ( -20.06177075545399191, 0.000000000000000000, 14.76272000528038220 ) ) ;
#45034=DIRECTION ( 'NONE',  ( 0.005002170337468016433, -0.7660444431189770143, -0.6427681459581293666 ) ) ;
#45035=AXIS2_PLACEMENT_3D ( 'NONE', #34714, #9742, #52592 ) ;
#45036=FACE_OUTER_BOUND ( 'NONE', #44948, .T. ) ;
#45037=EDGE_CURVE ( 'NONE', #40714, #49849, #17070, .T. ) ;
#45038=EDGE_LOOP ( 'NONE', ( #12977, #24282, #5302, #22605 ) ) ;
#45039=DIRECTION ( 'NONE',  ( -0.005961354470445682716, -0.6427876096865404731, 0.7660212471507180654 ) ) ;
#45040=AXIS2_PLACEMENT_3D ( 'NONE', #34050, #12739, #55915 ) ;
#45041=EDGE_LOOP ( 'NONE', ( #51386, #23624, #40006, #22820 ) ) ;
#45042=ADVANCED_FACE ( 'NONE', ( #12235 ), #24448, .F. ) ;
#45043=EDGE_CURVE ( 'NONE', #51697, #10299, #20484, .T. ) ;
#45044=ORIENTED_EDGE ( 'NONE', *, *, #38717, .F. ) ;
#45045=VECTOR ( 'NONE', #49090, 1000.000000000000227 ) ;
#45046=ORIENTED_EDGE ( 'NONE', *, *, #44914, .F. ) ;
#45047=FACE_OUTER_BOUND ( 'NONE', #30266, .T. ) ;
#45048=VERTEX_POINT ( 'NONE', #55383 ) ;
#45049=ORIENTED_EDGE ( 'NONE', *, *, #17358, .T. ) ;
#45050=CARTESIAN_POINT ( 'NONE',  ( -16.10199555257484860, 4.495856970884009485, 10.51435023889596643 ) ) ;
#45051=LINE ( 'NONE', #27724, #17669 ) ;
#45052=ORIENTED_EDGE ( 'NONE', *, *, #49057, .T. ) ;
#45053=VECTOR ( 'NONE', #52928, 1000.000000000000227 ) ;
#45054=ORIENTED_EDGE ( 'NONE', *, *, #28097, .T. ) ;
#45055=DIRECTION ( 'NONE',  ( 0.9999697198139515519, 0.000000000000000000, 0.007781995580013368816 ) ) ;
#45056=ORIENTED_EDGE ( 'NONE', *, *, #4468, .T. ) ;
#45058=VECTOR ( 'NONE', #3947, 1000.000000000000000 ) ;
#45059=VECTOR ( 'NONE', #43205, 1000.000000000000000 ) ;
#45060=DIRECTION ( 'NONE',  ( -0.005002170337468016433, -0.7660444431189770143, 0.6427681459581293666 ) ) ;
#45061=CARTESIAN_POINT ( 'NONE',  ( -13.53673582514181106, 0.000000000000000000, 12.22817484722816772 ) ) ;
#45062=CARTESIAN_POINT ( 'NONE',  ( -25.20200914511100265, -0.1191753592594197858, 6.570942640130446932 ) ) ;
#45063=CARTESIAN_POINT ( 'NONE',  ( -24.26908309836554878, 0.000000000000000000, 6.108867788427308376 ) ) ;
#45064=ORIENTED_EDGE ( 'NONE', *, *, #3656, .T. ) ;
#45065=CARTESIAN_POINT ( 'NONE',  ( -18.59746678161252476, -2.784623065533160524, 4.016364732897353740 ) ) ;
#45066=ORIENTED_EDGE ( 'NONE', *, *, #12544, .T. ) ;
#45067=FACE_OUTER_BOUND ( 'NONE', #49800, .T. ) ;
#45068=EDGE_CURVE ( 'NONE', #1446, #16052, #55127, .T. ) ;
#45069=VECTOR ( 'NONE', #15729, 999.9999999999998863 ) ;
#45070=CARTESIAN_POINT ( 'NONE',  ( -17.36532418587302473, -0.1191753592594177458, 13.67570816655714516 ) ) ;
#45071=DIRECTION ( 'NONE',  ( 0.9999697198139515519, 0.000000000000000000, 0.007781995580013368816 ) ) ;
#45072=CARTESIAN_POINT ( 'NONE',  ( -9.075990533167328067, 0.000000000000000000, 10.41622904950343909 ) ) ;
#45073=EDGE_CURVE ( 'NONE', #1575, #37986, #37511, .T. ) ;
#45074=PLANE ( 'NONE',  #23011 ) ;
#45075=DIRECTION ( 'NONE',  ( -0.5449076811759708816, 0.6444004775717707689, 0.5364919789714475140 ) ) ;
#45076=EDGE_LOOP ( 'NONE', ( #26234, #45170, #49216, #41035 ) ) ;
#45077=DIRECTION ( 'NONE',  ( 0.9321478471874541372, 0.000000000000000000, -0.3620778797217453771 ) ) ;
#45079=ORIENTED_EDGE ( 'NONE', *, *, #15912, .F. ) ;
#45080=DIRECTION ( 'NONE',  ( 0.9999697198139515519, 0.000000000000000000, 0.007781995580013368816 ) ) ;
#45081=LINE ( 'NONE', #54150, #30536 ) ;
#45082=AXIS2_PLACEMENT_3D ( 'NONE', #35126, #5291, #22329 ) ;
#45083=FACE_OUTER_BOUND ( 'NONE', #8588, .T. ) ;
#45084=ADVANCED_FACE ( 'NONE', ( #54832 ), #25304, .F. ) ;
#45085=DIRECTION ( 'NONE',  ( 0.005002170337468016433, -0.7660444431189770143, -0.6427681459581293666 ) ) ;
#45086=PLANE ( 'NONE',  #43193 ) ;
#45089=ORIENTED_EDGE ( 'NONE', *, *, #16092, .T. ) ;
#45091=DIRECTION ( 'NONE',  ( 0.5364919789714477361, 0.6444004775717706579, 0.5449076811759711036 ) ) ;
#45092=CARTESIAN_POINT ( 'NONE',  ( -19.25715946501773956, -2.460819163488159766, 4.282942814164549361 ) ) ;
#45093=AXIS2_PLACEMENT_3D ( 'NONE', #40294, #31516, #10184 ) ;
#45097=CARTESIAN_POINT ( 'NONE',  ( -18.66354898467281132, 0.000000000000000000, 14.21960318569776582 ) ) ;
#45098=VECTOR ( 'NONE', #10151, 999.9999999999998863 ) ;
#45100=CARTESIAN_POINT ( 'NONE',  ( -19.61264301455797465, 3.200641362704010007, 4.198031109838099795 ) ) ;
#45101=EDGE_CURVE ( 'NONE', #30427, #47379, #39772, .T. ) ;
#45102=ORIENTED_EDGE ( 'NONE', *, *, #31290, .F. ) ;
#45103=ADVANCED_FACE ( 'NONE', ( #588 ), #34957, .F. ) ;
#45104=ADVANCED_FACE ( 'NONE', ( #4301 ), #9373, .F. ) ;
#45105=ORIENTED_EDGE ( 'NONE', *, *, #28616, .F. ) ;
#45106=ORIENTED_EDGE ( 'NONE', *, *, #25886, .T. ) ;
#45107=EDGE_LOOP ( 'NONE', ( #25607, #20751, #42766, #55427 ) ) ;
#45108=ORIENTED_EDGE ( 'NONE', *, *, #54741, .F. ) ;
#45109=DIRECTION ( 'NONE',  ( -0.9999697198139514409, -0.000000000000000000, -0.007781995580013368816 ) ) ;
#45110=DIRECTION ( 'NONE',  ( -0.9999697198139514409, -0.000000000000000000, -0.007781995580013368816 ) ) ;
#45112=EDGE_LOOP ( 'NONE', ( #53953, #2489, #21537, #32660 ) ) ;
#45114=VERTEX_POINT ( 'NONE', #21614 ) ;
#45115=EDGE_CURVE ( 'NONE', #56197, #47765, #17917, .T. ) ;
#45116=VECTOR ( 'NONE', #45539, 999.9999999999998863 ) ;
#45117=DIRECTION ( 'NONE',  ( -0.7660212471507179544, -0.6427876096865405842, -0.005961354470445141482 ) ) ;
#45118=DIRECTION ( 'NONE',  ( 0.007781995580012662783, 0.000000000000000000, -0.9999697198139514409 ) ) ;
#45119=DIRECTION ( 'NONE',  ( 0.9999697198139515519, 0.000000000000000000, 0.007781995580013368816 ) ) ;
#45120=ORIENTED_EDGE ( 'NONE', *, *, #44876, .F. ) ;
#45121=CARTESIAN_POINT ( 'NONE',  ( -10.74029228357944987, 0.000000000000000000, 11.14194120806293320 ) ) ;
#45122=ORIENTED_EDGE ( 'NONE', *, *, #30, .F. ) ;
#45123=VECTOR ( 'NONE', #9588, 1000.000000000000227 ) ;
#45124=LINE ( 'NONE', #19252, #16439 ) ;
#45125=DIRECTION ( 'NONE',  ( 0.000000000000000000, -1.000000000000000000, 0.000000000000000000 ) ) ;
#45127=DIRECTION ( 'NONE',  ( -0.6427681459581293666, -0.7660444431189770143, -0.005002170337467561935 ) ) ;
#45128=DIRECTION ( 'NONE',  ( 0.005002170337468016433, -0.7660444431189770143, -0.6427681459581293666 ) ) ;
#45129=CARTESIAN_POINT ( 'NONE',  ( -15.40103151951671734, 0.000000000000000000, 12.95233060667165681 ) ) ;
#45130=CARTESIAN_POINT ( 'NONE',  ( -12.80458192191714595, 0.000000000000000000, 11.86454056839041726 ) ) ;
#45131=CARTESIAN_POINT ( 'NONE',  ( -16.26190025084746082, 0.000000000000000000, 4.155195174207322317 ) ) ;
#45132=EDGE_LOOP ( 'NONE', ( #38598, #26644, #18338, #32270 ) ) ;
#45133=DIRECTION ( 'NONE',  ( 0.005002170337468016433, -0.7660444431189770143, -0.6427681459581293666 ) ) ;
#45134=ORIENTED_EDGE ( 'NONE', *, *, #3677, .T. ) ;
#45135=DIRECTION ( 'NONE',  ( -0.5449076811759708816, 0.6444004775717707689, 0.5364919789714475140 ) ) ;
#45136=DIRECTION ( 'NONE',  ( -0.7660212471507179544, -0.6427876096865405842, -0.005961354470445141482 ) ) ;
#45137=DIRECTION ( 'NONE',  ( -0.6427681459581293666, -0.7660444431189770143, -0.005002170337467561935 ) ) ;
#45138=CARTESIAN_POINT ( 'NONE',  ( -31.72626587586518099, 0.000000000000000000, 9.005490826201270949 ) ) ;
#45139=ADVANCED_FACE ( 'NONE', ( #35240 ), #8542, .F. ) ;
#45140=CARTESIAN_POINT ( 'NONE',  ( -16.81190032086591302, 0.000000000000000000, 3.212244750653343583 ) ) ;
#45141=DIRECTION ( 'NONE',  ( -0.5364919789714478471, 0.6444004775717705469, -0.5449076811759709926 ) ) ;
#45142=DIRECTION ( 'NONE',  ( -0.7660212471507179544, -0.6427876096865405842, -0.005961354470445141482 ) ) ;
#45143=PLANE ( 'NONE',  #22093 ) ;
#45144=DIRECTION ( 'NONE',  ( -0.005002170337468016433, -0.7660444431189770143, 0.6427681459581293666 ) ) ;
#45145=VERTEX_POINT ( 'NONE', #17619 ) ;
#45146=LINE ( 'NONE', #14481, #22100 ) ;
#45147=DIRECTION ( 'NONE',  ( -0.7660212471507179544, -0.6427876096865405842, -0.005961354470445141482 ) ) ;
#45148=DIRECTION ( 'NONE',  ( 0.2426528472758541499, 0.7422098413412800966, 0.6246952433987894571 ) ) ;
#45149=CARTESIAN_POINT ( 'NONE',  ( -10.74029228357944987, 0.000000000000000000, 11.14194120806293320 ) ) ;
#45150=EDGE_CURVE ( 'NONE', #19093, #27501, #43457, .T. ) ;
#45151=CARTESIAN_POINT ( 'NONE',  ( -14.63340479688801032, 0.000000000000000000, 8.030515214035977678 ) ) ;
#45152=CARTESIAN_POINT ( 'NONE',  ( -9.391565570654567097, -0.1191753592594177180, 4.108658679188065932 ) ) ;
#45153=ADVANCED_FACE ( 'NONE', ( #848 ), #26694, .F. ) ;
#45154=DIRECTION ( 'NONE',  ( -0.005961354470445682716, -0.6427876096865404731, 0.7660212471507180654 ) ) ;
#45155=EDGE_CURVE ( 'NONE', #12359, #24475, #13908, .T. ) ;
#45156=LINE ( 'NONE', #49937, #23820 ) ;
#45157=VERTEX_POINT ( 'NONE', #9093 ) ;
#45158=VERTEX_POINT ( 'NONE', #9679 ) ;
#45159=CARTESIAN_POINT ( 'NONE',  ( -16.73647696259367024, 0.000000000000000000, 5.428824131507583139 ) ) ;
#45160=CARTESIAN_POINT ( 'NONE',  ( -14.46438462897659250, 2.067327705546506689, 2.234431356499322341 ) ) ;
#45161=ADVANCED_FACE ( 'NONE', ( #44305 ), #31237, .F. ) ;
#45162=AXIS2_PLACEMENT_3D ( 'NONE', #31591, #17965, #30995 ) ;
#45163=VERTEX_POINT ( 'NONE', #35491 ) ;
#45164=EDGE_CURVE ( 'NONE', #14416, #21318, #40030, .T. ) ;
#45165=LINE ( 'NONE', #1430, #46740 ) ;
#45166=EDGE_LOOP ( 'NONE', ( #15462, #84, #25692, #54548, #23099 ) ) ;
#45167=LINE ( 'NONE', #19297, #39272 ) ;
#45168=EDGE_CURVE ( 'NONE', #38799, #46492, #1116, .T. ) ;
#45169=ORIENTED_EDGE ( 'NONE', *, *, #13133, .F. ) ;
#45170=ORIENTED_EDGE ( 'NONE', *, *, #2621, .T. ) ;
#45171=ORIENTED_EDGE ( 'NONE', *, *, #29182, .T. ) ;
#45172=LINE ( 'NONE', #31259, #45626 ) ;
#45173=FACE_OUTER_BOUND ( 'NONE', #33855, .T. ) ;
#45174=FACE_OUTER_BOUND ( 'NONE', #384, .T. ) ;
#45176=ORIENTED_EDGE ( 'NONE', *, *, #42546, .F. ) ;
#45177=ORIENTED_EDGE ( 'NONE', *, *, #34237, .T. ) ;
#45178=EDGE_CURVE ( 'NONE', #37328, #31229, #22714, .T. ) ;
#45179=CARTESIAN_POINT ( 'NONE',  ( -10.27421835998572064, 0.000000000000000000, 10.96090226820206048 ) ) ;
#45181=PLANE ( 'NONE',  #22795 ) ;
#45182=ORIENTED_EDGE ( 'NONE', *, *, #55791, .T. ) ;
#45183=DIRECTION ( 'NONE',  ( 0.9999697198139515519, 0.000000000000000000, 0.007781995580013368816 ) ) ;
#45184=CARTESIAN_POINT ( 'NONE',  ( -14.30671182103509054, 0.7721120973665049902, 2.214510042402868972 ) ) ;
#45185=ORIENTED_EDGE ( 'NONE', *, *, #27610, .F. ) ;
#45186=DIRECTION ( 'NONE',  ( 0.9999697198139515519, 0.000000000000000000, 0.007781995580013368816 ) ) ;
#45187=CARTESIAN_POINT ( 'NONE',  ( -17.02322106989970507, -0.3560938001956550081, 3.878739497874950093 ) ) ;
#45188=ORIENTED_EDGE ( 'NONE', *, *, #14705, .F. ) ;
#45190=DIRECTION ( 'NONE',  ( 0.000000000000000000, -1.000000000000000000, 0.000000000000000000 ) ) ;
#45191=DIRECTION ( 'NONE',  ( 0.9999697198139515519, 0.000000000000000000, 0.007781995580013368816 ) ) ;
#45192=EDGE_LOOP ( 'NONE', ( #47208, #51158, #10630, #54115 ) ) ;
#45194=PLANE ( 'NONE',  #32829 ) ;
#45195=CARTESIAN_POINT ( 'NONE',  ( -14.87948577434532815, 0.000000000000000000, 5.643281722542411671 ) ) ;
#45196=CARTESIAN_POINT ( 'NONE',  ( -16.38411145131311031, -0.1191753592594183703, 7.008897628730038853 ) ) ;
#45197=EDGE_CURVE ( 'NONE', #9219, #41657, #47735, .T. ) ;
#45198=PLANE ( 'NONE',  #25949 ) ;
#45199=CARTESIAN_POINT ( 'NONE',  ( -9.342070512798265725, 0.000000000000000000, 10.59882438848031505 ) ) ;
#45200=LINE ( 'NONE', #50276, #42440 ) ;
#45202=EDGE_LOOP ( 'NONE', ( #47016, #42526, #7104, #16867 ) ) ;
#45203=DIRECTION ( 'NONE',  ( 0.5449076811759707706, 0.6444004775717708799, -0.5364919789714476250 ) ) ;
#45204=CARTESIAN_POINT ( 'NONE',  ( -13.03375205539139969, 0.000000000000000000, 7.304299941940480601 ) ) ;
#45206=EDGE_LOOP ( 'NONE', ( #10161, #30322, #22876, #17484 ) ) ;
#45207=PLANE ( 'NONE',  #16616 ) ;
#45208=CARTESIAN_POINT ( 'NONE',  ( -13.92853720701018183, 0.000000000000000000, 2.865351679311290756 ) ) ;
#45210=EDGE_CURVE ( 'NONE', #18030, #5375, #17322, .T. ) ;
#45211=LINE ( 'NONE', #49997, #42184 ) ;
#45212=DIRECTION ( 'NONE',  ( 0.9999697198139515519, 0.000000000000000000, 0.007781995580013368816 ) ) ;
#45213=EDGE_CURVE ( 'NONE', #29102, #42137, #2529, .T. ) ;
#45214=DIRECTION ( 'NONE',  ( -0.5364919789714478471, 0.6444004775717705469, -0.5449076811759709926 ) ) ;
#45215=ORIENTED_EDGE ( 'NONE', *, *, #41667, .T. ) ;
#45216=ORIENTED_EDGE ( 'NONE', *, *, #48178, .T. ) ;
#45217=DIRECTION ( 'NONE',  ( 0.5364919789714477361, 0.6444004775717706579, 0.5449076811759711036 ) ) ;
#45219=CARTESIAN_POINT ( 'NONE',  ( -22.40634380310664397, 0.000000000000000000, 5.584705972946605534 ) ) ;
#45220=ORIENTED_EDGE ( 'NONE', *, *, #32348, .T. ) ;
#45221=EDGE_CURVE ( 'NONE', #40778, #23767, #6510, .T. ) ;
#45222=DIRECTION ( 'NONE',  ( 0.7660212471507180654, -0.6427876096865404731, 0.005961354470445141482 ) ) ;
#45223=VERTEX_POINT ( 'NONE', #45151 ) ;
#45224=DIRECTION ( 'NONE',  ( 0.6427681459581294776, -0.7660444431189769032, 0.005002170337467562802 ) ) ;
#45225=EDGE_CURVE ( 'NONE', #23847, #55136, #5675, .T. ) ;
#45226=VERTEX_POINT ( 'NONE', #18761 ) ;
#45227=PLANE ( 'NONE',  #12028 ) ;
#45228=LINE ( 'NONE', #36163, #49551 ) ;
#45229=DIRECTION ( 'NONE',  ( -0.7660212471507179544, -0.6427876096865405842, -0.005961354470445141482 ) ) ;
#45230=ORIENTED_EDGE ( 'NONE', *, *, #24107, .F. ) ;
#45231=EDGE_CURVE ( 'NONE', #29572, #23095, #5977, .T. ) ;
#45232=VECTOR ( 'NONE', #35862, 1000.000000000000000 ) ;
#45233=LINE ( 'NONE', #24213, #43910 ) ;
#45236=EDGE_LOOP ( 'NONE', ( #41131, #26291, #32719, #20009 ) ) ;
#45237=DIRECTION ( 'NONE',  ( -0.7660212471507179544, -0.6427876096865405842, -0.005961354470445141482 ) ) ;
#45238=VERTEX_POINT ( 'NONE', #53644 ) ;
#45239=DIRECTION ( 'NONE',  ( 0.000000000000000000, -0.000000000000000000, -1.000000000000000000 ) ) ;
#45240=ORIENTED_EDGE ( 'NONE', *, *, #3479, .F. ) ;
#45241=CARTESIAN_POINT ( 'NONE',  ( -19.73901266685368938, -4.079838673713159558, 11.04494491366336995 ) ) ;
#45242=CARTESIAN_POINT ( 'NONE',  ( -9.542064456761055524, 0.000000000000000000, 10.59726798936431180 ) ) ;
#45243=ORIENTED_EDGE ( 'NONE', *, *, #38262, .F. ) ;
#45244=CARTESIAN_POINT ( 'NONE',  ( -15.57145852836868549, -4.727446477803165514, 2.778974125015922336 ) ) ;
#45245=VERTEX_POINT ( 'NONE', #19281 ) ;
#45246=DIRECTION ( 'NONE',  ( -0.005002170337468016433, -0.7660444431189770143, 0.6427681459581293666 ) ) ;
#45247=DIRECTION ( 'NONE',  ( -0.005002170337468016433, -0.7660444431189770143, 0.6427681459581293666 ) ) ;
#45248=PLANE ( 'NONE',  #27778 ) ;
#45249=CARTESIAN_POINT ( 'NONE',  ( -17.74482636761137044, -0.1191753592594197858, 3.674319602356483916 ) ) ;
#45250=DIRECTION ( 'NONE',  ( 0.6427681459581294776, -0.7660444431189769032, 0.005002170337467562802 ) ) ;
#45251=CARTESIAN_POINT ( 'NONE',  ( -15.60102546347950536, 0.000000000000000000, 12.95077420755565356 ) ) ;
#45252=LINE ( 'NONE', #27362, #31056 ) ;
#45253=ORIENTED_EDGE ( 'NONE', *, *, #54692, .T. ) ;
#45254=EDGE_CURVE ( 'NONE', #8803, #50386, #27537, .T. ) ;
#45255=EDGE_LOOP ( 'NONE', ( #38831, #55410, #8066, #7245 ) ) ;
#45256=CARTESIAN_POINT ( 'NONE',  ( 2.072287782118878319, 0.000000000000000000, -2.950529333540147015 ) ) ;
#45257=LINE ( 'NONE', #10055, #19432 ) ;
#45258=ADVANCED_FACE ( 'NONE', ( #6254 ), #6796, .F. ) ;
#45259=DIRECTION ( 'NONE',  ( 0.005002170337468016433, -0.7660444431189770143, -0.6427681459581293666 ) ) ;
#45260=CARTESIAN_POINT ( 'NONE',  ( -24.27063949748155380, 0.000000000000000000, 6.308861732390097288 ) ) ;
#45261=CARTESIAN_POINT ( 'NONE',  ( -11.25011315801890532, -0.1191753592594183703, 4.094195032116028976 ) ) ;
#45262=EDGE_LOOP ( 'NONE', ( #5159, #48222, #45713, #14397 ) ) ;
#45263=EDGE_CURVE ( 'NONE', #25181, #49693, #23557, .T. ) ;
#45264=FACE_OUTER_BOUND ( 'NONE', #19625, .T. ) ;
#45265=LINE ( 'NONE', #23417, #23230 ) ;
#45266=ORIENTED_EDGE ( 'NONE', *, *, #41298, .F. ) ;
#45267=DIRECTION ( 'NONE',  ( 0.007781995580012662783, 0.000000000000000000, -0.9999697198139514409 ) ) ;
#45268=CARTESIAN_POINT ( 'NONE',  ( -12.62677952751046995, -0.1191753592594201328, 1.867489077265416908 ) ) ;
#45269=ORIENTED_EDGE ( 'NONE', *, *, #47669, .T. ) ;
#45270=EDGE_CURVE ( 'NONE', #49166, #44182, #36918, .T. ) ;
#45271=EDGE_CURVE ( 'NONE', #32587, #42240, #14756, .T. ) ;
#45272=ADVANCED_FACE ( 'NONE', ( #15316 ), #11037, .F. ) ;
#45273=VECTOR ( 'NONE', #19065, 999.9999999999998863 ) ;
#45275=CARTESIAN_POINT ( 'NONE',  ( -25.20278734466900517, 0.000000000000000000, 6.670939612111840944 ) ) ;
#45276=PLANE ( 'NONE',  #30456 ) ;
#45277=EDGE_CURVE ( 'NONE', #45990, #40411, #49400, .T. ) ;
#45278=FACE_OUTER_BOUND ( 'NONE', #29747, .T. ) ;
#45279=CARTESIAN_POINT ( 'NONE',  ( -16.40332474553500575, -2.946525016555659793, 3.158919932820265064 ) ) ;
#45281=EDGE_LOOP ( 'NONE', ( #49990, #53259, #5559, #21262 ) ) ;
#45282=CARTESIAN_POINT ( 'NONE',  ( -12.13851405436063047, 0.000000000000000000, 11.68505802764555135 ) ) ;
#45283=DIRECTION ( 'NONE',  ( -0.5364919789714478471, 0.6444004775717705469, -0.5449076811759709926 ) ) ;
#45284=LINE ( 'NONE', #39901, #26073 ) ;
#45285=LINE ( 'NONE', #40179, #51828 ) ;
#45286=EDGE_CURVE ( 'NONE', #23729, #30483, #1950, .T. ) ;
#45288=ORIENTED_EDGE ( 'NONE', *, *, #38149, .F. ) ;
#45289=CARTESIAN_POINT ( 'NONE',  ( -16.29926294641613538, 0.000000000000000000, 8.956221316558263368 ) ) ;
#45290=EDGE_CURVE ( 'NONE', #30787, #23833, #32381, .T. ) ;
#45291=CARTESIAN_POINT ( 'NONE',  ( -31.72626587586518099, 0.000000000000000000, 9.005490826201270949 ) ) ;
#45292=CARTESIAN_POINT ( 'NONE',  ( -12.11256978495757330, 0.9340140483890051470, 1.357065242325779408 ) ) ;
#45293=ORIENTED_EDGE ( 'NONE', *, *, #6459, .T. ) ;
#45294=EDGE_CURVE ( 'NONE', #7889, #22392, #45399, .T. ) ;
#45295=LINE ( 'NONE', #6397, #45593 ) ;
#45296=ORIENTED_EDGE ( 'NONE', *, *, #4251, .F. ) ;
#45297=FACE_OUTER_BOUND ( 'NONE', #24152, .T. ) ;
#45298=LINE ( 'NONE', #6400, #23899 ) ;
#45299=ORIENTED_EDGE ( 'NONE', *, *, #19245, .F. ) ;
#45300=EDGE_CURVE ( 'NONE', #33876, #39389, #48853, .T. ) ;
#45301=CARTESIAN_POINT ( 'NONE',  ( -17.74482636761137044, -0.1191753592594197858, 3.674319602356483916 ) ) ;
#45303=ADVANCED_FACE ( 'NONE', ( #19580 ), #28358, .T. ) ;
#45304=EDGE_LOOP ( 'NONE', ( #19978, #5231, #41248, #46941 ) ) ;
#45305=ORIENTED_EDGE ( 'NONE', *, *, #8804, .F. ) ;
#45306=FACE_OUTER_BOUND ( 'NONE', #34, .T. ) ;
#45307=ORIENTED_EDGE ( 'NONE', *, *, #39241, .F. ) ;
#45308=ORIENTED_EDGE ( 'NONE', *, *, #12763, .T. ) ;
#45309=CARTESIAN_POINT ( 'NONE',  ( -14.63208714249872955, 0.000000000000000000, 7.861199454741004899 ) ) ;
#45310=EDGE_LOOP ( 'NONE', ( #16485, #13974, #6846, #48802 ) ) ;
#45311=EDGE_LOOP ( 'NONE', ( #34626, #37833, #42080, #7419 ) ) ;
#45312=DIRECTION ( 'NONE',  ( -0.5449076811759708816, 0.6444004775717707689, 0.5364919789714475140 ) ) ;
#45313=ORIENTED_EDGE ( 'NONE', *, *, #26268, .F. ) ;
#45314=VERTEX_POINT ( 'NONE', #14487 ) ;
#45315=CARTESIAN_POINT ( 'NONE',  ( 2.072287782118878319, 0.000000000000000000, -2.950529333540147015 ) ) ;
#45316=CARTESIAN_POINT ( 'NONE',  ( -11.72049816187055882, -0.1191753592594181482, 4.829198526863549112 ) ) ;
#45317=PLANE ( 'NONE',  #49544 ) ;
#45318=CARTESIAN_POINT ( 'NONE',  ( -18.67619601524082285, 0.000000000000000000, 3.936400510096834893 ) ) ;
#45319=ORIENTED_EDGE ( 'NONE', *, *, #33159, .T. ) ;
#45320=CARTESIAN_POINT ( 'NONE',  ( -14.50257143590650699, -0.1191753592594186895, 4.068883649739962749 ) ) ;
#45321=ORIENTED_EDGE ( 'NONE', *, *, #43920, .F. ) ;
#45322=ORIENTED_EDGE ( 'NONE', *, *, #36509, .T. ) ;
#45325=LINE ( 'NONE', #6436, #8590 ) ;
#45326=DIRECTION ( 'NONE',  ( 0.2426528472758542054, 0.7422098413412800966, 0.6246952433987894571 ) ) ;
#45327=CARTESIAN_POINT ( 'NONE',  ( -9.342070512798265725, 0.000000000000000000, 10.59882438848031505 ) ) ;
#45328=EDGE_LOOP ( 'NONE', ( #12687, #32859, #3446, #23432 ) ) ;
#45329=CARTESIAN_POINT ( 'NONE',  ( -11.20636620717317378, 0.000000000000000000, 11.32298014792380414 ) ) ;
#45330=ORIENTED_EDGE ( 'NONE', *, *, #52288, .T. ) ;
#45331=ADVANCED_FACE ( 'NONE', ( #31798 ), #49109, .F. ) ;
#45332=EDGE_CURVE ( 'NONE', #21088, #37252, #29501, .T. ) ;
#45333=DIRECTION ( 'NONE',  ( 0.007781995580012663651, 0.000000000000000000, -0.9999697198139515519 ) ) ;
#45334=LINE ( 'NONE', #14675, #6054 ) ;
#45335=DIRECTION ( 'NONE',  ( -0.005002170337468016433, -0.7660444431189770143, 0.6427681459581293666 ) ) ;
#45336=DIRECTION ( 'NONE',  ( 0.6427681459581294776, -0.7660444431189769032, 0.005002170337467562802 ) ) ;
#45337=EDGE_CURVE ( 'NONE', #46574, #29949, #50219, .T. ) ;
#45338=DIRECTION ( 'NONE',  ( 0.9999697198139515519, 0.000000000000000000, 0.007781995580013368816 ) ) ;
#45339=VERTEX_POINT ( 'NONE', #55321 ) ;
#45340=CARTESIAN_POINT ( 'NONE',  ( -17.90272870724953691, 0.000000000000000000, 10.17240138478555878 ) ) ;
#45341=FACE_OUTER_BOUND ( 'NONE', #53908, .T. ) ;
#45342=CARTESIAN_POINT ( 'NONE',  ( -9.969791507445457057, 0.000000000000000000, 5.850816112169488825 ) ) ;
#45344=PLANE ( 'NONE',  #17635 ) ;
#45345=CARTESIAN_POINT ( 'NONE',  ( -17.43559644546093779, 0.000000000000000000, 9.855368259716744461 ) ) ;
#45346=CARTESIAN_POINT ( 'NONE',  ( -14.01545677930355183, 0.000000000000000000, 2.126011111488108174 ) ) ;
#45348=CARTESIAN_POINT ( 'NONE',  ( -14.69713173337877166, 0.1245042932765033361, 2.794518955481596567 ) ) ;
#45350=ADVANCED_FACE ( 'NONE', ( #25245 ), #11330, .F. ) ;
#45352=ORIENTED_EDGE ( 'NONE', *, *, #16464, .T. ) ;
#45353=ORIENTED_EDGE ( 'NONE', *, *, #55921, .T. ) ;
#45354=EDGE_CURVE ( 'NONE', #19918, #47531, #45983, .T. ) ;
#45355=EDGE_LOOP ( 'NONE', ( #29788, #55946, #50744, #24224 ) ) ;
#45356=DIRECTION ( 'NONE',  ( 0.007781995580012663651, -3.146120232559066537E-19, -0.9999697198139514409 ) ) ;
#45357=EDGE_CURVE ( 'NONE', #23572, #21327, #7090, .T. ) ;
#45358=CARTESIAN_POINT ( 'NONE',  ( -10.86137571651779510, 0.000000000000000000, 1.000553606503651771 ) ) ;
#45359=VERTEX_POINT ( 'NONE', #16414 ) ;
#45360=FACE_OUTER_BOUND ( 'NONE', #20857, .T. ) ;
#45361=ADVANCED_FACE ( 'NONE', ( #46509 ), #42281, .F. ) ;
#45362=ORIENTED_EDGE ( 'NONE', *, *, #42502, .T. ) ;
#45363=ORIENTED_EDGE ( 'NONE', *, *, #32558, .F. ) ;
#45364=VECTOR ( 'NONE', #27993, 1000.000000000000227 ) ;
#45365=PLANE ( 'NONE',  #20182 ) ;
#45366=DIRECTION ( 'NONE',  ( 0.000000000000000000, -0.000000000000000000, -1.000000000000000000 ) ) ;
#45367=CARTESIAN_POINT ( 'NONE',  ( -16.96233738810400737, 0.000000000000000000, 8.751055061711459970 ) ) ;
#45368=ORIENTED_EDGE ( 'NONE', *, *, #27316, .F. ) ;
#45369=CARTESIAN_POINT ( 'NONE',  ( -11.92213221946999724, 2.876837460659007473, 6.233662532057125283 ) ) ;
#45370=LINE ( 'NONE', #25222, #27313 ) ;
#45371=LINE ( 'NONE', #5641, #5783 ) ;
#45372=CARTESIAN_POINT ( 'NONE',  ( -18.16068458728576118, 0.000000000000000000, 9.311067372743988102 ) ) ;
#45373=LINE ( 'NONE', #33180, #33289 ) ;
#45374=DIRECTION ( 'NONE',  ( -0.9999697198139514409, -0.000000000000000000, -0.007781995580013368816 ) ) ;
#45375=LINE ( 'NONE', #6490, #41989 ) ;
#45376=DIRECTION ( 'NONE',  ( 0.000000000000000000, -1.000000000000000000, 0.000000000000000000 ) ) ;
#45377=DIRECTION ( 'NONE',  ( -0.5449076811759708816, 0.6444004775717707689, 0.5364919789714475140 ) ) ;
#45378=ORIENTED_EDGE ( 'NONE', *, *, #23980, .F. ) ;
#45379=LINE ( 'NONE', #32360, #38293 ) ;
#45380=VERTEX_POINT ( 'NONE', #41972 ) ;
#45381=ADVANCED_FACE ( 'NONE', ( #12475 ), #16710, .F. ) ;
#45382=LINE ( 'NONE', #6496, #26551 ) ;
#45383=DIRECTION ( 'NONE',  ( 0.5449076811759707706, 0.6444004775717708799, -0.5364919789714476250 ) ) ;
#45384=LINE ( 'NONE', #46731, #14054 ) ;
#45385=CARTESIAN_POINT ( 'NONE',  ( -11.20636620717317378, 0.000000000000000000, 11.32298014792380414 ) ) ;
#45386=DIRECTION ( 'NONE',  ( 0.9999697198139515519, 0.000000000000000000, 0.007781995580013368816 ) ) ;
#45387=DIRECTION ( 'NONE',  ( -0.005961354470445682716, -0.6427876096865404731, 0.7660212471507180654 ) ) ;
#45388=ADVANCED_FACE ( 'NONE', ( #50779 ), #37748, .F. ) ;
#45389=EDGE_CURVE ( 'NONE', #33376, #30431, #11873, .T. ) ;
#45390=LINE ( 'NONE', #6502, #35239 ) ;
#45391=DIRECTION ( 'NONE',  ( -0.005961354470445682716, -0.6427876096865404731, 0.7660212471507180654 ) ) ;
#45393=CARTESIAN_POINT ( 'NONE',  ( -21.59278666343760733, 5.467268677019012202, 14.24141207810885668 ) ) ;
#45394=CARTESIAN_POINT ( 'NONE',  ( -21.42872037518206696, -2.784623065533158304, 9.575615298689720944 ) ) ;
#45395=FACE_OUTER_BOUND ( 'NONE', #51595, .T. ) ;
#45396=CARTESIAN_POINT ( 'NONE',  ( -15.91085239395617634, -0.1191753592594211320, 5.904584430724759692 ) ) ;
#45397=DIRECTION ( 'NONE',  ( 0.000000000000000000, -0.000000000000000000, -1.000000000000000000 ) ) ;
#45398=VECTOR ( 'NONE', #1160, 999.9999999999998863 ) ;
#45399=LINE ( 'NONE', #31539, #26414 ) ;
#45400=DIRECTION ( 'NONE',  ( -0.5449076811759708816, 0.6444004775717707689, 0.5364919789714475140 ) ) ;
#45401=LINE ( 'NONE', #6513, #44061 ) ;
#45402=CARTESIAN_POINT ( 'NONE',  ( -18.23586646982717951, 4.333955019861511992, 3.627085705124660997 ) ) ;
#45403=EDGE_CURVE ( 'NONE', #6183, #2694, #34041, .T. ) ;
#45404=ORIENTED_EDGE ( 'NONE', *, *, #22246, .T. ) ;
#45405=AXIS2_PLACEMENT_3D ( 'NONE', #15940, #46293, #8249 ) ;
#45406=LINE ( 'NONE', #37174, #33976 ) ;
#45408=CARTESIAN_POINT ( 'NONE',  ( 2.072287782118878319, 0.000000000000000000, -2.950529333540147015 ) ) ;
#45409=PLANE ( 'NONE',  #31267 ) ;
#45410=ORIENTED_EDGE ( 'NONE', *, *, #37111, .T. ) ;
#45411=PLANE ( 'NONE',  #42200 ) ;
#45412=ORIENTED_EDGE ( 'NONE', *, *, #10507, .T. ) ;
#45413=FACE_OUTER_BOUND ( 'NONE', #46788, .T. ) ;
#45414=ORIENTED_EDGE ( 'NONE', *, *, #5917, .F. ) ;
#45415=ORIENTED_EDGE ( 'NONE', *, *, #34688, .F. ) ;
#45416=ORIENTED_EDGE ( 'NONE', *, *, #42309, .F. ) ;
#45417=CARTESIAN_POINT ( 'NONE',  ( -22.40634380310664397, 0.000000000000000000, 5.584705972946605534 ) ) ;
#45419=CARTESIAN_POINT ( 'NONE',  ( -17.75008747281315280, -0.1166911823299055240, 3.676363194284736124 ) ) ;
#45420=VECTOR ( 'NONE', #8474, 999.9999999999998863 ) ;
#45421=AXIS2_PLACEMENT_3D ( 'NONE', #50457, #40818, #11263 ) ;
#45423=EDGE_CURVE ( 'NONE', #11772, #36118, #47089, .T. ) ;
#45424=EDGE_LOOP ( 'NONE', ( #24789, #21375, #37074, #27151 ) ) ;
#45425=LINE ( 'NONE', #20138, #28202 ) ;
#45426=EDGE_LOOP ( 'NONE', ( #584, #19641, #18352, #21215 ) ) ;
#45427=CARTESIAN_POINT ( 'NONE',  ( -16.74090741521495929, 0.000000000000000000, 5.998127778728137294 ) ) ;
#45428=ORIENTED_EDGE ( 'NONE', *, *, #34854, .T. ) ;
#45429=DIRECTION ( 'NONE',  ( 0.005961354470445682716, -0.6427876096865404731, -0.7660212471507180654 ) ) ;
#45430=FACE_OUTER_BOUND ( 'NONE', #49774, .T. ) ;
#45431=EDGE_CURVE ( 'NONE', #52348, #39606, #15571, .T. ) ;
#45432=ORIENTED_EDGE ( 'NONE', *, *, #1140, .F. ) ;
#45433=VECTOR ( 'NONE', #41417, 1000.000000000000114 ) ;
#45436=EDGE_CURVE ( 'NONE', #18658, #1854, #51057, .T. ) ;
#45437=AXIS2_PLACEMENT_3D ( 'NONE', #53385, #19847, #54464 ) ;
#45438=DIRECTION ( 'NONE',  ( 0.007781995580012662783, 0.000000000000000000, -0.9999697198139514409 ) ) ;
#45439=ORIENTED_EDGE ( 'NONE', *, *, #8058, .T. ) ;
#45440=CARTESIAN_POINT ( 'NONE',  ( -14.00280974873554030, 0.000000000000000000, 12.40921378708904044 ) ) ;
#45441=CARTESIAN_POINT ( 'NONE',  ( -22.40556560354864146, -0.1191753592594197858, 5.484709000965211523 ) ) ;
#45442=CARTESIAN_POINT ( 'NONE',  ( -15.40103151951671734, 0.000000000000000000, 12.95233060667165681 ) ) ;
#45443=EDGE_CURVE ( 'NONE', #38354, #55994, #46232, .T. ) ;
#45444=ORIENTED_EDGE ( 'NONE', *, *, #43077, .T. ) ;
#45445=EDGE_CURVE ( 'NONE', #24462, #41178, #32904, .T. ) ;
#45446=DIRECTION ( 'NONE',  ( 0.000000000000000000, -0.000000000000000000, -1.000000000000000000 ) ) ;
#45447=DIRECTION ( 'NONE',  ( -0.7660212471507179544, -0.6427876096865405842, -0.005961354470445141482 ) ) ;
#45448=DIRECTION ( 'NONE',  ( 0.005961354470445682716, -0.6427876096865404731, -0.7660212471507180654 ) ) ;
#45449=DIRECTION ( 'NONE',  ( 0.005002170337468016433, -0.7660444431189770143, -0.6427681459581293666 ) ) ;
#45450=DIRECTION ( 'NONE',  ( -0.9999697198139514409, -0.000000000000000000, -0.007781995580013368816 ) ) ;
#45451=EDGE_CURVE ( 'NONE', #40926, #50934, #34326, .T. ) ;
#45452=DIRECTION ( 'NONE',  ( 0.5364919789714477361, 0.6444004775717706579, 0.5449076811759711036 ) ) ;
#45454=ORIENTED_EDGE ( 'NONE', *, *, #31253, .T. ) ;
#45455=DIRECTION ( 'NONE',  ( -0.005961354470445682716, -0.6427876096865404731, 0.7660212471507180654 ) ) ;
#45456=LINE ( 'NONE', #19643, #37668 ) ;
#45458=ORIENTED_EDGE ( 'NONE', *, *, #39415, .T. ) ;
#45459=PLANE ( 'NONE',  #50129 ) ;
#45460=DIRECTION ( 'NONE',  ( 0.5449076811759707706, 0.6444004775717708799, -0.5364919789714476250 ) ) ;
#45461=EDGE_CURVE ( 'NONE', #29027, #46912, #34583, .T. ) ;
#45462=AXIS2_PLACEMENT_3D ( 'NONE', #21483, #26030, #12941 ) ;
#45463=VECTOR ( 'NONE', #30672, 1000.000000000000114 ) ;
#45464=CARTESIAN_POINT ( 'NONE',  ( -18.65485795953289028, -2.298917212465660054, 4.054153975076401295 ) ) ;
#45465=DIRECTION ( 'NONE',  ( -0.7660212471507179544, -0.6427876096865405842, -0.005961354470445141482 ) ) ;
#45466=FACE_OUTER_BOUND ( 'NONE', #40570, .T. ) ;
#45467=EDGE_CURVE ( 'NONE', #22414, #51971, #5070, .T. ) ;
#45468=VERTEX_POINT ( 'NONE', #17554 ) ;
#45469=VECTOR ( 'NONE', #22567, 999.9999999999998863 ) ;
#45470=ORIENTED_EDGE ( 'NONE', *, *, #28773, .F. ) ;
#45471=PLANE ( 'NONE',  #53129 ) ;
#45472=LINE ( 'NONE', #5759, #32049 ) ;
#45473=ORIENTED_EDGE ( 'NONE', *, *, #52470, .T. ) ;
#45474=LINE ( 'NONE', #23904, #38551 ) ;
#45475=ORIENTED_EDGE ( 'NONE', *, *, #37584, .F. ) ;
#45476=DIRECTION ( 'NONE',  ( -0.7660212471507179544, -0.6427876096865405842, -0.005961354470445141482 ) ) ;
#45477=VECTOR ( 'NONE', #26960, 1000.000000000000000 ) ;
#45478=ORIENTED_EDGE ( 'NONE', *, *, #23129, .T. ) ;
#45479=ORIENTED_EDGE ( 'NONE', *, *, #49650, .F. ) ;
#45480=CARTESIAN_POINT ( 'NONE',  ( -15.06668613446144356, 2.229229656569007734, 2.463220195587470407 ) ) ;
#45481=DIRECTION ( 'NONE',  ( -0.5449076811759708816, 0.6444004775717707689, 0.5364919789714475140 ) ) ;
#45482=CARTESIAN_POINT ( 'NONE',  ( -11.24149099750305858, -0.1191753592594186895, 2.986265922342736356 ) ) ;
#45483=ORIENTED_EDGE ( 'NONE', *, *, #45231, .T. ) ;
#45484=LINE ( 'NONE', #49500, #12039 ) ;
#45485=EDGE_CURVE ( 'NONE', #35767, #22808, #21552, .T. ) ;
#45486=ORIENTED_EDGE ( 'NONE', *, *, #21152, .F. ) ;
#45487=ORIENTED_EDGE ( 'NONE', *, *, #18134, .T. ) ;
#45488=ORIENTED_EDGE ( 'NONE', *, *, #39448, .F. ) ;
#45489=CARTESIAN_POINT ( 'NONE',  ( -17.59803301417029076, -3.756034771668160577, 9.681898340685158644 ) ) ;
#45490=ORIENTED_EDGE ( 'NONE', *, *, #11508, .T. ) ;
#45491=DIRECTION ( 'NONE',  ( 0.005961354470445682716, -0.6427876096865404731, -0.7660212471507180654 ) ) ;
#45492=ORIENTED_EDGE ( 'NONE', *, *, #9103, .T. ) ;
#45493=CARTESIAN_POINT ( 'NONE',  ( -8.509919637592204822, -0.1191753592594197858, 10.23596830920056711 ) ) ;
#45494=DIRECTION ( 'NONE',  ( 0.005002170337468016433, -0.7660444431189770143, -0.6427681459581293666 ) ) ;
#45495=VECTOR ( 'NONE', #47289, 999.9999999999998863 ) ;
#45496=AXIS2_PLACEMENT_3D ( 'NONE', #13422, #5187, #4599 ) ;
#45497=ORIENTED_EDGE ( 'NONE', *, *, #13209, .F. ) ;
#45498=LINE ( 'NONE', #6617, #49491 ) ;
#45499=VERTEX_POINT ( 'NONE', #30640 ) ;
#45500=EDGE_CURVE ( 'NONE', #48900, #20306, #30884, .T. ) ;
#45501=LINE ( 'NONE', #11148, #1977 ) ;
#45502=CARTESIAN_POINT ( 'NONE',  ( -14.46888367232926420, 0.000000000000000000, 12.59025272694991315 ) ) ;
#45503=VECTOR ( 'NONE', #35120, 1000.000000000000227 ) ;
#45504=DIRECTION ( 'NONE',  ( 0.6427681459581294776, -0.7660444431189769032, 0.005002170337467562802 ) ) ;
#45505=CARTESIAN_POINT ( 'NONE',  ( -19.10263103866113354, 2.553033558614007603, 8.491394756296369195 ) ) ;
#45506=CARTESIAN_POINT ( 'NONE',  ( -12.48530657876094985, 3.038739411681508518, 1.434697112697735255 ) ) ;
#45507=DIRECTION ( 'NONE',  ( -0.6427681459581293666, -0.7660444431189770143, -0.005002170337467561935 ) ) ;
#45509=ORIENTED_EDGE ( 'NONE', *, *, #4451, .F. ) ;
#45510=VERTEX_POINT ( 'NONE', #30054 ) ;
#45511=EDGE_CURVE ( 'NONE', #41874, #13391, #47941, .T. ) ;
#45513=LINE ( 'NONE', #3207, #48462 ) ;
#45514=VECTOR ( 'NONE', #45948, 999.9999999999998863 ) ;
#45515=CARTESIAN_POINT ( 'NONE',  ( -11.24723910451362485, -0.1191753592594192307, 3.724885328858265954 ) ) ;
#45516=VECTOR ( 'NONE', #20221, 1000.000000000000000 ) ;
#45517=ADVANCED_FACE ( 'NONE', ( #39128 ), #8783, .F. ) ;
#45518=LINE ( 'NONE', #23412, #17927 ) ;
#45519=CARTESIAN_POINT ( 'NONE',  ( -18.12463954610636563, 0.000000000000000000, 4.679356989688026935 ) ) ;
#45521=CARTESIAN_POINT ( 'NONE',  ( -15.98995279184259388, 0.000000000000000000, 3.218641336381011353 ) ) ;
#45522=DIRECTION ( 'NONE',  ( 0.000000000000000000, -0.000000000000000000, -1.000000000000000000 ) ) ;
#45523=EDGE_LOOP ( 'NONE', ( #20623, #49074, #20192, #35443 ) ) ;
#45524=LINE ( 'NONE', #29055, #6647 ) ;
#45525=DIRECTION ( 'NONE',  ( -0.7660212471507179544, -0.6427876096865405842, -0.005961354470445141482 ) ) ;
#45526=VERTEX_POINT ( 'NONE', #12732 ) ;
#45527=EDGE_CURVE ( 'NONE', #873, #26892, #43401, .T. ) ;
#45529=FACE_OUTER_BOUND ( 'NONE', #26270, .T. ) ;
#45530=CARTESIAN_POINT ( 'NONE',  ( -12.60458797795435615, 0.000000000000000000, 11.86609696750642229 ) ) ;
#45531=CARTESIAN_POINT ( 'NONE',  ( -20.54049170961573267, 0.000000000000000000, 4.660556269540326646 ) ) ;
#45533=EDGE_CURVE ( 'NONE', #43351, #17923, #4500, .T. ) ;
#45534=ORIENTED_EDGE ( 'NONE', *, *, #40906, .F. ) ;
#45535=ORIENTED_EDGE ( 'NONE', *, *, #18097, .F. ) ;
#45536=CARTESIAN_POINT ( 'NONE',  ( -12.33850799832341849, 0.000000000000000000, 11.68350162852954632 ) ) ;
#45537=CARTESIAN_POINT ( 'NONE',  ( -9.962725746045613562, 0.000000000000000000, 4.942880946358983785 ) ) ;
#45538=VECTOR ( 'NONE', #3065, 1000.000000000000000 ) ;
#45539=DIRECTION ( 'NONE',  ( -0.3620778797217457656, 0.000000000000000000, -0.9321478471874539151 ) ) ;
#45540=VECTOR ( 'NONE', #43806, 999.9999999999998863 ) ;
#45541=CARTESIAN_POINT ( 'NONE',  ( -19.59569683186026268, 0.000000000000000000, 14.58168106541950948 ) ) ;
#45543=CARTESIAN_POINT ( 'NONE',  ( -14.48163787323972684, -3.432230869623162928, 2.396974931197724423 ) ) ;
#45544=DIRECTION ( 'NONE',  ( 0.007781995580012663651, 0.000000000000000000, -0.9999697198139515519 ) ) ;
#45545=ORIENTED_EDGE ( 'NONE', *, *, #43466, .F. ) ;
#45546=LINE ( 'NONE', #1823, #48289 ) ;
#45547=PLANE ( 'NONE',  #6036 ) ;
#45548=VECTOR ( 'NONE', #24335, 1000.000000000000227 ) ;
#45549=CARTESIAN_POINT ( 'NONE',  ( -15.03495456790438389, -0.1191753592594197858, 12.77051346725278158 ) ) ;
#45550=AXIS2_PLACEMENT_3D ( 'NONE', #40914, #33519, #45446 ) ;
#45551=ORIENTED_EDGE ( 'NONE', *, *, #19874, .F. ) ;
#45552=FACE_OUTER_BOUND ( 'NONE', #14937, .T. ) ;
#45553=PLANE ( 'NONE',  #36828 ) ;
#45554=EDGE_CURVE ( 'NONE', #11685, #9839, #34883, .T. ) ;
#45555=DIRECTION ( 'NONE',  ( 0.000000000000000000, -1.000000000000000000, 0.000000000000000000 ) ) ;
#45556=ORIENTED_EDGE ( 'NONE', *, *, #28012, .T. ) ;
#45557=CARTESIAN_POINT ( 'NONE',  ( -16.16356523649682231, -2.622721114510657703, 7.264741553452760847 ) ) ;
#45558=AXIS2_PLACEMENT_3D ( 'NONE', #25156, #34242, #25412 ) ;
#45559=EDGE_CURVE ( 'NONE', #36400, #26435, #18110, .T. ) ;
#45560=EDGE_LOOP ( 'NONE', ( #22947, #13146, #18332, #20712 ) ) ;
#45561=ORIENTED_EDGE ( 'NONE', *, *, #12956, .F. ) ;
#45562=ORIENTED_EDGE ( 'NONE', *, *, #26889, .T. ) ;
#45563=EDGE_CURVE ( 'NONE', #45990, #29528, #52202, .T. ) ;
#45564=ORIENTED_EDGE ( 'NONE', *, *, #19239, .T. ) ;
#45566=VERTEX_POINT ( 'NONE', #48492 ) ;
#45567=PLANE ( 'NONE',  #23875 ) ;
#45568=ORIENTED_EDGE ( 'NONE', *, *, #31886, .F. ) ;
#45569=ADVANCED_FACE ( 'NONE', ( #39424 ), #21247, .F. ) ;
#45570=EDGE_CURVE ( 'NONE', #16052, #43303, #17858, .T. ) ;
#45572=ORIENTED_EDGE ( 'NONE', *, *, #29591, .F. ) ;
#45573=DIRECTION ( 'NONE',  ( 0.5364919789714477361, 0.6444004775717706579, 0.5449076811759711036 ) ) ;
#45575=VECTOR ( 'NONE', #50653, 999.9999999999998863 ) ;
#45576=ORIENTED_EDGE ( 'NONE', *, *, #47172, .T. ) ;
#45577=ORIENTED_EDGE ( 'NONE', *, *, #27782, .T. ) ;
#45578=PLANE ( 'NONE',  #8543 ) ;
#45579=CARTESIAN_POINT ( 'NONE',  ( -10.00813838035478298, 0.000000000000000000, 10.77830692922518452 ) ) ;
#45580=PLANE ( 'NONE',  #44102 ) ;
#45581=CARTESIAN_POINT ( 'NONE',  ( -13.08330893211609869, 0.000000000000000000, 1.763933231766363630 ) ) ;
#45582=VECTOR ( 'NONE', #32771, 999.9999999999998863 ) ;
#45583=ORIENTED_EDGE ( 'NONE', *, *, #12676, .F. ) ;
#45584=CARTESIAN_POINT ( 'NONE',  ( -11.21979143729918960, -0.1191753592594197858, 1.139774444304266554 ) ) ;
#45585=EDGE_LOOP ( 'NONE', ( #15495, #50936, #4205, #20708 ) ) ;
#45586=VECTOR ( 'NONE', #49111, 1000.000000000000227 ) ;
#45587=VECTOR ( 'NONE', #18366, 1000.000000000000000 ) ;
#45588=ORIENTED_EDGE ( 'NONE', *, *, #11401, .F. ) ;
#45590=FACE_OUTER_BOUND ( 'NONE', #17318, .T. ) ;
#45591=EDGE_CURVE ( 'NONE', #5666, #18978, #26629, .T. ) ;
#45593=VECTOR ( 'NONE', #48732, 999.9999999999998863 ) ;
#45595=CARTESIAN_POINT ( 'NONE',  ( -13.13096402496594983, 3.200641362704009119, 7.234631225313592928 ) ) ;
#45596=EDGE_CURVE ( 'NONE', #51597, #34934, #14691, .T. ) ;
#45597=DIRECTION ( 'NONE',  ( -0.005002170337468016433, -0.7660444431189770143, 0.6427681459581293666 ) ) ;
#45598=LINE ( 'NONE', #36833, #1392 ) ;
#45599=VERTEX_POINT ( 'NONE', #41081 ) ;
#45600=LINE ( 'NONE', #24034, #3876 ) ;
#45601=ORIENTED_EDGE ( 'NONE', *, *, #37510, .F. ) ;
#45602=ADVANCED_FACE ( 'NONE', ( #32312 ), #18687, .F. ) ;
#45603=DIRECTION ( 'NONE',  ( 0.7660212471507180654, -0.6427876096865404731, 0.005961354470445141482 ) ) ;
#45604=PLANE ( 'NONE',  #37778 ) ;
#45605=CARTESIAN_POINT ( 'NONE',  ( -10.24173896645031867, 0.000000000000000000, 6.787369949995797569 ) ) ;
#45606=VECTOR ( 'NONE', #8519, 999.9999999999998863 ) ;
#45608=VECTOR ( 'NONE', #50173, 1000.000000000000114 ) ;
#45609=DIRECTION ( 'NONE',  ( -0.5364919789714478471, 0.6444004775717705469, -0.5449076811759709926 ) ) ;
#45610=ORIENTED_EDGE ( 'NONE', *, *, #21050, .T. ) ;
#45611=CARTESIAN_POINT ( 'NONE',  ( -11.15951654611136057, 0.000000000000000000, 5.302899313428722117 ) ) ;
#45612=FACE_OUTER_BOUND ( 'NONE', #51926, .T. ) ;
#45613=DIRECTION ( 'NONE',  ( 0.005002170337468016433, -0.7660444431189770143, -0.6427681459581293666 ) ) ;
#45614=VECTOR ( 'NONE', #31204, 1000.000000000000114 ) ;
#45615=DIRECTION ( 'NONE',  ( 0.000000000000000000, 1.000000000000000000, 0.000000000000000000 ) ) ;
#45616=CARTESIAN_POINT ( 'NONE',  ( -29.93654370153088706, -1.000000000000000000, 22.35628214185738116 ) ) ;
#45617=AXIS2_PLACEMENT_3D ( 'NONE', #36984, #24451, #54279 ) ;
#45618=LINE ( 'NONE', #28040, #23660 ) ;
#45619=CARTESIAN_POINT ( 'NONE',  ( -10.82493838822988153, -0.1941918491731542684, 1.079899066930483320 ) ) ;
#45620=CARTESIAN_POINT ( 'NONE',  ( -17.26532721389163072, 0.000000000000000000, 13.67648636611514590 ) ) ;
#45621=AXIS2_PLACEMENT_3D ( 'NONE', #51702, #9, #4851 ) ;
#45622=FACE_OUTER_BOUND ( 'NONE', #22030, .T. ) ;
#45623=VECTOR ( 'NONE', #17478, 1000.000000000000000 ) ;
#45624=VECTOR ( 'NONE', #47989, 999.9999999999998863 ) ;
#45625=EDGE_LOOP ( 'NONE', ( #19796, #45230, #39826, #52756 ) ) ;
#45626=VECTOR ( 'NONE', #5692, 999.9999999999998863 ) ;
#45627=EDGE_LOOP ( 'NONE', ( #17152, #15672, #48928, #12601 ) ) ;
#45628=VERTEX_POINT ( 'NONE', #36852 ) ;
#45629=AXIS2_PLACEMENT_3D ( 'NONE', #6574, #20756, #38071 ) ;
#45630=ORIENTED_EDGE ( 'NONE', *, *, #52659, .T. ) ;
#45631=ORIENTED_EDGE ( 'NONE', *, *, #53852, .F. ) ;
#45632=DIRECTION ( 'NONE',  ( 0.007781995580012663651, -3.146120232559066537E-19, -0.9999697198139514409 ) ) ;
#45633=CARTESIAN_POINT ( 'NONE',  ( -15.45483765763093764, -0.1191753592594179401, 7.016129452266057775 ) ) ;
#45634=ADVANCED_FACE ( 'NONE', ( #19505 ), #14154, .F. ) ;
#45635=EDGE_CURVE ( 'NONE', #13109, #4654, #10448, .T. ) ;
#45637=LINE ( 'NONE', #41404, #45765 ) ;
#45638=EDGE_LOOP ( 'NONE', ( #37590, #48473, #13611, #46776 ) ) ;
#45639=ADVANCED_FACE ( 'NONE', ( #44793 ), #31741, .F. ) ;
#45640=ORIENTED_EDGE ( 'NONE', *, *, #51842, .T. ) ;
#45642=DIRECTION ( 'NONE',  ( 0.007781995580012662783, 0.000000000000000000, -0.9999697198139514409 ) ) ;
#45643=LINE ( 'NONE', #6763, #28663 ) ;
#45644=EDGE_LOOP ( 'NONE', ( #5691, #12148, #37966, #7351 ) ) ;
#45645=LINE ( 'NONE', #45369, #29186 ) ;
#45646=VECTOR ( 'NONE', #14125, 1000.000000000000227 ) ;
#45647=DIRECTION ( 'NONE',  ( 0.6427681459581294776, -0.7660444431189769032, 0.005002170337467562802 ) ) ;
#45648=LINE ( 'NONE', #20926, #52019 ) ;
#45649=VECTOR ( 'NONE', #42900, 999.9999999999998863 ) ;
#45651=PLANE ( 'NONE',  #51693 ) ;
#45652=LINE ( 'NONE', #41418, #27865 ) ;
#45654=FACE_OUTER_BOUND ( 'NONE', #748, .T. ) ;
#45655=CARTESIAN_POINT ( 'NONE',  ( -17.76365187430995718, -0.1191753592594196748, 5.151501377137190474 ) ) ;
#45656=EDGE_CURVE ( 'NONE', #9765, #34966, #22655, .T. ) ;
#45657=AXIS2_PLACEMENT_3D ( 'NONE', #5552, #27712, #39361 ) ;
#45658=DIRECTION ( 'NONE',  ( 0.005002170337468016433, -0.7660444431189770143, -0.6427681459581293666 ) ) ;
#45659=EDGE_LOOP ( 'NONE', ( #49186, #15025, #14615, #28842 ) ) ;
#45660=CARTESIAN_POINT ( 'NONE',  ( -10.00813838035478298, 0.000000000000000000, 10.77830692922518452 ) ) ;
#45661=ORIENTED_EDGE ( 'NONE', *, *, #5348, .F. ) ;
#45662=VECTOR ( 'NONE', #28778, 1000.000000000000227 ) ;
#45663=VECTOR ( 'NONE', #22391, 1000.000000000000227 ) ;
#45664=ADVANCED_FACE ( 'NONE', ( #39967 ), #23757, .F. ) ;
#45665=CARTESIAN_POINT ( 'NONE',  ( -26.13337879274045505, 0.000000000000000000, 6.833023547870798353 ) ) ;
#45666=LINE ( 'NONE', #6237, #21407 ) ;
#45667=DIRECTION ( 'NONE',  ( 0.005961354470445682716, -0.6427876096865404731, -0.7660212471507180654 ) ) ;
#45668=FACE_OUTER_BOUND ( 'NONE', #50305, .T. ) ;
#45669=DIRECTION ( 'NONE',  ( 0.005002170337468016433, -0.7660444431189770143, -0.6427681459581293666 ) ) ;
#45670=EDGE_CURVE ( 'NONE', #42137, #713, #53859, .T. ) ;
#45671=AXIS2_PLACEMENT_3D ( 'NONE', #48444, #42568, #55342 ) ;
#45673=AXIS2_PLACEMENT_3D ( 'NONE', #40314, #19012, #27837 ) ;
#45674=LINE ( 'NONE', #31533, #19268 ) ;
#45675=CARTESIAN_POINT ( 'NONE',  ( -15.56842669758074571, 0.000000000000000000, 8.761902797015491018 ) ) ;
#45676=PLANE ( 'NONE',  #23131 ) ;
#45677=CARTESIAN_POINT ( 'NONE',  ( -20.54126990917373519, -0.1191753592594197858, 4.760553241521720658 ) ) ;
#45678=CARTESIAN_POINT ( 'NONE',  ( -9.858694684501937644, -9.497542338669614281, 0.6110782424775126342 ) ) ;
#45679=CARTESIAN_POINT ( 'NONE',  ( -19.45503627000849889, -1.000000000000000000, 7.556996783084074742 ) ) ;
#45680=FACE_OUTER_BOUND ( 'NONE', #31268, .T. ) ;
#45681=DIRECTION ( 'NONE',  ( -0.5364919789714478471, 0.6444004775717705469, -0.5449076811759709926 ) ) ;
#45682=CARTESIAN_POINT ( 'NONE',  ( -20.54049170961573267, 0.000000000000000000, 4.660556269540326646 ) ) ;
#45683=ORIENTED_EDGE ( 'NONE', *, *, #32776, .T. ) ;
#45684=CARTESIAN_POINT ( 'NONE',  ( -18.39746900504187010, 0.000000000000000000, 14.03700784672088808 ) ) ;
#45685=ORIENTED_EDGE ( 'NONE', *, *, #12676, .T. ) ;
#45687=DIRECTION ( 'NONE',  ( -0.5449076811759708816, 0.6444004775717707689, 0.5364919789714475140 ) ) ;
#45688=CARTESIAN_POINT ( 'NONE',  ( -16.06709938707323460, 0.000000000000000000, 13.13181314741652628 ) ) ;
#45689=VECTOR ( 'NONE', #30547, 1000.000000000000000 ) ;
#45690=VERTEX_POINT ( 'NONE', #53037 ) ;
#45691=VECTOR ( 'NONE', #52176, 1000.000000000000114 ) ;
#45692=ORIENTED_EDGE ( 'NONE', *, *, #50006, .F. ) ;
#45693=PLANE ( 'NONE',  #26581 ) ;
#45695=ORIENTED_EDGE ( 'NONE', *, *, #23918, .F. ) ;
#45696=EDGE_LOOP ( 'NONE', ( #23106, #14788, #3731, #25673 ) ) ;
#45697=CARTESIAN_POINT ( 'NONE',  ( -17.41416041653468127, 0.000000000000000000, 7.100884577617416760 ) ) ;
#45698=VECTOR ( 'NONE', #9467, 999.9999999999998863 ) ;
#45699=PLANE ( 'NONE',  #41359 ) ;
#45700=DIRECTION ( 'NONE',  ( -0.9999697198139514409, -0.000000000000000000, -0.007781995580013368816 ) ) ;
#45701=AXIS2_PLACEMENT_3D ( 'NONE', #36666, #49726, #10823 ) ;
#45702=ADVANCED_FACE ( 'NONE', ( #53336 ), #9889, .F. ) ;
#45703=EDGE_LOOP ( 'NONE', ( #32480, #1844, #37401, #17025 ) ) ;
#45704=VERTEX_POINT ( 'NONE', #27468 ) ;
#45705=EDGE_CURVE ( 'NONE', #33893, #4507, #1637, .T. ) ;
#45706=EDGE_CURVE ( 'NONE', #40865, #40267, #49334, .T. ) ;
#45707=VECTOR ( 'NONE', #22657, 1000.000000000000227 ) ;
#45708=AXIS2_PLACEMENT_3D ( 'NONE', #17198, #25184, #11809 ) ;
#45709=DIRECTION ( 'NONE',  ( -0.005002170337468016433, -0.7660444431189770143, 0.6427681459581293666 ) ) ;
#45710=CARTESIAN_POINT ( 'NONE',  ( -16.81190032086591302, 0.000000000000000000, 3.212244750653343583 ) ) ;
#45711=ORIENTED_EDGE ( 'NONE', *, *, #55792, .T. ) ;
#45712=DIRECTION ( 'NONE',  ( 0.7660212471507180654, -0.6427876096865404731, 0.005961354470445141482 ) ) ;
#45713=ORIENTED_EDGE ( 'NONE', *, *, #38698, .F. ) ;
#45714=CARTESIAN_POINT ( 'NONE',  ( -15.22089569151837196, 4.010151117816510791, 9.374975078733013945 ) ) ;
#45715=DIRECTION ( 'NONE',  ( 0.5449076811759707706, 0.6444004775717708799, -0.5364919789714476250 ) ) ;
#45716=ORIENTED_EDGE ( 'NONE', *, *, #45101, .F. ) ;
#45717=FACE_OUTER_BOUND ( 'NONE', #10996, .T. ) ;
#45718=VECTOR ( 'NONE', #16064, 1000.000000000000114 ) ;
#45719=DIRECTION ( 'NONE',  ( 0.5364919789714477361, 0.6444004775717706579, 0.5449076811759711036 ) ) ;
#45720=EDGE_LOOP ( 'NONE', ( #37768, #52827, #32409, #23103 ) ) ;
#45721=DIRECTION ( 'NONE',  ( -0.7660212471507179544, -0.6427876096865405842, -0.005961354470445141482 ) ) ;
#45723=AXIS2_PLACEMENT_3D ( 'NONE', #29621, #38389, #20790 ) ;
#45724=LINE ( 'NONE', #33259, #50079 ) ;
#45725=ORIENTED_EDGE ( 'NONE', *, *, #24450, .T. ) ;
#45726=VECTOR ( 'NONE', #48046, 999.9999999999998863 ) ;
#45727=LINE ( 'NONE', #46566, #9281 ) ;
#45728=PLANE ( 'NONE',  #27846 ) ;
#45729=LINE ( 'NONE', #42028, #21260 ) ;
#45731=FACE_OUTER_BOUND ( 'NONE', #54502, .T. ) ;
#45732=EDGE_CURVE ( 'NONE', #16069, #17592, #14978, .T. ) ;
#45733=DIRECTION ( 'NONE',  ( 0.005002170337468016433, -0.7660444431189770143, -0.6427681459581293666 ) ) ;
#45734=CARTESIAN_POINT ( 'NONE',  ( -16.24565193759350379, -1.651309408375659871, 3.138998618723810363 ) ) ;
#45736=VECTOR ( 'NONE', #39881, 1000.000000000000227 ) ;
#45737=EDGE_LOOP ( 'NONE', ( #23741, #56068, #11831, #4373 ) ) ;
#45738=EDGE_CURVE ( 'NONE', #17790, #32862, #29428, .T. ) ;
#45739=LINE ( 'NONE', #37503, #32246 ) ;
#45741=ORIENTED_EDGE ( 'NONE', *, *, #21133, .T. ) ;
#45743=DIRECTION ( 'NONE',  ( 0.6427681459581294776, -0.7660444431189769032, 0.005002170337467562802 ) ) ;
#45744=FACE_OUTER_BOUND ( 'NONE', #10289, .T. ) ;
#45745=ADVANCED_FACE ( 'NONE', ( #7027 ), #33416, .F. ) ;
#45746=AXIS2_PLACEMENT_3D ( 'NONE', #36895, #45376, #11015 ) ;
#45747=ADVANCED_FACE ( 'NONE', ( #16347 ), #51293, .F. ) ;
#45748=CARTESIAN_POINT ( 'NONE',  ( -15.96710241509184058, -0.1191753592594218814, 13.13259134697452879 ) ) ;
#45749=DIRECTION ( 'NONE',  ( 0.005002170337468016433, -0.7660444431189770143, -0.6427681459581293666 ) ) ;
#45750=CARTESIAN_POINT ( 'NONE',  ( -9.936859264498066224, 0.000000000000000000, 1.619093617039103039 ) ) ;
#45751=ORIENTED_EDGE ( 'NONE', *, *, #54635, .F. ) ;
#45753=VECTOR ( 'NONE', #26481, 999.9999999999998863 ) ;
#45754=ORIENTED_EDGE ( 'NONE', *, *, #32289, .F. ) ;
#45756=LINE ( 'NONE', #54841, #14825 ) ;
#45757=VERTEX_POINT ( 'NONE', #41381 ) ;
#45759=ORIENTED_EDGE ( 'NONE', *, *, #2887, .T. ) ;
#45760=PLANE ( 'NONE',  #9310 ) ;
#45761=EDGE_CURVE ( 'NONE', #47810, #9986, #33674, .T. ) ;
#45762=VECTOR ( 'NONE', #15044, 999.9999999999998863 ) ;
#45763=ORIENTED_EDGE ( 'NONE', *, *, #27439, .F. ) ;
#45765=VECTOR ( 'NONE', #2490, 1000.000000000000000 ) ;
#45766=FACE_OUTER_BOUND ( 'NONE', #35272, .T. ) ;
#45767=ADVANCED_FACE ( 'NONE', ( #15797 ), #50453, .F. ) ;
#45768=DIRECTION ( 'NONE',  ( 0.5364919789714477361, 0.6444004775717706579, 0.5449076811759711036 ) ) ;
#45769=VECTOR ( 'NONE', #22577, 999.9999999999998863 ) ;
#45771=ORIENTED_EDGE ( 'NONE', *, *, #300, .T. ) ;
#45772=DIRECTION ( 'NONE',  ( 0.5364919789714477361, 0.6444004775717706579, 0.5449076811759711036 ) ) ;
#45773=EDGE_CURVE ( 'NONE', #34236, #43196, #7868, .T. ) ;
#45774=VECTOR ( 'NONE', #18731, 1000.000000000000227 ) ;
#45775=EDGE_LOOP ( 'NONE', ( #1532, #49863, #47119, #33455 ) ) ;
#45776=EDGE_CURVE ( 'NONE', #8547, #11287, #16637, .T. ) ;
#45777=ORIENTED_EDGE ( 'NONE', *, *, #39853, .T. ) ;
#45778=ORIENTED_EDGE ( 'NONE', *, *, #19125, .F. ) ;
#45779=VECTOR ( 'NONE', #35330, 1000.000000000000000 ) ;
#45780=DIRECTION ( 'NONE',  ( -0.9999697198139514409, -0.000000000000000000, -0.007781995580013368816 ) ) ;
#45781=VECTOR ( 'NONE', #3695, 1000.000000000000227 ) ;
#45782=EDGE_LOOP ( 'NONE', ( #53869, #47355, #47785, #46386 ) ) ;
#45783=VECTOR ( 'NONE', #23892, 1000.000000000000227 ) ;
#45784=AXIS2_PLACEMENT_3D ( 'NONE', #46321, #40776, #53543 ) ;
#45785=CARTESIAN_POINT ( 'NONE',  ( -32.65841372305263235, 0.000000000000000000, 9.367568705923016381 ) ) ;
#45786=ORIENTED_EDGE ( 'NONE', *, *, #1719, .T. ) ;
#45787=CARTESIAN_POINT ( 'NONE',  ( -18.39746900504187010, 0.000000000000000000, 14.03700784672088808 ) ) ;
#45788=FACE_OUTER_BOUND ( 'NONE', #5891, .T. ) ;
#45789=AXIS2_PLACEMENT_3D ( 'NONE', #39247, #4894, #22218 ) ;
#45790=EDGE_LOOP ( 'NONE', ( #39602, #42223, #7113 ) ) ;
#45791=PLANE ( 'NONE',  #15040 ) ;
#45792=VERTEX_POINT ( 'NONE', #54999 ) ;
#45793=EDGE_CURVE ( 'NONE', #16632, #16077, #28876, .T. ) ;
#45794=AXIS2_PLACEMENT_3D ( 'NONE', #39200, #14767, #32098 ) ;
#45795=DIRECTION ( 'NONE',  ( -0.005002170337468016433, -0.7660444431189770143, 0.6427681459581293666 ) ) ;
#45796=VECTOR ( 'NONE', #24560, 1000.000000000000000 ) ;
#45797=FACE_OUTER_BOUND ( 'NONE', #15223, .T. ) ;
#45798=CARTESIAN_POINT ( 'NONE',  ( -12.38392586161602260, -3.108426967578159061, 6.593727315006988832 ) ) ;
#45799=LINE ( 'NONE', #7452, #44746 ) ;
#45800=LINE ( 'NONE', #28779, #10601 ) ;
#45802=ORIENTED_EDGE ( 'NONE', *, *, #2442, .T. ) ;
#45803=ORIENTED_EDGE ( 'NONE', *, *, #11863, .F. ) ;
#45804=CARTESIAN_POINT ( 'NONE',  ( -18.19747506107908563, 0.000000000000000000, 14.03856424583689311 ) ) ;
#45805=PLANE ( 'NONE',  #5832 ) ;
#45806=DIRECTION ( 'NONE',  ( -0.5364919789714478471, 0.6444004775717705469, -0.5449076811759709926 ) ) ;
#45807=CARTESIAN_POINT ( 'NONE',  ( -13.33442604019040267, -2.622721114510660367, 1.977186495200478067 ) ) ;
#45808=AXIS2_PLACEMENT_3D ( 'NONE', #28810, #46112, #7217 ) ;
#45809=DIRECTION ( 'NONE',  ( 0.007781995580012662783, 0.000000000000000000, -0.9999697198139514409 ) ) ;
#45810=ORIENTED_EDGE ( 'NONE', *, *, #49426, .T. ) ;
#45811=AXIS2_PLACEMENT_3D ( 'NONE', #12694, #33696, #3605 ) ;
#45812=DIRECTION ( 'NONE',  ( -0.5364919789714478471, 0.6444004775717705469, -0.5449076811759709926 ) ) ;
#45813=CARTESIAN_POINT ( 'NONE',  ( -18.79657489303680507, 0.000000000000000000, 5.612798029282330070 ) ) ;
#45814=EDGE_LOOP ( 'NONE', ( #38659, #48801, #28394, #36581 ) ) ;
#45815=CARTESIAN_POINT ( 'NONE',  ( -12.33850799832341849, 0.000000000000000000, 11.68350162852954632 ) ) ;
#45816=FACE_OUTER_BOUND ( 'NONE', #26166, .T. ) ;
#45817=VECTOR ( 'NONE', #31150, 1000.000000000000114 ) ;
#45818=ORIENTED_EDGE ( 'NONE', *, *, #10341, .F. ) ;
#45819=PLANE ( 'NONE',  #42514 ) ;
#45820=LINE ( 'NONE', #2648, #50499 ) ;
#45821=EDGE_CURVE ( 'NONE', #46187, #23847, #25189, .T. ) ;
#45822=AXIS2_PLACEMENT_3D ( 'NONE', #8757, #22635, #52713 ) ;
#45823=CARTESIAN_POINT ( 'NONE',  ( -19.41483227295923797, -3.756034771668161909, 4.302864128261002286 ) ) ;
#45824=FACE_OUTER_BOUND ( 'NONE', #21171, .T. ) ;
#45825=CARTESIAN_POINT ( 'NONE',  ( -10.28842178966973897, 0.000000000000000000, 0.8776935365639153552 ) ) ;
#45826=ORIENTED_EDGE ( 'NONE', *, *, #19417, .T. ) ;
#45827=EDGE_CURVE ( 'NONE', #1558, #52378, #46175, .T. ) ;
#45828=AXIS2_PLACEMENT_3D ( 'NONE', #16190, #24165, #37789 ) ;
#45829=VECTOR ( 'NONE', #11446, 1000.000000000000114 ) ;
#45830=ORIENTED_EDGE ( 'NONE', *, *, #45043, .T. ) ;
#45832=DIRECTION ( 'NONE',  ( 0.9999697198139515519, 0.000000000000000000, 0.007781995580013368816 ) ) ;
#45834=VECTOR ( 'NONE', #32568, 1000.000000000000227 ) ;
#45835=EDGE_CURVE ( 'NONE', #19669, #45947, #38212, .T. ) ;
#45836=LINE ( 'NONE', #42132, #35711 ) ;
#45837=VECTOR ( 'NONE', #31504, 1000.000000000000114 ) ;
#45838=LINE ( 'NONE', #23975, #55516 ) ;
#45839=LINE ( 'NONE', #53518, #2209 ) ;
#45840=EDGE_LOOP ( 'NONE', ( #53203, #19160, #46988, #33665 ) ) ;
#45841=EDGE_CURVE ( 'NONE', #7759, #2042, #16094, .T. ) ;
#45843=ADVANCED_FACE ( 'NONE', ( #7278 ), #3004, .F. ) ;
#45844=AXIS2_PLACEMENT_3D ( 'NONE', #25131, #42437, #33910 ) ;
#45845=CARTESIAN_POINT ( 'NONE',  ( -15.72321562200438372, 5.143464774974011888, 11.43005398624366187 ) ) ;
#45846=VECTOR ( 'NONE', #28494, 1000.000000000000227 ) ;
#45847=DIRECTION ( 'NONE',  ( 0.000000000000000000, -1.000000000000000000, 0.000000000000000000 ) ) ;
#45848=EDGE_LOOP ( 'NONE', ( #41179, #48117, #8489, #53835 ) ) ;
#45849=PLANE ( 'NONE',  #7534 ) ;
#45850=EDGE_CURVE ( 'NONE', #14352, #54876, #42207, .T. ) ;
#45851=CARTESIAN_POINT ( 'NONE',  ( -18.62310398945015066, 3.686347215771511365, 3.798163987937305919 ) ) ;
#45852=DIRECTION ( 'NONE',  ( 0.000000000000000000, -0.000000000000000000, -1.000000000000000000 ) ) ;
#45853=VERTEX_POINT ( 'NONE', #37950 ) ;
#45854=FACE_OUTER_BOUND ( 'NONE', #16300, .T. ) ;
#45855=EDGE_CURVE ( 'NONE', #7829, #44519, #26449, .T. ) ;
#45856=EDGE_LOOP ( 'NONE', ( #7517, #19521, #30858, #1873 ) ) ;
#45857=EDGE_CURVE ( 'NONE', #33602, #46316, #6730, .T. ) ;
#45858=AXIS2_PLACEMENT_3D ( 'NONE', #25572, #26410, #12800 ) ;
#45859=ORIENTED_EDGE ( 'NONE', *, *, #47299, .T. ) ;
#45861=ORIENTED_EDGE ( 'NONE', *, *, #16662, .F. ) ;
#45862=AXIS2_PLACEMENT_3D ( 'NONE', #38935, #12801, #12245 ) ;
#45863=ORIENTED_EDGE ( 'NONE', *, *, #37393, .T. ) ;
#45865=VECTOR ( 'NONE', #34186, 1000.000000000000227 ) ;
#45866=ORIENTED_EDGE ( 'NONE', *, *, #27070, .T. ) ;
#45867=EDGE_CURVE ( 'NONE', #9132, #38515, #54410, .T. ) ;
#45868=EDGE_LOOP ( 'NONE', ( #43759, #39205, #17101, #52310 ) ) ;
#45869=CARTESIAN_POINT ( 'NONE',  ( 2.072287782118878319, 0.000000000000000000, -2.950529333540147015 ) ) ;
#45870=ORIENTED_EDGE ( 'NONE', *, *, #8182, .F. ) ;
#45871=VECTOR ( 'NONE', #48550, 1000.000000000000227 ) ;
#45873=ORIENTED_EDGE ( 'NONE', *, *, #22648, .F. ) ;
#45874=ADVANCED_FACE ( 'NONE', ( #26556 ), #47879, .F. ) ;
#45875=VECTOR ( 'NONE', #38266, 1000.000000000000114 ) ;
#45876=AXIS2_PLACEMENT_3D ( 'NONE', #14522, #10259, #5185 ) ;
#45877=CARTESIAN_POINT ( 'NONE',  ( -14.56888064431065821, -0.1191753592594197858, 12.58947452739191064 ) ) ;
#45879=DIRECTION ( 'NONE',  ( 0.9999697198139515519, 0.000000000000000000, 0.007781995580013368816 ) ) ;
#45880=CARTESIAN_POINT ( 'NONE',  ( -15.25049964999576524, 0.7721120973665037690, 4.072300582551036996 ) ) ;
#45881=VECTOR ( 'NONE', #14412, 999.9999999999998863 ) ;
#45882=LINE ( 'NONE', #50115, #13789 ) ;
#45883=ORIENTED_EDGE ( 'NONE', *, *, #23891, .F. ) ;
#45884=AXIS2_PLACEMENT_3D ( 'NONE', #272, #9092, #26401 ) ;
#45885=ORIENTED_EDGE ( 'NONE', *, *, #7006, .T. ) ;
#45886=VECTOR ( 'NONE', #15826, 999.9999999999998863 ) ;
#45887=LINE ( 'NONE', #7001, #24044 ) ;
#45888=CARTESIAN_POINT ( 'NONE',  ( -26.13415699229845757, -0.1191753592594197858, 6.933020519852192365 ) ) ;
#45889=AXIS2_PLACEMENT_3D ( 'NONE', #53727, #27334, #1514 ) ;
#45891=VECTOR ( 'NONE', #35714, 999.9999999999998863 ) ;
#45892=FACE_OUTER_BOUND ( 'NONE', #48091, .T. ) ;
#45894=PLANE ( 'NONE',  #8672 ) ;
#45895=ORIENTED_EDGE ( 'NONE', *, *, #19239, .F. ) ;
#45896=CARTESIAN_POINT ( 'NONE',  ( -30.79567442779373110, 0.000000000000000000, 8.843406890442315316 ) ) ;
#45897=ORIENTED_EDGE ( 'NONE', *, *, #27978, .F. ) ;
#45898=CARTESIAN_POINT ( 'NONE',  ( -15.54986472215976967, 0.000000000000000000, 6.376728818173926783 ) ) ;
#45899=CARTESIAN_POINT ( 'NONE',  ( -22.48440822228507585, -4.565544526780660917, 12.90847583326981507 ) ) ;
#45900=DIRECTION ( 'NONE',  ( 0.6427681459581294776, -0.7660444431189769032, 0.005002170337467562802 ) ) ;
#45901=EDGE_CURVE ( 'NONE', #26799, #3531, #52417, .T. ) ;
#45902=CARTESIAN_POINT ( 'NONE',  ( -13.96101589989143932, 4.172053068839010059, 9.151303665917755126 ) ) ;
#45903=CARTESIAN_POINT ( 'NONE',  ( -14.50544548941179102, -0.1191753592594190225, 4.438193352997728880 ) ) ;
#45904=VECTOR ( 'NONE', #12948, 999.9999999999998863 ) ;
#45905=EDGE_LOOP ( 'NONE', ( #13407, #47895, #14540, #43302 ) ) ;
#45907=PLANE ( 'NONE',  #36702 ) ;
#45908=DIRECTION ( 'NONE',  ( -0.005961354470445682716, -0.6427876096865404731, 0.7660212471507180654 ) ) ;
#45909=VECTOR ( 'NONE', #46354, 1000.000000000000114 ) ;
#45910=EDGE_CURVE ( 'NONE', #15181, #24601, #30271, .T. ) ;
#45912=DIRECTION ( 'NONE',  ( 0.007781995580012663651, 0.000000000000000000, -0.9999697198139515519 ) ) ;
#45913=AXIS2_PLACEMENT_3D ( 'NONE', #9757, #5757, #48649 ) ;
#45914=DIRECTION ( 'NONE',  ( 0.007781995580012663651, -3.146120232559066537E-19, -0.9999697198139514409 ) ) ;
#45915=DIRECTION ( 'NONE',  ( -0.005002170337468016433, -0.7660444431189770143, 0.6427681459581293666 ) ) ;
#45916=CARTESIAN_POINT ( 'NONE',  ( -27.06552663992790997, 0.000000000000000000, 7.195101427592543786 ) ) ;
#45917=EDGE_CURVE ( 'NONE', #608, #46062, #4440, .T. ) ;
#45918=VECTOR ( 'NONE', #24038, 999.9999999999998863 ) ;
#45919=CARTESIAN_POINT ( 'NONE',  ( -14.40910077049367821, 0.000000000000000000, 4.908278227794890647 ) ) ;
#45920=CARTESIAN_POINT ( 'NONE',  ( -24.27063949748155380, 0.000000000000000000, 6.308861732390097288 ) ) ;
#45921=ORIENTED_EDGE ( 'NONE', *, *, #41680, .F. ) ;
#45922=VECTOR ( 'NONE', #22895, 999.9999999999998863 ) ;
#45923=ORIENTED_EDGE ( 'NONE', *, *, #44562, .T. ) ;
#45924=VECTOR ( 'NONE', #20800, 1000.000000000000000 ) ;
#45925=EDGE_CURVE ( 'NONE', #41663, #26368, #21750, .T. ) ;
#45926=VECTOR ( 'NONE', #2733, 999.9999999999998863 ) ;
#45927=ADVANCED_FACE ( 'NONE', ( #8980 ), #29984, .F. ) ;
#45928=ORIENTED_EDGE ( 'NONE', *, *, #12449, .T. ) ;
#45929=AXIS2_PLACEMENT_3D ( 'NONE', #5822, #48974, #10908 ) ;
#45930=ORIENTED_EDGE ( 'NONE', *, *, #37041, .F. ) ;
#45931=ORIENTED_EDGE ( 'NONE', *, *, #54706, .F. ) ;
#45933=EDGE_LOOP ( 'NONE', ( #20651, #24186, #1775, #52008 ) ) ;
#45934=LINE ( 'NONE', #28609, #55912 ) ;
#45935=LINE ( 'NONE', #7044, #35652 ) ;
#45936=LINE ( 'NONE', #42770, #55770 ) ;
#45937=EDGE_CURVE ( 'NONE', #14383, #36112, #52123, .T. ) ;
#45938=EDGE_LOOP ( 'NONE', ( #34404, #28781, #36364, #50392 ) ) ;
#45939=LINE ( 'NONE', #2739, #34035 ) ;
#45940=ORIENTED_EDGE ( 'NONE', *, *, #1772, .F. ) ;
#45941=FACE_OUTER_BOUND ( 'NONE', #4732, .T. ) ;
#45942=ORIENTED_EDGE ( 'NONE', *, *, #5350, .T. ) ;
#45943=AXIS2_PLACEMENT_3D ( 'NONE', #7741, #55709, #25912 ) ;
#45945=CARTESIAN_POINT ( 'NONE',  ( -13.20213141079607766, 0.000000000000000000, 3.240336806989069451 ) ) ;
#45946=DIRECTION ( 'NONE',  ( -0.5364919789714478471, 0.6444004775717705469, -0.5449076811759709926 ) ) ;
#45947=VERTEX_POINT ( 'NONE', #729 ) ;
#45948=DIRECTION ( 'NONE',  ( 0.007781995580012663651, 0.000000000000000000, -0.9999697198139515519 ) ) ;
#45949=ORIENTED_EDGE ( 'NONE', *, *, #7231, .F. ) ;
#45950=LINE ( 'NONE', #42249, #42747 ) ;
#45951=VECTOR ( 'NONE', #42691, 1000.000000000000227 ) ;
#45952=FACE_OUTER_BOUND ( 'NONE', #4106, .T. ) ;
#45953=DIRECTION ( 'NONE',  ( -0.9999697198139514409, -0.000000000000000000, -0.007781995580013368816 ) ) ;
#45954=FACE_OUTER_BOUND ( 'NONE', #11335, .T. ) ;
#45955=VECTOR ( 'NONE', #42120, 1000.000000000000227 ) ;
#45957=CARTESIAN_POINT ( 'NONE',  ( -19.71292464457911109, 4.981562823951513508, 4.180163181755506052 ) ) ;
#45958=CARTESIAN_POINT ( 'NONE',  ( -15.54862763595785147, 3.848249166794009746, 9.236568611826525554 ) ) ;
#45959=DIRECTION ( 'NONE',  ( -0.5449076811759708816, 0.6444004775717707689, 0.5364919789714475140 ) ) ;
#45960=CARTESIAN_POINT ( 'NONE',  ( -11.22999478348192959, -0.1191753592594201883, 1.509027109311680270 ) ) ;
#45961=ORIENTED_EDGE ( 'NONE', *, *, #53591, .F. ) ;
#45963=VERTEX_POINT ( 'NONE', #18049 ) ;
#45964=EDGE_CURVE ( 'NONE', #43762, #50088, #56115, .T. ) ;
#45965=VECTOR ( 'NONE', #24931, 1000.000000000000227 ) ;
#45966=PLANE ( 'NONE',  #12936 ) ;
#45967=CARTESIAN_POINT ( 'NONE',  ( -26.13337879274045505, 0.000000000000000000, 6.833023547870798353 ) ) ;
#45968=DIRECTION ( 'NONE',  ( 0.5364919789714477361, 0.6444004775717706579, 0.5449076811759711036 ) ) ;
#45969=EDGE_CURVE ( 'NONE', #34227, #47810, #17473, .T. ) ;
#45970=LINE ( 'NONE', #32368, #39567 ) ;
#45971=FACE_OUTER_BOUND ( 'NONE', #21330, .T. ) ;
#45972=AXIS2_PLACEMENT_3D ( 'NONE', #6051, #26769, #5210 ) ;
#45973=DIRECTION ( 'NONE',  ( 0.9999697198139515519, 0.000000000000000000, 0.007781995580013368816 ) ) ;
#45974=ORIENTED_EDGE ( 'NONE', *, *, #41523, .F. ) ;
#45975=LINE ( 'NONE', #20399, #41042 ) ;
#45976=DIRECTION ( 'NONE',  ( 0.000000000000000000, -0.000000000000000000, -1.000000000000000000 ) ) ;
#45977=CARTESIAN_POINT ( 'NONE',  ( -19.73004039461353543, 0.000000000000000000, 6.144191668299053610 ) ) ;
#45978=CARTESIAN_POINT ( 'NONE',  ( -12.95637603891941581, 1.905425754524005200, 5.041145850896452174 ) ) ;
#45979=EDGE_CURVE ( 'NONE', #9978, #940, #47032, .T. ) ;
#45980=DIRECTION ( 'NONE',  ( -0.005002170337468016433, -0.7660444431189770143, 0.6427681459581293666 ) ) ;
#45982=ADVANCED_FACE ( 'NONE', ( #21177 ), #55832, .F. ) ;
#45983=LINE ( 'NONE', #38277, #40929 ) ;
#45984=CARTESIAN_POINT ( 'NONE',  ( -11.80534666676753908, 0.000000000000000000, 2.881874839035335256 ) ) ;
#45985=EDGE_CURVE ( 'NONE', #41838, #47834, #51572, .T. ) ;
#45986=FACE_OUTER_BOUND ( 'NONE', #15687, .T. ) ;
#45987=CARTESIAN_POINT ( 'NONE',  ( -19.98606118697598788, 0.000000000000000000, 5.034203045873751670 ) ) ;
#45988=ORIENTED_EDGE ( 'NONE', *, *, #25657, .T. ) ;
#45989=LINE ( 'NONE', #24392, #20341 ) ;
#45990=VERTEX_POINT ( 'NONE', #8398 ) ;
#45991=CARTESIAN_POINT ( 'NONE',  ( -19.22961988024793101, -0.1191753592594177458, 14.39986392600063603 ) ) ;
#45992=LINE ( 'NONE', #7101, #30160 ) ;
#45993=ORIENTED_EDGE ( 'NONE', *, *, #10139, .F. ) ;
#45994=VECTOR ( 'NONE', #48073, 1000.000000000000000 ) ;
#45995=ORIENTED_EDGE ( 'NONE', *, *, #17800, .T. ) ;
#45996=DIRECTION ( 'NONE',  ( 0.007781995580012663651, 0.000000000000000000, -0.9999697198139515519 ) ) ;
#45997=ADVANCED_FACE ( 'NONE', ( #25725 ), #22021, .F. ) ;
#45998=EDGE_CURVE ( 'NONE', #36664, #37392, #8709, .T. ) ;
#45999=VECTOR ( 'NONE', #40250, 999.9999999999998863 ) ;
#46000=EDGE_LOOP ( 'NONE', ( #7732, #15530, #29939, #32713 ) ) ;
#46002=ORIENTED_EDGE ( 'NONE', *, *, #8154, .T. ) ;
#46003=EDGE_CURVE ( 'NONE', #29224, #28898, #14076, .T. ) ;
#46004=LINE ( 'NONE', #45417, #44754 ) ;
#46006=CARTESIAN_POINT ( 'NONE',  ( -9.342070512798265725, 0.000000000000000000, 10.59882438848031505 ) ) ;
#46007=ADVANCED_FACE ( 'NONE', ( #44435 ), #27129, .F. ) ;
#46008=VECTOR ( 'NONE', #9215, 1000.000000000000227 ) ;
#46009=VERTEX_POINT ( 'NONE', #31407 ) ;
#46010=VERTEX_POINT ( 'NONE', #10081 ) ;
#46011=ADVANCED_FACE ( 'NONE', ( #5284 ), #19146, .F. ) ;
#46012=CARTESIAN_POINT ( 'NONE',  ( 2.072287782118878319, 0.000000000000000000, -2.950529333540147015 ) ) ;
#46013=LINE ( 'NONE', #7116, #12765 ) ;
#46015=DIRECTION ( 'NONE',  ( 0.000000000000000000, -0.000000000000000000, -1.000000000000000000 ) ) ;
#46016=ORIENTED_EDGE ( 'NONE', *, *, #31942, .F. ) ;
#46017=LINE ( 'NONE', #45714, #37589 ) ;
#46018=PLANE ( 'NONE',  #21257 ) ;
#46019=ORIENTED_EDGE ( 'NONE', *, *, #22198, .T. ) ;
#46021=DIRECTION ( 'NONE',  ( 0.000000000000000000, -1.000000000000000000, 0.000000000000000000 ) ) ;
#46022=ORIENTED_EDGE ( 'NONE', *, *, #41605, .T. ) ;
#46023=DIRECTION ( 'NONE',  ( 0.7660212471507180654, -0.6427876096865404731, 0.005961354470445141482 ) ) ;
#46024=CARTESIAN_POINT ( 'NONE',  ( -13.96877395608413863, 0.000000000000000000, 8.035687524919993052 ) ) ;
#46025=VERTEX_POINT ( 'NONE', #9537 ) ;
#46027=CARTESIAN_POINT ( 'NONE',  ( -24.26908309836554878, 0.000000000000000000, 6.108867788427308376 ) ) ;
#46028=DIRECTION ( 'NONE',  ( -0.5364919789714478471, 0.6444004775717705469, -0.5449076811759709926 ) ) ;
#46029=PLANE ( 'NONE',  #516 ) ;
#46030=DIRECTION ( 'NONE',  ( 0.5449076811759707706, 0.6444004775717708799, -0.5364919789714476250 ) ) ;
#46031=DIRECTION ( 'NONE',  ( -0.6427681459581293666, -0.7660444431189770143, -0.005002170337467561935 ) ) ;
#46032=VECTOR ( 'NONE', #27976, 999.9999999999998863 ) ;
#46033=DIRECTION ( 'NONE',  ( 0.007781995580012662783, 0.000000000000000000, -0.9999697198139514409 ) ) ;
#46034=VERTEX_POINT ( 'NONE', #5540 ) ;
#46035=LINE ( 'NONE', #7143, #35006 ) ;
#46036=DIRECTION ( 'NONE',  ( 0.5364919789714477361, 0.6444004775717706579, 0.5449076811759711036 ) ) ;
#46037=ORIENTED_EDGE ( 'NONE', *, *, #3553, .T. ) ;
#46038=LINE ( 'NONE', #7146, #20209 ) ;
#46039=DIRECTION ( 'NONE',  ( 0.005961354470445682716, -0.6427876096865404731, -0.7660212471507180654 ) ) ;
#46040=EDGE_CURVE ( 'NONE', #17429, #10323, #45285, .T. ) ;
#46041=VECTOR ( 'NONE', #50638, 999.9999999999998863 ) ;
#46042=LINE ( 'NONE', #16215, #17715 ) ;
#46043=ADVANCED_FACE ( 'NONE', ( #22858 ), #35647, .F. ) ;
#46044=DIRECTION ( 'NONE',  ( 0.5364919789714477361, 0.6444004775717706579, 0.5449076811759711036 ) ) ;
#46045=CARTESIAN_POINT ( 'NONE',  ( -13.73672976910459909, 0.000000000000000000, 12.22661844811216270 ) ) ;
#46046=VERTEX_POINT ( 'NONE', #40755 ) ;
#46047=EDGE_LOOP ( 'NONE', ( #19460, #17080, #40466, #42997 ) ) ;
#46048=DIRECTION ( 'NONE',  ( 0.005002170337468016433, -0.7660444431189770143, -0.6427681459581293666 ) ) ;
#46049=DIRECTION ( 'NONE',  ( -0.7660212471507179544, -0.6427876096865405842, -0.005961354470445141482 ) ) ;
#46050=LINE ( 'NONE', #14625, #55600 ) ;
#46051=ORIENTED_EDGE ( 'NONE', *, *, #8032, .T. ) ;
#46052=DIRECTION ( 'NONE',  ( 0.6427681459581294776, -0.7660444431189769032, 0.005002170337467562802 ) ) ;
#46053=ORIENTED_EDGE ( 'NONE', *, *, #42472, .T. ) ;
#46054=CARTESIAN_POINT ( 'NONE',  ( -19.22961988024793101, -0.1191753592594177458, 14.39986392600063603 ) ) ;
#46055=ORIENTED_EDGE ( 'NONE', *, *, #54915, .F. ) ;
#46056=VERTEX_POINT ( 'NONE', #44178 ) ;
#46057=PLANE ( 'NONE',  #30250 ) ;
#46058=DIRECTION ( 'NONE',  ( 0.000000000000000000, -1.000000000000000000, 0.000000000000000000 ) ) ;
#46059=CARTESIAN_POINT ( 'NONE',  ( 2.072287782118878319, 0.000000000000000000, -2.950529333540147015 ) ) ;
#46060=EDGE_LOOP ( 'NONE', ( #41367, #20972, #14830, #47396 ) ) ;
#46061=LINE ( 'NONE', #7171, #22025 ) ;
#46062=VERTEX_POINT ( 'NONE', #36474 ) ;
#46063=EDGE_CURVE ( 'NONE', #47902, #11899, #18611, .T. ) ;
#46064=ORIENTED_EDGE ( 'NONE', *, *, #55907, .F. ) ;
#46065=ORIENTED_EDGE ( 'NONE', *, *, #27782, .F. ) ;
#46066=LINE ( 'NONE', #10868, #31340 ) ;
#46067=EDGE_CURVE ( 'NONE', #51780, #32296, #2098, .T. ) ;
#46068=LINE ( 'NONE', #53297, #32185 ) ;
#46069=ORIENTED_EDGE ( 'NONE', *, *, #52923, .T. ) ;
#46070=DIRECTION ( 'NONE',  ( -0.005961354470445682716, -0.6427876096865404731, 0.7660212471507180654 ) ) ;
#46071=EDGE_LOOP ( 'NONE', ( #8463, #34428, #10646, #34655, #41995 ) ) ;
#46072=DIRECTION ( 'NONE',  ( 0.007781995580012663651, -3.146120232559066537E-19, -0.9999697198139514409 ) ) ;
#46073=LINE ( 'NONE', #7181, #34051 ) ;
#46074=VECTOR ( 'NONE', #2834, 1000.000000000000114 ) ;
#46075=ORIENTED_EDGE ( 'NONE', *, *, #21812, .F. ) ;
#46076=EDGE_CURVE ( 'NONE', #49857, #14113, #14907, .T. ) ;
#46077=FACE_OUTER_BOUND ( 'NONE', #31316, .T. ) ;
#46078=VERTEX_POINT ( 'NONE', #14366 ) ;
#46079=LINE ( 'NONE', #32725, #44589 ) ;
#46080=CARTESIAN_POINT ( 'NONE',  ( -16.79925329029790149, 0.000000000000000000, 13.49544742625427496 ) ) ;
#46081=FACE_OUTER_BOUND ( 'NONE', #44835, .T. ) ;
#46082=LINE ( 'NONE', #41802, #7568 ) ;
#46083=DIRECTION ( 'NONE',  ( -0.9999697198139514409, -0.000000000000000000, -0.007781995580013368816 ) ) ;
#46084=DIRECTION ( 'NONE',  ( 0.007781995580012663651, -3.146120232559066537E-19, -0.9999697198139514409 ) ) ;
#46085=EDGE_LOOP ( 'NONE', ( #26812, #11877, #16379, #20771 ) ) ;
#46086=ORIENTED_EDGE ( 'NONE', *, *, #51919, .T. ) ;
#46087=DIRECTION ( 'NONE',  ( 0.000000000000000000, -0.000000000000000000, -1.000000000000000000 ) ) ;
#46088=CARTESIAN_POINT ( 'NONE',  ( -19.12407506631472032, 5.305366725996512045, 13.01677197203713554 ) ) ;
#46089=DIRECTION ( 'NONE',  ( 0.5449076811759707706, 0.6444004775717708799, -0.5364919789714476250 ) ) ;
#46090=DIRECTION ( 'NONE',  ( -0.5449076811759708816, 0.6444004775717707689, 0.5364919789714475140 ) ) ;
#46091=PLANE ( 'NONE',  #52416 ) ;
#46092=PLANE ( 'NONE',  #53054 ) ;
#46093=VERTEX_POINT ( 'NONE', #31677 ) ;
#46094=DIRECTION ( 'NONE',  ( -0.005002170337468016433, -0.7660444431189770143, 0.6427681459581293666 ) ) ;
#46095=CARTESIAN_POINT ( 'NONE',  ( -13.94290747453659485, 0.000000000000000000, 4.711900195600111196 ) ) ;
#46096=VERTEX_POINT ( 'NONE', #48982 ) ;
#46097=LINE ( 'NONE', #46356, #50164 ) ;
#46098=ADVANCED_FACE ( 'NONE', ( #52669 ), #18309, .F. ) ;
#46099=CARTESIAN_POINT ( 'NONE',  ( -19.87054375134978557, -1.588720260541462981, 6.487297621897504030 ) ) ;
#46100=EDGE_LOOP ( 'NONE', ( #35078, #23768, #44021, #35690 ) ) ;
#46103=DIRECTION ( 'NONE',  ( -0.5364919789714478471, 0.6444004775717705469, -0.5449076811759709926 ) ) ;
#46104=CARTESIAN_POINT ( 'NONE',  ( -9.503836956215090837, 0.000000000000000000, 5.685116264642521955 ) ) ;
#46105=EDGE_CURVE ( 'NONE', #547, #30844, #23689, .T. ) ;
#46106=EDGE_CURVE ( 'NONE', #50616, #4253, #13773, .T. ) ;
#46107=DIRECTION ( 'NONE',  ( 0.000000000000000000, -1.000000000000000000, 0.000000000000000000 ) ) ;
#46108=LINE ( 'NONE', #50068, #39214 ) ;
#46109=EDGE_LOOP ( 'NONE', ( #10262, #13719, #50654, #50178 ) ) ;
#46110=ORIENTED_EDGE ( 'NONE', *, *, #28232, .F. ) ;
#46111=CARTESIAN_POINT ( 'NONE',  ( -16.23115121177390208, -4.403642575758163424, 3.045552206283119734 ) ) ;
#46112=DIRECTION ( 'NONE',  ( -0.005961354470445682716, -0.6427876096865404731, 0.7660212471507180654 ) ) ;
#46113=CARTESIAN_POINT ( 'NONE',  ( -19.67789331192963331, -0.1191753592594191058, 6.983264656678034754 ) ) ;
#46114=DIRECTION ( 'NONE',  ( -0.005961354470445682716, -0.6427876096865404731, 0.7660212471507180654 ) ) ;
#46115=VECTOR ( 'NONE', #17968, 1000.000000000000227 ) ;
#46116=CARTESIAN_POINT ( 'NONE',  ( -16.94796712057759080, 0.000000000000000000, 6.904506545422637309 ) ) ;
#46118=EDGE_LOOP ( 'NONE', ( #40569, #37139, #6317 ) ) ;
#46119=LINE ( 'NONE', #7223, #45582 ) ;
#46120=EDGE_CURVE ( 'NONE', #40102, #1292, #10371, .T. ) ;
#46121=DIRECTION ( 'NONE',  ( 0.9999697198139515519, 0.000000000000000000, 0.007781995580013368816 ) ) ;
#46122=DIRECTION ( 'NONE',  ( 0.007781995580012662783, 0.000000000000000000, -0.9999697198139514409 ) ) ;
#46123=ORIENTED_EDGE ( 'NONE', *, *, #49439, .F. ) ;
#46124=DIRECTION ( 'NONE',  ( 0.5449076811759707706, 0.6444004775717708799, -0.5364919789714476250 ) ) ;
#46125=CARTESIAN_POINT ( 'NONE',  ( -12.70458494993575194, -0.1191753592594197858, 11.86531876794841978 ) ) ;
#46126=CARTESIAN_POINT ( 'NONE',  ( -14.39249272523662704, 5.305366725996514710, 2.103195701879582824 ) ) ;
#46127=ORIENTED_EDGE ( 'NONE', *, *, #46284, .T. ) ;
#46128=LINE ( 'NONE', #45557, #47673 ) ;
#46129=ORIENTED_EDGE ( 'NONE', *, *, #45277, .T. ) ;
#46130=ORIENTED_EDGE ( 'NONE', *, *, #31232, .F. ) ;
#46131=EDGE_LOOP ( 'NONE', ( #47812, #39085, #2625, #33105 ) ) ;
#46132=ORIENTED_EDGE ( 'NONE', *, *, #475, .F. ) ;
#46133=ORIENTED_EDGE ( 'NONE', *, *, #172, .F. ) ;
#46134=CARTESIAN_POINT ( 'NONE',  ( -10.84028925556084388, -0.1191753592594197858, 11.14116300850493246 ) ) ;
#46135=ORIENTED_EDGE ( 'NONE', *, *, #16828, .F. ) ;
#46136=ORIENTED_EDGE ( 'NONE', *, *, #35590, .F. ) ;
#46137=CARTESIAN_POINT ( 'NONE',  ( -18.58508473505288805, 0.000000000000000000, 4.137115615367276789 ) ) ;
#46138=EDGE_CURVE ( 'NONE', #7759, #20365, #6133, .T. ) ;
#46139=ORIENTED_EDGE ( 'NONE', *, *, #29580, .F. ) ;
#46140=ORIENTED_EDGE ( 'NONE', *, *, #38678, .T. ) ;
#46141=DIRECTION ( 'NONE',  ( 0.9999697198139515519, 0.000000000000000000, 0.007781995580013368816 ) ) ;
#46143=FACE_OUTER_BOUND ( 'NONE', #50255, .T. ) ;
#46144=CARTESIAN_POINT ( 'NONE',  ( -13.01908042430739698, -0.03228989815065527735, 1.937343867007571330 ) ) ;
#46145=DIRECTION ( 'NONE',  ( -0.6246952433987893460, -0.7422098413412802076, 0.2426528472758542054 ) ) ;
#46146=VERTEX_POINT ( 'NONE', #37600 ) ;
#46147=EDGE_CURVE ( 'NONE', #9627, #12842, #41836, .T. ) ;
#46149=ORIENTED_EDGE ( 'NONE', *, *, #44572, .T. ) ;
#46150=CARTESIAN_POINT ( 'NONE',  ( -19.28279667285536902, 3.362543313726509719, 4.064742069204503316 ) ) ;
#46151=CARTESIAN_POINT ( 'NONE',  ( -15.07373161129755346, 0.000000000000000000, 4.903105916910880602 ) ) ;
#46152=EDGE_CURVE ( 'NONE', #5277, #25140, #16032, .T. ) ;
#46153=EDGE_CURVE ( 'NONE', #42919, #2132, #2662, .T. ) ;
#46155=DIRECTION ( 'NONE',  ( -0.9999697198139514409, -0.000000000000000000, -0.007781995580013368816 ) ) ;
#46156=FACE_OUTER_BOUND ( 'NONE', #17796, .T. ) ;
#46157=PLANE ( 'NONE',  #20444 ) ;
#46158=VERTEX_POINT ( 'NONE', #19726 ) ;
#46159=CARTESIAN_POINT ( 'NONE',  ( -27.06708303904391144, 0.000000000000000000, 7.395095371555332697 ) ) ;
#46160=ADVANCED_FACE ( 'NONE', ( #24816 ), #3520, .F. ) ;
#46161=VERTEX_POINT ( 'NONE', #46116 ) ;
#46162=PLANE ( 'NONE',  #7496 ) ;
#46163=CARTESIAN_POINT ( 'NONE',  ( -14.79106777481693058, 5.143464774974011888, 11.06797610652191644 ) ) ;
#46164=EDGE_CURVE ( 'NONE', #6174, #38693, #54614, .T. ) ;
#46165=FACE_OUTER_BOUND ( 'NONE', #47874, .T. ) ;
#46166=LINE ( 'NONE', #32303, #34055 ) ;
#46167=EDGE_CURVE ( 'NONE', #3767, #9065, #7220, .T. ) ;
#46168=CARTESIAN_POINT ( 'NONE',  ( -11.87243407472968926, 0.000000000000000000, 11.50246268866867361 ) ) ;
#46169=ORIENTED_EDGE ( 'NONE', *, *, #4480, .T. ) ;
#46170=ORIENTED_EDGE ( 'NONE', *, *, #24588, .F. ) ;
#46171=LINE ( 'NONE', #2714, #14843 ) ;
#46172=PLANE ( 'NONE',  #16797 ) ;
#46173=LINE ( 'NONE', #7277, #38797 ) ;
#46175=LINE ( 'NONE', #42491, #21019 ) ;
#46176=FACE_OUTER_BOUND ( 'NONE', #3160, .T. ) ;
#46177=CARTESIAN_POINT ( 'NONE',  ( -22.40556560354864146, -0.1191753592594197858, 5.484709000965211523 ) ) ;
#46178=DIRECTION ( 'NONE',  ( -0.9321478471874540261, 0.000000000000000000, 0.3620778797217457656 ) ) ;
#46179=EDGE_CURVE ( 'NONE', #23956, #40778, #10915, .T. ) ;
#46183=ORIENTED_EDGE ( 'NONE', *, *, #50713, .F. ) ;
#46184=ORIENTED_EDGE ( 'NONE', *, *, #31474, .F. ) ;
#46185=EDGE_LOOP ( 'NONE', ( #17425, #22410, #55269, #46972 ) ) ;
#46186=ORIENTED_EDGE ( 'NONE', *, *, #31442, .T. ) ;
#46187=VERTEX_POINT ( 'NONE', #19983 ) ;
#46188=CARTESIAN_POINT ( 'NONE',  ( -13.03243440100211892, 0.000000000000000000, 7.134984182645506046 ) ) ;
#46189=DIRECTION ( 'NONE',  ( 0.005961354470445682716, -0.6427876096865404731, -0.7660212471507180654 ) ) ;
#46190=CARTESIAN_POINT ( 'NONE',  ( -10.74029228357944987, 0.000000000000000000, 11.14194120806293320 ) ) ;
#46191=ORIENTED_EDGE ( 'NONE', *, *, #35865, .T. ) ;
#46193=EDGE_CURVE ( 'NONE', #9089, #41560, #37304, .T. ) ;
#46194=EDGE_LOOP ( 'NONE', ( #8300, #54630, #28149, #8578 ) ) ;
#46195=CARTESIAN_POINT ( 'NONE',  ( -15.96710241509184058, -0.1191753592594218814, 13.13259134697452879 ) ) ;
#46196=EDGE_LOOP ( 'NONE', ( #28048, #23159, #15074, #29799 ) ) ;
#46198=CARTESIAN_POINT ( 'NONE',  ( 2.072287782118878319, 0.000000000000000000, -2.950529333540147015 ) ) ;
#46199=DIRECTION ( 'NONE',  ( 0.007781995580012663651, 0.000000000000000000, -0.9999697198139515519 ) ) ;
#46200=VERTEX_POINT ( 'NONE', #42133 ) ;
#46201=CARTESIAN_POINT ( 'NONE',  ( -22.40634380310664397, 0.000000000000000000, 5.584705972946605534 ) ) ;
#46202=ORIENTED_EDGE ( 'NONE', *, *, #39999, .F. ) ;
#46203=CARTESIAN_POINT ( 'NONE',  ( -32.65841372305263235, 0.000000000000000000, 9.367568705923016381 ) ) ;
#46204=CARTESIAN_POINT ( 'NONE',  ( -14.56888064431065821, -0.1191753592594197858, 12.58947452739191064 ) ) ;
#46206=LINE ( 'NONE', #41671, #31479 ) ;
#46207=DIRECTION ( 'NONE',  ( -0.005002170337468016433, -0.7660444431189770143, 0.6427681459581293666 ) ) ;
#46209=DIRECTION ( 'NONE',  ( -0.7660212471507179544, -0.6427876096865405842, -0.005961354470445141482 ) ) ;
#46210=CARTESIAN_POINT ( 'NONE',  ( -14.66887761629205222, 0.000000000000000000, 12.58869632783390990 ) ) ;
#46211=CARTESIAN_POINT ( 'NONE',  ( -15.88130887279446490, 0.000000000000000000, 3.050160814894388839 ) ) ;
#46212=VERTEX_POINT ( 'NONE', #33062 ) ;
#46213=PLANE ( 'NONE',  #51944 ) ;
#46214=ORIENTED_EDGE ( 'NONE', *, *, #1623, .T. ) ;
#46215=CARTESIAN_POINT ( 'NONE',  ( 2.072287782118878319, 0.000000000000000000, -2.950529333540147015 ) ) ;
#46216=CARTESIAN_POINT ( 'NONE',  ( -11.36657625147399386, 0.000000000000000000, 6.209278080123224797 ) ) ;
#46217=ADVANCED_FACE ( 'NONE', ( #55198 ), #54926, .F. ) ;
#46218=DIRECTION ( 'NONE',  ( 0.5364919789714477361, 0.6444004775717706579, 0.5449076811759711036 ) ) ;
#46219=CARTESIAN_POINT ( 'NONE',  ( -14.20280369269832832, 0.000000000000000000, 12.40765738797303719 ) ) ;
#46220=DIRECTION ( 'NONE',  ( 0.005961354470445682716, -0.6427876096865404731, -0.7660212471507180654 ) ) ;
#46221=EDGE_CURVE ( 'NONE', #1131, #45245, #33355, .T. ) ;
#46222=ADVANCED_FACE ( 'NONE', ( #33607 ), #41579, .F. ) ;
#46223=CARTESIAN_POINT ( 'NONE',  ( -13.78642791384490529, 2.876837460659008805, 6.957818291500617924 ) ) ;
#46225=ORIENTED_EDGE ( 'NONE', *, *, #30109, .T. ) ;
#46226=FACE_OUTER_BOUND ( 'NONE', #47281, .T. ) ;
#46227=DIRECTION ( 'NONE',  ( 0.007781995580012663651, 0.000000000000000000, -0.9999697198139515519 ) ) ;
#46228=CARTESIAN_POINT ( 'NONE',  ( -14.94760462649100496, 0.000000000000000000, 2.488088991209854051 ) ) ;
#46229=DIRECTION ( 'NONE',  ( 0.5364919789714477361, 0.6444004775717706579, 0.5449076811759711036 ) ) ;
#46230=DIRECTION ( 'NONE',  ( 0.5449076811759707706, 0.6444004775717708799, -0.5364919789714476250 ) ) ;
#46231=ADVANCED_FACE ( 'NONE', ( #50917 ), #32767, .F. ) ;
#46232=LINE ( 'NONE', #19850, #30953 ) ;
#46233=DIRECTION ( 'NONE',  ( -0.005002170337468016433, -0.7660444431189770143, 0.6427681459581293666 ) ) ;
#46234=DIRECTION ( 'NONE',  ( -0.6427681459581293666, -0.7660444431189770143, -0.005002170337467561935 ) ) ;
#46235=CARTESIAN_POINT ( 'NONE',  ( -18.73437280588166942, -1.813211359398155809, 6.934787098642066994 ) ) ;
#46236=ORIENTED_EDGE ( 'NONE', *, *, #26125, .F. ) ;
#46237=EDGE_CURVE ( 'NONE', #24506, #4739, #7797, .T. ) ;
#46238=CARTESIAN_POINT ( 'NONE',  ( -7.673472522921562344, 7.485187178597575652, 6.199010895790313391 ) ) ;
#46239=CARTESIAN_POINT ( 'NONE',  ( -11.40636015113596180, 0.000000000000000000, 11.32142374880780089 ) ) ;
#46240=ORIENTED_EDGE ( 'NONE', *, *, #53584, .T. ) ;
#46241=PLANE ( 'NONE',  #50404 ) ;
#46242=CARTESIAN_POINT ( 'NONE',  ( -14.00280974873554030, 0.000000000000000000, 12.40921378708904044 ) ) ;
#46243=ORIENTED_EDGE ( 'NONE', *, *, #13677, .F. ) ;
#46244=EDGE_LOOP ( 'NONE', ( #18820, #39392, #33501, #45321 ) ) ;
#46245=LINE ( 'NONE', #47890, #47408 ) ;
#46246=AXIS2_PLACEMENT_3D ( 'NONE', #48183, #8456, #26331 ) ;
#46247=ORIENTED_EDGE ( 'NONE', *, *, #47268, .T. ) ;
#46249=ORIENTED_EDGE ( 'NONE', *, *, #51458, .T. ) ;
#46250=LINE ( 'NONE', #11352, #25700 ) ;
#46252=PLANE ( 'NONE',  #35797 ) ;
#46253=EDGE_CURVE ( 'NONE', #30294, #45499, #49819, .T. ) ;
#46254=ORIENTED_EDGE ( 'NONE', *, *, #10544, .T. ) ;
#46255=EDGE_CURVE ( 'NONE', #52840, #38691, #45838, .T. ) ;
#46256=ORIENTED_EDGE ( 'NONE', *, *, #37977, .T. ) ;
#46257=DIRECTION ( 'NONE',  ( -0.005002170337468016433, -0.7660444431189770143, 0.6427681459581293666 ) ) ;
#46258=DIRECTION ( 'NONE',  ( -0.005002170337468016433, -0.7660444431189770143, 0.6427681459581293666 ) ) ;
#46259=ORIENTED_EDGE ( 'NONE', *, *, #3579, .F. ) ;
#46260=EDGE_CURVE ( 'NONE', #5087, #30222, #25962, .T. ) ;
#46261=DIRECTION ( 'NONE',  ( 0.007781995580012663651, -3.146120232559066537E-19, -0.9999697198139514409 ) ) ;
#46262=ORIENTED_EDGE ( 'NONE', *, *, #2039, .F. ) ;
#46263=PLANE ( 'NONE',  #9460 ) ;
#46264=DIRECTION ( 'NONE',  ( -0.5449076811759708816, 0.6444004775717707689, 0.5364919789714475140 ) ) ;
#46265=EDGE_CURVE ( 'NONE', #2953, #46599, #30201, .T. ) ;
#46266=EDGE_CURVE ( 'NONE', #12870, #45853, #12875, .T. ) ;
#46267=ADVANCED_FACE ( 'NONE', ( #3783 ), #12609, .F. ) ;
#46268=EDGE_LOOP ( 'NONE', ( #24682, #5322, #51638, #52865 ) ) ;
#46269=CARTESIAN_POINT ( 'NONE',  ( -27.06552663992790997, 0.000000000000000000, 7.195101427592543786 ) ) ;
#46270=DIRECTION ( 'NONE',  ( 0.5449076811759707706, 0.6444004775717708799, -0.5364919789714476250 ) ) ;
#46271=ORIENTED_EDGE ( 'NONE', *, *, #20775, .F. ) ;
#46272=CARTESIAN_POINT ( 'NONE',  ( -14.93495759592298988, 0.000000000000000000, 12.77129166681078409 ) ) ;
#46274=DIRECTION ( 'NONE',  ( 0.007781995580012662783, 0.000000000000000000, -0.9999697198139514409 ) ) ;
#46275=ORIENTED_EDGE ( 'NONE', *, *, #40521, .T. ) ;
#46276=CARTESIAN_POINT ( 'NONE',  ( -18.34630826372213264, 0.000000000000000000, 7.462962457339162192 ) ) ;
#46277=DIRECTION ( 'NONE',  ( -0.5449076811759708816, 0.6444004775717707689, 0.5364919789714475140 ) ) ;
#46278=DIRECTION ( 'NONE',  ( -0.005002170337468016433, -0.7660444431189770143, 0.6427681459581293666 ) ) ;
#46279=EDGE_CURVE ( 'NONE', #18658, #19197, #17145, .T. ) ;
#46280=LINE ( 'NONE', #28721, #44044 ) ;
#46281=LINE ( 'NONE', #54268, #9535 ) ;
#46282=LINE ( 'NONE', #30104, #46074 ) ;
#46283=VECTOR ( 'NONE', #28426, 1000.000000000000227 ) ;
#46284=EDGE_CURVE ( 'NONE', #28225, #11772, #46970, .T. ) ;
#46285=LINE ( 'NONE', #29257, #45781 ) ;
#46286=ORIENTED_EDGE ( 'NONE', *, *, #48937, .T. ) ;
#46287=DIRECTION ( 'NONE',  ( 0.7660212471507180654, -0.6427876096865404731, 0.005961354470445141482 ) ) ;
#46288=CARTESIAN_POINT ( 'NONE',  ( -11.81684288078866807, 0.000000000000000000, 4.359113652066392675 ) ) ;
#46289=EDGE_CURVE ( 'NONE', #11344, #9180, #4083, .T. ) ;
#46290=LINE ( 'NONE', #51684, #32345 ) ;
#46291=ORIENTED_EDGE ( 'NONE', *, *, #39364, .F. ) ;
#46292=PLANE ( 'NONE',  #41981 ) ;
#46293=DIRECTION ( 'NONE',  ( 0.000000000000000000, -1.000000000000000000, 0.000000000000000000 ) ) ;
#46294=EDGE_CURVE ( 'NONE', #37913, #43375, #25652, .T. ) ;
#46295=DIRECTION ( 'NONE',  ( -0.2426528472758542054, 0.7422098413412800966, -0.6246952433987894571 ) ) ;
#46296=CARTESIAN_POINT ( 'NONE',  ( -18.19747506107908563, 0.000000000000000000, 14.03856424583689311 ) ) ;
#46297=EDGE_CURVE ( 'NONE', #16744, #46741, #47223, .T. ) ;
#46299=ORIENTED_EDGE ( 'NONE', *, *, #46592, .F. ) ;
#46300=ORIENTED_EDGE ( 'NONE', *, *, #14827, .F. ) ;
#46301=PLANE ( 'NONE',  #24986 ) ;
#46302=PLANE ( 'NONE',  #6677 ) ;
#46303=AXIS2_PLACEMENT_3D ( 'NONE', #1890, #20047, #53862 ) ;
#46304=ORIENTED_EDGE ( 'NONE', *, *, #36191, .F. ) ;
#46305=LINE ( 'NONE', #46598, #53065 ) ;
#46306=ORIENTED_EDGE ( 'NONE', *, *, #18343, .T. ) ;
#46307=DIRECTION ( 'NONE',  ( 0.5449076811759707706, 0.6444004775717708799, -0.5364919789714476250 ) ) ;
#46308=ORIENTED_EDGE ( 'NONE', *, *, #13164, .F. ) ;
#46309=EDGE_LOOP ( 'NONE', ( #10547, #45897, #43246, #20371 ) ) ;
#46310=ORIENTED_EDGE ( 'NONE', *, *, #14509, .F. ) ;
#46311=CARTESIAN_POINT ( 'NONE',  ( -10.86900711168552291, 0.000000000000000000, 1.981171496760848916 ) ) ;
#46312=LINE ( 'NONE', #50861, #3289 ) ;
#46313=CARTESIAN_POINT ( 'NONE',  ( -9.442067484779661513, -0.1191753592594197858, 10.59804618892231254 ) ) ;
#46314=AXIS2_PLACEMENT_3D ( 'NONE', #5183, #6288, #53424 ) ;
#46315=LINE ( 'NONE', #11128, #39246 ) ;
#46316=VERTEX_POINT ( 'NONE', #42682 ) ;
#46318=ORIENTED_EDGE ( 'NONE', *, *, #34890, .T. ) ;
#46319=ORIENTED_EDGE ( 'NONE', *, *, #49474, .F. ) ;
#46320=CARTESIAN_POINT ( 'NONE',  ( -14.39185644946198295, 0.000000000000000000, 2.692420008248304963 ) ) ;
#46321=CARTESIAN_POINT ( 'NONE',  ( -21.47419595591918906, 0.000000000000000000, 5.222628093224860102 ) ) ;
#46322=ORIENTED_EDGE ( 'NONE', *, *, #18702, .T. ) ;
#46323=DIRECTION ( 'NONE',  ( 0.5364919789714477361, 0.6444004775717706579, 0.5449076811759711036 ) ) ;
#46325=DIRECTION ( 'NONE',  ( -0.6427681459581293666, -0.7660444431189770143, -0.005002170337467561935 ) ) ;
#46326=FACE_OUTER_BOUND ( 'NONE', #30794, .T. ) ;
#46327=EDGE_CURVE ( 'NONE', #42852, #42669, #4633, .T. ) ;
#46328=EDGE_CURVE ( 'NONE', #33489, #23596, #55464, .T. ) ;
#46329=ORIENTED_EDGE ( 'NONE', *, *, #6967, .F. ) ;
#46331=VERTEX_POINT ( 'NONE', #21106 ) ;
#46332=EDGE_CURVE ( 'NONE', #3951, #11444, #69, .T. ) ;
#46333=CARTESIAN_POINT ( 'NONE',  ( -20.54049170961573267, 0.000000000000000000, 4.660556269540326646 ) ) ;
#46334=CARTESIAN_POINT ( 'NONE',  ( -19.60834386242827776, 0.000000000000000000, 4.298478389818581213 ) ) ;
#46335=FACE_OUTER_BOUND ( 'NONE', #8258, .T. ) ;
#46336=CARTESIAN_POINT ( 'NONE',  ( -13.14148572275694171, -1.813211359398156919, 4.762319820311594398 ) ) ;
#46337=PLANE ( 'NONE',  #46861 ) ;
#46338=FACE_OUTER_BOUND ( 'NONE', #50788, .T. ) ;
#46339=APPLICATION_CONTEXT ( 'automotive_design' ) ;
#46340=ORIENTED_EDGE ( 'NONE', *, *, #28270, .T. ) ;
#46341=AXIS2_PLACEMENT_3D ( 'NONE', #20405, #25503, #24386 ) ;
#46343=ORIENTED_EDGE ( 'NONE', *, *, #47064, .F. ) ;
#46344=VECTOR ( 'NONE', #12988, 999.9999999999998863 ) ;
#46345=LINE ( 'NONE', #7459, #39151 ) ;
#46346=DIRECTION ( 'NONE',  ( 0.005002170337468016433, -0.7660444431189770143, -0.6427681459581293666 ) ) ;
#46348=DIRECTION ( 'NONE',  ( -0.5449076811759708816, 0.6444004775717707689, 0.5364919789714475140 ) ) ;
#46349=FACE_OUTER_BOUND ( 'NONE', #37700, .T. ) ;
#46350=DIRECTION ( 'NONE',  ( 0.007781995580012663651, 0.000000000000000000, -0.9999697198139515519 ) ) ;
#46351=ORIENTED_EDGE ( 'NONE', *, *, #46040, .T. ) ;
#46352=CARTESIAN_POINT ( 'NONE',  ( -10.74029228357944987, 0.000000000000000000, 11.14194120806293320 ) ) ;
#46353=ADVANCED_FACE ( 'NONE', ( #34734 ), #30773, .F. ) ;
#46354=DIRECTION ( 'NONE',  ( 0.5449076811759707706, 0.6444004775717708799, -0.5364919789714476250 ) ) ;
#46355=ORIENTED_EDGE ( 'NONE', *, *, #1561, .T. ) ;
#46356=CARTESIAN_POINT ( 'NONE',  ( -12.70458494993575194, -0.1191753592594197858, 11.86531876794841978 ) ) ;
#46357=PLANE ( 'NONE',  #32266 ) ;
#46360=CARTESIAN_POINT ( 'NONE',  ( -16.83070019881521517, 0.4483081953215033444, 3.205243883113554570 ) ) ;
#46361=ADVANCED_FACE ( 'NONE', ( #34206 ), #16566, .F. ) ;
#46362=LINE ( 'NONE', #30696, #44056 ) ;
#46363=EDGE_CURVE ( 'NONE', #30649, #13281, #21947, .T. ) ;
#46364=DIRECTION ( 'NONE',  ( -0.9999697198139514409, -0.000000000000000000, -0.007781995580013368816 ) ) ;
#46365=AXIS2_PLACEMENT_3D ( 'NONE', #236, #25535, #42315 ) ;
#46366=DIRECTION ( 'NONE',  ( 0.9321478471874540261, 0.000000000000000000, -0.3620778797217457101 ) ) ;
#46367=ORIENTED_EDGE ( 'NONE', *, *, #3039, .F. ) ;
#46368=EDGE_CURVE ( 'NONE', #46316, #23729, #20829, .T. ) ;
#46369=ORIENTED_EDGE ( 'NONE', *, *, #50157, .T. ) ;
#46371=LINE ( 'NONE', #33351, #14982 ) ;
#46373=ADVANCED_FACE ( 'NONE', ( #8331 ), #56055, .F. ) ;
#46374=CARTESIAN_POINT ( 'NONE',  ( -11.20636620717317378, 0.000000000000000000, 11.32298014792380414 ) ) ;
#46375=DIRECTION ( 'NONE',  ( 0.007781995580012663651, 0.000000000000000000, -0.9999697198139515519 ) ) ;
#46376=EDGE_CURVE ( 'NONE', #51697, #27027, #29925, .T. ) ;
#46377=FACE_OUTER_BOUND ( 'NONE', #49614, .T. ) ;
#46378=ORIENTED_EDGE ( 'NONE', *, *, #48405, .F. ) ;
#46379=CARTESIAN_POINT ( 'NONE',  ( -19.51723258224034296, 0.000000000000000000, 4.499193495089023109 ) ) ;
#46380=CARTESIAN_POINT ( 'NONE',  ( -17.23560250149814976, 0.000000000000000000, 9.856924658832747710 ) ) ;
#46381=DIRECTION ( 'NONE',  ( 0.000000000000000000, -1.000000000000000000, 0.000000000000000000 ) ) ;
#46382=ORIENTED_EDGE ( 'NONE', *, *, #37078, .F. ) ;
#46385=DIRECTION ( 'NONE',  ( 0.007781995580012663651, -3.146120232559066537E-19, -0.9999697198139514409 ) ) ;
#46386=ORIENTED_EDGE ( 'NONE', *, *, #12978, .T. ) ;
#46387=AXIS2_PLACEMENT_3D ( 'NONE', #34267, #38804, #4159 ) ;
#46388=VECTOR ( 'NONE', #3890, 999.9999999999998863 ) ;
#46389=CARTESIAN_POINT ( 'NONE',  ( -17.72271011234543536, -2.298917212465660054, 3.692076095354655418 ) ) ;
#46390=ORIENTED_EDGE ( 'NONE', *, *, #12671, .T. ) ;
#46392=ORIENTED_EDGE ( 'NONE', *, *, #34456, .F. ) ;
#46393=EDGE_LOOP ( 'NONE', ( #20603, #16993, #31430, #50682 ) ) ;
#46394=VECTOR ( 'NONE', #46443, 1000.000000000000227 ) ;
#46395=ORIENTED_EDGE ( 'NONE', *, *, #16802, .F. ) ;
#46396=CARTESIAN_POINT ( 'NONE',  ( -32.65841372305263235, 0.000000000000000000, 9.367568705923016381 ) ) ;
#46397=ORIENTED_EDGE ( 'NONE', *, *, #53935, .T. ) ;
#46398=EDGE_CURVE ( 'NONE', #45566, #9012, #44374, .T. ) ;
#46399=ORIENTED_EDGE ( 'NONE', *, *, #20942, .F. ) ;
#46400=DIRECTION ( 'NONE',  ( -0.2426528472758541499, 0.7422098413412800966, -0.6246952433987894571 ) ) ;
#46401=VERTEX_POINT ( 'NONE', #19858 ) ;
#46402=VECTOR ( 'NONE', #39991, 999.9999999999998863 ) ;
#46404=ADVANCED_FACE ( 'NONE', ( #10015 ), #5475, .F. ) ;
#46405=EDGE_CURVE ( 'NONE', #37937, #16343, #22790, .T. ) ;
#46406=VECTOR ( 'NONE', #39232, 1000.000000000000227 ) ;
#46407=LINE ( 'NONE', #41046, #7514 ) ;
#46408=DIRECTION ( 'NONE',  ( -0.9999697198139514409, -0.000000000000000000, -0.007781995580013368816 ) ) ;
#46409=DIRECTION ( 'NONE',  ( 0.9999697198139515519, 0.000000000000000000, 0.007781995580013368816 ) ) ;
#46410=DIRECTION ( 'NONE',  ( 0.005002170337468016433, -0.7660444431189770143, -0.6427681459581293666 ) ) ;
#46411=ORIENTED_EDGE ( 'NONE', *, *, #526, .F. ) ;
#46412=EDGE_LOOP ( 'NONE', ( #3471, #25498, #44591 ) ) ;
#46413=DIRECTION ( 'NONE',  ( 0.7660212471507180654, -0.6427876096865404731, 0.005961354470445141482 ) ) ;
#46414=CARTESIAN_POINT ( 'NONE',  ( -20.54049170961573267, 0.000000000000000000, 4.660556269540326646 ) ) ;
#46416=CARTESIAN_POINT ( 'NONE',  ( -15.88130887279446490, 0.000000000000000000, 3.050160814894388839 ) ) ;
#46417=CARTESIAN_POINT ( 'NONE',  ( -11.71187600135471030, -0.1191753592594190225, 3.721269417090256049 ) ) ;
#46418=CARTESIAN_POINT ( 'NONE',  ( 2.072287782118878319, 0.000000000000000000, -2.950529333540147015 ) ) ;
#46419=ORIENTED_EDGE ( 'NONE', *, *, #3610, .T. ) ;
#46420=CARTESIAN_POINT ( 'NONE',  ( 2.072287782118878319, 0.000000000000000000, -2.950529333540147015 ) ) ;
#46421=DIRECTION ( 'NONE',  ( 0.7660212471507180654, -0.6427876096865404731, 0.005961354470445141482 ) ) ;
#46422=ORIENTED_EDGE ( 'NONE', *, *, #20827, .T. ) ;
#46423=VECTOR ( 'NONE', #2538, 999.9999999999998863 ) ;
#46424=VECTOR ( 'NONE', #30389, 1000.000000000000227 ) ;
#46425=PLANE ( 'NONE',  #37938 ) ;
#46426=DIRECTION ( 'NONE',  ( 0.005961354470445682716, -0.6427876096865404731, -0.7660212471507180654 ) ) ;
#46427=CARTESIAN_POINT ( 'NONE',  ( -30.79567442779373110, 0.000000000000000000, 8.843406890442315316 ) ) ;
#46428=PLANE ( 'NONE',  #18699 ) ;
#46429=EDGE_CURVE ( 'NONE', #49589, #12571, #40108, .T. ) ;
#46430=FACE_OUTER_BOUND ( 'NONE', #45310, .T. ) ;
#46431=EDGE_LOOP ( 'NONE', ( #22623, #10573, #27995, #1071 ) ) ;
#46432=VECTOR ( 'NONE', #10454, 999.9999999999998863 ) ;
#46433=AXIS2_PLACEMENT_3D ( 'NONE', #22140, #10195, #36069 ) ;
#46434=EDGE_CURVE ( 'NONE', #29543, #29153, #10298, .T. ) ;
#46435=EDGE_LOOP ( 'NONE', ( #22121, #7073, #12813, #49728 ) ) ;
#46436=CARTESIAN_POINT ( 'NONE',  ( -12.75218409439548850, 3.848249166794009746, 8.150334972661291033 ) ) ;
#46437=DIRECTION ( 'NONE',  ( -0.6427681459581293666, -0.7660444431189770143, -0.005002170337467561935 ) ) ;
#46439=DIRECTION ( 'NONE',  ( 0.5449076811759707706, 0.6444004775717708799, -0.5364919789714476250 ) ) ;
#46440=EDGE_CURVE ( 'NONE', #34418, #21379, #22532, .T. ) ;
#46441=VECTOR ( 'NONE', #43567, 1000.000000000000227 ) ;
#46442=PLANE ( 'NONE',  #31205 ) ;
#46443=DIRECTION ( 'NONE',  ( 0.007781995580012663651, -3.146120232559066537E-19, -0.9999697198139514409 ) ) ;
#46444=CARTESIAN_POINT ( 'NONE',  ( -26.13493519185646008, 0.000000000000000000, 7.033017491833586377 ) ) ;
#46446=DIRECTION ( 'NONE',  ( 0.9321478471874540261, 0.000000000000000000, -0.3620778797217456546 ) ) ;
#46447=ORIENTED_EDGE ( 'NONE', *, *, #28371, .F. ) ;
#46448=LINE ( 'NONE', #25738, #31298 ) ;
#46449=EDGE_CURVE ( 'NONE', #9219, #37763, #11342, .T. ) ;
#46450=ORIENTED_EDGE ( 'NONE', *, *, #20676, .F. ) ;
#46451=VECTOR ( 'NONE', #8973, 999.9999999999998863 ) ;
#46452=EDGE_CURVE ( 'NONE', #39023, #3804, #27065, .T. ) ;
#46453=EDGE_LOOP ( 'NONE', ( #20226, #36791, #35133, #32539 ) ) ;
#46454=VERTEX_POINT ( 'NONE', #44943 ) ;
#46455=EDGE_LOOP ( 'NONE', ( #18391, #53052, #7852, #7184 ) ) ;
#46456=ORIENTED_EDGE ( 'NONE', *, *, #31484, .T. ) ;
#46457=LINE ( 'NONE', #7580, #23285 ) ;
#46458=CARTESIAN_POINT ( 'NONE',  ( -21.14709236723027530, 3.362543313726509719, 4.788897828647994181 ) ) ;
#46459=ADVANCED_FACE ( 'NONE', ( #44637 ), #37177, .F. ) ;
#46460=CARTESIAN_POINT ( 'NONE',  ( -14.49613859905933211, -0.6798977022406558213, 2.490421343638416829 ) ) ;
#46461=VECTOR ( 'NONE', #16098, 1000.000000000000114 ) ;
#46462=VECTOR ( 'NONE', #8450, 999.9999999999998863 ) ;
#46463=ORIENTED_EDGE ( 'NONE', *, *, #39709, .F. ) ;
#46465=LINE ( 'NONE', #28897, #39466 ) ;
#46466=ORIENTED_EDGE ( 'NONE', *, *, #20839, .T. ) ;
#46467=LINE ( 'NONE', #12435, #8683 ) ;
#46468=ORIENTED_EDGE ( 'NONE', *, *, #911, .F. ) ;
#46469=ADVANCED_FACE ( 'NONE', ( #17988 ), #6065, .F. ) ;
#46470=VECTOR ( 'NONE', #28447, 1000.000000000000000 ) ;
#46473=CARTESIAN_POINT ( 'NONE',  ( -15.13495153988577968, 0.000000000000000000, 12.76973526769478084 ) ) ;
#46474=DIRECTION ( 'NONE',  ( -0.9999697198139514409, -0.000000000000000000, -0.007781995580013368816 ) ) ;
#46475=ORIENTED_EDGE ( 'NONE', *, *, #36729, .F. ) ;
#46476=CARTESIAN_POINT ( 'NONE',  ( -13.20500546430136346, 0.000000000000000000, 3.609646510246834694 ) ) ;
#46477=ORIENTED_EDGE ( 'NONE', *, *, #11938, .F. ) ;
#46478=ADVANCED_FACE ( 'NONE', ( #36155 ), #53455, .F. ) ;
#46479=PLANE ( 'NONE',  #5555 ) ;
#46480=AXIS2_PLACEMENT_3D ( 'NONE', #17897, #31779, #31519 ) ;
#46481=LINE ( 'NONE', #15834, #31153 ) ;
#46483=EDGE_CURVE ( 'NONE', #48923, #43832, #32915, .T. ) ;
#46484=CARTESIAN_POINT ( 'NONE',  ( -10.94028622754223967, 0.000000000000000000, 11.14038480894692995 ) ) ;
#46485=CARTESIAN_POINT ( 'NONE',  ( -18.29747203306047609, -0.1191753592594177458, 14.03778604627889059 ) ) ;
#46486=LINE ( 'NONE', #51876, #44715 ) ;
#46487=CARTESIAN_POINT ( 'NONE',  ( -16.81345671998191449, 0.000000000000000000, 3.412238694616132495 ) ) ;
#46488=DIRECTION ( 'NONE',  ( 0.5449076811759707706, 0.6444004775717708799, -0.5364919789714476250 ) ) ;
#46489=FACE_OUTER_BOUND ( 'NONE', #14134, .T. ) ;
#46491=CARTESIAN_POINT ( 'NONE',  ( -17.43300170430006091, 0.6102101463440035012, 3.434032722201703081 ) ) ;
#46492=VERTEX_POINT ( 'NONE', #53201 ) ;
#46494=DIRECTION ( 'NONE',  ( -0.9999697198139514409, -0.000000000000000000, -0.007781995580013368816 ) ) ;
#46495=CARTESIAN_POINT ( 'NONE',  ( -23.33849165029409889, 0.000000000000000000, 5.946783852668351855 ) ) ;
#46496=CARTESIAN_POINT ( 'NONE',  ( -8.609916609573598834, 0.000000000000000000, 10.23519010964256637 ) ) ;
#46497=AXIS2_PLACEMENT_3D ( 'NONE', #50223, #28667, #49692 ) ;
#46498=DIRECTION ( 'NONE',  ( 0.5364919789714477361, 0.6444004775717706579, 0.5449076811759711036 ) ) ;
#46499=CARTESIAN_POINT ( 'NONE',  ( -15.33681816505984763, 0.000000000000000000, 4.701052460296081925 ) ) ;
#46500=LINE ( 'NONE', #46223, #49288 ) ;
#46501=ORIENTED_EDGE ( 'NONE', *, *, #37848, .T. ) ;
#46502=DIRECTION ( 'NONE',  ( 0.005961354470445682716, -0.6427876096865404731, -0.7660212471507180654 ) ) ;
#46503=VECTOR ( 'NONE', #24668, 1000.000000000000227 ) ;
#46504=DIRECTION ( 'NONE',  ( -0.005002170337468016433, -0.7660444431189770143, 0.6427681459581293666 ) ) ;
#46505=CARTESIAN_POINT ( 'NONE',  ( -10.30359504330503917, -0.1191753592594205352, 1.885568636105463547 ) ) ;
#46506=CARTESIAN_POINT ( 'NONE',  ( -18.67775241435682432, 0.000000000000000000, 4.136394454059623804 ) ) ;
#46507=VECTOR ( 'NONE', #52968, 1000.000000000000227 ) ;
#46509=FACE_OUTER_BOUND ( 'NONE', #52211, .T. ) ;
#46510=EDGE_CURVE ( 'NONE', #7643, #14573, #50230, .T. ) ;
#46511=FACE_OUTER_BOUND ( 'NONE', #1782, .T. ) ;
#46512=FACE_OUTER_BOUND ( 'NONE', #14021, .T. ) ;
#46513=DIRECTION ( 'NONE',  ( 0.007781995580012663651, 0.000000000000000000, -0.9999697198139515519 ) ) ;
#46514=ORIENTED_EDGE ( 'NONE', *, *, #29835, .T. ) ;
#46515=VECTOR ( 'NONE', #1707, 999.9999999999998863 ) ;
#46516=DIRECTION ( 'NONE',  ( 0.007781995580012662783, 0.000000000000000000, -0.9999697198139514409 ) ) ;
#46517=AXIS2_PLACEMENT_3D ( 'NONE', #13078, #30408, #7992 ) ;
#46518=CARTESIAN_POINT ( 'NONE',  ( -19.07403171432551758, 0.000000000000000000, 7.257293088956358496 ) ) ;
#46519=ORIENTED_EDGE ( 'NONE', *, *, #20239, .F. ) ;
#46520=ORIENTED_EDGE ( 'NONE', *, *, #52219, .F. ) ;
#46521=LINE ( 'NONE', #46242, #30114 ) ;
#46522=EDGE_CURVE ( 'NONE', #6267, #44587, #4921, .T. ) ;
#46523=ORIENTED_EDGE ( 'NONE', *, *, #18929, .F. ) ;
#46524=AXIS2_PLACEMENT_3D ( 'NONE', #8813, #47966, #43430 ) ;
#46525=EDGE_LOOP ( 'NONE', ( #9901, #11323, #31449, #39005 ) ) ;
#46526=LINE ( 'NONE', #38029, #49237 ) ;
#46527=EDGE_CURVE ( 'NONE', #15160, #9839, #35309, .T. ) ;
#46528=VECTOR ( 'NONE', #52692, 999.9999999999998863 ) ;
#46529=EDGE_CURVE ( 'NONE', #19170, #12202, #48344, .T. ) ;
#46530=VERTEX_POINT ( 'NONE', #25256 ) ;
#46531=VERTEX_POINT ( 'NONE', #28950 ) ;
#46532=ORIENTED_EDGE ( 'NONE', *, *, #47239, .F. ) ;
#46533=CARTESIAN_POINT ( 'NONE',  ( -14.46888367232926420, 0.000000000000000000, 12.59025272694991315 ) ) ;
#46534=DIRECTION ( 'NONE',  ( 0.5364919789714477361, 0.6444004775717706579, 0.5449076811759711036 ) ) ;
#46536=LINE ( 'NONE', #42844, #14916 ) ;
#46537=VECTOR ( 'NONE', #10637, 1000.000000000000227 ) ;
#46538=EDGE_CURVE ( 'NONE', #38354, #19178, #46521, .T. ) ;
#46539=EDGE_LOOP ( 'NONE', ( #538, #42515, #25819, #41116 ) ) ;
#46540=ORIENTED_EDGE ( 'NONE', *, *, #18074, .F. ) ;
#46541=AXIS2_PLACEMENT_3D ( 'NONE', #39001, #51765, #12874 ) ;
#46542=ADVANCED_FACE ( 'NONE', ( #20419 ), #50532, .F. ) ;
#46544=DIRECTION ( 'NONE',  ( -0.7660212471507179544, -0.6427876096865405842, -0.005961354470445141482 ) ) ;
#46545=EDGE_LOOP ( 'NONE', ( #24843, #10103, #13655, #43728 ) ) ;
#46546=AXIS2_PLACEMENT_3D ( 'NONE', #37063, #24281, #54361 ) ;
#46547=DIRECTION ( 'NONE',  ( -0.5364919789714478471, 0.6444004775717705469, -0.5449076811759709926 ) ) ;
#46548=ORIENTED_EDGE ( 'NONE', *, *, #45761, .F. ) ;
#46549=LINE ( 'NONE', #39387, #54802 ) ;
#46550=CARTESIAN_POINT ( 'NONE',  ( -19.22790012936460613, -0.06318563913204579274, 8.141745193239319889 ) ) ;
#46551=VECTOR ( 'NONE', #20799, 1000.000000000000227 ) ;
#46552=EDGE_CURVE ( 'NONE', #21327, #29513, #24969, .T. ) ;
#46553=AXIS2_PLACEMENT_3D ( 'NONE', #44786, #31161, #9604 ) ;
#46554=ORIENTED_EDGE ( 'NONE', *, *, #4962, .T. ) ;
#46555=DIRECTION ( 'NONE',  ( 0.005961354470445682716, -0.6427876096865404731, -0.7660212471507180654 ) ) ;
#46557=AXIS2_PLACEMENT_3D ( 'NONE', #24958, #43403, #38867 ) ;
#46558=LINE ( 'NONE', #7378, #9130 ) ;
#46559=VECTOR ( 'NONE', #4831, 1000.000000000000114 ) ;
#46560=ORIENTED_EDGE ( 'NONE', *, *, #24144, .T. ) ;
#46561=LINE ( 'NONE', #8229, #47621 ) ;
#46562=CARTESIAN_POINT ( 'NONE',  ( -31.72626587586518099, 0.000000000000000000, 9.005490826201270949 ) ) ;
#46563=LINE ( 'NONE', #42329, #16695 ) ;
#46564=CARTESIAN_POINT ( 'NONE',  ( -14.60909471445646979, 0.000000000000000000, 4.906721828678888286 ) ) ;
#46565=ORIENTED_EDGE ( 'NONE', *, *, #26362, .F. ) ;
#46566=CARTESIAN_POINT ( 'NONE',  ( -15.19872173456531250, -2.622721114510660367, 2.701342254643969376 ) ) ;
#46567=DIRECTION ( 'NONE',  ( 0.000000000000000000, -0.000000000000000000, -1.000000000000000000 ) ) ;
#46568=PLANE ( 'NONE',  #7681 ) ;
#46569=LINE ( 'NONE', #47723, #53141 ) ;
#46570=DIRECTION ( 'NONE',  ( 0.005961354470445682716, -0.6427876096865404731, -0.7660212471507180654 ) ) ;
#46571=LINE ( 'NONE', #33799, #34266 ) ;
#46572=LINE ( 'NONE', #28419, #6804 ) ;
#46573=VECTOR ( 'NONE', #26509, 1000.000000000000227 ) ;
#46574=VERTEX_POINT ( 'NONE', #29516 ) ;
#46575=CARTESIAN_POINT ( 'NONE',  ( -16.02444143390598796, 0.000000000000000000, 7.650357775474186717 ) ) ;
#46576=PLANE ( 'NONE',  #33233 ) ;
#46577=EDGE_LOOP ( 'NONE', ( #21714, #36373, #55665, #54251 ) ) ;
#46578=DIRECTION ( 'NONE',  ( -0.7660212471507179544, -0.6427876096865405842, -0.005961354470445141482 ) ) ;
#46579=CARTESIAN_POINT ( 'NONE',  ( -12.19663127273277681, -0.1191753592594185784, 6.302821428126598846 ) ) ;
#46580=AXIS2_PLACEMENT_3D ( 'NONE', #36888, #9922, #6227 ) ;
#46581=DIRECTION ( 'NONE',  ( 0.9999697198139515519, 0.000000000000000000, 0.007781995580013368816 ) ) ;
#46582=EDGE_CURVE ( 'NONE', #46034, #44456, #34337, .T. ) ;
#46583=VECTOR ( 'NONE', #8760, 1000.000000000000000 ) ;
#46585=DIRECTION ( 'NONE',  ( 0.9999697198139515519, 0.000000000000000000, 0.007781995580013368816 ) ) ;
#46586=ORIENTED_EDGE ( 'NONE', *, *, #30229, .F. ) ;
#46587=ADVANCED_FACE ( 'NONE', ( #16427 ), #33749, .F. ) ;
#46588=VERTEX_POINT ( 'NONE', #12176 ) ;
#46589=LINE ( 'NONE', #7708, #49479 ) ;
#46590=VECTOR ( 'NONE', #14247, 999.9999999999998863 ) ;
#46591=DIRECTION ( 'NONE',  ( -0.2426528472758541499, 0.7422098413412800966, -0.6246952433987894571 ) ) ;
#46592=EDGE_CURVE ( 'NONE', #53062, #15552, #42562, .T. ) ;
#46593=EDGE_CURVE ( 'NONE', #29013, #54969, #7944, .T. ) ;
#46594=EDGE_CURVE ( 'NONE', #37965, #20238, #25513, .T. ) ;
#46595=VECTOR ( 'NONE', #15918, 999.9999999999998863 ) ;
#46596=CARTESIAN_POINT ( 'NONE',  ( -20.54204810873173415, 0.000000000000000000, 4.860550213503115558 ) ) ;
#46597=ORIENTED_EDGE ( 'NONE', *, *, #32908, .F. ) ;
#46598=CARTESIAN_POINT ( 'NONE',  ( -13.99061985836883437, 0.9340140483890049250, 3.848629169735781730 ) ) ;
#46599=VERTEX_POINT ( 'NONE', #3651 ) ;
#46600=CARTESIAN_POINT ( 'NONE',  ( -22.42633980038347730, -4.565544526780663581, 5.446808323701739951 ) ) ;
#46601=EDGE_CURVE ( 'NONE', #33592, #5503, #55918, .T. ) ;
#46602=AXIS2_PLACEMENT_3D ( 'NONE', #14643, #14928, #10693 ) ;
#46603=EDGE_LOOP ( 'NONE', ( #53533, #31498, #15974, #17441 ) ) ;
#46604=VECTOR ( 'NONE', #53269, 1000.000000000000227 ) ;
#46605=VERTEX_POINT ( 'NONE', #2791 ) ;
#46607=DIRECTION ( 'NONE',  ( 0.5449076811759707706, 0.6444004775717708799, -0.5364919789714476250 ) ) ;
#46608=DIRECTION ( 'NONE',  ( 0.000000000000000000, -0.000000000000000000, -1.000000000000000000 ) ) ;
#46609=DIRECTION ( 'NONE',  ( -0.5364919789714478471, 0.6444004775717705469, -0.5449076811759709926 ) ) ;
#46611=EDGE_CURVE ( 'NONE', #44519, #7829, #49152, .T. ) ;
#46612=ORIENTED_EDGE ( 'NONE', *, *, #5661, .T. ) ;
#46613=ADVANCED_FACE ( 'NONE', ( #20116 ), #51379, .F. ) ;
#46614=ORIENTED_EDGE ( 'NONE', *, *, #32690, .F. ) ;
#46615=VECTOR ( 'NONE', #36814, 1000.000000000000227 ) ;
#46616=ORIENTED_EDGE ( 'NONE', *, *, #16702, .T. ) ;
#46617=DIRECTION ( 'NONE',  ( 0.5364919789714477361, 0.6444004775717706579, 0.5449076811759711036 ) ) ;
#46618=AXIS2_PLACEMENT_3D ( 'NONE', #44386, #26502, #39596 ) ;
#46619=LINE ( 'NONE', #21643, #36721 ) ;
#46620=ADVANCED_FACE ( 'NONE', ( #29207 ), #51640, .F. ) ;
#46621=ORIENTED_EDGE ( 'NONE', *, *, #1863, .F. ) ;
#46622=FACE_OUTER_BOUND ( 'NONE', #24869, .T. ) ;
#46623=ORIENTED_EDGE ( 'NONE', *, *, #28227, .F. ) ;
#46624=VECTOR ( 'NONE', #32554, 999.9999999999998863 ) ;
#46625=CARTESIAN_POINT ( 'NONE',  ( -17.32775551252169777, -0.1191753592594162470, 8.848214321482844369 ) ) ;
#46626=LINE ( 'NONE', #16246, #1306 ) ;
#46627=EDGE_CURVE ( 'NONE', #13033, #7193, #45992, .T. ) ;
#46628=VERTEX_POINT ( 'NONE', #7640 ) ;
#46629=PLANE ( 'NONE',  #16815 ) ;
#46630=VECTOR ( 'NONE', #34845, 999.9999999999998863 ) ;
#46631=ORIENTED_EDGE ( 'NONE', *, *, #15292, .T. ) ;
#46632=CARTESIAN_POINT ( 'NONE',  ( 2.072287782118878319, 0.000000000000000000, -2.950529333540147015 ) ) ;
#46633=DIRECTION ( 'NONE',  ( -0.005961354470445682716, -0.6427876096865404731, 0.7660212471507180654 ) ) ;
#46634=ORIENTED_EDGE ( 'NONE', *, *, #55716, .F. ) ;
#46636=DIRECTION ( 'NONE',  ( -0.5449076811759708816, 0.6444004775717707689, 0.5364919789714475140 ) ) ;
#46637=DIRECTION ( 'NONE',  ( 0.000000000000000000, -1.000000000000000000, 0.000000000000000000 ) ) ;
#46638=VECTOR ( 'NONE', #41176, 999.9999999999998863 ) ;
#46639=CARTESIAN_POINT ( 'NONE',  ( -18.67619601524082285, 0.000000000000000000, 3.936400510096834893 ) ) ;
#46640=ORIENTED_EDGE ( 'NONE', *, *, #24842, .T. ) ;
#46641=VECTOR ( 'NONE', #33183, 1000.000000000000227 ) ;
#46642=EDGE_LOOP ( 'NONE', ( #6020, #20120, #14102, #16013 ) ) ;
#46643=FACE_OUTER_BOUND ( 'NONE', #4170, .T. ) ;
#46644=CARTESIAN_POINT ( 'NONE',  ( -25.20278734466900517, 0.000000000000000000, 6.670939612111840944 ) ) ;
#46645=DIRECTION ( 'NONE',  ( 0.007781995580012662783, 0.000000000000000000, -0.9999697198139514409 ) ) ;
#46646=DIRECTION ( 'NONE',  ( 0.007781995580012662783, 0.000000000000000000, -0.9999697198139514409 ) ) ;
#46647=DIRECTION ( 'NONE',  ( 0.007781995580012663651, 0.000000000000000000, -0.9999697198139515519 ) ) ;
#46648=AXIS2_PLACEMENT_3D ( 'NONE', #30886, #31742, #43657 ) ;
#46649=VECTOR ( 'NONE', #28365, 1000.000000000000227 ) ;
#46650=DIRECTION ( 'NONE',  ( 0.000000000000000000, -0.000000000000000000, -1.000000000000000000 ) ) ;
#46651=ORIENTED_EDGE ( 'NONE', *, *, #18661, .T. ) ;
#46652=DIRECTION ( 'NONE',  ( 0.007781995580012663651, 0.000000000000000000, -0.9999697198139515519 ) ) ;
#46653=PLANE ( 'NONE',  #38660 ) ;
#46654=ORIENTED_EDGE ( 'NONE', *, *, #26298, .F. ) ;
#46655=LINE ( 'NONE', #32504, #22289 ) ;
#46656=ORIENTED_EDGE ( 'NONE', *, *, #45263, .T. ) ;
#46657=CARTESIAN_POINT ( 'NONE',  ( -11.17520446802705614, 0.000000000000000000, 7.318763589012519333 ) ) ;
#46658=LINE ( 'NONE', #32755, #2466 ) ;
#46659=EDGE_CURVE ( 'NONE', #24728, #9006, #3392, .T. ) ;
#46660=DIRECTION ( 'NONE',  ( 0.005961354470445682716, -0.6427876096865404731, -0.7660212471507180654 ) ) ;
#46661=CARTESIAN_POINT ( 'NONE',  ( -24.26908309836554878, 0.000000000000000000, 6.108867788427308376 ) ) ;
#46663=AXIS2_PLACEMENT_3D ( 'NONE', #40249, #44790, #49625 ) ;
#46664=EDGE_LOOP ( 'NONE', ( #44188, #7650, #18237, #27994 ) ) ;
#46665=ORIENTED_EDGE ( 'NONE', *, *, #21253, .F. ) ;
#46666=AXIS2_PLACEMENT_3D ( 'NONE', #35828, #53151, #5177 ) ;
#46667=DIRECTION ( 'NONE',  ( 0.000000000000000000, -0.000000000000000000, -1.000000000000000000 ) ) ;
#46668=DIRECTION ( 'NONE',  ( 0.6427681459581294776, -0.7660444431189769032, 0.005002170337467562802 ) ) ;
#46670=VECTOR ( 'NONE', #49979, 1000.000000000000227 ) ;
#46671=ADVANCED_FACE ( 'NONE', ( #38877 ), #26636, .F. ) ;
#46672=EDGE_CURVE ( 'NONE', #11685, #34978, #52742, .T. ) ;
#46673=EDGE_CURVE ( 'NONE', #49950, #20904, #25812, .T. ) ;
#46674=DIRECTION ( 'NONE',  ( -0.7660212471507179544, -0.6427876096865405842, -0.005961354470445141482 ) ) ;
#46675=CARTESIAN_POINT ( 'NONE',  ( -18.67697421479882181, -0.1191753592594197858, 4.036397482078229793 ) ) ;
#46676=PLANE ( 'NONE',  #40335 ) ;
#46677=VECTOR ( 'NONE', #9725, 999.9999999999998863 ) ;
#46678=ORIENTED_EDGE ( 'NONE', *, *, #44656, .T. ) ;
#46679=EDGE_CURVE ( 'NONE', #37343, #25250, #18387, .T. ) ;
#46680=CARTESIAN_POINT ( 'NONE',  ( -19.45503627000849889, 0.000000000000000000, 7.556996783084074742 ) ) ;
#46681=PLANE ( 'NONE',  #36845 ) ;
#46682=CARTESIAN_POINT ( 'NONE',  ( -14.16629225735672115, -0.8417996532631574214, 2.357132303004818130 ) ) ;
#46683=ORIENTED_EDGE ( 'NONE', *, *, #50432, .F. ) ;
#46684=AXIS2_PLACEMENT_3D ( 'NONE', #33560, #8576, #25067 ) ;
#46685=DIRECTION ( 'NONE',  ( 0.000000000000000000, -0.000000000000000000, -1.000000000000000000 ) ) ;
#46686=FACE_OUTER_BOUND ( 'NONE', #51782, .T. ) ;
#46687=FACE_OUTER_BOUND ( 'NONE', #36515, .T. ) ;
#46688=AXIS2_PLACEMENT_3D ( 'NONE', #39759, #577, #44003 ) ;
#46689=VERTEX_POINT ( 'NONE', #47676 ) ;
#46691=ORIENTED_EDGE ( 'NONE', *, *, #29487, .T. ) ;
#46692=EDGE_CURVE ( 'NONE', #44862, #30431, #17865, .T. ) ;
#46693=VECTOR ( 'NONE', #32240, 1000.000000000000000 ) ;
#46694=ORIENTED_EDGE ( 'NONE', *, *, #50759, .T. ) ;
#46695=VECTOR ( 'NONE', #52942, 999.9999999999998863 ) ;
#46696=ORIENTED_EDGE ( 'NONE', *, *, #45706, .F. ) ;
#46697=EDGE_CURVE ( 'NONE', #16476, #44308, #52212, .T. ) ;
#46698=ORIENTED_EDGE ( 'NONE', *, *, #31713, .T. ) ;
#46699=DIRECTION ( 'NONE',  ( -0.5364919789714478471, 0.6444004775717705469, -0.5449076811759709926 ) ) ;
#46700=VERTEX_POINT ( 'NONE', #31179 ) ;
#46701=PLANE ( 'NONE',  #52158 ) ;
#46702=EDGE_CURVE ( 'NONE', #18842, #39017, #43665, .T. ) ;
#46703=VERTEX_POINT ( 'NONE', #21562 ) ;
#46704=PLANE ( 'NONE',  #36799 ) ;
#46705=ORIENTED_EDGE ( 'NONE', *, *, #32567, .T. ) ;
#46707=EDGE_CURVE ( 'NONE', #39606, #18021, #44253, .T. ) ;
#46708=AXIS2_PLACEMENT_3D ( 'NONE', #38430, #24810, #50378 ) ;
#46709=LINE ( 'NONE', #16906, #42000 ) ;
#46710=AXIS2_PLACEMENT_3D ( 'NONE', #37976, #26057, #51008 ) ;
#46711=CARTESIAN_POINT ( 'NONE',  ( -15.33351336157133105, -1.651309408375655874, 5.348069112848596873 ) ) ;
#46713=FACE_OUTER_BOUND ( 'NONE', #11208, .T. ) ;
#46715=VECTOR ( 'NONE', #18152, 1000.000000000000227 ) ;
#46716=ORIENTED_EDGE ( 'NONE', *, *, #14638, .F. ) ;
#46717=ORIENTED_EDGE ( 'NONE', *, *, #47322, .F. ) ;
#46718=CARTESIAN_POINT ( 'NONE',  ( -18.82244137458435063, 0.000000000000000000, 8.936585358602211926 ) ) ;
#46719=CARTESIAN_POINT ( 'NONE',  ( -10.74029228357944987, 0.000000000000000000, 11.14194120806293320 ) ) ;
#46720=AXIS2_PLACEMENT_3D ( 'NONE', #20928, #38253, #4212 ) ;
#46722=CARTESIAN_POINT ( 'NONE',  ( -16.79925329029790149, 0.000000000000000000, 13.49544742625427496 ) ) ;
#46723=VECTOR ( 'NONE', #1780, 1000.000000000000227 ) ;
#46724=VECTOR ( 'NONE', #2352, 1000.000000000000000 ) ;
#46725=DIRECTION ( 'NONE',  ( 0.9999697198139515519, 0.000000000000000000, 0.007781995580013368816 ) ) ;
#46726=VECTOR ( 'NONE', #39619, 1000.000000000000227 ) ;
#46727=DIRECTION ( 'NONE',  ( -0.005002170337468016433, -0.7660444431189770143, 0.6427681459581293666 ) ) ;
#46728=PLANE ( 'NONE',  #5102 ) ;
#46730=DIRECTION ( 'NONE',  ( 0.2426528472758541499, 0.7422098413412800966, 0.6246952433987894571 ) ) ;
#46731=CARTESIAN_POINT ( 'NONE',  ( -8.875996589204540044, 0.000000000000000000, 10.41778544861944233 ) ) ;
#46732=ORIENTED_EDGE ( 'NONE', *, *, #5627, .T. ) ;
#46733=VECTOR ( 'NONE', #10438, 999.9999999999998863 ) ;
#46734=DIRECTION ( 'NONE',  ( 0.000000000000000000, -1.000000000000000000, 0.000000000000000000 ) ) ;
#46735=CARTESIAN_POINT ( 'NONE',  ( 2.072287782118878319, 0.000000000000000000, -2.950529333540147015 ) ) ;
#46736=VECTOR ( 'NONE', #38099, 999.9999999999998863 ) ;
#46737=PLANE ( 'NONE',  #49897 ) ;
#46738=DIRECTION ( 'NONE',  ( 0.005002170337468016433, -0.7660444431189770143, -0.6427681459581293666 ) ) ;
#46739=FACE_OUTER_BOUND ( 'NONE', #53153, .T. ) ;
#46740=VECTOR ( 'NONE', #5989, 1000.000000000000227 ) ;
#46741=VERTEX_POINT ( 'NONE', #53046 ) ;
#46742=VECTOR ( 'NONE', #25100, 1000.000000000000227 ) ;
#46743=ORIENTED_EDGE ( 'NONE', *, *, #48981, .T. ) ;
#46744=CARTESIAN_POINT ( 'NONE',  ( -9.110551994824897193, 0.000000000000000000, 3.538847790438064411 ) ) ;
#46746=CARTESIAN_POINT ( 'NONE',  ( -20.54204810873173415, 0.000000000000000000, 4.860550213503115558 ) ) ;
#46747=EDGE_CURVE ( 'NONE', #547, #26572, #1058, .T. ) ;
#46748=CARTESIAN_POINT ( 'NONE',  ( -15.43560933383329292, -0.6798977022406551551, 3.793474551966180108 ) ) ;
#46749=CARTESIAN_POINT ( 'NONE',  ( -17.74560456716937296, 0.000000000000000000, 3.774316574337878372 ) ) ;
#46750=EDGE_CURVE ( 'NONE', #35444, #37821, #18116, .T. ) ;
#46751=DIRECTION ( 'NONE',  ( -0.9999697198139514409, -0.000000000000000000, -0.007781995580013368816 ) ) ;
#46752=EDGE_CURVE ( 'NONE', #4570, #4586, #35190, .T. ) ;
#46753=DIRECTION ( 'NONE',  ( 0.000000000000000000, -1.000000000000000000, 0.000000000000000000 ) ) ;
#46754=AXIS2_PLACEMENT_3D ( 'NONE', #43729, #12540, #17924 ) ;
#46755=DIRECTION ( 'NONE',  ( -0.005002170337468016433, -0.7660444431189770143, 0.6427681459581293666 ) ) ;
#46757=AXIS2_PLACEMENT_3D ( 'NONE', #19752, #54644, #37914 ) ;
#46758=DIRECTION ( 'NONE',  ( -0.7660212471507179544, -0.6427876096865405842, -0.005961354470445141482 ) ) ;
#46759=ORIENTED_EDGE ( 'NONE', *, *, #32582, .T. ) ;
#46760=DIRECTION ( 'NONE',  ( 0.007781995580012663651, -3.146120232559066537E-19, -0.9999697198139514409 ) ) ;
#46761=VECTOR ( 'NONE', #34500, 1000.000000000000227 ) ;
#46762=ORIENTED_EDGE ( 'NONE', *, *, #20724, .F. ) ;
#46764=ORIENTED_EDGE ( 'NONE', *, *, #43336, .T. ) ;
#46765=EDGE_LOOP ( 'NONE', ( #25507, #4868, #19064, #18905 ) ) ;
#46766=ORIENTED_EDGE ( 'NONE', *, *, #44883, .F. ) ;
#46767=AXIS2_PLACEMENT_3D ( 'NONE', #54312, #7746, #25074 ) ;
#46768=VECTOR ( 'NONE', #36792, 1000.000000000000000 ) ;
#46769=ORIENTED_EDGE ( 'NONE', *, *, #20659, .F. ) ;
#46770=VERTEX_POINT ( 'NONE', #9622 ) ;
#46771=DIRECTION ( 'NONE',  ( 0.000000000000000000, -1.000000000000000000, 0.000000000000000000 ) ) ;
#46772=LINE ( 'NONE', #7893, #24772 ) ;
#46773=FACE_OUTER_BOUND ( 'NONE', #32254, .T. ) ;
#46774=VECTOR ( 'NONE', #50064, 999.9999999999998863 ) ;
#46775=VECTOR ( 'NONE', #15479, 999.9999999999998863 ) ;
#46776=ORIENTED_EDGE ( 'NONE', *, *, #4393, .T. ) ;
#46777=CARTESIAN_POINT ( 'NONE',  ( -27.06708303904391144, 0.000000000000000000, 7.395095371555332697 ) ) ;
#46778=ORIENTED_EDGE ( 'NONE', *, *, #6770, .T. ) ;
#46779=CARTESIAN_POINT ( 'NONE',  ( -14.20280369269832832, 0.000000000000000000, 12.40765738797303719 ) ) ;
#46780=ORIENTED_EDGE ( 'NONE', *, *, #54971, .T. ) ;
#46781=EDGE_CURVE ( 'NONE', #50643, #3193, #43138, .T. ) ;
#46782=AXIS2_PLACEMENT_3D ( 'NONE', #27140, #44448, #5551 ) ;
#46783=VECTOR ( 'NONE', #20037, 1000.000000000000227 ) ;
#46785=ADVANCED_FACE ( 'NONE', ( #22663 ), #39973, .F. ) ;
#46786=LINE ( 'NONE', #52636, #43689 ) ;
#46788=EDGE_LOOP ( 'NONE', ( #53475, #37452, #50186, #13795 ) ) ;
#46789=CARTESIAN_POINT ( 'NONE',  ( -16.76809155115178385, 0.000000000000000000, 9.491230867342991928 ) ) ;
#46790=VERTEX_POINT ( 'NONE', #8485 ) ;
#46791=CARTESIAN_POINT ( 'NONE',  ( -19.25258962936204199, 0.000000000000000000, 4.501253007741028433 ) ) ;
#46792=EDGE_CURVE ( 'NONE', #37525, #29163, #51907, .T. ) ;
#46793=LINE ( 'NONE', #7909, #1221 ) ;
#46794=VECTOR ( 'NONE', #35654, 999.9999999999998863 ) ;
#46795=DIRECTION ( 'NONE',  ( -0.7660212471507179544, -0.6427876096865405842, -0.005961354470445141482 ) ) ;
#46796=DIRECTION ( 'NONE',  ( 0.005961354470445682716, -0.6427876096865404731, -0.7660212471507180654 ) ) ;
#46797=DIRECTION ( 'NONE',  ( 0.000000000000000000, -0.000000000000000000, -1.000000000000000000 ) ) ;
#46799=CARTESIAN_POINT ( 'NONE',  ( -16.81190032086591302, 0.000000000000000000, 3.212244750653343583 ) ) ;
#46800=CARTESIAN_POINT ( 'NONE',  ( -16.99924723426068951, 0.000000000000000000, 13.49389102713827171 ) ) ;
#46801=ORIENTED_EDGE ( 'NONE', *, *, #41297, .T. ) ;
#46802=DIRECTION ( 'NONE',  ( 0.000000000000000000, -1.000000000000000000, 0.000000000000000000 ) ) ;
#46803=ORIENTED_EDGE ( 'NONE', *, *, #46821, .T. ) ;
#46804=AXIS2_PLACEMENT_3D ( 'NONE', #32216, #19129, #15427 ) ;
#46805=LINE ( 'NONE', #38852, #51914 ) ;
#46806=PLANE ( 'NONE',  #31471 ) ;
#46807=CARTESIAN_POINT ( 'NONE',  ( -8.875996589204540044, 0.000000000000000000, 10.41778544861944233 ) ) ;
#46808=AXIS2_PLACEMENT_3D ( 'NONE', #12722, #34030, #16145 ) ;
#46809=CARTESIAN_POINT ( 'NONE',  ( -11.77243710274829525, -0.1191753592594197858, 11.50324088822667612 ) ) ;
#46810=DIRECTION ( 'NONE',  ( 0.000000000000000000, -0.000000000000000000, -1.000000000000000000 ) ) ;
#46811=VECTOR ( 'NONE', #9356, 999.9999999999998863 ) ;
#46812=CARTESIAN_POINT ( 'NONE',  ( -9.954103585529763265, 0.000000000000000000, 3.834951836585689389 ) ) ;
#46813=AXIS2_PLACEMENT_3D ( 'NONE', #41269, #7451, #15414 ) ;
#46814=ORIENTED_EDGE ( 'NONE', *, *, #25324, .F. ) ;
#46815=LINE ( 'NONE', #32896, #30143 ) ;
#46817=DIRECTION ( 'NONE',  ( 0.7660212471507180654, -0.6427876096865404731, 0.005961354470445141482 ) ) ;
#46818=EDGE_CURVE ( 'NONE', #36758, #51910, #34593, .T. ) ;
#46819=FACE_OUTER_BOUND ( 'NONE', #16903, .T. ) ;
#46820=VECTOR ( 'NONE', #24852, 1000.000000000000227 ) ;
#46821=EDGE_CURVE ( 'NONE', #49645, #37012, #22102, .T. ) ;
#46822=VECTOR ( 'NONE', #49524, 999.9999999999998863 ) ;
#46823=DIRECTION ( 'NONE',  ( 0.000000000000000000, -1.000000000000000000, 0.000000000000000000 ) ) ;
#46824=LINE ( 'NONE', #48794, #4016 ) ;
#46825=CARTESIAN_POINT ( 'NONE',  ( -14.10280672071693431, -0.1191753592594197858, 12.40843558753103792 ) ) ;
#46826=EDGE_CURVE ( 'NONE', #4575, #3699, #26103, .T. ) ;
#46827=CARTESIAN_POINT ( 'NONE',  ( -13.93584171313674958, 0.000000000000000000, 3.803965029789607044 ) ) ;
#46828=VERTEX_POINT ( 'NONE', #39136 ) ;
#46829=VECTOR ( 'NONE', #31260, 999.9999999999998863 ) ;
#46830=AXIS2_PLACEMENT_3D ( 'NONE', #25110, #46107, #42420 ) ;
#46831=FACE_OUTER_BOUND ( 'NONE', #27567, .T. ) ;
#46832=DIRECTION ( 'NONE',  ( 0.5364919789714477361, 0.6444004775717706579, 0.5449076811759711036 ) ) ;
#46833=ORIENTED_EDGE ( 'NONE', *, *, #9128, .F. ) ;
#46834=VERTEX_POINT ( 'NONE', #30648 ) ;
#46835=DIRECTION ( 'NONE',  ( 0.9999697198139515519, 0.000000000000000000, 0.007781995580013368816 ) ) ;
#46838=LINE ( 'NONE', #2795, #50159 ) ;
#46839=VECTOR ( 'NONE', #11384, 999.9999999999998863 ) ;
#46840=EDGE_CURVE ( 'NONE', #31761, #20073, #18698, .T. ) ;
#46841=ORIENTED_EDGE ( 'NONE', *, *, #33178, .F. ) ;
#46843=EDGE_LOOP ( 'NONE', ( #48353, #44698, #3114, #1642 ) ) ;
#46844=LINE ( 'NONE', #3945, #19322 ) ;
#46845=DIRECTION ( 'NONE',  ( -0.7660212471507179544, -0.6427876096865405842, -0.005961354470445141482 ) ) ;
#46846=VECTOR ( 'NONE', #23551, 1000.000000000000114 ) ;
#46847=CARTESIAN_POINT ( 'NONE',  ( -15.88788263391494660, -0.1191753592594200495, 2.953019594114145274 ) ) ;
#46849=EDGE_LOOP ( 'NONE', ( #9717, #39603, #24444, #29622 ) ) ;
#46850=ORIENTED_EDGE ( 'NONE', *, *, #10986, .T. ) ;
#46851=AXIS2_PLACEMENT_3D ( 'NONE', #38199, #46426, #50441 ) ;
#46852=LINE ( 'NONE', #7366, #48421 ) ;
#46853=CARTESIAN_POINT ( 'NONE',  ( -15.87975247367846166, 0.000000000000000000, 2.850166870931599927 ) ) ;
#46854=ORIENTED_EDGE ( 'NONE', *, *, #49593, .T. ) ;
#46856=DIRECTION ( 'NONE',  ( 0.5449076811759707706, 0.6444004775717708799, -0.5364919789714476250 ) ) ;
#46857=ORIENTED_EDGE ( 'NONE', *, *, #23661, .F. ) ;
#46858=PLANE ( 'NONE',  #31226 ) ;
#46859=DIRECTION ( 'NONE',  ( 0.007781995580012662783, 0.000000000000000000, -0.9999697198139514409 ) ) ;
#46860=VERTEX_POINT ( 'NONE', #31748 ) ;
#46861=AXIS2_PLACEMENT_3D ( 'NONE', #4806, #39461, #52510 ) ;
#46862=DIRECTION ( 'NONE',  ( 0.5364919789714477361, 0.6444004775717706579, 0.5449076811759711036 ) ) ;
#46863=EDGE_CURVE ( 'NONE', #5052, #33621, #49054, .T. ) ;
#46864=VECTOR ( 'NONE', #46534, 999.9999999999998863 ) ;
#46865=CARTESIAN_POINT ( 'NONE',  ( -17.42409743439815983, 2.017525632630139398, 12.78552735456895739 ) ) ;
#46866=AXIS2_PLACEMENT_3D ( 'NONE', #32383, #19283, #49935 ) ;
#46867=ORIENTED_EDGE ( 'NONE', *, *, #37307, .T. ) ;
#46868=PLANE ( 'NONE',  #8632 ) ;
#46869=FACE_OUTER_BOUND ( 'NONE', #34335, .T. ) ;
#46870=CARTESIAN_POINT ( 'NONE',  ( -11.33783571642116783, 0.000000000000000000, 2.516181047545578586 ) ) ;
#46871=CARTESIAN_POINT ( 'NONE',  ( -1.451368222102410455, 5.185123052344191130, 3.782134281800667797 ) ) ;
#46872=VERTEX_POINT ( 'NONE', #27200 ) ;
#46873=EDGE_CURVE ( 'NONE', #34917, #21011, #41090, .T. ) ;
#46874=LINE ( 'NONE', #3688, #6568 ) ;
#46875=DIRECTION ( 'NONE',  ( 0.000000000000000000, -1.000000000000000000, 0.000000000000000000 ) ) ;
#46876=LINE ( 'NONE', #21006, #18545 ) ;
#46877=CARTESIAN_POINT ( 'NONE',  ( -12.01504067337997483, -3.270328918600661439, 1.444030332666087268 ) ) ;
#46878=EDGE_CURVE ( 'NONE', #55101, #54363, #53868, .T. ) ;
#46879=DIRECTION ( 'NONE',  ( -0.6427681459581293666, -0.7660444431189770143, -0.005002170337467561935 ) ) ;
#46880=FACE_OUTER_BOUND ( 'NONE', #30457, .T. ) ;
#46881=EDGE_CURVE ( 'NONE', #16954, #349, #10983, .T. ) ;
#46882=VECTOR ( 'NONE', #622, 1000.000000000000227 ) ;
#46883=LINE ( 'NONE', #54819, #36718 ) ;
#46885=CARTESIAN_POINT ( 'NONE',  ( -20.06674461129317422, -3.917936722690659401, 10.90653844675688156 ) ) ;
#46886=EDGE_LOOP ( 'NONE', ( #88, #28172, #50611, #35344 ) ) ;
#46887=FACE_OUTER_BOUND ( 'NONE', #20815, .T. ) ;
#46888=EDGE_CURVE ( 'NONE', #19170, #17361, #44799, .T. ) ;
#46889=DIRECTION ( 'NONE',  ( 0.000000000000000000, -0.000000000000000000, -1.000000000000000000 ) ) ;
#46890=EDGE_CURVE ( 'NONE', #22139, #28250, #23238, .T. ) ;
#46891=VECTOR ( 'NONE', #17789, 999.9999999999998863 ) ;
#46892=DIRECTION ( 'NONE',  ( 0.6427681459581294776, -0.7660444431189769032, 0.005002170337467562802 ) ) ;
#46893=CARTESIAN_POINT ( 'NONE',  ( -14.26657388737785936, -2.622721114510660367, 2.339264374922224388 ) ) ;
#46894=EDGE_CURVE ( 'NONE', #40362, #25201, #10737, .T. ) ;
#46895=LINE ( 'NONE', #26998, #7518 ) ;
#46896=EDGE_LOOP ( 'NONE', ( #44717, #22775, #19683, #47240 ) ) ;
#46897=VECTOR ( 'NONE', #44168, 999.9999999999998863 ) ;
#46898=VERTEX_POINT ( 'NONE', #15265 ) ;
#46899=LINE ( 'NONE', #37822, #39509 ) ;
#46900=LINE ( 'NONE', #52279, #53134 ) ;
#46901=ORIENTED_EDGE ( 'NONE', *, *, #46297, .F. ) ;
#46903=ADVANCED_FACE ( 'NONE', ( #45622 ), #44505, .F. ) ;
#46904=VECTOR ( 'NONE', #43023, 1000.000000000000114 ) ;
#46905=ORIENTED_EDGE ( 'NONE', *, *, #16058, .F. ) ;
#46906=CARTESIAN_POINT ( 'NONE',  ( -12.23851102634202448, -0.1191753592594197858, 11.68427982808754884 ) ) ;
#46907=ORIENTED_EDGE ( 'NONE', *, *, #851, .T. ) ;
#46908=DIRECTION ( 'NONE',  ( 0.000000000000000000, -1.000000000000000000, 0.000000000000000000 ) ) ;
#46909=EDGE_CURVE ( 'NONE', #13509, #28907, #18970, .T. ) ;
#46910=ORIENTED_EDGE ( 'NONE', *, *, #7013, .F. ) ;
#46911=ORIENTED_EDGE ( 'NONE', *, *, #39377, .F. ) ;
#46912=VERTEX_POINT ( 'NONE', #14163 ) ;
#46913=DIRECTION ( 'NONE',  ( -0.5364919789714478471, 0.6444004775717705469, -0.5449076811759709926 ) ) ;
#46914=PLANE ( 'NONE',  #30509 ) ;
#46915=DIRECTION ( 'NONE',  ( 0.007781995580012663651, -3.146120232559066537E-19, -0.9999697198139514409 ) ) ;
#46916=CARTESIAN_POINT ( 'NONE',  ( -19.16801431701463443, 4.333955019861511992, 3.989163584846405985 ) ) ;
#46917=EDGE_LOOP ( 'NONE', ( #46016, #39734, #14015, #1967 ) ) ;
#46918=ORIENTED_EDGE ( 'NONE', *, *, #12951, .F. ) ;
#46919=VERTEX_POINT ( 'NONE', #53588 ) ;
#46920=CARTESIAN_POINT ( 'NONE',  ( -14.10280672071693431, -0.1191753592594197858, 12.40843558753103792 ) ) ;
#46921=CARTESIAN_POINT ( 'NONE',  ( -14.03425665725284865, 0.4483081953215033444, 2.119010243948319161 ) ) ;
#46922=VERTEX_POINT ( 'NONE', #31487 ) ;
#46923=CARTESIAN_POINT ( 'NONE',  ( -27.99767448711536133, 0.000000000000000000, 7.557179307314289218 ) ) ;
#46924=ORIENTED_EDGE ( 'NONE', *, *, #10264, .F. ) ;
#46925=DIRECTION ( 'NONE',  ( 0.007781995580012663651, -3.146120232559066537E-19, -0.9999697198139514409 ) ) ;
#46926=CARTESIAN_POINT ( 'NONE',  ( 2.072287782118878319, 0.000000000000000000, -2.950529333540147015 ) ) ;
#46927=EDGE_LOOP ( 'NONE', ( #32785, #9332, #42507, #48430 ) ) ;
#46928=FACE_OUTER_BOUND ( 'NONE', #16593, .T. ) ;
#46929=EDGE_CURVE ( 'NONE', #7041, #1224, #36556, .T. ) ;
#46931=VECTOR ( 'NONE', #54090, 1000.000000000000227 ) ;
#46932=CARTESIAN_POINT ( 'NONE',  ( -10.27421835998572064, 0.000000000000000000, 10.96090226820206048 ) ) ;
#46933=LINE ( 'NONE', #25611, #53845 ) ;
#46934=ORIENTED_EDGE ( 'NONE', *, *, #41643, .F. ) ;
#46935=DIRECTION ( 'NONE',  ( 0.000000000000000000, -0.000000000000000000, -1.000000000000000000 ) ) ;
#46936=DIRECTION ( 'NONE',  ( 0.007781995580012663651, 0.000000000000000000, -0.9999697198139515519 ) ) ;
#46937=CARTESIAN_POINT ( 'NONE',  ( -15.76926926996742573, 4.172053068839010947, 2.674141106593023842 ) ) ;
#46938=CARTESIAN_POINT ( 'NONE',  ( -16.81190032086591302, 0.000000000000000000, 3.212244750653343583 ) ) ;
#46939=ORIENTED_EDGE ( 'NONE', *, *, #49838, .F. ) ;
#46940=EDGE_CURVE ( 'NONE', #31213, #15482, #14986, .T. ) ;
#46941=ORIENTED_EDGE ( 'NONE', *, *, #38950, .F. ) ;
#46942=AXIS2_PLACEMENT_3D ( 'NONE', #26602, #39944, #5583 ) ;
#46943=FACE_OUTER_BOUND ( 'NONE', #51448, .T. ) ;
#46944=CARTESIAN_POINT ( 'NONE',  ( -18.35559287531120987, -2.460819163488158878, 7.850490845989765987 ) ) ;
#46945=LINE ( 'NONE', #42, #53094 ) ;
#46946=PLANE ( 'NONE',  #19448 ) ;
#46947=CARTESIAN_POINT ( 'NONE',  ( -20.06177075545399191, 0.000000000000000000, 14.76272000528038220 ) ) ;
#46948=EDGE_CURVE ( 'NONE', #19740, #1987, #48798, .T. ) ;
#46949=CARTESIAN_POINT ( 'NONE',  ( -13.49707129784320436, 0.000000000000000000, 7.131368270877496585 ) ) ;
#46950=VERTEX_POINT ( 'NONE', #22938 ) ;
#46951=PLANE ( 'NONE',  #11391 ) ;
#46952=LINE ( 'NONE', #7773, #19606 ) ;
#46953=ORIENTED_EDGE ( 'NONE', *, *, #14142, .F. ) ;
#46954=LINE ( 'NONE', #47501, #14107 ) ;
#46955=VERTEX_POINT ( 'NONE', #1350 ) ;
#46956=PLANE ( 'NONE',  #8967 ) ;
#46957=DIRECTION ( 'NONE',  ( -0.005002170337468016433, -0.7660444431189770143, 0.6427681459581293666 ) ) ;
#46958=ADVANCED_FACE ( 'NONE', ( #36034 ), #49635, .F. ) ;
#46959=CARTESIAN_POINT ( 'NONE',  ( -14.46888367232926420, 0.000000000000000000, 12.59025272694991315 ) ) ;
#46960=PLANE ( 'NONE',  #44111 ) ;
#46961=EDGE_CURVE ( 'NONE', #6604, #36649, #32019, .T. ) ;
#46963=VERTEX_POINT ( 'NONE', #27780 ) ;
#46966=LINE ( 'NONE', #37595, #5011 ) ;
#46967=DIRECTION ( 'NONE',  ( 0.000000000000000000, -1.000000000000000000, 0.000000000000000000 ) ) ;
#46968=LINE ( 'NONE', #38432, #29564 ) ;
#46969=EDGE_CURVE ( 'NONE', #43426, #46161, #6203, .T. ) ;
#46970=LINE ( 'NONE', #39277, #13813 ) ;
#46971=PLANE ( 'NONE',  #37616 ) ;
#46972=ORIENTED_EDGE ( 'NONE', *, *, #25933, .F. ) ;
#46973=FACE_OUTER_BOUND ( 'NONE', #37864, .T. ) ;
#46974=CARTESIAN_POINT ( 'NONE',  ( -13.49209884813190818, -3.917936722690662954, 1.997107809296931658 ) ) ;
#46975=PLANE ( 'NONE',  #1530 ) ;
#46976=ORIENTED_EDGE ( 'NONE', *, *, #48806, .F. ) ;
#46977=DIRECTION ( 'NONE',  ( 0.5364919789714477361, 0.6444004775717706579, 0.5449076811759711036 ) ) ;
#46979=FACE_OUTER_BOUND ( 'NONE', #38821, .T. ) ;
#46980=ORIENTED_EDGE ( 'NONE', *, *, #35710, .T. ) ;
#46981=VECTOR ( 'NONE', #37497, 999.9999999999998863 ) ;
#46982=FACE_OUTER_BOUND ( 'NONE', #54605, .T. ) ;
#46983=ORIENTED_EDGE ( 'NONE', *, *, #26749, .F. ) ;
#46984=ORIENTED_EDGE ( 'NONE', *, *, #47849, .T. ) ;
#46985=ORIENTED_EDGE ( 'NONE', *, *, #40950, .F. ) ;
#46986=ORIENTED_EDGE ( 'NONE', *, *, #7457, .F. ) ;
#46987=CARTESIAN_POINT ( 'NONE',  ( -18.76354595665420177, -0.1191753592594177458, 14.21882498613976331 ) ) ;
#46988=ORIENTED_EDGE ( 'NONE', *, *, #22344, .F. ) ;
#46989=EDGE_CURVE ( 'NONE', #38231, #7720, #28044, .T. ) ;
#46990=DIRECTION ( 'NONE',  ( -0.7660212471507179544, -0.6427876096865405842, -0.005961354470445141482 ) ) ;
#46991=VERTEX_POINT ( 'NONE', #41640 ) ;
#46992=PLANE ( 'NONE',  #7770 ) ;
#46993=ORIENTED_EDGE ( 'NONE', *, *, #34585, .T. ) ;
#46994=EDGE_CURVE ( 'NONE', #33913, #36677, #7565, .T. ) ;
#46995=ORIENTED_EDGE ( 'NONE', *, *, #54831, .F. ) ;
#46996=CARTESIAN_POINT ( 'NONE',  ( -12.60458797795435615, 0.000000000000000000, 11.86609696750642229 ) ) ;
#46997=DIRECTION ( 'NONE',  ( 0.5364919789714477361, 0.6444004775717706579, 0.5449076811759711036 ) ) ;
#46998=ADVANCED_FACE ( 'NONE', ( #3860 ), #29742, .F. ) ;
#46999=CARTESIAN_POINT ( 'NONE',  ( -24.26908309836554878, 0.000000000000000000, 6.108867788427308376 ) ) ;
#47000=DIRECTION ( 'NONE',  ( 0.5449076811759707706, 0.6444004775717708799, -0.5364919789714476250 ) ) ;
#47001=CARTESIAN_POINT ( 'NONE',  ( -17.20841836556132876, 0.000000000000000000, 6.363821570217892187 ) ) ;
#47002=ORIENTED_EDGE ( 'NONE', *, *, #28155, .T. ) ;
#47003=ADVANCED_FACE ( 'NONE', ( #12417 ), #24593, .T. ) ;
#47004=ADVANCED_FACE ( 'NONE', ( #20344 ), #55265, .F. ) ;
#47005=ADVANCED_FACE ( 'NONE', ( #47039 ), #8139, .F. ) ;
#47006=ORIENTED_EDGE ( 'NONE', *, *, #46840, .F. ) ;
#47009=CARTESIAN_POINT ( 'NONE',  ( -19.94981257973373090, -1.391042808123044372, 6.283224763914724953 ) ) ;
#47010=LINE ( 'NONE', #42183, #28521 ) ;
#47011=DIRECTION ( 'NONE',  ( 0.9999697198139515519, 0.000000000000000000, 0.007781995580013368816 ) ) ;
#47012=LINE ( 'NONE', #51272, #35919 ) ;
#47014=LINE ( 'NONE', #47863, #33792 ) ;
#47015=DIRECTION ( 'NONE',  ( 0.000000000000000000, -1.000000000000000000, 0.000000000000000000 ) ) ;
#47016=ORIENTED_EDGE ( 'NONE', *, *, #42107, .F. ) ;
#47017=AXIS2_PLACEMENT_3D ( 'NONE', #22452, #52526, #39760 ) ;
#47018=CARTESIAN_POINT ( 'NONE',  ( -15.60102546347950536, 0.000000000000000000, 12.95077420755565356 ) ) ;
#47019=FACE_OUTER_BOUND ( 'NONE', #36985, .T. ) ;
#47020=LINE ( 'NONE', #52595, #33612 ) ;
#47021=EDGE_CURVE ( 'NONE', #33592, #22613, #3589, .T. ) ;
#47022=DIRECTION ( 'NONE',  ( 0.000000000000000000, -1.000000000000000000, 0.000000000000000000 ) ) ;
#47023=LINE ( 'NONE', #50715, #46783 ) ;
#47024=EDGE_CURVE ( 'NONE', #54767, #42084, #12101, .T. ) ;
#47025=ORIENTED_EDGE ( 'NONE', *, *, #2626, .F. ) ;
#47027=EDGE_CURVE ( 'NONE', #36758, #12750, #50728, .T. ) ;
#47029=LINE ( 'NONE', #20041, #30430 ) ;
#47030=CARTESIAN_POINT ( 'NONE',  ( -10.94028622754223967, 0.000000000000000000, 11.14038480894692995 ) ) ;
#47031=EDGE_CURVE ( 'NONE', #22170, #17803, #11820, .T. ) ;
#47032=LINE ( 'NONE', #47589, #22814 ) ;
#47033=LINE ( 'NONE', #55259, #39417 ) ;
#47034=CARTESIAN_POINT ( 'NONE',  ( -9.110551994824897193, -1.000000000000000000, 3.538847790438064411 ) ) ;
#47035=PLANE ( 'NONE',  #13888 ) ;
#47036=EDGE_CURVE ( 'NONE', #28250, #34243, #20050, .T. ) ;
#47037=CARTESIAN_POINT ( 'NONE',  ( -14.00280974873554030, 0.000000000000000000, 12.40921378708904044 ) ) ;
#47039=FACE_OUTER_BOUND ( 'NONE', #44031, .T. ) ;
#47040=ORIENTED_EDGE ( 'NONE', *, *, #20051, .F. ) ;
#47041=DIRECTION ( 'NONE',  ( 0.9999697198139515519, 0.000000000000000000, 0.007781995580013368816 ) ) ;
#47042=ORIENTED_EDGE ( 'NONE', *, *, #23561, .F. ) ;
#47043=EDGE_LOOP ( 'NONE', ( #29969, #37516, #4515, #3267 ) ) ;
#47044=ORIENTED_EDGE ( 'NONE', *, *, #25193, .F. ) ;
#47046=ORIENTED_EDGE ( 'NONE', *, *, #39732, .T. ) ;
#47047=ORIENTED_EDGE ( 'NONE', *, *, #45964, .T. ) ;
#47048=CARTESIAN_POINT ( 'NONE',  ( -18.42808488909577846, -4.727446477803161073, 11.59857078128931995 ) ) ;
#47049=LINE ( 'NONE', #20356, #51968 ) ;
#47050=LINE ( 'NONE', #55279, #30320 ) ;
#47051=VECTOR ( 'NONE', #16860, 999.9999999999998863 ) ;
#47052=ORIENTED_EDGE ( 'NONE', *, *, #4620, .T. ) ;
#47053=LINE ( 'NONE', #25464, #53045 ) ;
#47054=ORIENTED_EDGE ( 'NONE', *, *, #3433, .T. ) ;
#47055=PLANE ( 'NONE',  #12274 ) ;
#47056=ORIENTED_EDGE ( 'NONE', *, *, #7920, .F. ) ;
#47058=LINE ( 'NONE', #38241, #34619 ) ;
#47059=CARTESIAN_POINT ( 'NONE',  ( -22.40556560354864146, -0.1191753592594197858, 5.484709000965211523 ) ) ;
#47060=ORIENTED_EDGE ( 'NONE', *, *, #14690, .F. ) ;
#47061=CARTESIAN_POINT ( 'NONE',  ( -17.90178974141802470, 0.000000000000000000, 10.05174629191152391 ) ) ;
#47062=EDGE_LOOP ( 'NONE', ( #29864, #44034, #51749, #52651, #37575 ) ) ;
#47063=EDGE_CURVE ( 'NONE', #7707, #28385, #42497, .T. ) ;
#47064=EDGE_CURVE ( 'NONE', #10235, #49289, #29138, .T. ) ;
#47065=LINE ( 'NONE', #38840, #29132 ) ;
#47066=DIRECTION ( 'NONE',  ( 0.005961354470445682716, -0.6427876096865404731, -0.7660212471507180654 ) ) ;
#47067=EDGE_CURVE ( 'NONE', #16632, #36484, #42756, .T. ) ;
#47068=CARTESIAN_POINT ( 'NONE',  ( -17.06301742894022055, -2.622721114510660367, 3.425498014087459797 ) ) ;
#47069=CARTESIAN_POINT ( 'NONE',  ( 2.072287782118878319, 0.000000000000000000, -2.950529333540147015 ) ) ;
#47070=DIRECTION ( 'NONE',  ( 0.005961354470445682716, -0.6427876096865404731, -0.7660212471507180654 ) ) ;
#47071=CARTESIAN_POINT ( 'NONE',  ( -19.60990026154428278, 0.000000000000000000, 4.498472333781370125 ) ) ;
#47072=CARTESIAN_POINT ( 'NONE',  ( -8.843397823305778616, 0.000000000000000000, 6.228914038079274462 ) ) ;
#47073=CARTESIAN_POINT ( 'NONE',  ( -27.99923088623136636, 0.000000000000000000, 7.757173251277078130 ) ) ;
#47074=ORIENTED_EDGE ( 'NONE', *, *, #35052, .T. ) ;
#47075=DIRECTION ( 'NONE',  ( -0.9999697198139514409, -0.000000000000000000, -0.007781995580013368816 ) ) ;
#47076=ORIENTED_EDGE ( 'NONE', *, *, #24842, .F. ) ;
#47077=DIRECTION ( 'NONE',  ( 0.6427681459581294776, -0.7660444431189769032, 0.005002170337467562802 ) ) ;
#47078=DIRECTION ( 'NONE',  ( -0.5364919789714478471, 0.6444004775717705469, -0.5449076811759709926 ) ) ;
#47079=DIRECTION ( 'NONE',  ( 0.7660212471507180654, -0.6427876096865404731, 0.005961354470445141482 ) ) ;
#47080=LINE ( 'NONE', #50771, #34947 ) ;
#47081=CARTESIAN_POINT ( 'NONE',  ( -32.65841372305263235, 0.000000000000000000, 9.367568705923016381 ) ) ;
#47082=EDGE_CURVE ( 'NONE', #17974, #52765, #32841, .T. ) ;
#47083=CARTESIAN_POINT ( 'NONE',  ( -27.06708303904391144, 0.000000000000000000, 7.395095371555332697 ) ) ;
#47084=VERTEX_POINT ( 'NONE', #33144 ) ;
#47086=CARTESIAN_POINT ( 'NONE',  ( -19.05323196117389628, 5.305366725996514710, 3.913585100488310875 ) ) ;
#47087=PLANE ( 'NONE',  #22751 ) ;
#47088=AXIS2_PLACEMENT_3D ( 'NONE', #24714, #20167, #25025 ) ;
#47089=LINE ( 'NONE', #15864, #17334 ) ;
#47091=EDGE_CURVE ( 'NONE', #54809, #42711, #37684, .T. ) ;
#47092=DIRECTION ( 'NONE',  ( 0.007781995580012662783, 0.000000000000000000, -0.9999697198139514409 ) ) ;
#47093=FACE_OUTER_BOUND ( 'NONE', #46412, .T. ) ;
#47094=ORIENTED_EDGE ( 'NONE', *, *, #22336, .T. ) ;
#47095=DIRECTION ( 'NONE',  ( 0.5364919789714477361, 0.6444004775717706579, 0.5449076811759711036 ) ) ;
#47096=LINE ( 'NONE', #8200, #25091 ) ;
#47097=ORIENTED_EDGE ( 'NONE', *, *, #53423, .F. ) ;
#47098=EDGE_CURVE ( 'NONE', #7373, #23301, #37375, .T. ) ;
#47099=ORIENTED_EDGE ( 'NONE', *, *, #13750, .T. ) ;
#47100=DIRECTION ( 'NONE',  ( -0.7660212471507179544, -0.6427876096865405842, -0.005961354470445141482 ) ) ;
#47102=ORIENTED_EDGE ( 'NONE', *, *, #8753, .T. ) ;
#47103=EDGE_CURVE ( 'NONE', #23572, #16010, #50462, .T. ) ;
#47104=VERTEX_POINT ( 'NONE', #38812 ) ;
#47105=VERTEX_POINT ( 'NONE', #43602 ) ;
#47106=ORIENTED_EDGE ( 'NONE', *, *, #38407, .F. ) ;
#47108=CARTESIAN_POINT ( 'NONE',  ( -9.345197321036080140, -9.000137384199520696, 0.4116184280635072357 ) ) ;
#47109=ORIENTED_EDGE ( 'NONE', *, *, #53587, .F. ) ;
#47112=ORIENTED_EDGE ( 'NONE', *, *, #217, .T. ) ;
#47113=ORIENTED_EDGE ( 'NONE', *, *, #49105, .F. ) ;
#47114=PLANE ( 'NONE',  #52023 ) ;
#47115=DIRECTION ( 'NONE',  ( 0.9999697198139515519, 0.000000000000000000, 0.007781995580013368816 ) ) ;
#47116=ORIENTED_EDGE ( 'NONE', *, *, #15711, .T. ) ;
#47117=FACE_OUTER_BOUND ( 'NONE', #53808, .T. ) ;
#47118=DIRECTION ( 'NONE',  ( -0.5364919789714478471, 0.6444004775717705469, -0.5449076811759709926 ) ) ;
#47119=ORIENTED_EDGE ( 'NONE', *, *, #38605, .T. ) ;
#47120=CARTESIAN_POINT ( 'NONE',  ( -17.79170326090322263, 3.200641362704009119, 9.045020623922320979 ) ) ;
#47121=EDGE_CURVE ( 'NONE', #34236, #22478, #39074, .T. ) ;
#47122=ORIENTED_EDGE ( 'NONE', *, *, #40140, .T. ) ;
#47123=DIRECTION ( 'NONE',  ( 0.5364919789714477361, 0.6444004775717706579, 0.5449076811759711036 ) ) ;
#47124=ADVANCED_FACE ( 'NONE', ( #13782 ), #56124, .F. ) ;
#47125=EDGE_CURVE ( 'NONE', #36041, #10112, #147, .T. ) ;
#47126=LINE ( 'NONE', #8820, #48120 ) ;
#47127=ORIENTED_EDGE ( 'NONE', *, *, #49782, .F. ) ;
#47128=PLANE ( 'NONE',  #40361 ) ;
#47129=LINE ( 'NONE', #38626, #36534 ) ;
#47130=LINE ( 'NONE', #5648, #23944 ) ;
#47131=LINE ( 'NONE', #8232, #50969 ) ;
#47132=ORIENTED_EDGE ( 'NONE', *, *, #3192, .T. ) ;
#47133=CARTESIAN_POINT ( 'NONE',  ( -34.64355613791357769, 0.000000000000000000, 10.23836012842048326 ) ) ;
#47134=LINE ( 'NONE', #55368, #33268 ) ;
#47135=LINE ( 'NONE', #30099, #31234 ) ;
#47136=LINE ( 'NONE', #25554, #15034 ) ;
#47137=CARTESIAN_POINT ( 'NONE',  ( -14.29926954212191248, -2.622721114510659035, 6.540585794009272647 ) ) ;
#47138=CARTESIAN_POINT ( 'NONE',  ( -12.06004980474070898, 0.000000000000000000, 1.602570457315059205 ) ) ;
#47139=ADVANCED_FACE ( 'NONE', ( #44189 ), #38510, .F. ) ;
#47140=DIRECTION ( 'NONE',  ( -0.005961354470445682716, -0.6427876096865404731, 0.7660212471507180654 ) ) ;
#47141=ORIENTED_EDGE ( 'NONE', *, *, #54596, .F. ) ;
#47142=CARTESIAN_POINT ( 'NONE',  ( -10.90768746164348002, 0.000000000000000000, 6.951513398406762079 ) ) ;
#47143=ORIENTED_EDGE ( 'NONE', *, *, #42322, .F. ) ;
#47144=DIRECTION ( 'NONE',  ( -0.005961354470445682716, -0.6427876096865404731, 0.7660212471507180654 ) ) ;
#47145=CARTESIAN_POINT ( 'NONE',  ( -14.01623497886155256, -0.1191753592594197858, 2.226008083469502630 ) ) ;
#47146=DIRECTION ( 'NONE',  ( -0.005002170337468016433, -0.7660444431189770143, 0.6427681459581293666 ) ) ;
#47147=FACE_OUTER_BOUND ( 'NONE', #7553, .T. ) ;
#47148=DIRECTION ( 'NONE',  ( -0.5364919789714478471, 0.6444004775717705469, -0.5449076811759709926 ) ) ;
#47149=ORIENTED_EDGE ( 'NONE', *, *, #25143, .F. ) ;
#47150=VECTOR ( 'NONE', #49276, 1000.000000000000227 ) ;
#47151=ORIENTED_EDGE ( 'NONE', *, *, #51435, .T. ) ;
#47152=PLANE ( 'NONE',  #20487 ) ;
#47153=LINE ( 'NONE', #13089, #28639 ) ;
#47154=ORIENTED_EDGE ( 'NONE', *, *, #4619, .F. ) ;
#47155=DIRECTION ( 'NONE',  ( 0.9999697198139515519, 0.000000000000000000, 0.007781995580013368816 ) ) ;
#47156=EDGE_LOOP ( 'NONE', ( #34343, #20858, #48683, #15278, #45470 ) ) ;
#47157=CARTESIAN_POINT ( 'NONE',  ( -10.29290469531352592, -0.1166911823299086465, 0.7797401565107704435 ) ) ;
#47158=ADVANCED_FACE ( 'NONE', ( #8407 ), #17211, .F. ) ;
#47159=ORIENTED_EDGE ( 'NONE', *, *, #30, .T. ) ;
#47160=CARTESIAN_POINT ( 'NONE',  ( -16.28201862538443834, 0.000000000000000000, 6.740363097011673688 ) ) ;
#47161=VERTEX_POINT ( 'NONE', #39357 ) ;
#47162=EDGE_LOOP ( 'NONE', ( #38705, #48800, #54825, #27872 ) ) ;
#47163=EDGE_LOOP ( 'NONE', ( #49902, #54290, #9902, #18203 ) ) ;
#47165=DIRECTION ( 'NONE',  ( 0.000000000000000000, -0.000000000000000000, -1.000000000000000000 ) ) ;
#47166=PLANE ( 'NONE',  #2165 ) ;
#47167=ADVANCED_FACE ( 'NONE', ( #52134 ), #31107, .F. ) ;
#47168=LINE ( 'NONE', #12818, #18493 ) ;
#47169=ORIENTED_EDGE ( 'NONE', *, *, #43381, .F. ) ;
#47170=ORIENTED_EDGE ( 'NONE', *, *, #52635, .F. ) ;
#47171=EDGE_CURVE ( 'NONE', #12432, #47173, #4712, .T. ) ;
#47172=EDGE_CURVE ( 'NONE', #40878, #3654, #26290, .T. ) ;
#47173=VERTEX_POINT ( 'NONE', #47300 ) ;
#47174=CARTESIAN_POINT ( 'NONE',  ( -20.43500284407263834, 4.657758921906509642, 12.46314610441118198 ) ) ;
#47175=DIRECTION ( 'NONE',  ( 0.5449076811759707706, 0.6444004775717708799, -0.5364919789714476250 ) ) ;
#47176=EDGE_LOOP ( 'NONE', ( #13642, #18063, #5438, #49821, #43359 ) ) ;
#47177=DIRECTION ( 'NONE',  ( 0.000000000000000000, -1.000000000000000000, 0.000000000000000000 ) ) ;
#47178=ADVANCED_FACE ( 'NONE', ( #22031 ), #13251, .F. ) ;
#47179=EDGE_LOOP ( 'NONE', ( #34936, #42566, #24452, #40323 ) ) ;
#47181=LINE ( 'NONE', #8879, #43954 ) ;
#47182=ORIENTED_EDGE ( 'NONE', *, *, #32819, .F. ) ;
#47183=ADVANCED_FACE ( 'NONE', ( #21759 ), #51581, .F. ) ;
#47184=DIRECTION ( 'NONE',  ( -0.005002170337468016433, -0.7660444431189770143, 0.6427681459581293666 ) ) ;
#47185=ORIENTED_EDGE ( 'NONE', *, *, #36561, .F. ) ;
#47186=EDGE_CURVE ( 'NONE', #52765, #46212, #17483, .T. ) ;
#47188=DIRECTION ( 'NONE',  ( 0.5449076811759707706, 0.6444004775717708799, -0.5364919789714476250 ) ) ;
#47189=DIRECTION ( 'NONE',  ( 0.005002170337468016433, -0.7660444431189770143, -0.6427681459581293666 ) ) ;
#47191=CARTESIAN_POINT ( 'NONE',  ( -15.44334144360980865, -0.1191753592594183703, 5.538890639235001245 ) ) ;
#47192=DIRECTION ( 'NONE',  ( -0.9999697198139514409, -0.000000000000000000, -0.007781995580013368816 ) ) ;
#47193=DIRECTION ( 'NONE',  ( -0.5364919789714478471, 0.6444004775717705469, -0.5449076811759709926 ) ) ;
#47194=LINE ( 'NONE', #13132, #44573 ) ;
#47195=ORIENTED_EDGE ( 'NONE', *, *, #26354, .T. ) ;
#47196=ADVANCED_FACE ( 'NONE', ( #738 ), #25736, .F. ) ;
#47197=CARTESIAN_POINT ( 'NONE',  ( -19.60912206198628027, -0.1191753592594197858, 4.398475361799976113 ) ) ;
#47198=CARTESIAN_POINT ( 'NONE',  ( -17.26532721389163072, 0.000000000000000000, 13.67648636611514590 ) ) ;
#47199=LINE ( 'NONE', #34176, #20450 ) ;
#47200=CARTESIAN_POINT ( 'NONE',  ( -11.22056963685719211, 0.000000000000000000, 1.239771416285661010 ) ) ;
#47201=DIRECTION ( 'NONE',  ( -0.6427681459581293666, -0.7660444431189770143, -0.005002170337467561935 ) ) ;
#47202=EDGE_CURVE ( 'NONE', #41560, #35868, #9547, .T. ) ;
#47203=DIRECTION ( 'NONE',  ( 0.007781995580012662783, 0.000000000000000000, -0.9999697198139514409 ) ) ;
#47204=ORIENTED_EDGE ( 'NONE', *, *, #4221, .F. ) ;
#47205=LINE ( 'NONE', #34436, #10783 ) ;
#47206=CARTESIAN_POINT ( 'NONE',  ( -17.74404816805336793, 0.000000000000000000, 3.574322630375089460 ) ) ;
#47207=PLANE ( 'NONE',  #1441 ) ;
#47208=ORIENTED_EDGE ( 'NONE', *, *, #27592, .T. ) ;
#47209=CARTESIAN_POINT ( 'NONE',  ( -16.27339646486858982, 0.000000000000000000, 5.632433987238382400 ) ) ;
#47210=PLANE ( 'NONE',  #12314 ) ;
#47211=ORIENTED_EDGE ( 'NONE', *, *, #9110, .F. ) ;
#47213=DIRECTION ( 'NONE',  ( -0.5449076811759708816, 0.6444004775717707689, 0.5364919789714475140 ) ) ;
#47214=AXIS2_PLACEMENT_3D ( 'NONE', #8874, #26179, #4585 ) ;
#47215=DIRECTION ( 'NONE',  ( 0.007781995580012663651, 0.000000000000000000, -0.9999697198139515519 ) ) ;
#47217=ORIENTED_EDGE ( 'NONE', *, *, #48870, .T. ) ;
#47218=VERTEX_POINT ( 'NONE', #47601 ) ;
#47219=LINE ( 'NONE', #30193, #14032 ) ;
#47221=CARTESIAN_POINT ( 'NONE',  ( -15.40103151951671734, 0.000000000000000000, 12.95233060667165681 ) ) ;
#47222=CARTESIAN_POINT ( 'NONE',  ( -18.76354595665420177, -0.1191753592594177458, 14.21882498613976331 ) ) ;
#47223=LINE ( 'NONE', #52051, #19235 ) ;
#47224=VECTOR ( 'NONE', #46270, 1000.000000000000114 ) ;
#47225=CARTESIAN_POINT ( 'NONE',  ( -18.86354292863559579, 0.000000000000000000, 14.21804678658176080 ) ) ;
#47226=ADVANCED_FACE ( 'NONE', ( #5293 ), #55841, .F. ) ;
#47227=ORIENTED_EDGE ( 'NONE', *, *, #50792, .T. ) ;
#47228=CARTESIAN_POINT ( 'NONE',  ( 2.072287782118878319, 0.000000000000000000, -2.950529333540147015 ) ) ;
#47229=VECTOR ( 'NONE', #16412, 1000.000000000000227 ) ;
#47230=CARTESIAN_POINT ( 'NONE',  ( -19.07690576783079806, 0.000000000000000000, 7.626602792214121962 ) ) ;
#47231=ORIENTED_EDGE ( 'NONE', *, *, #34918, .T. ) ;
#47232=DIRECTION ( 'NONE',  ( 0.005002170337468016433, -0.7660444431189770143, -0.6427681459581293666 ) ) ;
#47233=CARTESIAN_POINT ( 'NONE',  ( -15.33969221856512988, 0.000000000000000000, 5.070362163553848056 ) ) ;
#47235=EDGE_CURVE ( 'NONE', #55625, #9472, #14374, .T. ) ;
#47236=ORIENTED_EDGE ( 'NONE', *, *, #35979, .T. ) ;
#47237=CARTESIAN_POINT ( 'NONE',  ( -18.53018086135774212, -3.756034771668160577, 10.04397622040690408 ) ) ;
#47238=ORIENTED_EDGE ( 'NONE', *, *, #23798, .T. ) ;
#47239=EDGE_CURVE ( 'NONE', #30300, #30276, #45295, .T. ) ;
#47240=ORIENTED_EDGE ( 'NONE', *, *, #31766, .F. ) ;
#47241=ORIENTED_EDGE ( 'NONE', *, *, #34968, .F. ) ;
#47242=ORIENTED_EDGE ( 'NONE', *, *, #15461, .F. ) ;
#47243=DIRECTION ( 'NONE',  ( -0.005961354470445682716, -0.6427876096865404731, 0.7660212471507180654 ) ) ;
#47244=ORIENTED_EDGE ( 'NONE', *, *, #56147, .F. ) ;
#47245=DIRECTION ( 'NONE',  ( -0.7660212471507179544, -0.6427876096865405842, -0.005961354470445141482 ) ) ;
#47246=VECTOR ( 'NONE', #5407, 999.9999999999998863 ) ;
#47247=AXIS2_PLACEMENT_3D ( 'NONE', #21897, #22188, #30972 ) ;
#47248=EDGE_LOOP ( 'NONE', ( #27124, #14996, #46086, #28978 ) ) ;
#47249=CARTESIAN_POINT ( 'NONE',  ( -10.40281381572843244, 0.000000000000000000, 1.784793464566069687 ) ) ;
#47250=EDGE_CURVE ( 'NONE', #37328, #35631, #49570, .T. ) ;
#47251=ORIENTED_EDGE ( 'NONE', *, *, #10157, .T. ) ;
#47252=DIRECTION ( 'NONE',  ( 0.007781995580012663651, 0.000000000000000000, -0.9999697198139515519 ) ) ;
#47253=ORIENTED_EDGE ( 'NONE', *, *, #3582, .F. ) ;
#47254=ADVANCED_FACE ( 'NONE', ( #1829 ), #39912, .F. ) ;
#47255=CARTESIAN_POINT ( 'NONE',  ( -15.81450767503806532, 0.000000000000000000, 6.374669305521920570 ) ) ;
#47256=LINE ( 'NONE', #46711, #43024 ) ;
#47257=CARTESIAN_POINT ( 'NONE',  ( -10.27421835998572064, 0.000000000000000000, 10.96090226820206048 ) ) ;
#47258=CARTESIAN_POINT ( 'NONE',  ( -15.88130887279446490, 0.000000000000000000, 3.050160814894388839 ) ) ;
#47259=LINE ( 'NONE', #33103, #53708 ) ;
#47261=EDGE_CURVE ( 'NONE', #29343, #22728, #23696, .T. ) ;
#47262=VERTEX_POINT ( 'NONE', #36787 ) ;
#47263=LINE ( 'NONE', #47559, #53066 ) ;
#47264=DIRECTION ( 'NONE',  ( 0.9999697198139515519, 0.000000000000000000, 0.007781995580013368816 ) ) ;
#47266=VECTOR ( 'NONE', #17039, 999.9999999999998863 ) ;
#47267=CARTESIAN_POINT ( 'NONE',  ( -19.26983395039373903, 0.000000000000000000, 6.717111227287613673 ) ) ;
#47268=EDGE_CURVE ( 'NONE', #39753, #14310, #6143, .T. ) ;
#47269=FACE_OUTER_BOUND ( 'NONE', #44473, .T. ) ;
#47270=CARTESIAN_POINT ( 'NONE',  ( -11.30636317915456779, -0.1191753592594197858, 11.32220194836580340 ) ) ;
#47271=CARTESIAN_POINT ( 'NONE',  ( -13.47982697681151087, 0.000000000000000000, 4.915510051330911345 ) ) ;
#47272=ORIENTED_EDGE ( 'NONE', *, *, #1104, .F. ) ;
#47273=DIRECTION ( 'NONE',  ( -0.2426528472758541499, 0.7422098413412800966, -0.6246952433987894571 ) ) ;
#47274=CARTESIAN_POINT ( 'NONE',  ( -18.19747506107908563, 0.000000000000000000, 14.03856424583689311 ) ) ;
#47275=ORIENTED_EDGE ( 'NONE', *, *, #13487, .F. ) ;
#47276=CARTESIAN_POINT ( 'NONE',  ( -26.13493519185646008, 0.000000000000000000, 7.033017491833586377 ) ) ;
#47278=CARTESIAN_POINT ( 'NONE',  ( -20.54204810873173415, 0.000000000000000000, 4.860550213503115558 ) ) ;
#47279=DIRECTION ( 'NONE',  ( -0.5449076811759708816, 0.6444004775717707689, 0.5364919789714475140 ) ) ;
#47280=CARTESIAN_POINT ( 'NONE',  ( -22.40478740399063895, 0.000000000000000000, 5.384712028983816623 ) ) ;
#47281=EDGE_LOOP ( 'NONE', ( #43209, #9147, #10625, #53772 ) ) ;
#47283=CARTESIAN_POINT ( 'NONE',  ( -8.743798853363076162, -0.1191753592594191058, 4.483031819370165927 ) ) ;
#47284=PLANE ( 'NONE',  #23177 ) ;
#47285=LINE ( 'NONE', #8397, #29727 ) ;
#47286=EDGE_CURVE ( 'NONE', #2953, #17094, #41021, .T. ) ;
#47287=VECTOR ( 'NONE', #14620, 1000.000000000000000 ) ;
#47288=VECTOR ( 'NONE', #33447, 999.9999999999998863 ) ;
#47289=DIRECTION ( 'NONE',  ( 0.9999697198139515519, 0.000000000000000000, 0.007781995580013368816 ) ) ;
#47290=LINE ( 'NONE', #16638, #53896 ) ;
#47291=ADVANCED_FACE ( 'NONE', ( #10926 ), #23167, .F. ) ;
#47292=FACE_OUTER_BOUND ( 'NONE', #32259, .T. ) ;
#47293=CARTESIAN_POINT ( 'NONE',  ( -19.91685214842295437, -2.137015261443159009, 4.549520895431744982 ) ) ;
#47294=ORIENTED_EDGE ( 'NONE', *, *, #42144, .F. ) ;
#47295=DIRECTION ( 'NONE',  ( -0.6246952433987894571, 0.7422098413412802076, 0.2426528472758539834 ) ) ;
#47296=LINE ( 'NONE', #8406, #34174 ) ;
#47297=ADVANCED_FACE ( 'NONE', ( #45552 ), #32250, .F. ) ;
#47298=AXIS2_PLACEMENT_3D ( 'NONE', #11460, #28785, #46087 ) ;
#47299=EDGE_CURVE ( 'NONE', #33755, #14069, #44446, .T. ) ;
#47300=CARTESIAN_POINT ( 'NONE',  ( -12.29872409866145055, 0.000000000000000000, 6.571355959844968453 ) ) ;
#47302=DIRECTION ( 'NONE',  ( -0.7660212471507179544, -0.6427876096865405842, -0.005961354470445141482 ) ) ;
#47303=EDGE_CURVE ( 'NONE', #37046, #37070, #990, .T. ) ;
#47304=EDGE_CURVE ( 'NONE', #3167, #33190, #18319, .T. ) ;
#47305=EDGE_CURVE ( 'NONE', #27291, #34236, #35657, .T. ) ;
#47306=ORIENTED_EDGE ( 'NONE', *, *, #41760, .F. ) ;
#47307=ORIENTED_EDGE ( 'NONE', *, *, #6249, .T. ) ;
#47308=VECTOR ( 'NONE', #51331, 999.9999999999998863 ) ;
#47309=ORIENTED_EDGE ( 'NONE', *, *, #55163, .T. ) ;
#47310=ORIENTED_EDGE ( 'NONE', *, *, #34059, .F. ) ;
#47311=EDGE_LOOP ( 'NONE', ( #47471, #35385, #37846, #47025, #10691 ) ) ;
#47313=LINE ( 'NONE', #8420, #47680 ) ;
#47314=LINE ( 'NONE', #52437, #23838 ) ;
#47315=LINE ( 'NONE', #26305, #53057 ) ;
#47316=VERTEX_POINT ( 'NONE', #40763 ) ;
#47318=EDGE_CURVE ( 'NONE', #56078, #11098, #52973, .T. ) ;
#47320=CARTESIAN_POINT ( 'NONE',  ( -16.79925329029790149, 0.000000000000000000, 13.49544742625427496 ) ) ;
#47321=ORIENTED_EDGE ( 'NONE', *, *, #8648, .F. ) ;
#47322=EDGE_CURVE ( 'NONE', #41338, #40788, #31416, .T. ) ;
#47323=LINE ( 'NONE', #478, #7645 ) ;
#47324=ADVANCED_FACE ( 'NONE', ( #40496 ), #22868, .F. ) ;
#47325=CARTESIAN_POINT ( 'NONE',  ( -16.81345671998191449, 0.000000000000000000, 3.412238694616132495 ) ) ;
#47326=PLANE ( 'NONE',  #48604 ) ;
#47327=ORIENTED_EDGE ( 'NONE', *, *, #12284, .F. ) ;
#47328=LINE ( 'NONE', #12131, #3811 ) ;
#47330=ORIENTED_EDGE ( 'NONE', *, *, #44388, .T. ) ;
#47331=VECTOR ( 'NONE', #26485, 999.9999999999998863 ) ;
#47332=EDGE_CURVE ( 'NONE', #46401, #39009, #25130, .T. ) ;
#47333=VECTOR ( 'NONE', #3619, 1000.000000000000227 ) ;
#47334=CARTESIAN_POINT ( 'NONE',  ( -14.92276770555628929, 0.9340140483890027046, 4.210707049457523610 ) ) ;
#47335=CARTESIAN_POINT ( 'NONE',  ( -17.74404816805336793, 0.000000000000000000, 3.574322630375089460 ) ) ;
#47336=DIRECTION ( 'NONE',  ( -0.9999697198139514409, -0.000000000000000000, -0.007781995580013368816 ) ) ;
#47337=AXIS2_PLACEMENT_3D ( 'NONE', #38972, #42946, #38712 ) ;
#47338=CARTESIAN_POINT ( 'NONE',  ( -2.882214333898595271, 3.377503723539708513, -2.098823647966802319 ) ) ;
#47339=DIRECTION ( 'NONE',  ( 0.5364919789714477361, 0.6444004775717706579, 0.5449076811759711036 ) ) ;
#47340=DIRECTION ( 'NONE',  ( 0.9999697198139515519, 0.000000000000000000, 0.007781995580013368816 ) ) ;
#47341=CARTESIAN_POINT ( 'NONE',  ( -15.88130887279446490, 0.000000000000000000, 3.050160814894388839 ) ) ;
#47343=ORIENTED_EDGE ( 'NONE', *, *, #2027, .T. ) ;
#47345=ORIENTED_EDGE ( 'NONE', *, *, #40174, .F. ) ;
#47346=LINE ( 'NONE', #12719, #53739 ) ;
#47347=CARTESIAN_POINT ( 'NONE',  ( -17.74560456716937296, 0.000000000000000000, 3.774316574337878372 ) ) ;
#47348=PLANE ( 'NONE',  #28109 ) ;
#47349=VECTOR ( 'NONE', #18985, 999.9999999999998863 ) ;
#47350=LINE ( 'NONE', #24944, #22251 ) ;
#47351=DIRECTION ( 'NONE',  ( 0.000000000000000000, -0.000000000000000000, -1.000000000000000000 ) ) ;
#47352=DIRECTION ( 'NONE',  ( 0.5449076811759707706, 0.6444004775717708799, -0.5364919789714476250 ) ) ;
#47353=CARTESIAN_POINT ( 'NONE',  ( -14.06380102061297066, -0.1191753592594185784, 7.396286890827852289 ) ) ;
#47355=ORIENTED_EDGE ( 'NONE', *, *, #34302, .F. ) ;
#47357=CARTESIAN_POINT ( 'NONE',  ( -10.22736869892390743, 0.000000000000000000, 4.940821433706977572 ) ) ;
#47358=DIRECTION ( 'NONE',  ( -0.6427681459581293666, -0.7660444431189770143, -0.005002170337467561935 ) ) ;
#47359=CARTESIAN_POINT ( 'NONE',  ( -26.13337879274045505, 0.000000000000000000, 6.833023547870798353 ) ) ;
#47360=LINE ( 'NONE', #7628, #52982 ) ;
#47361=VECTOR ( 'NONE', #43522, 999.9999999999998863 ) ;
#47362=PLANE ( 'NONE',  #10519 ) ;
#47363=CARTESIAN_POINT ( 'NONE',  ( -12.65264600905801551, -0.1191753592594188005, 5.191276406585294545 ) ) ;
#47364=EDGE_LOOP ( 'NONE', ( #56162, #44663, #53393, #42070 ) ) ;
#47365=DIRECTION ( 'NONE',  ( 0.005002170337468016433, -0.7660444431189770143, -0.6427681459581293666 ) ) ;
#47366=ADVANCED_FACE ( 'NONE', ( #24531 ), #11502, .F. ) ;
#47367=CARTESIAN_POINT ( 'NONE',  ( -17.74560456716937296, 0.000000000000000000, 3.774316574337878372 ) ) ;
#47368=ORIENTED_EDGE ( 'NONE', *, *, #12138, .T. ) ;
#47369=VECTOR ( 'NONE', #55202, 999.9999999999998863 ) ;
#47370=ORIENTED_EDGE ( 'NONE', *, *, #17869, .F. ) ;
#47371=DIRECTION ( 'NONE',  ( 0.000000000000000000, -1.000000000000000000, 0.000000000000000000 ) ) ;
#47372=ADVANCED_FACE ( 'NONE', ( #54936 ), #45849, .F. ) ;
#47373=EDGE_CURVE ( 'NONE', #34361, #12737, #28824, .T. ) ;
#47374=VECTOR ( 'NONE', #32384, 1000.000000000000000 ) ;
#47375=VECTOR ( 'NONE', #4813, 999.9999999999998863 ) ;
#47376=ORIENTED_EDGE ( 'NONE', *, *, #19241, .F. ) ;
#47377=ADVANCED_FACE ( 'NONE', ( #19736 ), #3251, .F. ) ;
#47378=VECTOR ( 'NONE', #21186, 1000.000000000000000 ) ;
#47379=VERTEX_POINT ( 'NONE', #11199 ) ;
#47381=VECTOR ( 'NONE', #39114, 999.9999999999998863 ) ;
#47382=ORIENTED_EDGE ( 'NONE', *, *, #35584, .T. ) ;
#47384=ORIENTED_EDGE ( 'NONE', *, *, #36983, .F. ) ;
#47386=FACE_OUTER_BOUND ( 'NONE', #12860, .T. ) ;
#47387=ORIENTED_EDGE ( 'NONE', *, *, #8575, .F. ) ;
#47388=VECTOR ( 'NONE', #32804, 1000.000000000000227 ) ;
#47389=ORIENTED_EDGE ( 'NONE', *, *, #45533, .T. ) ;
#47390=EDGE_CURVE ( 'NONE', #31490, #17094, #12032, .T. ) ;
#47391=CARTESIAN_POINT ( 'NONE',  ( -16.33317936670417225, 0.000000000000000000, 13.31440848639340224 ) ) ;
#47392=ORIENTED_EDGE ( 'NONE', *, *, #54466, .F. ) ;
#47393=EDGE_CURVE ( 'NONE', #38849, #11370, #33909, .T. ) ;
#47394=CARTESIAN_POINT ( 'NONE',  ( -20.54126990917373519, -0.1191753592594197858, 4.760553241521720658 ) ) ;
#47395=DIRECTION ( 'NONE',  ( 0.6427681459581294776, -0.7660444431189769032, 0.005002170337467562802 ) ) ;
#47396=ORIENTED_EDGE ( 'NONE', *, *, #38145, .T. ) ;
#47397=CARTESIAN_POINT ( 'NONE',  ( -17.10590788104098792, -4.889348428825664783, 3.369840843825817167 ) ) ;
#47398=ORIENTED_EDGE ( 'NONE', *, *, #47560, .T. ) ;
#47400=DIRECTION ( 'NONE',  ( 0.5449076811759707706, 0.6444004775717708799, -0.5364919789714476250 ) ) ;
#47401=VECTOR ( 'NONE', #52804, 1000.000000000000227 ) ;
#47403=LINE ( 'NONE', #13057, #2779 ) ;
#47404=ORIENTED_EDGE ( 'NONE', *, *, #7758, .F. ) ;
#47405=LINE ( 'NONE', #25004, #26733 ) ;
#47406=CARTESIAN_POINT ( 'NONE',  ( -16.81267852042391198, -0.1191753592594197858, 3.312241722634738039 ) ) ;
#47407=DIRECTION ( 'NONE',  ( 0.5449076811759707706, 0.6444004775717708799, -0.5364919789714476250 ) ) ;
#47408=VECTOR ( 'NONE', #11887, 1000.000000000000227 ) ;
#47409=DIRECTION ( 'NONE',  ( 0.007781995580012663651, -3.146120232559066537E-19, -0.9999697198139514409 ) ) ;
#47410=ORIENTED_EDGE ( 'NONE', *, *, #32047, .T. ) ;
#47411=VECTOR ( 'NONE', #3010, 999.9999999999998863 ) ;
#47412=VECTOR ( 'NONE', #32297, 999.9999999999998863 ) ;
#47413=CARTESIAN_POINT ( 'NONE',  ( -19.60834386242827776, 0.000000000000000000, 4.298478389818581213 ) ) ;
#47414=CARTESIAN_POINT ( 'NONE',  ( -14.93495759592298988, 0.000000000000000000, 12.77129166681078409 ) ) ;
#47415=DIRECTION ( 'NONE',  ( 0.005002170337468016433, -0.7660444431189770143, -0.6427681459581293666 ) ) ;
#47416=CARTESIAN_POINT ( 'NONE',  ( -15.06355305166570346, 0.000000000000000000, 3.595182863174795962 ) ) ;
#47417=CARTESIAN_POINT ( 'NONE',  ( -16.23605725028139091, -4.889348428825661230, 11.01282148875231748 ) ) ;
#47418=PLANE ( 'NONE',  #11343 ) ;
#47419=LINE ( 'NONE', #33524, #13427 ) ;
#47420=VECTOR ( 'NONE', #44954, 1000.000000000000227 ) ;
#47421=FACE_OUTER_BOUND ( 'NONE', #46577, .T. ) ;
#47422=PLANE ( 'NONE',  #23194 ) ;
#47423=VECTOR ( 'NONE', #47500, 1000.000000000000114 ) ;
#47424=EDGE_LOOP ( 'NONE', ( #38936, #49592, #30462, #36868 ) ) ;
#47426=DIRECTION ( 'NONE',  ( 0.5364919789714477361, 0.6444004775717706579, 0.5449076811759711036 ) ) ;
#47427=ORIENTED_EDGE ( 'NONE', *, *, #34582, .F. ) ;
#47428=DIRECTION ( 'NONE',  ( 0.5449076811759707706, 0.6444004775717708799, -0.5364919789714476250 ) ) ;
#47431=VECTOR ( 'NONE', #1386, 999.9999999999998863 ) ;
#47432=VECTOR ( 'NONE', #33991, 1000.000000000000227 ) ;
#47433=DIRECTION ( 'NONE',  ( 0.005002170337468016433, -0.7660444431189770143, -0.6427681459581293666 ) ) ;
#47434=FACE_OUTER_BOUND ( 'NONE', #13257, .T. ) ;
#47435=ORIENTED_EDGE ( 'NONE', *, *, #53331, .T. ) ;
#47436=VERTEX_POINT ( 'NONE', #24825 ) ;
#47437=DIRECTION ( 'NONE',  ( -0.7660212471507179544, -0.6427876096865405842, -0.005961354470445141482 ) ) ;
#47438=PLANE ( 'NONE',  #8667 ) ;
#47439=ORIENTED_EDGE ( 'NONE', *, *, #43847, .T. ) ;
#47440=VECTOR ( 'NONE', #11719, 1000.000000000000114 ) ;
#47441=DIRECTION ( 'NONE',  ( 0.000000000000000000, -1.000000000000000000, 0.000000000000000000 ) ) ;
#47442=EDGE_CURVE ( 'NONE', #17725, #12293, #55207, .T. ) ;
#47444=LINE ( 'NONE', #8859, #47635 ) ;
#47446=ORIENTED_EDGE ( 'NONE', *, *, #44725, .F. ) ;
#47447=DIRECTION ( 'NONE',  ( -0.5449076811759708816, 0.6444004775717707689, 0.5364919789714475140 ) ) ;
#47448=ADVANCED_FACE ( 'NONE', ( #28524 ), #24279, .F. ) ;
#47449=EDGE_CURVE ( 'NONE', #24475, #16658, #17994, .T. ) ;
#47450=ORIENTED_EDGE ( 'NONE', *, *, #3078, .T. ) ;
#47451=ORIENTED_EDGE ( 'NONE', *, *, #54482, .T. ) ;
#47452=VERTEX_POINT ( 'NONE', #25388 ) ;
#47453=LINE ( 'NONE', #43743, #51999 ) ;
#47454=AXIS2_PLACEMENT_3D ( 'NONE', #14092, #14633, #10386 ) ;
#47455=LINE ( 'NONE', #26426, #33217 ) ;
#47456=DIRECTION ( 'NONE',  ( 0.000000000000000000, -0.000000000000000000, -1.000000000000000000 ) ) ;
#47457=VECTOR ( 'NONE', #47192, 1000.000000000000227 ) ;
#47459=DIRECTION ( 'NONE',  ( 0.000000000000000000, -0.000000000000000000, -1.000000000000000000 ) ) ;
#47460=ORIENTED_EDGE ( 'NONE', *, *, #56176, .F. ) ;
#47461=EDGE_LOOP ( 'NONE', ( #7774, #39777, #31890, #7000 ) ) ;
#47462=VECTOR ( 'NONE', #49127, 1000.000000000000114 ) ;
#47463=ORIENTED_EDGE ( 'NONE', *, *, #2928, .F. ) ;
#47464=VECTOR ( 'NONE', #5345, 1000.000000000000000 ) ;
#47466=VERTEX_POINT ( 'NONE', #8929 ) ;
#47467=FACE_OUTER_BOUND ( 'NONE', #54133, .T. ) ;
#47468=ORIENTED_EDGE ( 'NONE', *, *, #3007, .F. ) ;
#47469=DIRECTION ( 'NONE',  ( -0.7660212471507179544, -0.6427876096865405842, -0.005961354470445141482 ) ) ;
#47470=DIRECTION ( 'NONE',  ( -0.005002170337468016433, -0.7660444431189770143, 0.6427681459581293666 ) ) ;
#47471=ORIENTED_EDGE ( 'NONE', *, *, #20025, .F. ) ;
#47472=DIRECTION ( 'NONE',  ( 0.9999697198139515519, 0.000000000000000000, 0.007781995580013368816 ) ) ;
#47473=ORIENTED_EDGE ( 'NONE', *, *, #54583, .T. ) ;
#47474=EDGE_CURVE ( 'NONE', #3804, #21256, #8339, .T. ) ;
#47475=DIRECTION ( 'NONE',  ( 0.007781995580012662783, 0.000000000000000000, -0.9999697198139514409 ) ) ;
#47476=VECTOR ( 'NONE', #49139, 999.9999999999998863 ) ;
#47477=ORIENTED_EDGE ( 'NONE', *, *, #24478, .F. ) ;
#47478=ADVANCED_FACE ( 'NONE', ( #38748 ), #43294, .F. ) ;
#47479=CARTESIAN_POINT ( 'NONE',  ( 4.452747148193316740, 0.000000000000000000, 0.4159841754879232689 ) ) ;
#47480=FACE_OUTER_BOUND ( 'NONE', #13991, .T. ) ;
#47481=CARTESIAN_POINT ( 'NONE',  ( -16.81190032086591302, 0.000000000000000000, 3.212244750653343583 ) ) ;
#47482=ADVANCED_FACE ( 'NONE', ( #42986 ), #48075, .F. ) ;
#47483=ORIENTED_EDGE ( 'NONE', *, *, #9979, .F. ) ;
#47484=VECTOR ( 'NONE', #16982, 1000.000000000000227 ) ;
#47485=DIRECTION ( 'NONE',  ( 0.5364919789714477361, 0.6444004775717706579, 0.5449076811759711036 ) ) ;
#47486=LINE ( 'NONE', #17375, #11983 ) ;
#47487=EDGE_CURVE ( 'NONE', #17816, #25199, #21425, .T. ) ;
#47488=PLANE ( 'NONE',  #19476 ) ;
#47490=CARTESIAN_POINT ( 'NONE',  ( -16.06709938707323460, 0.000000000000000000, 13.13181314741652628 ) ) ;
#47491=DIRECTION ( 'NONE',  ( 0.000000000000000000, -1.000000000000000000, 0.000000000000000000 ) ) ;
#47492=DIRECTION ( 'NONE',  ( 0.7660212471507180654, -0.6427876096865404731, 0.005961354470445141482 ) ) ;
#47493=DIRECTION ( 'NONE',  ( 0.6427681459581294776, -0.7660444431189769032, 0.005002170337467562802 ) ) ;
#47494=ORIENTED_EDGE ( 'NONE', *, *, #25517, .F. ) ;
#47495=DIRECTION ( 'NONE',  ( 0.000000000000000000, -1.000000000000000000, 0.000000000000000000 ) ) ;
#47496=DIRECTION ( 'NONE',  ( 0.000000000000000000, -0.000000000000000000, -1.000000000000000000 ) ) ;
#47497=DIRECTION ( 'NONE',  ( -0.005002170337468016433, -0.7660444431189770143, 0.6427681459581293666 ) ) ;
#47498=ORIENTED_EDGE ( 'NONE', *, *, #18651, .F. ) ;
#47499=AXIS2_PLACEMENT_3D ( 'NONE', #9116, #9966, #43479 ) ;
#47500=DIRECTION ( 'NONE',  ( 0.5449076811759707706, 0.6444004775717708799, -0.5364919789714476250 ) ) ;
#47501=CARTESIAN_POINT ( 'NONE',  ( -18.26762043990991202, -2.946525016555662457, 3.883075692263754153 ) ) ;
#47502=VERTEX_POINT ( 'NONE', #13714 ) ;
#47503=VECTOR ( 'NONE', #34094, 999.9999999999998863 ) ;
#47505=DIRECTION ( 'NONE',  ( -0.6427681459581293666, -0.7660444431189770143, -0.005002170337467561935 ) ) ;
#47506=ADVANCED_FACE ( 'NONE', ( #21955 ), #52061, .F. ) ;
#47507=CARTESIAN_POINT ( 'NONE',  ( -15.00169697481098297, -0.1191753592594168437, 8.496984177065126431 ) ) ;
#47509=EDGE_LOOP ( 'NONE', ( #21582, #16859, #907, #4452 ) ) ;
#47510=VECTOR ( 'NONE', #21266, 999.9999999999998863 ) ;
#47511=AXIS2_PLACEMENT_3D ( 'NONE', #8977, #26553, #13510 ) ;
#47512=EDGE_LOOP ( 'NONE', ( #10698, #43003, #9754, #7265 ) ) ;
#47513=DIRECTION ( 'NONE',  ( 0.000000000000000000, -1.000000000000000000, 0.000000000000000000 ) ) ;
#47514=FACE_OUTER_BOUND ( 'NONE', #25811, .T. ) ;
#47515=CARTESIAN_POINT ( 'NONE',  ( -13.45720677381246411, 0.000000000000000000, 2.008862543950673540 ) ) ;
#47516=ADVANCED_FACE ( 'NONE', ( #42693 ), #34464, .F. ) ;
#47517=DIRECTION ( 'NONE',  ( -0.005002170337468016433, -0.7660444431189770143, 0.6427681459581293666 ) ) ;
#47518=DIRECTION ( 'NONE',  ( 0.005961354470445682716, -0.6427876096865404731, -0.7660212471507180654 ) ) ;
#47520=FACE_OUTER_BOUND ( 'NONE', #21360, .T. ) ;
#47521=EDGE_LOOP ( 'NONE', ( #13347, #1206, #13077, #31346 ) ) ;
#47522=CARTESIAN_POINT ( 'NONE',  ( -14.07242318112881740, -0.1191753592594177180, 8.504216000601145353 ) ) ;
#47524=DIRECTION ( 'NONE',  ( -0.005961354470445682716, -0.6427876096865404731, 0.7660212471507180654 ) ) ;
#47525=ORIENTED_EDGE ( 'NONE', *, *, #2104, .T. ) ;
#47526=VECTOR ( 'NONE', #53139, 999.9999999999998863 ) ;
#47528=DIRECTION ( 'NONE',  ( 0.007781995580012663651, 0.000000000000000000, -0.9999697198139515519 ) ) ;
#47529=VECTOR ( 'NONE', #8111, 1000.000000000000227 ) ;
#47530=CARTESIAN_POINT ( 'NONE',  ( -16.48488662285251038, 0.000000000000000000, 7.108116401153436570 ) ) ;
#47531=VERTEX_POINT ( 'NONE', #17716 ) ;
#47533=FACE_OUTER_BOUND ( 'NONE', #13101, .T. ) ;
#47534=VECTOR ( 'NONE', #46141, 999.9999999999998863 ) ;
#47535=ORIENTED_EDGE ( 'NONE', *, *, #30371, .F. ) ;
#47536=ADVANCED_FACE ( 'NONE', ( #8641 ), #39011, .F. ) ;
#47537=ORIENTED_EDGE ( 'NONE', *, *, #9788, .T. ) ;
#47538=ORIENTED_EDGE ( 'NONE', *, *, #15351, .T. ) ;
#47539=ORIENTED_EDGE ( 'NONE', *, *, #22259, .T. ) ;
#47540=VECTOR ( 'NONE', #41922, 1000.000000000000114 ) ;
#47541=LINE ( 'NONE', #43825, #53840 ) ;
#47542=EDGE_LOOP ( 'NONE', ( #46780, #50014, #34156, #13158 ) ) ;
#47544=VECTOR ( 'NONE', #46348, 1000.000000000000227 ) ;
#47545=ORIENTED_EDGE ( 'NONE', *, *, #36546, .T. ) ;
#47546=DIRECTION ( 'NONE',  ( 0.6427681459581294776, -0.7660444431189769032, 0.005002170337467562802 ) ) ;
#47547=ORIENTED_EDGE ( 'NONE', *, *, #6221, .F. ) ;
#47548=PLANE ( 'NONE',  #49191 ) ;
#47549=ORIENTED_EDGE ( 'NONE', *, *, #40065, .T. ) ;
#47550=VECTOR ( 'NONE', #45914, 1000.000000000000227 ) ;
#47551=AXIS2_PLACEMENT_3D ( 'NONE', #50428, #51260, #37927 ) ;
#47552=FACE_OUTER_BOUND ( 'NONE', #8262, .T. ) ;
#47553=DIRECTION ( 'NONE',  ( 0.9999697198139515519, 0.000000000000000000, 0.007781995580013368816 ) ) ;
#47554=CARTESIAN_POINT ( 'NONE',  ( -11.64544826116150134, 2.553033558614006271, 5.594771718522403070 ) ) ;
#47555=PLANE ( 'NONE',  #55009 ) ;
#47556=CARTESIAN_POINT ( 'NONE',  ( -1.602266347997184592, -7.552920495778074894, 3.840748238420124139 ) ) ;
#47557=ORIENTED_EDGE ( 'NONE', *, *, #13245, .F. ) ;
#47558=VERTEX_POINT ( 'NONE', #52361 ) ;
#47559=CARTESIAN_POINT ( 'NONE',  ( -15.58595925418828898, -1.975113310420658852, 2.872420537456616074 ) ) ;
#47560=EDGE_CURVE ( 'NONE', #14388, #30483, #4384, .T. ) ;
#47561=LINE ( 'NONE', #43571, #12177 ) ;
#47562=DIRECTION ( 'NONE',  ( 0.9999697198139515519, 0.000000000000000000, 0.007781995580013368816 ) ) ;
#47563=VECTOR ( 'NONE', #6420, 999.9999999999998863 ) ;
#47564=LINE ( 'NONE', #9216, #18697 ) ;
#47565=VECTOR ( 'NONE', #49696, 1000.000000000000227 ) ;
#47566=LINE ( 'NONE', #26013, #22222 ) ;
#47567=DIRECTION ( 'NONE',  ( -0.8531650599175529814, -0.4028455766673920135, 0.3313982828793697877 ) ) ;
#47568=ORIENTED_EDGE ( 'NONE', *, *, #30414, .F. ) ;
#47569=DIRECTION ( 'NONE',  ( 0.007781995580012662783, 0.000000000000000000, -0.9999697198139514409 ) ) ;
#47570=DIRECTION ( 'NONE',  ( -0.5364919789714478471, 0.6444004775717705469, -0.5449076811759709926 ) ) ;
#47571=AXIS2_PLACEMENT_3D ( 'NONE', #51739, #13139, #34175 ) ;
#47572=ORIENTED_EDGE ( 'NONE', *, *, #32861, .T. ) ;
#47573=EDGE_CURVE ( 'NONE', #24462, #1358, #78, .T. ) ;
#47574=PLANE ( 'NONE',  #12532 ) ;
#47575=DIRECTION ( 'NONE',  ( -0.5449076811759708816, 0.6444004775717707689, 0.5364919789714475140 ) ) ;
#47576=CARTESIAN_POINT ( 'NONE',  ( -20.18892918444406348, 0.000000000000000000, 5.401956350015513664 ) ) ;
#47578=EDGE_CURVE ( 'NONE', #38849, #55928, #3792, .T. ) ;
#47582=VERTEX_POINT ( 'NONE', #55771 ) ;
#47583=VECTOR ( 'NONE', #40830, 1000.000000000000227 ) ;
#47584=LINE ( 'NONE', #29981, #22132 ) ;
#47586=LINE ( 'NONE', #3849, #17023 ) ;
#47587=EDGE_CURVE ( 'NONE', #46034, #33489, #16883, .T. ) ;
#47588=VECTOR ( 'NONE', #8899, 1000.000000000000114 ) ;
#47589=CARTESIAN_POINT ( 'NONE',  ( -14.20280369269832832, 0.000000000000000000, 12.40765738797303719 ) ) ;
#47590=EDGE_CURVE ( 'NONE', #678, #27743, #12616, .T. ) ;
#47591=LINE ( 'NONE', #25727, #54789 ) ;
#47592=DIRECTION ( 'NONE',  ( 0.9999697198139515519, 0.000000000000000000, 0.007781995580013368816 ) ) ;
#47593=FACE_OUTER_BOUND ( 'NONE', #31263, .T. ) ;
#47594=ADVANCED_FACE ( 'NONE', ( #40417 ), #53210, .F. ) ;
#47595=ORIENTED_EDGE ( 'NONE', *, *, #10965, .F. ) ;
#47596=AXIS2_PLACEMENT_3D ( 'NONE', #37305, #2099, #53794 ) ;
#47597=CARTESIAN_POINT ( 'NONE',  ( -27.06708303904391144, 0.000000000000000000, 7.395095371555332697 ) ) ;
#47598=VECTOR ( 'NONE', #35345, 999.9999999999998863 ) ;
#47599=DIRECTION ( 'NONE',  ( -0.005002170337468016433, -0.7660444431189770143, 0.6427681459581293666 ) ) ;
#47600=ORIENTED_EDGE ( 'NONE', *, *, #37307, .F. ) ;
#47601=CARTESIAN_POINT ( 'NONE',  ( -11.70325384083886000, -0.1191753592594189115, 2.613340307316962985 ) ) ;
#47602=ORIENTED_EDGE ( 'NONE', *, *, #27977, .F. ) ;
#47603=CARTESIAN_POINT ( 'NONE',  ( -8.836332061905933344, 0.000000000000000000, 5.320978872268770310 ) ) ;
#47604=ADVANCED_FACE ( 'NONE', ( #31335 ), #14845, .F. ) ;
#47605=EDGE_LOOP ( 'NONE', ( #36695, #41341, #14236, #52411 ) ) ;
#47606=VERTEX_POINT ( 'NONE', #19371 ) ;
#47607=VECTOR ( 'NONE', #10208, 999.9999999999998863 ) ;
#47608=ADVANCED_FACE ( 'NONE', ( #1513 ), #5770, .F. ) ;
#47609=ORIENTED_EDGE ( 'NONE', *, *, #16202, .T. ) ;
#47610=ORIENTED_EDGE ( 'NONE', *, *, #9307, .T. ) ;
#47611=ORIENTED_EDGE ( 'NONE', *, *, #36604, .F. ) ;
#47612=VECTOR ( 'NONE', #51596, 999.9999999999998863 ) ;
#47614=DIRECTION ( 'NONE',  ( -0.5449076811759708816, 0.6444004775717707689, 0.5364919789714475140 ) ) ;
#47615=DIRECTION ( 'NONE',  ( -0.9999697198139514409, -0.000000000000000000, -0.007781995580013368816 ) ) ;
#47616=DIRECTION ( 'NONE',  ( 0.005002170337468016433, -0.7660444431189770143, -0.6427681459581293666 ) ) ;
#47617=VECTOR ( 'NONE', #27677, 1000.000000000000227 ) ;
#47618=ORIENTED_EDGE ( 'NONE', *, *, #38661, .F. ) ;
#47619=LINE ( 'NONE', #39091, #48538 ) ;
#47620=VERTEX_POINT ( 'NONE', #23089 ) ;
#47621=VECTOR ( 'NONE', #30385, 999.9999999999998863 ) ;
#47622=VERTEX_POINT ( 'NONE', #22539 ) ;
#47623=VECTOR ( 'NONE', #90, 1000.000000000000000 ) ;
#47624=VECTOR ( 'NONE', #20237, 1000.000000000000114 ) ;
#47625=DIRECTION ( 'NONE',  ( 0.000000000000000000, -0.000000000000000000, -1.000000000000000000 ) ) ;
#47626=AXIS2_PLACEMENT_3D ( 'NONE', #2592, #53446, #54003 ) ;
#47627=LINE ( 'NONE', #12700, #17812 ) ;
#47628=VERTEX_POINT ( 'NONE', #53463 ) ;
#47629=PLANE ( 'NONE',  #36448 ) ;
#47630=ORIENTED_EDGE ( 'NONE', *, *, #47063, .F. ) ;
#47631=AXIS2_PLACEMENT_3D ( 'NONE', #26334, #26617, #39704 ) ;
#47632=DIRECTION ( 'NONE',  ( 0.5449076811759707706, 0.6444004775717708799, -0.5364919789714476250 ) ) ;
#47633=EDGE_CURVE ( 'NONE', #9930, #49888, #36706, .T. ) ;
#47634=CARTESIAN_POINT ( 'NONE',  ( -12.85804337256432639, 5.143464774974015441, 1.512328983069690214 ) ) ;
#47635=VECTOR ( 'NONE', #21627, 1000.000000000000114 ) ;
#47636=CARTESIAN_POINT ( 'NONE',  ( -1.086233639165236964, 0.000000000000000000, -2.796443541562362078 ) ) ;
#47637=VECTOR ( 'NONE', #35293, 999.9999999999998863 ) ;
#47638=CARTESIAN_POINT ( 'NONE',  ( -18.86354292863559579, 0.000000000000000000, 14.21804678658176080 ) ) ;
#47639=CARTESIAN_POINT ( 'NONE',  ( -17.26532721389163072, 0.000000000000000000, 13.67648636611514590 ) ) ;
#47640=CARTESIAN_POINT ( 'NONE',  ( -17.46532115785441519, 0.000000000000000000, 13.67492996699914265 ) ) ;
#47641=CARTESIAN_POINT ( 'NONE',  ( -16.38123739780782984, -0.1191753592594194527, 6.639587925472277163 ) ) ;
#47642=CARTESIAN_POINT ( 'NONE',  ( -20.38395485794165651, 5.143464774974010112, 13.24044338485239081 ) ) ;
#47643=ORIENTED_EDGE ( 'NONE', *, *, #12734, .F. ) ;
#47644=DIRECTION ( 'NONE',  ( -0.5449076811759708816, 0.6444004775717707689, 0.5364919789714475140 ) ) ;
#47645=ADVANCED_FACE ( 'NONE', ( #19087 ), #5227, .F. ) ;
#47646=EDGE_CURVE ( 'NONE', #5305, #39923, #10024, .T. ) ;
#47647=CARTESIAN_POINT ( 'NONE',  ( -23.33693525117809386, 0.000000000000000000, 5.746789908705562944 ) ) ;
#47648=PLANE ( 'NONE',  #32354 ) ;
#47649=DIRECTION ( 'NONE',  ( -0.005002170337468016433, -0.7660444431189770143, 0.6427681459581293666 ) ) ;
#47650=FACE_OUTER_BOUND ( 'NONE', #1242, .T. ) ;
#47651=CARTESIAN_POINT ( 'NONE',  ( -19.05966144679910457, 0.000000000000000000, 5.410744572667534946 ) ) ;
#47652=EDGE_CURVE ( 'NONE', #46401, #35539, #6330, .T. ) ;
#47653=PLANE ( 'NONE',  #24131 ) ;
#47654=VECTOR ( 'NONE', #15793, 1000.000000000000227 ) ;
#47655=FACE_OUTER_BOUND ( 'NONE', #43358, .T. ) ;
#47658=ORIENTED_EDGE ( 'NONE', *, *, #39784, .F. ) ;
#47659=CARTESIAN_POINT ( 'NONE',  ( -17.74482636761137044, -0.1191753592594197858, 3.674319602356483916 ) ) ;
#47660=CARTESIAN_POINT ( 'NONE',  ( -14.66887761629205222, 0.000000000000000000, 12.58869632783390990 ) ) ;
#47661=PLANE ( 'NONE',  #10956 ) ;
#47662=VECTOR ( 'NONE', #34441, 1000.000000000000114 ) ;
#47663=DIRECTION ( 'NONE',  ( 0.5449076811759707706, 0.6444004775717708799, -0.5364919789714476250 ) ) ;
#47664=ADVANCED_FACE ( 'NONE', ( #18843 ), #49494, .F. ) ;
#47665=VECTOR ( 'NONE', #52457, 999.9999999999998863 ) ;
#47667=CARTESIAN_POINT ( 'NONE',  ( -15.96710241509184058, -0.1191753592594218814, 13.13259134697452879 ) ) ;
#47668=CARTESIAN_POINT ( 'NONE',  ( -15.08235377181340198, 0.000000000000000000, 6.011035026684171889 ) ) ;
#47669=EDGE_CURVE ( 'NONE', #45628, #26746, #35888, .T. ) ;
#47670=PLANE ( 'NONE',  #43058 ) ;
#47671=VECTOR ( 'NONE', #47472, 999.9999999999998863 ) ;
#47672=CARTESIAN_POINT ( 'NONE',  ( -27.99845268667336384, -0.1191753592594197858, 7.657176279295684118 ) ) ;
#47673=VECTOR ( 'NONE', #6402, 1000.000000000000114 ) ;
#47674=ADVANCED_FACE ( 'NONE', ( #18250 ), #45227, .F. ) ;
#47675=VERTEX_POINT ( 'NONE', #23380 ) ;
#47676=CARTESIAN_POINT ( 'NONE',  ( -19.26827755127773401, 0.000000000000000000, 6.517117283324824761 ) ) ;
#47677=VECTOR ( 'NONE', #3063, 1000.000000000000227 ) ;
#47678=ADVANCED_FACE ( 'NONE', ( #23630 ), #40947, .T. ) ;
#47679=ORIENTED_EDGE ( 'NONE', *, *, #44720, .T. ) ;
#47680=VECTOR ( 'NONE', #52148, 999.9999999999998863 ) ;
#47681=AXIS2_PLACEMENT_3D ( 'NONE', #24388, #50782, #24127 ) ;
#47682=AXIS2_PLACEMENT_3D ( 'NONE', #31336, #31621, #44383 ) ;
#47683=ORIENTED_EDGE ( 'NONE', *, *, #3652, .F. ) ;
#47684=AXIS2_PLACEMENT_3D ( 'NONE', #52334, #3765, #13437 ) ;
#47685=ORIENTED_EDGE ( 'NONE', *, *, #34652, .F. ) ;
#47686=ORIENTED_EDGE ( 'NONE', *, *, #31577, .F. ) ;
#47687=ORIENTED_EDGE ( 'NONE', *, *, #319, .T. ) ;
#47688=DIRECTION ( 'NONE',  ( 0.007781995580012663651, -3.146120232559066537E-19, -0.9999697198139514409 ) ) ;
#47689=CARTESIAN_POINT ( 'NONE',  ( -20.54126990917373519, -0.1191753592594197858, 4.760553241521720658 ) ) ;
#47691=AXIS2_PLACEMENT_3D ( 'NONE', #9756, #40685, #40400 ) ;
#47693=ORIENTED_EDGE ( 'NONE', *, *, #48849, .F. ) ;
#47694=CARTESIAN_POINT ( 'NONE',  ( -9.088448639303150500, -8.751434906964478344, 0.3118885208565043698 ) ) ;
#47695=CARTESIAN_POINT ( 'NONE',  ( -11.59828696140490223, 0.000000000000000000, 1.975496072340833242 ) ) ;
#47696=ORIENTED_EDGE ( 'NONE', *, *, #33278, .F. ) ;
#47697=VECTOR ( 'NONE', #8117, 1000.000000000000227 ) ;
#47698=FACE_OUTER_BOUND ( 'NONE', #2145, .T. ) ;
#47699=EDGE_CURVE ( 'NONE', #5535, #30132, #40696, .T. ) ;
#47700=ORIENTED_EDGE ( 'NONE', *, *, #19930, .T. ) ;
#47701=LINE ( 'NONE', #35756, #54494 ) ;
#47702=VECTOR ( 'NONE', #23601, 1000.000000000000227 ) ;
#47703=ADVANCED_FACE ( 'NONE', ( #52898 ), #9766, .F. ) ;
#47704=CARTESIAN_POINT ( 'NONE',  ( -14.62059092847759878, 0.000000000000000000, 6.383960641709946593 ) ) ;
#47705=AXIS2_PLACEMENT_3D ( 'NONE', #22985, #27828, #1099 ) ;
#47706=VECTOR ( 'NONE', #52638, 999.9999999999998863 ) ;
#47707=EDGE_LOOP ( 'NONE', ( #20717, #53058, #8858, #51857 ) ) ;
#47708=CARTESIAN_POINT ( 'NONE',  ( -27.99845268667336384, -0.1191753592594197858, 7.657176279295684118 ) ) ;
#47709=CARTESIAN_POINT ( 'NONE',  ( -9.342070512798265725, 0.000000000000000000, 10.59882438848031505 ) ) ;
#47710=DIRECTION ( 'NONE',  ( -0.5449076811759708816, 0.6444004775717707689, 0.5364919789714475140 ) ) ;
#47711=EDGE_CURVE ( 'NONE', #18282, #31194, #48929, .T. ) ;
#47712=LINE ( 'NONE', #42866, #33751 ) ;
#47713=ORIENTED_EDGE ( 'NONE', *, *, #36436, .F. ) ;
#47714=EDGE_CURVE ( 'NONE', #1256, #36728, #41526, .T. ) ;
#47715=VECTOR ( 'NONE', #6378, 999.9999999999998863 ) ;
#47716=ADVANCED_FACE ( 'NONE', ( #45766 ), #33550, .F. ) ;
#47717=EDGE_CURVE ( 'NONE', #24728, #13033, #37532, .T. ) ;
#47718=VECTOR ( 'NONE', #52764, 1000.000000000000227 ) ;
#47719=LINE ( 'NONE', #16465, #37361 ) ;
#47720=DIRECTION ( 'NONE',  ( 0.005002170337468016433, -0.7660444431189770143, -0.6427681459581293666 ) ) ;
#47721=DIRECTION ( 'NONE',  ( 0.5449076811759707706, 0.6444004775717708799, -0.5364919789714476250 ) ) ;
#47722=CARTESIAN_POINT ( 'NONE',  ( -21.47341775636118655, -0.1191753592594197858, 5.122631121243466090 ) ) ;
#47723=CARTESIAN_POINT ( 'NONE',  ( -18.39746900504187010, 0.000000000000000000, 14.03700784672088808 ) ) ;
#47724=EDGE_CURVE ( 'NONE', #10313, #8687, #3459, .T. ) ;
#47725=DIRECTION ( 'NONE',  ( 0.7660212471507180654, -0.6427876096865404731, 0.005961354470445141482 ) ) ;
#47726=CARTESIAN_POINT ( 'NONE',  ( -20.34003895477433588, 0.5857317160611430484, 5.278610298956506242 ) ) ;
#47729=DIRECTION ( 'NONE',  ( 0.6427681459581294776, -0.7660444431189769032, 0.005002170337467562802 ) ) ;
#47730=LINE ( 'NONE', #21312, #26787 ) ;
#47732=ORIENTED_EDGE ( 'NONE', *, *, #41993, .T. ) ;
#47733=FACE_OUTER_BOUND ( 'NONE', #30291, .T. ) ;
#47734=DIRECTION ( 'NONE',  ( 0.007781995580012663651, -3.146120232559066537E-19, -0.9999697198139514409 ) ) ;
#47735=LINE ( 'NONE', #51688, #12804 ) ;
#47736=CARTESIAN_POINT ( 'NONE',  ( -2.207734231944874725, 7.028681301134739989, 4.075932526321295768 ) ) ;
#47737=EDGE_CURVE ( 'NONE', #41560, #16128, #6894, .T. ) ;
#47739=AXIS2_PLACEMENT_3D ( 'NONE', #25443, #51578, #43057 ) ;
#47740=ORIENTED_EDGE ( 'NONE', *, *, #33091, .F. ) ;
#47741=EDGE_CURVE ( 'NONE', #26517, #28129, #15655, .T. ) ;
#47742=ORIENTED_EDGE ( 'NONE', *, *, #47852, .T. ) ;
#47743=EDGE_CURVE ( 'NONE', #14924, #53717, #15962, .T. ) ;
#47744=FACE_OUTER_BOUND ( 'NONE', #41785, .T. ) ;
#47745=DIRECTION ( 'NONE',  ( 0.5449076811759707706, 0.6444004775717708799, -0.5364919789714476250 ) ) ;
#47746=ORIENTED_EDGE ( 'NONE', *, *, #22696, .F. ) ;
#47747=VECTOR ( 'NONE', #39485, 1000.000000000000114 ) ;
#47748=DIRECTION ( 'NONE',  ( 0.000000000000000000, -1.000000000000000000, 0.000000000000000000 ) ) ;
#47749=EDGE_CURVE ( 'NONE', #49950, #7904, #6592, .T. ) ;
#47750=VERTEX_POINT ( 'NONE', #15143 ) ;
#47751=FACE_OUTER_BOUND ( 'NONE', #6743, .T. ) ;
#47752=VECTOR ( 'NONE', #17143, 999.9999999999998863 ) ;
#47753=ORIENTED_EDGE ( 'NONE', *, *, #33967, .T. ) ;
#47754=DIRECTION ( 'NONE',  ( -0.7660212471507179544, -0.6427876096865405842, -0.005961354470445141482 ) ) ;
#47755=EDGE_CURVE ( 'NONE', #14310, #44131, #54292, .T. ) ;
#47756=AXIS2_PLACEMENT_3D ( 'NONE', #29485, #12151, #33460 ) ;
#47757=VERTEX_POINT ( 'NONE', #2333 ) ;
#47758=ORIENTED_EDGE ( 'NONE', *, *, #55858, .F. ) ;
#47760=CARTESIAN_POINT ( 'NONE',  ( -15.66124530601080700, -1.489407457353157049, 5.209662645942111148 ) ) ;
#47761=PLANE ( 'NONE',  #6021 ) ;
#47762=CARTESIAN_POINT ( 'NONE',  ( -15.87975247367846166, 0.000000000000000000, 2.850166870931599927 ) ) ;
#47763=VECTOR ( 'NONE', #52640, 1000.000000000000114 ) ;
#47764=DIRECTION ( 'NONE',  ( -0.005002170337468016433, -0.7660444431189770143, 0.6427681459581293666 ) ) ;
#47765=VERTEX_POINT ( 'NONE', #32996 ) ;
#47766=ORIENTED_EDGE ( 'NONE', *, *, #4687, .F. ) ;
#47767=VECTOR ( 'NONE', #10745, 1000.000000000000227 ) ;
#47768=AXIS2_PLACEMENT_3D ( 'NONE', #2391, #51207, #6951 ) ;
#47770=DIRECTION ( 'NONE',  ( 0.9999697198139515519, 0.000000000000000000, 0.007781995580013368816 ) ) ;
#47771=VERTEX_POINT ( 'NONE', #33298 ) ;
#47772=LINE ( 'NONE', #34155, #52013 ) ;
#47773=ORIENTED_EDGE ( 'NONE', *, *, #41669, .F. ) ;
#47774=DIRECTION ( 'NONE',  ( 0.7660212471507180654, -0.6427876096865404731, 0.005961354470445141482 ) ) ;
#47775=DIRECTION ( 'NONE',  ( 0.5449076811759707706, 0.6444004775717708799, -0.5364919789714476250 ) ) ;
#47776=ORIENTED_EDGE ( 'NONE', *, *, #12784, .F. ) ;
#47777=CARTESIAN_POINT ( 'NONE',  ( -14.56888064431065821, -0.1191753592594197858, 12.58947452739191064 ) ) ;
#47778=ORIENTED_EDGE ( 'NONE', *, *, #18897, .F. ) ;
#47779=AXIS2_PLACEMENT_3D ( 'NONE', #3128, #11666, #28983 ) ;
#47780=PLANE ( 'NONE',  #18201 ) ;
#47781=ORIENTED_EDGE ( 'NONE', *, *, #53050, .F. ) ;
#47782=DIRECTION ( 'NONE',  ( -0.5449076811759708816, 0.6444004775717707689, 0.5364919789714475140 ) ) ;
#47783=PLANE ( 'NONE',  #21189 ) ;
#47784=DIRECTION ( 'NONE',  ( 0.5364919789714477361, 0.6444004775717706579, 0.5449076811759711036 ) ) ;
#47785=ORIENTED_EDGE ( 'NONE', *, *, #43431, .F. ) ;
#47786=ADVANCED_FACE ( 'NONE', ( #32459 ), #46057, .F. ) ;
#47787=EDGE_CURVE ( 'NONE', #1287, #55683, #50308, .T. ) ;
#47788=CARTESIAN_POINT ( 'NONE',  ( -14.10280672071693431, -0.1191753592594197858, 12.40843558753103792 ) ) ;
#47789=CARTESIAN_POINT ( 'NONE',  ( 2.072287782118878319, 0.000000000000000000, -2.950529333540147015 ) ) ;
#47790=VECTOR ( 'NONE', #18316, 999.9999999999998863 ) ;
#47791=CARTESIAN_POINT ( 'NONE',  ( -17.73140113748535285, 0.000000000000000000, 13.85752530597602039 ) ) ;
#47792=CARTESIAN_POINT ( 'NONE',  ( -17.26532721389163072, 0.000000000000000000, 13.67648636611514590 ) ) ;
#47793=ADVANCED_FACE ( 'NONE', ( #10859 ), #25055, .F. ) ;
#47794=CARTESIAN_POINT ( 'NONE',  ( -14.72233906693923267, 5.143464774974014553, 2.236484742513179746 ) ) ;
#47795=LINE ( 'NONE', #30748, #23395 ) ;
#47796=AXIS2_PLACEMENT_3D ( 'NONE', #6946, #41294, #16019 ) ;
#47797=CARTESIAN_POINT ( 'NONE',  ( -23.33693525117809386, 0.000000000000000000, 5.746789908705562944 ) ) ;
#47798=EDGE_LOOP ( 'NONE', ( #33379, #2665, #18791, #31653 ) ) ;
#47799=DIRECTION ( 'NONE',  ( 0.3313982828793700097, 0.4028455766673916805, 0.8531650599175528704 ) ) ;
#47801=CARTESIAN_POINT ( 'NONE',  ( -18.82703149329399395, -0.8417996532631562001, 4.167521701613545737 ) ) ;
#47802=EDGE_LOOP ( 'NONE', ( #44062, #23620, #27551, #50748 ) ) ;
#47803=DIRECTION ( 'NONE',  ( 0.9999697198139515519, 0.000000000000000000, 0.007781995580013368816 ) ) ;
#47804=ORIENTED_EDGE ( 'NONE', *, *, #27568, .T. ) ;
#47805=DIRECTION ( 'NONE',  ( -0.7660212471507179544, -0.6427876096865405842, -0.005961354470445141482 ) ) ;
#47806=VECTOR ( 'NONE', #10489, 999.9999999999998863 ) ;
#47807=DIRECTION ( 'NONE',  ( -0.5364919789714478471, 0.6444004775717705469, -0.5449076811759709926 ) ) ;
#47808=DIRECTION ( 'NONE',  ( 0.007781995580012663651, -3.146120232559066537E-19, -0.9999697198139514409 ) ) ;
#47809=DIRECTION ( 'NONE',  ( 0.000000000000000000, -1.000000000000000000, 0.000000000000000000 ) ) ;
#47810=VERTEX_POINT ( 'NONE', #15390 ) ;
#47811=AXIS2_PLACEMENT_3D ( 'NONE', #10215, #14758, #5676 ) ;
#47812=ORIENTED_EDGE ( 'NONE', *, *, #51502, .F. ) ;
#47813=DIRECTION ( 'NONE',  ( 0.000000000000000000, -0.000000000000000000, -1.000000000000000000 ) ) ;
#47814=LINE ( 'NONE', #663, #41329 ) ;
#47815=CARTESIAN_POINT ( 'NONE',  ( 2.072287782118878319, 0.000000000000000000, -2.950529333540147015 ) ) ;
#47816=FACE_OUTER_BOUND ( 'NONE', #33518, .T. ) ;
#47817=DIRECTION ( 'NONE',  ( 0.007781995580012662783, 0.000000000000000000, -0.9999697198139514409 ) ) ;
#47818=DIRECTION ( 'NONE',  ( 0.005961354470445682716, -0.6427876096865404731, -0.7660212471507180654 ) ) ;
#47819=ORIENTED_EDGE ( 'NONE', *, *, #52302, .T. ) ;
#47820=FACE_OUTER_BOUND ( 'NONE', #5867, .T. ) ;
#47821=EDGE_CURVE ( 'NONE', #37913, #54234, #29015, .T. ) ;
#47822=DIRECTION ( 'NONE',  ( -0.9999697198139514409, -0.000000000000000000, -0.007781995580013368816 ) ) ;
#47823=ORIENTED_EDGE ( 'NONE', *, *, #16838, .T. ) ;
#47824=ADVANCED_FACE ( 'NONE', ( #28753 ), #50015, .F. ) ;
#47825=DIRECTION ( 'NONE',  ( 0.9999697198139515519, 0.000000000000000000, 0.007781995580013368816 ) ) ;
#47826=CARTESIAN_POINT ( 'NONE',  ( -14.01701317841955508, 0.000000000000000000, 2.326005055450897085 ) ) ;
#47827=LINE ( 'NONE', #8931, #11256 ) ;
#47828=EDGE_LOOP ( 'NONE', ( #38113, #30001, #32635, #31052 ) ) ;
#47829=DIRECTION ( 'NONE',  ( 0.9999697198139515519, 0.000000000000000000, 0.007781995580013368816 ) ) ;
#47830=EDGE_CURVE ( 'NONE', #53467, #33120, #29287, .T. ) ;
#47831=VERTEX_POINT ( 'NONE', #20194 ) ;
#47832=EDGE_LOOP ( 'NONE', ( #47141, #17359, #42021, #33784 ) ) ;
#47833=AXIS2_PLACEMENT_3D ( 'NONE', #20333, #19789, #33966 ) ;
#47834=VERTEX_POINT ( 'NONE', #46311 ) ;
#47835=ORIENTED_EDGE ( 'NONE', *, *, #2754, .F. ) ;
#47836=DIRECTION ( 'NONE',  ( 0.9999697198139515519, 0.000000000000000000, 0.007781995580013368816 ) ) ;
#47837=ORIENTED_EDGE ( 'NONE', *, *, #4675, .F. ) ;
#47839=VECTOR ( 'NONE', #10056, 999.9999999999998863 ) ;
#47840=EDGE_LOOP ( 'NONE', ( #10720, #27483, #13333, #29583 ) ) ;
#47841=LINE ( 'NONE', #4948, #37683 ) ;
#47842=VERTEX_POINT ( 'NONE', #7422 ) ;
#47843=DIRECTION ( 'NONE',  ( 0.6427681459581294776, -0.7660444431189769032, 0.005002170337467562802 ) ) ;
#47844=ORIENTED_EDGE ( 'NONE', *, *, #47390, .F. ) ;
#47845=DIRECTION ( 'NONE',  ( -0.005961354470445682716, -0.6427876096865404731, 0.7660212471507180654 ) ) ;
#47846=LINE ( 'NONE', #34770, #26831 ) ;
#47847=DIRECTION ( 'NONE',  ( -0.7660212471507179544, -0.6427876096865405842, -0.005961354470445141482 ) ) ;
#47848=DIRECTION ( 'NONE',  ( 0.5449076811759707706, 0.6444004775717708799, -0.5364919789714476250 ) ) ;
#47849=EDGE_CURVE ( 'NONE', #14819, #18282, #42065, .T. ) ;
#47850=CARTESIAN_POINT ( 'NONE',  ( -17.74404816805336793, 0.000000000000000000, 3.574322630375089460 ) ) ;
#47851=ORIENTED_EDGE ( 'NONE', *, *, #12053, .T. ) ;
#47852=EDGE_CURVE ( 'NONE', #44098, #33926, #8012, .T. ) ;
#47853=EDGE_LOOP ( 'NONE', ( #14784, #28421, #55153, #6374 ) ) ;
#47854=PLANE ( 'NONE',  #38553 ) ;
#47855=CARTESIAN_POINT ( 'NONE',  ( -29.86197018149027116, 0.000000000000000000, 8.281335066757780083 ) ) ;
#47856=EDGE_CURVE ( 'NONE', #48678, #42632, #43477, .T. ) ;
#47857=ADVANCED_FACE ( 'NONE', ( #4021 ), #48016, .F. ) ;
#47858=PLANE ( 'NONE',  #19700 ) ;
#47859=DIRECTION ( 'NONE',  ( 0.000000000000000000, -0.000000000000000000, -1.000000000000000000 ) ) ;
#47860=PLANE ( 'NONE',  #15839 ) ;
#47861=CARTESIAN_POINT ( 'NONE',  ( -11.77243710274829525, -0.1191753592594197858, 11.50324088822667612 ) ) ;
#47862=ORIENTED_EDGE ( 'NONE', *, *, #1593, .F. ) ;
#47863=CARTESIAN_POINT ( 'NONE',  ( -18.39746900504187010, 0.000000000000000000, 14.03700784672088808 ) ) ;
#47864=LINE ( 'NONE', #31078, #6835 ) ;
#47865=VERTEX_POINT ( 'NONE', #13105 ) ;
#47867=CARTESIAN_POINT ( 'NONE',  ( -18.61226887098971261, 0.000000000000000000, 7.630218703982132311 ) ) ;
#47868=FACE_OUTER_BOUND ( 'NONE', #11193, .T. ) ;
#47869=CARTESIAN_POINT ( 'NONE',  ( -15.79151524699580555, 0.000000000000000000, 3.420191679459803957 ) ) ;
#47870=CARTESIAN_POINT ( 'NONE',  ( -13.53673582514181106, 0.000000000000000000, 12.22817484722816772 ) ) ;
#47871=ADVANCED_FACE ( 'NONE', ( #8865 ), #34666, .F. ) ;
#47872=LINE ( 'NONE', #33733, #46451 ) ;
#47873=VERTEX_POINT ( 'NONE', #3723 ) ;
#47874=EDGE_LOOP ( 'NONE', ( #53661, #28601, #2005, #26145 ) ) ;
#47875=PLANE ( 'NONE',  #4915 ) ;
#47876=FACE_OUTER_BOUND ( 'NONE', #14769, .T. ) ;
#47877=DIRECTION ( 'NONE',  ( 0.7660212471507180654, -0.6427876096865404731, 0.005961354470445141482 ) ) ;
#47878=AXIS2_PLACEMENT_3D ( 'NONE', #17120, #29049, #47201 ) ;
#47879=PLANE ( 'NONE',  #21913 ) ;
#47880=FACE_OUTER_BOUND ( 'NONE', #16655, .T. ) ;
#47881=LINE ( 'NONE', #1576, #41858 ) ;
#47882=DIRECTION ( 'NONE',  ( 0.000000000000000000, -1.000000000000000000, 0.000000000000000000 ) ) ;
#47883=ORIENTED_EDGE ( 'NONE', *, *, #53891, .T. ) ;
#47884=DIRECTION ( 'NONE',  ( -0.5364919789714478471, 0.6444004775717705469, -0.5449076811759709926 ) ) ;
#47885=DIRECTION ( 'NONE',  ( 0.5449076811759707706, 0.6444004775717708799, -0.5364919789714476250 ) ) ;
#47886=ORIENTED_EDGE ( 'NONE', *, *, #36641, .F. ) ;
#47887=DIRECTION ( 'NONE',  ( 0.5449076811759707706, 0.6444004775717708799, -0.5364919789714476250 ) ) ;
#47888=ORIENTED_EDGE ( 'NONE', *, *, #33420, .T. ) ;
#47889=FACE_OUTER_BOUND ( 'NONE', #15084, .T. ) ;
#47890=CARTESIAN_POINT ( 'NONE',  ( -21.19256270521356100, 3.362543313726507499, 10.63173860971578577 ) ) ;
#47891=VERTEX_POINT ( 'NONE', #21041 ) ;
#47892=EDGE_CURVE ( 'NONE', #16343, #31601, #47453, .T. ) ;
#47893=ORIENTED_EDGE ( 'NONE', *, *, #43279, .F. ) ;
#47894=ORIENTED_EDGE ( 'NONE', *, *, #12913, .T. ) ;
#47895=ORIENTED_EDGE ( 'NONE', *, *, #41088, .T. ) ;
#47896=VERTEX_POINT ( 'NONE', #29867 ) ;
#47898=LINE ( 'NONE', #12690, #55011 ) ;
#47899=DIRECTION ( 'NONE',  ( 0.5449076811759707706, 0.6444004775717708799, -0.5364919789714476250 ) ) ;
#47900=DIRECTION ( 'NONE',  ( -0.5449076811759708816, 0.6444004775717707689, 0.5364919789714475140 ) ) ;
#47901=EDGE_CURVE ( 'NONE', #13341, #41396, #42910, .T. ) ;
#47902=VERTEX_POINT ( 'NONE', #17343 ) ;
#47903=LINE ( 'NONE', #7897, #41284 ) ;
#47904=ORIENTED_EDGE ( 'NONE', *, *, #38161, .T. ) ;
#47905=ADVANCED_FACE ( 'NONE', ( #51455 ), #30716, .F. ) ;
#47906=EDGE_LOOP ( 'NONE', ( #11142, #38395, #38933, #51957 ) ) ;
#47907=EDGE_CURVE ( 'NONE', #50552, #19938, #8269, .T. ) ;
#47908=DIRECTION ( 'NONE',  ( 0.000000000000000000, -1.000000000000000000, 0.000000000000000000 ) ) ;
#47909=CARTESIAN_POINT ( 'NONE',  ( -11.77950995886804719, -2.946525016555658905, 6.093242968378755897 ) ) ;
#47910=CARTESIAN_POINT ( 'NONE',  ( -17.74404816805336793, 0.000000000000000000, 3.574322630375089460 ) ) ;
#47911=EDGE_CURVE ( 'NONE', #16557, #30900, #25587, .T. ) ;
#47912=ORIENTED_EDGE ( 'NONE', *, *, #36238, .F. ) ;
#47913=FACE_OUTER_BOUND ( 'NONE', #4524, .T. ) ;
#47914=VERTEX_POINT ( 'NONE', #38675 ) ;
#47915=AXIS2_PLACEMENT_3D ( 'NONE', #39479, #264, #5396 ) ;
#47916=CARTESIAN_POINT ( 'NONE',  ( -19.07846216694679953, 0.000000000000000000, 7.826596736176912650 ) ) ;
#47917=EDGE_CURVE ( 'NONE', #41918, #7829, #22180, .T. ) ;
#47918=DIRECTION ( 'NONE',  ( -0.5364919789714478471, 0.6444004775717705469, -0.5449076811759709926 ) ) ;
#47919=EDGE_CURVE ( 'NONE', #40788, #29014, #55996, .T. ) ;
#47920=FACE_OUTER_BOUND ( 'NONE', #55943, .T. ) ;
#47921=LINE ( 'NONE', #9019, #40410 ) ;
#47923=CARTESIAN_POINT ( 'NONE',  ( -10.43442840428654073, 0.000000000000000000, 5.847200200401478476 ) ) ;
#47924=DIRECTION ( 'NONE',  ( -0.6246952433987894571, 0.7422098413412802076, 0.2426528472758539834 ) ) ;
#47926=ORIENTED_EDGE ( 'NONE', *, *, #26719, .F. ) ;
#47927=CARTESIAN_POINT ( 'NONE',  ( -14.51438381650843468, 4.819660872929010687, 10.42908529298719778 ) ) ;
#47928=EDGE_CURVE ( 'NONE', #51537, #13509, #16504, .T. ) ;
#47930=DIRECTION ( 'NONE',  ( 0.9999697198139515519, 0.000000000000000000, 0.007781995580013368816 ) ) ;
#47931=DIRECTION ( 'NONE',  ( 0.005002170337468016433, -0.7660444431189770143, -0.6427681459581293666 ) ) ;
#47933=DIRECTION ( 'NONE',  ( 0.005961354470445682716, -0.6427876096865404731, -0.7660212471507180654 ) ) ;
#47934=LINE ( 'NONE', #4228, #7806 ) ;
#47936=LINE ( 'NONE', #39122, #28312 ) ;
#47937=EDGE_LOOP ( 'NONE', ( #23674, #35438, #9580, #56001 ) ) ;
#47938=FACE_OUTER_BOUND ( 'NONE', #22524, .T. ) ;
#47939=FACE_OUTER_BOUND ( 'NONE', #24968, .T. ) ;
#47940=FACE_OUTER_BOUND ( 'NONE', #51089, .T. ) ;
#47941=LINE ( 'NONE', #17007, #42709 ) ;
#47942=CARTESIAN_POINT ( 'NONE',  ( -19.17193283235963008, -0.1191753592594166911, 6.987202158121982087 ) ) ;
#47943=DIRECTION ( 'NONE',  ( 0.9999697198139515519, 0.000000000000000000, 0.007781995580013368816 ) ) ;
#47944=DIRECTION ( 'NONE',  ( -0.7660212471507179544, -0.6427876096865405842, -0.005961354470445141482 ) ) ;
#47945=DIRECTION ( 'NONE',  ( 0.000000000000000000, -0.000000000000000000, -1.000000000000000000 ) ) ;
#47947=EDGE_LOOP ( 'NONE', ( #33686, #51000, #30255, #32993 ) ) ;
#47948=CARTESIAN_POINT ( 'NONE',  ( -16.99924723426068951, 0.000000000000000000, 13.49389102713827171 ) ) ;
#47949=AXIS2_PLACEMENT_3D ( 'NONE', #38992, #33594, #55 ) ;
#47950=VERTEX_POINT ( 'NONE', #34405 ) ;
#47951=EDGE_CURVE ( 'NONE', #30420, #53062, #51706, .T. ) ;
#47952=ORIENTED_EDGE ( 'NONE', *, *, #50461, .F. ) ;
#47953=ORIENTED_EDGE ( 'NONE', *, *, #25179, .T. ) ;
#47954=ORIENTED_EDGE ( 'NONE', *, *, #44980, .F. ) ;
#47955=ORIENTED_EDGE ( 'NONE', *, *, #21885, .F. ) ;
#47956=DIRECTION ( 'NONE',  ( 0.000000000000000000, -1.000000000000000000, 0.000000000000000000 ) ) ;
#47957=LINE ( 'NONE', #47689, #34864 ) ;
#47958=EDGE_LOOP ( 'NONE', ( #23802, #35398, #16620, #8850 ) ) ;
#47959=VERTEX_POINT ( 'NONE', #4322 ) ;
#47960=EDGE_CURVE ( 'NONE', #5651, #46530, #34980, .T. ) ;
#47962=EDGE_LOOP ( 'NONE', ( #49564, #55062, #16911, #14290 ) ) ;
#47963=LINE ( 'NONE', #22119, #11029 ) ;
#47964=LINE ( 'NONE', #9064, #2295 ) ;
#47966=DIRECTION ( 'NONE',  ( 0.7660212471507180654, -0.6427876096865404731, 0.005961354470445141482 ) ) ;
#47967=ORIENTED_EDGE ( 'NONE', *, *, #4863, .F. ) ;
#47968=LINE ( 'NONE', #43686, #44529 ) ;
#47969=EDGE_CURVE ( 'NONE', #2279, #8289, #51151, .T. ) ;
#47970=EDGE_CURVE ( 'NONE', #39093, #45157, #52821, .T. ) ;
#47971=LINE ( 'NONE', #20735, #23634 ) ;
#47972=ORIENTED_EDGE ( 'NONE', *, *, #2429, .F. ) ;
#47973=PLANE ( 'NONE',  #5915 ) ;
#47974=FACE_OUTER_BOUND ( 'NONE', #51084, .T. ) ;
#47975=CARTESIAN_POINT ( 'NONE',  ( -10.94028622754223967, 0.000000000000000000, 11.14038480894692995 ) ) ;
#47977=CARTESIAN_POINT ( 'NONE',  ( -12.30199656298181132, -0.8417996532631574214, 1.632976543561326821 ) ) ;
#47978=EDGE_LOOP ( 'NONE', ( #28496, #27260, #5246, #51996 ) ) ;
#47979=EDGE_CURVE ( 'NONE', #29147, #29422, #9700, .T. ) ;
#47981=FACE_OUTER_BOUND ( 'NONE', #5173, .T. ) ;
#47982=DIRECTION ( 'NONE',  ( 0.007781995580012662783, 0.000000000000000000, -0.9999697198139514409 ) ) ;
#47983=LINE ( 'NONE', #13892, #3125 ) ;
#47984=DIRECTION ( 'NONE',  ( 0.000000000000000000, -0.000000000000000000, -1.000000000000000000 ) ) ;
#47986=PLANE ( 'NONE',  #39443 ) ;
#47989=DIRECTION ( 'NONE',  ( 0.5364919789714477361, 0.6444004775717706579, 0.5449076811759711036 ) ) ;
#47991=DIRECTION ( 'NONE',  ( -0.005961354470445682716, -0.6427876096865404731, 0.7660212471507180654 ) ) ;
#47992=ORIENTED_EDGE ( 'NONE', *, *, #23850, .F. ) ;
#47994=CARTESIAN_POINT ( 'NONE',  ( -13.17065887352947762, -0.1191753592594197858, 12.04635770780929427 ) ) ;
#47995=CARTESIAN_POINT ( 'NONE',  ( -14.58996710526761120, 0.000000000000000000, 2.448865125390635278 ) ) ;
#47996=DIRECTION ( 'NONE',  ( 0.6427681459581294776, -0.7660444431189769032, 0.005002170337467562802 ) ) ;
#47997=DIRECTION ( 'NONE',  ( 0.5364919789714477361, 0.6444004775717706579, 0.5449076811759711036 ) ) ;
#47998=LINE ( 'NONE', #53117, #50107 ) ;
#47999=EDGE_LOOP ( 'NONE', ( #11638, #7039, #21640, #26300 ) ) ;
#48000=ORIENTED_EDGE ( 'NONE', *, *, #45155, .F. ) ;
#48001=CARTESIAN_POINT ( 'NONE',  ( -13.04137698704457904, 0.000000000000000000, 8.284087284458621525 ) ) ;
#48002=CARTESIAN_POINT ( 'NONE',  ( -11.67244013076689946, 0.000000000000000000, 11.50401908778467863 ) ) ;
#48003=ORIENTED_EDGE ( 'NONE', *, *, #45443, .T. ) ;
#48004=EDGE_CURVE ( 'NONE', #34779, #4575, #45172, .T. ) ;
#48005=CARTESIAN_POINT ( 'NONE',  ( 2.072287782118878319, 0.000000000000000000, -2.950529333540147015 ) ) ;
#48006=ORIENTED_EDGE ( 'NONE', *, *, #54297, .T. ) ;
#48007=CARTESIAN_POINT ( 'NONE',  ( -18.98470430123549946, -2.137015261443159009, 4.187443015709999550 ) ) ;
#48008=EDGE_CURVE ( 'NONE', #14391, #2309, #9964, .T. ) ;
#48009=ORIENTED_EDGE ( 'NONE', *, *, #19422, .F. ) ;
#48010=DIRECTION ( 'NONE',  ( -0.5364919789714478471, 0.6444004775717705469, -0.5449076811759709926 ) ) ;
#48011=ORIENTED_EDGE ( 'NONE', *, *, #306, .F. ) ;
#48012=VERTEX_POINT ( 'NONE', #27554 ) ;
#48013=EDGE_CURVE ( 'NONE', #1358, #29284, #44322, .T. ) ;
#48014=VERTEX_POINT ( 'NONE', #5160 ) ;
#48015=ADVANCED_FACE ( 'NONE', ( #9393 ), #1439, .F. ) ;
#48016=PLANE ( 'NONE',  #6654 ) ;
#48017=DIRECTION ( 'NONE',  ( -0.6427681459581293666, -0.7660444431189770143, -0.005002170337467561935 ) ) ;
#48018=CARTESIAN_POINT ( 'NONE',  ( -4.032439601142493224, -5.958259985714265738, 4.784710058972824420 ) ) ;
#48019=EDGE_CURVE ( 'NONE', #7643, #44870, #1135, .T. ) ;
#48020=EDGE_CURVE ( 'NONE', #7759, #45468, #48278, .T. ) ;
#48021=ADVANCED_FACE ( 'NONE', ( #6273 ), #14778, .T. ) ;
#48022=LINE ( 'NONE', #39793, #9327 ) ;
#48023=VERTEX_POINT ( 'NONE', #53405 ) ;
#48025=DIRECTION ( 'NONE',  ( 0.5449076811759707706, 0.6444004775717708799, -0.5364919789714476250 ) ) ;
#48026=ORIENTED_EDGE ( 'NONE', *, *, #21365, .T. ) ;
#48027=DIRECTION ( 'NONE',  ( -0.6427681459581293666, -0.7660444431189770143, -0.005002170337467561935 ) ) ;
#48030=DIRECTION ( 'NONE',  ( 0.005002170337468016433, -0.7660444431189770143, -0.6427681459581293666 ) ) ;
#48031=ORIENTED_EDGE ( 'NONE', *, *, #17691, .T. ) ;
#48032=CARTESIAN_POINT ( 'NONE',  ( -32.65841372305263235, 0.000000000000000000, 9.367568705923016381 ) ) ;
#48033=EDGE_CURVE ( 'NONE', #23836, #23840, #14501, .T. ) ;
#48034=ORIENTED_EDGE ( 'NONE', *, *, #10188, .F. ) ;
#48035=EDGE_CURVE ( 'NONE', #2673, #39014, #39789, .T. ) ;
#48036=LINE ( 'NONE', #35005, #1896 ) ;
#48037=ORIENTED_EDGE ( 'NONE', *, *, #43492, .T. ) ;
#48038=DIRECTION ( 'NONE',  ( 0.6427681459581294776, -0.7660444431189769032, 0.005002170337467562802 ) ) ;
#48039=CARTESIAN_POINT ( 'NONE',  ( -22.02184903649736469, 3.848249166794010634, 5.113186466190691171 ) ) ;
#48040=EDGE_CURVE ( 'NONE', #18921, #4591, #27862, .T. ) ;
#48041=CARTESIAN_POINT ( 'NONE',  ( -14.66887761629205222, 0.000000000000000000, 12.58869632783390990 ) ) ;
#48042=VERTEX_POINT ( 'NONE', #609 ) ;
#48043=FACE_OUTER_BOUND ( 'NONE', #20990, .T. ) ;
#48044=ADVANCED_FACE ( 'NONE', ( #17937 ), #26714, .F. ) ;
#48045=LINE ( 'NONE', #17115, #10142 ) ;
#48046=DIRECTION ( 'NONE',  ( 0.5364919789714477361, 0.6444004775717706579, 0.5449076811759711036 ) ) ;
#48047=CARTESIAN_POINT ( 'NONE',  ( -12.36248183396243583, -0.3560938001956550081, 2.068350099266224262 ) ) ;
#48048=CARTESIAN_POINT ( 'NONE',  ( -15.50102849149811135, -0.1191753592594197858, 12.95155240711365430 ) ) ;
#48049=DIRECTION ( 'NONE',  ( -0.9999697198139514409, -0.000000000000000000, -0.007781995580013368816 ) ) ;
#48050=FILL_AREA_STYLE_COLOUR ( '', #43083 ) ;
#48051=ORIENTED_EDGE ( 'NONE', *, *, #8696, .T. ) ;
#48052=CARTESIAN_POINT ( 'NONE',  ( -13.67826452165829565, 0.000000000000000000, 4.713959708252118297 ) ) ;
#48053=DIRECTION ( 'NONE',  ( 0.005002170337468016433, -0.7660444431189770143, -0.6427681459581293666 ) ) ;
#48054=CARTESIAN_POINT ( 'NONE',  ( -20.54126990917373874, -1.000000000000000000, 4.760553241521714440 ) ) ;
#48055=ORIENTED_EDGE ( 'NONE', *, *, #35877, .F. ) ;
#48056=DIRECTION ( 'NONE',  ( 0.000000000000000000, -0.000000000000000000, -1.000000000000000000 ) ) ;
#48057=PLANE ( 'NONE',  #29978 ) ;
#48058=EDGE_LOOP ( 'NONE', ( #12228, #18065, #44045, #2705 ) ) ;
#48059=LINE ( 'NONE', #31602, #25290 ) ;
#48060=DIRECTION ( 'NONE',  ( 0.007781995580012663651, 0.000000000000000000, -0.9999697198139515519 ) ) ;
#48061=CARTESIAN_POINT ( 'NONE',  ( -10.84028925556084388, -0.1191753592594197858, 11.14116300850493246 ) ) ;
#48062=CARTESIAN_POINT ( 'NONE',  ( -18.82088497546834915, 0.000000000000000000, 8.736591414639422126 ) ) ;
#48063=EDGE_LOOP ( 'NONE', ( #3023, #52425, #14330, #25847 ) ) ;
#48065=FACE_OUTER_BOUND ( 'NONE', #23379, .T. ) ;
#48066=CARTESIAN_POINT ( 'NONE',  ( -28.92982233430281980, 0.000000000000000000, 7.919257187036034651 ) ) ;
#48067=CARTESIAN_POINT ( 'NONE',  ( -28.93060053386082231, -0.1191753592594197858, 8.019254159017428663 ) ) ;
#48068=CARTESIAN_POINT ( 'NONE',  ( -19.21426901291696865, -0.1941918491731554619, 4.338599984426191547 ) ) ;
#48069=DIRECTION ( 'NONE',  ( -0.9999697198139514409, -0.000000000000000000, -0.007781995580013368816 ) ) ;
#48070=DIRECTION ( 'NONE',  ( 0.9999697198139515519, 0.000000000000000000, 0.007781995580013368816 ) ) ;
#48071=ORIENTED_EDGE ( 'NONE', *, *, #51642, .F. ) ;
#48072=FACE_OUTER_BOUND ( 'NONE', #43712, .T. ) ;
#48073=DIRECTION ( 'NONE',  ( -0.5364919789714478471, 0.6444004775717705469, -0.5449076811759709926 ) ) ;
#48074=ORIENTED_EDGE ( 'NONE', *, *, #15381, .T. ) ;
#48075=PLANE ( 'NONE',  #15665 ) ;
#48076=DIRECTION ( 'NONE',  ( 0.000000000000000000, -0.000000000000000000, -1.000000000000000000 ) ) ;
#48077=FACE_OUTER_BOUND ( 'NONE', #12300, .T. ) ;
#48078=EDGE_CURVE ( 'NONE', #23836, #3799, #18183, .T. ) ;
#48079=ADVANCED_FACE ( 'NONE', ( #13929 ), #48584, .F. ) ;
#48080=VERTEX_POINT ( 'NONE', #31559 ) ;
#48081=CARTESIAN_POINT ( 'NONE',  ( -12.23851102634202448, -0.1191753592594197858, 11.68427982808754884 ) ) ;
#48082=VERTEX_POINT ( 'NONE', #11891 ) ;
#48083=EDGE_CURVE ( 'NONE', #44937, #13109, #50800, .T. ) ;
#48084=VECTOR ( 'NONE', #2210, 1000.000000000000227 ) ;
#48085=ORIENTED_EDGE ( 'NONE', *, *, #40100, .T. ) ;
#48086=ORIENTED_EDGE ( 'NONE', *, *, #4519, .T. ) ;
#48087=ORIENTED_EDGE ( 'NONE', *, *, #14827, .T. ) ;
#48088=CARTESIAN_POINT ( 'NONE',  ( -27.06630483948590893, -0.1191753592594197858, 7.295098399573937797 ) ) ;
#48089=ORIENTED_EDGE ( 'NONE', *, *, #13934, .T. ) ;
#48090=CARTESIAN_POINT ( 'NONE',  ( -14.16301979303636038, 0.000000000000000000, 7.295511719288459318 ) ) ;
#48091=EDGE_LOOP ( 'NONE', ( #42517, #36064, #53217, #35396 ) ) ;
#48092=DIRECTION ( 'NONE',  ( 0.5449076811759707706, 0.6444004775717708799, -0.5364919789714476250 ) ) ;
#48093=ORIENTED_EDGE ( 'NONE', *, *, #27573, .F. ) ;
#48094=DIRECTION ( 'NONE',  ( -0.005002170337468016433, -0.7660444431189770143, 0.6427681459581293666 ) ) ;
#48095=VERTEX_POINT ( 'NONE', #23842 ) ;
#48096=ADVANCED_FACE ( 'NONE', ( #50543 ), #50241, .F. ) ;
#48097=DIRECTION ( 'NONE',  ( 0.8531650599175529814, -0.4028455766673920135, -0.3313982828793697877 ) ) ;
#48100=DIRECTION ( 'NONE',  ( 0.005961354470445682716, -0.6427876096865404731, -0.7660212471507180654 ) ) ;
#48101=ADVANCED_FACE ( 'NONE', ( #37771 ), #16174, .F. ) ;
#48102=CARTESIAN_POINT ( 'NONE',  ( -19.54735067093493939, 2.562506240245330247, 7.319338878784295233 ) ) ;
#48103=LINE ( 'NONE', #47556, #32873 ) ;
#48104=VERTEX_POINT ( 'NONE', #45697 ) ;
#48105=EDGE_CURVE ( 'NONE', #8726, #43397, #46250, .T. ) ;
#48106=ORIENTED_EDGE ( 'NONE', *, *, #18475, .F. ) ;
#48107=CARTESIAN_POINT ( 'NONE',  ( -19.78481654831908187, 1.743523803501507485, 4.311398836375244237 ) ) ;
#48108=DIRECTION ( 'NONE',  ( 0.5449076811759707706, 0.6444004775717708799, -0.5364919789714476250 ) ) ;
#48109=CARTESIAN_POINT ( 'NONE',  ( -13.45869596940543111, 3.038739411681507185, 7.096224758407104538 ) ) ;
#48110=CARTESIAN_POINT ( 'NONE',  ( -9.036602278258525800, 2.977129085626424754, 3.729226913157295265 ) ) ;
#48111=DIRECTION ( 'NONE',  ( -0.5364919789714478471, 0.6444004775717705469, -0.5449076811759709926 ) ) ;
#48112=LINE ( 'NONE', #26265, #53137 ) ;
#48113=ORIENTED_EDGE ( 'NONE', *, *, #7952, .T. ) ;
#48114=CARTESIAN_POINT ( 'NONE',  ( -21.69200269479475551, 4.010151117816511679, 4.979897425557093804 ) ) ;
#48115=ADVANCED_FACE ( 'NONE', ( #7356 ), #54236, .F. ) ;
#48117=ORIENTED_EDGE ( 'NONE', *, *, #33053, .T. ) ;
#48118=DIRECTION ( 'NONE',  ( -0.7660212471507179544, -0.6427876096865405842, -0.005961354470445141482 ) ) ;
#48119=DIRECTION ( 'NONE',  ( 0.005002170337468016433, -0.7660444431189770143, -0.6427681459581293666 ) ) ;
#48120=VECTOR ( 'NONE', #55950, 1000.000000000000227 ) ;
#48121=DIRECTION ( 'NONE',  ( 0.005961354470445682716, -0.6427876096865404731, -0.7660212471507180654 ) ) ;
#48122=DIRECTION ( 'NONE',  ( 0.005002170337468016433, -0.7660444431189770143, -0.6427681459581293666 ) ) ;
#48123=AXIS2_PLACEMENT_3D ( 'NONE', #38650, #11936, #29577 ) ;
#48124=CARTESIAN_POINT ( 'NONE',  ( -14.35031752825289431, -2.137015261443157232, 5.763288513568061155 ) ) ;
#48125=VERTEX_POINT ( 'NONE', #55085 ) ;
#48126=ORIENTED_EDGE ( 'NONE', *, *, #10414, .F. ) ;
#48127=CARTESIAN_POINT ( 'NONE',  ( -17.46532115785441519, 0.000000000000000000, 13.67492996699914265 ) ) ;
#48128=LINE ( 'NONE', #8396, #41281 ) ;
#48129=FACE_OUTER_BOUND ( 'NONE', #38309, .T. ) ;
#48131=CARTESIAN_POINT ( 'NONE',  ( -11.34933193044230038, 0.000000000000000000, 3.993419860576636005 ) ) ;
#48133=CARTESIAN_POINT ( 'NONE',  ( -23.33693525117809386, 0.000000000000000000, 5.746789908705562944 ) ) ;
#48134=DIRECTION ( 'NONE',  ( -0.9999697198139514409, -0.000000000000000000, -0.007781995580013368816 ) ) ;
#48135=CARTESIAN_POINT ( 'NONE',  ( -24.26908309836554878, 0.000000000000000000, 6.108867788427308376 ) ) ;
#48136=ORIENTED_EDGE ( 'NONE', *, *, #2312, .F. ) ;
#48138=ORIENTED_EDGE ( 'NONE', *, *, #20827, .F. ) ;
#48139=CARTESIAN_POINT ( 'NONE',  ( -12.33850799832341849, 0.000000000000000000, 11.68350162852954632 ) ) ;
#48140=CARTESIAN_POINT ( 'NONE',  ( -10.86325900467495842, 0.000000000000000000, 1.242552090245319540 ) ) ;
#48141=ADVANCED_FACE ( 'NONE', ( #11642 ), #53955, .F. ) ;
#48142=VERTEX_POINT ( 'NONE', #33496 ) ;
#48143=AXIS2_PLACEMENT_3D ( 'NONE', #32935, #49429, #10811 ) ;
#48144=VERTEX_POINT ( 'NONE', #28685 ) ;
#48145=EDGE_CURVE ( 'NONE', #47896, #5013, #23573, .T. ) ;
#48146=ADVANCED_FACE ( 'NONE', ( #28958 ), #2801, .F. ) ;
#48148=VERTEX_POINT ( 'NONE', #1968 ) ;
#48149=EDGE_LOOP ( 'NONE', ( #29940, #24530, #7125, #23659, #45044 ) ) ;
#48150=EDGE_LOOP ( 'NONE', ( #26110, #35624, #39436, #52042 ) ) ;
#48151=DIRECTION ( 'NONE',  ( 0.5449076811759707706, 0.6444004775717708799, -0.5364919789714476250 ) ) ;
#48152=DIRECTION ( 'NONE',  ( 0.000000000000000000, -0.000000000000000000, -1.000000000000000000 ) ) ;
#48153=DIRECTION ( 'NONE',  ( -0.7660212471507179544, -0.6427876096865405842, -0.005961354470445141482 ) ) ;
#48154=VECTOR ( 'NONE', #14193, 1000.000000000000227 ) ;
#48155=ORIENTED_EDGE ( 'NONE', *, *, #47749, .T. ) ;
#48156=CARTESIAN_POINT ( 'NONE',  ( -21.03941874682061197, 4.819660872929009798, 12.96363045103941403 ) ) ;
#48157=ORIENTED_EDGE ( 'NONE', *, *, #11972, .F. ) ;
#48158=ORIENTED_EDGE ( 'NONE', *, *, #14407, .T. ) ;
#48159=VECTOR ( 'NONE', #2168, 1000.000000000000227 ) ;
#48160=LINE ( 'NONE', #30605, #29275 ) ;
#48161=CARTESIAN_POINT ( 'NONE',  ( -10.00813838035478298, 0.000000000000000000, 10.77830692922518452 ) ) ;
#48162=DIRECTION ( 'NONE',  ( 0.007781995580012663651, 0.000000000000000000, -0.9999697198139515519 ) ) ;
#48163=EDGE_LOOP ( 'NONE', ( #26316, #10160, #17628, #22049 ) ) ;
#48164=DIRECTION ( 'NONE',  ( -0.7660212471507179544, -0.6427876096865405842, -0.005961354470445141482 ) ) ;
#48165=ORIENTED_EDGE ( 'NONE', *, *, #46522, .T. ) ;
#48166=DIRECTION ( 'NONE',  ( 0.5449076811759707706, 0.6444004775717708799, -0.5364919789714476250 ) ) ;
#48167=CARTESIAN_POINT ( 'NONE',  ( -14.07383107636587738, -0.1191753592594190225, 8.685127515039473778 ) ) ;
#48169=CARTESIAN_POINT ( 'NONE',  ( -13.73672976910459909, 0.000000000000000000, 12.22661844811216270 ) ) ;
#48170=DIRECTION ( 'NONE',  ( 0.000000000000000000, -1.000000000000000000, 0.000000000000000000 ) ) ;
#48172=EDGE_CURVE ( 'NONE', #33376, #38808, #15069, .T. ) ;
#48173=CARTESIAN_POINT ( 'NONE',  ( -21.47419595591918906, 0.000000000000000000, 5.222628093224860102 ) ) ;
#48174=PLANE ( 'NONE',  #9425 ) ;
#48175=CARTESIAN_POINT ( 'NONE',  ( -13.08486533123210194, 0.000000000000000000, 1.963927175729152541 ) ) ;
#48176=VERTEX_POINT ( 'NONE', #32401 ) ;
#48177=CARTESIAN_POINT ( 'NONE',  ( -24.26986129792355129, -0.1191753592594197858, 6.208864760408702388 ) ) ;
#48178=EDGE_CURVE ( 'NONE', #49806, #36594, #19604, .T. ) ;
#48179=VECTOR ( 'NONE', #33738, 1000.000000000000000 ) ;
#48180=VECTOR ( 'NONE', #34925, 999.9999999999998863 ) ;
#48181=DIRECTION ( 'NONE',  ( 0.007781995580012663651, -3.146120232559066537E-19, -0.9999697198139514409 ) ) ;
#48182=CARTESIAN_POINT ( 'NONE',  ( -19.62219946167430251, -0.1191753592594169547, 5.137037730065149077 ) ) ;
#48183=CARTESIAN_POINT ( 'NONE',  ( -11.20636620717317378, 0.000000000000000000, 11.32298014792380414 ) ) ;
#48184=EDGE_CURVE ( 'NONE', #171, #25528, #46004, .T. ) ;
#48186=LINE ( 'NONE', #53327, #42191 ) ;
#48187=LINE ( 'NONE', #53028, #54037 ) ;
#48188=PLANE ( 'NONE',  #29205 ) ;
#48189=EDGE_LOOP ( 'NONE', ( #50881, #28835, #16433, #20982 ) ) ;
#48190=LINE ( 'NONE', #9298, #51104 ) ;
#48191=FACE_OUTER_BOUND ( 'NONE', #19526, .T. ) ;
#48192=LINE ( 'NONE', #38864, #2786 ) ;
#48194=FACE_OUTER_BOUND ( 'NONE', #36150, .T. ) ;
#48195=DIRECTION ( 'NONE',  ( 0.5364919789714477361, 0.6444004775717706579, 0.5449076811759711036 ) ) ;
#48196=ADVANCED_FACE ( 'NONE', ( #15334 ), #32650, .F. ) ;
#48197=CARTESIAN_POINT ( 'NONE',  ( -14.56888064431065821, -0.1191753592594197858, 12.58947452739191064 ) ) ;
#48198=AXIS2_PLACEMENT_3D ( 'NONE', #17582, #52234, #34919 ) ;
#48199=CARTESIAN_POINT ( 'NONE',  ( -29.93654370153088706, -1.000000000000000000, 22.35628214185738116 ) ) ;
#48200=DIRECTION ( 'NONE',  ( 0.007781995580012663651, -3.146120232559066537E-19, -0.9999697198139514409 ) ) ;
#48201=ADVANCED_FACE ( 'NONE', ( #54781 ), #7110, .F. ) ;
#48203=EDGE_CURVE ( 'NONE', #30292, #33948, #9557, .T. ) ;
#48204=EDGE_CURVE ( 'NONE', #18526, #22565, #46844, .T. ) ;
#48205=ORIENTED_EDGE ( 'NONE', *, *, #29223, .F. ) ;
#48206=ORIENTED_EDGE ( 'NONE', *, *, #9500, .F. ) ;
#48207=ORIENTED_EDGE ( 'NONE', *, *, #54672, .F. ) ;
#48208=ORIENTED_EDGE ( 'NONE', *, *, #16068, .F. ) ;
#48209=PLANE ( 'NONE',  #28707 ) ;
#48210=CARTESIAN_POINT ( 'NONE',  ( -11.62702749645772826, 0.000000000000000000, 5.668593104918477898 ) ) ;
#48211=EDGE_CURVE ( 'NONE', #52307, #21963, #16728, .T. ) ;
#48212=VECTOR ( 'NONE', #25438, 1000.000000000000227 ) ;
#48213=AXIS2_PLACEMENT_3D ( 'NONE', #33325, #24778, #38118 ) ;
#48214=ORIENTED_EDGE ( 'NONE', *, *, #22789, .F. ) ;
#48215=ORIENTED_EDGE ( 'NONE', *, *, #35787, .F. ) ;
#48216=EDGE_CURVE ( 'NONE', #2943, #3628, #31118, .T. ) ;
#48217=AXIS2_PLACEMENT_3D ( 'NONE', #45256, #14041, #31911 ) ;
#48218=CARTESIAN_POINT ( 'NONE',  ( -16.37261523729198132, -0.1191753592594188005, 5.531658815698983211 ) ) ;
#48219=VERTEX_POINT ( 'NONE', #43147 ) ;
#48220=PLANE ( 'NONE',  #25508 ) ;
#48221=LINE ( 'NONE', #811, #55861 ) ;
#48222=ORIENTED_EDGE ( 'NONE', *, *, #38197, .T. ) ;
#48223=DIRECTION ( 'NONE',  ( 0.6246952433987894571, -0.7422098413412800966, -0.2426528472758541777 ) ) ;
#48224=ORIENTED_EDGE ( 'NONE', *, *, #35979, .F. ) ;
#48225=FACE_OUTER_BOUND ( 'NONE', #12110, .T. ) ;
#48226=VECTOR ( 'NONE', #6703, 999.9999999999998863 ) ;
#48228=AXIS2_PLACEMENT_3D ( 'NONE', #40142, #23115, #45246 ) ;
#48229=CARTESIAN_POINT ( 'NONE',  ( -17.26532721389163072, 0.000000000000000000, 13.67648636611514590 ) ) ;
#48230=CARTESIAN_POINT ( 'NONE',  ( -31.72626587586518099, 0.000000000000000000, 9.005490826201270949 ) ) ;
#48231=ORIENTED_EDGE ( 'NONE', *, *, #13526, .T. ) ;
#48232=DIRECTION ( 'NONE',  ( -0.005002170337468016433, -0.7660444431189770143, 0.6427681459581293666 ) ) ;
#48233=PLANE ( 'NONE',  #21121 ) ;
#48234=CARTESIAN_POINT ( 'NONE',  ( -8.935550834329328396, -0.1191753592594181482, 5.220203700729370233 ) ) ;
#48235=ORIENTED_EDGE ( 'NONE', *, *, #34843, .F. ) ;
#48236=DIRECTION ( 'NONE',  ( -0.5364919789714478471, 0.6444004775717705469, -0.5449076811759709926 ) ) ;
#48237=ORIENTED_EDGE ( 'NONE', *, *, #21775, .F. ) ;
#48238=DIRECTION ( 'NONE',  ( -0.9999697198139514409, -0.000000000000000000, -0.007781995580013368816 ) ) ;
#48239=CARTESIAN_POINT ( 'NONE',  ( -17.92052085394417205, 1.743523803501506375, 3.587243076931753816 ) ) ;
#48240=CARTESIAN_POINT ( 'NONE',  ( -16.73515930820439124, 0.000000000000000000, 5.259508372212608585 ) ) ;
#48241=CARTESIAN_POINT ( 'NONE',  ( -11.67244013076689946, 0.000000000000000000, 11.50401908778467863 ) ) ;
#48242=ADVANCED_FACE ( 'NONE', ( #25265 ), #18330, .F. ) ;
#48243=DIRECTION ( 'NONE',  ( -0.6427681459581293666, -0.7660444431189770143, -0.005002170337467561935 ) ) ;
#48244=LINE ( 'NONE', #9359, #15921 ) ;
#48245=LINE ( 'NONE', #43707, #16166 ) ;
#48246=PLANE ( 'NONE',  #31126 ) ;
#48247=SURFACE_STYLE_USAGE ( .BOTH. , #32076 ) ;
#48248=DIRECTION ( 'NONE',  ( -0.5364919789714478471, 0.6444004775717705469, -0.5449076811759709926 ) ) ;
#48249=ORIENTED_EDGE ( 'NONE', *, *, #31704, .T. ) ;
#48250=VECTOR ( 'NONE', #42272, 999.9999999999998863 ) ;
#48251=CARTESIAN_POINT ( 'NONE',  ( -6.903226477722774312, 6.739079746892438827, 5.899821174169304960 ) ) ;
#48252=DIRECTION ( 'NONE',  ( 0.7660212471507180654, -0.6427876096865404731, 0.005961354470445141482 ) ) ;
#48253=CARTESIAN_POINT ( 'NONE',  ( -14.86798956032420094, 0.000000000000000000, 4.166042909511353365 ) ) ;
#48254=ADVANCED_FACE ( 'NONE', ( #35671 ), #14101, .F. ) ;
#48256=VECTOR ( 'NONE', #14201, 1000.000000000000227 ) ;
#48257=CARTESIAN_POINT ( 'NONE',  ( -24.26908309836554878, 0.000000000000000000, 6.108867788427308376 ) ) ;
#48259=CARTESIAN_POINT ( 'NONE',  ( -16.00300540497972790, 0.000000000000000000, 4.895874093374860792 ) ) ;
#48260=ADVANCED_FACE ( 'NONE', ( #7953 ), #29809, .F. ) ;
#48261=DIRECTION ( 'NONE',  ( 0.007781995580012663651, -3.146120232559066537E-19, -0.9999697198139514409 ) ) ;
#48262=ORIENTED_EDGE ( 'NONE', *, *, #34804, .T. ) ;
#48263=VECTOR ( 'NONE', #13027, 999.9999999999998863 ) ;
#48264=VECTOR ( 'NONE', #28717, 1000.000000000000227 ) ;
#48265=EDGE_LOOP ( 'NONE', ( #11695, #22477, #40945, #52366 ) ) ;
#48266=DIRECTION ( 'NONE',  ( -0.6427681459581293666, -0.7660444431189770143, -0.005002170337467561935 ) ) ;
#48267=DIRECTION ( 'NONE',  ( -0.7660212471507179544, -0.6427876096865405842, -0.005961354470445141482 ) ) ;
#48268=ORIENTED_EDGE ( 'NONE', *, *, #22829, .T. ) ;
#48269=ADVANCED_FACE ( 'NONE', ( #3661 ), #29529, .F. ) ;
#48270=DIRECTION ( 'NONE',  ( 0.007781995580012662783, 0.000000000000000000, -0.9999697198139514409 ) ) ;
#48272=ORIENTED_EDGE ( 'NONE', *, *, #30978, .T. ) ;
#48274=EDGE_CURVE ( 'NONE', #42565, #30246, #44203, .T. ) ;
#48275=ORIENTED_EDGE ( 'NONE', *, *, #20528, .F. ) ;
#48276=VERTEX_POINT ( 'NONE', #24981 ) ;
#48277=ORIENTED_EDGE ( 'NONE', *, *, #22692, .F. ) ;
#48278=LINE ( 'NONE', #52551, #18441 ) ;
#48279=LINE ( 'NONE', #44039, #51373 ) ;
#48280=DIRECTION ( 'NONE',  ( 0.000000000000000000, -1.000000000000000000, 0.000000000000000000 ) ) ;
#48281=EDGE_CURVE ( 'NONE', #47104, #40951, #42303, .T. ) ;
#48282=DIRECTION ( 'NONE',  ( -0.005002170337468016433, -0.7660444431189770143, 0.6427681459581293666 ) ) ;
#48283=EDGE_LOOP ( 'NONE', ( #46911, #46743, #32452, #52249 ) ) ;
#48285=AXIS2_PLACEMENT_3D ( 'NONE', #18894, #4983, #49250 ) ;
#48286=EDGE_CURVE ( 'NONE', #47084, #17177, #8209, .T. ) ;
#48287=DIRECTION ( 'NONE',  ( -0.5449076811759708816, 0.6444004775717707689, 0.5364919789714475140 ) ) ;
#48288=ORIENTED_EDGE ( 'NONE', *, *, #44980, .T. ) ;
#48289=VECTOR ( 'NONE', #6665, 1000.000000000000227 ) ;
#48290=FACE_OUTER_BOUND ( 'NONE', #45720, .T. ) ;
#48291=ORIENTED_EDGE ( 'NONE', *, *, #22220, .F. ) ;
#48292=PLANE ( 'NONE',  #34211 ) ;
#48293=PLANE ( 'NONE',  #33988 ) ;
#48294=VECTOR ( 'NONE', #23761, 1000.000000000000114 ) ;
#48295=AXIS2_PLACEMENT_3D ( 'NONE', #46420, #37099, #20624 ) ;
#48296=ORIENTED_EDGE ( 'NONE', *, *, #10222, .F. ) ;
#48297=LINE ( 'NONE', #55714, #13213 ) ;
#48298=EDGE_LOOP ( 'NONE', ( #30853, #2613, #9113, #34907 ) ) ;
#48299=VECTOR ( 'NONE', #36995, 1000.000000000000227 ) ;
#48300=DIRECTION ( 'NONE',  ( -0.5364919789714478471, 0.6444004775717705469, -0.5449076811759709926 ) ) ;
#48301=VECTOR ( 'NONE', #27517, 999.9999999999998863 ) ;
#48302=ORIENTED_EDGE ( 'NONE', *, *, #10545, .F. ) ;
#48303=CARTESIAN_POINT ( 'NONE',  ( -9.987828218865807628, 0.6049996566053985614, 1.280352617363947898 ) ) ;
#48304=CARTESIAN_POINT ( 'NONE',  ( -19.06334656290779250, 0.000000000000000000, 8.565378508916090539 ) ) ;
#48305=CARTESIAN_POINT ( 'NONE',  ( -18.76354595665420177, -0.1191753592594177458, 14.21882498613976331 ) ) ;
#48307=CARTESIAN_POINT ( 'NONE',  ( -19.72429228760297448, 0.000000000000000000, 5.405572261783524013 ) ) ;
#48308=DIRECTION ( 'NONE',  ( -0.7660212471507179544, -0.6427876096865405842, -0.005961354470445141482 ) ) ;
#48309=DIRECTION ( 'NONE',  ( 0.5364919789714477361, 0.6444004775717706579, 0.5449076811759711036 ) ) ;
#48310=VECTOR ( 'NONE', #51031, 999.9999999999998863 ) ;
#48311=EDGE_CURVE ( 'NONE', #19751, #27927, #4256, .T. ) ;
#48313=VECTOR ( 'NONE', #47899, 1000.000000000000114 ) ;
#48314=DIRECTION ( 'NONE',  ( 0.5364919789714477361, 0.6444004775717706579, 0.5449076811759711036 ) ) ;
#48315=PLANE ( 'NONE',  #50585 ) ;
#48316=CARTESIAN_POINT ( 'NONE',  ( -13.28410798335889176, 1.743523803501505709, 4.902739383989964672 ) ) ;
#48317=ORIENTED_EDGE ( 'NONE', *, *, #52128, .T. ) ;
#48318=DIRECTION ( 'NONE',  ( 0.005002170337468016433, -0.7660444431189770143, -0.6427681459581293666 ) ) ;
#48319=PLANE ( 'NONE',  #9589 ) ;
#48320=FACE_OUTER_BOUND ( 'NONE', #37306, .T. ) ;
#48321=EDGE_LOOP ( 'NONE', ( #21569, #52972, #34842, #37100 ) ) ;
#48322=LINE ( 'NONE', #43786, #267 ) ;
#48323=CARTESIAN_POINT ( 'NONE',  ( -15.96710241509184058, -0.1191753592594218814, 13.13259134697452879 ) ) ;
#48324=EDGE_LOOP ( 'NONE', ( #15301, #5588, #18642, #30085 ) ) ;
#48325=EDGE_CURVE ( 'NONE', #24915, #1847, #20718, .T. ) ;
#48326=VECTOR ( 'NONE', #33859, 1000.000000000000227 ) ;
#48327=ADVANCED_FACE ( 'NONE', ( #51077 ), #55927, .F. ) ;
#48328=EDGE_CURVE ( 'NONE', #8596, #8862, #38886, .T. ) ;
#48329=CARTESIAN_POINT ( 'NONE',  ( -10.94028622754223967, 0.000000000000000000, 11.14038480894692995 ) ) ;
#48330=CARTESIAN_POINT ( 'NONE',  ( -14.39030005034598148, 0.000000000000000000, 2.492426064285516940 ) ) ;
#48331=AXIS2_PLACEMENT_3D ( 'NONE', #40933, #49176, #23365 ) ;
#48332=DIRECTION ( 'NONE',  ( 0.007781995580012663651, -3.146120232559066537E-19, -0.9999697198139514409 ) ) ;
#48333=EDGE_CURVE ( 'NONE', #29115, #5375, #35387, .T. ) ;
#48334=CARTESIAN_POINT ( 'NONE',  ( -9.305160666641581813, 0.000000000000000000, 5.855988423053500647 ) ) ;
#48336=VERTEX_POINT ( 'NONE', #31965 ) ;
#48337=CARTESIAN_POINT ( 'NONE',  ( -18.92731312331513038, -2.622721114510660367, 4.149653773530951106 ) ) ;
#48338=CARTESIAN_POINT ( 'NONE',  ( -17.69892174394995621, 0.000000000000000000, 9.683992987769761029 ) ) ;
#48339=VECTOR ( 'NONE', #12810, 1000.000000000000114 ) ;
#48340=LINE ( 'NONE', #10011, #31423 ) ;
#48341=AXIS2_PLACEMENT_3D ( 'NONE', #7606, #15024, #45658 ) ;
#48342=FACE_OUTER_BOUND ( 'NONE', #44593, .T. ) ;
#48343=AXIS2_PLACEMENT_3D ( 'NONE', #45006, #53504, #27375 ) ;
#48344=LINE ( 'NONE', #9456, #54565 ) ;
#48345=ADVANCED_FACE ( 'NONE', ( #45306 ), #22879, .F. ) ;
#48346=CARTESIAN_POINT ( 'NONE',  ( -17.68455147642353964, 0.000000000000000000, 7.837444471480940145 ) ) ;
#48347=ORIENTED_EDGE ( 'NONE', *, *, #7894, .T. ) ;
#48348=CARTESIAN_POINT ( 'NONE',  ( -14.09507759759798340, -4.565544526780662693, 9.649774915774109729 ) ) ;
#48349=ADVANCED_FACE ( 'NONE', ( #36497 ), #6406, .F. ) ;
#48350=VECTOR ( 'NONE', #55402, 1000.000000000000000 ) ;
#48352=VECTOR ( 'NONE', #6309, 1000.000000000000227 ) ;
#48353=ORIENTED_EDGE ( 'NONE', *, *, #4675, .T. ) ;
#48354=ADVANCED_FACE ( 'NONE', ( #15219 ), #53815, .F. ) ;
#48355=CARTESIAN_POINT ( 'NONE',  ( -19.45503627000849889, -1.000000000000000000, 7.556996783084074742 ) ) ;
#48356=PLANE ( 'NONE',  #17773 ) ;
#48357=CARTESIAN_POINT ( 'NONE',  ( -14.02843573335194094, -0.1134144341941982215, 2.230747270852929454 ) ) ;
#48359=EDGE_CURVE ( 'NONE', #54876, #12832, #23709, .T. ) ;
#48360=CARTESIAN_POINT ( 'NONE',  ( -23.33849165029409889, 0.000000000000000000, 5.946783852668351855 ) ) ;
#48361=ORIENTED_EDGE ( 'NONE', *, *, #36430, .T. ) ;
#48362=VECTOR ( 'NONE', #46699, 1000.000000000000000 ) ;
#48363=ORIENTED_EDGE ( 'NONE', *, *, #39715, .T. ) ;
#48364=ORIENTED_EDGE ( 'NONE', *, *, #16073, .F. ) ;
#48365=VERTEX_POINT ( 'NONE', #49003 ) ;
#48366=CARTESIAN_POINT ( 'NONE',  ( -11.82127333340995179, 0.000000000000000000, 4.928417299286945052 ) ) ;
#48367=ORIENTED_EDGE ( 'NONE', *, *, #16603, .T. ) ;
#48368=AXIS2_PLACEMENT_3D ( 'NONE', #10182, #40843, #28330 ) ;
#48369=CARTESIAN_POINT ( 'NONE',  ( -10.30072098979975692, -0.1191753592594199940, 1.516258932847700303 ) ) ;
#48371=ORIENTED_EDGE ( 'NONE', *, *, #53363, .F. ) ;
#48372=DIRECTION ( 'NONE',  ( -0.5364919789714478471, 0.6444004775717705469, -0.5449076811759709926 ) ) ;
#48373=ORIENTED_EDGE ( 'NONE', *, *, #51519, .F. ) ;
#48374=DIRECTION ( 'NONE',  ( 0.007781995580012663651, 0.000000000000000000, -0.9999697198139515519 ) ) ;
#48375=VECTOR ( 'NONE', #35570, 1000.000000000000000 ) ;
#48376=ORIENTED_EDGE ( 'NONE', *, *, #11932, .T. ) ;
#48377=FACE_OUTER_BOUND ( 'NONE', #23934, .T. ) ;
#48378=LINE ( 'NONE', #9492, #32044 ) ;
#48379=DIRECTION ( 'NONE',  ( 0.9999697198139515519, 0.000000000000000000, 0.007781995580013368816 ) ) ;
#48380=CARTESIAN_POINT ( 'NONE',  ( -11.75806593121445864, -0.1941918491731561003, 1.567865752637991994 ) ) ;
#48381=FACE_OUTER_BOUND ( 'NONE', #6569, .T. ) ;
#48382=AXIS2_PLACEMENT_3D ( 'NONE', #33073, #7232, #54938 ) ;
#48383=DIRECTION ( 'NONE',  ( -0.7660212471507179544, -0.6427876096865405842, -0.005961354470445141482 ) ) ;
#48384=ORIENTED_EDGE ( 'NONE', *, *, #33563, .F. ) ;
#48385=EDGE_CURVE ( 'NONE', #22163, #31339, #49836, .T. ) ;
#48387=AXIS2_PLACEMENT_3D ( 'NONE', #11321, #24111, #7929 ) ;
#48388=EDGE_LOOP ( 'NONE', ( #43901, #28133, #1770, #50165 ) ) ;
#48389=CARTESIAN_POINT ( 'NONE',  ( -12.13851405436063047, 0.000000000000000000, 11.68505802764555135 ) ) ;
#48390=CARTESIAN_POINT ( 'NONE',  ( -18.19747506107908563, 0.000000000000000000, 14.03856424583689311 ) ) ;
#48392=LINE ( 'NONE', #1548, #38765 ) ;
#48393=VECTOR ( 'NONE', #10395, 999.9999999999998863 ) ;
#48394=VECTOR ( 'NONE', #33470, 999.9999999999998863 ) ;
#48395=CARTESIAN_POINT ( 'NONE',  ( -20.54126990917373519, -0.1191753592594197858, 4.760553241521720658 ) ) ;
#48396=ORIENTED_EDGE ( 'NONE', *, *, #11109, .T. ) ;
#48397=LINE ( 'NONE', #53766, #46695 ) ;
#48398=LINE ( 'NONE', #39329, #11411 ) ;
#48400=DIRECTION ( 'NONE',  ( 0.9999697198139515519, 0.000000000000000000, 0.007781995580013368816 ) ) ;
#48401=LINE ( 'NONE', #1255, #6794 ) ;
#48402=ORIENTED_EDGE ( 'NONE', *, *, #14449, .T. ) ;
#48403=EDGE_CURVE ( 'NONE', #12574, #26765, #49582, .T. ) ;
#48404=ADVANCED_FACE ( 'NONE', ( #45047 ), #48744, .F. ) ;
#48405=EDGE_CURVE ( 'NONE', #8121, #17210, #27149, .T. ) ;
#48406=CARTESIAN_POINT ( 'NONE',  ( -18.67619601524082285, 0.000000000000000000, 3.936400510096834893 ) ) ;
#48407=LINE ( 'NONE', #22006, #13339 ) ;
#48408=LINE ( 'NONE', #18296, #40470 ) ;
#48409=EDGE_CURVE ( 'NONE', #36728, #1702, #18633, .T. ) ;
#48410=CARTESIAN_POINT ( 'NONE',  ( -12.28878428375632303, 0.000000000000000000, 5.294111090776699058 ) ) ;
#48411=CARTESIAN_POINT ( 'NONE',  ( -27.06708303904391144, 0.000000000000000000, 7.395095371555332697 ) ) ;
#48412=ORIENTED_EDGE ( 'NONE', *, *, #50958, .F. ) ;
#48413=AXIS2_PLACEMENT_3D ( 'NONE', #7739, #54307, #15403 ) ;
#48414=ORIENTED_EDGE ( 'NONE', *, *, #4088, .T. ) ;
#48415=LINE ( 'NONE', #9532, #32113 ) ;
#48417=CARTESIAN_POINT ( 'NONE',  ( -12.93729377823301618, -3.756034771668160577, 7.871508942076431481 ) ) ;
#48418=VECTOR ( 'NONE', #31375, 1000.000000000000000 ) ;
#48419=DIRECTION ( 'NONE',  ( 0.5364919789714477361, 0.6444004775717706579, 0.5449076811759711036 ) ) ;
#48420=PLANE ( 'NONE',  #30372 ) ;
#48421=VECTOR ( 'NONE', #20985, 1000.000000000000227 ) ;
#48422=ORIENTED_EDGE ( 'NONE', *, *, #28039, .F. ) ;
#48423=FACE_OUTER_BOUND ( 'NONE', #15117, .T. ) ;
#48424=DIRECTION ( 'NONE',  ( 0.007781995580012663651, 0.000000000000000000, -0.9999697198139515519 ) ) ;
#48425=EDGE_CURVE ( 'NONE', #37378, #43993, #23180, .T. ) ;
#48426=FACE_OUTER_BOUND ( 'NONE', #22852, .T. ) ;
#48427=CARTESIAN_POINT ( 'NONE',  ( -23.33693525117809386, 0.000000000000000000, 5.746789908705562944 ) ) ;
#48428=EDGE_CURVE ( 'NONE', #28121, #17110, #17692, .T. ) ;
#48429=VECTOR ( 'NONE', #3725, 1000.000000000000227 ) ;
#48430=ORIENTED_EDGE ( 'NONE', *, *, #7998, .F. ) ;
#48431=DIRECTION ( 'NONE',  ( 0.005002170337468016433, -0.7660444431189770143, -0.6427681459581293666 ) ) ;
#48432=ORIENTED_EDGE ( 'NONE', *, *, #9650, .T. ) ;
#48433=FACE_OUTER_BOUND ( 'NONE', #11853, .T. ) ;
#48434=CARTESIAN_POINT ( 'NONE',  ( -11.40636015113596180, 0.000000000000000000, 11.32142374880780089 ) ) ;
#48435=VECTOR ( 'NONE', #33516, 999.9999999999998863 ) ;
#48436=EDGE_LOOP ( 'NONE', ( #19697, #28291, #55632, #44912 ) ) ;
#48437=EDGE_CURVE ( 'NONE', #8206, #52695, #39566, .T. ) ;
#48438=CARTESIAN_POINT ( 'NONE',  ( -14.46888367232926420, 0.000000000000000000, 12.59025272694991315 ) ) ;
#48439=ORIENTED_EDGE ( 'NONE', *, *, #38161, .F. ) ;
#48440=EDGE_CURVE ( 'NONE', #32882, #43375, #52872, .T. ) ;
#48441=VECTOR ( 'NONE', #51831, 999.9999999999998863 ) ;
#48442=ORIENTED_EDGE ( 'NONE', *, *, #36318, .F. ) ;
#48443=ORIENTED_EDGE ( 'NONE', *, *, #25329, .T. ) ;
#48444=CARTESIAN_POINT ( 'NONE',  ( -14.94916102560700821, 0.000000000000000000, 2.688082935172642962 ) ) ;
#48445=VECTOR ( 'NONE', #4156, 999.9999999999998863 ) ;
#48446=VERTEX_POINT ( 'NONE', #26214 ) ;
#48447=ORIENTED_EDGE ( 'NONE', *, *, #16651, .T. ) ;
#48448=CARTESIAN_POINT ( 'NONE',  ( -12.77485720952366677, 0.000000000000000000, 8.044978861108015522 ) ) ;
#48449=CARTESIAN_POINT ( 'NONE',  ( 2.072287782118878319, 0.000000000000000000, -2.950529333540147015 ) ) ;
#48450=ORIENTED_EDGE ( 'NONE', *, *, #31484, .F. ) ;
#48451=EDGE_LOOP ( 'NONE', ( #9254, #55688, #40982, #12829 ) ) ;
#48452=CARTESIAN_POINT ( 'NONE',  ( -12.74899072797612476, 0.000000000000000000, 4.721191531788137219 ) ) ;
#48453=EDGE_LOOP ( 'NONE', ( #54126, #18876, #56065, #4787 ) ) ;
#48454=EDGE_LOOP ( 'NONE', ( #3017, #35449, #13121, #12657 ) ) ;
#48455=VECTOR ( 'NONE', #27875, 999.9999999999998863 ) ;
#48456=LINE ( 'NONE', #27427, #43788 ) ;
#48457=PLANE ( 'NONE',  #12170 ) ;
#48459=DIRECTION ( 'NONE',  ( 0.007781995580012663651, -3.146120232559066537E-19, -0.9999697198139514409 ) ) ;
#48460=ORIENTED_EDGE ( 'NONE', *, *, #49458, .T. ) ;
#48461=LINE ( 'NONE', #31448, #38267 ) ;
#48462=VECTOR ( 'NONE', #55173, 1000.000000000000000 ) ;
#48463=ORIENTED_EDGE ( 'NONE', *, *, #27869, .F. ) ;
#48464=LINE ( 'NONE', #18662, #39346 ) ;
#48465=DIRECTION ( 'NONE',  ( 0.9999697198139515519, 0.000000000000000000, 0.007781995580013368816 ) ) ;
#48466=AXIS2_PLACEMENT_3D ( 'NONE', #30252, #43573, #47859 ) ;
#48467=CARTESIAN_POINT ( 'NONE',  ( -14.01701317841955508, 0.000000000000000000, 2.326005055450897085 ) ) ;
#48468=DIRECTION ( 'NONE',  ( 0.005002170337468016433, -0.7660444431189770143, -0.6427681459581293666 ) ) ;
#48470=DIRECTION ( 'NONE',  ( 0.9999697198139515519, 0.000000000000000000, 0.007781995580013368816 ) ) ;
#48471=AXIS2_PLACEMENT_3D ( 'NONE', #46190, #24343, #42510 ) ;
#48472=CARTESIAN_POINT ( 'NONE',  ( -17.83139810946674686, -0.1191753592594197858, 13.85674710641801788 ) ) ;
#48473=ORIENTED_EDGE ( 'NONE', *, *, #49174, .F. ) ;
#48474=DIRECTION ( 'NONE',  ( -0.2426528472758541499, 0.7422098413412800966, -0.6246952433987894571 ) ) ;
#48476=ADVANCED_FACE ( 'NONE', ( #27055 ), #40098, .F. ) ;
#48478=CARTESIAN_POINT ( 'NONE',  ( -17.83139810946674686, -0.1191753592594197858, 13.85674710641801788 ) ) ;
#48479=CARTESIAN_POINT ( 'NONE',  ( -8.409922665610809034, 0.000000000000000000, 10.23674650875856962 ) ) ;
#48481=CARTESIAN_POINT ( 'NONE',  ( -13.24528089218730287, 4.495856970884011261, 1.683407265882337134 ) ) ;
#48482=EDGE_CURVE ( 'NONE', #54373, #5690, #18519, .T. ) ;
#48483=EDGE_CURVE ( 'NONE', #7363, #47810, #8913, .T. ) ;
#48484=FACE_OUTER_BOUND ( 'NONE', #33691, .T. ) ;
#48485=AXIS2_PLACEMENT_3D ( 'NONE', #43534, #44106, #9174 ) ;
#48487=VECTOR ( 'NONE', #17698, 999.9999999999998863 ) ;
#48488=VERTEX_POINT ( 'NONE', #35032 ) ;
#48489=CARTESIAN_POINT ( 'NONE',  ( -11.50051463717167621, 0.000000000000000000, 7.685564019862313856 ) ) ;
#48490=CARTESIAN_POINT ( 'NONE',  ( -10.41011832185500019, 0.000000000000000000, 2.723406815044388196 ) ) ;
#48491=PLANE ( 'NONE',  #9178 ) ;
#48492=CARTESIAN_POINT ( 'NONE',  ( -19.52585474275619148, 0.000000000000000000, 5.607122604862315285 ) ) ;
#48493=CARTESIAN_POINT ( 'NONE',  ( -17.74482636761137044, -0.1191753592594197858, 3.674319602356483916 ) ) ;
#48495=CARTESIAN_POINT ( 'NONE',  ( -17.37239704199277313, -2.946525016555660237, 8.265710246709229381 ) ) ;
#48496=AXIS2_PLACEMENT_3D ( 'NONE', #9885, #512, #22394 ) ;
#48497=DIRECTION ( 'NONE',  ( 0.007781995580012663651, 0.000000000000000000, -0.9999697198139515519 ) ) ;
#48498=VECTOR ( 'NONE', #27851, 1000.000000000000000 ) ;
#48499=DIRECTION ( 'NONE',  ( 0.5364919789714477361, 0.6444004775717706579, 0.5449076811759711036 ) ) ;
#48500=VECTOR ( 'NONE', #28414, 999.9999999999998863 ) ;
#48501=VERTEX_POINT ( 'NONE', #14294 ) ;
#48502=AXIS2_PLACEMENT_3D ( 'NONE', #42327, #7974, #33785 ) ;
#48503=EDGE_CURVE ( 'NONE', #33244, #52569, #22779, .T. ) ;
#48504=ORIENTED_EDGE ( 'NONE', *, *, #21705, .F. ) ;
#48505=VERTEX_POINT ( 'NONE', #30489 ) ;
#48506=AXIS2_PLACEMENT_3D ( 'NONE', #53743, #32188, #23645 ) ;
#48507=VECTOR ( 'NONE', #16850, 999.9999999999998863 ) ;
#48508=ORIENTED_EDGE ( 'NONE', *, *, #52903, .F. ) ;
#48509=EDGE_CURVE ( 'NONE', #1256, #38849, #13444, .T. ) ;
#48510=VECTOR ( 'NONE', #53643, 1000.000000000000227 ) ;
#48511=AXIS2_PLACEMENT_3D ( 'NONE', #49286, #15669, #5861 ) ;
#48513=CARTESIAN_POINT ( 'NONE',  ( -16.74797317661480278, 0.000000000000000000, 6.906062944538641446 ) ) ;
#48514=ADVANCED_FACE ( 'NONE', ( #17977 ), #5209, .F. ) ;
#48515=LINE ( 'NONE', #18123, #50285 ) ;
#48516=AXIS2_PLACEMENT_3D ( 'NONE', #3132, #46570, #7688 ) ;
#48517=ORIENTED_EDGE ( 'NONE', *, *, #30691, .F. ) ;
#48519=EDGE_CURVE ( 'NONE', #42240, #693, #21934, .T. ) ;
#48520=AXIS2_PLACEMENT_3D ( 'NONE', #44314, #5416, #22727 ) ;
#48523=ORIENTED_EDGE ( 'NONE', *, *, #39212, .F. ) ;
#48524=DIRECTION ( 'NONE',  ( 0.7660212471507180654, -0.6427876096865404731, 0.005961354470445141482 ) ) ;
#48525=CARTESIAN_POINT ( 'NONE',  ( -21.47263955680318404, 0.000000000000000000, 5.022634149262071190 ) ) ;
#48526=ORIENTED_EDGE ( 'NONE', *, *, #3032, .F. ) ;
#48527=CARTESIAN_POINT ( 'NONE',  ( -24.27063949748155380, 0.000000000000000000, 6.308861732390097288 ) ) ;
#48528=ORIENTED_EDGE ( 'NONE', *, *, #2244, .T. ) ;
#48529=CARTESIAN_POINT ( 'NONE',  ( -27.06630483948590893, -0.1191753592594197858, 7.295098399573937797 ) ) ;
#48530=CARTESIAN_POINT ( 'NONE',  ( -9.964043400434892561, 0.000000000000000000, 5.112196705653958340 ) ) ;
#48531=VECTOR ( 'NONE', #20637, 1000.000000000000227 ) ;
#48532=LINE ( 'NONE', #40591, #10985 ) ;
#48533=LINE ( 'NONE', #5948, #4272 ) ;
#48534=ORIENTED_EDGE ( 'NONE', *, *, #8873, .F. ) ;
#48535=DIRECTION ( 'NONE',  ( 0.9999697198139515519, 0.000000000000000000, 0.007781995580013368816 ) ) ;
#48537=CARTESIAN_POINT ( 'NONE',  ( -17.26532721389163072, 0.000000000000000000, 13.67648636611514590 ) ) ;
#48538=VECTOR ( 'NONE', #29455, 1000.000000000000227 ) ;
#48539=ORIENTED_EDGE ( 'NONE', *, *, #2086, .F. ) ;
#48540=CARTESIAN_POINT ( 'NONE',  ( -14.06092696710768664, -0.1191753592594177180, 7.026977187570086159 ) ) ;
#48541=EDGE_CURVE ( 'NONE', #41332, #18331, #31311, .T. ) ;
#48542=EDGE_LOOP ( 'NONE', ( #25600, #26707, #13, #22891 ) ) ;
#48544=EDGE_CURVE ( 'NONE', #27953, #2695, #58, .T. ) ;
#48545=FACE_OUTER_BOUND ( 'NONE', #25836, .T. ) ;
#48546=CARTESIAN_POINT ( 'NONE',  ( -16.56142742775368149, 0.1245042932765021287, 3.518674714925085212 ) ) ;
#48547=CARTESIAN_POINT ( 'NONE',  ( -16.83437808062778629, -0.1191753592594196748, 5.158733200673210284 ) ) ;
#48548=FACE_OUTER_BOUND ( 'NONE', #11676, .T. ) ;
#48549=VECTOR ( 'NONE', #34560, 999.9999999999998863 ) ;
#48550=DIRECTION ( 'NONE',  ( 0.007781995580012662783, 0.000000000000000000, -0.9999697198139514409 ) ) ;
#48551=FACE_OUTER_BOUND ( 'NONE', #36377, .T. ) ;
#48552=ADVANCED_FACE ( 'NONE', ( #35560 ), #4909, .F. ) ;
#48553=CARTESIAN_POINT ( 'NONE',  ( 1.086233639165236964, 0.000000000000000000, 2.796443541562362078 ) ) ;
#48554=LINE ( 'NONE', #1402, #36559 ) ;
#48555=VECTOR ( 'NONE', #25917, 1000.000000000000227 ) ;
#48556=VECTOR ( 'NONE', #12787, 999.9999999999998863 ) ;
#48557=CARTESIAN_POINT ( 'NONE',  ( -14.46888367232926420, 0.000000000000000000, 12.59025272694991315 ) ) ;
#48558=EDGE_LOOP ( 'NONE', ( #7571, #27966, #52003, #24692 ) ) ;
#48559=LINE ( 'NONE', #36331, #30251 ) ;
#48560=CARTESIAN_POINT ( 'NONE',  ( 2.072287782118878319, 0.000000000000000000, -2.950529333540147015 ) ) ;
#48561=CARTESIAN_POINT ( 'NONE',  ( -17.89161118178617826, 0.000000000000000000, 8.743823238175442825 ) ) ;
#48562=CARTESIAN_POINT ( 'NONE',  ( -5.750715776775079391, -5.518302702908891355, -0.9846002728345305544 ) ) ;
#48563=AXIS2_PLACEMENT_3D ( 'NONE', #2994, #23491, #36274 ) ;
#48564=VECTOR ( 'NONE', #20784, 999.9999999999998863 ) ;
#48565=CARTESIAN_POINT ( 'NONE',  ( -19.12512386491386707, 2.067327705546508021, 4.044820755108049504 ) ) ;
#48566=CARTESIAN_POINT ( 'NONE',  ( -16.74222506960423829, 0.000000000000000000, 6.167443538023113625 ) ) ;
#48567=CARTESIAN_POINT ( 'NONE',  ( -19.01034150907313247, 3.038739411681508518, 3.969242270749952617 ) ) ;
#48568=EDGE_CURVE ( 'NONE', #37070, #26836, #48640, .T. ) ;
#48569=ORIENTED_EDGE ( 'NONE', *, *, #33563, .T. ) ;
#48570=AXIS2_PLACEMENT_3D ( 'NONE', #29932, #51230, #33367 ) ;
#48571=VECTOR ( 'NONE', #12724, 1000.000000000000000 ) ;
#48572=VERTEX_POINT ( 'NONE', #30762 ) ;
#48573=LINE ( 'NONE', #10223, #44078 ) ;
#48575=ORIENTED_EDGE ( 'NONE', *, *, #26887, .T. ) ;
#48576=CARTESIAN_POINT ( 'NONE',  ( -14.96915702288384153, -4.565544526780664469, 2.550185285927776935 ) ) ;
#48577=ORIENTED_EDGE ( 'NONE', *, *, #40525, .F. ) ;
#48578=CARTESIAN_POINT ( 'NONE',  ( -10.00813838035478298, 0.000000000000000000, 10.77830692922518452 ) ) ;
#48579=VECTOR ( 'NONE', #5986, 1000.000000000000114 ) ;
#48580=EDGE_LOOP ( 'NONE', ( #15408, #6664, #44739, #38923, #2439 ) ) ;
#48581=ORIENTED_EDGE ( 'NONE', *, *, #890, .T. ) ;
#48582=ORIENTED_EDGE ( 'NONE', *, *, #39993, .F. ) ;
#48583=VECTOR ( 'NONE', #43831, 1000.000000000000114 ) ;
#48584=PLANE ( 'NONE',  #42921 ) ;
#48585=FACE_OUTER_BOUND ( 'NONE', #34147, .T. ) ;
#48586=VECTOR ( 'NONE', #18669, 1000.000000000000000 ) ;
#48587=FACE_OUTER_BOUND ( 'NONE', #8571, .T. ) ;
#48588=PLANE ( 'NONE',  #29316 ) ;
#48589=VERTEX_POINT ( 'NONE', #48330 ) ;
#48590=ADVANCED_FACE ( 'NONE', ( #9443 ), #53187, .F. ) ;
#48591=VECTOR ( 'NONE', #10200, 1000.000000000000227 ) ;
#48592=EDGE_LOOP ( 'NONE', ( #51188, #19222, #6695, #39148 ) ) ;
#48593=AXIS2_PLACEMENT_3D ( 'NONE', #8037, #42651, #3747 ) ;
#48594=DIRECTION ( 'NONE',  ( 0.5449076811759707706, 0.6444004775717708799, -0.5364919789714476250 ) ) ;
#48596=CARTESIAN_POINT ( 'NONE',  ( -16.79925329029790149, 0.000000000000000000, 13.49544742625427496 ) ) ;
#48597=VECTOR ( 'NONE', #20310, 999.9999999999998863 ) ;
#48598=ORIENTED_EDGE ( 'NONE', *, *, #22834, .T. ) ;
#48599=DIRECTION ( 'NONE',  ( 0.007781995580012662783, 0.000000000000000000, -0.9999697198139514409 ) ) ;
#48600=CARTESIAN_POINT ( 'NONE',  ( -9.961169346929608537, 0.000000000000000000, 4.742887002396194873 ) ) ;
#48601=VECTOR ( 'NONE', #33889, 999.9999999999998863 ) ;
#48602=ADVANCED_FACE ( 'NONE', ( #21678 ), #38993, .F. ) ;
#48603=VERTEX_POINT ( 'NONE', #41973 ) ;
#48604=AXIS2_PLACEMENT_3D ( 'NONE', #43087, #25474, #4201 ) ;
#48605=FACE_OUTER_BOUND ( 'NONE', #36422, .T. ) ;
#48606=ORIENTED_EDGE ( 'NONE', *, *, #47390, .T. ) ;
#48607=ADVANCED_FACE ( 'NONE', ( #27843 ), #33213, .F. ) ;
#48608=EDGE_CURVE ( 'NONE', #47316, #43061, #19583, .T. ) ;
#48609=VECTOR ( 'NONE', #36996, 1000.000000000000227 ) ;
#48610=DIRECTION ( 'NONE',  ( -0.5449076811759708816, 0.6444004775717707689, 0.5364919789714475140 ) ) ;
#48612=ORIENTED_EDGE ( 'NONE', *, *, #23614, .T. ) ;
#48613=CARTESIAN_POINT ( 'NONE',  ( -18.67775241435682432, 0.000000000000000000, 4.136394454059623804 ) ) ;
#48614=CARTESIAN_POINT ( 'NONE',  ( -24.26908309836554878, 0.000000000000000000, 6.108867788427308376 ) ) ;
#48615=LINE ( 'NONE', #14524, #35587 ) ;
#48616=EDGE_CURVE ( 'NONE', #56109, #42504, #23558, .T. ) ;
#48617=ORIENTED_EDGE ( 'NONE', *, *, #12316, .F. ) ;
#48618=PLANE ( 'NONE',  #12971 ) ;
#48619=EDGE_CURVE ( 'NONE', #49950, #23038, #6511, .T. ) ;
#48620=DIRECTION ( 'NONE',  ( 0.7660212471507180654, -0.6427876096865404731, 0.005961354470445141482 ) ) ;
#48621=DIRECTION ( 'NONE',  ( 0.5364919789714477361, 0.6444004775717706579, 0.5449076811759711036 ) ) ;
#48623=DIRECTION ( 'NONE',  ( 0.7660212471507180654, -0.6427876096865404731, 0.005961354470445141482 ) ) ;
#48624=EDGE_CURVE ( 'NONE', #17655, #13435, #2530, .T. ) ;
#48625=DIRECTION ( 'NONE',  ( 0.5364919789714477361, 0.6444004775717706579, 0.5449076811759711036 ) ) ;
#48626=VECTOR ( 'NONE', #31683, 1000.000000000000227 ) ;
#48627=DIRECTION ( 'NONE',  ( 0.007781995580012663651, -3.146120232559066537E-19, -0.9999697198139514409 ) ) ;
#48628=ORIENTED_EDGE ( 'NONE', *, *, #18083, .T. ) ;
#48629=DIRECTION ( 'NONE',  ( -0.005961354470445682716, -0.6427876096865404731, 0.7660212471507180654 ) ) ;
#48630=CARTESIAN_POINT ( 'NONE',  ( -21.47419595591918906, 0.000000000000000000, 5.222628093224860102 ) ) ;
#48631=CARTESIAN_POINT ( 'NONE',  ( -21.47263955680318404, 0.000000000000000000, 5.022634149262071190 ) ) ;
#48632=VERTEX_POINT ( 'NONE', #45984 ) ;
#48633=LINE ( 'NONE', #35857, #48352 ) ;
#48634=DIRECTION ( 'NONE',  ( 0.6427681459581294776, -0.7660444431189769032, 0.005002170337467562802 ) ) ;
#48635=VECTOR ( 'NONE', #965, 1000.000000000000227 ) ;
#48636=ORIENTED_EDGE ( 'NONE', *, *, #9713, .T. ) ;
#48637=ADVANCED_FACE ( 'NONE', ( #11038 ), #32905, .F. ) ;
#48638=CARTESIAN_POINT ( 'NONE',  ( -8.568815055522351898, 0.000000000000000000, 4.953728681663013056 ) ) ;
#48639=AXIS2_PLACEMENT_3D ( 'NONE', #27473, #2478, #2180 ) ;
#48640=LINE ( 'NONE', #13697, #25744 ) ;
#48642=DIRECTION ( 'NONE',  ( 0.000000000000000000, -1.000000000000000000, 0.000000000000000000 ) ) ;
#48643=ADVANCED_FACE ( 'NONE', ( #55069 ), #15318, .F. ) ;
#48645=AXIS2_PLACEMENT_3D ( 'NONE', #31527, #27237, #40305 ) ;
#48646=ORIENTED_EDGE ( 'NONE', *, *, #51890, .T. ) ;
#48647=DIRECTION ( 'NONE',  ( -0.9999697198139514409, -0.000000000000000000, -0.007781995580013368816 ) ) ;
#48648=FACE_OUTER_BOUND ( 'NONE', #8738, .T. ) ;
#48649=DIRECTION ( 'NONE',  ( 0.005002170337468016433, -0.7660444431189770143, -0.6427681459581293666 ) ) ;
#48650=AXIS2_PLACEMENT_3D ( 'NONE', #847, #31797, #35786 ) ;
#48651=CARTESIAN_POINT ( 'NONE',  ( -10.00813838035478298, 0.000000000000000000, 10.77830692922518452 ) ) ;
#48652=VECTOR ( 'NONE', #24853, 1000.000000000000000 ) ;
#48653=DIRECTION ( 'NONE',  ( -0.5364919789714478471, 0.6444004775717705469, -0.5449076811759709926 ) ) ;
#48654=LINE ( 'NONE', #35049, #52129 ) ;
#48655=ORIENTED_EDGE ( 'NONE', *, *, #14504, .F. ) ;
#48656=DIRECTION ( 'NONE',  ( -0.7660212471507179544, -0.6427876096865405842, -0.005961354470445141482 ) ) ;
#48657=AXIS2_PLACEMENT_3D ( 'NONE', #18976, #44806, #23514 ) ;
#48659=DIRECTION ( 'NONE',  ( -0.6427681459581293666, -0.7660444431189770143, -0.005002170337467561935 ) ) ;
#48661=CARTESIAN_POINT ( 'NONE',  ( -29.86352658060627618, 0.000000000000000000, 8.481329010720569883 ) ) ;
#48662=CARTESIAN_POINT ( 'NONE',  ( -24.26908309836554878, 0.000000000000000000, 6.108867788427308376 ) ) ;
#48663=CARTESIAN_POINT ( 'NONE',  ( -16.81345671998191449, 0.000000000000000000, 3.412238694616132495 ) ) ;
#48664=ORIENTED_EDGE ( 'NONE', *, *, #9721, .T. ) ;
#48665=CARTESIAN_POINT ( 'NONE',  ( -26.13493519185646008, 0.000000000000000000, 7.033017491833586377 ) ) ;
#48666=ADVANCED_FACE ( 'NONE', ( #36919 ), #28665, .F. ) ;
#48667=ORIENTED_EDGE ( 'NONE', *, *, #9369, .T. ) ;
#48668=AXIS2_PLACEMENT_3D ( 'NONE', #43444, #35769, #44547 ) ;
#48669=EDGE_LOOP ( 'NONE', ( #54579, #17097, #23753, #51221 ) ) ;
#48670=VERTEX_POINT ( 'NONE', #41695 ) ;
#48671=VERTEX_POINT ( 'NONE', #45152 ) ;
#48674=ORIENTED_EDGE ( 'NONE', *, *, #19223, .T. ) ;
#48675=LINE ( 'NONE', #18008, #45779 ) ;
#48676=PLANE ( 'NONE',  #5030 ) ;
#48677=ADVANCED_FACE ( 'NONE', ( #7092 ), #50524, .F. ) ;
#48678=VERTEX_POINT ( 'NONE', #20407 ) ;
#48679=PLANE ( 'NONE',  #38609 ) ;
#48680=AXIS2_PLACEMENT_3D ( 'NONE', #10379, #49568, #23982 ) ;
#48681=ORIENTED_EDGE ( 'NONE', *, *, #45178, .T. ) ;
#48682=CARTESIAN_POINT ( 'NONE',  ( -16.06709938707323460, 0.000000000000000000, 13.13181314741652628 ) ) ;
#48683=ORIENTED_EDGE ( 'NONE', *, *, #16794, .F. ) ;
#48684=EDGE_CURVE ( 'NONE', #20189, #36118, #11623, .T. ) ;
#48685=VECTOR ( 'NONE', #2767, 999.9999999999998863 ) ;
#48686=DIRECTION ( 'NONE',  ( 0.000000000000000000, -0.000000000000000000, -1.000000000000000000 ) ) ;
#48687=FACE_OUTER_BOUND ( 'NONE', #14867, .T. ) ;
#48688=CARTESIAN_POINT ( 'NONE',  ( -15.05780494465513897, 0.000000000000000000, 2.856563456659266809 ) ) ;
#48689=DIRECTION ( 'NONE',  ( 0.007781995580012662783, 0.000000000000000000, -0.9999697198139514409 ) ) ;
#48690=DIRECTION ( 'NONE',  ( 0.5364919789714477361, 0.6444004775717706579, 0.5449076811759711036 ) ) ;
#48691=DIRECTION ( 'NONE',  ( 0.9999697198139515519, 0.000000000000000000, 0.007781995580013368816 ) ) ;
#48692=ORIENTED_EDGE ( 'NONE', *, *, #25878, .F. ) ;
#48693=ORIENTED_EDGE ( 'NONE', *, *, #57, .F. ) ;
#48694=VECTOR ( 'NONE', #44534, 1000.000000000000114 ) ;
#48695=EDGE_CURVE ( 'NONE', #9006, #4182, #20106, .T. ) ;
#48696=DIRECTION ( 'NONE',  ( 0.005002170337468016433, -0.7660444431189770143, -0.6427681459581293666 ) ) ;
#48697=LINE ( 'NONE', #1546, #43915 ) ;
#48698=ADVANCED_FACE ( 'NONE', ( #3076 ), #37439, .F. ) ;
#48699=DIRECTION ( 'NONE',  ( -0.005002170337468016433, -0.7660444431189770143, 0.6427681459581293666 ) ) ;
#48700=VECTOR ( 'NONE', #24959, 999.9999999999998863 ) ;
#48701=LINE ( 'NONE', #9805, #32183 ) ;
#48702=ORIENTED_EDGE ( 'NONE', *, *, #50119, .F. ) ;
#48703=DIRECTION ( 'NONE',  ( 0.000000000000000000, -0.000000000000000000, -1.000000000000000000 ) ) ;
#48704=CARTESIAN_POINT ( 'NONE',  ( -15.88053067323646417, -0.1191753592594197858, 2.950163842912994383 ) ) ;
#48705=ORIENTED_EDGE ( 'NONE', *, *, #39770, .T. ) ;
#48706=LINE ( 'NONE', #44696, #15708 ) ;
#48707=CARTESIAN_POINT ( 'NONE',  ( -9.075990533167328067, 0.000000000000000000, 10.41622904950343909 ) ) ;
#48708=ORIENTED_EDGE ( 'NONE', *, *, #2239, .T. ) ;
#48709=EDGE_CURVE ( 'NONE', #38932, #39994, #49402, .T. ) ;
#48710=CARTESIAN_POINT ( 'NONE',  ( -11.34801427605302138, 0.000000000000000000, 3.824104101281660562 ) ) ;
#48711=DIRECTION ( 'NONE',  ( 0.005002170337468016433, -0.7660444431189770143, -0.6427681459581293666 ) ) ;
#48712=CARTESIAN_POINT ( 'NONE',  ( -12.15271748404464880, 0.000000000000000000, 1.601849296007406664 ) ) ;
#48713=LINE ( 'NONE', #19423, #53207 ) ;
#48714=VECTOR ( 'NONE', #20789, 999.9999999999998863 ) ;
#48715=DIRECTION ( 'NONE',  ( -0.7660212471507179544, -0.6427876096865405842, -0.005961354470445141482 ) ) ;
#48716=EDGE_CURVE ( 'NONE', #52840, #46588, #19282, .T. ) ;
#48718=ORIENTED_EDGE ( 'NONE', *, *, #25731, .T. ) ;
#48719=CARTESIAN_POINT ( 'NONE',  ( -20.74129076085852930, 1.743523803501506819, 7.799362421763929909 ) ) ;
#48720=DIRECTION ( 'NONE',  ( 0.007781995580012663651, -3.146120232559066537E-19, -0.9999697198139514409 ) ) ;
#48721=DIRECTION ( 'NONE',  ( 0.9999697198139515519, 0.000000000000000000, 0.007781995580013368816 ) ) ;
#48722=CARTESIAN_POINT ( 'NONE',  ( -18.66354898467281132, 0.000000000000000000, 14.21960318569776582 ) ) ;
#48723=VECTOR ( 'NONE', #36160, 1000.000000000000227 ) ;
#48724=LINE ( 'NONE', #35958, #29390 ) ;
#48725=ORIENTED_EDGE ( 'NONE', *, *, #20069, .T. ) ;
#48727=CARTESIAN_POINT ( 'NONE',  ( -32.65919192261063841, -0.1191753592594197858, 9.467565677904410393 ) ) ;
#48728=DIRECTION ( 'NONE',  ( 0.005002170337468016433, -0.7660444431189770143, -0.6427681459581293666 ) ) ;
#48729=VECTOR ( 'NONE', #46103, 1000.000000000000000 ) ;
#48730=DIRECTION ( 'NONE',  ( -0.6427681459581293666, -0.7660444431189770143, -0.005002170337467561935 ) ) ;
#48731=ORIENTED_EDGE ( 'NONE', *, *, #29913, .F. ) ;
#48732=DIRECTION ( 'NONE',  ( 0.9999697198139515519, 0.000000000000000000, 0.007781995580013368816 ) ) ;
#48733=EDGE_LOOP ( 'NONE', ( #943, #10801, #37326, #44391 ) ) ;
#48734=CARTESIAN_POINT ( 'NONE',  ( 1.086233639165236964, 0.000000000000000000, 2.796443541562362078 ) ) ;
#48735=ADVANCED_FACE ( 'NONE', ( #45680 ), #7936, .F. ) ;
#48737=VERTEX_POINT ( 'NONE', #13018 ) ;
#48738=VECTOR ( 'NONE', #30550, 1000.000000000000114 ) ;
#48739=DIRECTION ( 'NONE',  ( 0.007781995580012663651, -3.146120232559066537E-19, -0.9999697198139514409 ) ) ;
#48740=ADVANCED_FACE ( 'NONE', ( #46511 ), #20957, .F. ) ;
#48741=ORIENTED_EDGE ( 'NONE', *, *, #6596, .T. ) ;
#48742=ORIENTED_EDGE ( 'NONE', *, *, #42966, .F. ) ;
#48743=VERTEX_POINT ( 'NONE', #17262 ) ;
#48744=PLANE ( 'NONE',  #46602 ) ;
#48745=EDGE_LOOP ( 'NONE', ( #40777, #13031, #10105, #18801 ) ) ;
#48746=EDGE_CURVE ( 'NONE', #30407, #4309, #38279, .T. ) ;
#48747=ORIENTED_EDGE ( 'NONE', *, *, #24056, .F. ) ;
#48749=CARTESIAN_POINT ( 'NONE',  ( -13.22224978533305695, 0.000000000000000000, 5.825504729793420822 ) ) ;
#48750=EDGE_LOOP ( 'NONE', ( #16456, #38776, #23333, #46065 ) ) ;
#48751=ADVANCED_FACE ( 'NONE', ( #38579 ), #16711, .F. ) ;
#48752=ADVANCED_FACE ( 'NONE', ( #55908 ), #34044, .F. ) ;
#48754=EDGE_LOOP ( 'NONE', ( #9564, #23452, #55139, #11691 ) ) ;
#48755=LINE ( 'NONE', #26307, #28549 ) ;
#48756=ORIENTED_EDGE ( 'NONE', *, *, #27019, .T. ) ;
#48757=ORIENTED_EDGE ( 'NONE', *, *, #21474, .F. ) ;
#48758=CARTESIAN_POINT ( 'NONE',  ( -13.70413100320583943, 0.000000000000000000, 8.037747037571998376 ) ) ;
#48759=CARTESIAN_POINT ( 'NONE',  ( 2.072287782118878319, 0.000000000000000000, -2.950529333540147015 ) ) ;
#48760=DIRECTION ( 'NONE',  ( -0.9999697198139514409, -0.000000000000000000, -0.007781995580013368816 ) ) ;
#48761=LINE ( 'NONE', #36000, #43182 ) ;
#48762=ORIENTED_EDGE ( 'NONE', *, *, #28084, .T. ) ;
#48763=DIRECTION ( 'NONE',  ( 0.007781995580012663651, -3.146120232559066537E-19, -0.9999697198139514409 ) ) ;
#48764=ORIENTED_EDGE ( 'NONE', *, *, #29169, .F. ) ;
#48765=ADVANCED_FACE ( 'NONE', ( #29793 ), #42818, .F. ) ;
#48766=DIRECTION ( 'NONE',  ( -0.7660212471507179544, -0.6427876096865405842, -0.005961354470445141482 ) ) ;
#48767=EDGE_CURVE ( 'NONE', #8862, #9909, #4501, .T. ) ;
#48768=CARTESIAN_POINT ( 'NONE',  ( -14.94760462649100496, 0.000000000000000000, 2.488088991209854051 ) ) ;
#48769=VECTOR ( 'NONE', #53271, 999.9999999999998863 ) ;
#48770=DIRECTION ( 'NONE',  ( 0.9999697198139515519, 0.000000000000000000, 0.007781995580013368816 ) ) ;
#48771=CARTESIAN_POINT ( 'NONE',  ( -12.29010193814559848, 0.000000000000000000, 5.463426850071675389 ) ) ;
#48772=FACE_OUTER_BOUND ( 'NONE', #2383, .T. ) ;
#48773=ADVANCED_FACE ( 'NONE', ( #51899 ), #56178, .F. ) ;
#48774=DIRECTION ( 'NONE',  ( 0.9999697198139515519, 0.000000000000000000, 0.007781995580013368816 ) ) ;
#48775=DIRECTION ( 'NONE',  ( 0.005002170337468016433, -0.7660444431189770143, -0.6427681459581293666 ) ) ;
#48776=ORIENTED_EDGE ( 'NONE', *, *, #52345, .F. ) ;
#48777=CARTESIAN_POINT ( 'NONE',  ( -13.73280004183141401, 5.629170628041515023, 1.836617620612386537 ) ) ;
#48778=ORIENTED_EDGE ( 'NONE', *, *, #48849, .T. ) ;
#48779=EDGE_CURVE ( 'NONE', #29572, #6907, #33739, .T. ) ;
#48781=CARTESIAN_POINT ( 'NONE',  ( 2.072287782118878319, 0.000000000000000000, -2.950529333540147015 ) ) ;
#48782=DIRECTION ( 'NONE',  ( 0.6427681459581294776, -0.7660444431189769032, 0.005002170337467562802 ) ) ;
#48783=DIRECTION ( 'NONE',  ( 0.7660212471507180654, -0.6427876096865404731, 0.005961354470445141482 ) ) ;
#48784=CARTESIAN_POINT ( 'NONE',  ( -10.47421230394850866, 0.000000000000000000, 10.95934586908605723 ) ) ;
#48785=DIRECTION ( 'NONE',  ( 0.7660212471507180654, -0.6427876096865404731, 0.005961354470445141482 ) ) ;
#48786=EDGE_CURVE ( 'NONE', #11442, #45245, #47360, .T. ) ;
#48787=CARTESIAN_POINT ( 'NONE',  ( -18.19747506107908563, 0.000000000000000000, 14.03856424583689311 ) ) ;
#48790=CARTESIAN_POINT ( 'NONE',  ( -17.64806569016193194, 1.419719901456505617, 3.491743278477204449 ) ) ;
#48791=LINE ( 'NONE', #22928, #21291 ) ;
#48792=DIRECTION ( 'NONE',  ( -0.7660212471507179544, -0.6427876096865405842, -0.005961354470445141482 ) ) ;
#48793=CARTESIAN_POINT ( 'NONE',  ( -18.86354292863559579, 0.000000000000000000, 14.21804678658176080 ) ) ;
#48794=CARTESIAN_POINT ( 'NONE',  ( -19.31455064293810509, -1.975113310420659740, 4.320732056343596028 ) ) ;
#48795=CARTESIAN_POINT ( 'NONE',  ( -20.22944524586242210, 0.6102101463440047224, 4.520266361366938490 ) ) ;
#48796=CARTESIAN_POINT ( 'NONE',  ( -10.47421230394850866, 0.000000000000000000, 10.95934586908605723 ) ) ;
#48798=LINE ( 'NONE', #32320, #33754 ) ;
#48799=ORIENTED_EDGE ( 'NONE', *, *, #45706, .T. ) ;
#48800=ORIENTED_EDGE ( 'NONE', *, *, #17916, .F. ) ;
#48801=ORIENTED_EDGE ( 'NONE', *, *, #26233, .F. ) ;
#48802=ORIENTED_EDGE ( 'NONE', *, *, #35440, .F. ) ;
#48803=ORIENTED_EDGE ( 'NONE', *, *, #14977, .T. ) ;
#48804=PLANE ( 'NONE',  #7886 ) ;
#48805=PLANE ( 'NONE',  #1322 ) ;
#48806=EDGE_CURVE ( 'NONE', #29609, #3681, #8784, .T. ) ;
#48808=VECTOR ( 'NONE', #52260, 1000.000000000000114 ) ;
#48809=ORIENTED_EDGE ( 'NONE', *, *, #47951, .F. ) ;
#48810=EDGE_LOOP ( 'NONE', ( #14704, #32030, #28006, #35303 ) ) ;
#48811=EDGE_LOOP ( 'NONE', ( #22881, #5678, #28772, #18072 ) ) ;
#48812=EDGE_CURVE ( 'NONE', #10313, #48572, #25800, .T. ) ;
#48814=ORIENTED_EDGE ( 'NONE', *, *, #55092, .T. ) ;
#48816=DIRECTION ( 'NONE',  ( -0.5449076811759708816, 0.6444004775717707689, 0.5364919789714475140 ) ) ;
#48817=ORIENTED_EDGE ( 'NONE', *, *, #21273, .T. ) ;
#48818=DIRECTION ( 'NONE',  ( 0.007781995580012663651, -3.146120232559066537E-19, -0.9999697198139514409 ) ) ;
#48819=ORIENTED_EDGE ( 'NONE', *, *, #13677, .T. ) ;
#48820=DIRECTION ( 'NONE',  ( 0.000000000000000000, -1.000000000000000000, 0.000000000000000000 ) ) ;
#48821=PLANE ( 'NONE',  #14860 ) ;
#48822=ADVANCED_FACE ( 'NONE', ( #33477 ), #50781, .F. ) ;
#48823=DIRECTION ( 'NONE',  ( 0.9999697198139515519, 0.000000000000000000, 0.007781995580013368816 ) ) ;
#48824=PLANE ( 'NONE',  #23321 ) ;
#48825=ORIENTED_EDGE ( 'NONE', *, *, #45210, .T. ) ;
#48826=DIRECTION ( 'NONE',  ( 0.5364919789714477361, 0.6444004775717706579, 0.5449076811759711036 ) ) ;
#48827=CARTESIAN_POINT ( 'NONE',  ( -19.52142429013490599, 0.000000000000000000, 5.037818957641762019 ) ) ;
#48828=CARTESIAN_POINT ( 'NONE',  ( -16.46895995621009234, 0.000000000000000000, 5.061573940901824997 ) ) ;
#48829=ORIENTED_EDGE ( 'NONE', *, *, #55303, .F. ) ;
#48830=CARTESIAN_POINT ( 'NONE',  ( -12.23851102634202448, -0.1191753592594197858, 11.68427982808754884 ) ) ;
#48831=ORIENTED_EDGE ( 'NONE', *, *, #27910, .F. ) ;
#48832=EDGE_CURVE ( 'NONE', #21379, #7579, #46824, .T. ) ;
#48833=LINE ( 'NONE', #52519, #21966 ) ;
#48834=DIRECTION ( 'NONE',  ( 0.007781995580012663651, -3.146120232559066537E-19, -0.9999697198139514409 ) ) ;
#48835=DIRECTION ( 'NONE',  ( 0.5364919789714477361, 0.6444004775717706579, 0.5449076811759711036 ) ) ;
#48836=CARTESIAN_POINT ( 'NONE',  ( -9.508028664109653860, 0.000000000000000000, 6.223741727195261753 ) ) ;
#48838=EDGE_CURVE ( 'NONE', #15196, #48501, #9040, .T. ) ;
#48839=FACE_OUTER_BOUND ( 'NONE', #19050, .T. ) ;
#48840=PLANE ( 'NONE',  #38839 ) ;
#48841=DIRECTION ( 'NONE',  ( -0.6427681459581293666, -0.7660444431189770143, -0.005002170337467561935 ) ) ;
#48843=EDGE_CURVE ( 'NONE', #3673, #44660, #5072, .T. ) ;
#48844=LINE ( 'NONE', #27530, #41912 ) ;
#48845=ORIENTED_EDGE ( 'NONE', *, *, #39371, .F. ) ;
#48846=LINE ( 'NONE', #9943, #26634 ) ;
#48847=CARTESIAN_POINT ( 'NONE',  ( -18.71591809603438961, -0.1191753592594151645, 8.098747179663282836 ) ) ;
#48848=CARTESIAN_POINT ( 'NONE',  ( -15.92234860797731066, -0.1191753592594211320, 7.381823243755817110 ) ) ;
#48849=EDGE_CURVE ( 'NONE', #27501, #20973, #39968, .T. ) ;
#48850=CARTESIAN_POINT ( 'NONE',  ( -14.56888064431065821, -0.1191753592594197858, 12.58947452739191064 ) ) ;
#48851=VECTOR ( 'NONE', #27896, 1000.000000000000000 ) ;
#48852=ADVANCED_FACE ( 'NONE', ( #36030 ), #26343, .F. ) ;
#48853=LINE ( 'NONE', #32627, #10097 ) ;
#48854=CARTESIAN_POINT ( 'NONE',  ( -20.05727171210132198, 2.067327705546508021, 4.406898634829794936 ) ) ;
#48855=CARTESIAN_POINT ( 'NONE',  ( -19.60912206198628027, -0.1191753592594197858, 4.398475361799976113 ) ) ;
#48856=ORIENTED_EDGE ( 'NONE', *, *, #17842, .F. ) ;
#48857=EDGE_LOOP ( 'NONE', ( #52315, #7418, #35605 ) ) ;
#48858=CARTESIAN_POINT ( 'NONE',  ( -17.73140113748535285, 0.000000000000000000, 13.85752530597602039 ) ) ;
#48859=CARTESIAN_POINT ( 'NONE',  ( -14.89804774976630597, 0.000000000000000000, 8.028455701383972354 ) ) ;
#48860=VERTEX_POINT ( 'NONE', #18689 ) ;
#48861=DIRECTION ( 'NONE',  ( 0.000000000000000000, -1.000000000000000000, 0.000000000000000000 ) ) ;
#48862=VERTEX_POINT ( 'NONE', #27469 ) ;
#48863=CARTESIAN_POINT ( 'NONE',  ( -12.26866590921934552, 0.000000000000000000, 2.708943167972348132 ) ) ;
#48864=ORIENTED_EDGE ( 'NONE', *, *, #51997, .F. ) ;
#48866=EDGE_LOOP ( 'NONE', ( #25545, #11966, #27561, #30738 ) ) ;
#48867=CARTESIAN_POINT ( 'NONE',  ( -10.00813838035478298, 0.000000000000000000, 10.77830692922518452 ) ) ;
#48868=CARTESIAN_POINT ( 'NONE',  ( 2.072287782118878319, 0.000000000000000000, -2.950529333540147015 ) ) ;
#48869=CARTESIAN_POINT ( 'NONE',  ( 2.072287782118878319, 0.000000000000000000, -2.950529333540147015 ) ) ;
#48870=EDGE_CURVE ( 'NONE', #3819, #8281, #53337, .T. ) ;
#48871=DIRECTION ( 'NONE',  ( 0.007781995580012663651, -3.146120232559066537E-19, -0.9999697198139514409 ) ) ;
#48872=ORIENTED_EDGE ( 'NONE', *, *, #2710, .F. ) ;
#48873=VERTEX_POINT ( 'NONE', #22932 ) ;
#48874=EDGE_CURVE ( 'NONE', #40198, #54534, #1053, .T. ) ;
#48875=EDGE_CURVE ( 'NONE', #49166, #49589, #23233, .T. ) ;
#48877=ORIENTED_EDGE ( 'NONE', *, *, #7804, .T. ) ;
#48878=DIRECTION ( 'NONE',  ( 0.5449076811759707706, 0.6444004775717708799, -0.5364919789714476250 ) ) ;
#48879=EDGE_LOOP ( 'NONE', ( #18566, #35642, #35127, #27220 ) ) ;
#48880=DIRECTION ( 'NONE',  ( 0.9999697198139515519, 0.000000000000000000, 0.007781995580013368816 ) ) ;
#48881=DIRECTION ( 'NONE',  ( 0.007781995580012662783, 0.000000000000000000, -0.9999697198139514409 ) ) ;
#48882=( GEOMETRIC_REPRESENTATION_CONTEXT ( 3 ) GLOBAL_UNCERTAINTY_ASSIGNED_CONTEXT ( ( #33645 ) ) GLOBAL_UNIT_ASSIGNED_CONTEXT ( ( #27242, #35778, #14477 ) ) REPRESENTATION_CONTEXT ( 'NONE', 'WORKASPACE' ) );
#48883=ORIENTED_EDGE ( 'NONE', *, *, #12634, .T. ) ;
#48884=PLANE ( 'NONE',  #24067 ) ;
#48885=ORIENTED_EDGE ( 'NONE', *, *, #48172, .T. ) ;
#48886=ADVANCED_FACE ( 'NONE', ( #35723 ), #40254, .F. ) ;
#48887=PLANE ( 'NONE',  #20912 ) ;
#48888=VERTEX_POINT ( 'NONE', #5352 ) ;
#48889=LINE ( 'NONE', #26445, #46677 ) ;
#48890=PLANE ( 'NONE',  #35754 ) ;
#48891=LINE ( 'NONE', #15100, #12846 ) ;
#48892=ORIENTED_EDGE ( 'NONE', *, *, #34646, .F. ) ;
#48893=CARTESIAN_POINT ( 'NONE',  ( -14.36685551739899758, -4.403642575758163424, 2.321396446839630201 ) ) ;
#48894=DIRECTION ( 'NONE',  ( -0.7660212471507179544, -0.6427876096865405842, -0.005961354470445141482 ) ) ;
#48895=PLANE ( 'NONE',  #50412 ) ;
#48896=EDGE_CURVE ( 'NONE', #9006, #43180, #39717, .T. ) ;
#48897=CARTESIAN_POINT ( 'NONE',  ( -25.20278734466900517, 0.000000000000000000, 6.670939612111840944 ) ) ;
#48898=LINE ( 'NONE', #23058, #9785 ) ;
#48900=VERTEX_POINT ( 'NONE', #206 ) ;
#48901=LINE ( 'NONE', #39820, #27078 ) ;
#48902=DIRECTION ( 'NONE',  ( -0.9999697198139514409, -0.000000000000000000, -0.007781995580013368816 ) ) ;
#48903=FACE_OUTER_BOUND ( 'NONE', #53503, .T. ) ;
#48904=VERTEX_POINT ( 'NONE', #47942 ) ;
#48905=DIRECTION ( 'NONE',  ( 0.007781995580012663651, 0.000000000000000000, -0.9999697198139515519 ) ) ;
#48906=CARTESIAN_POINT ( 'NONE',  ( -13.73672976910459909, 0.000000000000000000, 12.22661844811216270 ) ) ;
#48907=EDGE_LOOP ( 'NONE', ( #39667, #41102, #21570 ) ) ;
#48908=DIRECTION ( 'NONE',  ( -0.6427681459581293666, -0.7660444431189770143, -0.005002170337467561935 ) ) ;
#48909=EDGE_CURVE ( 'NONE', #16440, #20884, #10150, .T. ) ;
#48910=DIRECTION ( 'NONE',  ( 0.9999697198139515519, 0.000000000000000000, 0.007781995580013368816 ) ) ;
#48911=PLANE ( 'NONE',  #24206 ) ;
#48912=LINE ( 'NONE', #13699, #34673 ) ;
#48913=ORIENTED_EDGE ( 'NONE', *, *, #41169, .T. ) ;
#48914=ORIENTED_EDGE ( 'NONE', *, *, #126, .T. ) ;
#48915=CARTESIAN_POINT ( 'NONE',  ( -12.60458797795435615, 0.000000000000000000, 11.86609696750642229 ) ) ;
#48916=CARTESIAN_POINT ( 'NONE',  ( -9.870572735022063782, -0.1191753592594185784, 5.951591283708881797 ) ) ;
#48917=CARTESIAN_POINT ( 'NONE',  ( -15.40103151951671734, 0.000000000000000000, 12.95233060667165681 ) ) ;
#48918=EDGE_CURVE ( 'NONE', #33161, #27147, #43948, .T. ) ;
#48919=DIRECTION ( 'NONE',  ( -0.005961354470445682716, -0.6427876096865404731, 0.7660212471507180654 ) ) ;
#48920=DIRECTION ( 'NONE',  ( -0.005002170337468016433, -0.7660444431189770143, 0.6427681459581293666 ) ) ;
#48922=CARTESIAN_POINT ( 'NONE',  ( -18.47913287522675674, -4.241740624735661491, 10.82127350084811290 ) ) ;
#48923=VERTEX_POINT ( 'NONE', #52737 ) ;
#48924=EDGE_CURVE ( 'NONE', #18021, #15763, #52479, .T. ) ;
#48925=CARTESIAN_POINT ( 'NONE',  ( -8.621502653355362256, 6.299122464087065332, 0.1305108423619513736 ) ) ;
#48926=ADVANCED_FACE ( 'NONE', ( #48194 ), #14156, .F. ) ;
#48927=DIRECTION ( 'NONE',  ( -0.7660212471507179544, -0.6427876096865405842, -0.005961354470445141482 ) ) ;
#48928=ORIENTED_EDGE ( 'NONE', *, *, #43668, .T. ) ;
#48929=LINE ( 'NONE', #40115, #7494 ) ;
#48930=EDGE_CURVE ( 'NONE', #17110, #20373, #9615, .T. ) ;
#48931=CARTESIAN_POINT ( 'NONE',  ( -29.86274838104827367, -0.1191753592594197858, 8.381332038739175871 ) ) ;
#48933=VERTEX_POINT ( 'NONE', #22399 ) ;
#48934=FACE_OUTER_BOUND ( 'NONE', #28111, .T. ) ;
#48935=ADVANCED_FACE ( 'NONE', ( #31171 ), #26936, .F. ) ;
#48936=EDGE_LOOP ( 'NONE', ( #30569, #38076, #42593 ) ) ;
#48937=EDGE_CURVE ( 'NONE', #33164, #22818, #5609, .T. ) ;
#48938=VERTEX_POINT ( 'NONE', #53583 ) ;
#48939=EDGE_LOOP ( 'NONE', ( #27852, #39256, #1830, #6341 ) ) ;
#48940=ORIENTED_EDGE ( 'NONE', *, *, #5515, .T. ) ;
#48942=ORIENTED_EDGE ( 'NONE', *, *, #11401, .T. ) ;
#48943=CARTESIAN_POINT ( 'NONE',  ( 2.072287782118878319, 0.000000000000000000, -2.950529333540147015 ) ) ;
#48944=DIRECTION ( 'NONE',  ( -0.9999697198139514409, -0.000000000000000000, -0.007781995580013368816 ) ) ;
#48945=ADVANCED_FACE ( 'NONE', ( #50455 ), #15798, .F. ) ;
#48946=ORIENTED_EDGE ( 'NONE', *, *, #53779, .F. ) ;
#48947=ORIENTED_EDGE ( 'NONE', *, *, #28585, .F. ) ;
#48948=CARTESIAN_POINT ( 'NONE',  ( -13.27065584551087163, 0.000000000000000000, 12.04557950825129176 ) ) ;
#48949=VERTEX_POINT ( 'NONE', #54688 ) ;
#48950=EDGE_CURVE ( 'NONE', #2679, #34678, #10979, .T. ) ;
#48951=FACE_OUTER_BOUND ( 'NONE', #14850, .T. ) ;
#48952=DIRECTION ( 'NONE',  ( -0.5364919789714478471, 0.6444004775717705469, -0.5449076811759709926 ) ) ;
#48953=DIRECTION ( 'NONE',  ( 0.007781995580012663651, 0.000000000000000000, -0.9999697198139515519 ) ) ;
#48954=CARTESIAN_POINT ( 'NONE',  ( 2.072287782118878319, 0.000000000000000000, -2.950529333540147015 ) ) ;
#48955=CARTESIAN_POINT ( 'NONE',  ( -21.47419595591918906, 0.000000000000000000, 5.222628093224860102 ) ) ;
#48957=VERTEX_POINT ( 'NONE', #33138 ) ;
#48958=ORIENTED_EDGE ( 'NONE', *, *, #10539, .F. ) ;
#48960=DIRECTION ( 'NONE',  ( 0.5364919789714477361, 0.6444004775717706579, 0.5449076811759711036 ) ) ;
#48961=FACE_OUTER_BOUND ( 'NONE', #51148, .T. ) ;
#48962=CARTESIAN_POINT ( 'NONE',  ( -18.96000877805918350, -2.622721114510659035, 8.350975192617999809 ) ) ;
#48963=ORIENTED_EDGE ( 'NONE', *, *, #53436, .F. ) ;
#48964=CARTESIAN_POINT ( 'NONE',  ( -21.51982916103365540, 5.467268677019013978, 4.866529699019949362 ) ) ;
#48965=CARTESIAN_POINT ( 'NONE',  ( -14.20280369269832832, 0.000000000000000000, 12.40765738797303719 ) ) ;
#48966=ORIENTED_EDGE ( 'NONE', *, *, #50044, .T. ) ;
#48967=FACE_OUTER_BOUND ( 'NONE', #4295, .T. ) ;
#48968=CARTESIAN_POINT ( 'NONE',  ( -12.15193928448664629, -0.1191753592594197858, 1.501852324026012209 ) ) ;
#48969=ORIENTED_EDGE ( 'NONE', *, *, #33660, .T. ) ;
#48971=CARTESIAN_POINT ( 'NONE',  ( -17.83139810946674686, -0.1191753592594197858, 13.85674710641801788 ) ) ;
#48972=ADVANCED_FACE ( 'NONE', ( #46176 ), #2174, .F. ) ;
#48973=DIRECTION ( 'NONE',  ( -0.5364919789714478471, 0.6444004775717705469, -0.5449076811759709926 ) ) ;
#48974=DIRECTION ( 'NONE',  ( -0.7660212471507179544, -0.6427876096865405842, -0.005961354470445141482 ) ) ;
#48975=DIRECTION ( 'NONE',  ( -0.5364919789714478471, 0.6444004775717705469, -0.5449076811759709926 ) ) ;
#48976=ORIENTED_EDGE ( 'NONE', *, *, #52566, .T. ) ;
#48977=VERTEX_POINT ( 'NONE', #20046 ) ;
#48978=LINE ( 'NONE', #22319, #19408 ) ;
#48979=PLANE ( 'NONE',  #31315 ) ;
#48980=DIRECTION ( 'NONE',  ( 0.7660212471507180654, -0.6427876096865404731, 0.005961354470445141482 ) ) ;
#48981=EDGE_CURVE ( 'NONE', #12878, #21230, #7279, .T. ) ;
#48982=CARTESIAN_POINT ( 'NONE',  ( -11.63409325785757353, 0.000000000000000000, 6.576528270728981163 ) ) ;
#48983=CARTESIAN_POINT ( 'NONE',  ( -8.957215931586203439, 8.728699564772798070, 6.697660431825324778 ) ) ;
#48984=VERTEX_POINT ( 'NONE', #49630 ) ;
#48986=CARTESIAN_POINT ( 'NONE',  ( -24.27063949748155380, 0.000000000000000000, 6.308861732390097288 ) ) ;
#48987=EDGE_CURVE ( 'NONE', #18068, #42908, #12155, .T. ) ;
#48988=VECTOR ( 'NONE', #34315, 999.9999999999998863 ) ;
#48989=CARTESIAN_POINT ( 'NONE',  ( -22.40634380310664397, 0.000000000000000000, 5.584705972946605534 ) ) ;
#48990=DIRECTION ( 'NONE',  ( -0.6427681459581293666, -0.7660444431189770143, -0.005002170337467561935 ) ) ;
#48991=ORIENTED_EDGE ( 'NONE', *, *, #17194, .T. ) ;
#48992=CARTESIAN_POINT ( 'NONE',  ( -11.67244013076689946, 0.000000000000000000, 11.50401908778467863 ) ) ;
#48993=ORIENTED_EDGE ( 'NONE', *, *, #43247, .F. ) ;
#48994=LINE ( 'NONE', #48734, #19587 ) ;
#48995=DIRECTION ( 'NONE',  ( -0.5449076811759708816, 0.6444004775717707689, 0.5364919789714475140 ) ) ;
#48996=EDGE_LOOP ( 'NONE', ( #51929, #42933, #9851, #13448 ) ) ;
#48997=LINE ( 'NONE', #27143, #16341 ) ;
#48998=EDGE_CURVE ( 'NONE', #41994, #16631, #40560, .T. ) ;
#48999=ORIENTED_EDGE ( 'NONE', *, *, #21094, .T. ) ;
#49000=ADVANCED_FACE ( 'NONE', ( #32836 ), #54163, .F. ) ;
#49001=ORIENTED_EDGE ( 'NONE', *, *, #29648, .T. ) ;
#49002=ORIENTED_EDGE ( 'NONE', *, *, #8092, .T. ) ;
#49003=CARTESIAN_POINT ( 'NONE',  ( -13.94578152804187710, 0.000000000000000000, 5.081209898857876439 ) ) ;
#49004=VERTEX_POINT ( 'NONE', #49335 ) ;
#49005=ORIENTED_EDGE ( 'NONE', *, *, #49440, .T. ) ;
#49006=LINE ( 'NONE', #14932, #2995 ) ;
#49007=DIRECTION ( 'NONE',  ( -0.7660212471507179544, -0.6427876096865405842, -0.005961354470445141482 ) ) ;
#49008=ORIENTED_EDGE ( 'NONE', *, *, #40746, .F. ) ;
#49009=ADVANCED_FACE ( 'NONE', ( #41383 ), #2474, .F. ) ;
#49010=ORIENTED_EDGE ( 'NONE', *, *, #11307, .F. ) ;
#49011=LINE ( 'NONE', #44749, #12260 ) ;
#49012=VERTEX_POINT ( 'NONE', #27774 ) ;
#49014=EDGE_CURVE ( 'NONE', #44514, #40957, #19507, .T. ) ;
#49015=CARTESIAN_POINT ( 'NONE',  ( -28.93060053386082231, -0.1191753592594197858, 8.019254159017428663 ) ) ;
#49016=PLANE ( 'NONE',  #2185 ) ;
#49017=CARTESIAN_POINT ( 'NONE',  ( -26.13337879274045505, 0.000000000000000000, 6.833023547870798353 ) ) ;
#49018=CARTESIAN_POINT ( 'NONE',  ( -9.342070512798265725, 0.000000000000000000, 10.59882438848031505 ) ) ;
#49019=ORIENTED_EDGE ( 'NONE', *, *, #39929, .F. ) ;
#49020=DIRECTION ( 'NONE',  ( 0.7660212471507180654, -0.6427876096865404731, 0.005961354470445141482 ) ) ;
#49021=ORIENTED_EDGE ( 'NONE', *, *, #7854, .T. ) ;
#49022=DIRECTION ( 'NONE',  ( -0.6427681459581293666, -0.7660444431189770143, -0.005002170337467561935 ) ) ;
#49023=AXIS2_PLACEMENT_3D ( 'NONE', #28151, #10281, #49473 ) ;
#49024=LINE ( 'NONE', #10124, #53288 ) ;
#49026=FACE_OUTER_BOUND ( 'NONE', #9697, .T. ) ;
#49028=PLANE ( 'NONE',  #10497 ) ;
#49029=VERTEX_POINT ( 'NONE', #41082 ) ;
#49030=CARTESIAN_POINT ( 'NONE',  ( -12.07861178016168502, 0.000000000000000000, 3.987744436156619887 ) ) ;
#49031=ORIENTED_EDGE ( 'NONE', *, *, #17428, .F. ) ;
#49032=LINE ( 'NONE', #5893, #42838 ) ;
#49033=CARTESIAN_POINT ( 'NONE',  ( -18.33612970409028264, 0.000000000000000000, 6.155039403603081105 ) ) ;
#49034=PLANE ( 'NONE',  #50796 ) ;
#49035=EDGE_CURVE ( 'NONE', #17943, #45757, #40817, .T. ) ;
#49036=CARTESIAN_POINT ( 'NONE',  ( -25.20123094555300369, 0.000000000000000000, 6.470945668149052032 ) ) ;
#49037=DIRECTION ( 'NONE',  ( 0.6427681459581294776, -0.7660444431189769032, 0.005002170337467562802 ) ) ;
#49039=EDGE_CURVE ( 'NONE', #18181, #54123, #11262, .T. ) ;
#49040=EDGE_LOOP ( 'NONE', ( #25375, #51838, #35394, #50740 ) ) ;
#49041=EDGE_CURVE ( 'NONE', #18842, #32386, #36549, .T. ) ;
#49042=DIRECTION ( 'NONE',  ( -0.005961354470445682716, -0.6427876096865404731, 0.7660212471507180654 ) ) ;
#49043=DIRECTION ( 'NONE',  ( -0.7660212471507179544, -0.6427876096865405842, -0.005961354470445141482 ) ) ;
#49044=PLANE ( 'NONE',  #41784 ) ;
#49045=ADVANCED_FACE ( 'NONE', ( #14979 ), #45344, .F. ) ;
#49046=EDGE_CURVE ( 'NONE', #9899, #15809, #54411, .T. ) ;
#49047=EDGE_CURVE ( 'NONE', #24514, #13246, #50153, .T. ) ;
#49048=AXIS2_PLACEMENT_3D ( 'NONE', #3668, #46544, #51399 ) ;
#49049=CARTESIAN_POINT ( 'NONE',  ( -10.47421230394850866, 0.000000000000000000, 10.95934586908605723 ) ) ;
#49050=CARTESIAN_POINT ( 'NONE',  ( -16.81345671998191449, 0.000000000000000000, 3.412238694616132495 ) ) ;
#49051=CARTESIAN_POINT ( 'NONE',  ( -15.87975247367846166, 0.000000000000000000, 2.850166870931599927 ) ) ;
#49052=DIRECTION ( 'NONE',  ( 0.007781995580012663651, 0.000000000000000000, -0.9999697198139515519 ) ) ;
#49053=DIRECTION ( 'NONE',  ( 0.005002170337468016433, -0.7660444431189770143, -0.6427681459581293666 ) ) ;
#49054=LINE ( 'NONE', #19795, #6566 ) ;
#49055=EDGE_LOOP ( 'NONE', ( #46501, #20098, #52005, #37244 ) ) ;
#49056=VECTOR ( 'NONE', #45438, 1000.000000000000227 ) ;
#49057=EDGE_CURVE ( 'NONE', #33913, #24475, #47290, .T. ) ;
#49058=AXIS2_PLACEMENT_3D ( 'NONE', #32310, #48792, #14430 ) ;
#49059=ADVANCED_FACE ( 'NONE', ( #16349 ), #20890, .F. ) ;
#49060=ORIENTED_EDGE ( 'NONE', *, *, #5906, .F. ) ;
#49061=ORIENTED_EDGE ( 'NONE', *, *, #28706, .T. ) ;
#49062=ORIENTED_EDGE ( 'NONE', *, *, #53812, .T. ) ;
#49063=ADVANCED_FACE ( 'NONE', ( #55001 ), #29429, .F. ) ;
#49064=EDGE_LOOP ( 'NONE', ( #2074, #43070, #25569, #17738 ) ) ;
#49065=CARTESIAN_POINT ( 'NONE',  ( -15.87975247367846166, 0.000000000000000000, 2.850166870931599927 ) ) ;
#49066=DIRECTION ( 'NONE',  ( -0.005961354470445682716, -0.6427876096865404731, 0.7660212471507180654 ) ) ;
#49067=ADVANCED_FACE ( 'NONE', ( #4160 ), #37677, .F. ) ;
#49068=VERTEX_POINT ( 'NONE', #51573 ) ;
#49069=ORIENTED_EDGE ( 'NONE', *, *, #9891, .F. ) ;
#49070=ORIENTED_EDGE ( 'NONE', *, *, #9048, .T. ) ;
#49073=PLANE ( 'NONE',  #44016 ) ;
#49074=ORIENTED_EDGE ( 'NONE', *, *, #30660, .F. ) ;
#49075=FACE_OUTER_BOUND ( 'NONE', #27036, .T. ) ;
#49076=ORIENTED_EDGE ( 'NONE', *, *, #26905, .F. ) ;
#49077=VECTOR ( 'NONE', #52735, 999.9999999999998863 ) ;
#49078=AXIS2_PLACEMENT_3D ( 'NONE', #1081, #32046, #44530 ) ;
#49079=CARTESIAN_POINT ( 'NONE',  ( -13.50701111274833011, 0.000000000000000000, 8.408613139945765980 ) ) ;
#49080=CARTESIAN_POINT ( 'NONE',  ( -27.99767448711536133, 0.000000000000000000, 7.557179307314289218 ) ) ;
#49081=CARTESIAN_POINT ( 'NONE',  ( -15.89855235162775848, 0.4483081953215033444, 2.843166003391808694 ) ) ;
#49082=CARTESIAN_POINT ( 'NONE',  ( -14.86887539286270687, -2.784623065533160524, 2.568053214010371565 ) ) ;
#49083=DIRECTION ( 'NONE',  ( -0.6427681459581293666, -0.7660444431189770143, -0.005002170337467561935 ) ) ;
#49085=DIRECTION ( 'NONE',  ( 0.6427681459581294776, -0.7660444431189769032, 0.005002170337467562802 ) ) ;
#49086=ORIENTED_EDGE ( 'NONE', *, *, #37563, .T. ) ;
#49087=DIRECTION ( 'NONE',  ( 0.9999697198139515519, 0.000000000000000000, 0.007781995580013368816 ) ) ;
#49088=VERTEX_POINT ( 'NONE', #38214 ) ;
#49089=FACE_OUTER_BOUND ( 'NONE', #2457, .T. ) ;
#49090=DIRECTION ( 'NONE',  ( 0.007781995580012662783, 0.000000000000000000, -0.9999697198139514409 ) ) ;
#49091=CARTESIAN_POINT ( 'NONE',  ( -13.21650167832249245, 0.000000000000000000, 5.086885323277891224 ) ) ;
#49093=ADVANCED_FACE ( 'NONE', ( #8400 ), #50723, .F. ) ;
#49094=LINE ( 'NONE', #39758, #14155 ) ;
#49095=CARTESIAN_POINT ( 'NONE',  ( 1.086233639165236964, 0.000000000000000000, 2.796443541562362078 ) ) ;
#49097=VECTOR ( 'NONE', #23522, 1000.000000000000227 ) ;
#49098=DIRECTION ( 'NONE',  ( -0.5364919789714478471, 0.6444004775717705469, -0.5449076811759709926 ) ) ;
#49099=FILL_AREA_STYLE_COLOUR ( '', #24385 ) ;
#49100=CARTESIAN_POINT ( 'NONE',  ( -13.27065584551087163, 0.000000000000000000, 12.04557950825129176 ) ) ;
#49101=EDGE_LOOP ( 'NONE', ( #37390, #38239, #18552, #54939 ) ) ;
#49102=CARTESIAN_POINT ( 'NONE',  ( -13.00369386594929288, 0.000000000000000000, 3.441887150067862056 ) ) ;
#49103=CARTESIAN_POINT ( 'NONE',  ( -15.78652251423055830, -5.536956232915666298, 2.836684681291425925 ) ) ;
#49104=PLANE ( 'NONE',  #20961 ) ;
#49105=EDGE_CURVE ( 'NONE', #2279, #10471, #56116, .T. ) ;
#49106=CARTESIAN_POINT ( 'NONE',  ( -29.86274838104827367, -0.1191753592594197858, 8.381332038739175871 ) ) ;
#49107=ADVANCED_FACE ( 'NONE', ( #25190 ), #38805, .F. ) ;
#49108=EDGE_CURVE ( 'NONE', #42922, #18997, #47591, .T. ) ;
#49109=PLANE ( 'NONE',  #20937 ) ;
#49110=ADVANCED_FACE ( 'NONE', ( #43051 ), #46442, .F. ) ;
#49111=DIRECTION ( 'NONE',  ( 0.007781995580012663651, -3.146120232559066537E-19, -0.9999697198139514409 ) ) ;
#49112=VERTEX_POINT ( 'NONE', #17202 ) ;
#49113=ORIENTED_EDGE ( 'NONE', *, *, #37628, .T. ) ;
#49114=DIRECTION ( 'NONE',  ( 0.007781995580012662783, 0.000000000000000000, -0.9999697198139514409 ) ) ;
#49115=PLANE ( 'NONE',  #1438 ) ;
#49116=VECTOR ( 'NONE', #53582, 999.9999999999998863 ) ;
#49117=VECTOR ( 'NONE', #19116, 999.9999999999998863 ) ;
#49118=EDGE_LOOP ( 'NONE', ( #2379, #54231, #37460, #2418 ) ) ;
#49119=DIRECTION ( 'NONE',  ( 0.005002170337468016433, -0.7660444431189770143, -0.6427681459581293666 ) ) ;
#49120=ORIENTED_EDGE ( 'NONE', *, *, #13668, .F. ) ;
#49121=CARTESIAN_POINT ( 'NONE',  ( -18.67697421479882181, -0.1191753592594197858, 4.036397482078229793 ) ) ;
#49122=EDGE_CURVE ( 'NONE', #50938, #47628, #21486, .T. ) ;
#49123=ORIENTED_EDGE ( 'NONE', *, *, #51011, .T. ) ;
#49124=ORIENTED_EDGE ( 'NONE', *, *, #10122, .T. ) ;
#49125=VERTEX_POINT ( 'NONE', #16944 ) ;
#49126=EDGE_CURVE ( 'NONE', #49857, #39974, #47033, .T. ) ;
#49127=DIRECTION ( 'NONE',  ( 0.5449076811759707706, 0.6444004775717708799, -0.5364919789714476250 ) ) ;
#49128=DIRECTION ( 'NONE',  ( 0.000000000000000000, -0.000000000000000000, -1.000000000000000000 ) ) ;
#49129=DIRECTION ( 'NONE',  ( 0.000000000000000000, -0.000000000000000000, -1.000000000000000000 ) ) ;
#49131=CARTESIAN_POINT ( 'NONE',  ( -19.60990026154428278, 0.000000000000000000, 4.498472333781370125 ) ) ;
#49132=ORIENTED_EDGE ( 'NONE', *, *, #48083, .T. ) ;
#49133=VECTOR ( 'NONE', #39099, 1000.000000000000114 ) ;
#49135=EDGE_CURVE ( 'NONE', #53347, #46741, #24589, .T. ) ;
#49136=VECTOR ( 'NONE', #7448, 1000.000000000000227 ) ;
#49137=CARTESIAN_POINT ( 'NONE',  ( -21.47419595591918906, 0.000000000000000000, 5.222628093224860102 ) ) ;
#49138=ORIENTED_EDGE ( 'NONE', *, *, #46332, .T. ) ;
#49139=DIRECTION ( 'NONE',  ( 0.9999697198139515519, 0.000000000000000000, 0.007781995580013368816 ) ) ;
#49140=EDGE_LOOP ( 'NONE', ( #35214, #12084, #22519, #16306 ) ) ;
#49141=DIRECTION ( 'NONE',  ( -0.5364919789714478471, 0.6444004775717705469, -0.5449076811759709926 ) ) ;
#49142=DIRECTION ( 'NONE',  ( 0.000000000000000000, -0.000000000000000000, -1.000000000000000000 ) ) ;
#49143=ORIENTED_EDGE ( 'NONE', *, *, #31330, .T. ) ;
#49144=CARTESIAN_POINT ( 'NONE',  ( -17.73140113748535285, 0.000000000000000000, 13.85752530597602039 ) ) ;
#49145=ORIENTED_EDGE ( 'NONE', *, *, #31173, .F. ) ;
#49146=DIRECTION ( 'NONE',  ( 0.000000000000000000, -1.000000000000000000, 0.000000000000000000 ) ) ;
#49147=ORIENTED_EDGE ( 'NONE', *, *, #17132, .T. ) ;
#49148=CARTESIAN_POINT ( 'NONE',  ( -29.86352658060627618, 0.000000000000000000, 8.481329010720569883 ) ) ;
#49149=LINE ( 'NONE', #27585, #13982 ) ;
#49150=CARTESIAN_POINT ( 'NONE',  ( -22.09649345868086812, -4.727446477803164626, 5.313519283068141696 ) ) ;
#49151=EDGE_LOOP ( 'NONE', ( #21578, #3745, #9724, #18312 ) ) ;
#49152=CIRCLE ( 'NONE', #39185, 2.125000000000000000 ) ;
#49153=AXIS2_PLACEMENT_3D ( 'NONE', #42592, #54512, #3425 ) ;
#49154=CARTESIAN_POINT ( 'NONE',  ( -18.60652076397914811, 0.000000000000000000, 6.891599297466603602 ) ) ;
#49155=CARTESIAN_POINT ( 'NONE',  ( -22.78182334992371594, 5.305366725996514710, 5.361896619375292161 ) ) ;
#49156=DIRECTION ( 'NONE',  ( 0.005961354470445682716, -0.6427876096865404731, -0.7660212471507180654 ) ) ;
#49157=DIRECTION ( 'NONE',  ( 0.005002170337468016433, -0.7660444431189770143, -0.6427681459581293666 ) ) ;
#49158=FACE_OUTER_BOUND ( 'NONE', #36122, .T. ) ;
#49159=CARTESIAN_POINT ( 'NONE',  ( -14.69670185910160143, -4.241740624735665044, 2.454685487473226679 ) ) ;
#49161=AXIS2_PLACEMENT_3D ( 'NONE', #36670, #1995, #32671 ) ;
#49162=ORIENTED_EDGE ( 'NONE', *, *, #37010, .T. ) ;
#49163=DIRECTION ( 'NONE',  ( 0.007781995580012662783, 0.000000000000000000, -0.9999697198139514409 ) ) ;
#49166=VERTEX_POINT ( 'NONE', #20336 ) ;
#49167=LINE ( 'NONE', #36683, #53785 ) ;
#49168=LINE ( 'NONE', #11400, #14572 ) ;
#49169=ORIENTED_EDGE ( 'NONE', *, *, #397, .F. ) ;
#49170=EDGE_CURVE ( 'NONE', #48176, #6556, #7559, .T. ) ;
#49171=LINE ( 'NONE', #45464, #30405 ) ;
#49173=EDGE_CURVE ( 'NONE', #21011, #55542, #20641, .T. ) ;
#49174=EDGE_CURVE ( 'NONE', #38344, #25308, #18612, .T. ) ;
#49175=CARTESIAN_POINT ( 'NONE',  ( -15.56870600992515108, 0.6102101463440035012, 2.709876962758211771 ) ) ;
#49176=DIRECTION ( 'NONE',  ( 0.000000000000000000, -1.000000000000000000, 0.000000000000000000 ) ) ;
#49177=VERTEX_POINT ( 'NONE', #35649 ) ;
#49178=ORIENTED_EDGE ( 'NONE', *, *, #33640, .F. ) ;
#49179=LINE ( 'NONE', #54012, #35020 ) ;
#49181=DIRECTION ( 'NONE',  ( -0.005961354470445682716, -0.6427876096865404731, 0.7660212471507180654 ) ) ;
#49182=CARTESIAN_POINT ( 'NONE',  ( -16.81267852042391198, -0.1191753592594197858, 3.312241722634738039 ) ) ;
#49183=EDGE_LOOP ( 'NONE', ( #47112, #49138, #43305, #23552 ) ) ;
#49184=DIRECTION ( 'NONE',  ( 0.007781995580012663651, -3.146120232559066537E-19, -0.9999697198139514409 ) ) ;
#49185=VECTOR ( 'NONE', #23147, 1000.000000000000227 ) ;
#49186=ORIENTED_EDGE ( 'NONE', *, *, #8094, .T. ) ;
#49187=DIRECTION ( 'NONE',  ( 0.000000000000000000, 0.000000000000000000, 1.000000000000000000 ) ) ;
#49188=DIRECTION ( 'NONE',  ( 0.7660212471507180654, -0.6427876096865404731, 0.005961354470445141482 ) ) ;
#49189=ORIENTED_EDGE ( 'NONE', *, *, #19798, .T. ) ;
#49190=DIRECTION ( 'NONE',  ( 0.005961354470445682716, -0.6427876096865404731, -0.7660212471507180654 ) ) ;
#49191=AXIS2_PLACEMENT_3D ( 'NONE', #8663, #15450, #41582 ) ;
#49192=CARTESIAN_POINT ( 'NONE',  ( -11.73774248290225408, -0.1191753592594185784, 7.045056746410134352 ) ) ;
#49193=PLANE ( 'NONE',  #25775 ) ;
#49194=ORIENTED_EDGE ( 'NONE', *, *, #22506, .F. ) ;
#49195=VECTOR ( 'NONE', #37679, 999.9999999999998863 ) ;
#49196=VECTOR ( 'NONE', #47644, 1000.000000000000227 ) ;
#49197=CARTESIAN_POINT ( 'NONE',  ( -15.12932141704740197, -3.594132820645660420, 8.457258234613435732 ) ) ;
#49198=ORIENTED_EDGE ( 'NONE', *, *, #22764, .F. ) ;
#49199=EDGE_CURVE ( 'NONE', #8011, #51712, #13514, .T. ) ;
#49200=ORIENTED_EDGE ( 'NONE', *, *, #14407, .F. ) ;
#49201=VECTOR ( 'NONE', #216, 999.9999999999998863 ) ;
#49202=ORIENTED_EDGE ( 'NONE', *, *, #46659, .F. ) ;
#49203=CARTESIAN_POINT ( 'NONE',  ( -13.73672976910459909, 0.000000000000000000, 12.22661844811216270 ) ) ;
#49204=AXIS2_PLACEMENT_3D ( 'NONE', #41136, #19264, #54743 ) ;
#49205=EDGE_CURVE ( 'NONE', #43426, #55768, #26857, .T. ) ;
#49206=VERTEX_POINT ( 'NONE', #44180 ) ;
#49207=DIRECTION ( 'NONE',  ( 0.5449076811759707706, 0.6444004775717708799, -0.5364919789714476250 ) ) ;
#49208=EDGE_CURVE ( 'NONE', #16314, #29707, #34807, .T. ) ;
#49209=VERTEX_POINT ( 'NONE', #40182 ) ;
#49210=DIRECTION ( 'NONE',  ( 0.6427681459581294776, -0.7660444431189769032, 0.005002170337467562802 ) ) ;
#49211=DIRECTION ( 'NONE',  ( 0.005961354470445682716, -0.6427876096865404731, -0.7660212471507180654 ) ) ;
#49212=ORIENTED_EDGE ( 'NONE', *, *, #17842, .T. ) ;
#49213=EDGE_CURVE ( 'NONE', #35002, #8314, #52418, .T. ) ;
#49214=DIRECTION ( 'NONE',  ( 0.6427681459581294776, -0.7660444431189769032, 0.005002170337467562802 ) ) ;
#49215=AXIS2_PLACEMENT_3D ( 'NONE', #34020, #29477, #46797 ) ;
#49216=ORIENTED_EDGE ( 'NONE', *, *, #14912, .T. ) ;
#49217=AXIS2_PLACEMENT_3D ( 'NONE', #34144, #38683, #38951 ) ;
#49218=FACE_OUTER_BOUND ( 'NONE', #51539, .T. ) ;
#49219=CARTESIAN_POINT ( 'NONE',  ( -11.20636620717317378, 0.000000000000000000, 11.32298014792380414 ) ) ;
#49220=CARTESIAN_POINT ( 'NONE',  ( -6.646477795989845561, 6.490377269657392922, 5.800091266962301262 ) ) ;
#49221=DIRECTION ( 'NONE',  ( 0.5449076811759707706, 0.6444004775717708799, -0.5364919789714476250 ) ) ;
#49223=LINE ( 'NONE', #10048, #16480 ) ;
#49224=LINE ( 'NONE', #18577, #3891 ) ;
#49225=ORIENTED_EDGE ( 'NONE', *, *, #33533, .T. ) ;
#49226=AXIS2_PLACEMENT_3D ( 'NONE', #45315, #20300, #3273 ) ;
#49227=ORIENTED_EDGE ( 'NONE', *, *, #5359, .F. ) ;
#49228=FACE_OUTER_BOUND ( 'NONE', #10934, .T. ) ;
#49229=FACE_OUTER_BOUND ( 'NONE', #31888, .T. ) ;
#49230=VECTOR ( 'NONE', #12797, 999.9999999999998863 ) ;
#49231=DIRECTION ( 'NONE',  ( -0.9999697198139514409, -0.000000000000000000, -0.007781995580013368816 ) ) ;
#49232=CYLINDRICAL_SURFACE ( 'NONE', #44905, 2.125000000000000000 ) ;
#49233=ORIENTED_EDGE ( 'NONE', *, *, #52873, .T. ) ;
#49234=CARTESIAN_POINT ( 'NONE',  ( -9.342070512798265725, 0.000000000000000000, 10.59882438848031505 ) ) ;
#49235=CARTESIAN_POINT ( 'NONE',  ( -14.14002736499410062, 0.000000000000000000, 4.341034093226343593 ) ) ;
#49236=ORIENTED_EDGE ( 'NONE', *, *, #40650, .F. ) ;
#49237=VECTOR ( 'NONE', #3093, 999.9999999999998863 ) ;
#49238=DIRECTION ( 'NONE',  ( -0.6427681459581293666, -0.7660444431189770143, -0.005002170337467561935 ) ) ;
#49239=EDGE_CURVE ( 'NONE', #19103, #904, #39065, .T. ) ;
#49241=ORIENTED_EDGE ( 'NONE', *, *, #13460, .T. ) ;
#49242=VECTOR ( 'NONE', #11599, 1000.000000000000114 ) ;
#49243=VECTOR ( 'NONE', #22304, 999.9999999999998863 ) ;
#49245=LINE ( 'NONE', #18295, #43263 ) ;
#49246=LINE ( 'NONE', #15434, #46774 ) ;
#49247=EDGE_CURVE ( 'NONE', #485, #2953, #48724, .T. ) ;
#49248=EDGE_CURVE ( 'NONE', #44511, #12432, #9825, .T. ) ;
#49249=DIRECTION ( 'NONE',  ( 0.007781995580012663651, -3.146120232559066537E-19, -0.9999697198139514409 ) ) ;
#49250=DIRECTION ( 'NONE',  ( 0.005002170337468016433, -0.7660444431189770143, -0.6427681459581293666 ) ) ;
#49251=ORIENTED_EDGE ( 'NONE', *, *, #16702, .F. ) ;
#49252=AXIS2_PLACEMENT_3D ( 'NONE', #13177, #25972, #47232 ) ;
#49253=VECTOR ( 'NONE', #45080, 999.9999999999998863 ) ;
#49254=ORIENTED_EDGE ( 'NONE', *, *, #44272, .T. ) ;
#49255=CARTESIAN_POINT ( 'NONE',  ( -29.86197018149027116, 0.000000000000000000, 8.281335066757780083 ) ) ;
#49257=LINE ( 'NONE', #15199, #10677 ) ;
#49258=DIRECTION ( 'NONE',  ( 0.5364919789714477361, 0.6444004775717706579, 0.5449076811759711036 ) ) ;
#49259=VECTOR ( 'NONE', #12454, 1000.000000000000000 ) ;
#49260=DIRECTION ( 'NONE',  ( -0.5364919789714478471, 0.6444004775717705469, -0.5449076811759709926 ) ) ;
#49261=ORIENTED_EDGE ( 'NONE', *, *, #20488, .F. ) ;
#49263=VECTOR ( 'NONE', #50683, 1000.000000000000227 ) ;
#49264=CARTESIAN_POINT ( 'NONE',  ( -14.94916102560700821, 0.000000000000000000, 2.688082935172642962 ) ) ;
#49265=ADVANCED_FACE ( 'NONE', ( #53275 ), #31408, .F. ) ;
#49266=CARTESIAN_POINT ( 'NONE',  ( -7.020097852742797073, 1.644072297827783524, 8.920596959107028212 ) ) ;
#49267=CARTESIAN_POINT ( 'NONE',  ( -18.36642663825911015, 0.000000000000000000, 10.04813038014351356 ) ) ;
#49268=ORIENTED_EDGE ( 'NONE', *, *, #13043, .F. ) ;
#49269=DIRECTION ( 'NONE',  ( 0.5364919789714477361, 0.6444004775717706579, 0.5449076811759711036 ) ) ;
#49270=ORIENTED_EDGE ( 'NONE', *, *, #39371, .T. ) ;
#49271=FACE_OUTER_BOUND ( 'NONE', #12257, .T. ) ;
#49273=AXIS2_PLACEMENT_3D ( 'NONE', #25686, #47845, #34484 ) ;
#49274=CARTESIAN_POINT ( 'NONE',  ( -13.04471763214503000, 0.9340140483890038148, 1.719143122047526395 ) ) ;
#49275=ORIENTED_EDGE ( 'NONE', *, *, #41083, .T. ) ;
#49276=DIRECTION ( 'NONE',  ( -0.9999697198139514409, -0.000000000000000000, -0.007781995580013368816 ) ) ;
#49278=ORIENTED_EDGE ( 'NONE', *, *, #17496, .T. ) ;
#49279=ORIENTED_EDGE ( 'NONE', *, *, #30412, .T. ) ;
#49280=ORIENTED_EDGE ( 'NONE', *, *, #2500, .F. ) ;
#49281=DIRECTION ( 'NONE',  ( -0.6427681459581293666, -0.7660444431189770143, -0.005002170337467561935 ) ) ;
#49282=ORIENTED_EDGE ( 'NONE', *, *, #34618, .T. ) ;
#49283=ORIENTED_EDGE ( 'NONE', *, *, #16493, .T. ) ;
#49284=VECTOR ( 'NONE', #18546, 999.9999999999998863 ) ;
#49285=CARTESIAN_POINT ( 'NONE',  ( 2.072287782118878319, 0.000000000000000000, -2.950529333540147015 ) ) ;
#49286=CARTESIAN_POINT ( 'NONE',  ( -16.53317331066696383, 0.000000000000000000, 13.31285208727739899 ) ) ;
#49287=VERTEX_POINT ( 'NONE', #48131 ) ;
#49288=VECTOR ( 'NONE', #6788, 1000.000000000000227 ) ;
#49289=VERTEX_POINT ( 'NONE', #4994 ) ;
#49290=CARTESIAN_POINT ( 'NONE',  ( -19.60834386242827776, 0.000000000000000000, 4.298478389818581213 ) ) ;
#49292=ORIENTED_EDGE ( 'NONE', *, *, #53313, .F. ) ;
#49293=VERTEX_POINT ( 'NONE', #43348 ) ;
#49294=AXIS2_PLACEMENT_3D ( 'NONE', #26169, #13403, #55695 ) ;
#49296=CARTESIAN_POINT ( 'NONE',  ( -11.87243407472968926, 0.000000000000000000, 11.50246268866867361 ) ) ;
#49297=CYLINDRICAL_SURFACE ( 'NONE', #51160, 6.999999999999988454 ) ;
#49298=DIRECTION ( 'NONE',  ( -0.005961354470445682716, -0.6427876096865404731, 0.7660212471507180654 ) ) ;
#49299=CARTESIAN_POINT ( 'NONE',  ( -27.99767448711536133, 0.000000000000000000, 7.557179307314289218 ) ) ;
#49300=ORIENTED_EDGE ( 'NONE', *, *, #21401, .F. ) ;
#49301=LINE ( 'NONE', #45584, #23758 ) ;
#49302=ORIENTED_EDGE ( 'NONE', *, *, #43166, .T. ) ;
#49303=EDGE_CURVE ( 'NONE', #19083, #17592, #4441, .T. ) ;
#49304=LINE ( 'NONE', #40534, #19385 ) ;
#49305=ADVANCED_FACE ( 'NONE', ( #22323 ), #48420, .F. ) ;
#49306=EDGE_CURVE ( 'NONE', #36934, #12677, #39651, .T. ) ;
#49307=LINE ( 'NONE', #5882, #44152 ) ;
#49308=CARTESIAN_POINT ( 'NONE',  ( -1.086233639165236964, 0.000000000000000000, -2.796443541562362078 ) ) ;
#49309=DIRECTION ( 'NONE',  ( 0.007781995580012662783, 0.000000000000000000, -0.9999697198139514409 ) ) ;
#49310=AXIS2_PLACEMENT_3D ( 'NONE', #23926, #54041, #2617 ) ;
#49311=LINE ( 'NONE', #18947, #14866 ) ;
#49312=DIRECTION ( 'NONE',  ( 0.007781995580012663651, 0.000000000000000000, -0.9999697198139515519 ) ) ;
#49313=ORIENTED_EDGE ( 'NONE', *, *, #21807, .F. ) ;
#49314=DIRECTION ( 'NONE',  ( 0.6427681459581294776, -0.7660444431189769032, 0.005002170337467562802 ) ) ;
#49315=EDGE_CURVE ( 'NONE', #54647, #19170, #17475, .T. ) ;
#49316=AXIS2_PLACEMENT_3D ( 'NONE', #21785, #767, #5041 ) ;
#49317=ORIENTED_EDGE ( 'NONE', *, *, #17818, .T. ) ;
#49319=FACE_OUTER_BOUND ( 'NONE', #1954, .T. ) ;
#49322=VECTOR ( 'NONE', #48470, 999.9999999999998863 ) ;
#49323=CARTESIAN_POINT ( 'NONE',  ( -10.88625143271721996, 0.000000000000000000, 4.197029716307435265 ) ) ;
#49324=ADVANCED_FACE ( 'NONE', ( #47880 ), #26283, .F. ) ;
#49325=FACE_OUTER_BOUND ( 'NONE', #8333, .T. ) ;
#49326=PLANE ( 'NONE',  #43850 ) ;
#49327=ORIENTED_EDGE ( 'NONE', *, *, #46153, .T. ) ;
#49328=AXIS2_PLACEMENT_3D ( 'NONE', #42067, #29290, #7424 ) ;
#49329=DIRECTION ( 'NONE',  ( -0.005961354470445682716, -0.6427876096865404731, 0.7660212471507180654 ) ) ;
#49330=FACE_OUTER_BOUND ( 'NONE', #8145, .T. ) ;
#49331=FACE_OUTER_BOUND ( 'NONE', #40939, .T. ) ;
#49332=VECTOR ( 'NONE', #36591, 999.9999999999998863 ) ;
#49333=EDGE_CURVE ( 'NONE', #27150, #621, #731, .T. ) ;
#49334=LINE ( 'NONE', #23499, #52721 ) ;
#49335=CARTESIAN_POINT ( 'NONE',  ( 3.882677180727608590, -1.000000000000000000, 1.710209902397122672 ) ) ;
#49336=LINE ( 'NONE', #6734, #2036 ) ;
#49337=EDGE_CURVE ( 'NONE', #42498, #21652, #36475, .T. ) ;
#49338=VECTOR ( 'NONE', #2243, 999.9999999999998863 ) ;
#49339=VECTOR ( 'NONE', #14616, 999.9999999999998863 ) ;
#49341=CARTESIAN_POINT ( 'NONE',  ( -23.33849165029409889, 0.000000000000000000, 5.946783852668351855 ) ) ;
#49342=ORIENTED_EDGE ( 'NONE', *, *, #26541, .F. ) ;
#49343=AXIS2_PLACEMENT_3D ( 'NONE', #44468, #5573, #18652 ) ;
#49344=ORIENTED_EDGE ( 'NONE', *, *, #42546, .T. ) ;
#49345=ORIENTED_EDGE ( 'NONE', *, *, #32752, .T. ) ;
#49346=ORIENTED_EDGE ( 'NONE', *, *, #23312, .T. ) ;
#49347=VECTOR ( 'NONE', #21892, 999.9999999999998863 ) ;
#49348=ORIENTED_EDGE ( 'NONE', *, *, #11175, .T. ) ;
#49349=CARTESIAN_POINT ( 'NONE',  ( -10.84028925556084388, -0.1191753592594197858, 11.14116300850493246 ) ) ;
#49350=LINE ( 'NONE', #27795, #9475 ) ;
#49351=AXIS2_PLACEMENT_3D ( 'NONE', #48390, #27667, #19123 ) ;
#49352=ORIENTED_EDGE ( 'NONE', *, *, #45467, .T. ) ;
#49353=ORIENTED_EDGE ( 'NONE', *, *, #20124, .T. ) ;
#49354=EDGE_CURVE ( 'NONE', #27552, #43561, #10372, .T. ) ;
#49355=ORIENTED_EDGE ( 'NONE', *, *, #6917, .F. ) ;
#49356=AXIS2_PLACEMENT_3D ( 'NONE', #34607, #17036, #3953 ) ;
#49358=AXIS2_PLACEMENT_3D ( 'NONE', #6275, #50244, #1709 ) ;
#49359=DIRECTION ( 'NONE',  ( 0.9999697198139515519, 0.000000000000000000, 0.007781995580013368816 ) ) ;
#49360=CARTESIAN_POINT ( 'NONE',  ( -17.71921124711865048, 0.9340140483890049250, 5.296940688622762572 ) ) ;
#49361=VERTEX_POINT ( 'NONE', #10673 ) ;
#49362=LINE ( 'NONE', #1660, #10149 ) ;
#49363=ADVANCED_FACE ( 'NONE', ( #36778 ), #2664, .F. ) ;
#49364=EDGE_CURVE ( 'NONE', #53438, #44267, #15203, .T. ) ;
#49365=VECTOR ( 'NONE', #15842, 999.9999999999998863 ) ;
#49366=ORIENTED_EDGE ( 'NONE', *, *, #30532, .T. ) ;
#49367=CARTESIAN_POINT ( 'NONE',  ( -14.14445781761538790, 0.000000000000000000, 4.910337740446896859 ) ) ;
#49368=PLANE ( 'NONE',  #48368 ) ;
#49369=EDGE_CURVE ( 'NONE', #10323, #6907, #54353, .T. ) ;
#49370=AXIS2_PLACEMENT_3D ( 'NONE', #3854, #34520, #29134 ) ;
#49371=CARTESIAN_POINT ( 'NONE',  ( -17.67149886328640918, 0.000000000000000000, 6.160211714487092927 ) ) ;
#49372=CARTESIAN_POINT ( 'NONE',  ( -14.00280974873554030, 0.000000000000000000, 12.40921378708904044 ) ) ;
#49373=AXIS2_PLACEMENT_3D ( 'NONE', #25376, #7791, #20824 ) ;
#49374=CARTESIAN_POINT ( 'NONE',  ( -27.06708303904391144, 0.000000000000000000, 7.395095371555332697 ) ) ;
#49375=DIRECTION ( 'NONE',  ( 0.6427681459581294776, -0.7660444431189769032, 0.005002170337467562802 ) ) ;
#49376=DIRECTION ( 'NONE',  ( 0.6427681459581294776, -0.7660444431189769032, 0.005002170337467562802 ) ) ;
#49377=VERTEX_POINT ( 'NONE', #27700 ) ;
#49378=DIRECTION ( 'NONE',  ( -0.9999697198139514409, -0.000000000000000000, -0.007781995580013368816 ) ) ;
#49379=ORIENTED_EDGE ( 'NONE', *, *, #17643, .T. ) ;
#49380=DIRECTION ( 'NONE',  ( 0.005961354470445682716, -0.6427876096865404731, -0.7660212471507180654 ) ) ;
#49381=LINE ( 'NONE', #11315, #43172 ) ;
#49382=DIRECTION ( 'NONE',  ( 0.005002170337468016433, -0.7660444431189770143, -0.6427681459581293666 ) ) ;
#49383=EDGE_CURVE ( 'NONE', #6267, #54772, #15447, .T. ) ;
#49384=CARTESIAN_POINT ( 'NONE',  ( -18.39746900504187010, 0.000000000000000000, 14.03700784672088808 ) ) ;
#49385=DIRECTION ( 'NONE',  ( 0.005961354470445682716, -0.6427876096865404731, -0.7660212471507180654 ) ) ;
#49386=PLANE ( 'NONE',  #52122 ) ;
#49387=FACE_OUTER_BOUND ( 'NONE', #6323, .T. ) ;
#49388=EDGE_CURVE ( 'NONE', #43351, #17276, #19984, .T. ) ;
#49389=AXIS2_PLACEMENT_3D ( 'NONE', #44012, #12596, #28353 ) ;
#49390=DIRECTION ( 'NONE',  ( 0.007781995580012662783, 0.000000000000000000, -0.9999697198139514409 ) ) ;
#49391=VECTOR ( 'NONE', #50229, 1000.000000000000000 ) ;
#49392=DIRECTION ( 'NONE',  ( 0.7660212471507180654, -0.6427876096865404731, 0.005961354470445141482 ) ) ;
#49394=LINE ( 'NONE', #1408, #11226 ) ;
#49395=CARTESIAN_POINT ( 'NONE',  ( -8.470913937488239398, -0.1191753592594177180, 5.223819612497378806 ) ) ;
#49396=DIRECTION ( 'NONE',  ( 0.7660212471507180654, -0.6427876096865404731, 0.005961354470445141482 ) ) ;
#49397=VECTOR ( 'NONE', #53375, 1000.000000000000227 ) ;
#49399=EDGE_CURVE ( 'NONE', #54019, #29728, #11192, .T. ) ;
#49400=LINE ( 'NONE', #10518, #22777 ) ;
#49401=VECTOR ( 'NONE', #22972, 1000.000000000000227 ) ;
#49402=LINE ( 'NONE', #24125, #356 ) ;
#49403=DIRECTION ( 'NONE',  ( 0.5364919789714477361, 0.6444004775717706579, 0.5449076811759711036 ) ) ;
#49404=CARTESIAN_POINT ( 'NONE',  ( -16.33815322254335456, -3.917936722690661178, 9.458226927869903378 ) ) ;
#49405=VERTEX_POINT ( 'NONE', #32518 ) ;
#49406=AXIS2_PLACEMENT_3D ( 'NONE', #27670, #6637, #32498 ) ;
#49407=ORIENTED_EDGE ( 'NONE', *, *, #9110, .T. ) ;
#49408=LINE ( 'NONE', #40880, #45028 ) ;
#49409=VECTOR ( 'NONE', #44743, 999.9999999999998863 ) ;
#49410=DIRECTION ( 'NONE',  ( 0.005002170337468016433, -0.7660444431189770143, -0.6427681459581293666 ) ) ;
#49411=VECTOR ( 'NONE', #19006, 999.9999999999998863 ) ;
#49412=ORIENTED_EDGE ( 'NONE', *, *, #1235, .F. ) ;
#49413=DIRECTION ( 'NONE',  ( 0.007781995580012663651, -3.146120232559066537E-19, -0.9999697198139514409 ) ) ;
#49414=ORIENTED_EDGE ( 'NONE', *, *, #52843, .T. ) ;
#49415=CARTESIAN_POINT ( 'NONE',  ( -12.13851405436063047, 0.000000000000000000, 11.68505802764555135 ) ) ;
#49416=VECTOR ( 'NONE', #28234, 1000.000000000000227 ) ;
#49417=ORIENTED_EDGE ( 'NONE', *, *, #22344, .T. ) ;
#49418=VECTOR ( 'NONE', #43570, 999.9999999999998863 ) ;
#49419=ORIENTED_EDGE ( 'NONE', *, *, #52504, .T. ) ;
#49420=EDGE_LOOP ( 'NONE', ( #24248, #21893, #12111, #16657 ) ) ;
#49422=PLANE ( 'NONE',  #43191 ) ;
#49423=DIRECTION ( 'NONE',  ( -0.005002170337468016433, -0.7660444431189770143, 0.6427681459581293666 ) ) ;
#49424=EDGE_CURVE ( 'NONE', #41786, #32587, #49820, .T. ) ;
#49425=ORIENTED_EDGE ( 'NONE', *, *, #9583, .F. ) ;
#49426=EDGE_CURVE ( 'NONE', #46034, #32323, #45839, .T. ) ;
#49427=ORIENTED_EDGE ( 'NONE', *, *, #1443, .T. ) ;
#49428=AXIS2_PLACEMENT_3D ( 'NONE', #22854, #54089, #28229 ) ;
#49429=DIRECTION ( 'NONE',  ( -0.7660212471507179544, -0.6427876096865405842, -0.005961354470445141482 ) ) ;
#49430=VECTOR ( 'NONE', #8157, 1000.000000000000227 ) ;
#49431=ORIENTED_EDGE ( 'NONE', *, *, #10640, .T. ) ;
#49432=EDGE_CURVE ( 'NONE', #27005, #39305, #49563, .T. ) ;
#49433=DIRECTION ( 'NONE',  ( 0.000000000000000000, -1.000000000000000000, 0.000000000000000000 ) ) ;
#49434=ORIENTED_EDGE ( 'NONE', *, *, #40845, .T. ) ;
#49435=AXIS2_PLACEMENT_3D ( 'NONE', #23673, #6373, #2080 ) ;
#49436=DIRECTION ( 'NONE',  ( -0.5449076811759708816, 0.6444004775717707689, 0.5364919789714475140 ) ) ;
#49437=DIRECTION ( 'NONE',  ( 0.9999697198139515519, 0.000000000000000000, 0.007781995580013368816 ) ) ;
#49438=EDGE_CURVE ( 'NONE', #21318, #38106, #6964, .T. ) ;
#49439=EDGE_CURVE ( 'NONE', #18068, #48023, #24271, .T. ) ;
#49440=EDGE_CURVE ( 'NONE', #47558, #37012, #23439, .T. ) ;
#49441=ORIENTED_EDGE ( 'NONE', *, *, #24597, .F. ) ;
#49442=LINE ( 'NONE', #18489, #41301 ) ;
#49443=VECTOR ( 'NONE', #13554, 1000.000000000000227 ) ;
#49445=CARTESIAN_POINT ( 'NONE',  ( -16.79925329029790149, 0.000000000000000000, 13.49544742625427496 ) ) ;
#49446=VECTOR ( 'NONE', #40990, 1000.000000000000227 ) ;
#49447=ORIENTED_EDGE ( 'NONE', *, *, #30429, .F. ) ;
#49448=LINE ( 'NONE', #50266, #35831 ) ;
#49449=CARTESIAN_POINT ( 'NONE',  ( -13.56180142820320711, -0.1191753592594188560, 2.598876660244924697 ) ) ;
#49450=AXIS2_PLACEMENT_3D ( 'NONE', #12639, #34771, #25688 ) ;
#49451=CARTESIAN_POINT ( 'NONE',  ( -19.34018785077573455, 2.876837460659008361, 4.102531311383550872 ) ) ;
#49452=ORIENTED_EDGE ( 'NONE', *, *, #14484, .F. ) ;
#49453=VECTOR ( 'NONE', #1629, 999.9999999999998863 ) ;
#49454=VECTOR ( 'NONE', #30084, 1000.000000000000227 ) ;
#49455=DIRECTION ( 'NONE',  ( 0.007781995580012663651, -3.146120232559066537E-19, -0.9999697198139514409 ) ) ;
#49456=DIRECTION ( 'NONE',  ( -0.005002170337468016433, -0.7660444431189770143, 0.6427681459581293666 ) ) ;
#49457=CARTESIAN_POINT ( 'NONE',  ( -19.60990026154428278, 0.000000000000000000, 4.498472333781370125 ) ) ;
#49458=EDGE_CURVE ( 'NONE', #50643, #46950, #6662, .T. ) ;
#49459=DIRECTION ( 'NONE',  ( -0.6427681459581293666, -0.7660444431189770143, -0.005002170337467561935 ) ) ;
#49460=DIRECTION ( 'NONE',  ( 0.9999697198139515519, 0.000000000000000000, 0.007781995580013368816 ) ) ;
#49461=FACE_OUTER_BOUND ( 'NONE', #24832, .T. ) ;
#49462=AXIS2_PLACEMENT_3D ( 'NONE', #33684, #30284, #24898 ) ;
#49463=EDGE_CURVE ( 'NONE', #345, #36408, #2402, .T. ) ;
#49464=AXIS2_PLACEMENT_3D ( 'NONE', #38414, #16854, #32144 ) ;
#49466=ORIENTED_EDGE ( 'NONE', *, *, #12437, .F. ) ;
#49467=CARTESIAN_POINT ( 'NONE',  ( -9.908141408373387193, -0.1191753592594197858, 10.77908512878318703 ) ) ;
#49468=DIRECTION ( 'NONE',  ( 0.5449076811759707706, 0.6444004775717708799, -0.5364919789714476250 ) ) ;
#49469=EDGE_CURVE ( 'NONE', #8976, #42837, #10083, .T. ) ;
#49471=VERTEX_POINT ( 'NONE', #25123 ) ;
#49472=CARTESIAN_POINT ( 'NONE',  ( -27.99923088623136636, 0.000000000000000000, 7.757173251277078130 ) ) ;
#49473=DIRECTION ( 'NONE',  ( 0.6427681459581294776, -0.7660444431189769032, 0.005002170337467562802 ) ) ;
#49474=EDGE_CURVE ( 'NONE', #12755, #33580, #56056, .T. ) ;
#49475=CARTESIAN_POINT ( 'NONE',  ( -19.12962290826653700, 0.000000000000000000, 14.40064212555863854 ) ) ;
#49476=FACE_OUTER_BOUND ( 'NONE', #15920, .T. ) ;
#49478=DIRECTION ( 'NONE',  ( 0.000000000000000000, -0.000000000000000000, -1.000000000000000000 ) ) ;
#49479=VECTOR ( 'NONE', #2598, 1000.000000000000227 ) ;
#49480=ORIENTED_EDGE ( 'NONE', *, *, #55513, .T. ) ;
#49481=ORIENTED_EDGE ( 'NONE', *, *, #3546, .F. ) ;
#49482=VECTOR ( 'NONE', #18175, 999.9999999999998863 ) ;
#49483=CARTESIAN_POINT ( 'NONE',  ( 2.072287782118878319, 0.000000000000000000, -2.950529333540147015 ) ) ;
#49484=CARTESIAN_POINT ( 'NONE',  ( -18.76354595665420177, -0.1191753592594177458, 14.21882498613976331 ) ) ;
#49485=VECTOR ( 'NONE', #40234, 1000.000000000000227 ) ;
#49486=DIRECTION ( 'NONE',  ( 0.005002170337468016433, -0.7660444431189770143, -0.6427681459581293666 ) ) ;
#49487=ORIENTED_EDGE ( 'NONE', *, *, #52504, .F. ) ;
#49488=DIRECTION ( 'NONE',  ( 0.2426528472758541499, 0.7422098413412800966, 0.6246952433987894571 ) ) ;
#49489=ORIENTED_EDGE ( 'NONE', *, *, #20055, .T. ) ;
#49491=VECTOR ( 'NONE', #52920, 999.9999999999998863 ) ;
#49492=VECTOR ( 'NONE', #17228, 1000.000000000000227 ) ;
#49493=VERTEX_POINT ( 'NONE', #51516 ) ;
#49494=PLANE ( 'NONE',  #3882 ) ;
#49495=CARTESIAN_POINT ( 'NONE',  ( -9.309591119262865533, 0.000000000000000000, 6.425292070274053913 ) ) ;
#49496=CARTESIAN_POINT ( 'NONE',  ( -20.54049170961573267, 0.000000000000000000, 4.660556269540326646 ) ) ;
#49497=AXIS2_PLACEMENT_3D ( 'NONE', #5530, #31394, #4690 ) ;
#49498=ORIENTED_EDGE ( 'NONE', *, *, #18343, .F. ) ;
#49499=VECTOR ( 'NONE', #35689, 1000.000000000000000 ) ;
#49500=CARTESIAN_POINT ( 'NONE',  ( -11.87243407472968926, 0.000000000000000000, 11.50246268866867361 ) ) ;
#49501=VECTOR ( 'NONE', #28096, 999.9999999999998863 ) ;
#49502=ORIENTED_EDGE ( 'NONE', *, *, #241, .F. ) ;
#49503=VECTOR ( 'NONE', #8930, 1000.000000000000114 ) ;
#49504=ORIENTED_EDGE ( 'NONE', *, *, #20470, .T. ) ;
#49505=VECTOR ( 'NONE', #16340, 1000.000000000000000 ) ;
#49506=ORIENTED_EDGE ( 'NONE', *, *, #10139, .T. ) ;
#49507=CARTESIAN_POINT ( 'NONE',  ( -9.208861310085005414, 0.000000000000000000, 6.795408042747278721 ) ) ;
#49508=VERTEX_POINT ( 'NONE', #12610 ) ;
#49509=DIRECTION ( 'NONE',  ( 0.000000000000000000, -0.000000000000000000, -1.000000000000000000 ) ) ;
#49510=VERTEX_POINT ( 'NONE', #42430 ) ;
#49511=CARTESIAN_POINT ( 'NONE',  ( -13.94158982014731585, 0.000000000000000000, 4.542584436305137530 ) ) ;
#49512=CARTESIAN_POINT ( 'NONE',  ( -13.08486533123210194, 0.000000000000000000, 1.963927175729152541 ) ) ;
#49514=EDGE_CURVE ( 'NONE', #5690, #24397, #38434, .T. ) ;
#49515=ORIENTED_EDGE ( 'NONE', *, *, #21811, .T. ) ;
#49516=FACE_OUTER_BOUND ( 'NONE', #25124, .T. ) ;
#49517=ORIENTED_EDGE ( 'NONE', *, *, #43340, .F. ) ;
#49518=EDGE_CURVE ( 'NONE', #21707, #51781, #8332, .T. ) ;
#49519=AXIS2_PLACEMENT_3D ( 'NONE', #2854, #24199, #20491 ) ;
#49521=PLANE ( 'NONE',  #30227 ) ;
#49522=CARTESIAN_POINT ( 'NONE',  ( -26.13337879274045505, 0.000000000000000000, 6.833023547870798353 ) ) ;
#49523=LINE ( 'NONE', #14871, #29344 ) ;
#49524=DIRECTION ( 'NONE',  ( 0.9999697198139515519, 0.000000000000000000, 0.007781995580013368816 ) ) ;
#49525=PLANE ( 'NONE',  #55477 ) ;
#49526=PLANE ( 'NONE',  #2949 ) ;
#49527=AXIS2_PLACEMENT_3D ( 'NONE', #31920, #2642, #45522 ) ;
#49528=ORIENTED_EDGE ( 'NONE', *, *, #52482, .F. ) ;
#49529=VERTEX_POINT ( 'NONE', #50664 ) ;
#49530=PLANE ( 'NONE',  #48217 ) ;
#49531=DIRECTION ( 'NONE',  ( 0.6246952433987893460, 0.7422098413412802076, -0.2426528472758539279 ) ) ;
#49532=AXIS2_PLACEMENT_3D ( 'NONE', #53916, #15035, #6785 ) ;
#49533=LINE ( 'NONE', #6365, #49661 ) ;
#49534=AXIS2_PLACEMENT_3D ( 'NONE', #55961, #38914, #31220 ) ;
#49535=VECTOR ( 'NONE', #51478, 999.9999999999998863 ) ;
#49536=LINE ( 'NONE', #10654, #49446 ) ;
#49537=VERTEX_POINT ( 'NONE', #42979 ) ;
#49538=LINE ( 'NONE', #18882, #53994 ) ;
#49539=DIRECTION ( 'NONE',  ( 0.000000000000000000, -1.000000000000000000, 0.000000000000000000 ) ) ;
#49540=ORIENTED_EDGE ( 'NONE', *, *, #31513, .F. ) ;
#49541=PLANE ( 'NONE',  #34733 ) ;
#49542=LINE ( 'NONE', #14351, #40355 ) ;
#49543=ORIENTED_EDGE ( 'NONE', *, *, #36843, .F. ) ;
#49544=AXIS2_PLACEMENT_3D ( 'NONE', #1608, #22627, #39934 ) ;
#49545=LINE ( 'NONE', #2084, #41540 ) ;
#49546=DIRECTION ( 'NONE',  ( -0.005961354470445682716, -0.6427876096865404731, 0.7660212471507180654 ) ) ;
#49547=VECTOR ( 'NONE', #38835, 999.9999999999998863 ) ;
#49548=DIRECTION ( 'NONE',  ( -0.7660212471507179544, -0.6427876096865405842, -0.005961354470445141482 ) ) ;
#49549=EDGE_CURVE ( 'NONE', #25319, #53748, #25654, .T. ) ;
#49550=DIRECTION ( 'NONE',  ( 0.000000000000000000, -1.000000000000000000, 0.000000000000000000 ) ) ;
#49551=VECTOR ( 'NONE', #19672, 999.9999999999998863 ) ;
#49552=DIRECTION ( 'NONE',  ( 0.007781995580012663651, -3.146120232559066537E-19, -0.9999697198139514409 ) ) ;
#49553=ORIENTED_EDGE ( 'NONE', *, *, #22061, .F. ) ;
#49554=VECTOR ( 'NONE', #47215, 999.9999999999998863 ) ;
#49555=ADVANCED_FACE ( 'NONE', ( #37893 ), #46971, .F. ) ;
#49556=ORIENTED_EDGE ( 'NONE', *, *, #50337, .F. ) ;
#49557=CARTESIAN_POINT ( 'NONE',  ( -19.79569077582305070, 0.000000000000000000, 14.58012466630350445 ) ) ;
#49558=DIRECTION ( 'NONE',  ( 0.000000000000000000, -1.000000000000000000, 0.000000000000000000 ) ) ;
#49559=LINE ( 'NONE', #44713, #54183 ) ;
#49560=ADVANCED_FACE ( 'NONE', ( #21418 ), #33356, .F. ) ;
#49561=CARTESIAN_POINT ( 'NONE',  ( 2.072287782118878319, 0.000000000000000000, -2.950529333540147015 ) ) ;
#49562=EDGE_CURVE ( 'NONE', #40568, #33926, #11493, .T. ) ;
#49563=LINE ( 'NONE', #6134, #33974 ) ;
#49564=ORIENTED_EDGE ( 'NONE', *, *, #7778, .F. ) ;
#49565=PLANE ( 'NONE',  #16561 ) ;
#49566=VECTOR ( 'NONE', #27985, 1000.000000000000227 ) ;
#49567=PLANE ( 'NONE',  #32305 ) ;
#49568=DIRECTION ( 'NONE',  ( 0.005961354470445682716, -0.6427876096865404731, -0.7660212471507180654 ) ) ;
#49569=ORIENTED_EDGE ( 'NONE', *, *, #29521, .T. ) ;
#49570=LINE ( 'NONE', #40190, #42876 ) ;
#49571=EDGE_LOOP ( 'NONE', ( #3604, #23685, #48831, #14500 ) ) ;
#49572=DIRECTION ( 'NONE',  ( 0.7660212471507180654, -0.6427876096865404731, 0.005961354470445141482 ) ) ;
#49573=VECTOR ( 'NONE', #4549, 999.9999999999998863 ) ;
#49574=PLANE ( 'NONE',  #27511 ) ;
#49575=VERTEX_POINT ( 'NONE', #25381 ) ;
#49576=CARTESIAN_POINT ( 'NONE',  ( -8.831901609284649624, 0.000000000000000000, 4.751675225048217044 ) ) ;
#49577=AXIS2_PLACEMENT_3D ( 'NONE', #20414, #38021, #21255 ) ;
#49578=ORIENTED_EDGE ( 'NONE', *, *, #53231, .F. ) ;
#49579=VERTEX_POINT ( 'NONE', #16289 ) ;
#49580=VECTOR ( 'NONE', #11800, 1000.000000000000227 ) ;
#49581=ORIENTED_EDGE ( 'NONE', *, *, #42416, .T. ) ;
#49582=LINE ( 'NONE', #36236, #48393 ) ;
#49583=VERTEX_POINT ( 'NONE', #7221 ) ;
#49584=ORIENTED_EDGE ( 'NONE', *, *, #38087, .T. ) ;
#49585=CARTESIAN_POINT ( 'NONE',  ( -17.66443310188656213, 0.000000000000000000, 5.252276548676588774 ) ) ;
#49586=ORIENTED_EDGE ( 'NONE', *, *, #27211, .F. ) ;
#49587=EDGE_CURVE ( 'NONE', #16962, #17624, #20572, .T. ) ;
#49588=AXIS2_PLACEMENT_3D ( 'NONE', #37020, #36738, #41548 ) ;
#49589=VERTEX_POINT ( 'NONE', #29360 ) ;
#49590=DIRECTION ( 'NONE',  ( -0.6427681459581293666, -0.7660444431189770143, -0.005002170337467561935 ) ) ;
#49591=EDGE_LOOP ( 'NONE', ( #6515, #16938, #21030, #56137 ) ) ;
#49592=ORIENTED_EDGE ( 'NONE', *, *, #5709, .F. ) ;
#49593=EDGE_CURVE ( 'NONE', #37525, #36530, #24817, .T. ) ;
#49594=ADVANCED_FACE ( 'NONE', ( #46377 ), #46676, .F. ) ;
#49595=AXIS2_PLACEMENT_3D ( 'NONE', #32853, #46771, #55018 ) ;
#49596=VECTOR ( 'NONE', #45681, 1000.000000000000000 ) ;
#49597=CARTESIAN_POINT ( 'NONE',  ( -9.403061784675696089, -0.1191753592594190225, 5.585897492219126015 ) ) ;
#49598=CARTESIAN_POINT ( 'NONE',  ( -14.63915290389857304, 0.000000000000000000, 8.769134620551508164 ) ) ;
#49599=FACE_OUTER_BOUND ( 'NONE', #33539, .T. ) ;
#49600=DIRECTION ( 'NONE',  ( 0.9321478471874541372, 0.000000000000000000, -0.3620778797217453771 ) ) ;
#49601=ORIENTED_EDGE ( 'NONE', *, *, #2718, .F. ) ;
#49602=DIRECTION ( 'NONE',  ( 0.6427681459581294776, -0.7660444431189769032, 0.005002170337467562802 ) ) ;
#49603=VERTEX_POINT ( 'NONE', #42684 ) ;
#49604=ORIENTED_EDGE ( 'NONE', *, *, #16608, .T. ) ;
#49605=CARTESIAN_POINT ( 'NONE',  ( -11.40636015113596180, 0.000000000000000000, 11.32142374880780089 ) ) ;
#49606=AXIS2_PLACEMENT_3D ( 'NONE', #7982, #42871, #54813 ) ;
#49607=ADVANCED_FACE ( 'NONE', ( #28816 ), #24524, .F. ) ;
#49608=PLANE ( 'NONE',  #2472 ) ;
#49609=DIRECTION ( 'NONE',  ( 0.005002170337468016433, -0.7660444431189770143, -0.6427681459581293666 ) ) ;
#49610=LINE ( 'NONE', #27446, #32099 ) ;
#49611=DIRECTION ( 'NONE',  ( -0.7660212471507179544, -0.6427876096865405842, -0.005961354470445141482 ) ) ;
#49612=VERTEX_POINT ( 'NONE', #37601 ) ;
#49613=LINE ( 'NONE', #45329, #28357 ) ;
#49614=EDGE_LOOP ( 'NONE', ( #25352, #43016, #34278, #28177 ) ) ;
#49615=LINE ( 'NONE', #41068, #43813 ) ;
#49616=DIRECTION ( 'NONE',  ( 0.9999697198139515519, 0.000000000000000000, 0.007781995580013368816 ) ) ;
#49617=VECTOR ( 'NONE', #29364, 999.9999999999998863 ) ;
#49618=DIRECTION ( 'NONE',  ( 0.6427681459581294776, -0.7660444431189769032, 0.005002170337467562802 ) ) ;
#49619=DIRECTION ( 'NONE',  ( -0.7660212471507179544, -0.6427876096865405842, -0.005961354470445141482 ) ) ;
#49620=CARTESIAN_POINT ( 'NONE',  ( -12.13851405436063047, 0.000000000000000000, 11.68505802764555135 ) ) ;
#49621=VECTOR ( 'NONE', #6122, 1000.000000000000227 ) ;
#49623=ORIENTED_EDGE ( 'NONE', *, *, #15764, .F. ) ;
#49625=DIRECTION ( 'NONE',  ( 0.005002170337468016433, -0.7660444431189770143, -0.6427681459581293666 ) ) ;
#49626=CARTESIAN_POINT ( 'NONE',  ( 2.072287782118878319, 0.000000000000000000, -2.950529333540147015 ) ) ;
#49627=VECTOR ( 'NONE', #51873, 999.9999999999998863 ) ;
#49628=DIRECTION ( 'NONE',  ( -0.005002170337468016433, -0.7660444431189770143, 0.6427681459581293666 ) ) ;
#49629=EDGE_CURVE ( 'NONE', #3020, #40968, #54927, .T. ) ;
#49630=CARTESIAN_POINT ( 'NONE',  ( -16.92365703814605027, 0.000000000000000000, 3.780713160065547029 ) ) ;
#49631=CARTESIAN_POINT ( 'NONE',  ( -19.60990026154428278, 0.000000000000000000, 4.498472333781370125 ) ) ;
#49632=CARTESIAN_POINT ( 'NONE',  ( -22.29929853844754462, 4.657758921906511418, 13.18730186385467462 ) ) ;
#49633=AXIS2_PLACEMENT_3D ( 'NONE', #38146, #46674, #42428 ) ;
#49634=CARTESIAN_POINT ( 'NONE',  ( -12.85428006665745215, 2.876837460659007473, 6.595740411778870715 ) ) ;
#49635=PLANE ( 'NONE',  #8392 ) ;
#49636=ORIENTED_EDGE ( 'NONE', *, *, #53780, .F. ) ;
#49637=EDGE_CURVE ( 'NONE', #47161, #42624, #7799, .T. ) ;
#49638=ORIENTED_EDGE ( 'NONE', *, *, #31406, .F. ) ;
#49639=ADVANCED_FACE ( 'NONE', ( #47520 ), #43289, .F. ) ;
#49641=ADVANCED_FACE ( 'NONE', ( #31326 ), #17705, .F. ) ;
#49642=ORIENTED_EDGE ( 'NONE', *, *, #49041, .F. ) ;
#49643=EDGE_LOOP ( 'NONE', ( #42619, #46548, #54235, #9512 ) ) ;
#49644=ORIENTED_EDGE ( 'NONE', *, *, #5, .F. ) ;
#49645=VERTEX_POINT ( 'NONE', #920 ) ;
#49646=DIRECTION ( 'NONE',  ( 0.007781995580012663651, -3.146120232559066537E-19, -0.9999697198139514409 ) ) ;
#49647=ADVANCED_FACE ( 'NONE', ( #12876 ), #5220, .F. ) ;
#49648=CARTESIAN_POINT ( 'NONE',  ( -15.79438930050108780, 0.000000000000000000, 3.789501382717568312 ) ) ;
#49649=ORIENTED_EDGE ( 'NONE', *, *, #44801, .T. ) ;
#49650=EDGE_CURVE ( 'NONE', #33225, #55548, #48654, .T. ) ;
#49651=ORIENTED_EDGE ( 'NONE', *, *, #6171, .F. ) ;
#49652=EDGE_LOOP ( 'NONE', ( #46422, #7906, #24396, #5788 ) ) ;
#49653=ADVANCED_FACE ( 'NONE', ( #22533 ), #21948, .F. ) ;
#49654=VECTOR ( 'NONE', #33670, 1000.000000000000227 ) ;
#49655=DIRECTION ( 'NONE',  ( 0.7660212471507180654, -0.6427876096865404731, 0.005961354470445141482 ) ) ;
#49656=LINE ( 'NONE', #36880, #32798 ) ;
#49657=DIRECTION ( 'NONE',  ( -0.5364919789714478471, 0.6444004775717705469, -0.5449076811759709926 ) ) ;
#49658=ORIENTED_EDGE ( 'NONE', *, *, #41605, .F. ) ;
#49659=CARTESIAN_POINT ( 'NONE',  ( -13.65814614712131636, 0.000000000000000000, 2.128791785447766483 ) ) ;
#49660=ADVANCED_FACE ( 'NONE', ( #364 ), #4636, .F. ) ;
#49661=VECTOR ( 'NONE', #36450, 1000.000000000000227 ) ;
#49662=DIRECTION ( 'NONE',  ( -0.7660212471507179544, -0.6427876096865405842, -0.005961354470445141482 ) ) ;
#49663=LINE ( 'NONE', #36058, #8498 ) ;
#49664=EDGE_CURVE ( 'NONE', #39014, #55340, #52610, .T. ) ;
#49666=DIRECTION ( 'NONE',  ( -0.9999697198139514409, -0.000000000000000000, -0.007781995580013368816 ) ) ;
#49667=CARTESIAN_POINT ( 'NONE',  ( -15.47613562217328287, 1.581621852479004442, 5.488488676526967147 ) ) ;
#49668=DIRECTION ( 'NONE',  ( 0.007781995580012663651, 0.000000000000000000, -0.9999697198139515519 ) ) ;
#49669=LINE ( 'NONE', #10763, #46641 ) ;
#49670=DIRECTION ( 'NONE',  ( 0.000000000000000000, -0.000000000000000000, -1.000000000000000000 ) ) ;
#49671=EDGE_LOOP ( 'NONE', ( #44071, #43737, #4627 ) ) ;
#49672=FACE_OUTER_BOUND ( 'NONE', #42714, .T. ) ;
#49673=ORIENTED_EDGE ( 'NONE', *, *, #41680, .T. ) ;
#49675=LINE ( 'NONE', #24104, #30496 ) ;
#49676=DIRECTION ( 'NONE',  ( 0.5449076811759707706, 0.6444004775717708799, -0.5364919789714476250 ) ) ;
#49678=PLANE ( 'NONE',  #51353 ) ;
#49679=CARTESIAN_POINT ( 'NONE',  ( -20.16176772743538237, -0.1191753592594197858, 14.76194180572237968 ) ) ;
#49680=CARTESIAN_POINT ( 'NONE',  ( 2.072287782118878319, 0.000000000000000000, -2.950529333540147015 ) ) ;
#49681=PLANE ( 'NONE',  #16649 ) ;
#49683=DIRECTION ( 'NONE',  ( 0.9999697198139515519, 0.000000000000000000, 0.007781995580013368816 ) ) ;
#49684=LINE ( 'NONE', #32377, #31177 ) ;
#49685=LINE ( 'NONE', #50777, #18583 ) ;
#49686=FACE_OUTER_BOUND ( 'NONE', #1262, .T. ) ;
#49687=DIRECTION ( 'NONE',  ( -0.005961354470445682716, -0.6427876096865404731, 0.7660212471507180654 ) ) ;
#49688=DIRECTION ( 'NONE',  ( 0.9999697198139515519, 0.000000000000000000, 0.007781995580013368816 ) ) ;
#49689=EDGE_CURVE ( 'NONE', #7355, #44724, #34735, .T. ) ;
#49690=DIRECTION ( 'NONE',  ( -0.5449076811759708816, 0.6444004775717707689, 0.5364919789714475140 ) ) ;
#49691=DIRECTION ( 'NONE',  ( -0.5364919789714478471, 0.6444004775717705469, -0.5449076811759709926 ) ) ;
#49692=DIRECTION ( 'NONE',  ( 0.6427681459581294776, -0.7660444431189769032, 0.005002170337467562802 ) ) ;
#49693=VERTEX_POINT ( 'NONE', #39842 ) ;
#49694=ORIENTED_EDGE ( 'NONE', *, *, #48425, .T. ) ;
#49695=CARTESIAN_POINT ( 'NONE',  ( -18.29747203306047609, -0.1191753592594177458, 14.03778604627889059 ) ) ;
#49696=DIRECTION ( 'NONE',  ( 0.007781995580012663651, -3.146120232559066537E-19, -0.9999697198139514409 ) ) ;
#49697=AXIS2_PLACEMENT_3D ( 'NONE', #19339, #53696, #23878 ) ;
#49698=VERTEX_POINT ( 'NONE', #4922 ) ;
#49699=LINE ( 'NONE', #2257, #23162 ) ;
#49700=ORIENTED_EDGE ( 'NONE', *, *, #43624, .F. ) ;
#49701=DIRECTION ( 'NONE',  ( -0.005002170337468016433, -0.7660444431189770143, 0.6427681459581293666 ) ) ;
#49702=ADVANCED_FACE ( 'NONE', ( #13708 ), #40109, .F. ) ;
#49703=ORIENTED_EDGE ( 'NONE', *, *, #51923, .F. ) ;
#49704=ORIENTED_EDGE ( 'NONE', *, *, #8814, .F. ) ;
#49705=ORIENTED_EDGE ( 'NONE', *, *, #11147, .T. ) ;
#49706=DIRECTION ( 'NONE',  ( 0.6427681459581294776, -0.7660444431189769032, 0.005002170337467562802 ) ) ;
#49707=LINE ( 'NONE', #31817, #14168 ) ;
#49708=FACE_OUTER_BOUND ( 'NONE', #38451, .T. ) ;
#49709=EDGE_CURVE ( 'NONE', #22830, #50706, #31025, .T. ) ;
#49710=VERTEX_POINT ( 'NONE', #48346 ) ;
#49711=ORIENTED_EDGE ( 'NONE', *, *, #56142, .F. ) ;
#49712=ADVANCED_FACE ( 'NONE', ( #71 ), #4379, .F. ) ;
#49713=DIRECTION ( 'NONE',  ( 0.007781995580012663651, 0.000000000000000000, -0.9999697198139515519 ) ) ;
#49714=ORIENTED_EDGE ( 'NONE', *, *, #16680, .F. ) ;
#49715=DIRECTION ( 'NONE',  ( 0.007781995580012662783, 0.000000000000000000, -0.9999697198139514409 ) ) ;
#49716=ORIENTED_EDGE ( 'NONE', *, *, #43556, .F. ) ;
#49717=CARTESIAN_POINT ( 'NONE',  ( -10.47421230394850866, 0.000000000000000000, 10.95934586908605723 ) ) ;
#49718=LINE ( 'NONE', #36951, #24013 ) ;
#49719=EDGE_CURVE ( 'NONE', #44308, #54486, #26781, .T. ) ;
#49720=ORIENTED_EDGE ( 'NONE', *, *, #14688, .F. ) ;
#49721=CARTESIAN_POINT ( 'NONE',  ( -20.06177075545399191, 0.000000000000000000, 14.76272000528038220 ) ) ;
#49722=ADVANCED_FACE ( 'NONE', ( #44375 ), #5476, .F. ) ;
#49723=CARTESIAN_POINT ( 'NONE',  ( -12.31143384783145045, -0.8417996532631565332, 2.845647379707433089 ) ) ;
#49724=EDGE_LOOP ( 'NONE', ( #37230, #47862, #19708, #42524 ) ) ;
#49725=CARTESIAN_POINT ( 'NONE',  ( -14.66887761629205222, 0.000000000000000000, 12.58869632783390990 ) ) ;
#49726=DIRECTION ( 'NONE',  ( -0.005961354470445682716, -0.6427876096865404731, 0.7660212471507180654 ) ) ;
#49727=CARTESIAN_POINT ( 'NONE',  ( -17.46532115785441519, 0.000000000000000000, 13.67492996699914265 ) ) ;
#49728=ORIENTED_EDGE ( 'NONE', *, *, #28588, .F. ) ;
#49730=CARTESIAN_POINT ( 'NONE',  ( -16.68496742766923191, 1.905425754524007198, 6.489457369783435681 ) ) ;
#49731=DIRECTION ( 'NONE',  ( 0.7660212471507180654, -0.6427876096865404731, 0.005961354470445141482 ) ) ;
#49732=CARTESIAN_POINT ( 'NONE',  ( -16.81345671998191449, 0.000000000000000000, 3.412238694616132495 ) ) ;
#49733=PLANE ( 'NONE',  #30490 ) ;
#49734=CARTESIAN_POINT ( 'NONE',  ( -16.81345671998191449, 0.000000000000000000, 3.412238694616132495 ) ) ;
#49735=DIRECTION ( 'NONE',  ( -0.005002170337468016433, -0.7660444431189770143, 0.6427681459581293666 ) ) ;
#49736=DIRECTION ( 'NONE',  ( 0.007781995580012663651, 0.000000000000000000, -0.9999697198139515519 ) ) ;
#49737=ORIENTED_EDGE ( 'NONE', *, *, #25977, .F. ) ;
#49738=LINE ( 'NONE', #6866, #39840 ) ;
#49739=DIRECTION ( 'NONE',  ( -0.005961354470445682716, -0.6427876096865404731, 0.7660212471507180654 ) ) ;
#49741=ORIENTED_EDGE ( 'NONE', *, *, #43186, .F. ) ;
#49742=CARTESIAN_POINT ( 'NONE',  ( -11.88160593113000907, -1.975113310420658852, 4.538648407496340020 ) ) ;
#49743=CARTESIAN_POINT ( 'NONE',  ( -21.79697860796153464, 3.524445264749008988, 11.13222295634402137 ) ) ;
#49744=EDGE_CURVE ( 'NONE', #33688, #44617, #34458, .T. ) ;
#49745=DIRECTION ( 'NONE',  ( 0.007781995580012662783, 0.000000000000000000, -0.9999697198139514409 ) ) ;
#49746=EDGE_CURVE ( 'NONE', #49698, #1575, #26224, .T. ) ;
#49747=DIRECTION ( 'NONE',  ( -0.6427681459581293666, -0.7660444431189770143, -0.005002170337467561935 ) ) ;
#49748=LINE ( 'NONE', #15374, #22933 ) ;
#49750=EDGE_CURVE ( 'NONE', #21379, #8596, #10603, .T. ) ;
#49751=VERTEX_POINT ( 'NONE', #54286 ) ;
#49752=ADVANCED_FACE ( 'NONE', ( #32165 ), #19081, .F. ) ;
#49754=EDGE_CURVE ( 'NONE', #9106, #33384, #6067, .T. ) ;
#49755=EDGE_CURVE ( 'NONE', #38597, #18224, #24203, .T. ) ;
#49756=ADVANCED_FACE ( 'NONE', ( #15136 ), #10300, .F. ) ;
#49757=CARTESIAN_POINT ( 'NONE',  ( -15.53681210902263921, 0.000000000000000000, 4.699496061180079565 ) ) ;
#49758=ORIENTED_EDGE ( 'NONE', *, *, #12853, .F. ) ;
#49759=LINE ( 'NONE', #50008, #25828 ) ;
#49760=ORIENTED_EDGE ( 'NONE', *, *, #9442, .T. ) ;
#49761=CARTESIAN_POINT ( 'NONE',  ( -32.10901097986136676, -1.000000000000000000, 16.76339505873265168 ) ) ;
#49762=ORIENTED_EDGE ( 'NONE', *, *, #34376, .F. ) ;
#49763=EDGE_LOOP ( 'NONE', ( #15353, #25313, #38985, #44886 ) ) ;
#49764=DIRECTION ( 'NONE',  ( -0.5449076811759708816, 0.6444004775717707689, 0.5364919789714475140 ) ) ;
#49765=PLANE ( 'NONE',  #6904 ) ;
#49766=CARTESIAN_POINT ( 'NONE',  ( -12.06424151263527023, 0.000000000000000000, 2.141195919867798558 ) ) ;
#49767=ORIENTED_EDGE ( 'NONE', *, *, #46193, .T. ) ;
#49768=AXIS2_PLACEMENT_3D ( 'NONE', #51204, #47805, #20556 ) ;
#49769=CARTESIAN_POINT ( 'NONE',  ( -15.88053067323646417, -0.1191753592594197858, 2.950163842912994383 ) ) ;
#49771=EDGE_LOOP ( 'NONE', ( #35808, #18117, #3284, #6745 ) ) ;
#49772=EDGE_CURVE ( 'NONE', #12737, #31264, #6884, .T. ) ;
#49773=EDGE_LOOP ( 'NONE', ( #1696, #14731, #53320, #42011 ) ) ;
#49774=EDGE_LOOP ( 'NONE', ( #41898, #48347, #45640, #53724 ) ) ;
#49775=CARTESIAN_POINT ( 'NONE',  ( -20.16884058355513432, -2.946525016555658905, 9.351943885874463902 ) ) ;
#49776=EDGE_CURVE ( 'NONE', #43469, #50912, #1504, .T. ) ;
#49777=EDGE_LOOP ( 'NONE', ( #26047, #25262, #18754, #3950 ) ) ;
#49778=CARTESIAN_POINT ( 'NONE',  ( -9.908141408373387193, -0.1191753592594197858, 10.77908512878318703 ) ) ;
#49779=EDGE_LOOP ( 'NONE', ( #758, #5776, #28309, #31954 ) ) ;
#49780=CARTESIAN_POINT ( 'NONE',  ( -15.86710544311044302, 0.000000000000000000, 13.13336954653252953 ) ) ;
#49781=DIRECTION ( 'NONE',  ( 0.6427681459581294776, -0.7660444431189769032, 0.005002170337467562802 ) ) ;
#49782=EDGE_CURVE ( 'NONE', #9324, #13476, #49759, .T. ) ;
#49785=EDGE_LOOP ( 'NONE', ( #13760, #44972, #27154, #6308 ) ) ;
#49786=FACE_OUTER_BOUND ( 'NONE', #18632, .T. ) ;
#49787=CARTESIAN_POINT ( 'NONE',  ( -17.74560456716937296, 0.000000000000000000, 3.774316574337878372 ) ) ;
#49788=CARTESIAN_POINT ( 'NONE',  ( -14.94916102560700821, 0.000000000000000000, 2.688082935172642962 ) ) ;
#49789=DIRECTION ( 'NONE',  ( 0.6427681459581294776, -0.7660444431189769032, 0.005002170337467562802 ) ) ;
#49790=PLANE ( 'NONE',  #7840 ) ;
#49791=DIRECTION ( 'NONE',  ( 0.007781995580012662783, 0.000000000000000000, -0.9999697198139514409 ) ) ;
#49792=FACE_OUTER_BOUND ( 'NONE', #7263, .T. ) ;
#49793=ORIENTED_EDGE ( 'NONE', *, *, #29872, .T. ) ;
#49794=ORIENTED_EDGE ( 'NONE', *, *, #46328, .T. ) ;
#49797=CARTESIAN_POINT ( 'NONE',  ( -13.00788557384385413, 0.000000000000000000, 3.980512612620602297 ) ) ;
#49798=CARTESIAN_POINT ( 'NONE',  ( -20.37303252807906162, -1.003701604285655469, 6.242754764109628596 ) ) ;
#49799=DIRECTION ( 'NONE',  ( 0.5449076811759707706, 0.6444004775717708799, -0.5364919789714476250 ) ) ;
#49800=EDGE_LOOP ( 'NONE', ( #11945, #30594, #52588, #12545 ) ) ;
#49801=CARTESIAN_POINT ( 'NONE',  ( -11.77243710274829525, -0.1191753592594197858, 11.50324088822667612 ) ) ;
#49802=DIRECTION ( 'NONE',  ( 0.000000000000000000, -0.000000000000000000, -1.000000000000000000 ) ) ;
#49803=ORIENTED_EDGE ( 'NONE', *, *, #3742, .T. ) ;
#49804=LINE ( 'NONE', #32748, #20251 ) ;
#49805=CARTESIAN_POINT ( 'NONE',  ( -21.47263955680318404, 0.000000000000000000, 5.022634149262071190 ) ) ;
#49806=VERTEX_POINT ( 'NONE', #36990 ) ;
#49808=DIRECTION ( 'NONE',  ( 0.005002170337468016433, -0.7660444431189770143, -0.6427681459581293666 ) ) ;
#49809=CARTESIAN_POINT ( 'NONE',  ( -16.29638889291085135, 0.000000000000000000, 8.586911613300497237 ) ) ;
#49810=CARTESIAN_POINT ( 'NONE',  ( -12.37052422292021348, 4.010151117816511679, 1.359118628339639256 ) ) ;
#49811=LINE ( 'NONE', #33347, #52828 ) ;
#49812=ORIENTED_EDGE ( 'NONE', *, *, #7350, .F. ) ;
#49813=EDGE_LOOP ( 'NONE', ( #32699, #18336, #1217, #43586 ) ) ;
#49814=DIRECTION ( 'NONE',  ( 0.9999697198139515519, 0.000000000000000000, 0.007781995580013368816 ) ) ;
#49815=CARTESIAN_POINT ( 'NONE',  ( -10.47421230394850866, 0.000000000000000000, 10.95934586908605723 ) ) ;
#49816=CARTESIAN_POINT ( 'NONE',  ( -13.69263478918470867, 0.000000000000000000, 6.560508224540939182 ) ) ;
#49817=ADVANCED_FACE ( 'NONE', ( #15385 ), #40940, .F. ) ;
#49819=LINE ( 'NONE', #45543, #50029 ) ;
#49820=LINE ( 'NONE', #14908, #28532 ) ;
#49821=ORIENTED_EDGE ( 'NONE', *, *, #31749, .T. ) ;
#49822=EDGE_CURVE ( 'NONE', #40102, #35268, #36157, .T. ) ;
#49823=DIRECTION ( 'NONE',  ( 0.6427681459581294776, -0.7660444431189769032, 0.005002170337467562802 ) ) ;
#49824=PLANE ( 'NONE',  #35064 ) ;
#49826=VERTEX_POINT ( 'NONE', #28163 ) ;
#49827=DIRECTION ( 'NONE',  ( -0.5364919789714478471, 0.6444004775717705469, -0.5449076811759709926 ) ) ;
#49828=DIRECTION ( 'NONE',  ( -0.005961354470445682716, -0.6427876096865404731, 0.7660212471507180654 ) ) ;
#49829=PLANE ( 'NONE',  #46546 ) ;
#49830=ORIENTED_EDGE ( 'NONE', *, *, #2687, .F. ) ;
#49831=DIRECTION ( 'NONE',  ( 0.9999697198139515519, 0.000000000000000000, 0.007781995580013368816 ) ) ;
#49832=ORIENTED_EDGE ( 'NONE', *, *, #35393, .T. ) ;
#49833=EDGE_CURVE ( 'NONE', #9862, #21743, #45474, .T. ) ;
#49834=ORIENTED_EDGE ( 'NONE', *, *, #40012, .T. ) ;
#49835=EDGE_LOOP ( 'NONE', ( #41794, #48991, #46271 ) ) ;
#49836=LINE ( 'NONE', #36797, #19367 ) ;
#49837=EDGE_LOOP ( 'NONE', ( #47823, #41258, #8215, #46696 ) ) ;
#49838=EDGE_CURVE ( 'NONE', #22139, #54019, #53202, .T. ) ;
#49839=ORIENTED_EDGE ( 'NONE', *, *, #1905, .T. ) ;
#49840=LINE ( 'NONE', #46134, #6666 ) ;
#49841=EDGE_LOOP ( 'NONE', ( #10394, #33088, #38624 ) ) ;
#49843=EDGE_CURVE ( 'NONE', #25320, #6407, #31614, .T. ) ;
#49844=ORIENTED_EDGE ( 'NONE', *, *, #3159, .F. ) ;
#49846=VERTEX_POINT ( 'NONE', #5763 ) ;
#49847=ORIENTED_EDGE ( 'NONE', *, *, #42302, .T. ) ;
#49848=EDGE_CURVE ( 'NONE', #44182, #22811, #53457, .T. ) ;
#49849=VERTEX_POINT ( 'NONE', #20768 ) ;
#49850=DIRECTION ( 'NONE',  ( -0.5449076811759708816, 0.6444004775717707689, 0.5364919789714475140 ) ) ;
#49851=CARTESIAN_POINT ( 'NONE',  ( -20.54204810873173415, 0.000000000000000000, 4.860550213503115558 ) ) ;
#49852=DIRECTION ( 'NONE',  ( 0.007781995580012663651, -3.146120232559066537E-19, -0.9999697198139514409 ) ) ;
#49853=LINE ( 'NONE', #7251, #3328 ) ;
#49854=ORIENTED_EDGE ( 'NONE', *, *, #18491, .T. ) ;
#49855=CARTESIAN_POINT ( 'NONE',  ( 2.072287782118878319, 0.000000000000000000, -2.950529333540147015 ) ) ;
#49856=EDGE_LOOP ( 'NONE', ( #45863, #24923, #51312, #53193, #385 ) ) ;
#49857=VERTEX_POINT ( 'NONE', #47157 ) ;
#49860=CARTESIAN_POINT ( 'NONE',  ( -12.30091215004045679, 2.229229656569005957, 5.317958784709427178 ) ) ;
#49861=CARTESIAN_POINT ( 'NONE',  ( -17.57617378642196115, 4.657758921906512306, 3.360507623857465820 ) ) ;
#49862=DIRECTION ( 'NONE',  ( 0.6427681459581294776, -0.7660444431189769032, 0.005002170337467562802 ) ) ;
#49863=ORIENTED_EDGE ( 'NONE', *, *, #43017, .F. ) ;
#49865=ORIENTED_EDGE ( 'NONE', *, *, #29946, .T. ) ;
#49866=DIRECTION ( 'NONE',  ( 0.007781995580012662783, 0.000000000000000000, -0.9999697198139514409 ) ) ;
#49867=DIRECTION ( 'NONE',  ( 0.9999697198139515519, 0.000000000000000000, 0.007781995580013368816 ) ) ;
#49868=LINE ( 'NONE', #37103, #26320 ) ;
#49869=DIRECTION ( 'NONE',  ( -0.005961354470445682716, -0.6427876096865404731, 0.7660212471507180654 ) ) ;
#49870=DIRECTION ( 'NONE',  ( 0.000000000000000000, -0.000000000000000000, -1.000000000000000000 ) ) ;
#49871=VECTOR ( 'NONE', #23220, 999.9999999999998863 ) ;
#49872=EDGE_LOOP ( 'NONE', ( #53410, #39211, #6157, #14498 ) ) ;
#49873=CARTESIAN_POINT ( 'NONE',  ( -19.60990026154428278, 0.000000000000000000, 4.498472333781370125 ) ) ;
#49874=CARTESIAN_POINT ( 'NONE',  ( -15.55420528410555292, 3.362543313726509719, 2.616430550317521586 ) ) ;
#49875=LINE ( 'NONE', #27191, #24564 ) ;
#49876=EDGE_CURVE ( 'NONE', #37328, #2943, #11949, .T. ) ;
#49877=DIRECTION ( 'NONE',  ( -0.7660212471507179544, -0.6427876096865405842, -0.005961354470445141482 ) ) ;
#49878=DIRECTION ( 'NONE',  ( 0.000000000000000000, -1.000000000000000000, 0.000000000000000000 ) ) ;
#49879=EDGE_CURVE ( 'NONE', #55101, #38023, #34130, .T. ) ;
#49880=DIRECTION ( 'NONE',  ( -0.5449076811759708816, 0.6444004775717707689, 0.5364919789714475140 ) ) ;
#49881=ADVANCED_FACE ( 'NONE', ( #25045 ), #20495, .F. ) ;
#49882=CARTESIAN_POINT ( 'NONE',  ( 1.086233639165236964, 0.000000000000000000, 2.796443541562362078 ) ) ;
#49883=LINE ( 'NONE', #54414, #25135 ) ;
#49884=CARTESIAN_POINT ( 'NONE',  ( -11.90068819181640691, 0.1245042932765045296, 1.708285316316361158 ) ) ;
#49885=ORIENTED_EDGE ( 'NONE', *, *, #2857, .T. ) ;
#49886=ORIENTED_EDGE ( 'NONE', *, *, #19365, .F. ) ;
#49887=ORIENTED_EDGE ( 'NONE', *, *, #34330, .F. ) ;
#49888=VERTEX_POINT ( 'NONE', #2601 ) ;
#49890=CARTESIAN_POINT ( 'NONE',  ( -13.27065584551087163, 0.000000000000000000, 12.04557950825129176 ) ) ;
#49892=ORIENTED_EDGE ( 'NONE', *, *, #17125, .F. ) ;
#49893=CARTESIAN_POINT ( 'NONE',  ( -14.39473050296726697, 0.000000000000000000, 3.061729711506068874 ) ) ;
#49894=EDGE_LOOP ( 'NONE', ( #34841, #51311, #17990, #33017 ) ) ;
#49895=VERTEX_POINT ( 'NONE', #29008 ) ;
#49896=ADVANCED_FACE ( 'NONE', ( #42056 ), #50853, .F. ) ;
#49897=AXIS2_PLACEMENT_3D ( 'NONE', #7857, #24039, #45900 ) ;
#49899=EDGE_CURVE ( 'NONE', #27583, #37134, #11690, .T. ) ;
#49900=DIRECTION ( 'NONE',  ( 0.005002170337468016433, -0.7660444431189770143, -0.6427681459581293666 ) ) ;
#49901=DIRECTION ( 'NONE',  ( 0.007781995580012662783, 0.000000000000000000, -0.9999697198139514409 ) ) ;
#49902=ORIENTED_EDGE ( 'NONE', *, *, #11109, .F. ) ;
#49903=CARTESIAN_POINT ( 'NONE',  ( -18.86354292863559579, 0.000000000000000000, 14.21804678658176080 ) ) ;
#49904=LINE ( 'NONE', #28329, #33673 ) ;
#49905=EDGE_CURVE ( 'NONE', #21119, #23033, #3715, .T. ) ;
#49906=DIRECTION ( 'NONE',  ( 0.5364919789714477361, 0.6444004775717706579, 0.5449076811759711036 ) ) ;
#49907=PLANE ( 'NONE',  #25502 ) ;
#49908=DIRECTION ( 'NONE',  ( 0.9999697198139515519, 0.000000000000000000, 0.007781995580013368816 ) ) ;
#49909=DIRECTION ( 'NONE',  ( -0.9999697198139514409, -0.000000000000000000, -0.007781995580013368816 ) ) ;
#49910=CARTESIAN_POINT ( 'NONE',  ( -16.81267852042391198, -0.1191753592594197858, 3.312241722634738039 ) ) ;
#49911=DIRECTION ( 'NONE',  ( 0.5364919789714477361, 0.6444004775717706579, 0.5449076811759711036 ) ) ;
#49912=LINE ( 'NONE', #41425, #49242 ) ;
#49913=EDGE_LOOP ( 'NONE', ( #55134, #17453, #44579, #50103 ) ) ;
#49914=CARTESIAN_POINT ( 'NONE',  ( -15.09804169372909399, 0.000000000000000000, 8.026899302267967329 ) ) ;
#49915=ORIENTED_EDGE ( 'NONE', *, *, #26987, .F. ) ;
#49916=DIRECTION ( 'NONE',  ( 0.9321478471874541372, 0.000000000000000000, -0.3620778797217453771 ) ) ;
#49917=CARTESIAN_POINT ( 'NONE',  ( -17.36532418587302473, -0.1191753592594177458, 13.67570816655714516 ) ) ;
#49918=CARTESIAN_POINT ( 'NONE',  ( 2.072287782118878319, 0.000000000000000000, -2.950529333540147015 ) ) ;
#49919=DIRECTION ( 'NONE',  ( 0.007781995580012662783, 0.000000000000000000, -0.9999697198139514409 ) ) ;
#49920=LINE ( 'NONE', #19005, #10548 ) ;
#49921=CARTESIAN_POINT ( 'NONE',  ( -18.67775241435682432, 0.000000000000000000, 4.136394454059623804 ) ) ;
#49922=EDGE_CURVE ( 'NONE', #20261, #52731, #29592, .T. ) ;
#49925=CARTESIAN_POINT ( 'NONE',  ( -20.08683635851538796, -0.1191753592594195638, 5.133421818297142281 ) ) ;
#49926=PLANE ( 'NONE',  #9403 ) ;
#49927=LINE ( 'NONE', #23554, #31265 ) ;
#49928=ADVANCED_FACE ( 'NONE', ( #33544 ), #8006, .F. ) ;
#49929=LINE ( 'NONE', #31796, #40907 ) ;
#49930=CARTESIAN_POINT ( 'NONE',  ( -21.47263955680318404, 0.000000000000000000, 5.022634149262071190 ) ) ;
#49931=VECTOR ( 'NONE', #35275, 1000.000000000000227 ) ;
#49932=EDGE_CURVE ( 'NONE', #16959, #35406, #50300, .T. ) ;
#49933=CARTESIAN_POINT ( 'NONE',  ( -12.13851405436063047, 0.000000000000000000, 11.68505802764555135 ) ) ;
#49934=DIRECTION ( 'NONE',  ( 0.5449076811759707706, 0.6444004775717708799, -0.5364919789714476250 ) ) ;
#49935=DIRECTION ( 'NONE',  ( -0.005002170337468016433, -0.7660444431189770143, 0.6427681459581293666 ) ) ;
#49936=EDGE_CURVE ( 'NONE', #50536, #44267, #46305, .T. ) ;
#49937=CARTESIAN_POINT ( 'NONE',  ( -23.33693525117809386, 0.000000000000000000, 5.746789908705562944 ) ) ;
#49938=VERTEX_POINT ( 'NONE', #2861 ) ;
#49939=VECTOR ( 'NONE', #28936, 1000.000000000000227 ) ;
#49940=FACE_OUTER_BOUND ( 'NONE', #450, .T. ) ;
#49941=EDGE_LOOP ( 'NONE', ( #45551, #28696, #38728, #35920 ) ) ;
#49942=CARTESIAN_POINT ( 'NONE',  ( -16.27758817276315284, 0.000000000000000000, 6.171059449791123086 ) ) ;
#49943=DIRECTION ( 'NONE',  ( 0.6427681459581294776, -0.7660444431189769032, 0.005002170337467562802 ) ) ;
#49944=ORIENTED_EDGE ( 'NONE', *, *, #20936, .T. ) ;
#49945=CARTESIAN_POINT ( 'NONE',  ( -11.67244013076689946, 0.000000000000000000, 11.50401908778467863 ) ) ;
#49946=ORIENTED_EDGE ( 'NONE', *, *, #5419, .T. ) ;
#49948=EDGE_CURVE ( 'NONE', #38604, #187, #16224, .T. ) ;
#49949=VERTEX_POINT ( 'NONE', #7160 ) ;
#49950=VERTEX_POINT ( 'NONE', #8263 ) ;
#49951=ORIENTED_EDGE ( 'NONE', *, *, #37584, .T. ) ;
#49952=CARTESIAN_POINT ( 'NONE',  ( -19.29729739867497074, 0.6102101463440047224, 4.158188481645193058 ) ) ;
#49953=CARTESIAN_POINT ( 'NONE',  ( -22.40556560354864146, -0.1191753592594197858, 5.484709000965211523 ) ) ;
#49954=CARTESIAN_POINT ( 'NONE',  ( 2.072287782118878319, 0.000000000000000000, -2.950529333540147015 ) ) ;
#49955=VECTOR ( 'NONE', #55906, 1000.000000000000114 ) ;
#49956=VECTOR ( 'NONE', #6830, 999.9999999999998863 ) ;
#49957=ORIENTED_EDGE ( 'NONE', *, *, #39830, .F. ) ;
#49958=ORIENTED_EDGE ( 'NONE', *, *, #5235, .T. ) ;
#49959=LINE ( 'NONE', #28389, #9157 ) ;
#49960=ORIENTED_EDGE ( 'NONE', *, *, #32084, .T. ) ;
#49961=CARTESIAN_POINT ( 'NONE',  ( -26.13415699229845757, -0.1191753592594197858, 6.933020519852192365 ) ) ;
#49962=ORIENTED_EDGE ( 'NONE', *, *, #40608, .T. ) ;
#49963=DIRECTION ( 'NONE',  ( 0.000000000000000000, -0.000000000000000000, -1.000000000000000000 ) ) ;
#49964=DIRECTION ( 'NONE',  ( -0.5364919789714478471, 0.6444004775717705469, -0.5449076811759709926 ) ) ;
#49966=VECTOR ( 'NONE', #40293, 999.9999999999998863 ) ;
#49967=LINE ( 'NONE', #20145, #18266 ) ;
#49970=CARTESIAN_POINT ( 'NONE',  ( -12.80458192191714595, 0.000000000000000000, 11.86454056839041726 ) ) ;
#49971=ORIENTED_EDGE ( 'NONE', *, *, #35542, .T. ) ;
#49972=LINE ( 'NONE', #11079, #51358 ) ;
#49973=DIRECTION ( 'NONE',  ( 0.5364919789714477361, 0.6444004775717706579, 0.5449076811759711036 ) ) ;
#49974=CARTESIAN_POINT ( 'NONE',  ( -20.54049170961573267, 0.000000000000000000, 4.660556269540326646 ) ) ;
#49976=ADVANCED_FACE ( 'NONE', ( #54843 ), #41519, .F. ) ;
#49977=CARTESIAN_POINT ( 'NONE',  ( -13.36481033154660913, 0.000000000000000000, 8.409719779305810050 ) ) ;
#49978=FACE_OUTER_BOUND ( 'NONE', #44811, .T. ) ;
#49979=DIRECTION ( 'NONE',  ( -0.5449076811759708816, 0.6444004775717707689, 0.5364919789714475140 ) ) ;
#49980=CARTESIAN_POINT ( 'NONE',  ( -9.037643660258000367, 0.000000000000000000, 5.488738232447742504 ) ) ;
#49981=EDGE_CURVE ( 'NONE', #26517, #7643, #16495, .T. ) ;
#49983=DIRECTION ( 'NONE',  ( -0.9999697198139514409, -0.000000000000000000, -0.007781995580013368816 ) ) ;
#49984=ADVANCED_FACE ( 'NONE', ( #15952 ), #33291, .F. ) ;
#49986=EDGE_LOOP ( 'NONE', ( #9566, #44979, #1324, #49556 ) ) ;
#49987=DIRECTION ( 'NONE',  ( 0.000000000000000000, -0.000000000000000000, -1.000000000000000000 ) ) ;
#49988=LINE ( 'NONE', #50580, #16833 ) ;
#49990=ORIENTED_EDGE ( 'NONE', *, *, #33239, .T. ) ;
#49991=CARTESIAN_POINT ( 'NONE',  ( -12.37340416382502539, 4.495856970884011261, 9.066038720008986473 ) ) ;
#49992=EDGE_CURVE ( 'NONE', #47218, #45990, #21336, .T. ) ;
#49993=LINE ( 'NONE', #2590, #39056 ) ;
#49994=AXIS2_PLACEMENT_3D ( 'NONE', #27395, #1269, #31941 ) ;
#49995=AXIS2_PLACEMENT_3D ( 'NONE', #5378, #48820, #9921 ) ;
#49996=EDGE_CURVE ( 'NONE', #30649, #54306, #13396, .T. ) ;
#49997=CARTESIAN_POINT ( 'NONE',  ( -15.88053067323646417, -0.1191753592594197858, 2.950163842912994383 ) ) ;
#49998=CARTESIAN_POINT ( 'NONE',  ( -16.47913851584194234, 0.000000000000000000, 6.369496994637906973 ) ) ;
#50000=CARTESIAN_POINT ( 'NONE',  ( -18.72338561947129065, 5.467268677019013090, 3.780296059854713953 ) ) ;
#50001=ORIENTED_EDGE ( 'NONE', *, *, #20483, .F. ) ;
#50002=AXIS2_PLACEMENT_3D ( 'NONE', #47034, #51574, #51832 ) ;
#50003=ORIENTED_EDGE ( 'NONE', *, *, #53680, .T. ) ;
#50005=LINE ( 'NONE', #41516, #7560 ) ;
#50006=EDGE_CURVE ( 'NONE', #25279, #3929, #43735, .T. ) ;
#50007=ORIENTED_EDGE ( 'NONE', *, *, #35845, .F. ) ;
#50008=CARTESIAN_POINT ( 'NONE',  ( -13.08330893211609869, 0.000000000000000000, 1.763933231766363630 ) ) ;
#50009=ORIENTED_EDGE ( 'NONE', *, *, #35347, .F. ) ;
#50010=CARTESIAN_POINT ( 'NONE',  ( -20.54204810873173415, 0.000000000000000000, 4.860550213503115558 ) ) ;
#50011=VECTOR ( 'NONE', #8435, 999.9999999999998863 ) ;
#50012=ADVANCED_FACE ( 'NONE', ( #17082 ), #4314, .F. ) ;
#50013=ORIENTED_EDGE ( 'NONE', *, *, #38039, .T. ) ;
#50014=ORIENTED_EDGE ( 'NONE', *, *, #54831, .T. ) ;
#50015=PLANE ( 'NONE',  #39325 ) ;
#50016=CARTESIAN_POINT ( 'NONE',  ( -18.67619601524082285, 0.000000000000000000, 3.936400510096834893 ) ) ;
#50017=CARTESIAN_POINT ( 'NONE',  ( -19.32961685222932147, 0.000000000000000000, 14.39908572644263351 ) ) ;
#50018=EDGE_LOOP ( 'NONE', ( #21195, #25061, #29002, #31278 ) ) ;
#50019=FACE_OUTER_BOUND ( 'NONE', #52292, .T. ) ;
#50020=ORIENTED_EDGE ( 'NONE', *, *, #38894, .F. ) ;
#50021=ORIENTED_EDGE ( 'NONE', *, *, #30945, .T. ) ;
#50022=EDGE_LOOP ( 'NONE', ( #12040, #44993, #54368, #50026, #17714, #30375, #31209 ) ) ;
#50023=CARTESIAN_POINT ( 'NONE',  ( -17.62763697264768226, -0.5179957512181538881, 4.379223844503182583 ) ) ;
#50024=ORIENTED_EDGE ( 'NONE', *, *, #47743, .T. ) ;
#50025=DIRECTION ( 'NONE',  ( 0.000000000000000000, -1.000000000000000000, 0.000000000000000000 ) ) ;
#50026=ORIENTED_EDGE ( 'NONE', *, *, #21805, .F. ) ;
#50027=LINE ( 'NONE', #36428, #3179 ) ;
#50028=CARTESIAN_POINT ( 'NONE',  ( -16.96808549511456832, 0.000000000000000000, 9.489674468226988679 ) ) ;
#50029=VECTOR ( 'NONE', #6661, 999.9999999999998863 ) ;
#50030=VECTOR ( 'NONE', #3750, 999.9999999999998863 ) ;
#50031=ORIENTED_EDGE ( 'NONE', *, *, #21630, .F. ) ;
#50032=DIRECTION ( 'NONE',  ( 0.7660212471507180654, -0.6427876096865404731, 0.005961354470445141482 ) ) ;
#50033=EDGE_CURVE ( 'NONE', #18681, #16694, #38665, .T. ) ;
#50034=EDGE_LOOP ( 'NONE', ( #10674, #50021, #48764, #8146 ) ) ;
#50035=DIRECTION ( 'NONE',  ( -0.5449076811759708816, 0.6444004775717707689, 0.5364919789714475140 ) ) ;
#50036=DIRECTION ( 'NONE',  ( 0.9999697198139515519, 0.000000000000000000, 0.007781995580013368816 ) ) ;
#50037=VECTOR ( 'NONE', #40374, 1000.000000000000227 ) ;
#50038=CARTESIAN_POINT ( 'NONE',  ( -18.59083284206345610, 0.000000000000000000, 4.875735021882804610 ) ) ;
#50040=CARTESIAN_POINT ( 'NONE',  ( -12.33850799832341849, 0.000000000000000000, 11.68350162852954632 ) ) ;
#50041=DIRECTION ( 'NONE',  ( 0.5364919789714477361, 0.6444004775717706579, 0.5449076811759711036 ) ) ;
#50042=DIRECTION ( 'NONE',  ( 0.005002170337468016433, -0.7660444431189770143, -0.6427681459581293666 ) ) ;
#50043=ORIENTED_EDGE ( 'NONE', *, *, #32256, .F. ) ;
#50044=EDGE_CURVE ( 'NONE', #19093, #19489, #5152, .T. ) ;
#50045=ADVANCED_FACE ( 'NONE', ( #47751 ), #35502, .F. ) ;
#50046=ORIENTED_EDGE ( 'NONE', *, *, #49936, .T. ) ;
#50047=CARTESIAN_POINT ( 'NONE',  ( -18.36355258475382612, 0.000000000000000000, 9.678820676885749208 ) ) ;
#50048=CARTESIAN_POINT ( 'NONE',  ( -13.36006324802803569, 3.524445264749011208, 1.758985750240432022 ) ) ;
#50049=AXIS2_PLACEMENT_3D ( 'NONE', #39390, #35153, #52448 ) ;
#50051=DIRECTION ( 'NONE',  ( 0.007781995580012662783, 0.000000000000000000, -0.9999697198139514409 ) ) ;
#50052=ADVANCED_FACE ( 'NONE', ( #39506 ), #34658, .F. ) ;
#50053=CARTESIAN_POINT ( 'NONE',  ( -10.68470108963842868, 0.000000000000000000, 3.998592171460650047 ) ) ;
#50054=ORIENTED_EDGE ( 'NONE', *, *, #12364, .T. ) ;
#50055=DIRECTION ( 'NONE',  ( 0.005961354470445682716, -0.6427876096865404731, -0.7660212471507180654 ) ) ;
#50056=LINE ( 'NONE', #41286, #22335 ) ;
#50057=ORIENTED_EDGE ( 'NONE', *, *, #14260, .F. ) ;
#50058=DIRECTION ( 'NONE',  ( 0.007781995580012663651, -3.146120232559066537E-19, -0.9999697198139514409 ) ) ;
#50059=LINE ( 'NONE', #11738, #19559 ) ;
#50060=EDGE_LOOP ( 'NONE', ( #55952, #14099, #12758, #34223 ) ) ;
#50061=LINE ( 'NONE', #14893, #18902 ) ;
#50062=PLANE ( 'NONE',  #51438 ) ;
#50063=EDGE_CURVE ( 'NONE', #33161, #29115, #22171, .T. ) ;
#50064=DIRECTION ( 'NONE',  ( 0.9999697198139515519, 0.000000000000000000, 0.007781995580013368816 ) ) ;
#50065=VECTOR ( 'NONE', #31605, 1000.000000000000114 ) ;
#50066=CARTESIAN_POINT ( 'NONE',  ( 2.072287782118878319, 0.000000000000000000, -2.950529333540147015 ) ) ;
#50067=ADVANCED_FACE ( 'NONE', ( #4848 ), #25888, .F. ) ;
#50068=CARTESIAN_POINT ( 'NONE',  ( -15.40103151951671734, 0.000000000000000000, 12.95233060667165681 ) ) ;
#50069=ORIENTED_EDGE ( 'NONE', *, *, #42118, .F. ) ;
#50070=EDGE_LOOP ( 'NONE', ( #20736, #14455, #11883, #34992 ) ) ;
#50071=ADVANCED_FACE ( 'NONE', ( #17632 ), #42902, .F. ) ;
#50072=LINE ( 'NONE', #36772, #26667 ) ;
#50073=DIRECTION ( 'NONE',  ( 0.007781995580012662783, 0.000000000000000000, -0.9999697198139514409 ) ) ;
#50075=DIRECTION ( 'NONE',  ( 0.9999697198139515519, 0.000000000000000000, 0.007781995580013368816 ) ) ;
#50076=VECTOR ( 'NONE', #11626, 1000.000000000000227 ) ;
#50077=DIRECTION ( 'NONE',  ( 0.5449076811759707706, 0.6444004775717708799, -0.5364919789714476250 ) ) ;
#50078=EDGE_CURVE ( 'NONE', #33009, #35551, #47444, .T. ) ;
#50079=VECTOR ( 'NONE', #29557, 1000.000000000000227 ) ;
#50080=DIRECTION ( 'NONE',  ( -0.005002170337468016433, -0.7660444431189770143, 0.6427681459581293666 ) ) ;
#50081=DIRECTION ( 'NONE',  ( -0.9999697198139514409, -0.000000000000000000, -0.007781995580013368816 ) ) ;
#50082=EDGE_LOOP ( 'NONE', ( #33429, #20455, #39296, #55346 ) ) ;
#50083=FACE_OUTER_BOUND ( 'NONE', #52917, .T. ) ;
#50084=FACE_OUTER_BOUND ( 'NONE', #8622, .T. ) ;
#50085=AXIS2_PLACEMENT_3D ( 'NONE', #12743, #11632, #33223 ) ;
#50086=LINE ( 'NONE', #24529, #12408 ) ;
#50087=VECTOR ( 'NONE', #1626, 1000.000000000000227 ) ;
#50088=VERTEX_POINT ( 'NONE', #38940 ) ;
#50090=DIRECTION ( 'NONE',  ( 0.000000000000000000, -0.000000000000000000, -1.000000000000000000 ) ) ;
#50091=CARTESIAN_POINT ( 'NONE',  ( -18.19747506107908563, 0.000000000000000000, 14.03856424583689311 ) ) ;
#50092=ORIENTED_EDGE ( 'NONE', *, *, #36228, .T. ) ;
#50093=CARTESIAN_POINT ( 'NONE',  ( -17.42410023143980879, 0.000000000000000000, 8.378129446685687043 ) ) ;
#50094=VECTOR ( 'NONE', #52388, 999.9999999999998863 ) ;
#50095=ORIENTED_EDGE ( 'NONE', *, *, #1682, .T. ) ;
#50096=ORIENTED_EDGE ( 'NONE', *, *, #51024, .F. ) ;
#50097=ORIENTED_EDGE ( 'NONE', *, *, #42760, .F. ) ;
#50098=EDGE_LOOP ( 'NONE', ( #45483, #34661, #17148, #30215 ) ) ;
#50099=EDGE_LOOP ( 'NONE', ( #17612, #47837, #9400, #48364 ) ) ;
#50100=LINE ( 'NONE', #28538, #51072 ) ;
#50101=ORIENTED_EDGE ( 'NONE', *, *, #41489, .F. ) ;
#50102=ADVANCED_FACE ( 'NONE', ( #7 ), #13095, .F. ) ;
#50103=ORIENTED_EDGE ( 'NONE', *, *, #46994, .F. ) ;
#50104=PLANE ( 'NONE',  #32263 ) ;
#50105=ORIENTED_EDGE ( 'NONE', *, *, #6944, .F. ) ;
#50106=EDGE_CURVE ( 'NONE', #49029, #51817, #599, .T. ) ;
#50107=VECTOR ( 'NONE', #52539, 999.9999999999998863 ) ;
#50108=ORIENTED_EDGE ( 'NONE', *, *, #4124, .T. ) ;
#50109=EDGE_LOOP ( 'NONE', ( #45352, #54487, #10790, #26503 ) ) ;
#50110=LINE ( 'NONE', #6994, #17620 ) ;
#50111=CARTESIAN_POINT ( 'NONE',  ( -15.07217521218155021, 0.000000000000000000, 4.703111972948089914 ) ) ;
#50113=CARTESIAN_POINT ( 'NONE',  ( -23.33771345073609638, -0.1191753592594197858, 5.846786880686956955 ) ) ;
#50115=CARTESIAN_POINT ( 'NONE',  ( -18.19747506107908563, 0.000000000000000000, 14.03856424583689311 ) ) ;
#50116=EDGE_LOOP ( 'NONE', ( #6465, #30647, #49147, #51730 ) ) ;
#50117=ADVANCED_FACE ( 'NONE', ( #21882 ), #52545, .F. ) ;
#50118=EDGE_CURVE ( 'NONE', #48023, #40238, #41265, .T. ) ;
#50119=EDGE_CURVE ( 'NONE', #16052, #4269, #6524, .T. ) ;
#50120=AXIS2_PLACEMENT_3D ( 'NONE', #22026, #34522, #26860 ) ;
#50121=AXIS2_PLACEMENT_3D ( 'NONE', #29777, #52463, #13295 ) ;
#50122=ORIENTED_EDGE ( 'NONE', *, *, #22297, .T. ) ;
#50123=DIRECTION ( 'NONE',  ( 0.007781995580012663651, -3.146120232559066537E-19, -0.9999697198139514409 ) ) ;
#50124=DIRECTION ( 'NONE',  ( 0.7660212471507180654, -0.6427876096865404731, 0.005961354470445141482 ) ) ;
#50126=EDGE_CURVE ( 'NONE', #6083, #25619, #36346, .T. ) ;
#50128=VECTOR ( 'NONE', #31686, 1000.000000000000114 ) ;
#50129=AXIS2_PLACEMENT_3D ( 'NONE', #11103, #41752, #23887 ) ;
#50130=LINE ( 'NONE', #45595, #37606 ) ;
#50131=CARTESIAN_POINT ( 'NONE',  ( -16.53317331066696383, 0.000000000000000000, 13.31285208727739899 ) ) ;
#50132=DIRECTION ( 'NONE',  ( -0.6246952433987893460, -0.7422098413412802076, 0.2426528472758542054 ) ) ;
#50133=VERTEX_POINT ( 'NONE', #40629 ) ;
#50134=LINE ( 'NONE', #41366, #18390 ) ;
#50135=ORIENTED_EDGE ( 'NONE', *, *, #12209, .T. ) ;
#50136=FACE_OUTER_BOUND ( 'NONE', #18881, .T. ) ;
#50137=CARTESIAN_POINT ( 'NONE',  ( -10.07321481412883912, -0.2242460341567873994, 1.060529934425493259 ) ) ;
#50139=AXIS2_PLACEMENT_3D ( 'NONE', #5647, #18145, #5950 ) ;
#50141=VECTOR ( 'NONE', #160, 1000.000000000000000 ) ;
#50142=ADVANCED_FACE ( 'NONE', ( #14237 ), #1126, .F. ) ;
#50143=CARTESIAN_POINT ( 'NONE',  ( -18.67697421479882181, -0.1191753592594197858, 4.036397482078229793 ) ) ;
#50144=ADVANCED_FACE ( 'NONE', ( #35803 ), #14495, .F. ) ;
#50146=ADVANCED_FACE ( 'NONE', ( #10227 ), #45411, .F. ) ;
#50147=CARTESIAN_POINT ( 'NONE',  ( -16.38920120867433639, -3.432230869623160263, 8.680929647428692775 ) ) ;
#50148=DIRECTION ( 'NONE',  ( 0.000000000000000000, -1.000000000000000000, 0.000000000000000000 ) ) ;
#50149=DIRECTION ( 'NONE',  ( -0.5364919789714478471, 0.6444004775717705469, -0.5449076811759709926 ) ) ;
#50150=VECTOR ( 'NONE', #25151, 1000.000000000000227 ) ;
#50151=EDGE_CURVE ( 'NONE', #29873, #9919, #19026, .T. ) ;
#50152=CARTESIAN_POINT ( 'NONE',  ( -25.20200914511100265, -0.1191753592594197858, 6.570942640130446932 ) ) ;
#50153=LINE ( 'NONE', #33971, #23074 ) ;
#50154=AXIS2_PLACEMENT_3D ( 'NONE', #23901, #44635, #14303 ) ;
#50155=DIRECTION ( 'NONE',  ( 0.000000000000000000, -0.000000000000000000, -1.000000000000000000 ) ) ;
#50156=DIRECTION ( 'NONE',  ( 0.007781995580012663651, 0.000000000000000000, -0.9999697198139515519 ) ) ;
#50157=EDGE_CURVE ( 'NONE', #6183, #30608, #44868, .T. ) ;
#50159=VECTOR ( 'NONE', #50237, 1000.000000000000227 ) ;
#50160=DIRECTION ( 'NONE',  ( 0.6246952433987894571, -0.7422098413412800966, -0.2426528472758541777 ) ) ;
#50161=EDGE_LOOP ( 'NONE', ( #28249, #19856, #11515, #1722 ) ) ;
#50162=VECTOR ( 'NONE', #9137, 999.9999999999998863 ) ;
#50164=VECTOR ( 'NONE', #2079, 1000.000000000000227 ) ;
#50165=ORIENTED_EDGE ( 'NONE', *, *, #45596, .T. ) ;
#50166=AXIS2_PLACEMENT_3D ( 'NONE', #46533, #28113, #40890 ) ;
#50167=ORIENTED_EDGE ( 'NONE', *, *, #18726, .F. ) ;
#50168=ORIENTED_EDGE ( 'NONE', *, *, #35887, .T. ) ;
#50169=VECTOR ( 'NONE', #51360, 1000.000000000000227 ) ;
#50170=ORIENTED_EDGE ( 'NONE', *, *, #1654, .F. ) ;
#50171=ORIENTED_EDGE ( 'NONE', *, *, #9856, .F. ) ;
#50172=CARTESIAN_POINT ( 'NONE',  ( 2.072287782118878319, 0.000000000000000000, -2.950529333540147015 ) ) ;
#50173=DIRECTION ( 'NONE',  ( 0.5449076811759707706, 0.6444004775717708799, -0.5364919789714476250 ) ) ;
#50174=FACE_OUTER_BOUND ( 'NONE', #30067, .T. ) ;
#50176=DIRECTION ( 'NONE',  ( -0.5364919789714478471, 0.6444004775717705469, -0.5449076811759709926 ) ) ;
#50177=ORIENTED_EDGE ( 'NONE', *, *, #27090, .T. ) ;
#50178=ORIENTED_EDGE ( 'NONE', *, *, #34890, .F. ) ;
#50180=VECTOR ( 'NONE', #12279, 1000.000000000000227 ) ;
#50181=CARTESIAN_POINT ( 'NONE',  ( -10.00813838035478298, 0.000000000000000000, 10.77830692922518452 ) ) ;
#50182=CARTESIAN_POINT ( 'NONE',  ( -16.79925329029790149, 0.000000000000000000, 13.49544742625427496 ) ) ;
#50183=ORIENTED_EDGE ( 'NONE', *, *, #24102, .F. ) ;
#50184=LINE ( 'NONE', #23788, #7413 ) ;
#50185=AXIS2_PLACEMENT_3D ( 'NONE', #26318, #34557, #13551 ) ;
#50186=ORIENTED_EDGE ( 'NONE', *, *, #32299, .T. ) ;
#50187=EDGE_CURVE ( 'NONE', #45704, #21256, #27261, .T. ) ;
#50188=CARTESIAN_POINT ( 'NONE',  ( -10.23599085943975595, 0.000000000000000000, 6.048750543480270636 ) ) ;
#50189=FACE_OUTER_BOUND ( 'NONE', #30722, .T. ) ;
#50190=VECTOR ( 'NONE', #50805, 1000.000000000000227 ) ;
#50191=EDGE_CURVE ( 'NONE', #32397, #37255, #45165, .T. ) ;
#50192=ADVANCED_FACE ( 'NONE', ( #23308 ), #6266, .F. ) ;
#50193=LINE ( 'NONE', #6487, #29033 ) ;
#50194=FACE_OUTER_BOUND ( 'NONE', #28157, .T. ) ;
#50195=DIRECTION ( 'NONE',  ( 0.5364919789714477361, 0.6444004775717706579, 0.5449076811759711036 ) ) ;
#50196=LINE ( 'NONE', #1667, #24721 ) ;
#50197=DIRECTION ( 'NONE',  ( 0.5449076811759707706, 0.6444004775717708799, -0.5364919789714476250 ) ) ;
#50198=CARTESIAN_POINT ( 'NONE',  ( -19.52429834364018646, 0.000000000000000000, 5.407128660899526373 ) ) ;
#50199=VECTOR ( 'NONE', #11764, 1000.000000000000227 ) ;
#50200=FACE_OUTER_BOUND ( 'NONE', #11203, .T. ) ;
#50201=ORIENTED_EDGE ( 'NONE', *, *, #20362, .T. ) ;
#50203=EDGE_LOOP ( 'NONE', ( #40066, #3935, #25559, #52544 ) ) ;
#50204=AXIS2_PLACEMENT_3D ( 'NONE', #34697, #52016, #39545 ) ;
#50205=LINE ( 'NONE', #11314, #11097 ) ;
#50206=DIRECTION ( 'NONE',  ( -0.9999697198139514409, -0.000000000000000000, -0.007781995580013368816 ) ) ;
#50207=LINE ( 'NONE', #50511, #3271 ) ;
#50208=PLANE ( 'NONE',  #44092 ) ;
#50209=DIRECTION ( 'NONE',  ( 0.007781995580012663651, -3.146120232559066537E-19, -0.9999697198139514409 ) ) ;
#50210=AXIS2_PLACEMENT_3D ( 'NONE', #31698, #40201, #1596 ) ;
#50212=VECTOR ( 'NONE', #12938, 1000.000000000000227 ) ;
#50213=ORIENTED_EDGE ( 'NONE', *, *, #38620, .T. ) ;
#50214=CARTESIAN_POINT ( 'NONE',  ( -25.20123094555300369, 0.000000000000000000, 6.470945668149052032 ) ) ;
#50215=CARTESIAN_POINT ( 'NONE',  ( -21.80678505063549011, 3.038739411681508518, 5.055475909915189803 ) ) ;
#50216=DIRECTION ( 'NONE',  ( 0.005002170337468016433, -0.7660444431189770143, -0.6427681459581293666 ) ) ;
#50217=DIRECTION ( 'NONE',  ( -0.5449076811759708816, 0.6444004775717707689, 0.5364919789714475140 ) ) ;
#50218=DIRECTION ( 'NONE',  ( -0.005961354470445682716, -0.6427876096865404731, 0.7660212471507180654 ) ) ;
#50219=LINE ( 'NONE', #7935, #36394 ) ;
#50220=DIRECTION ( 'NONE',  ( 0.005002170337468016433, -0.7660444431189770143, -0.6427681459581293666 ) ) ;
#50221=ADVANCED_FACE ( 'NONE', ( #9691 ), #19294, .F. ) ;
#50222=DIRECTION ( 'NONE',  ( 0.007781995580012662783, 0.000000000000000000, -0.9999697198139514409 ) ) ;
#50223=CARTESIAN_POINT ( 'NONE',  ( -9.075990533167328067, 0.000000000000000000, 10.41622904950343909 ) ) ;
#50224=VERTEX_POINT ( 'NONE', #36633 ) ;
#50225=CARTESIAN_POINT ( 'NONE',  ( -11.37232435848456191, 0.000000000000000000, 6.947897486638751730 ) ) ;
#50226=EDGE_LOOP ( 'NONE', ( #3969, #28761, #25413, #27576, #20865 ) ) ;
#50227=VECTOR ( 'NONE', #30140, 1000.000000000000227 ) ;
#50228=ADVANCED_FACE ( 'NONE', ( #53946 ), #15062, .F. ) ;
#50229=DIRECTION ( 'NONE',  ( -0.3620778797217455991, 0.000000000000000000, -0.9321478471874540261 ) ) ;
#50230=LINE ( 'NONE', #52890, #40076 ) ;
#50231=EDGE_CURVE ( 'NONE', #21366, #26301, #49699, .T. ) ;
#50232=VECTOR ( 'NONE', #11160, 1000.000000000000000 ) ;
#50233=ORIENTED_EDGE ( 'NONE', *, *, #46552, .F. ) ;
#50234=ADVANCED_FACE ( 'NONE', ( #54228 ), #27006, .F. ) ;
#50235=VECTOR ( 'NONE', #47924, 1000.000000000000114 ) ;
#50236=ORIENTED_EDGE ( 'NONE', *, *, #56053, .F. ) ;
#50237=DIRECTION ( 'NONE',  ( 0.007781995580012662783, 0.000000000000000000, -0.9999697198139514409 ) ) ;
#50238=ORIENTED_EDGE ( 'NONE', *, *, #3418, .F. ) ;
#50239=ORIENTED_EDGE ( 'NONE', *, *, #29371, .F. ) ;
#50241=PLANE ( 'NONE',  #51062 ) ;
#50242=VECTOR ( 'NONE', #33552, 999.9999999999998863 ) ;
#50244=DIRECTION ( 'NONE',  ( -0.7660212471507179544, -0.6427876096865405842, -0.005961354470445141482 ) ) ;
#50246=ORIENTED_EDGE ( 'NONE', *, *, #10194, .F. ) ;
#50247=EDGE_LOOP ( 'NONE', ( #32103, #30713, #24202, #28752 ) ) ;
#50248=VECTOR ( 'NONE', #18381, 1000.000000000000227 ) ;
#50250=LINE ( 'NONE', #42006, #50190 ) ;
#50251=CARTESIAN_POINT ( 'NONE',  ( -13.46921766719642122, -1.651309408375655874, 4.623913353405106008 ) ) ;
#50252=ORIENTED_EDGE ( 'NONE', *, *, #26319, .F. ) ;
#50253=CARTESIAN_POINT ( 'NONE',  ( -17.36532418587302473, -0.1191753592594177458, 13.67570816655714516 ) ) ;
#50254=EDGE_CURVE ( 'NONE', #29163, #441, #51303, .T. ) ;
#50255=EDGE_LOOP ( 'NONE', ( #32916, #41624, #13034, #1063 ) ) ;
#50257=LINE ( 'NONE', #36659, #24904 ) ;
#50258=EDGE_CURVE ( 'NONE', #14573, #21242, #46448, .T. ) ;
#50259=EDGE_LOOP ( 'NONE', ( #34850, #45870, #1012, #12798 ) ) ;
#50260=DIRECTION ( 'NONE',  ( -0.005002170337468016433, -0.7660444431189770143, 0.6427681459581293666 ) ) ;
#50261=EDGE_CURVE ( 'NONE', #33384, #18589, #21761, .T. ) ;
#50263=VECTOR ( 'NONE', #44757, 1000.000000000000000 ) ;
#50264=DIRECTION ( 'NONE',  ( 0.000000000000000000, 1.000000000000000000, 0.000000000000000000 ) ) ;
#50265=VERTEX_POINT ( 'NONE', #47603 ) ;
#50266=CARTESIAN_POINT ( 'NONE',  ( -16.41880516715173144, -0.1941918491731536578, 3.378255151246715826 ) ) ;
#50267=VECTOR ( 'NONE', #46859, 1000.000000000000227 ) ;
#50268=CARTESIAN_POINT ( 'NONE',  ( -17.39248564288169874, 0.000000000000000000, 4.315722710850279142 ) ) ;
#50269=EDGE_LOOP ( 'NONE', ( #23628, #24808, #34065, #51198 ) ) ;
#50270=VECTOR ( 'NONE', #38404, 1000.000000000000000 ) ;
#50271=DIRECTION ( 'NONE',  ( 0.000000000000000000, -1.000000000000000000, 0.000000000000000000 ) ) ;
#50272=LINE ( 'NONE', #55656, #10621 ) ;
#50273=FACE_OUTER_BOUND ( 'NONE', #15827, .T. ) ;
#50274=LINE ( 'NONE', #15106, #17754 ) ;
#50275=LINE ( 'NONE', #11388, #10432 ) ;
#50276=CARTESIAN_POINT ( 'NONE',  ( -27.06708303904391144, 0.000000000000000000, 7.395095371555332697 ) ) ;
#50277=EDGE_CURVE ( 'NONE', #34543, #43670, #50992, .T. ) ;
#50278=CARTESIAN_POINT ( 'NONE',  ( -16.49129718093630004, -2.460819163488158878, 7.126335086546274233 ) ) ;
#50279=VECTOR ( 'NONE', #13494, 1000.000000000000227 ) ;
#50280=ORIENTED_EDGE ( 'NONE', *, *, #28036, .T. ) ;
#50282=DIRECTION ( 'NONE',  ( 0.007781995580012662783, 0.000000000000000000, -0.9999697198139514409 ) ) ;
#50284=ORIENTED_EDGE ( 'NONE', *, *, #36546, .F. ) ;
#50285=VECTOR ( 'NONE', #13039, 1000.000000000000227 ) ;
#50286=DIRECTION ( 'NONE',  ( 0.007781995580012663651, -3.146120232559066537E-19, -0.9999697198139514409 ) ) ;
#50287=FACE_OUTER_BOUND ( 'NONE', #40828, .T. ) ;
#50288=VECTOR ( 'NONE', #20544, 1000.000000000000000 ) ;
#50289=LINE ( 'NONE', #45748, #44910 ) ;
#50290=DIRECTION ( 'NONE',  ( -0.5449076811759708816, 0.6444004775717707689, 0.5364919789714475140 ) ) ;
#50291=DIRECTION ( 'NONE',  ( 0.9999697198139515519, 0.000000000000000000, 0.007781995580013368816 ) ) ;
#50292=ORIENTED_EDGE ( 'NONE', *, *, #12982, .T. ) ;
#50293=VECTOR ( 'NONE', #3785, 1000.000000000000114 ) ;
#50294=VECTOR ( 'NONE', #47095, 999.9999999999998863 ) ;
#50295=VERTEX_POINT ( 'NONE', #3862 ) ;
#50296=DIRECTION ( 'NONE',  ( 0.000000000000000000, -0.000000000000000000, -1.000000000000000000 ) ) ;
#50297=CARTESIAN_POINT ( 'NONE',  ( -15.13495153988577968, 0.000000000000000000, 12.76973526769478084 ) ) ;
#50298=CARTESIAN_POINT ( 'NONE',  ( -15.47473988553288038, -0.1159828484229817602, 9.229288071583351183 ) ) ;
#50299=VERTEX_POINT ( 'NONE', #12955 ) ;
#50300=LINE ( 'NONE', #38363, #40379 ) ;
#50301=EDGE_CURVE ( 'NONE', #44396, #1167, #34531, .T. ) ;
#50302=ORIENTED_EDGE ( 'NONE', *, *, #825, .F. ) ;
#50303=DIRECTION ( 'NONE',  ( 0.000000000000000000, 0.000000000000000000, 1.000000000000000000 ) ) ;
#50304=VECTOR ( 'NONE', #35488, 1000.000000000000227 ) ;
#50305=EDGE_LOOP ( 'NONE', ( #3389, #56148, #37798, #12622 ) ) ;
#50306=ORIENTED_EDGE ( 'NONE', *, *, #15636, .F. ) ;
#50307=VECTOR ( 'NONE', #10699, 1000.000000000000227 ) ;
#50308=LINE ( 'NONE', #11957, #32073 ) ;
#50310=VECTOR ( 'NONE', #419, 1000.000000000000227 ) ;
#50311=LINE ( 'NONE', #28755, #35749 ) ;
#50312=ADVANCED_FACE ( 'NONE', ( #20648 ), #51841, .F. ) ;
#50313=ORIENTED_EDGE ( 'NONE', *, *, #15953, .T. ) ;
#50315=AXIS2_PLACEMENT_3D ( 'NONE', #17593, #4808, #48232 ) ;
#50316=ORIENTED_EDGE ( 'NONE', *, *, #1072, .T. ) ;
#50317=EDGE_CURVE ( 'NONE', #8089, #54118, #42758, .T. ) ;
#50320=ORIENTED_EDGE ( 'NONE', *, *, #7502, .F. ) ;
#50321=AXIS2_PLACEMENT_3D ( 'NONE', #4226, #25237, #30330 ) ;
#50322=FACE_OUTER_BOUND ( 'NONE', #2120, .T. ) ;
#50323=AXIS2_PLACEMENT_3D ( 'NONE', #41817, #15699, #11731 ) ;
#50324=PLANE ( 'NONE',  #24031 ) ;
#50325=ORIENTED_EDGE ( 'NONE', *, *, #21286, .F. ) ;
#50326=VECTOR ( 'NONE', #17746, 999.9999999999998863 ) ;
#50327=DIRECTION ( 'NONE',  ( 0.9999697198139515519, 0.000000000000000000, 0.007781995580013368816 ) ) ;
#50328=EDGE_CURVE ( 'NONE', #4025, #42332, #8722, .T. ) ;
#50330=LINE ( 'NONE', #32720, #53936 ) ;
#50331=CARTESIAN_POINT ( 'NONE',  ( -12.91584975057942941, -1.003701604285655469, 3.346131726335665579 ) ) ;
#50332=AXIS2_PLACEMENT_3D ( 'NONE', #13967, #18504, #14531 ) ;
#50333=ORIENTED_EDGE ( 'NONE', *, *, #38781, .F. ) ;
#50334=ADVANCED_FACE ( 'NONE', ( #4450 ), #11822, .F. ) ;
#50335=DIRECTION ( 'NONE',  ( -0.6427681459581293666, -0.7660444431189770143, -0.005002170337467561935 ) ) ;
#50336=EDGE_LOOP ( 'NONE', ( #49711, #17163, #28367, #32436 ) ) ;
#50337=EDGE_CURVE ( 'NONE', #38002, #47502, #12682, .T. ) ;
#50338=AXIS2_PLACEMENT_3D ( 'NONE', #31809, #48861, #10797 ) ;
#50339=CARTESIAN_POINT ( 'NONE',  ( -15.65072360821981334, 2.876837460659007473, 7.681974050944107013 ) ) ;
#50340=VECTOR ( 'NONE', #33118, 999.9999999999998863 ) ;
#50342=LINE ( 'NONE', #50627, #35038 ) ;
#50344=DIRECTION ( 'NONE',  ( -0.005002170337468016433, -0.7660444431189770143, 0.6427681459581293666 ) ) ;
#50345=DIRECTION ( 'NONE',  ( 0.9999697198139515519, 0.000000000000000000, 0.007781995580013368816 ) ) ;
#50346=ORIENTED_EDGE ( 'NONE', *, *, #135, .T. ) ;
#50347=EDGE_CURVE ( 'NONE', #4182, #43916, #55267, .T. ) ;
#50348=ORIENTED_EDGE ( 'NONE', *, *, #1798, .F. ) ;
#50349=CARTESIAN_POINT ( 'NONE',  ( 2.072287782118878319, 0.000000000000000000, -2.950529333540147015 ) ) ;
#50350=LINE ( 'NONE', #6931, #25764 ) ;
#50351=CARTESIAN_POINT ( 'NONE',  ( -22.40556560354864146, -0.1191753592594197858, 5.484709000965211523 ) ) ;
#50352=DIRECTION ( 'NONE',  ( -0.005002170337468016433, -0.7660444431189770143, 0.6427681459581293666 ) ) ;
#50353=LINE ( 'NONE', #49798, #10686 ) ;
#50354=VECTOR ( 'NONE', #42489, 999.9999999999998863 ) ;
#50355=EDGE_CURVE ( 'NONE', #44511, #39352, #29438, .T. ) ;
#50356=DIRECTION ( 'NONE',  ( 0.6427681459581294776, -0.7660444431189769032, 0.005002170337467562802 ) ) ;
#50357=ORIENTED_EDGE ( 'NONE', *, *, #30669, .F. ) ;
#50358=AXIS2_PLACEMENT_3D ( 'NONE', #29273, #51135, #38357 ) ;
#50359=DIRECTION ( 'NONE',  ( 0.000000000000000000, -0.000000000000000000, -1.000000000000000000 ) ) ;
#50360=CARTESIAN_POINT ( 'NONE',  ( -15.13495153988577968, 0.000000000000000000, 12.76973526769478084 ) ) ;
#50361=ORIENTED_EDGE ( 'NONE', *, *, #46294, .F. ) ;
#50362=DIRECTION ( 'NONE',  ( -0.5364919789714478471, 0.6444004775717705469, -0.5449076811759709926 ) ) ;
#50363=DIRECTION ( 'NONE',  ( 0.007781995580012662783, 0.000000000000000000, -0.9999697198139514409 ) ) ;
#50364=VECTOR ( 'NONE', #41064, 1000.000000000000227 ) ;
#50365=EDGE_LOOP ( 'NONE', ( #23919, #33106, #52434, #15810 ) ) ;
#50366=CARTESIAN_POINT ( 'NONE',  ( -25.20278734466900517, 0.000000000000000000, 6.670939612111840944 ) ) ;
#50368=VECTOR ( 'NONE', #21530, 999.9999999999998863 ) ;
#50369=FACE_OUTER_BOUND ( 'NONE', #23421, .T. ) ;
#50370=CARTESIAN_POINT ( 'NONE',  ( -13.50659957395150812, -1.165603555308157846, 2.090554221737622953 ) ) ;
#50371=LINE ( 'NONE', #23430, #51900 ) ;
#50373=ORIENTED_EDGE ( 'NONE', *, *, #3144, .T. ) ;
#50374=VECTOR ( 'NONE', #35000, 999.9999999999998863 ) ;
#50375=VECTOR ( 'NONE', #48944, 1000.000000000000227 ) ;
#50376=ORIENTED_EDGE ( 'NONE', *, *, #25043, .F. ) ;
#50377=DIRECTION ( 'NONE',  ( -0.5449076811759708816, 0.6444004775717707689, 0.5364919789714475140 ) ) ;
#50378=DIRECTION ( 'NONE',  ( -0.005002170337468016433, -0.7660444431189770143, 0.6427681459581293666 ) ) ;
#50379=CARTESIAN_POINT ( 'NONE',  ( -14.40622671698839774, 0.000000000000000000, 4.538968524537128069 ) ) ;
#50380=VECTOR ( 'NONE', #55592, 1000.000000000000227 ) ;
#50381=CARTESIAN_POINT ( 'NONE',  ( -27.06630483948590893, -0.1191753592594197858, 7.295098399573937797 ) ) ;
#50382=VECTOR ( 'NONE', #53738, 1000.000000000000227 ) ;
#50383=DIRECTION ( 'NONE',  ( 0.9999697198139515519, 0.000000000000000000, 0.007781995580013368816 ) ) ;
#50384=DIRECTION ( 'NONE',  ( 0.5364919789714477361, 0.6444004775717706579, 0.5449076811759711036 ) ) ;
#50385=EDGE_CURVE ( 'NONE', #31029, #47959, #38222, .T. ) ;
#50386=VERTEX_POINT ( 'NONE', #55843 ) ;
#50387=CARTESIAN_POINT ( 'NONE',  ( -27.06630483948590893, -0.1191753592594197858, 7.295098399573937797 ) ) ;
#50388=VECTOR ( 'NONE', #41023, 999.9999999999998863 ) ;
#50389=LINE ( 'NONE', #27590, #36005 ) ;
#50390=VECTOR ( 'NONE', #52590, 999.9999999999998863 ) ;
#50391=CARTESIAN_POINT ( 'NONE',  ( -13.07066190154808361, 0.000000000000000000, 12.04713590736729678 ) ) ;
#50392=ORIENTED_EDGE ( 'NONE', *, *, #45431, .T. ) ;
#50395=LINE ( 'NONE', #10928, #41129 ) ;
#50396=ORIENTED_EDGE ( 'NONE', *, *, #13920, .F. ) ;
#50397=DIRECTION ( 'NONE',  ( -0.005961354470445682716, -0.6427876096865404731, 0.7660212471507180654 ) ) ;
#50398=ORIENTED_EDGE ( 'NONE', *, *, #27490, .F. ) ;
#50399=ADVANCED_FACE ( 'NONE', ( #42499 ), #29993, .F. ) ;
#50400=VECTOR ( 'NONE', #21028, 1000.000000000000227 ) ;
#50401=ORIENTED_EDGE ( 'NONE', *, *, #50277, .T. ) ;
#50402=ORIENTED_EDGE ( 'NONE', *, *, #51759, .T. ) ;
#50403=ORIENTED_EDGE ( 'NONE', *, *, #26730, .T. ) ;
#50404=AXIS2_PLACEMENT_3D ( 'NONE', #45688, #41160, #2254 ) ;
#50405=ORIENTED_EDGE ( 'NONE', *, *, #17536, .F. ) ;
#50406=DIRECTION ( 'NONE',  ( 0.6427681459581294776, -0.7660444431189769032, 0.005002170337467562802 ) ) ;
#50407=AXIS2_PLACEMENT_3D ( 'NONE', #12653, #30254, #3294 ) ;
#50408=EDGE_LOOP ( 'NONE', ( #1756, #21744, #28282, #5469 ) ) ;
#50409=VERTEX_POINT ( 'NONE', #56126 ) ;
#50410=ADVANCED_FACE ( 'NONE', ( #16952 ), #34277, .F. ) ;
#50411=EDGE_LOOP ( 'NONE', ( #12824, #43569, #56128, #8161 ) ) ;
#50412=AXIS2_PLACEMENT_3D ( 'NONE', #30993, #52856, #23346 ) ;
#50413=ORIENTED_EDGE ( 'NONE', *, *, #47261, .F. ) ;
#50414=EDGE_CURVE ( 'NONE', #13801, #17105, #9835, .T. ) ;
#50415=AXIS2_PLACEMENT_3D ( 'NONE', #40303, #27826, #40856 ) ;
#50416=VECTOR ( 'NONE', #27659, 999.9999999999998863 ) ;
#50417=DIRECTION ( 'NONE',  ( 0.7660212471507180654, -0.6427876096865404731, 0.005961354470445141482 ) ) ;
#50418=CARTESIAN_POINT ( 'NONE',  ( -8.653915872335209869, -10.43490457594507781, 6.579848388698870565 ) ) ;
#50419=CARTESIAN_POINT ( 'NONE',  ( -25.20278734466900517, 0.000000000000000000, 6.670939612111840944 ) ) ;
#50420=DIRECTION ( 'NONE',  ( -0.5449076811759708816, 0.6444004775717707689, 0.5364919789714475140 ) ) ;
#50421=ORIENTED_EDGE ( 'NONE', *, *, #20271, .F. ) ;
#50422=DIRECTION ( 'NONE',  ( 0.5449076811759707706, 0.6444004775717708799, -0.5364919789714476250 ) ) ;
#50423=ORIENTED_EDGE ( 'NONE', *, *, #44605, .T. ) ;
#50424=VECTOR ( 'NONE', #24874, 999.9999999999998863 ) ;
#50427=VECTOR ( 'NONE', #1020, 1000.000000000000114 ) ;
#50428=CARTESIAN_POINT ( 'NONE',  ( -10.94028622754223967, 0.000000000000000000, 11.14038480894692995 ) ) ;
#50429=FACE_OUTER_BOUND ( 'NONE', #45107, .T. ) ;
#50430=AXIS2_PLACEMENT_3D ( 'NONE', #19926, #40418, #19088 ) ;
#50431=CARTESIAN_POINT ( 'NONE',  ( -19.63691669459172928, -5.051250379848162275, 12.59953947454578760 ) ) ;
#50432=EDGE_CURVE ( 'NONE', #16632, #46605, #14091, .T. ) ;
#50433=VECTOR ( 'NONE', #54404, 999.9999999999998863 ) ;
#50434=FACE_OUTER_BOUND ( 'NONE', #2675, .T. ) ;
#50435=LINE ( 'NONE', #28567, #32196 ) ;
#50436=DIRECTION ( 'NONE',  ( -0.6427681459581293666, -0.7660444431189770143, -0.005002170337467561935 ) ) ;
#50437=EDGE_LOOP ( 'NONE', ( #4695, #33929, #30706, #21597 ) ) ;
#50438=FACE_OUTER_BOUND ( 'NONE', #45856, .T. ) ;
#50439=ORIENTED_EDGE ( 'NONE', *, *, #27529, .F. ) ;
#50440=CARTESIAN_POINT ( 'NONE',  ( -13.53673582514181106, 0.000000000000000000, 12.22817484722816772 ) ) ;
#50441=DIRECTION ( 'NONE',  ( -0.005002170337468016433, -0.7660444431189770143, 0.6427681459581293666 ) ) ;
#50442=LINE ( 'NONE', #11802, #34470 ) ;
#50443=LINE ( 'NONE', #15784, #44015 ) ;
#50444=DIRECTION ( 'NONE',  ( -0.9999697198139514409, -0.000000000000000000, -0.007781995580013368816 ) ) ;
#50445=VECTOR ( 'NONE', #13518, 1000.000000000000000 ) ;
#50446=ORIENTED_EDGE ( 'NONE', *, *, #31707, .F. ) ;
#50447=ORIENTED_EDGE ( 'NONE', *, *, #9836, .F. ) ;
#50448=DIRECTION ( 'NONE',  ( 0.007781995580012663651, -3.146120232559066537E-19, -0.9999697198139514409 ) ) ;
#50449=CARTESIAN_POINT ( 'NONE',  ( -28.92982233430281980, 0.000000000000000000, 7.919257187036034651 ) ) ;
#50450=CARTESIAN_POINT ( 'NONE',  ( -18.33193799619571962, 0.000000000000000000, 5.616413941050340419 ) ) ;
#50451=VECTOR ( 'NONE', #30755, 1000.000000000000000 ) ;
#50452=ADVANCED_FACE ( 'NONE', ( #26292 ), #5005, .F. ) ;
#50453=PLANE ( 'NONE',  #8301 ) ;
#50454=VECTOR ( 'NONE', #29511, 999.9999999999998863 ) ;
#50455=FACE_OUTER_BOUND ( 'NONE', #34150, .T. ) ;
#50456=ADVANCED_FACE ( 'NONE', ( #5846 ), #22870, .F. ) ;
#50457=CARTESIAN_POINT ( 'NONE',  ( -8.409922665610809034, 0.000000000000000000, 10.23674650875856962 ) ) ;
#50458=CARTESIAN_POINT ( 'NONE',  ( 2.072287782118878319, 0.000000000000000000, -2.950529333540147015 ) ) ;
#50459=AXIS2_PLACEMENT_3D ( 'NONE', #20322, #33404, #3300 ) ;
#50460=CARTESIAN_POINT ( 'NONE',  ( -14.66887761629205222, 0.000000000000000000, 12.58869632783390990 ) ) ;
#50461=EDGE_CURVE ( 'NONE', #43270, #30420, #52680, .T. ) ;
#50462=LINE ( 'NONE', #52678, #20163 ) ;
#50463=ADVANCED_FACE ( 'NONE', ( #22606 ), #17793, .F. ) ;
#50464=VECTOR ( 'NONE', #5874, 1000.000000000000227 ) ;
#50465=EDGE_CURVE ( 'NONE', #43561, #12378, #53285, .T. ) ;
#50466=ADVANCED_FACE ( 'NONE', ( #52428 ), #14376, .F. ) ;
#50467=ORIENTED_EDGE ( 'NONE', *, *, #27030, .T. ) ;
#50468=AXIS2_PLACEMENT_3D ( 'NONE', #50951, #29395, #7835 ) ;
#50469=VECTOR ( 'NONE', #13267, 1000.000000000000227 ) ;
#50470=ORIENTED_EDGE ( 'NONE', *, *, #40726, .T. ) ;
#50471=VECTOR ( 'NONE', #34446, 999.9999999999998863 ) ;
#50472=VERTEX_POINT ( 'NONE', #40498 ) ;
#50473=EDGE_LOOP ( 'NONE', ( #43250, #19045, #624, #31821 ) ) ;
#50474=ORIENTED_EDGE ( 'NONE', *, *, #34325, .F. ) ;
#50475=CARTESIAN_POINT ( 'NONE',  ( -17.70023939833923521, 0.000000000000000000, 9.853308747064737361 ) ) ;
#50476=CARTESIAN_POINT ( 'NONE',  ( -12.65839411606857823, -0.1191753592594179401, 5.929895813100822366 ) ) ;
#50477=LINE ( 'NONE', #30599, #37608 ) ;
#50478=VERTEX_POINT ( 'NONE', #35659 ) ;
#50479=LINE ( 'NONE', #33437, #9559 ) ;
#50480=EDGE_CURVE ( 'NONE', #9219, #40728, #22033, .T. ) ;
#50481=ORIENTED_EDGE ( 'NONE', *, *, #21447, .T. ) ;
#50482=CARTESIAN_POINT ( 'NONE',  ( -19.86442598447069585, 1.771796430571655145, 6.503047446853179814 ) ) ;
#50483=EDGE_LOOP ( 'NONE', ( #52819, #6801, #52820, #26412 ) ) ;
#50484=VECTOR ( 'NONE', #18435, 1000.000000000000000 ) ;
#50485=EDGE_CURVE ( 'NONE', #12432, #43913, #1586, .T. ) ;
#50487=EDGE_CURVE ( 'NONE', #36594, #22669, #48994, .T. ) ;
#50488=LINE ( 'NONE', #20071, #8280 ) ;
#50489=LINE ( 'NONE', #28903, #42280 ) ;
#50490=ORIENTED_EDGE ( 'NONE', *, *, #42608, .T. ) ;
#50491=DIRECTION ( 'NONE',  ( -0.7660212471507179544, -0.6427876096865405842, -0.005961354470445141482 ) ) ;
#50492=ORIENTED_EDGE ( 'NONE', *, *, #46179, .T. ) ;
#50493=EDGE_CURVE ( 'NONE', #45245, #46200, #9248, .T. ) ;
#50494=FACE_OUTER_BOUND ( 'NONE', #36650, .T. ) ;
#50495=VECTOR ( 'NONE', #54357, 999.9999999999998863 ) ;
#50496=CARTESIAN_POINT ( 'NONE',  ( -18.67775241435682432, 0.000000000000000000, 4.136394454059623804 ) ) ;
#50497=EDGE_CURVE ( 'NONE', #27027, #8286, #52136, .T. ) ;
#50498=CARTESIAN_POINT ( 'NONE',  ( -27.99845268667336384, -0.1191753592594197858, 7.657176279295684118 ) ) ;
#50499=VECTOR ( 'NONE', #12007, 999.9999999999998863 ) ;
#50500=LINE ( 'NONE', #55295, #6841 ) ;
#50501=PLANE ( 'NONE',  #29266 ) ;
#50502=CARTESIAN_POINT ( 'NONE',  ( -14.97381569168726756, 0.4483081953215047322, 3.433409769016318780 ) ) ;
#50503=LINE ( 'NONE', #37724, #26652 ) ;
#50504=PLANE ( 'NONE',  #41970 ) ;
#50505=ORIENTED_EDGE ( 'NONE', *, *, #26454, .F. ) ;
#50506=DIRECTION ( 'NONE',  ( 0.7660212471507180654, -0.6427876096865404731, 0.005961354470445141482 ) ) ;
#50507=ORIENTED_EDGE ( 'NONE', *, *, #30371, .T. ) ;
#50508=VECTOR ( 'NONE', #15294, 1000.000000000000000 ) ;
#50509=LINE ( 'NONE', #1933, #4784 ) ;
#50510=CARTESIAN_POINT ( 'NONE',  ( -13.53673582514181106, 0.000000000000000000, 12.22817484722816772 ) ) ;
#50511=CARTESIAN_POINT ( 'NONE',  ( -14.64608374724779161, 0.6102101463440037232, 3.571816235922804950 ) ) ;
#50512=LINE ( 'NONE', #10504, #15075 ) ;
#50513=LINE ( 'NONE', #24642, #37657 ) ;
#50514=VECTOR ( 'NONE', #39832, 1000.000000000000114 ) ;
#50515=CARTESIAN_POINT ( 'NONE',  ( -24.27063949748155380, 0.000000000000000000, 6.308861732390097288 ) ) ;
#50517=VERTEX_POINT ( 'NONE', #13253 ) ;
#50518=DIRECTION ( 'NONE',  ( 0.007781995580012663651, -3.146120232559066537E-19, -0.9999697198139514409 ) ) ;
#50519=PLANE ( 'NONE',  #42924 ) ;
#50520=DIRECTION ( 'NONE',  ( 0.007781995580012663651, -3.146120232559066537E-19, -0.9999697198139514409 ) ) ;
#50521=DIRECTION ( 'NONE',  ( -0.005961354470445682716, -0.6427876096865404731, 0.7660212471507180654 ) ) ;
#50524=PLANE ( 'NONE',  #33894 ) ;
#50525=PLANE ( 'NONE',  #47681 ) ;
#50526=CARTESIAN_POINT ( 'NONE',  ( -12.60458797795435615, 0.000000000000000000, 11.86609696750642229 ) ) ;
#50527=ORIENTED_EDGE ( 'NONE', *, *, #7570, .F. ) ;
#50528=LINE ( 'NONE', #41156, #6774 ) ;
#50529=PLANE ( 'NONE',  #45040 ) ;
#50530=ORIENTED_EDGE ( 'NONE', *, *, #5579, .F. ) ;
#50531=DIRECTION ( 'NONE',  ( 0.007781995580012663651, -3.146120232559066537E-19, -0.9999697198139514409 ) ) ;
#50532=PLANE ( 'NONE',  #5623 ) ;
#50533=ADVANCED_FACE ( 'NONE', ( #47889 ), #43891, .F. ) ;
#50534=EDGE_CURVE ( 'NONE', #25308, #41647, #740, .T. ) ;
#50535=ORIENTED_EDGE ( 'NONE', *, *, #27181, .F. ) ;
#50536=VERTEX_POINT ( 'NONE', #31109 ) ;
#50537=DIRECTION ( 'NONE',  ( 0.007781995580012662783, 0.000000000000000000, -0.9999697198139514409 ) ) ;
#50538=ADVANCED_FACE ( 'NONE', ( #48433 ), #7230, .F. ) ;
#50539=VECTOR ( 'NONE', #48721, 999.9999999999998863 ) ;
#50540=EDGE_LOOP ( 'NONE', ( #28644, #30002 ) ) ;
#50541=ORIENTED_EDGE ( 'NONE', *, *, #42354, .T. ) ;
#50542=ORIENTED_EDGE ( 'NONE', *, *, #15678, .F. ) ;
#50543=FACE_OUTER_BOUND ( 'NONE', #31065, .T. ) ;
#50545=DIRECTION ( 'NONE',  ( 0.7660212471507180654, -0.6427876096865404731, 0.005961354470445141482 ) ) ;
#50546=VECTOR ( 'NONE', #55237, 999.9999999999998863 ) ;
#50547=EDGE_LOOP ( 'NONE', ( #28045, #27836, #9498, #48432 ) ) ;
#50548=EDGE_LOOP ( 'NONE', ( #52305, #34830, #18104, #23781 ) ) ;
#50549=ADVANCED_FACE ( 'NONE', ( #6399 ), #11200, .F. ) ;
#50550=DIRECTION ( 'NONE',  ( 0.005961354470445682716, -0.6427876096865404731, -0.7660212471507180654 ) ) ;
#50551=DIRECTION ( 'NONE',  ( 0.9999697198139515519, 0.000000000000000000, 0.007781995580013368816 ) ) ;
#50552=VERTEX_POINT ( 'NONE', #24280 ) ;
#50553=CARTESIAN_POINT ( 'NONE',  ( -10.66170866159616715, 0.000000000000000000, 1.044114545398534766 ) ) ;
#50554=VERTEX_POINT ( 'NONE', #23698 ) ;
#50555=DIRECTION ( 'NONE',  ( 0.000000000000000000, -1.000000000000000000, 0.000000000000000000 ) ) ;
#50556=CARTESIAN_POINT ( 'NONE',  ( -10.43730245779182475, 0.000000000000000000, 6.216509903659242831 ) ) ;
#50557=ORIENTED_EDGE ( 'NONE', *, *, #21277, .F. ) ;
#50558=ADVANCED_FACE ( 'NONE', ( #33072 ), #54102, .F. ) ;
#50559=LINE ( 'NONE', #7123, #14114 ) ;
#50560=ADVANCED_FACE ( 'NONE', ( #10927 ), #1831, .F. ) ;
#50561=LINE ( 'NONE', #28127, #29104 ) ;
#50562=ORIENTED_EDGE ( 'NONE', *, *, #24261, .F. ) ;
#50564=LINE ( 'NONE', #6290, #16764 ) ;
#50565=LINE ( 'NONE', #2826, #46595 ) ;
#50566=DIRECTION ( 'NONE',  ( -0.005961354470445682716, -0.6427876096865404731, 0.7660212471507180654 ) ) ;
#50567=ADVANCED_FACE ( 'NONE', ( #45297 ), #37313, .F. ) ;
#50568=ORIENTED_EDGE ( 'NONE', *, *, #52466, .F. ) ;
#50569=FACE_OUTER_BOUND ( 'NONE', #1620, .T. ) ;
#50570=FACE_OUTER_BOUND ( 'NONE', #23174, .T. ) ;
#50571=EDGE_CURVE ( 'NONE', #18631, #37343, #11504, .T. ) ;
#50572=DIRECTION ( 'NONE',  ( 0.9999697198139515519, 0.000000000000000000, 0.007781995580013368816 ) ) ;
#50573=DIRECTION ( 'NONE',  ( -0.7660212471507179544, -0.6427876096865405842, -0.005961354470445141482 ) ) ;
#50574=LINE ( 'NONE', #37496, #8644 ) ;
#50575=CARTESIAN_POINT ( 'NONE',  ( -12.18800911221693006, -0.1191753592594174960, 5.194892318353301341 ) ) ;
#50577=DIRECTION ( 'NONE',  ( -0.005961354470445682716, -0.6427876096865404731, 0.7660212471507180654 ) ) ;
#50578=ORIENTED_EDGE ( 'NONE', *, *, #2007, .F. ) ;
#50579=CARTESIAN_POINT ( 'NONE',  ( -19.84110863911566014, -3.108426967578157729, 9.490350352780952292 ) ) ;
#50580=CARTESIAN_POINT ( 'NONE',  ( -14.44988390315699434, 4.819660872929013351, 2.140984944058630823 ) ) ;
#50581=CARTESIAN_POINT ( 'NONE',  ( -15.40103151951671734, 0.000000000000000000, 12.95233060667165681 ) ) ;
#50582=ORIENTED_EDGE ( 'NONE', *, *, #9910, .F. ) ;
#50583=CARTESIAN_POINT ( 'NONE',  ( -11.15508609349007507, 0.000000000000000000, 4.733595666208168851 ) ) ;
#50585=AXIS2_PLACEMENT_3D ( 'NONE', #34708, #31296, #53171 ) ;
#50586=LINE ( 'NONE', #34386, #4094 ) ;
#50587=DIRECTION ( 'NONE',  ( -0.005002170337468016433, -0.7660444431189770143, 0.6427681459581293666 ) ) ;
#50588=CARTESIAN_POINT ( 'NONE',  ( -18.63389729487044377, -0.006848592768176286170, 9.670969966159701059 ) ) ;
#50589=ORIENTED_EDGE ( 'NONE', *, *, #35668, .T. ) ;
#50590=ORIENTED_EDGE ( 'NONE', *, *, #24813, .F. ) ;
#50591=DIRECTION ( 'NONE',  ( 0.000000000000000000, -1.000000000000000000, 0.000000000000000000 ) ) ;
#50592=DIRECTION ( 'NONE',  ( 0.000000000000000000, -1.000000000000000000, 0.000000000000000000 ) ) ;
#50593=ADVANCED_FACE ( 'NONE', ( #49271 ), #45553, .F. ) ;
#50594=ORIENTED_EDGE ( 'NONE', *, *, #39394, .F. ) ;
#50595=CARTESIAN_POINT ( 'NONE',  ( 2.072287782118878319, 0.000000000000000000, -2.950529333540147015 ) ) ;
#50596=VERTEX_POINT ( 'NONE', #28825 ) ;
#50597=LINE ( 'NONE', #29010, #28391 ) ;
#50598=EDGE_CURVE ( 'NONE', #8140, #38515, #14919, .T. ) ;
#50599=EDGE_CURVE ( 'NONE', #25448, #54376, #18913, .T. ) ;
#50600=ORIENTED_EDGE ( 'NONE', *, *, #9337, .T. ) ;
#50601=ORIENTED_EDGE ( 'NONE', *, *, #4263, .F. ) ;
#50602=EDGE_LOOP ( 'NONE', ( #49720, #43823, #31328, #53884 ) ) ;
#50603=DIRECTION ( 'NONE',  ( 0.9321478471874540261, 0.000000000000000000, -0.3620778797217457101 ) ) ;
#50604=CARTESIAN_POINT ( 'NONE',  ( -12.54767912962405774, 0.000000000000000000, 4.553432171609165913 ) ) ;
#50605=DIRECTION ( 'NONE',  ( -0.005961354470445682716, -0.6427876096865404731, 0.7660212471507180654 ) ) ;
#50606=VERTEX_POINT ( 'NONE', #15456 ) ;
#50608=ORIENTED_EDGE ( 'NONE', *, *, #10807, .F. ) ;
#50609=ADVANCED_FACE ( 'NONE', ( #32525 ), #6973, .T. ) ;
#50610=ORIENTED_EDGE ( 'NONE', *, *, #32424, .F. ) ;
#50611=ORIENTED_EDGE ( 'NONE', *, *, #50933, .F. ) ;
#50612=PLANE ( 'NONE',  #23203 ) ;
#50613=DIRECTION ( 'NONE',  ( -0.6427681459581293666, -0.7660444431189770143, -0.005002170337467561935 ) ) ;
#50614=ORIENTED_EDGE ( 'NONE', *, *, #36355, .T. ) ;
#50615=CARTESIAN_POINT ( 'NONE',  ( 2.072287782118878319, -1.000000000000000000, -2.950529333540147015 ) ) ;
#50616=VERTEX_POINT ( 'NONE', #32778 ) ;
#50617=CARTESIAN_POINT ( 'NONE',  ( -15.80013740751165230, 0.000000000000000000, 4.528120789233099686 ) ) ;
#50618=LINE ( 'NONE', #37851, #40415 ) ;
#50619=VECTOR ( 'NONE', #56222, 999.9999999999998863 ) ;
#50620=VERTEX_POINT ( 'NONE', #36227 ) ;
#50621=CARTESIAN_POINT ( 'NONE',  ( -27.99767448711536133, 0.000000000000000000, 7.557179307314289218 ) ) ;
#50622=ORIENTED_EDGE ( 'NONE', *, *, #23882, .F. ) ;
#50623=ADVANCED_FACE ( 'NONE', ( #27711 ), #10682, .F. ) ;
#50624=LINE ( 'NONE', #28473, #24643 ) ;
#50625=DIRECTION ( 'NONE',  ( 0.007781995580012663651, -3.146120232559066537E-19, -0.9999697198139514409 ) ) ;
#50626=ADVANCED_FACE ( 'NONE', ( #6145 ), #14632, .F. ) ;
#50627=CARTESIAN_POINT ( 'NONE',  ( -14.94760462649100496, 0.000000000000000000, 2.488088991209854051 ) ) ;
#50628=LINE ( 'NONE', #45505, #3015 ) ;
#50629=LINE ( 'NONE', #46937, #38682 ) ;
#50631=ORIENTED_EDGE ( 'NONE', *, *, #23618, .F. ) ;
#50632=ORIENTED_EDGE ( 'NONE', *, *, #29748, .F. ) ;
#50634=EDGE_CURVE ( 'NONE', #21969, #25655, #40765, .T. ) ;
#50636=CARTESIAN_POINT ( 'NONE',  ( -9.808144436391993182, 0.000000000000000000, 10.77986332834118777 ) ) ;
#50637=DIRECTION ( 'NONE',  ( 0.007781995580012662783, 0.000000000000000000, -0.9999697198139514409 ) ) ;
#50638=DIRECTION ( 'NONE',  ( 0.5364919789714477361, 0.6444004775717706579, 0.5449076811759711036 ) ) ;
#50639=CARTESIAN_POINT ( 'NONE',  ( -19.94320461137762024, -2.137015261443157232, 7.935755791898535527 ) ) ;
#50640=EDGE_LOOP ( 'NONE', ( #25316, #11989, #41406, #4521 ) ) ;
#50641=CARTESIAN_POINT ( 'NONE',  ( -15.79283290138508455, 0.000000000000000000, 3.589507438754780289 ) ) ;
#50642=CARTESIAN_POINT ( 'NONE',  ( -14.66887761629205222, 0.000000000000000000, 12.58869632783390990 ) ) ;
#50643=VERTEX_POINT ( 'NONE', #3793 ) ;
#50644=CARTESIAN_POINT ( 'NONE',  ( -17.46532115785441519, 0.000000000000000000, 13.67492996699914265 ) ) ;
#50645=LINE ( 'NONE', #49805, #2323 ) ;
#50646=ORIENTED_EDGE ( 'NONE', *, *, #16421, .T. ) ;
#50647=EDGE_CURVE ( 'NONE', #28808, #12905, #25664, .T. ) ;
#50648=DIRECTION ( 'NONE',  ( -0.005961354470445682716, -0.6427876096865404731, 0.7660212471507180654 ) ) ;
#50649=DIRECTION ( 'NONE',  ( -0.6427681459581293666, -0.7660444431189770143, -0.005002170337467561935 ) ) ;
#50651=EDGE_CURVE ( 'NONE', #53756, #33683, #8341, .T. ) ;
#50652=CARTESIAN_POINT ( 'NONE',  ( -18.67775241435682432, 0.000000000000000000, 4.136394454059623804 ) ) ;
#50653=DIRECTION ( 'NONE',  ( 0.9999697198139515519, 0.000000000000000000, 0.007781995580013368816 ) ) ;
#50654=ORIENTED_EDGE ( 'NONE', *, *, #13361, .F. ) ;
#50655=ORIENTED_EDGE ( 'NONE', *, *, #18760, .F. ) ;
#50656=DIRECTION ( 'NONE',  ( -0.7660212471507179544, -0.6427876096865405842, -0.005961354470445141482 ) ) ;
#50657=CARTESIAN_POINT ( 'NONE',  ( -14.66887761629205222, 0.000000000000000000, 12.58869632783390990 ) ) ;
#50659=EDGE_CURVE ( 'NONE', #48678, #47622, #25973, .T. ) ;
#50660=FACE_OUTER_BOUND ( 'NONE', #53472, .T. ) ;
#50661=VECTOR ( 'NONE', #45203, 1000.000000000000114 ) ;
#50662=DIRECTION ( 'NONE',  ( -0.005002170337468016433, -0.7660444431189770143, 0.6427681459581293666 ) ) ;
#50663=EDGE_CURVE ( 'NONE', #14307, #29351, #3252, .T. ) ;
#50664=CARTESIAN_POINT ( 'NONE',  ( -17.19404809803491574, 0.000000000000000000, 4.517273053929070414 ) ) ;
#50665=VERTEX_POINT ( 'NONE', #16884 ) ;
#50666=CARTESIAN_POINT ( 'NONE',  ( -20.89679648621866193, -4.889348428825661230, 12.82321088736104642 ) ) ;
#50667=EDGE_CURVE ( 'NONE', #14388, #31826, #38749, .T. ) ;
#50668=CARTESIAN_POINT ( 'NONE',  ( -8.910664554068135956, -10.68360705318012194, 6.679578295905873375 ) ) ;
#50669=PLANE ( 'NONE',  #22420 ) ;
#50670=ORIENTED_EDGE ( 'NONE', *, *, #36917, .T. ) ;
#50671=CARTESIAN_POINT ( 'NONE',  ( -27.06552663992790997, 0.000000000000000000, 7.195101427592543786 ) ) ;
#50672=DIRECTION ( 'NONE',  ( 0.6427681459581294776, -0.7660444431189769032, 0.005002170337467562802 ) ) ;
#50673=DIRECTION ( 'NONE',  ( 0.9321478471874540261, 0.000000000000000000, -0.3620778797217457101 ) ) ;
#50675=ORIENTED_EDGE ( 'NONE', *, *, #30073, .T. ) ;
#50676=ADVANCED_FACE ( 'NONE', ( #37900 ), #29368, .F. ) ;
#50677=DIRECTION ( 'NONE',  ( 0.005961354470445682716, -0.6427876096865404731, -0.7660212471507180654 ) ) ;
#50678=ORIENTED_EDGE ( 'NONE', *, *, #51305, .T. ) ;
#50680=ORIENTED_EDGE ( 'NONE', *, *, #24056, .T. ) ;
#50681=VERTEX_POINT ( 'NONE', #47233 ) ;
#50682=ORIENTED_EDGE ( 'NONE', *, *, #12182, .T. ) ;
#50683=DIRECTION ( 'NONE',  ( -0.9999697198139514409, -0.000000000000000000, -0.007781995580013368816 ) ) ;
#50684=ORIENTED_EDGE ( 'NONE', *, *, #13298, .T. ) ;
#50685=EDGE_LOOP ( 'NONE', ( #18838, #55784, #45942, #33998 ) ) ;
#50686=DIRECTION ( 'NONE',  ( 0.9999697198139515519, 0.000000000000000000, 0.007781995580013368816 ) ) ;
#50687=VERTEX_POINT ( 'NONE', #4097 ) ;
#50688=EDGE_LOOP ( 'NONE', ( #48136, #50009, #22693, #13528 ) ) ;
#50689=DIRECTION ( 'NONE',  ( 0.007781995580012663651, -3.146120232559066537E-19, -0.9999697198139514409 ) ) ;
#50690=DIRECTION ( 'NONE',  ( 0.6427681459581294776, -0.7660444431189769032, 0.005002170337467562802 ) ) ;
#50691=DIRECTION ( 'NONE',  ( -0.7660212471507179544, -0.6427876096865405842, -0.005961354470445141482 ) ) ;
#50692=DIRECTION ( 'NONE',  ( 0.000000000000000000, -0.000000000000000000, -1.000000000000000000 ) ) ;
#50693=FACE_OUTER_BOUND ( 'NONE', #47707, .T. ) ;
#50694=ORIENTED_EDGE ( 'NONE', *, *, #24580, .F. ) ;
#50695=ORIENTED_EDGE ( 'NONE', *, *, #37962, .F. ) ;
#50696=LINE ( 'NONE', #37344, #52088 ) ;
#50697=EDGE_CURVE ( 'NONE', #19093, #27972, #21426, .T. ) ;
#50698=DIRECTION ( 'NONE',  ( -0.6246952433987894571, 0.7422098413412802076, 0.2426528472758539834 ) ) ;
#50699=PRODUCT_DEFINITION_CONTEXT ( 'detailed design', #46339, 'design' ) ;
#50700=CARTESIAN_POINT ( 'NONE',  ( -28.92982233430281980, 0.000000000000000000, 7.919257187036034651 ) ) ;
#50701=LINE ( 'NONE', #11791, #38629 ) ;
#50702=DIRECTION ( 'NONE',  ( 0.9321478471874540261, 0.000000000000000000, -0.3620778797217456546 ) ) ;
#50703=CARTESIAN_POINT ( 'NONE',  ( -10.23730851382903495, 0.000000000000000000, 6.218066302775246079 ) ) ;
#50704=ORIENTED_EDGE ( 'NONE', *, *, #25179, .F. ) ;
#50705=DIRECTION ( 'NONE',  ( 0.6427681459581294776, -0.7660444431189769032, 0.005002170337467562802 ) ) ;
#50706=VERTEX_POINT ( 'NONE', #12033 ) ;
#50707=ADVANCED_FACE ( 'NONE', ( #34465 ), #2945, .F. ) ;
#50708=DIRECTION ( 'NONE',  ( 0.5364919789714477361, 0.6444004775717706579, 0.5449076811759711036 ) ) ;
#50709=CARTESIAN_POINT ( 'NONE',  ( -18.39746900504187010, 0.000000000000000000, 14.03700784672088808 ) ) ;
#50710=CARTESIAN_POINT ( 'NONE',  ( -21.47419595591918906, 0.000000000000000000, 5.222628093224860102 ) ) ;
#50711=DIRECTION ( 'NONE',  ( 0.000000000000000000, -0.000000000000000000, -1.000000000000000000 ) ) ;
#50712=CARTESIAN_POINT ( 'NONE',  ( -23.33849165029409889, 0.000000000000000000, 5.946783852668351855 ) ) ;
#50713=EDGE_CURVE ( 'NONE', #50620, #6417, #20840, .T. ) ;
#50714=ADVANCED_FACE ( 'NONE', ( #34215 ), #16042, .F. ) ;
#50715=CARTESIAN_POINT ( 'NONE',  ( -10.94028622754223967, 0.000000000000000000, 11.14038480894692995 ) ) ;
#50716=ORIENTED_EDGE ( 'NONE', *, *, #13468, .F. ) ;
#50718=CARTESIAN_POINT ( 'NONE',  ( -15.83306965045904668, 0.000000000000000000, 8.759843284363483917 ) ) ;
#50719=DIRECTION ( 'NONE',  ( -0.6427681459581293666, -0.7660444431189770143, -0.005002170337467561935 ) ) ;
#50720=CARTESIAN_POINT ( 'NONE',  ( -13.49264084522192064, 0.000000000000000000, 6.562064623656943319 ) ) ;
#50721=CARTESIAN_POINT ( 'NONE',  ( -21.47263955680318404, 0.000000000000000000, 5.022634149262071190 ) ) ;
#50722=EDGE_CURVE ( 'NONE', #51840, #14307, #11763, .T. ) ;
#50723=PLANE ( 'NONE',  #25790 ) ;
#50725=CARTESIAN_POINT ( 'NONE',  ( -12.07243185130034213, -2.784623065533160524, 1.481819574845134602 ) ) ;
#50726=EDGE_CURVE ( 'NONE', #33095, #23836, #55473, .T. ) ;
#50727=PLANE ( 'NONE',  #21484 ) ;
#50728=LINE ( 'NONE', #38220, #31949 ) ;
#50729=ORIENTED_EDGE ( 'NONE', *, *, #47749, .F. ) ;
#50730=ADVANCED_FACE ( 'NONE', ( #46686 ), #7811, .F. ) ;
#50731=VERTEX_POINT ( 'NONE', #12617 ) ;
#50732=EDGE_CURVE ( 'NONE', #36692, #37781, #676, .T. ) ;
#50733=ORIENTED_EDGE ( 'NONE', *, *, #14983, .T. ) ;
#50734=ORIENTED_EDGE ( 'NONE', *, *, #17133, .F. ) ;
#50735=ORIENTED_EDGE ( 'NONE', *, *, #18893, .F. ) ;
#50736=ORIENTED_EDGE ( 'NONE', *, *, #10796, .F. ) ;
#50737=DIRECTION ( 'NONE',  ( 0.5364919789714477361, 0.6444004775717706579, 0.5449076811759711036 ) ) ;
#50738=DIRECTION ( 'NONE',  ( 0.9999697198139515519, 0.000000000000000000, 0.007781995580013368816 ) ) ;
#50739=DIRECTION ( 'NONE',  ( -0.9999697198139514409, -0.000000000000000000, -0.007781995580013368816 ) ) ;
#50740=ORIENTED_EDGE ( 'NONE', *, *, #55448, .F. ) ;
#50741=CARTESIAN_POINT ( 'NONE',  ( -21.47263955680318404, 0.000000000000000000, 5.022634149262071190 ) ) ;
#50742=EDGE_LOOP ( 'NONE', ( #46299, #48809, #17140, #9932 ) ) ;
#50743=LINE ( 'NONE', #46779, #18649 ) ;
#50744=ORIENTED_EDGE ( 'NONE', *, *, #46527, .T. ) ;
#50746=DIRECTION ( 'NONE',  ( 0.9999697198139515519, 0.000000000000000000, 0.007781995580013368816 ) ) ;
#50747=LINE ( 'NONE', #33172, #37747 ) ;
#50748=ORIENTED_EDGE ( 'NONE', *, *, #52495, .F. ) ;
#50749=LINE ( 'NONE', #38244, #30129 ) ;
#50750=EDGE_LOOP ( 'NONE', ( #855, #29803, #21967, #15895 ) ) ;
#50751=CARTESIAN_POINT ( 'NONE',  ( -13.10951999731236128, 0.4483081953215036219, 2.709254009572826138 ) ) ;
#50752=ADVANCED_FACE ( 'NONE', ( #35889 ), #48356, .F. ) ;
#50753=DIRECTION ( 'NONE',  ( 0.007781995580012663651, -3.146120232559066537E-19, -0.9999697198139514409 ) ) ;
#50754=DIRECTION ( 'NONE',  ( -0.5364919789714478471, 0.6444004775717705469, -0.5449076811759709926 ) ) ;
#50755=EDGE_CURVE ( 'NONE', #55136, #4507, #52362, .T. ) ;
#50756=CARTESIAN_POINT ( 'NONE',  ( -27.99923088623136636, 0.000000000000000000, 7.757173251277078130 ) ) ;
#50757=DIRECTION ( 'NONE',  ( 0.9999697198139515519, 0.000000000000000000, 0.007781995580013368816 ) ) ;
#50758=LINE ( 'NONE', #12142, #40286 ) ;
#50759=EDGE_CURVE ( 'NONE', #49826, #22994, #4930, .T. ) ;
#50760=CARTESIAN_POINT ( 'NONE',  ( -16.42972749701432278, 4.333955019861509328, 10.37594377198947804 ) ) ;
#50761=CARTESIAN_POINT ( 'NONE',  ( -22.20772426397657995, -4.241740624735659715, 12.26958501973509463 ) ) ;
#50762=VERTEX_POINT ( 'NONE', #9767 ) ;
#50764=ORIENTED_EDGE ( 'NONE', *, *, #35250, .T. ) ;
#50765=ADVANCED_FACE ( 'NONE', ( #30780 ), #27075, .F. ) ;
#50766=EDGE_CURVE ( 'NONE', #13246, #43824, #5482, .T. ) ;
#50767=ADVANCED_FACE ( 'NONE', ( #39012 ), #43816, .F. ) ;
#50769=PLANE ( 'NONE',  #29644 ) ;
#50770=DIRECTION ( 'NONE',  ( 0.007781995580012663651, 0.000000000000000000, -0.9999697198139515519 ) ) ;
#50771=CARTESIAN_POINT ( 'NONE',  ( -14.76859376284157044, -1.003701604285655025, 2.585921142092966640 ) ) ;
#50772=PLANE ( 'NONE',  #13180 ) ;
#50773=FACE_OUTER_BOUND ( 'NONE', #29445, .T. ) ;
#50774=ORIENTED_EDGE ( 'NONE', *, *, #5607, .T. ) ;
#50775=CARTESIAN_POINT ( 'NONE',  ( -18.45768884757317352, -1.489407457353155717, 6.295896285107346557 ) ) ;
#50776=CARTESIAN_POINT ( 'NONE',  ( -9.342070512798265725, 0.000000000000000000, 10.59882438848031505 ) ) ;
#50777=CARTESIAN_POINT ( 'NONE',  ( -20.01713377844408726, -3.917936722690662066, 4.531652967349151240 ) ) ;
#50778=FACE_OUTER_BOUND ( 'NONE', #40748, .T. ) ;
#50779=FACE_OUTER_BOUND ( 'NONE', #22263, .T. ) ;
#50780=EDGE_CURVE ( 'NONE', #28121, #19288, #79, .T. ) ;
#50781=PLANE ( 'NONE',  #43009 ) ;
#50782=DIRECTION ( 'NONE',  ( 0.005961354470445682716, -0.6427876096865404731, -0.7660212471507180654 ) ) ;
#50783=CARTESIAN_POINT ( 'NONE',  ( -14.97008238625287646, -0.1191753592594189115, 4.434577441229718531 ) ) ;
#50784=ORIENTED_EDGE ( 'NONE', *, *, #46003, .F. ) ;
#50785=ADVANCED_FACE ( 'NONE', ( #26230 ), #26496, .F. ) ;
#50787=FACE_OUTER_BOUND ( 'NONE', #23766, .T. ) ;
#50788=EDGE_LOOP ( 'NONE', ( #24065, #7963, #30063 ) ) ;
#50789=EDGE_CURVE ( 'NONE', #6267, #2187, #34744, .T. ) ;
#50790=ORIENTED_EDGE ( 'NONE', *, *, #18991, .F. ) ;
#50791=CARTESIAN_POINT ( 'NONE',  ( -23.33693525117809386, 0.000000000000000000, 5.746789908705562944 ) ) ;
#50792=EDGE_CURVE ( 'NONE', #16631, #36118, #13462, .T. ) ;
#50793=ORIENTED_EDGE ( 'NONE', *, *, #10297, .F. ) ;
#50795=CARTESIAN_POINT ( 'NONE',  ( -20.99889245848062558, -3.917936722690661178, 11.26861632647862876 ) ) ;
#50796=AXIS2_PLACEMENT_3D ( 'NONE', #41070, #14139, #31466 ) ;
#50797=ORIENTED_EDGE ( 'NONE', *, *, #24550, .F. ) ;
#50798=ORIENTED_EDGE ( 'NONE', *, *, #25835, .T. ) ;
#50799=ORIENTED_EDGE ( 'NONE', *, *, #17379, .T. ) ;
#50800=LINE ( 'NONE', #49952, #55609 ) ;
#50802=LINE ( 'NONE', #3663, #386 ) ;
#50803=ORIENTED_EDGE ( 'NONE', *, *, #40211, .F. ) ;
#50804=VERTEX_POINT ( 'NONE', #30514 ) ;
#50805=DIRECTION ( 'NONE',  ( 0.007781995580012662783, 0.000000000000000000, -0.9999697198139514409 ) ) ;
#50806=DIRECTION ( 'NONE',  ( -0.005002170337468016433, -0.7660444431189770143, 0.6427681459581293666 ) ) ;
#50807=ORIENTED_EDGE ( 'NONE', *, *, #35694, .F. ) ;
#50808=DIRECTION ( 'NONE',  ( -0.6427681459581293666, -0.7660444431189770143, -0.005002170337467561935 ) ) ;
#50809=ORIENTED_EDGE ( 'NONE', *, *, #20186, .T. ) ;
#50810=DIRECTION ( 'NONE',  ( 0.005002170337468016433, -0.7660444431189770143, -0.6427681459581293666 ) ) ;
#50811=LINE ( 'NONE', #47397, #35779 ) ;
#50813=DIRECTION ( 'NONE',  ( -0.005002170337468016433, -0.7660444431189770143, 0.6427681459581293666 ) ) ;
#50814=EDGE_CURVE ( 'NONE', #42842, #10997, #44115, .T. ) ;
#50815=DIRECTION ( 'NONE',  ( 0.000000000000000000, 0.000000000000000000, 1.000000000000000000 ) ) ;
#50816=ORIENTED_EDGE ( 'NONE', *, *, #52869, .F. ) ;
#50817=DIRECTION ( 'NONE',  ( 0.6427681459581294776, -0.7660444431189769032, 0.005002170337467562802 ) ) ;
#50818=FACE_OUTER_BOUND ( 'NONE', #16487, .T. ) ;
#50819=DIRECTION ( 'NONE',  ( -0.6427681459581293666, -0.7660444431189770143, -0.005002170337467561935 ) ) ;
#50820=ORIENTED_EDGE ( 'NONE', *, *, #17947, .T. ) ;
#50821=EDGE_CURVE ( 'NONE', #16969, #21242, #43541, .T. ) ;
#50822=ADVANCED_FACE ( 'NONE', ( #1208 ), #21956, .F. ) ;
#50824=AXIS2_PLACEMENT_3D ( 'NONE', #34295, #25473, #12128 ) ;
#50825=CARTESIAN_POINT ( 'NONE',  ( -19.73447084723482448, 0.000000000000000000, 6.713495315519605100 ) ) ;
#50826=FACE_OUTER_BOUND ( 'NONE', #41037, .T. ) ;
#50827=CARTESIAN_POINT ( 'NONE',  ( -12.20237937974333953, -0.1191753592594185784, 7.041440834642125779 ) ) ;
#50828=CARTESIAN_POINT ( 'NONE',  ( -16.72785480207782527, 0.000000000000000000, 4.320895021734290964 ) ) ;
#50829=ADVANCED_FACE ( 'NONE', ( #31032 ), #17995, .F. ) ;
#50830=CARTESIAN_POINT ( 'NONE',  ( -16.81345671998191449, 0.000000000000000000, 3.412238694616132495 ) ) ;
#50831=LINE ( 'NONE', #8241, #7994 ) ;
#50832=AXIS2_PLACEMENT_3D ( 'NONE', #5460, #44623, #48634 ) ;
#50834=VERTEX_POINT ( 'NONE', #18251 ) ;
#50835=LINE ( 'NONE', #2837, #30772 ) ;
#50837=FACE_OUTER_BOUND ( 'NONE', #55220, .T. ) ;
#50838=ORIENTED_EDGE ( 'NONE', *, *, #30971, .F. ) ;
#50839=CARTESIAN_POINT ( 'NONE',  ( -18.21825225188358743, -0.1191753592594171213, 3.858214293418511076 ) ) ;
#50840=CARTESIAN_POINT ( 'NONE',  ( -20.29238058347068829, -4.727446477803161073, 12.32272654073281259 ) ) ;
#50841=DIRECTION ( 'NONE',  ( 0.007781995580012663651, 0.000000000000000000, -0.9999697198139515519 ) ) ;
#50842=CARTESIAN_POINT ( 'NONE',  ( -11.47218654453707032, 0.000000000000000000, 1.237813275329368690 ) ) ;
#50843=ADVANCED_FACE ( 'NONE', ( #52899 ), #41527, .F. ) ;
#50844=LINE ( 'NONE', #33283, #34722 ) ;
#50845=ORIENTED_EDGE ( 'NONE', *, *, #32348, .F. ) ;
#50847=ADVANCED_FACE ( 'NONE', ( #15391 ), #14846, .F. ) ;
#50848=FACE_OUTER_BOUND ( 'NONE', #26578, .T. ) ;
#50849=CARTESIAN_POINT ( 'NONE',  ( -16.92497469253532927, 0.000000000000000000, 3.950028919360522917 ) ) ;
#50850=EDGE_CURVE ( 'NONE', #13341, #49579, #32705, .T. ) ;
#50851=VECTOR ( 'NONE', #2475, 1000.000000000000000 ) ;
#50852=ORIENTED_EDGE ( 'NONE', *, *, #45043, .F. ) ;
#50853=PLANE ( 'NONE',  #32244 ) ;
#50854=ORIENTED_EDGE ( 'NONE', *, *, #15787, .F. ) ;
#50855=DIRECTION ( 'NONE',  ( 0.9321478471874541372, 0.000000000000000000, -0.3620778797217453771 ) ) ;
#50856=EDGE_CURVE ( 'NONE', #32088, #32467, #6075, .T. ) ;
#50857=EDGE_LOOP ( 'NONE', ( #39447, #40770, #11484, #51639 ) ) ;
#50859=ORIENTED_EDGE ( 'NONE', *, *, #37762, .T. ) ;
#50860=CARTESIAN_POINT ( 'NONE',  ( -18.67619601524082285, 0.000000000000000000, 3.936400510096834893 ) ) ;
#50861=CARTESIAN_POINT ( 'NONE',  ( -14.56888064431065821, -0.1191753592594197858, 12.58947452739191064 ) ) ;
#50862=DIRECTION ( 'NONE',  ( 0.007781995580012663651, -3.146120232559066537E-19, -0.9999697198139514409 ) ) ;
#50863=AXIS2_PLACEMENT_3D ( 'NONE', #51175, #12837, #56018 ) ;
#50864=DIRECTION ( 'NONE',  ( -0.6427681459581293666, -0.7660444431189770143, -0.005002170337467561935 ) ) ;
#50865=ORIENTED_EDGE ( 'NONE', *, *, #29936, .F. ) ;
#50866=AXIS2_PLACEMENT_3D ( 'NONE', #19576, #19014, #9945 ) ;
#50867=ORIENTED_EDGE ( 'NONE', *, *, #32047, .F. ) ;
#50868=ORIENTED_EDGE ( 'NONE', *, *, #10738, .T. ) ;
#50869=LINE ( 'NONE', #47174, #18660 ) ;
#50871=VERTEX_POINT ( 'NONE', #15657 ) ;
#50872=DIRECTION ( 'NONE',  ( -0.5449076811759708816, 0.6444004775717707689, 0.5364919789714475140 ) ) ;
#50873=ORIENTED_EDGE ( 'NONE', *, *, #15449, .T. ) ;
#50874=PLANE ( 'NONE',  #31489 ) ;
#50875=PLANE ( 'NONE',  #36705 ) ;
#50876=ORIENTED_EDGE ( 'NONE', *, *, #25658, .F. ) ;
#50877=FACE_OUTER_BOUND ( 'NONE', #28832, .T. ) ;
#50878=ORIENTED_EDGE ( 'NONE', *, *, #40090, .F. ) ;
#50879=CARTESIAN_POINT ( 'NONE',  ( -9.841832199969237749, -0.1191753592594186895, 2.258494251131236030 ) ) ;
#50880=CARTESIAN_POINT ( 'NONE',  ( -11.82414738691523581, 0.000000000000000000, 5.297727002544709407 ) ) ;
#50881=ORIENTED_EDGE ( 'NONE', *, *, #8580, .T. ) ;
#50882=DIRECTION ( 'NONE',  ( 0.005961354470445682716, -0.6427876096865404731, -0.7660212471507180654 ) ) ;
#50883=PLANE ( 'NONE',  #16648 ) ;
#50884=LINE ( 'NONE', #33863, #26891 ) ;
#50885=DIRECTION ( 'NONE',  ( 0.6427681459581294776, -0.7660444431189769032, 0.005002170337467562802 ) ) ;
#50886=VERTEX_POINT ( 'NONE', #49192 ) ;
#50887=ADVANCED_FACE ( 'NONE', ( #6594 ), #37246, .F. ) ;
#50888=VECTOR ( 'NONE', #53114, 1000.000000000000000 ) ;
#50889=ORIENTED_EDGE ( 'NONE', *, *, #6082, .F. ) ;
#50890=AXIS2_PLACEMENT_3D ( 'NONE', #40289, #26662, #27810 ) ;
#50891=DIRECTION ( 'NONE',  ( -0.005002170337468016433, -0.7660444431189770143, 0.6427681459581293666 ) ) ;
#50892=DIRECTION ( 'NONE',  ( 0.9999697198139515519, 0.000000000000000000, 0.007781995580013368816 ) ) ;
#50894=EDGE_CURVE ( 'NONE', #37968, #37323, #28448, .T. ) ;
#50896=LINE ( 'NONE', #33872, #35800 ) ;
#50897=CARTESIAN_POINT ( 'NONE',  ( -21.77789634727513857, -5.375054281893161701, 13.96258604752399712 ) ) ;
#50898=FACE_OUTER_BOUND ( 'NONE', #46268, .T. ) ;
#50899=ORIENTED_EDGE ( 'NONE', *, *, #4292, .F. ) ;
#50900=CARTESIAN_POINT ( 'NONE',  ( -15.34699672469169762, 0.000000000000000000, 6.008975514032165677 ) ) ;
#50901=CARTESIAN_POINT ( 'NONE',  ( -16.79925329029790149, 0.000000000000000000, 13.49544742625427496 ) ) ;
#50902=VERTEX_POINT ( 'NONE', #23914 ) ;
#50903=CARTESIAN_POINT ( 'NONE',  ( -12.33850799832341849, 0.000000000000000000, 11.68350162852954632 ) ) ;
#50904=ORIENTED_EDGE ( 'NONE', *, *, #40404, .F. ) ;
#50905=CARTESIAN_POINT ( 'NONE',  ( -9.287916345609888324, 0.000000000000000000, 3.640130203506913631 ) ) ;
#50906=LINE ( 'NONE', #29347, #4264 ) ;
#50907=DIRECTION ( 'NONE',  ( -0.5449076811759708816, 0.6444004775717707689, 0.5364919789714475140 ) ) ;
#50908=DIRECTION ( 'NONE',  ( -0.005961354470445682716, -0.6427876096865404731, 0.7660212471507180654 ) ) ;
#50909=VECTOR ( 'NONE', #35267, 999.9999999999998863 ) ;
#50911=ORIENTED_EDGE ( 'NONE', *, *, #51742, .T. ) ;
#50912=VERTEX_POINT ( 'NONE', #31881 ) ;
#50914=CARTESIAN_POINT ( 'NONE',  ( 2.072287782118878319, 0.000000000000000000, -2.950529333540147015 ) ) ;
#50916=DIRECTION ( 'NONE',  ( 0.9999697198139515519, 0.000000000000000000, 0.007781995580013368816 ) ) ;
#50917=FACE_OUTER_BOUND ( 'NONE', #13486, .T. ) ;
#50918=CARTESIAN_POINT ( 'NONE',  ( -18.19747506107908563, 0.000000000000000000, 14.03856424583689311 ) ) ;
#50920=CARTESIAN_POINT ( 'NONE',  ( -12.63540168802631669, -0.1191753592594192307, 2.975418187038710194 ) ) ;
#50921=ADVANCED_FACE ( 'NONE', ( #5771 ), #2607, .F. ) ;
#50922=DIRECTION ( 'NONE',  ( -0.5364919789714478471, 0.6444004775717705469, -0.5449076811759709926 ) ) ;
#50923=DIRECTION ( 'NONE',  ( -0.7660212471507179544, -0.6427876096865405842, -0.005961354470445141482 ) ) ;
#50924=EDGE_LOOP ( 'NONE', ( #48575, #27001, #41287, #7284, #938 ) ) ;
#50925=EDGE_CURVE ( 'NONE', #9595, #21126, #45228, .T. ) ;
#50927=DIRECTION ( 'NONE',  ( 0.6427681459581294776, -0.7660444431189769032, 0.005002170337467562802 ) ) ;
#50928=DIRECTION ( 'NONE',  ( 0.9999697198139515519, 0.000000000000000000, 0.007781995580013368816 ) ) ;
#50929=VERTEX_POINT ( 'NONE', #23381 ) ;
#50930=AXIS2_PLACEMENT_3D ( 'NONE', #20045, #45615, #37367 ) ;
#50931=AXIS2_PLACEMENT_3D ( 'NONE', #34170, #52321, #17368 ) ;
#50932=CARTESIAN_POINT ( 'NONE',  ( -10.74029228357944987, 0.000000000000000000, 11.14194120806293320 ) ) ;
#50933=EDGE_CURVE ( 'NONE', #16128, #55340, #2334, .T. ) ;
#50934=VERTEX_POINT ( 'NONE', #2033 ) ;
#50935=ORIENTED_EDGE ( 'NONE', *, *, #22906, .F. ) ;
#50936=ORIENTED_EDGE ( 'NONE', *, *, #52997, .F. ) ;
#50937=VECTOR ( 'NONE', #46751, 1000.000000000000227 ) ;
#50938=VERTEX_POINT ( 'NONE', #14565 ) ;
#50939=LINE ( 'NONE', #20004, #16628 ) ;
#50942=ORIENTED_EDGE ( 'NONE', *, *, #4977, .T. ) ;
#50943=CARTESIAN_POINT ( 'NONE',  ( -12.17076479118523302, -0.1191753592594189115, 2.979034098806719211 ) ) ;
#50944=ORIENTED_EDGE ( 'NONE', *, *, #40614, .F. ) ;
#50945=VECTOR ( 'NONE', #55876, 999.9999999999998863 ) ;
#50946=VERTEX_POINT ( 'NONE', #49495 ) ;
#50947=VECTOR ( 'NONE', #55287, 999.9999999999998863 ) ;
#50948=DIRECTION ( 'NONE',  ( -0.5364919789714478471, 0.6444004775717705469, -0.5449076811759709926 ) ) ;
#50949=PLANE ( 'NONE',  #53872 ) ;
#50950=PLANE ( 'NONE',  #41254 ) ;
#50951=CARTESIAN_POINT ( 'NONE',  ( -19.60834386242827776, 0.000000000000000000, 4.298478389818581213 ) ) ;
#50952=ADVANCED_FACE ( 'NONE', ( #54293 ), #49765, .F. ) ;
#50953=CARTESIAN_POINT ( 'NONE',  ( -14.42280954203746646, -4.403642575758160760, 9.511368448867619563 ) ) ;
#50954=ORIENTED_EDGE ( 'NONE', *, *, #47250, .F. ) ;
#50955=ORIENTED_EDGE ( 'NONE', *, *, #28368, .T. ) ;
#50956=DIRECTION ( 'NONE',  ( -0.2426528472758542054, 0.7422098413412800966, -0.6246952433987894571 ) ) ;
#50957=LINE ( 'NONE', #10955, #7642 ) ;
#50958=EDGE_CURVE ( 'NONE', #27743, #661, #36415, .T. ) ;
#50959=CARTESIAN_POINT ( 'NONE',  ( -13.53673582514181106, 0.000000000000000000, 12.22817484722816772 ) ) ;
#50961=PLANE ( 'NONE',  #52131 ) ;
#50962=CARTESIAN_POINT ( 'NONE',  ( -13.97153759768243297, -2.784623065533160524, 6.678992260915761037 ) ) ;
#50963=VERTEX_POINT ( 'NONE', #6331 ) ;
#50964=VECTOR ( 'NONE', #2229, 999.9999999999998863 ) ;
#50965=LINE ( 'NONE', #30556, #22981 ) ;
#50967=VERTEX_POINT ( 'NONE', #23631 ) ;
#50968=AXIS2_PLACEMENT_3D ( 'NONE', #54479, #18835, #15580 ) ;
#50969=VECTOR ( 'NONE', #16757, 999.9999999999998863 ) ;
#50970=LINE ( 'NONE', #29415, #1651 ) ;
#50971=PLANE ( 'NONE',  #21449 ) ;
#50972=PLANE ( 'NONE',  #7272 ) ;
#50973=DIRECTION ( 'NONE',  ( -0.5449076811759708816, 0.6444004775717707689, 0.5364919789714475140 ) ) ;
#50974=DIRECTION ( 'NONE',  ( -0.6427681459581293666, -0.7660444431189770143, -0.005002170337467561935 ) ) ;
#50975=ADVANCED_FACE ( 'NONE', ( #36707 ), #54027, .F. ) ;
#50976=ORIENTED_EDGE ( 'NONE', *, *, #38355, .T. ) ;
#50977=AXIS2_PLACEMENT_3D ( 'NONE', #34894, #30890, #26349 ) ;
#50978=AXIS2_PLACEMENT_3D ( 'NONE', #18213, #48308, #9423 ) ;
#50979=ORIENTED_EDGE ( 'NONE', *, *, #44341, .T. ) ;
#50980=DIRECTION ( 'NONE',  ( -0.005002170337468016433, -0.7660444431189770143, 0.6427681459581293666 ) ) ;
#50981=CARTESIAN_POINT ( 'NONE',  ( -10.87475521869608919, 0.000000000000000000, 2.719790903276377403 ) ) ;
#50982=DIRECTION ( 'NONE',  ( 0.5449076811759707706, 0.6444004775717708799, -0.5364919789714476250 ) ) ;
#50983=DIRECTION ( 'NONE',  ( 0.005961354470445682716, -0.6427876096865404731, -0.7660212471507180654 ) ) ;
#50985=DIRECTION ( 'NONE',  ( -0.8531650599175527594, 0.4028455766673922356, 0.3313982828793700652 ) ) ;
#50986=DIRECTION ( 'NONE',  ( 0.5449076811759707706, 0.6444004775717708799, -0.5364919789714476250 ) ) ;
#50987=LINE ( 'NONE', #55836, #6598 ) ;
#50988=LINE ( 'NONE', #51298, #31412 ) ;
#50990=DIRECTION ( 'NONE',  ( -0.005961354470445682716, -0.6427876096865404731, 0.7660212471507180654 ) ) ;
#50991=ORIENTED_EDGE ( 'NONE', *, *, #49438, .T. ) ;
#50992=LINE ( 'NONE', #20899, #30418 ) ;
#50993=EDGE_LOOP ( 'NONE', ( #51074, #49254, #35793, #14991 ) ) ;
#50994=EDGE_CURVE ( 'NONE', #52435, #40267, #32460, .T. ) ;
#50995=AXIS2_PLACEMENT_3D ( 'NONE', #28087, #2232, #45144 ) ;
#50996=ORIENTED_EDGE ( 'NONE', *, *, #45979, .F. ) ;
#50997=ORIENTED_EDGE ( 'NONE', *, *, #2738, .F. ) ;
#50998=ORIENTED_EDGE ( 'NONE', *, *, #37873, .T. ) ;
#50999=ORIENTED_EDGE ( 'NONE', *, *, #54678, .T. ) ;
#51000=ORIENTED_EDGE ( 'NONE', *, *, #21133, .F. ) ;
#51001=VECTOR ( 'NONE', #16569, 1000.000000000000227 ) ;
#51002=DIRECTION ( 'NONE',  ( 0.005961354470445682716, -0.6427876096865404731, -0.7660212471507180654 ) ) ;
#51003=DIRECTION ( 'NONE',  ( -0.6427681459581293666, -0.7660444431189770143, -0.005002170337467561935 ) ) ;
#51004=CARTESIAN_POINT ( 'NONE',  ( -25.20200914511100265, -0.1191753592594197858, 6.570942640130446932 ) ) ;
#51005=ADVANCED_FACE ( 'NONE', ( #25588 ), #55997, .F. ) ;
#51007=VERTEX_POINT ( 'NONE', #37835 ) ;
#51008=DIRECTION ( 'NONE',  ( 0.000000000000000000, -0.000000000000000000, -1.000000000000000000 ) ) ;
#51009=ORIENTED_EDGE ( 'NONE', *, *, #7532, .F. ) ;
#51010=CARTESIAN_POINT ( 'NONE',  ( -19.60834386242827776, 0.000000000000000000, 4.298478389818581213 ) ) ;
#51011=EDGE_CURVE ( 'NONE', #46331, #34260, #17090, .T. ) ;
#51012=EDGE_LOOP ( 'NONE', ( #227, #8449, #50589, #31632 ) ) ;
#51013=EDGE_CURVE ( 'NONE', #37711, #55849, #38676, .T. ) ;
#51014=AXIS2_PLACEMENT_3D ( 'NONE', #2670, #54627, #15733 ) ;
#51015=VECTOR ( 'NONE', #43390, 999.9999999999998863 ) ;
#51017=CARTESIAN_POINT ( 'NONE',  ( -9.342070512798265725, 0.000000000000000000, 10.59882438848031505 ) ) ;
#51019=ADVANCED_FACE ( 'NONE', ( #16233 ), #15963, .F. ) ;
#51020=EDGE_LOOP ( 'NONE', ( #54016, #17086, #28471, #19466 ) ) ;
#51021=DIRECTION ( 'NONE',  ( -0.5449076811759708816, 0.6444004775717707689, 0.5364919789714475140 ) ) ;
#51022=ORIENTED_EDGE ( 'NONE', *, *, #10810, .T. ) ;
#51023=FACE_OUTER_BOUND ( 'NONE', #43683, .T. ) ;
#51024=EDGE_CURVE ( 'NONE', #1477, #36530, #34406, .T. ) ;
#51025=AXIS2_PLACEMENT_3D ( 'NONE', #41127, #2214, #19551 ) ;
#51026=DIRECTION ( 'NONE',  ( -0.7660212471507179544, -0.6427876096865405842, -0.005961354470445141482 ) ) ;
#51027=VECTOR ( 'NONE', #40775, 1000.000000000000227 ) ;
#51028=EDGE_CURVE ( 'NONE', #7819, #26523, #51456, .T. ) ;
#51029=DIRECTION ( 'NONE',  ( -0.9999697198139514409, -0.000000000000000000, -0.007781995580013368816 ) ) ;
#51030=CARTESIAN_POINT ( 'NONE',  ( -14.52490551429942656, -3.432230869623160263, 7.956773887985201021 ) ) ;
#51031=DIRECTION ( 'NONE',  ( 0.007781995580012663651, 0.000000000000000000, -0.9999697198139515519 ) ) ;
#51032=CARTESIAN_POINT ( 'NONE',  ( -18.15625413466447569, 0.000000000000000000, 8.741763725523435724 ) ) ;
#51033=CARTESIAN_POINT ( 'NONE',  ( -12.88624579210203436, -4.241740624735661491, 8.648806222517640308 ) ) ;
#51034=CARTESIAN_POINT ( 'NONE',  ( -11.13652411806909903, 0.000000000000000000, 2.348421687366606392 ) ) ;
#51035=VERTEX_POINT ( 'NONE', #55403 ) ;
#51036=FACE_OUTER_BOUND ( 'NONE', #48063, .T. ) ;
#51037=ORIENTED_EDGE ( 'NONE', *, *, #12524, .T. ) ;
#51038=VECTOR ( 'NONE', #5031, 1000.000000000000227 ) ;
#51039=EDGE_CURVE ( 'NONE', #32426, #31757, #46312, .T. ) ;
#51040=LINE ( 'NONE', #3631, #31089 ) ;
#51041=DIRECTION ( 'NONE',  ( 0.005961354470445682716, -0.6427876096865404731, -0.7660212471507180654 ) ) ;
#51042=CARTESIAN_POINT ( 'NONE',  ( -20.18285418839233714, 0.000000000000000000, 4.621332403721110538 ) ) ;
#51043=VECTOR ( 'NONE', #42611, 1000.000000000000227 ) ;
#51044=CARTESIAN_POINT ( 'NONE',  ( -14.61041236884574879, 0.000000000000000000, 5.076037587973862841 ) ) ;
#51045=PLANE ( 'NONE',  #30410 ) ;
#51046=ADVANCED_FACE ( 'NONE', ( #16804 ), #46914, .F. ) ;
#51047=LINE ( 'NONE', #33465, #48250 ) ;
#51049=ORIENTED_EDGE ( 'NONE', *, *, #39477, .T. ) ;
#51050=CARTESIAN_POINT ( 'NONE',  ( -12.38502494873981163, 1.257817950434005683, 1.452565040780329886 ) ) ;
#51051=VECTOR ( 'NONE', #14497, 1000.000000000000114 ) ;
#51052=DIRECTION ( 'NONE',  ( 0.005002170337468016433, -0.7660444431189770143, -0.6427681459581293666 ) ) ;
#51053=CARTESIAN_POINT ( 'NONE',  ( -11.20636620717317378, 0.000000000000000000, 11.32298014792380414 ) ) ;
#51054=CARTESIAN_POINT ( 'NONE',  ( -21.47419595591918906, 0.000000000000000000, 5.222628093224860102 ) ) ;
#51055=VECTOR ( 'NONE', #41638, 1000.000000000000227 ) ;
#51056=VECTOR ( 'NONE', #17608, 1000.000000000000227 ) ;
#51057=LINE ( 'NONE', #11622, #10976 ) ;
#51058=DIRECTION ( 'NONE',  ( -0.7660212471507179544, -0.6427876096865405842, -0.005961354470445141482 ) ) ;
#51059=DIRECTION ( 'NONE',  ( 0.5364919789714477361, 0.6444004775717706579, 0.5449076811759711036 ) ) ;
#51060=CARTESIAN_POINT ( 'NONE',  ( -18.19747506107908563, 0.000000000000000000, 14.03856424583689311 ) ) ;
#51062=AXIS2_PLACEMENT_3D ( 'NONE', #41997, #3098, #20431 ) ;
#51063=DIRECTION ( 'NONE',  ( 0.7660212471507180654, -0.6427876096865404731, 0.005961354470445141482 ) ) ;
#51064=AXIS2_PLACEMENT_3D ( 'NONE', #49472, #44086, #27050 ) ;
#51065=LINE ( 'NONE', #46239, #18850 ) ;
#51066=VERTEX_POINT ( 'NONE', #50604 ) ;
#51067=ORIENTED_EDGE ( 'NONE', *, *, #10725, .T. ) ;
#51069=ORIENTED_EDGE ( 'NONE', *, *, #49848, .F. ) ;
#51070=ADVANCED_FACE ( 'NONE', ( #55696 ), #12554, .F. ) ;
#51071=CARTESIAN_POINT ( 'NONE',  ( -14.00280974873554030, 0.000000000000000000, 12.40921378708904044 ) ) ;
#51072=VECTOR ( 'NONE', #6986, 999.9999999999998863 ) ;
#51073=ORIENTED_EDGE ( 'NONE', *, *, #38751, .T. ) ;
#51074=ORIENTED_EDGE ( 'NONE', *, *, #16748, .F. ) ;
#51075=ORIENTED_EDGE ( 'NONE', *, *, #18478, .T. ) ;
#51077=FACE_OUTER_BOUND ( 'NONE', #28783, .T. ) ;
#51078=CARTESIAN_POINT ( 'NONE',  ( -14.01701317841955508, 0.000000000000000000, 2.326005055450897085 ) ) ;
#51079=PLANE ( 'NONE',  #42093 ) ;
#51080=EDGE_CURVE ( 'NONE', #9247, #19141, #7423, .T. ) ;
#51081=VECTOR ( 'NONE', #99, 1000.000000000000227 ) ;
#51082=EDGE_CURVE ( 'NONE', #48904, #51697, #33834, .T. ) ;
#51083=VERTEX_POINT ( 'NONE', #21042 ) ;
#51084=EDGE_LOOP ( 'NONE', ( #33758, #21205, #46918, #12146 ) ) ;
#51085=AXIS2_PLACEMENT_3D ( 'NONE', #50297, #46049, #7156 ) ;
#51086=ADVANCED_FACE ( 'NONE', ( #7723 ), #8013, .F. ) ;
#51087=FACE_OUTER_BOUND ( 'NONE', #19745, .T. ) ;
#51088=CARTESIAN_POINT ( 'NONE',  ( -20.54049170961573267, 0.000000000000000000, 4.660556269540326646 ) ) ;
#51089=EDGE_LOOP ( 'NONE', ( #53704, #33487, #38315, #55159 ) ) ;
#51090=AXIS2_PLACEMENT_3D ( 'NONE', #54484, #37456, #54775 ) ;
#51091=DIRECTION ( 'NONE',  ( -0.7660212471507179544, -0.6427876096865405842, -0.005961354470445141482 ) ) ;
#51092=CARTESIAN_POINT ( 'NONE',  ( -12.80458192191714595, 0.000000000000000000, 11.86454056839041726 ) ) ;
#51093=ORIENTED_EDGE ( 'NONE', *, *, #22579, .T. ) ;
#51094=DIRECTION ( 'NONE',  ( 0.000000000000000000, -1.000000000000000000, 0.000000000000000000 ) ) ;
#51095=DIRECTION ( 'NONE',  ( -0.7660212471507179544, -0.6427876096865405842, -0.005961354470445141482 ) ) ;
#51096=AXIS2_PLACEMENT_3D ( 'NONE', #19395, #36737, #17668 ) ;
#51097=VECTOR ( 'NONE', #44241, 999.9999999999998863 ) ;
#51098=ORIENTED_EDGE ( 'NONE', *, *, #48178, .F. ) ;
#51099=FACE_OUTER_BOUND ( 'NONE', #44081, .T. ) ;
#51100=ADVANCED_FACE ( 'NONE', ( #25056 ), #29603, .F. ) ;
#51101=ADVANCED_FACE ( 'NONE', ( #7167 ), #8271, .F. ) ;
#51102=VECTOR ( 'NONE', #8195, 1000.000000000000227 ) ;
#51103=LINE ( 'NONE', #46865, #4634 ) ;
#51104=VECTOR ( 'NONE', #44789, 1000.000000000000114 ) ;
#51105=ORIENTED_EDGE ( 'NONE', *, *, #44876, .T. ) ;
#51106=DIRECTION ( 'NONE',  ( 0.7660212471507180654, -0.6427876096865404731, 0.005961354470445141482 ) ) ;
#51107=DIRECTION ( 'NONE',  ( -0.9999697198139514409, -0.000000000000000000, -0.007781995580013368816 ) ) ;
#51108=CARTESIAN_POINT ( 'NONE',  ( -0.8462754142284378833, 3.710276453311750267, 3.547095686184165153 ) ) ;
#51109=CARTESIAN_POINT ( 'NONE',  ( -18.91945046336710590, 0.000000000000000000, 8.935830411442143628 ) ) ;
#51110=ORIENTED_EDGE ( 'NONE', *, *, #15465, .F. ) ;
#51111=ADVANCED_FACE ( 'NONE', ( #54852 ), #24746, .F. ) ;
#51112=DIRECTION ( 'NONE',  ( -0.005961354470445682716, -0.6427876096865404731, 0.7660212471507180654 ) ) ;
#51113=CARTESIAN_POINT ( 'NONE',  ( -15.89273142772683300, -0.1134144341942070200, 2.954903030296413657 ) ) ;
#51114=LINE ( 'NONE', #21600, #27633 ) ;
#51115=DIRECTION ( 'NONE',  ( -0.6427681459581293666, -0.7660444431189770143, -0.005002170337467561935 ) ) ;
#51116=DIRECTION ( 'NONE',  ( -0.005002170337468016433, -0.7660444431189770143, 0.6427681459581293666 ) ) ;
#51117=DIRECTION ( 'NONE',  ( 0.5364919789714477361, 0.6444004775717706579, 0.5449076811759711036 ) ) ;
#51119=AXIS2_PLACEMENT_3D ( 'NONE', #50615, #50025, #32473 ) ;
#51122=LINE ( 'NONE', #20754, #26918 ) ;
#51123=ORIENTED_EDGE ( 'NONE', *, *, #47856, .T. ) ;
#51124=DIRECTION ( 'NONE',  ( -0.005961354470445682716, -0.6427876096865404731, 0.7660212471507180654 ) ) ;
#51125=FACE_OUTER_BOUND ( 'NONE', #35263, .T. ) ;
#51126=VECTOR ( 'NONE', #9867, 1000.000000000000114 ) ;
#51127=CARTESIAN_POINT ( 'NONE',  ( -19.30004991711850337, -4.727446477803165514, 4.227285643902905399 ) ) ;
#51128=VECTOR ( 'NONE', #38847, 1000.000000000000227 ) ;
#51129=LINE ( 'NONE', #12237, #40564 ) ;
#51130=PLANE ( 'NONE',  #28387 ) ;
#51132=ORIENTED_EDGE ( 'NONE', *, *, #42151, .F. ) ;
#51134=VECTOR ( 'NONE', #55998, 1000.000000000000227 ) ;
#51135=DIRECTION ( 'NONE',  ( 0.9321478471874540261, 0.000000000000000000, -0.3620778797217457101 ) ) ;
#51136=ORIENTED_EDGE ( 'NONE', *, *, #53604, .F. ) ;
#51137=ADVANCED_FACE ( 'NONE', ( #52552 ), #610, .F. ) ;
#51138=VECTOR ( 'NONE', #55106, 999.9999999999998863 ) ;
#51139=LINE ( 'NONE', #32695, #13004 ) ;
#51140=ORIENTED_EDGE ( 'NONE', *, *, #23995, .F. ) ;
#51141=CARTESIAN_POINT ( 'NONE',  ( -14.01701317841955508, 0.000000000000000000, 2.326005055450897085 ) ) ;
#51142=EDGE_CURVE ( 'NONE', #6164, #34166, #22735, .T. ) ;
#51143=EDGE_LOOP ( 'NONE', ( #30850, #32179, #30796, #44212 ) ) ;
#51144=FACE_OUTER_BOUND ( 'NONE', #38042, .T. ) ;
#51145=VECTOR ( 'NONE', #1889, 1000.000000000000227 ) ;
#51146=ORIENTED_EDGE ( 'NONE', *, *, #36244, .T. ) ;
#51147=VECTOR ( 'NONE', #24266, 1000.000000000000227 ) ;
#51148=EDGE_LOOP ( 'NONE', ( #43890, #23779, #18256, #25301 ) ) ;
#51149=ORIENTED_EDGE ( 'NONE', *, *, #13831, .T. ) ;
#51150=ADVANCED_FACE ( 'NONE', ( #40049 ), #39790, .F. ) ;
#51151=LINE ( 'NONE', #47760, #307 ) ;
#51152=CARTESIAN_POINT ( 'NONE',  ( -26.13415699229845757, -0.1191753592594197858, 6.933020519852192365 ) ) ;
#51153=CARTESIAN_POINT ( 'NONE',  ( -15.94144280372852762, 2.714935509636508204, 2.787508833130166952 ) ) ;
#51155=EDGE_CURVE ( 'NONE', #23097, #2132, #47455, .T. ) ;
#51156=ADVANCED_FACE ( 'NONE', ( #13404 ), #35513, .F. ) ;
#51157=DIRECTION ( 'NONE',  ( 0.9999697198139515519, 0.000000000000000000, 0.007781995580013368816 ) ) ;
#51158=ORIENTED_EDGE ( 'NONE', *, *, #46593, .T. ) ;
#51159=ORIENTED_EDGE ( 'NONE', *, *, #10565, .F. ) ;
#51160=AXIS2_PLACEMENT_3D ( 'NONE', #13807, #23196, #40785 ) ;
#51161=ORIENTED_EDGE ( 'NONE', *, *, #2385, .F. ) ;
#51162=LINE ( 'NONE', #33558, #20462 ) ;
#51163=LINE ( 'NONE', #21, #20368 ) ;
#51164=ORIENTED_EDGE ( 'NONE', *, *, #46529, .F. ) ;
#51165=CARTESIAN_POINT ( 'NONE',  ( -15.11879971925641009, 4.981562823951510843, 10.92956963961542982 ) ) ;
#51166=VERTEX_POINT ( 'NONE', #30964 ) ;
#51167=AXIS2_PLACEMENT_3D ( 'NONE', #22569, #22832, #23128 ) ;
#51168=LINE ( 'NONE', #42931, #15149 ) ;
#51169=FACE_OUTER_BOUND ( 'NONE', #12688, .T. ) ;
#51170=ORIENTED_EDGE ( 'NONE', *, *, #18549, .F. ) ;
#51171=CARTESIAN_POINT ( 'NONE',  ( -17.26532721389163072, 0.000000000000000000, 13.67648636611514590 ) ) ;
#51172=ADVANCED_FACE ( 'NONE', ( #51707 ), #43744, .F. ) ;
#51173=ORIENTED_EDGE ( 'NONE', *, *, #35397, .F. ) ;
#51174=EDGE_CURVE ( 'NONE', #25200, #606, #48279, .T. ) ;
#51175=CARTESIAN_POINT ( 'NONE',  ( -21.47419595591918906, 0.000000000000000000, 5.222628093224860102 ) ) ;
#51176=LINE ( 'NONE', #13601, #31110 ) ;
#51177=AXIS2_PLACEMENT_3D ( 'NONE', #4419, #26263, #39630 ) ;
#51178=ORIENTED_EDGE ( 'NONE', *, *, #49239, .T. ) ;
#51179=CARTESIAN_POINT ( 'NONE',  ( -19.45503627000849889, -1.000000000000000000, 7.556996783084074742 ) ) ;
#51180=CARTESIAN_POINT ( 'NONE',  ( -8.570132709911630897, 0.000000000000000000, 5.123044440957987611 ) ) ;
#51181=EDGE_CURVE ( 'NONE', #16744, #16632, #9395, .T. ) ;
#51182=CARTESIAN_POINT ( 'NONE',  ( -16.54374430921337691, 2.876837460659007473, 3.016297672218315906 ) ) ;
#51183=VECTOR ( 'NONE', #10806, 1000.000000000000227 ) ;
#51184=LINE ( 'NONE', #11723, #30990 ) ;
#51185=ORIENTED_EDGE ( 'NONE', *, *, #45857, .T. ) ;
#51186=AXIS2_PLACEMENT_3D ( 'NONE', #2509, #41674, #54447 ) ;
#51187=EDGE_CURVE ( 'NONE', #17041, #54371, #13931, .T. ) ;
#51188=ORIENTED_EDGE ( 'NONE', *, *, #39402, .T. ) ;
#51190=DIRECTION ( 'NONE',  ( 0.7660212471507180654, -0.6427876096865404731, 0.005961354470445141482 ) ) ;
#51191=DIRECTION ( 'NONE',  ( 0.9999697198139515519, 0.000000000000000000, 0.007781995580013368816 ) ) ;
#51192=DIRECTION ( 'NONE',  ( 0.005961354470445682716, -0.6427876096865404731, -0.7660212471507180654 ) ) ;
#51193=ADVANCED_FACE ( 'NONE', ( #48585 ), #25898, .F. ) ;
#51194=PLANE ( 'NONE',  #54189 ) ;
#51195=AXIS2_PLACEMENT_3D ( 'NONE', #17147, #30202, #13168 ) ;
#51196=AXIS2_PLACEMENT_3D ( 'NONE', #12065, #46413, #12382 ) ;
#51197=LINE ( 'NONE', #11467, #48507 ) ;
#51198=ORIENTED_EDGE ( 'NONE', *, *, #10071, .F. ) ;
#51199=DIRECTION ( 'NONE',  ( -0.5364919789714478471, 0.6444004775717705469, -0.5449076811759709926 ) ) ;
#51200=CARTESIAN_POINT ( 'NONE',  ( -9.908141408373387193, -0.1191753592594197858, 10.77908512878318703 ) ) ;
#51201=ORIENTED_EDGE ( 'NONE', *, *, #25075, .T. ) ;
#51202=CARTESIAN_POINT ( 'NONE',  ( -22.40478740399063895, 0.000000000000000000, 5.384712028983816623 ) ) ;
#51203=EDGE_LOOP ( 'NONE', ( #52233, #9108, #1962, #40114 ) ) ;
#51204=CARTESIAN_POINT ( 'NONE',  ( -16.53317331066696383, 0.000000000000000000, 13.31285208727739899 ) ) ;
#51205=DIRECTION ( 'NONE',  ( 0.007781995580012663651, 0.000000000000000000, -0.9999697198139515519 ) ) ;
#51207=DIRECTION ( 'NONE',  ( -0.005961354470445682716, -0.6427876096865404731, 0.7660212471507180654 ) ) ;
#51209=VECTOR ( 'NONE', #45091, 999.9999999999998863 ) ;
#51210=VERTEX_POINT ( 'NONE', #38948 ) ;
#51211=EDGE_LOOP ( 'NONE', ( #5420, #15970, #53292, #12632 ) ) ;
#51212=AXIS2_PLACEMENT_3D ( 'NONE', #24394, #7100, #49410 ) ;
#51214=FACE_OUTER_BOUND ( 'NONE', #24977, .T. ) ;
#51215=FACE_OUTER_BOUND ( 'NONE', #16198, .T. ) ;
#51216=VECTOR ( 'NONE', #38123, 999.9999999999998863 ) ;
#51217=DIRECTION ( 'NONE',  ( -0.7660212471507179544, -0.6427876096865405842, -0.005961354470445141482 ) ) ;
#51218=CARTESIAN_POINT ( 'NONE',  ( -13.62138192979224272, -0.1941918491731554897, 2.166132706095718508 ) ) ;
#51219=DIRECTION ( 'NONE',  ( 0.000000000000000000, -1.000000000000000000, 0.000000000000000000 ) ) ;
#51220=AXIS2_PLACEMENT_3D ( 'NONE', #36123, #44907, #6026 ) ;
#51221=ORIENTED_EDGE ( 'NONE', *, *, #7322, .F. ) ;
#51222=PLANE ( 'NONE',  #52832 ) ;
#51223=DIRECTION ( 'NONE',  ( -0.3620778797217457656, 0.000000000000000000, -0.9321478471874539151 ) ) ;
#51224=CARTESIAN_POINT ( 'NONE',  ( -15.60102546347950536, 0.000000000000000000, 12.95077420755565356 ) ) ;
#51225=VECTOR ( 'NONE', #51888, 1000.000000000000000 ) ;
#51226=VECTOR ( 'NONE', #2835, 999.9999999999998863 ) ;
#51227=ORIENTED_EDGE ( 'NONE', *, *, #27144, .T. ) ;
#51228=AXIS2_PLACEMENT_3D ( 'NONE', #22046, #30849, #31123 ) ;
#51230=DIRECTION ( 'NONE',  ( -0.7660212471507179544, -0.6427876096865405842, -0.005961354470445141482 ) ) ;
#51231=CARTESIAN_POINT ( 'NONE',  ( -16.44024919480531821, -2.946525016555658016, 7.903632366987483060 ) ) ;
#51232=AXIS2_PLACEMENT_3D ( 'NONE', #55371, #16470, #46879 ) ;
#51233=ADVANCED_FACE ( 'NONE', ( #298 ), #17344, .F. ) ;
#51234=ADVANCED_FACE ( 'NONE', ( #30436 ), #47761, .F. ) ;
#51236=LINE ( 'NONE', #39016, #22299 ) ;
#51237=EDGE_LOOP ( 'NONE', ( #20185, #44787, #49120, #38496 ) ) ;
#51238=ADVANCED_FACE ( 'NONE', ( #39208 ), #34981, .F. ) ;
#51239=VECTOR ( 'NONE', #53657, 1000.000000000000227 ) ;
#51241=VECTOR ( 'NONE', #2701, 1000.000000000000114 ) ;
#51243=ORIENTED_EDGE ( 'NONE', *, *, #45901, .T. ) ;
#51244=CARTESIAN_POINT ( 'NONE',  ( -23.33849165029409889, 0.000000000000000000, 5.946783852668351855 ) ) ;
#51245=EDGE_LOOP ( 'NONE', ( #6956, #38379, #25052, #55388 ) ) ;
#51247=EDGE_LOOP ( 'NONE', ( #54157, #25755, #3820, #42400 ) ) ;
#51249=ORIENTED_EDGE ( 'NONE', *, *, #43315, .T. ) ;
#51250=ORIENTED_EDGE ( 'NONE', *, *, #35532, .T. ) ;
#51251=AXIS2_PLACEMENT_3D ( 'NONE', #35955, #10078, #44432 ) ;
#51252=DIRECTION ( 'NONE',  ( 0.005002170337468016433, -0.7660444431189770143, -0.6427681459581293666 ) ) ;
#51253=DIRECTION ( 'NONE',  ( 0.5364919789714477361, 0.6444004775717706579, 0.5449076811759711036 ) ) ;
#51254=PLANE ( 'NONE',  #44008 ) ;
#51255=CARTESIAN_POINT ( 'NONE',  ( 2.072287782118878319, 0.000000000000000000, -2.950529333540147015 ) ) ;
#51256=CARTESIAN_POINT ( 'NONE',  ( -7.337759244690715832, 5.055610077911836697, -0.3681386936730630666 ) ) ;
#51257=AXIS2_PLACEMENT_3D ( 'NONE', #47274, #13759, #52401 ) ;
#51258=VERTEX_POINT ( 'NONE', #23843 ) ;
#51259=ORIENTED_EDGE ( 'NONE', *, *, #14359, .T. ) ;
#51260=DIRECTION ( 'NONE',  ( -0.7660212471507179544, -0.6427876096865405842, -0.005961354470445141482 ) ) ;
#51262=VECTOR ( 'NONE', #45374, 1000.000000000000227 ) ;
#51264=ADVANCED_FACE ( 'NONE', ( #45173 ), #6274, .F. ) ;
#51265=DIRECTION ( 'NONE',  ( 0.9999697198139515519, 0.000000000000000000, 0.007781995580013368816 ) ) ;
#51266=AXIS2_PLACEMENT_3D ( 'NONE', #38963, #29, #26187 ) ;
#51267=VECTOR ( 'NONE', #24611, 1000.000000000000114 ) ;
#51268=CARTESIAN_POINT ( 'NONE',  ( -13.53673582514181106, 0.000000000000000000, 12.22817484722816772 ) ) ;
#51269=EDGE_CURVE ( 'NONE', #25448, #39671, #1440, .T. ) ;
#51270=AXIS2_PLACEMENT_3D ( 'NONE', #24720, #11940, #46892 ) ;
#51271=DIRECTION ( 'NONE',  ( -0.005961354470445682716, -0.6427876096865404731, 0.7660212471507180654 ) ) ;
#51272=CARTESIAN_POINT ( 'NONE',  ( -12.70458494993575194, -0.1191753592594197858, 11.86531876794841978 ) ) ;
#51273=ORIENTED_EDGE ( 'NONE', *, *, #29298, .T. ) ;
#51274=DIRECTION ( 'NONE',  ( 0.5364919789714477361, 0.6444004775717706579, 0.5449076811759711036 ) ) ;
#51275=EDGE_CURVE ( 'NONE', #36877, #16502, #1708, .T. ) ;
#51276=CARTESIAN_POINT ( 'NONE',  ( -11.14071582596366383, 0.000000000000000000, 2.887047149919346634 ) ) ;
#51277=ORIENTED_EDGE ( 'NONE', *, *, #34056, .F. ) ;
#51278=VECTOR ( 'NONE', #37735, 999.9999999999998863 ) ;
#51280=CARTESIAN_POINT ( 'NONE',  ( -9.542064456761055524, 0.000000000000000000, 10.59726798936431180 ) ) ;
#51281=AXIS2_PLACEMENT_3D ( 'NONE', #11440, #6607, #10319 ) ;
#51282=DIRECTION ( 'NONE',  ( -0.9999697198139514409, -0.000000000000000000, -0.007781995580013368816 ) ) ;
#51283=EDGE_CURVE ( 'NONE', #14403, #12863, #1969, .T. ) ;
#51284=CARTESIAN_POINT ( 'NONE',  ( -12.35196013617144217, 1.743523803501505709, 4.540661504268221016 ) ) ;
#51285=FACE_OUTER_BOUND ( 'NONE', #24979, .T. ) ;
#51286=AXIS2_PLACEMENT_3D ( 'NONE', #27990, #31955, #45034 ) ;
#51287=ORIENTED_EDGE ( 'NONE', *, *, #53423, .T. ) ;
#51289=EDGE_LOOP ( 'NONE', ( #17075, #9995, #44126, #41642 ) ) ;
#51290=DIRECTION ( 'NONE',  ( -0.9999697198139514409, -0.000000000000000000, -0.007781995580013368816 ) ) ;
#51291=CARTESIAN_POINT ( 'NONE',  ( -13.08330893211609869, 0.000000000000000000, 1.763933231766363630 ) ) ;
#51292=FACE_OUTER_BOUND ( 'NONE', #2423, .T. ) ;
#51293=PLANE ( 'NONE',  #9235 ) ;
#51294=DIRECTION ( 'NONE',  ( -0.005961354470445682716, -0.6427876096865404731, 0.7660212471507180654 ) ) ;
#51296=DIRECTION ( 'NONE',  ( 0.7660212471507180654, -0.6427876096865404731, 0.005961354470445141482 ) ) ;
#51297=VECTOR ( 'NONE', #6879, 999.9999999999998863 ) ;
#51298=CARTESIAN_POINT ( 'NONE',  ( -20.54204810873173415, 0.000000000000000000, 4.860550213503115558 ) ) ;
#51299=DIRECTION ( 'NONE',  ( 0.005002170337468016433, -0.7660444431189770143, -0.6427681459581293666 ) ) ;
#51300=AXIS2_PLACEMENT_3D ( 'NONE', #26513, #40135, #9483 ) ;
#51301=CARTESIAN_POINT ( 'NONE',  ( -12.80458192191714595, 0.000000000000000000, 11.86454056839041726 ) ) ;
#51302=ORIENTED_EDGE ( 'NONE', *, *, #31232, .T. ) ;
#51303=LINE ( 'NONE', #26042, #24043 ) ;
#51304=VECTOR ( 'NONE', #16691, 1000.000000000000000 ) ;
#51305=EDGE_CURVE ( 'NONE', #32412, #24071, #36103, .T. ) ;
#51306=VERTEX_POINT ( 'NONE', #18783 ) ;
#51307=AXIS2_PLACEMENT_3D ( 'NONE', #27298, #44611, #39551 ) ;
#51308=ORIENTED_EDGE ( 'NONE', *, *, #47590, .T. ) ;
#51309=ADVANCED_FACE ( 'NONE', ( #14246 ), #45699, .F. ) ;
#51310=EDGE_CURVE ( 'NONE', #33398, #21014, #53406, .T. ) ;
#51311=ORIENTED_EDGE ( 'NONE', *, *, #11715, .T. ) ;
#51312=ORIENTED_EDGE ( 'NONE', *, *, #15340, .T. ) ;
#51313=VECTOR ( 'NONE', #20798, 999.9999999999998863 ) ;
#51314=ORIENTED_EDGE ( 'NONE', *, *, #56000, .F. ) ;
#51318=LINE ( 'NONE', #37697, #16729 ) ;
#51319=VECTOR ( 'NONE', #27120, 1000.000000000000000 ) ;
#51320=VECTOR ( 'NONE', #48162, 999.9999999999998863 ) ;
#51321=ORIENTED_EDGE ( 'NONE', *, *, #6055, .F. ) ;
#51322=DIRECTION ( 'NONE',  ( 0.005961354470445682716, -0.6427876096865404731, -0.7660212471507180654 ) ) ;
#51323=VECTOR ( 'NONE', #38017, 999.9999999999998863 ) ;
#51324=ORIENTED_EDGE ( 'NONE', *, *, #19630, .T. ) ;
#51326=VERTEX_POINT ( 'NONE', #44584 ) ;
#51327=EDGE_CURVE ( 'NONE', #29013, #55101, #32107, .T. ) ;
#51328=AXIS2_PLACEMENT_3D ( 'NONE', #35971, #9549, #18624 ) ;
#51329=AXIS2_PLACEMENT_3D ( 'NONE', #720, #43868, #48122 ) ;
#51330=DIRECTION ( 'NONE',  ( 0.6427681459581294776, -0.7660444431189769032, 0.005002170337467562802 ) ) ;
#51331=DIRECTION ( 'NONE',  ( 0.5364919789714477361, 0.6444004775717706579, 0.5449076811759711036 ) ) ;
#51332=PLANE ( 'NONE',  #35945 ) ;
#51333=ORIENTED_EDGE ( 'NONE', *, *, #12474, .F. ) ;
#51334=LINE ( 'NONE', #16127, #2903 ) ;
#51335=ORIENTED_EDGE ( 'NONE', *, *, #13612, .F. ) ;
#51336=LINE ( 'NONE', #34855, #20076 ) ;
#51337=DIRECTION ( 'NONE',  ( 0.005961354470445682716, -0.6427876096865404731, -0.7660212471507180654 ) ) ;
#51338=VECTOR ( 'NONE', #26701, 999.9999999999998863 ) ;
#51339=FACE_OUTER_BOUND ( 'NONE', #8267, .T. ) ;
#51340=CARTESIAN_POINT ( 'NONE',  ( -10.19678563399013527, 0.000000000000000000, 0.7424042488757021108 ) ) ;
#51341=LINE ( 'NONE', #25483, #49259 ) ;
#51342=CARTESIAN_POINT ( 'NONE',  ( -23.33693525117809386, 0.000000000000000000, 5.746789908705562944 ) ) ;
#51343=CARTESIAN_POINT ( 'NONE',  ( -26.13337879274045505, 0.000000000000000000, 6.833023547870798353 ) ) ;
#51344=LINE ( 'NONE', #47073, #15904 ) ;
#51347=EDGE_LOOP ( 'NONE', ( #46514, #54477, #31499, #53996 ) ) ;
#51348=AXIS2_PLACEMENT_3D ( 'NONE', #20551, #43269, #25631 ) ;
#51350=CARTESIAN_POINT ( 'NONE',  ( -16.53317331066696383, 0.000000000000000000, 13.31285208727739899 ) ) ;
#51351=DIRECTION ( 'NONE',  ( -0.9999697198139514409, -0.000000000000000000, -0.007781995580013368816 ) ) ;
#51352=EDGE_CURVE ( 'NONE', #32666, #54093, #2547, .T. ) ;
#51353=AXIS2_PLACEMENT_3D ( 'NONE', #15306, #49385, #6240 ) ;
#51354=DIRECTION ( 'NONE',  ( 0.9999697198139515519, 0.000000000000000000, 0.007781995580013368816 ) ) ;
#51355=DIRECTION ( 'NONE',  ( 0.000000000000000000, -1.000000000000000000, 0.000000000000000000 ) ) ;
#51356=VECTOR ( 'NONE', #26137, 999.9999999999998863 ) ;
#51357=DIRECTION ( 'NONE',  ( 0.005961354470445682716, -0.6427876096865404731, -0.7660212471507180654 ) ) ;
#51358=VECTOR ( 'NONE', #28408, 999.9999999999998863 ) ;
#51359=ORIENTED_EDGE ( 'NONE', *, *, #37050, .T. ) ;
#51360=DIRECTION ( 'NONE',  ( -0.9999697198139514409, -0.000000000000000000, -0.007781995580013368816 ) ) ;
#51361=DIRECTION ( 'NONE',  ( 0.6427681459581294776, -0.7660444431189769032, 0.005002170337467562802 ) ) ;
#51362=CARTESIAN_POINT ( 'NONE',  ( -15.77426360813536554, 4.657758921906511418, 10.65275670580245482 ) ) ;
#51363=VECTOR ( 'NONE', #46230, 1000.000000000000114 ) ;
#51364=EDGE_CURVE ( 'NONE', #35036, #26534, #49707, .T. ) ;
#51365=AXIS2_PLACEMENT_3D ( 'NONE', #14336, #5508, #22563 ) ;
#51366=DIRECTION ( 'NONE',  ( 0.000000000000000000, -1.000000000000000000, 0.000000000000000000 ) ) ;
#51368=ADVANCED_FACE ( 'NONE', ( #28382 ), #32651, .F. ) ;
#51369=PLANE ( 'NONE',  #36824 ) ;
#51370=EDGE_CURVE ( 'NONE', #33398, #8596, #27270, .T. ) ;
#51371=CARTESIAN_POINT ( 'NONE',  ( -11.30636317915456779, -0.1191753592594197858, 11.32220194836580340 ) ) ;
#51372=ORIENTED_EDGE ( 'NONE', *, *, #31045, .F. ) ;
#51373=VECTOR ( 'NONE', #5161, 1000.000000000000227 ) ;
#51374=AXIS2_PLACEMENT_3D ( 'NONE', #31395, #23680, #6124 ) ;
#51375=DIRECTION ( 'NONE',  ( 0.007781995580012663651, 0.000000000000000000, -0.9999697198139515519 ) ) ;
#51376=DIRECTION ( 'NONE',  ( -0.6427681459581293666, -0.7660444431189770143, -0.005002170337467561935 ) ) ;
#51377=ORIENTED_EDGE ( 'NONE', *, *, #48987, .T. ) ;
#51379=PLANE ( 'NONE',  #25609 ) ;
#51380=EDGE_CURVE ( 'NONE', #31427, #10254, #35813, .T. ) ;
#51381=ORIENTED_EDGE ( 'NONE', *, *, #17247, .F. ) ;
#51382=EDGE_CURVE ( 'NONE', #15410, #43254, #5693, .T. ) ;
#51383=ADVANCED_FACE ( 'NONE', ( #36353 ), #49422, .F. ) ;
#51384=VECTOR ( 'NONE', #47982, 1000.000000000000227 ) ;
#51385=ORIENTED_EDGE ( 'NONE', *, *, #49549, .F. ) ;
#51386=ORIENTED_EDGE ( 'NONE', *, *, #4608, .T. ) ;
#51387=EDGE_LOOP ( 'NONE', ( #47972, #9556, #44462, #52014 ) ) ;
#51388=DIRECTION ( 'NONE',  ( 0.9999697198139515519, 0.000000000000000000, 0.007781995580013368816 ) ) ;
#51389=CARTESIAN_POINT ( 'NONE',  ( -19.52961462879997967, -2.784623065533159636, 4.378442612619098284 ) ) ;
#51390=AXIS2_PLACEMENT_3D ( 'NONE', #17970, #31597, #44620 ) ;
#51391=FACE_OUTER_BOUND ( 'NONE', #38031, .T. ) ;
#51392=EDGE_CURVE ( 'NONE', #23998, #33602, #14779, .T. ) ;
#51393=AXIS2_PLACEMENT_3D ( 'NONE', #15515, #1892, #40565 ) ;
#51394=VERTEX_POINT ( 'NONE', #10541 ) ;
#51395=VERTEX_POINT ( 'NONE', #28114 ) ;
#51396=ADVANCED_FACE ( 'NONE', ( #6533 ), #24982, .F. ) ;
#51397=VECTOR ( 'NONE', #20689, 999.9999999999998863 ) ;
#51398=DIRECTION ( 'NONE',  ( 0.005961354470445682716, -0.6427876096865404731, -0.7660212471507180654 ) ) ;
#51399=DIRECTION ( 'NONE',  ( 0.6427681459581294776, -0.7660444431189769032, 0.005002170337467562802 ) ) ;
#51400=VERTEX_POINT ( 'NONE', #7357 ) ;
#51401=DIRECTION ( 'NONE',  ( 0.9999697198139515519, 0.000000000000000000, 0.007781995580013368816 ) ) ;
#51402=CARTESIAN_POINT ( 'NONE',  ( -19.90235142260334911, -4.889348428825664783, 4.456074482991054353 ) ) ;
#51403=ORIENTED_EDGE ( 'NONE', *, *, #53587, .T. ) ;
#51404=DIRECTION ( 'NONE',  ( -0.2426528472758541499, 0.7422098413412800966, -0.6246952433987894571 ) ) ;
#51405=ORIENTED_EDGE ( 'NONE', *, *, #52743, .F. ) ;
#51406=AXIS2_PLACEMENT_3D ( 'NONE', #48230, #26969, #19256 ) ;
#51407=CARTESIAN_POINT ( 'NONE',  ( -17.83749246818616996, -1.327505506330657781, 3.767654579712751861 ) ) ;
#51408=VECTOR ( 'NONE', #14175, 999.9999999999998863 ) ;
#51409=DIRECTION ( 'NONE',  ( -0.5449076811759708816, 0.6444004775717707689, 0.5364919789714475140 ) ) ;
#51410=AXIS2_PLACEMENT_3D ( 'NONE', #37817, #42352, #37513 ) ;
#51411=ORIENTED_EDGE ( 'NONE', *, *, #1036, .F. ) ;
#51412=FACE_OUTER_BOUND ( 'NONE', #26712, .T. ) ;
#51413=CARTESIAN_POINT ( 'NONE',  ( -9.808144436391993182, 0.000000000000000000, 10.77986332834118777 ) ) ;
#51414=CARTESIAN_POINT ( 'NONE',  ( -15.15892537552479702, -0.3560938001956562293, 3.154583738431461892 ) ) ;
#51415=DIRECTION ( 'NONE',  ( 0.5364919789714477361, 0.6444004775717706579, 0.5449076811759711036 ) ) ;
#51416=VERTEX_POINT ( 'NONE', #33232 ) ;
#51417=LINE ( 'NONE', #17599, #181 ) ;
#51418=LINE ( 'NONE', #21850, #25126 ) ;
#51419=CARTESIAN_POINT ( 'NONE',  ( -18.62175513582871034, 4.172053068839010059, 10.96169306452648229 ) ) ;
#51420=EDGE_CURVE ( 'NONE', #7759, #13509, #20432, .T. ) ;
#51421=DIRECTION ( 'NONE',  ( 0.6427681459581294776, -0.7660444431189769032, 0.005002170337467562802 ) ) ;
#51422=DIRECTION ( 'NONE',  ( 0.007781995580012662783, 0.000000000000000000, -0.9999697198139514409 ) ) ;
#51423=PLANE ( 'NONE',  #43378 ) ;
#51424=VECTOR ( 'NONE', #53150, 999.9999999999998863 ) ;
#51425=LINE ( 'NONE', #17061, #44007 ) ;
#51426=ORIENTED_EDGE ( 'NONE', *, *, #8457, .T. ) ;
#51428=ORIENTED_EDGE ( 'NONE', *, *, #27649, .T. ) ;
#51429=CARTESIAN_POINT ( 'NONE',  ( -11.20636620717317378, 0.000000000000000000, 11.32298014792380414 ) ) ;
#51430=CARTESIAN_POINT ( 'NONE',  ( -21.04681073720913886, 1.581621852479007106, 4.806765756730587036 ) ) ;
#51431=ADVANCED_FACE ( 'NONE', ( #42304 ), #11353, .F. ) ;
#51432=VECTOR ( 'NONE', #22250, 1000.000000000000227 ) ;
#51433=LINE ( 'NONE', #8251, #28566 ) ;
#51434=CARTESIAN_POINT ( 'NONE',  ( -18.67697421479882181, -0.1191753592594197858, 4.036397482078229793 ) ) ;
#51435=EDGE_CURVE ( 'NONE', #31757, #2279, #12493, .T. ) ;
#51436=DIRECTION ( 'NONE',  ( 0.007781995580012663651, -3.146120232559066537E-19, -0.9999697198139514409 ) ) ;
#51438=AXIS2_PLACEMENT_3D ( 'NONE', #33887, #2387, #50649 ) ;
#51439=VERTEX_POINT ( 'NONE', #29530 ) ;
#51440=PLANE ( 'NONE',  #30477 ) ;
#51441=PLANE ( 'NONE',  #26817 ) ;
#51442=VERTEX_POINT ( 'NONE', #15592 ) ;
#51443=LINE ( 'NONE', #29859, #5749 ) ;
#51444=VECTOR ( 'NONE', #32210, 1000.000000000000227 ) ;
#51445=ORIENTED_EDGE ( 'NONE', *, *, #38865, .F. ) ;
#51446=EDGE_CURVE ( 'NONE', #37283, #33305, #41713, .T. ) ;
#51447=DIRECTION ( 'NONE',  ( -0.005961354470445682716, -0.6427876096865404731, 0.7660212471507180654 ) ) ;
#51448=EDGE_LOOP ( 'NONE', ( #8747, #43361, #47835, #43977, #2612 ) ) ;
#51449=LINE ( 'NONE', #46600, #53769 ) ;
#51450=EDGE_CURVE ( 'NONE', #1435, #18921, #3100, .T. ) ;
#51451=ORIENTED_EDGE ( 'NONE', *, *, #22422, .T. ) ;
#51452=ORIENTED_EDGE ( 'NONE', *, *, #49905, .T. ) ;
#51455=FACE_OUTER_BOUND ( 'NONE', #36753, .T. ) ;
#51456=LINE ( 'NONE', #28754, #5129 ) ;
#51457=DIRECTION ( 'NONE',  ( 0.6427681459581294776, -0.7660444431189769032, 0.005002170337467562802 ) ) ;
#51458=EDGE_CURVE ( 'NONE', #28952, #9163, #11892, .T. ) ;
#51459=CARTESIAN_POINT ( 'NONE',  ( -17.93139508144814442, 0.000000000000000000, 13.85596890686001537 ) ) ;
#51460=ORIENTED_EDGE ( 'NONE', *, *, #50254, .F. ) ;
#51461=ORIENTED_EDGE ( 'NONE', *, *, #28877, .F. ) ;
#51463=EDGE_LOOP ( 'NONE', ( #13358, #24240, #1000, #10940 ) ) ;
#51464=DIRECTION ( 'NONE',  ( 0.9999697198139515519, 0.000000000000000000, 0.007781995580013368816 ) ) ;
#51465=CARTESIAN_POINT ( 'NONE',  ( -9.381698774953246556, -0.1191753592594195360, 2.840796620997148914 ) ) ;
#51466=ORIENTED_EDGE ( 'NONE', *, *, #17206, .F. ) ;
#51467=CARTESIAN_POINT ( 'NONE',  ( -17.42984833845037684, 0.000000000000000000, 9.116748853201215752 ) ) ;
#51468=VERTEX_POINT ( 'NONE', #33497 ) ;
#51469=FACE_OUTER_BOUND ( 'NONE', #17636, .T. ) ;
#51470=LINE ( 'NONE', #55157, #55754 ) ;
#51471=ORIENTED_EDGE ( 'NONE', *, *, #681, .T. ) ;
#51472=LINE ( 'NONE', #25606, #36768 ) ;
#51473=VERTEX_POINT ( 'NONE', #7954 ) ;
#51474=AXIS2_PLACEMENT_3D ( 'NONE', #5830, #23155, #32236 ) ;
#51475=CARTESIAN_POINT ( 'NONE',  ( -15.50102849149811135, -0.1191753592594197858, 12.95155240711365430 ) ) ;
#51476=CARTESIAN_POINT ( 'NONE',  ( -15.91947455447202664, -0.1191753592594193972, 7.012513540498049203 ) ) ;
#51477=ORIENTED_EDGE ( 'NONE', *, *, #6621, .F. ) ;
#51478=DIRECTION ( 'NONE',  ( 0.5364919789714477361, 0.6444004775717706579, 0.5449076811759711036 ) ) ;
#51479=DIRECTION ( 'NONE',  ( -0.6427681459581293666, -0.7660444431189770143, -0.005002170337467561935 ) ) ;
#51480=DIRECTION ( 'NONE',  ( 0.5449076811759707706, 0.6444004775717708799, -0.5364919789714476250 ) ) ;
#51481=CARTESIAN_POINT ( 'NONE',  ( -15.03495456790438389, -0.1191753592594197858, 12.77051346725278158 ) ) ;
#51482=ORIENTED_EDGE ( 'NONE', *, *, #32362, .T. ) ;
#51483=EDGE_CURVE ( 'NONE', #40757, #4596, #28686, .T. ) ;
#51484=VECTOR ( 'NONE', #29568, 1000.000000000000000 ) ;
#51485=CARTESIAN_POINT ( 'NONE',  ( 2.072287782118878319, 0.000000000000000000, -2.950529333540147015 ) ) ;
#51486=DIRECTION ( 'NONE',  ( 0.9999697198139515519, 0.000000000000000000, 0.007781995580013368816 ) ) ;
#51487=ADVANCED_FACE ( 'NONE', ( #24677 ), #19868, .F. ) ;
#51488=DIRECTION ( 'NONE',  ( 0.7660212471507180654, -0.6427876096865404731, 0.005961354470445141482 ) ) ;
#51489=CARTESIAN_POINT ( 'NONE',  ( -27.06552663992790997, 0.000000000000000000, 7.195101427592543786 ) ) ;
#51490=CARTESIAN_POINT ( 'NONE',  ( -18.19747506107908563, 0.000000000000000000, 14.03856424583689311 ) ) ;
#51492=CARTESIAN_POINT ( 'NONE',  ( -7.020097852742797073, 1.644072297827783524, 8.920596959107028212 ) ) ;
#51493=ORIENTED_EDGE ( 'NONE', *, *, #43113, .T. ) ;
#51494=LINE ( 'NONE', #12589, #52485 ) ;
#51495=ADVANCED_FACE ( 'NONE', ( #2802 ), #15892, .F. ) ;
#51497=FACE_OUTER_BOUND ( 'NONE', #5104, .T. ) ;
#51498=EDGE_LOOP ( 'NONE', ( #52085, #39920, #38591 ) ) ;
#51499=CARTESIAN_POINT ( 'NONE',  ( -31.72782227498118601, 0.000000000000000000, 9.205484770164058972 ) ) ;
#51500=ORIENTED_EDGE ( 'NONE', *, *, #37786, .F. ) ;
#51501=ADVANCED_FACE ( 'NONE', ( #43966 ), #4788, .F. ) ;
#51502=EDGE_CURVE ( 'NONE', #29764, #34537, #9054, .T. ) ;
#51503=EDGE_CURVE ( 'NONE', #36269, #13086, #55929, .T. ) ;
#51504=PLANE ( 'NONE',  #37088 ) ;
#51505=PLANE ( 'NONE',  #49389 ) ;
#51506=CARTESIAN_POINT ( 'NONE',  ( -31.72626587586518099, 0.000000000000000000, 9.005490826201270949 ) ) ;
#51508=EDGE_LOOP ( 'NONE', ( #30906, #35900, #17410, #38816 ) ) ;
#51509=ORIENTED_EDGE ( 'NONE', *, *, #45761, .T. ) ;
#51511=PLANE ( 'NONE',  #27764 ) ;
#51512=CARTESIAN_POINT ( 'NONE',  ( -20.26176469941677993, 0.000000000000000000, 14.76116360616437895 ) ) ;
#51514=DIRECTION ( 'NONE',  ( 0.000000000000000000, -0.000000000000000000, -1.000000000000000000 ) ) ;
#51515=EDGE_CURVE ( 'NONE', #27953, #49693, #51650, .T. ) ;
#51516=CARTESIAN_POINT ( 'NONE',  ( -15.06642710517098571, 0.000000000000000000, 3.964492566432560761 ) ) ;
#51517=ORIENTED_EDGE ( 'NONE', *, *, #25697, .F. ) ;
#51518=LINE ( 'NONE', #25125, #53726 ) ;
#51519=EDGE_CURVE ( 'NONE', #35036, #48042, #13038, .T. ) ;
#51520=LINE ( 'NONE', #13712, #24228 ) ;
#51521=VERTEX_POINT ( 'NONE', #22110 ) ;
#51522=EDGE_CURVE ( 'NONE', #10313, #3654, #35446, .T. ) ;
#51523=CARTESIAN_POINT ( 'NONE',  ( -19.60912206198628027, -0.1191753592594197858, 4.398475361799976113 ) ) ;
#51524=DIRECTION ( 'NONE',  ( 0.007781995580012662783, 0.000000000000000000, -0.9999697198139514409 ) ) ;
#51525=DIRECTION ( 'NONE',  ( 0.005002170337468016433, -0.7660444431189770143, -0.6427681459581293666 ) ) ;
#51526=VERTEX_POINT ( 'NONE', #25823 ) ;
#51527=EDGE_CURVE ( 'NONE', #49950, #13999, #39441, .T. ) ;
#51528=AXIS2_PLACEMENT_3D ( 'NONE', #32072, #45142, #7544 ) ;
#51529=LINE ( 'NONE', #34218, #22150 ) ;
#51530=ORIENTED_EDGE ( 'NONE', *, *, #8122, .F. ) ;
#51531=ORIENTED_EDGE ( 'NONE', *, *, #23920, .F. ) ;
#51532=ORIENTED_EDGE ( 'NONE', *, *, #1948, .T. ) ;
#51534=CARTESIAN_POINT ( 'NONE',  ( 2.072287782118878319, 0.000000000000000000, -2.950529333540147015 ) ) ;
#51535=EDGE_LOOP ( 'NONE', ( #30230, #45169, #5511, #18323 ) ) ;
#51536=DIRECTION ( 'NONE',  ( 0.005002170337468016433, -0.7660444431189770143, -0.6427681459581293666 ) ) ;
#51537=VERTEX_POINT ( 'NONE', #43419 ) ;
#51538=CARTESIAN_POINT ( 'NONE',  ( -17.93139508144814442, 0.000000000000000000, 13.85596890686001537 ) ) ;
#51539=EDGE_LOOP ( 'NONE', ( #18723, #17351, #50991, #47294 ) ) ;
#51540=CARTESIAN_POINT ( 'NONE',  ( -13.96170819468429336, 0.000000000000000000, 7.127752359109486235 ) ) ;
#51541=VERTEX_POINT ( 'NONE', #48513 ) ;
#51542=DIRECTION ( 'NONE',  ( -0.005961354470445682716, -0.6427876096865404731, 0.7660212471507180654 ) ) ;
#51543=CARTESIAN_POINT ( 'NONE',  ( -16.63288945721647494, -1.003701604285657911, 3.310076901536455729 ) ) ;
#51544=FACE_OUTER_BOUND ( 'NONE', #11999, .T. ) ;
#51545=DIRECTION ( 'NONE',  ( 0.007781995580012662783, 0.000000000000000000, -0.9999697198139514409 ) ) ;
#51546=CARTESIAN_POINT ( 'NONE',  ( 2.072287782118878319, 0.000000000000000000, -2.950529333540147015 ) ) ;
#51547=ORIENTED_EDGE ( 'NONE', *, *, #37977, .F. ) ;
#51548=EDGE_LOOP ( 'NONE', ( #46456, #22106, #15776, #19368 ) ) ;
#51549=CARTESIAN_POINT ( 'NONE',  ( -21.60330836122860276, -4.079838673713159558, 11.76910067310686081 ) ) ;
#51550=CARTESIAN_POINT ( 'NONE',  ( -8.372583192005976116, 0.000000000000000000, 5.438704338890580026 ) ) ;
#51551=DIRECTION ( 'NONE',  ( -0.9999697198139514409, -0.000000000000000000, -0.007781995580013368816 ) ) ;
#51552=DIRECTION ( 'NONE',  ( -0.005002170337468016433, -0.7660444431189770143, 0.6427681459581293666 ) ) ;
#51553=DIRECTION ( 'NONE',  ( -0.5364919789714478471, 0.6444004775717705469, -0.5449076811759709926 ) ) ;
#51554=DIRECTION ( 'NONE',  ( 0.005002170337468016433, -0.7660444431189770143, -0.6427681459581293666 ) ) ;
#51555=ORIENTED_EDGE ( 'NONE', *, *, #51450, .T. ) ;
#51556=PLANE ( 'NONE',  #42915 ) ;
#51557=CARTESIAN_POINT ( 'NONE',  ( -17.83139810946674686, -0.1191753592594197858, 13.85674710641801788 ) ) ;
#51558=ORIENTED_EDGE ( 'NONE', *, *, #31772, .F. ) ;
#51559=ADVANCED_FACE ( 'NONE', ( #35197 ), #48209, .F. ) ;
#51560=EDGE_CURVE ( 'NONE', #16382, #4739, #38888, .T. ) ;
#51561=VECTOR ( 'NONE', #39564, 1000.000000000000227 ) ;
#51562=DIRECTION ( 'NONE',  ( -0.6427681459581293666, -0.7660444431189770143, -0.005002170337467561935 ) ) ;
#51563=CARTESIAN_POINT ( 'NONE',  ( -12.54612273050805271, 0.000000000000000000, 4.353438227646377001 ) ) ;
#51564=CARTESIAN_POINT ( 'NONE',  ( -22.40478740399063895, 0.000000000000000000, 5.384712028983816623 ) ) ;
#51565=ADVANCED_FACE ( 'NONE', ( #4517 ), #17029, .F. ) ;
#51566=CARTESIAN_POINT ( 'NONE',  ( -7.296103114018933411, -3.208161209119383628, 8.210037920513791221 ) ) ;
#51567=ORIENTED_EDGE ( 'NONE', *, *, #54532, .T. ) ;
#51568=EDGE_LOOP ( 'NONE', ( #53548, #54417, #40888, #43603 ) ) ;
#51569=DIRECTION ( 'NONE',  ( 0.9999697198139515519, 0.000000000000000000, 0.007781995580013368816 ) ) ;
#51571=LINE ( 'NONE', #35114, #28774 ) ;
#51572=LINE ( 'NONE', #26282, #45495 ) ;
#51573=CARTESIAN_POINT ( 'NONE',  ( -12.53750056999220597, 0.000000000000000000, 3.245509117873082605 ) ) ;
#51574=DIRECTION ( 'NONE',  ( 0.9321478471874540261, 0.000000000000000000, -0.3620778797217457101 ) ) ;
#51575=CARTESIAN_POINT ( 'NONE',  ( 2.072287782118878319, 0.000000000000000000, -2.950529333540147015 ) ) ;
#51576=ORIENTED_EDGE ( 'NONE', *, *, #43595, .T. ) ;
#51577=EDGE_CURVE ( 'NONE', #28691, #25884, #56195, .T. ) ;
#51578=DIRECTION ( 'NONE',  ( -0.7660212471507179544, -0.6427876096865405842, -0.005961354470445141482 ) ) ;
#51579=CARTESIAN_POINT ( 'NONE',  ( -16.36043429343423483, -0.6798977022406571535, 3.214577103081905474 ) ) ;
#51580=ADVANCED_FACE ( 'NONE', ( #22417 ), #39730, .F. ) ;
#51581=PLANE ( 'NONE',  #11132 ) ;
#51582=ORIENTED_EDGE ( 'NONE', *, *, #43840, .T. ) ;
#51583=DIRECTION ( 'NONE',  ( 0.007781995580012663651, 0.000000000000000000, -0.9999697198139515519 ) ) ;
#51584=ORIENTED_EDGE ( 'NONE', *, *, #27869, .T. ) ;
#51585=ADVANCED_FACE ( 'NONE', ( #13861 ), #34346, .F. ) ;
#51586=ORIENTED_EDGE ( 'NONE', *, *, #15880, .T. ) ;
#51587=EDGE_CURVE ( 'NONE', #53425, #26718, #9632, .T. ) ;
#51588=ORIENTED_EDGE ( 'NONE', *, *, #36471, .F. ) ;
#51589=ORIENTED_EDGE ( 'NONE', *, *, #16450, .F. ) ;
#51590=ORIENTED_EDGE ( 'NONE', *, *, #33491, .F. ) ;
#51591=VERTEX_POINT ( 'NONE', #21269 ) ;
#51592=DIRECTION ( 'NONE',  ( 0.007781995580012663651, -3.146120232559066537E-19, -0.9999697198139514409 ) ) ;
#51593=CARTESIAN_POINT ( 'NONE',  ( -11.83408720182036511, 0.000000000000000000, 6.574971871612978802 ) ) ;
#51594=CARTESIAN_POINT ( 'NONE',  ( -8.581250235374994872, 0.000000000000000000, 6.551622587568105338 ) ) ;
#51595=EDGE_LOOP ( 'NONE', ( #41859, #18207, #48296, #9255 ) ) ;
#51596=DIRECTION ( 'NONE',  ( 0.8531650599175529814, -0.4028455766673920135, -0.3313982828793697877 ) ) ;
#51597=VERTEX_POINT ( 'NONE', #38601 ) ;
#51598=CARTESIAN_POINT ( 'NONE',  ( -27.06708303904391144, 0.000000000000000000, 7.395095371555332697 ) ) ;
#51599=ORIENTED_EDGE ( 'NONE', *, *, #17056, .T. ) ;
#51601=LINE ( 'NONE', #12699, #11062 ) ;
#51603=ORIENTED_EDGE ( 'NONE', *, *, #52568, .T. ) ;
#51604=CARTESIAN_POINT ( 'NONE',  ( -12.83169202443629509, 0.000000000000000000, 1.765891372722660169 ) ) ;
#51605=ORIENTED_EDGE ( 'NONE', *, *, #54254, .F. ) ;
#51606=FACE_OUTER_BOUND ( 'NONE', #33428, .T. ) ;
#51607=DIRECTION ( 'NONE',  ( 0.007781995580012662783, 0.000000000000000000, -0.9999697198139514409 ) ) ;
#51609=DIRECTION ( 'NONE',  ( 0.000000000000000000, -1.000000000000000000, 0.000000000000000000 ) ) ;
#51610=CARTESIAN_POINT ( 'NONE',  ( -17.93139508144814442, 0.000000000000000000, 13.85596890686001537 ) ) ;
#51611=DIRECTION ( 'NONE',  ( 0.007781995580012663651, 0.000000000000000000, -0.9999697198139515519 ) ) ;
#51612=DIRECTION ( 'NONE',  ( 0.005002170337468016433, -0.7660444431189770143, -0.6427681459581293666 ) ) ;
#51613=DIRECTION ( 'NONE',  ( 0.000000000000000000, -0.000000000000000000, -1.000000000000000000 ) ) ;
#51614=EDGE_LOOP ( 'NONE', ( #51724, #27343, #19307, #29414 ) ) ;
#51615=CARTESIAN_POINT ( 'NONE',  ( -11.15089438559551205, 0.000000000000000000, 4.194970203655428165 ) ) ;
#51616=ORIENTED_EDGE ( 'NONE', *, *, #52141, .F. ) ;
#51618=CARTESIAN_POINT ( 'NONE',  ( -20.54126990917373519, -0.1191753592594197858, 4.760553241521720658 ) ) ;
#51619=FACE_OUTER_BOUND ( 'NONE', #12489, .T. ) ;
#51620=CARTESIAN_POINT ( 'NONE',  ( -8.168214455200342172, -0.1191753592594182315, 5.964839429474373844 ) ) ;
#51621=CARTESIAN_POINT ( 'NONE',  ( -25.20278734466900517, 0.000000000000000000, 6.670939612111840944 ) ) ;
#51622=CARTESIAN_POINT ( 'NONE',  ( -9.289472744725888020, 0.000000000000000000, 3.840124147469701654 ) ) ;
#51623=EDGE_CURVE ( 'NONE', #12635, #49710, #36871, .T. ) ;
#51624=EDGE_CURVE ( 'NONE', #41029, #17901, #32332, .T. ) ;
#51627=ORIENTED_EDGE ( 'NONE', *, *, #44705, .F. ) ;
#51628=DIRECTION ( 'NONE',  ( -0.7660212471507179544, -0.6427876096865405842, -0.005961354470445141482 ) ) ;
#51629=FACE_OUTER_BOUND ( 'NONE', #17038, .T. ) ;
#51630=PLANE ( 'NONE',  #43622 ) ;
#51631=DIRECTION ( 'NONE',  ( -0.7660212471507179544, -0.6427876096865405842, -0.005961354470445141482 ) ) ;
#51632=CARTESIAN_POINT ( 'NONE',  ( -8.609916609573598834, 0.000000000000000000, 10.23519010964256637 ) ) ;
#51633=CARTESIAN_POINT ( 'NONE',  ( -15.80301146101693455, 0.000000000000000000, 4.897430492490863152 ) ) ;
#51634=CARTESIAN_POINT ( 'NONE',  ( 3.520599301005862269, -1.000000000000000000, 0.7780620552096689790 ) ) ;
#51635=ORIENTED_EDGE ( 'NONE', *, *, #39320, .T. ) ;
#51636=CARTESIAN_POINT ( 'NONE',  ( -17.75702712210175349, -0.1134144341941959455, 3.679058789739912072 ) ) ;
#51637=FACE_OUTER_BOUND ( 'NONE', #9789, .T. ) ;
#51638=ORIENTED_EDGE ( 'NONE', *, *, #376, .T. ) ;
#51639=ORIENTED_EDGE ( 'NONE', *, *, #46328, .F. ) ;
#51640=PLANE ( 'NONE',  #50085 ) ;
#51642=EDGE_CURVE ( 'NONE', #47757, #41032, #19527, .T. ) ;
#51643=EDGE_LOOP ( 'NONE', ( #9800, #52776, #27608, #41962 ) ) ;
#51644=ORIENTED_EDGE ( 'NONE', *, *, #54314, .F. ) ;
#51645=ORIENTED_EDGE ( 'NONE', *, *, #33878, .T. ) ;
#51646=ADVANCED_FACE ( 'NONE', ( #32031 ), #35740, .F. ) ;
#51648=DIRECTION ( 'NONE',  ( 0.005961354470445682716, -0.6427876096865404731, -0.7660212471507180654 ) ) ;
#51649=ORIENTED_EDGE ( 'NONE', *, *, #45937, .T. ) ;
#51650=LINE ( 'NONE', #26111, #44155 ) ;
#51652=ORIENTED_EDGE ( 'NONE', *, *, #32818, .F. ) ;
#51653=EDGE_CURVE ( 'NONE', #44974, #54122, #19233, .T. ) ;
#51654=ORIENTED_EDGE ( 'NONE', *, *, #24138, .F. ) ;
#51655=LINE ( 'NONE', #39736, #53757 ) ;
#51656=VERTEX_POINT ( 'NONE', #27209 ) ;
#51657=CARTESIAN_POINT ( 'NONE',  ( -27.99923088623136636, 0.000000000000000000, 7.757173251277078130 ) ) ;
#51658=LINE ( 'NONE', #33773, #49454 ) ;
#51659=ORIENTED_EDGE ( 'NONE', *, *, #16189, .F. ) ;
#51660=CARTESIAN_POINT ( 'NONE',  ( -18.89555915323239077, 4.010151117816511679, 3.893663786391856618 ) ) ;
#51661=ORIENTED_EDGE ( 'NONE', *, *, #17886, .T. ) ;
#51662=LINE ( 'NONE', #30088, #54529 ) ;
#51663=ADVANCED_FACE ( 'NONE', ( #36291 ), #23771, .F. ) ;
#51665=ORIENTED_EDGE ( 'NONE', *, *, #35117, .T. ) ;
#51666=FACE_OUTER_BOUND ( 'NONE', #46927, .T. ) ;
#51667=LINE ( 'NONE', #4534, #31097 ) ;
#51669=LINE ( 'NONE', #13359, #44654 ) ;
#51670=EDGE_CURVE ( 'NONE', #25200, #866, #6210, .T. ) ;
#51671=ORIENTED_EDGE ( 'NONE', *, *, #39050, .T. ) ;
#51672=EDGE_CURVE ( 'NONE', #31703, #25139, #10466, .T. ) ;
#51673=LINE ( 'NONE', #56215, #51874 ) ;
#51674=DIRECTION ( 'NONE',  ( 0.7660212471507180654, -0.6427876096865404731, 0.005961354470445141482 ) ) ;
#51675=DIRECTION ( 'NONE',  ( -0.5449076811759708816, 0.6444004775717707689, 0.5364919789714475140 ) ) ;
#51676=CARTESIAN_POINT ( 'NONE',  ( -14.30946433947862495, -4.889348428825665671, 2.283607204660580869 ) ) ;
#51677=PLANE ( 'NONE',  #15954 ) ;
#51678=CARTESIAN_POINT ( 'NONE',  ( -17.22278863308774532, 0.000000000000000000, 8.210370086506713960 ) ) ;
#51679=EDGE_CURVE ( 'NONE', #54483, #41210, #2191, .T. ) ;
#51680=CARTESIAN_POINT ( 'NONE',  ( -10.47421230394850866, 0.000000000000000000, 10.95934586908605723 ) ) ;
#51681=CARTESIAN_POINT ( 'NONE',  ( -24.26908309836554878, 0.000000000000000000, 6.108867788427308376 ) ) ;
#51682=LINE ( 'NONE', #21860, #6845 ) ;
#51683=ORIENTED_EDGE ( 'NONE', *, *, #2244, .F. ) ;
#51684=CARTESIAN_POINT ( 'NONE',  ( -0.8459003381547196554, -5.709362246987525147, 3.546949993899496167 ) ) ;
#51685=ORIENTED_EDGE ( 'NONE', *, *, #43834, .F. ) ;
#51686=DIRECTION ( 'NONE',  ( 0.007781995580012663651, -3.146120232559066537E-19, -0.9999697198139514409 ) ) ;
#51687=LINE ( 'NONE', #33277, #42647 ) ;
#51688=CARTESIAN_POINT ( 'NONE',  ( -23.33771345073609638, -0.1191753592594197858, 5.846786880686956955 ) ) ;
#51689=CARTESIAN_POINT ( 'NONE',  ( -18.22153117760466401, 2.067327705546506245, 7.352019596133413160 ) ) ;
#51690=CARTESIAN_POINT ( 'NONE',  ( -17.46532115785441519, 0.000000000000000000, 13.67492996699914265 ) ) ;
#51691=EDGE_CURVE ( 'NONE', #39994, #18681, #14442, .T. ) ;
#51692=ORIENTED_EDGE ( 'NONE', *, *, #25017, .T. ) ;
#51693=AXIS2_PLACEMENT_3D ( 'NONE', #41124, #19547, #19825 ) ;
#51694=VERTEX_POINT ( 'NONE', #10993 ) ;
#51695=DIRECTION ( 'NONE',  ( -0.005961354470445682716, -0.6427876096865404731, 0.7660212471507180654 ) ) ;
#51696=PLANE ( 'NONE',  #45862 ) ;
#51697=VERTEX_POINT ( 'NONE', #32589 ) ;
#51699=ORIENTED_EDGE ( 'NONE', *, *, #7502, .T. ) ;
#51700=DIRECTION ( 'NONE',  ( -0.6427681459581293666, -0.7660444431189770143, -0.005002170337467561935 ) ) ;
#51701=EDGE_LOOP ( 'NONE', ( #49714, #15916, #8317, #105 ) ) ;
#51702=CARTESIAN_POINT ( 'NONE',  ( -16.79925329029790149, 0.000000000000000000, 13.49544742625427496 ) ) ;
#51703=VERTEX_POINT ( 'NONE', #44263 ) ;
#51704=ORIENTED_EDGE ( 'NONE', *, *, #33697, .F. ) ;
#51705=ORIENTED_EDGE ( 'NONE', *, *, #8239, .T. ) ;
#51706=LINE ( 'NONE', #30435, #32949 ) ;
#51707=FACE_OUTER_BOUND ( 'NONE', #30635, .T. ) ;
#51708=LINE ( 'NONE', #12816, #33920 ) ;
#51709=LINE ( 'NONE', #55406, #49347 ) ;
#51710=VERTEX_POINT ( 'NONE', #5366 ) ;
#51711=ADVANCED_FACE ( 'NONE', ( #22671 ), #18400, .F. ) ;
#51712=VERTEX_POINT ( 'NONE', #39981 ) ;
#51713=ORIENTED_EDGE ( 'NONE', *, *, #30691, .T. ) ;
#51714=ADVANCED_FACE ( 'NONE', ( #18709 ), #1365, .F. ) ;
#51715=DIRECTION ( 'NONE',  ( 0.000000000000000000, -1.000000000000000000, 0.000000000000000000 ) ) ;
#51716=ORIENTED_EDGE ( 'NONE', *, *, #26995, .F. ) ;
#51717=FACE_OUTER_BOUND ( 'NONE', #26225, .T. ) ;
#51719=CARTESIAN_POINT ( 'NONE',  ( -22.40634380310664397, 0.000000000000000000, 5.584705972946605534 ) ) ;
#51720=DIRECTION ( 'NONE',  ( -0.005002170337468016433, -0.7660444431189770143, 0.6427681459581293666 ) ) ;
#51723=LINE ( 'NONE', #13122, #29510 ) ;
#51724=ORIENTED_EDGE ( 'NONE', *, *, #15337, .F. ) ;
#51725=EDGE_CURVE ( 'NONE', #28729, #43960, #14707, .T. ) ;
#51726=EDGE_CURVE ( 'NONE', #18328, #44507, #40829, .T. ) ;
#51727=VECTOR ( 'NONE', #55972, 999.9999999999998863 ) ;
#51728=LINE ( 'NONE', #33, #46406 ) ;
#51730=ORIENTED_EDGE ( 'NONE', *, *, #42005, .T. ) ;
#51731=DIRECTION ( 'NONE',  ( 0.9321478471874540261, 0.000000000000000000, -0.3620778797217456546 ) ) ;
#51732=CARTESIAN_POINT ( 'NONE',  ( -15.55118237654904867, 0.000000000000000000, 6.546044577468901338 ) ) ;
#51733=PLANE ( 'NONE',  #2844 ) ;
#51734=ADVANCED_FACE ( 'NONE', ( #1902 ), #48804, .F. ) ;
#51735=VERTEX_POINT ( 'NONE', #54708 ) ;
#51736=DIRECTION ( 'NONE',  ( 0.000000000000000000, -0.000000000000000000, -1.000000000000000000 ) ) ;
#51738=DIRECTION ( 'NONE',  ( 0.5449076811759707706, 0.6444004775717708799, -0.5364919789714476250 ) ) ;
#51739=CARTESIAN_POINT ( 'NONE',  ( -16.81345671998191449, 0.000000000000000000, 3.412238694616132495 ) ) ;
#51740=DIRECTION ( 'NONE',  ( -0.6427681459581293666, -0.7660444431189770143, -0.005002170337467561935 ) ) ;
#51741=CARTESIAN_POINT ( 'NONE',  ( -11.40636015113596180, 0.000000000000000000, 11.32142374880780089 ) ) ;
#51742=EDGE_CURVE ( 'NONE', #20189, #35085, #33990, .T. ) ;
#51743=PLANE ( 'NONE',  #53323 ) ;
#51745=VERTEX_POINT ( 'NONE', #46188 ) ;
#51746=FACE_OUTER_BOUND ( 'NONE', #41550, .T. ) ;
#51747=DIRECTION ( 'NONE',  ( -0.005002170337468016433, -0.7660444431189770143, 0.6427681459581293666 ) ) ;
#51748=FACE_OUTER_BOUND ( 'NONE', #17342, .T. ) ;
#51749=ORIENTED_EDGE ( 'NONE', *, *, #21590, .T. ) ;
#51750=LINE ( 'NONE', #12861, #47423 ) ;
#51751=CARTESIAN_POINT ( 'NONE',  ( -12.23851102634202448, -0.1191753592594197858, 11.68427982808754884 ) ) ;
#51752=EDGE_LOOP ( 'NONE', ( #10743, #53157, #31898, #45458 ) ) ;
#51753=ADVANCED_FACE ( 'NONE', ( #19804 ), #3335, .F. ) ;
#51754=DIRECTION ( 'NONE',  ( 0.5449076811759707706, 0.6444004775717708799, -0.5364919789714476250 ) ) ;
#51755=LINE ( 'NONE', #3771, #34888 ) ;
#51756=AXIS2_PLACEMENT_3D ( 'NONE', #6733, #24331, #50155 ) ;
#51757=DIRECTION ( 'NONE',  ( -0.6427681459581293666, -0.7660444431189770143, -0.005002170337467561935 ) ) ;
#51759=EDGE_CURVE ( 'NONE', #12964, #41663, #28892, .T. ) ;
#51760=ORIENTED_EDGE ( 'NONE', *, *, #5992, .F. ) ;
#51761=ORIENTED_EDGE ( 'NONE', *, *, #890, .F. ) ;
#51762=DIRECTION ( 'NONE',  ( -0.9999697198139514409, -0.000000000000000000, -0.007781995580013368816 ) ) ;
#51763=LINE ( 'NONE', #8327, #44935 ) ;
#51764=PLANE ( 'NONE',  #10591 ) ;
#51765=DIRECTION ( 'NONE',  ( 0.000000000000000000, -1.000000000000000000, 0.000000000000000000 ) ) ;
#51766=DIRECTION ( 'NONE',  ( -0.9999697198139514409, -0.000000000000000000, -0.007781995580013368816 ) ) ;
#51767=VECTOR ( 'NONE', #3420, 1000.000000000000114 ) ;
#51768=DIRECTION ( 'NONE',  ( 0.5449076811759707706, 0.6444004775717708799, -0.5364919789714476250 ) ) ;
#51769=ORIENTED_EDGE ( 'NONE', *, *, #54953, .T. ) ;
#51770=FACE_OUTER_BOUND ( 'NONE', #13090, .T. ) ;
#51772=LINE ( 'NONE', #4641, #31497 ) ;
#51773=ORIENTED_EDGE ( 'NONE', *, *, #36396, .T. ) ;
#51774=DIRECTION ( 'NONE',  ( -0.005961354470445682716, -0.6427876096865404731, 0.7660212471507180654 ) ) ;
#51775=DIRECTION ( 'NONE',  ( -0.6246952433987894571, 0.7422098413412802076, 0.2426528472758539834 ) ) ;
#51776=CARTESIAN_POINT ( 'NONE',  ( -14.01545677930355183, 0.000000000000000000, 2.126011111488108174 ) ) ;
#51777=ORIENTED_EDGE ( 'NONE', *, *, #53262, .F. ) ;
#51778=DIRECTION ( 'NONE',  ( 0.5449076811759707706, 0.6444004775717708799, -0.5364919789714476250 ) ) ;
#51779=EDGE_CURVE ( 'NONE', #46331, #14535, #33692, .T. ) ;
#51780=VERTEX_POINT ( 'NONE', #41920 ) ;
#51781=VERTEX_POINT ( 'NONE', #29450 ) ;
#51782=EDGE_LOOP ( 'NONE', ( #6056, #35302, #1652, #24612 ) ) ;
#51783=ORIENTED_EDGE ( 'NONE', *, *, #30731, .F. ) ;
#51784=DIRECTION ( 'NONE',  ( 0.000000000000000000, -0.000000000000000000, -1.000000000000000000 ) ) ;
#51785=ORIENTED_EDGE ( 'NONE', *, *, #26310, .F. ) ;
#51786=ADVANCED_FACE ( 'NONE', ( #25205 ), #38232, .F. ) ;
#51787=CARTESIAN_POINT ( 'NONE',  ( -15.66898763994628574, 2.391131607591508335, 2.692009034675617141 ) ) ;
#51788=EDGE_CURVE ( 'NONE', #45853, #1428, #45934, .T. ) ;
#51789=VECTOR ( 'NONE', #28094, 1000.000000000000227 ) ;
#51790=AXIS2_PLACEMENT_3D ( 'NONE', #32347, #49662, #10757 ) ;
#51791=ORIENTED_EDGE ( 'NONE', *, *, #48987, .F. ) ;
#51792=LINE ( 'NONE', #4401, #16853 ) ;
#51793=EDGE_LOOP ( 'NONE', ( #55781, #39686, #17062, #9401 ) ) ;
#51794=CARTESIAN_POINT ( 'NONE',  ( -12.60458797795435615, 0.000000000000000000, 11.86609696750642229 ) ) ;
#51796=EDGE_CURVE ( 'NONE', #7109, #50616, #16111, .T. ) ;
#51797=DIRECTION ( 'NONE',  ( 0.9999697198139515519, 0.000000000000000000, 0.007781995580013368816 ) ) ;
#51798=CARTESIAN_POINT ( 'NONE',  ( -12.30159815216673458, 0.000000000000000000, 6.940665663102732807 ) ) ;
#51799=PLANE ( 'NONE',  #37651 ) ;
#51800=DIRECTION ( 'NONE',  ( -0.9999697198139514409, -0.000000000000000000, -0.007781995580013368816 ) ) ;
#51801=DIRECTION ( 'NONE',  ( -0.6427681459581293666, -0.7660444431189770143, -0.005002170337467561935 ) ) ;
#51802=ORIENTED_EDGE ( 'NONE', *, *, #18938, .F. ) ;
#51803=ORIENTED_EDGE ( 'NONE', *, *, #23851, .T. ) ;
#51804=EDGE_CURVE ( 'NONE', #37629, #23769, #46457, .T. ) ;
#51805=CARTESIAN_POINT ( 'NONE',  ( -7.222176269732285547, -2.744276736922906856, 8.400358159916756051 ) ) ;
#51806=CARTESIAN_POINT ( 'NONE',  ( -16.38607150127187140, 1.581621852479007106, 2.996376358121860761 ) ) ;
#51807=VECTOR ( 'NONE', #43160, 1000.000000000000227 ) ;
#51808=EDGE_CURVE ( 'NONE', #17431, #27972, #55552, .T. ) ;
#51810=CARTESIAN_POINT ( 'NONE',  ( -13.97164800958942266, 0.000000000000000000, 8.404997228177755630 ) ) ;
#51811=EDGE_CURVE ( 'NONE', #33148, #223, #12115, .T. ) ;
#51812=DIRECTION ( 'NONE',  ( 0.9999697198139515519, 0.000000000000000000, 0.007781995580013368816 ) ) ;
#51813=LINE ( 'NONE', #38483, #47697 ) ;
#51814=ORIENTED_EDGE ( 'NONE', *, *, #55945, .T. ) ;
#51815=CARTESIAN_POINT ( 'NONE',  ( -17.98066455030807376, -5.375054281893166142, 3.694129481368514600 ) ) ;
#51816=DIRECTION ( 'NONE',  ( -0.9999697198139514409, -0.000000000000000000, -0.007781995580013368816 ) ) ;
#51817=VERTEX_POINT ( 'NONE', #20908 ) ;
#51818=EDGE_CURVE ( 'NONE', #31643, #46025, #20655, .T. ) ;
#51819=CARTESIAN_POINT ( 'NONE',  ( -13.64380565324295524, -2.946525016555660237, 6.817398727822249427 ) ) ;
#51822=LINE ( 'NONE', #51566, #20514 ) ;
#51824=ORIENTED_EDGE ( 'NONE', *, *, #3192, .F. ) ;
#51825=DIRECTION ( 'NONE',  ( 0.005961354470445682716, -0.6427876096865404731, -0.7660212471507180654 ) ) ;
#51826=DIRECTION ( 'NONE',  ( -0.5364919789714478471, 0.6444004775717705469, -0.5449076811759709926 ) ) ;
#51827=DIRECTION ( 'NONE',  ( 0.007781995580012663651, -3.146120232559066537E-19, -0.9999697198139514409 ) ) ;
#51828=VECTOR ( 'NONE', #27698, 999.9999999999998863 ) ;
#51829=AXIS2_PLACEMENT_3D ( 'NONE', #42398, #29632, #50885 ) ;
#51830=CARTESIAN_POINT ( 'NONE',  ( -27.99923088623136636, 0.000000000000000000, 7.757173251277078130 ) ) ;
#51831=DIRECTION ( 'NONE',  ( 0.5364919789714477361, 0.6444004775717706579, 0.5449076811759711036 ) ) ;
#51832=DIRECTION ( 'NONE',  ( -0.3620778797217457101, 0.000000000000000000, -0.9321478471874540261 ) ) ;
#51833=CARTESIAN_POINT ( 'NONE',  ( -12.75776174254319173, 3.362543313726510164, 1.530196911152285733 ) ) ;
#51834=ORIENTED_EDGE ( 'NONE', *, *, #37481, .T. ) ;
#51835=DIRECTION ( 'NONE',  ( 0.6427681459581294776, -0.7660444431189769032, 0.005002170337467562802 ) ) ;
#51836=DIRECTION ( 'NONE',  ( 0.007781995580012663651, 0.000000000000000000, -0.9999697198139515519 ) ) ;
#51837=AXIS2_PLACEMENT_3D ( 'NONE', #29737, #42209, #34521 ) ;
#51838=ORIENTED_EDGE ( 'NONE', *, *, #49755, .F. ) ;
#51839=CARTESIAN_POINT ( 'NONE',  ( -18.39746900504187010, 0.000000000000000000, 14.03700784672088808 ) ) ;
#51840=VERTEX_POINT ( 'NONE', #50475 ) ;
#51841=PLANE ( 'NONE',  #49462 ) ;
#51842=EDGE_CURVE ( 'NONE', #30962, #43904, #37971, .T. ) ;
#51843=ORIENTED_EDGE ( 'NONE', *, *, #52886, .T. ) ;
#51844=ADVANCED_FACE ( 'NONE', ( #11575 ), #24603, .F. ) ;
#51845=EDGE_LOOP ( 'NONE', ( #42895, #17387, #56075, #20059 ) ) ;
#51846=VECTOR ( 'NONE', #15681, 999.9999999999998863 ) ;
#51847=ORIENTED_EDGE ( 'NONE', *, *, #49932, .T. ) ;
#51848=VERTEX_POINT ( 'NONE', #3024 ) ;
#51849=ORIENTED_EDGE ( 'NONE', *, *, #46538, .F. ) ;
#51850=EDGE_LOOP ( 'NONE', ( #54073, #47683, #3598, #34672 ) ) ;
#51851=CARTESIAN_POINT ( 'NONE',  ( -16.58663476131414427, 5.143464774974012776, 2.960640501956672832 ) ) ;
#51852=LINE ( 'NONE', #21507, #48313 ) ;
#51853=DIRECTION ( 'NONE',  ( 0.000000000000000000, -1.000000000000000000, 0.000000000000000000 ) ) ;
#51854=EDGE_CURVE ( 'NONE', #53756, #1256, #7043, .T. ) ;
#51855=ADVANCED_FACE ( 'NONE', ( #41648 ), #37126, .F. ) ;
#51856=EDGE_CURVE ( 'NONE', #873, #4449, #40432, .T. ) ;
#51857=ORIENTED_EDGE ( 'NONE', *, *, #10376, .T. ) ;
#51858=DIRECTION ( 'NONE',  ( 0.000000000000000000, -0.000000000000000000, -1.000000000000000000 ) ) ;
#51859=ORIENTED_EDGE ( 'NONE', *, *, #35167, .F. ) ;
#51860=LINE ( 'NONE', #27647, #35885 ) ;
#51861=EDGE_CURVE ( 'NONE', #24462, #14078, #25750, .T. ) ;
#51862=ORIENTED_EDGE ( 'NONE', *, *, #37301, .T. ) ;
#51863=LINE ( 'NONE', #43623, #37418 ) ;
#51865=ORIENTED_EDGE ( 'NONE', *, *, #15202, .T. ) ;
#51866=CARTESIAN_POINT ( 'NONE',  ( -16.81267852042391198, -0.1191753592594197858, 3.312241722634738039 ) ) ;
#51867=VERTEX_POINT ( 'NONE', #21768 ) ;
#51868=VECTOR ( 'NONE', #21692, 999.9999999999998863 ) ;
#51869=VECTOR ( 'NONE', #18148, 1000.000000000000227 ) ;
#51870=LINE ( 'NONE', #29471, #46344 ) ;
#51871=CARTESIAN_POINT ( 'NONE',  ( -21.47263955680318404, 0.000000000000000000, 5.022634149262071190 ) ) ;
#51872=EDGE_CURVE ( 'NONE', #32655, #4253, #47898, .T. ) ;
#51873=DIRECTION ( 'NONE',  ( 0.5364919789714477361, 0.6444004775717706579, 0.5449076811759711036 ) ) ;
#51874=VECTOR ( 'NONE', #25551, 1000.000000000000227 ) ;
#51875=DIRECTION ( 'NONE',  ( 0.9999697198139515519, 0.000000000000000000, 0.007781995580013368816 ) ) ;
#51876=CARTESIAN_POINT ( 'NONE',  ( -20.54049170961573267, 0.000000000000000000, 4.660556269540326646 ) ) ;
#51878=EDGE_CURVE ( 'NONE', #11293, #24035, #38824, .T. ) ;
#51879=LINE ( 'NONE', #12996, #46583 ) ;
#51881=ORIENTED_EDGE ( 'NONE', *, *, #681, .F. ) ;
#51882=FACE_OUTER_BOUND ( 'NONE', #25331, .T. ) ;
#51883=EDGE_CURVE ( 'NONE', #18261, #187, #26303, .T. ) ;
#51884=FACE_OUTER_BOUND ( 'NONE', #14267, .T. ) ;
#51885=CARTESIAN_POINT ( 'NONE',  ( -12.33850799832341849, 0.000000000000000000, 11.68350162852954632 ) ) ;
#51886=LINE ( 'NONE', #43110, #4561 ) ;
#51887=AXIS2_PLACEMENT_3D ( 'NONE', #29468, #16676, #42525 ) ;
#51888=DIRECTION ( 'NONE',  ( -0.5364919789714478471, 0.6444004775717705469, -0.5449076811759709926 ) ) ;
#51889=CARTESIAN_POINT ( 'NONE',  ( -8.374569218570126594, 0.000000000000000000, 5.693904487294544126 ) ) ;
#51890=EDGE_CURVE ( 'NONE', #23769, #42201, #159, .T. ) ;
#51891=CARTESIAN_POINT ( 'NONE',  ( 2.072287782118878319, 0.000000000000000000, -2.950529333540147015 ) ) ;
#51892=DIRECTION ( 'NONE',  ( -0.9321478471874540261, 0.000000000000000000, 0.3620778797217457656 ) ) ;
#51894=ORIENTED_EDGE ( 'NONE', *, *, #9853, .T. ) ;
#51895=CARTESIAN_POINT ( 'NONE',  ( -16.48620427724178938, 0.000000000000000000, 7.277432160448412013 ) ) ;
#51896=FACE_OUTER_BOUND ( 'NONE', #53720, .T. ) ;
#51897=CARTESIAN_POINT ( 'NONE',  ( -20.54049170961573267, 0.000000000000000000, 4.660556269540326646 ) ) ;
#51899=FACE_OUTER_BOUND ( 'NONE', #16141, .T. ) ;
#51900=VECTOR ( 'NONE', #40747, 999.9999999999998863 ) ;
#51901=DIRECTION ( 'NONE',  ( 0.6427681459581294776, -0.7660444431189769032, 0.005002170337467562802 ) ) ;
#51902=CARTESIAN_POINT ( 'NONE',  ( -22.07366256627002699, 3.848249166794009746, 11.77111376987874358 ) ) ;
#51903=CARTESIAN_POINT ( 'NONE',  ( -10.03886374922923075, -0.1191753592594202438, 1.148964696635692562 ) ) ;
#51906=ORIENTED_EDGE ( 'NONE', *, *, #26090, .F. ) ;
#51907=LINE ( 'NONE', #56188, #36481 ) ;
#51908=VECTOR ( 'NONE', #35435, 1000.000000000000227 ) ;
#51909=AXIS2_PLACEMENT_3D ( 'NONE', #11601, #55301, #20088 ) ;
#51910=VERTEX_POINT ( 'NONE', #56133 ) ;
#51911=AXIS2_PLACEMENT_3D ( 'NONE', #12680, #4448, #8720 ) ;
#51912=EDGE_LOOP ( 'NONE', ( #12799, #36942, #27204, #10935 ) ) ;
#51914=VECTOR ( 'NONE', #56164, 1000.000000000000227 ) ;
#51915=ORIENTED_EDGE ( 'NONE', *, *, #28331, .F. ) ;
#51916=ORIENTED_EDGE ( 'NONE', *, *, #719, .F. ) ;
#51917=CARTESIAN_POINT ( 'NONE',  ( -11.30636317915456779, -0.1191753592594197858, 11.32220194836580340 ) ) ;
#51918=CARTESIAN_POINT ( 'NONE',  ( -13.08408713167409942, -0.1191753592594197858, 1.863930203747758085 ) ) ;
#51919=EDGE_CURVE ( 'NONE', #46599, #9606, #30597, .T. ) ;
#51920=EDGE_CURVE ( 'NONE', #15779, #49029, #43364, .T. ) ;
#51921=EDGE_LOOP ( 'NONE', ( #2513, #23247, #3810, #19353 ) ) ;
#51922=VECTOR ( 'NONE', #9209, 999.9999999999998863 ) ;
#51923=EDGE_CURVE ( 'NONE', #51035, #5744, #17499, .T. ) ;
#51924=AXIS2_PLACEMENT_3D ( 'NONE', #21961, #56067, #39289 ) ;
#51925=LINE ( 'NONE', #30374, #54773 ) ;
#51926=EDGE_LOOP ( 'NONE', ( #16271, #1597, #22058, #25318 ) ) ;
#51927=CARTESIAN_POINT ( 'NONE',  ( -27.99923088623136636, 0.000000000000000000, 7.757173251277078130 ) ) ;
#51928=CARTESIAN_POINT ( 'NONE',  ( -16.79925329029790149, 0.000000000000000000, 13.49544742625427496 ) ) ;
#51929=ORIENTED_EDGE ( 'NONE', *, *, #10507, .F. ) ;
#51930=DIRECTION ( 'NONE',  ( -0.5364919789714478471, 0.6444004775717705469, -0.5449076811759709926 ) ) ;
#51931=VECTOR ( 'NONE', #32276, 999.9999999999998863 ) ;
#51932=VERTEX_POINT ( 'NONE', #4183 ) ;
#51933=DIRECTION ( 'NONE',  ( 0.7660212471507180654, -0.6427876096865404731, 0.005961354470445141482 ) ) ;
#51934=VECTOR ( 'NONE', #48261, 1000.000000000000227 ) ;
#51935=CARTESIAN_POINT ( 'NONE',  ( 0.000000000000000000, 0.000000000000000000, 2.125000000000000000 ) ) ;
#51936=EDGE_LOOP ( 'NONE', ( #21774, #19120, #44641, #37538 ) ) ;
#51937=CARTESIAN_POINT ( 'NONE',  ( -19.60912206198628027, -0.1191753592594197858, 4.398475361799976113 ) ) ;
#51938=LINE ( 'NONE', #51413, #16583 ) ;
#51939=LINE ( 'NONE', #21001, #29385 ) ;
#51940=VECTOR ( 'NONE', #34133, 1000.000000000000227 ) ;
#51942=VERTEX_POINT ( 'NONE', #25459 ) ;
#51943=VECTOR ( 'NONE', #24937, 1000.000000000000114 ) ;
#51944=AXIS2_PLACEMENT_3D ( 'NONE', #54738, #11018, #16140 ) ;
#51945=DIRECTION ( 'NONE',  ( 0.5449076811759707706, 0.6444004775717708799, -0.5364919789714476250 ) ) ;
#51946=DIRECTION ( 'NONE',  ( 0.007781995580012663651, 0.000000000000000000, -0.9999697198139515519 ) ) ;
#51947=CARTESIAN_POINT ( 'NONE',  ( -11.67244013076689946, 0.000000000000000000, 11.50401908778467863 ) ) ;
#51948=LINE ( 'NONE', #35228, #5110 ) ;
#51949=LINE ( 'NONE', #16468, #6885 ) ;
#51950=EDGE_CURVE ( 'NONE', #43913, #5651, #47313, .T. ) ;
#51951=DIRECTION ( 'NONE',  ( 0.007781995580012663651, 0.000000000000000000, -0.9999697198139515519 ) ) ;
#51952=DIRECTION ( 'NONE',  ( 0.000000000000000000, 0.000000000000000000, 1.000000000000000000 ) ) ;
#51953=VECTOR ( 'NONE', #46124, 1000.000000000000114 ) ;
#51954=DIRECTION ( 'NONE',  ( 0.005961354470445682716, -0.6427876096865404731, -0.7660212471507180654 ) ) ;
#51955=CARTESIAN_POINT ( 'NONE',  ( -20.69132718766890022, -0.8417996532631562001, 4.891677461057035714 ) ) ;
#51956=AXIS2_PLACEMENT_3D ( 'NONE', #4551, #47144, #55971 ) ;
#51957=ORIENTED_EDGE ( 'NONE', *, *, #38842, .F. ) ;
#51959=EDGE_CURVE ( 'NONE', #39021, #8140, #17807, .T. ) ;
#51960=CARTESIAN_POINT ( 'NONE',  ( -17.46532115785441519, 0.000000000000000000, 13.67492996699914265 ) ) ;
#51961=EDGE_LOOP ( 'NONE', ( #7288, #8869, #17123, #29088 ) ) ;
#51962=CARTESIAN_POINT ( 'NONE',  ( -17.86155299234406968, 0.000000000000000000, 4.881410446302820283 ) ) ;
#51963=CARTESIAN_POINT ( 'NONE',  ( -13.54949002605227726, -3.432230869623161595, 2.034897051475980323 ) ) ;
#51964=EDGE_CURVE ( 'NONE', #27005, #34418, #43613, .T. ) ;
#51965=ADVANCED_FACE ( 'NONE', ( #26582 ), #55855, .F. ) ;
#51966=DIRECTION ( 'NONE',  ( -0.005002170337468016433, -0.7660444431189770143, 0.6427681459581293666 ) ) ;
#51967=VECTOR ( 'NONE', #55362, 1000.000000000000000 ) ;
#51968=VECTOR ( 'NONE', #42509, 1000.000000000000227 ) ;
#51969=FACE_OUTER_BOUND ( 'NONE', #50116, .T. ) ;
#51970=FACE_OUTER_BOUND ( 'NONE', #31871, .T. ) ;
#51971=VERTEX_POINT ( 'NONE', #4726 ) ;
#51972=ORIENTED_EDGE ( 'NONE', *, *, #55163, .F. ) ;
#51974=DIRECTION ( 'NONE',  ( -0.9999697198139514409, -0.000000000000000000, -0.007781995580013368816 ) ) ;
#51975=ORIENTED_EDGE ( 'NONE', *, *, #29108, .F. ) ;
#51976=VECTOR ( 'NONE', #38704, 1000.000000000000227 ) ;
#51977=FACE_OUTER_BOUND ( 'NONE', #43489, .T. ) ;
#51978=ORIENTED_EDGE ( 'NONE', *, *, #18533, .T. ) ;
#51979=DIRECTION ( 'NONE',  ( -0.9999697198139514409, -0.000000000000000000, -0.007781995580013368816 ) ) ;
#51980=VECTOR ( 'NONE', #32162, 1000.000000000000227 ) ;
#51981=ORIENTED_EDGE ( 'NONE', *, *, #32818, .T. ) ;
#51982=LINE ( 'NONE', #26708, #52882 ) ;
#51983=VERTEX_POINT ( 'NONE', #12429 ) ;
#51984=ORIENTED_EDGE ( 'NONE', *, *, #21695, .F. ) ;
#51985=ORIENTED_EDGE ( 'NONE', *, *, #48274, .T. ) ;
#51986=DIRECTION ( 'NONE',  ( 0.007781995580012663651, 0.000000000000000000, -0.9999697198139515519 ) ) ;
#51987=VECTOR ( 'NONE', #5230, 999.9999999999998863 ) ;
#51988=ADVANCED_FACE ( 'NONE', ( #5778 ), #52436, .F. ) ;
#51989=DIRECTION ( 'NONE',  ( -0.005002170337468016433, -0.7660444431189770143, 0.6427681459581293666 ) ) ;
#51991=VECTOR ( 'NONE', #15684, 1000.000000000000000 ) ;
#51992=VECTOR ( 'NONE', #15705, 1000.000000000000114 ) ;
#51993=EDGE_CURVE ( 'NONE', #44163, #42918, #13532, .T. ) ;
#51994=CARTESIAN_POINT ( 'NONE',  ( -12.29453239076688753, 0.000000000000000000, 6.032730497292229543 ) ) ;
#51995=ORIENTED_EDGE ( 'NONE', *, *, #54952, .F. ) ;
#51996=ORIENTED_EDGE ( 'NONE', *, *, #50651, .F. ) ;
#51997=EDGE_CURVE ( 'NONE', #13096, #37283, #30846, .T. ) ;
#51998=EDGE_CURVE ( 'NONE', #15364, #55560, #9258, .T. ) ;
#51999=VECTOR ( 'NONE', #8565, 1000.000000000000000 ) ;
#52000=ORIENTED_EDGE ( 'NONE', *, *, #46818, .F. ) ;
#52001=VECTOR ( 'NONE', #41632, 999.9999999999998863 ) ;
#52002=LINE ( 'NONE', #55152, #12231 ) ;
#52003=ORIENTED_EDGE ( 'NONE', *, *, #6679, .T. ) ;
#52004=DIRECTION ( 'NONE',  ( 0.7660212471507180654, -0.6427876096865404731, 0.005961354470445141482 ) ) ;
#52005=ORIENTED_EDGE ( 'NONE', *, *, #40941, .T. ) ;
#52006=CARTESIAN_POINT ( 'NONE',  ( -30.79411802867772607, 0.000000000000000000, 8.643412946479525516 ) ) ;
#52007=DIRECTION ( 'NONE',  ( -0.005961354470445682716, -0.6427876096865404731, 0.7660212471507180654 ) ) ;
#52008=ORIENTED_EDGE ( 'NONE', *, *, #19560, .F. ) ;
#52009=LINE ( 'NONE', #4875, #47671 ) ;
#52010=ORIENTED_EDGE ( 'NONE', *, *, #37894, .F. ) ;
#52011=EDGE_CURVE ( 'NONE', #34091, #37711, #44661, .T. ) ;
#52012=PLANE ( 'NONE',  #50863 ) ;
#52013=VECTOR ( 'NONE', #8023, 1000.000000000000227 ) ;
#52014=ORIENTED_EDGE ( 'NONE', *, *, #43340, .T. ) ;
#52015=CARTESIAN_POINT ( 'NONE',  ( -24.27063949748155380, 0.000000000000000000, 6.308861732390097288 ) ) ;
#52016=DIRECTION ( 'NONE',  ( 0.005961354470445682716, -0.6427876096865404731, -0.7660212471507180654 ) ) ;
#52017=DIRECTION ( 'NONE',  ( 0.9999697198139515519, 0.000000000000000000, 0.007781995580013368816 ) ) ;
#52018=EDGE_LOOP ( 'NONE', ( #23464, #45439, #43412, #48463 ) ) ;
#52019=VECTOR ( 'NONE', #50753, 1000.000000000000227 ) ;
#52020=LINE ( 'NONE', #40851, #52887 ) ;
#52021=DIRECTION ( 'NONE',  ( 0.007781995580012662783, 0.000000000000000000, -0.9999697198139514409 ) ) ;
#52023=AXIS2_PLACEMENT_3D ( 'NONE', #4265, #17882, #29816 ) ;
#52024=DIRECTION ( 'NONE',  ( -0.6427681459581293666, -0.7660444431189770143, -0.005002170337467561935 ) ) ;
#52025=PLANE ( 'NONE',  #27648 ) ;
#52026=FACE_OUTER_BOUND ( 'NONE', #4779, .T. ) ;
#52027=SURFACE_STYLE_FILL_AREA ( #4609 ) ;
#52028=ORIENTED_EDGE ( 'NONE', *, *, #23773, .F. ) ;
#52029=PLANE ( 'NONE',  #18941 ) ;
#52030=CARTESIAN_POINT ( 'NONE',  ( -18.24297520525825433, 4.819660872929008910, 11.87739681187417773 ) ) ;
#52031=CARTESIAN_POINT ( 'NONE',  ( -18.98145280571277027, -5.375054281893163477, 12.87635240835876438 ) ) ;
#52032=ORIENTED_EDGE ( 'NONE', *, *, #25254, .F. ) ;
#52033=VECTOR ( 'NONE', #39849, 999.9999999999998863 ) ;
#52034=CARTESIAN_POINT ( 'NONE',  ( -24.27063949748155380, 0.000000000000000000, 6.308861732390097288 ) ) ;
#52035=ORIENTED_EDGE ( 'NONE', *, *, #42708, .F. ) ;
#52036=AXIS2_PLACEMENT_3D ( 'NONE', #35217, #31212, #26381 ) ;
#52037=FACE_OUTER_BOUND ( 'NONE', #49856, .T. ) ;
#52038=ADVANCED_FACE ( 'NONE', ( #36424 ), #37257, .F. ) ;
#52039=DIRECTION ( 'NONE',  ( -0.5364919789714478471, 0.6444004775717705469, -0.5449076811759709926 ) ) ;
#52040=LINE ( 'NONE', #52600, #18750 ) ;
#52042=ORIENTED_EDGE ( 'NONE', *, *, #51861, .F. ) ;
#52043=AXIS2_PLACEMENT_3D ( 'NONE', #6798, #15866, #41152 ) ;
#52044=VECTOR ( 'NONE', #41304, 999.9999999999998863 ) ;
#52045=ORIENTED_EDGE ( 'NONE', *, *, #30144, .F. ) ;
#52046=CARTESIAN_POINT ( 'NONE',  ( -13.95727774206300786, 0.000000000000000000, 6.558448711888932969 ) ) ;
#52047=LINE ( 'NONE', #48066, #31358 ) ;
#52048=LINE ( 'NONE', #21944, #36090 ) ;
#52049=ADVANCED_FACE ( 'NONE', ( #54559 ), #15667, .F. ) ;
#52050=DIRECTION ( 'NONE',  ( 0.007781995580012663651, -3.146120232559066537E-19, -0.9999697198139514409 ) ) ;
#52051=CARTESIAN_POINT ( 'NONE',  ( -9.829290562097927619, 1.000354561442236001, 1.688498333329506051 ) ) ;
#52052=DIRECTION ( 'NONE',  ( 0.000000000000000000, -1.000000000000000000, 0.000000000000000000 ) ) ;
#52054=EDGE_CURVE ( 'NONE', #27710, #27265, #54305, .T. ) ;
#52056=EDGE_CURVE ( 'NONE', #11058, #20365, #54039, .T. ) ;
#52057=VECTOR ( 'NONE', #24994, 1000.000000000000227 ) ;
#52058=PLANE ( 'NONE',  #7016 ) ;
#52059=EDGE_LOOP ( 'NONE', ( #48993, #47307, #21830, #2415, #15386 ) ) ;
#52060=AXIS2_PLACEMENT_3D ( 'NONE', #9771, #22262, #1518 ) ;
#52061=PLANE ( 'NONE',  #39231 ) ;
#52062=ADVANCED_FACE ( 'NONE', ( #6338 ), #33004, .F. ) ;
#52063=CARTESIAN_POINT ( 'NONE',  ( -19.49193266702258853, -0.5179957512181551094, 5.103379603946674337 ) ) ;
#52064=VECTOR ( 'NONE', #33644, 1000.000000000000000 ) ;
#52065=LINE ( 'NONE', #56064, #52929 ) ;
#52066=EDGE_LOOP ( 'NONE', ( #20269, #42423, #34664, #13766 ) ) ;
#52067=DIRECTION ( 'NONE',  ( 0.5364919789714477361, 0.6444004775717706579, 0.5449076811759711036 ) ) ;
#52068=EDGE_CURVE ( 'NONE', #14352, #5802, #2045, .T. ) ;
#52069=VECTOR ( 'NONE', #36578, 1000.000000000000114 ) ;
#52070=ORIENTED_EDGE ( 'NONE', *, *, #31837, .F. ) ;
#52071=ADVANCED_FACE ( 'NONE', ( #50322 ), #19099, .F. ) ;
#52072=ORIENTED_EDGE ( 'NONE', *, *, #33697, .T. ) ;
#52073=ORIENTED_EDGE ( 'NONE', *, *, #19365, .T. ) ;
#52074=VERTEX_POINT ( 'NONE', #49507 ) ;
#52075=VECTOR ( 'NONE', #42570, 999.9999999999998863 ) ;
#52076=DIRECTION ( 'NONE',  ( -0.5364919789714478471, 0.6444004775717705469, -0.5449076811759709926 ) ) ;
#52077=VERTEX_POINT ( 'NONE', #36717 ) ;
#52079=VECTOR ( 'NONE', #18362, 999.9999999999998863 ) ;
#52080=EDGE_CURVE ( 'NONE', #45468, #41108, #24471, .T. ) ;
#52081=ORIENTED_EDGE ( 'NONE', *, *, #22725, .F. ) ;
#52082=DIRECTION ( 'NONE',  ( -0.9999697198139514409, -0.000000000000000000, -0.007781995580013368816 ) ) ;
#52083=ORIENTED_EDGE ( 'NONE', *, *, #20186, .F. ) ;
#52084=FACE_OUTER_BOUND ( 'NONE', #50640, .T. ) ;
#52085=ORIENTED_EDGE ( 'NONE', *, *, #5022, .T. ) ;
#52086=EDGE_CURVE ( 'NONE', #32862, #11430, #53474, .T. ) ;
#52087=VECTOR ( 'NONE', #39425, 1000.000000000000227 ) ;
#52088=VECTOR ( 'NONE', #41875, 1000.000000000000227 ) ;
#52089=FACE_OUTER_BOUND ( 'NONE', #35200, .T. ) ;
#52090=DIRECTION ( 'NONE',  ( 0.9999697198139515519, 0.000000000000000000, 0.007781995580013368816 ) ) ;
#52091=LINE ( 'NONE', #8669, #34142 ) ;
#52092=DIRECTION ( 'NONE',  ( -0.6427681459581293666, -0.7660444431189770143, -0.005002170337467561935 ) ) ;
#52093=DIRECTION ( 'NONE',  ( 0.5449076811759707706, 0.6444004775717708799, -0.5364919789714476250 ) ) ;
#52094=EDGE_LOOP ( 'NONE', ( #34475, #5221, #3410, #46169 ) ) ;
#52095=ORIENTED_EDGE ( 'NONE', *, *, #26297, .T. ) ;
#52096=DIRECTION ( 'NONE',  ( 0.5449076811759707706, 0.6444004775717708799, -0.5364919789714476250 ) ) ;
#52098=DIRECTION ( 'NONE',  ( 0.000000000000000000, -1.000000000000000000, 0.000000000000000000 ) ) ;
#52099=VECTOR ( 'NONE', #9268, 1000.000000000000227 ) ;
#52100=PLANE ( 'NONE',  #14162 ) ;
#52101=VECTOR ( 'NONE', #15579, 1000.000000000000227 ) ;
#52102=FACE_OUTER_BOUND ( 'NONE', #4389, .T. ) ;
#52103=LINE ( 'NONE', #50962, #54950 ) ;
#52104=ORIENTED_EDGE ( 'NONE', *, *, #28454, .F. ) ;
#52105=DIRECTION ( 'NONE',  ( 0.5364919789714477361, 0.6444004775717706579, 0.5449076811759711036 ) ) ;
#52106=DIRECTION ( 'NONE',  ( 0.007781995580012662783, 0.000000000000000000, -0.9999697198139514409 ) ) ;
#52108=EDGE_LOOP ( 'NONE', ( #50838, #48288, #50614, #21501 ) ) ;
#52109=LINE ( 'NONE', #16931, #24316 ) ;
#52111=EDGE_CURVE ( 'NONE', #6114, #93, #46066, .T. ) ;
#52112=CARTESIAN_POINT ( 'NONE',  ( -33.59056157024009082, 0.000000000000000000, 9.729646585644761814 ) ) ;
#52113=DIRECTION ( 'NONE',  ( 0.005002170337468016433, -0.7660444431189770143, -0.6427681459581293666 ) ) ;
#52114=DIRECTION ( 'NONE',  ( 0.7660212471507180654, -0.6427876096865404731, 0.005961354470445141482 ) ) ;
#52115=ORIENTED_EDGE ( 'NONE', *, *, #39489, .T. ) ;
#52116=VECTOR ( 'NONE', #39691, 1000.000000000000227 ) ;
#52117=ORIENTED_EDGE ( 'NONE', *, *, #29291, .T. ) ;
#52118=VECTOR ( 'NONE', #7434, 1000.000000000000227 ) ;
#52119=FACE_OUTER_BOUND ( 'NONE', #30657, .T. ) ;
#52121=DIRECTION ( 'NONE',  ( 0.007781995580012663651, 0.000000000000000000, -0.9999697198139515519 ) ) ;
#52122=AXIS2_PLACEMENT_3D ( 'NONE', #9668, #27523, #10505 ) ;
#52123=LINE ( 'NONE', #39064, #1037 ) ;
#52124=DIRECTION ( 'NONE',  ( 0.000000000000000000, -0.000000000000000000, -1.000000000000000000 ) ) ;
#52125=CARTESIAN_POINT ( 'NONE',  ( -18.33325565058499862, 0.000000000000000000, 5.785729700345316751 ) ) ;
#52126=PLANE ( 'NONE',  #31125 ) ;
#52127=ORIENTED_EDGE ( 'NONE', *, *, #46327, .F. ) ;
#52128=EDGE_CURVE ( 'NONE', #32474, #48923, #19937, .T. ) ;
#52129=VECTOR ( 'NONE', #669, 1000.000000000000000 ) ;
#52130=LINE ( 'NONE', #9830, #45904 ) ;
#52131=AXIS2_PLACEMENT_3D ( 'NONE', #16075, #54393, #54666 ) ;
#52132=PLANE ( 'NONE',  #37815 ) ;
#52133=ORIENTED_EDGE ( 'NONE', *, *, #20660, .T. ) ;
#52134=FACE_OUTER_BOUND ( 'NONE', #17290, .T. ) ;
#52135=ORIENTED_EDGE ( 'NONE', *, *, #51352, .T. ) ;
#52136=LINE ( 'NONE', #30838, #54931 ) ;
#52137=FACE_OUTER_BOUND ( 'NONE', #14448, .T. ) ;
#52138=EDGE_LOOP ( 'NONE', ( #50854, #843, #42702, #40832 ) ) ;
#52139=EDGE_CURVE ( 'NONE', #49589, #30407, #6908, .T. ) ;
#52140=ORIENTED_EDGE ( 'NONE', *, *, #18641, .F. ) ;
#52141=EDGE_CURVE ( 'NONE', #52348, #28760, #41251, .T. ) ;
#52142=AXIS2_PLACEMENT_3D ( 'NONE', #30882, #34580, #9609 ) ;
#52143=EDGE_LOOP ( 'NONE', ( #41183, #12420, #26590 ) ) ;
#52144=EDGE_LOOP ( 'NONE', ( #28528, #13423, #22953, #47410 ) ) ;
#52145=ORIENTED_EDGE ( 'NONE', *, *, #41044, .T. ) ;
#52146=VECTOR ( 'NONE', #163, 999.9999999999998863 ) ;
#52147=EDGE_LOOP ( 'NONE', ( #43524, #41853, #48051, #10898 ) ) ;
#52148=DIRECTION ( 'NONE',  ( 0.9999697198139515519, 0.000000000000000000, 0.007781995580013368816 ) ) ;
#52149=CARTESIAN_POINT ( 'NONE',  ( -20.54126990917373519, -0.1191753592594197858, 4.760553241521720658 ) ) ;
#52150=AXIS2_PLACEMENT_3D ( 'NONE', #2382, #45525, #12004 ) ;
#52152=ORIENTED_EDGE ( 'NONE', *, *, #27315, .F. ) ;
#52153=DIRECTION ( 'NONE',  ( 0.000000000000000000, -1.000000000000000000, 0.000000000000000000 ) ) ;
#52154=ORIENTED_EDGE ( 'NONE', *, *, #18798, .T. ) ;
#52155=VECTOR ( 'NONE', #45071, 999.9999999999998863 ) ;
#52156=ORIENTED_EDGE ( 'NONE', *, *, #38954, .F. ) ;
#52157=EDGE_CURVE ( 'NONE', #16476, #11761, #20208, .T. ) ;
#52158=AXIS2_PLACEMENT_3D ( 'NONE', #8356, #20853, #25401 ) ;
#52159=AXIS2_PLACEMENT_3D ( 'NONE', #37282, #28791, #46650 ) ;
#52160=DIRECTION ( 'NONE',  ( 0.007781995580012662783, 0.000000000000000000, -0.9999697198139514409 ) ) ;
#52161=DIRECTION ( 'NONE',  ( -0.6427681459581293666, -0.7660444431189770143, -0.005002170337467561935 ) ) ;
#52162=VECTOR ( 'NONE', #29704, 1000.000000000000227 ) ;
#52163=CARTESIAN_POINT ( 'NONE',  ( -10.76106947438395167, -0.1191753592594190225, 0.9615912556445452841 ) ) ;
#52164=EDGE_LOOP ( 'NONE', ( #51671, #27615, #37241, #19250 ) ) ;
#52165=DIRECTION ( 'NONE',  ( -0.3620778797217457101, 0.000000000000000000, -0.9321478471874540261 ) ) ;
#52166=EDGE_LOOP ( 'NONE', ( #7552, #1883, #47537, #23073 ) ) ;
#52167=VECTOR ( 'NONE', #41141, 1000.000000000000227 ) ;
#52168=DIRECTION ( 'NONE',  ( -0.5449076811759708816, 0.6444004775717707689, 0.5364919789714475140 ) ) ;
#52169=PLANE ( 'NONE',  #32095 ) ;
#52171=FACE_OUTER_BOUND ( 'NONE', #29315, .T. ) ;
#52172=VECTOR ( 'NONE', #6571, 1000.000000000000227 ) ;
#52173=CARTESIAN_POINT ( 'NONE',  ( -15.81582532942734431, 0.000000000000000000, 6.543985064816895125 ) ) ;
#52174=CARTESIAN_POINT ( 'NONE',  ( -18.75581683353525619, -4.565544526780660917, 11.46016431438283334 ) ) ;
#52175=PLANE ( 'NONE',  #7656 ) ;
#52176=DIRECTION ( 'NONE',  ( 0.6246952433987893460, 0.7422098413412802076, -0.2426528472758539279 ) ) ;
#52177=DIRECTION ( 'NONE',  ( -0.5449076811759708816, 0.6444004775717707689, 0.5364919789714475140 ) ) ;
#52178=ORIENTED_EDGE ( 'NONE', *, *, #1235, .T. ) ;
#52179=CARTESIAN_POINT ( 'NONE',  ( -17.14676106981525550, -2.137015261443158565, 6.849522152733298341 ) ) ;
#52180=EDGE_CURVE ( 'NONE', #8547, #46010, #28458, .T. ) ;
#52182=DIRECTION ( 'NONE',  ( 0.000000000000000000, -1.000000000000000000, 0.000000000000000000 ) ) ;
#52183=DIRECTION ( 'NONE',  ( 0.007781995580012662783, 0.000000000000000000, -0.9999697198139514409 ) ) ;
#52185=DIRECTION ( 'NONE',  ( -0.005961354470445682716, -0.6427876096865404731, 0.7660212471507180654 ) ) ;
#52186=PLANE ( 'NONE',  #32237 ) ;
#52187=DIRECTION ( 'NONE',  ( 0.005002170337468016433, -0.7660444431189770143, -0.6427681459581293666 ) ) ;
#52188=VECTOR ( 'NONE', #18304, 1000.000000000000227 ) ;
#52189=DIRECTION ( 'NONE',  ( -0.6427681459581293666, -0.7660444431189770143, -0.005002170337467561935 ) ) ;
#52190=ADVANCED_FACE ( 'NONE', ( #42075 ), #50612, .F. ) ;
#52192=VECTOR ( 'NONE', #47745, 1000.000000000000114 ) ;
#52193=ORIENTED_EDGE ( 'NONE', *, *, #8176, .T. ) ;
#52194=EDGE_CURVE ( 'NONE', #42137, #4086, #15977, .T. ) ;
#52196=DIRECTION ( 'NONE',  ( 0.007781995580012663651, 0.000000000000000000, -0.9999697198139515519 ) ) ;
#52197=CARTESIAN_POINT ( 'NONE',  ( -12.30447220567201860, 0.000000000000000000, 7.309975366360497162 ) ) ;
#52198=VECTOR ( 'NONE', #16076, 999.9999999999998863 ) ;
#52199=ADVANCED_FACE ( 'NONE', ( #20516 ), #55703, .F. ) ;
#52200=EDGE_CURVE ( 'NONE', #2695, #26378, #56005, .T. ) ;
#52201=EDGE_CURVE ( 'NONE', #28225, #12870, #55151, .T. ) ;
#52202=LINE ( 'NONE', #26342, #44528 ) ;
#52203=VECTOR ( 'NONE', #34705, 1000.000000000000114 ) ;
#52204=DIRECTION ( 'NONE',  ( 0.000000000000000000, -1.000000000000000000, 0.000000000000000000 ) ) ;
#52205=LINE ( 'NONE', #4502, #37702 ) ;
#52206=CARTESIAN_POINT ( 'NONE',  ( -14.66887761629205222, 0.000000000000000000, 12.58869632783390990 ) ) ;
#52207=CARTESIAN_POINT ( 'NONE',  ( -14.92512947252347466, -5.536956232915663634, 11.56644735637827104 ) ) ;
#52208=AXIS2_PLACEMENT_3D ( 'NONE', #48682, #2054, #36434 ) ;
#52209=DIRECTION ( 'NONE',  ( 0.7660212471507180654, -0.6427876096865404731, 0.005961354470445141482 ) ) ;
#52210=AXIS2_PLACEMENT_3D ( 'NONE', #51010, #42775, #55866 ) ;
#52211=EDGE_LOOP ( 'NONE', ( #16914, #45568, #44335, #36660 ) ) ;
#52212=LINE ( 'NONE', #43955, #23782 ) ;
#52213=VECTOR ( 'NONE', #47279, 1000.000000000000227 ) ;
#52214=ORIENTED_EDGE ( 'NONE', *, *, #50856, .T. ) ;
#52215=VECTOR ( 'NONE', #10624, 1000.000000000000227 ) ;
#52216=EDGE_CURVE ( 'NONE', #40111, #17065, #29023, .T. ) ;
#52217=AXIS2_PLACEMENT_3D ( 'NONE', #36920, #15319, #32630 ) ;
#52218=VECTOR ( 'NONE', #5295, 1000.000000000000114 ) ;
#52219=EDGE_CURVE ( 'NONE', #19083, #41253, #51162, .T. ) ;
#52220=ORIENTED_EDGE ( 'NONE', *, *, #32555, .F. ) ;
#52221=VECTOR ( 'NONE', #5061, 999.9999999999998863 ) ;
#52222=VERTEX_POINT ( 'NONE', #42636 ) ;
#52223=ORIENTED_EDGE ( 'NONE', *, *, #28853, .F. ) ;
#52224=ADVANCED_FACE ( 'NONE', ( #3469 ), #34151, .F. ) ;
#52225=ORIENTED_EDGE ( 'NONE', *, *, #53156, .T. ) ;
#52226=CARTESIAN_POINT ( 'NONE',  ( -14.66494788901886714, 5.629170628041515023, 2.198695500334132191 ) ) ;
#52227=CARTESIAN_POINT ( 'NONE',  ( -20.54126990917373519, -0.1191753592594197858, 4.760553241521720658 ) ) ;
#52228=EDGE_CURVE ( 'NONE', #4182, #17775, #50869, .T. ) ;
#52229=ORIENTED_EDGE ( 'NONE', *, *, #29913, .T. ) ;
#52230=EDGE_LOOP ( 'NONE', ( #2955, #31425, #31970 ) ) ;
#52231=VECTOR ( 'NONE', #52809, 1000.000000000000000 ) ;
#52232=DIRECTION ( 'NONE',  ( 0.007781995580012662783, 0.000000000000000000, -0.9999697198139514409 ) ) ;
#52233=ORIENTED_EDGE ( 'NONE', *, *, #54800, .T. ) ;
#52234=DIRECTION ( 'NONE',  ( -0.7660212471507179544, -0.6427876096865405842, -0.005961354470445141482 ) ) ;
#52235=LINE ( 'NONE', #13343, #488 ) ;
#52236=ORIENTED_EDGE ( 'NONE', *, *, #20159, .F. ) ;
#52237=VECTOR ( 'NONE', #16855, 1000.000000000000227 ) ;
#52238=DIRECTION ( 'NONE',  ( 0.007781995580012663651, 0.000000000000000000, -0.9999697198139515519 ) ) ;
#52239=VERTEX_POINT ( 'NONE', #46320 ) ;
#52240=DIRECTION ( 'NONE',  ( 0.007781995580012663651, -3.146120232559066537E-19, -0.9999697198139514409 ) ) ;
#52241=AXIS2_PLACEMENT_3D ( 'NONE', #35017, #43505, #21918 ) ;
#52242=LINE ( 'NONE', #13351, #3687 ) ;
#52243=VECTOR ( 'NONE', #40604, 1000.000000000000114 ) ;
#52244=VECTOR ( 'NONE', #100, 1000.000000000000114 ) ;
#52245=EDGE_LOOP ( 'NONE', ( #10602, #50446, #20513, #36156 ) ) ;
#52246=PLANE ( 'NONE',  #13169 ) ;
#52247=DIRECTION ( 'NONE',  ( 0.007781995580012662783, 0.000000000000000000, -0.9999697198139514409 ) ) ;
#52248=CARTESIAN_POINT ( 'NONE',  ( -12.80458192191714595, 0.000000000000000000, 11.86454056839041726 ) ) ;
#52249=ORIENTED_EDGE ( 'NONE', *, *, #24626, .F. ) ;
#52250=CARTESIAN_POINT ( 'NONE',  ( -9.764049456472102761, 0.000000000000000000, 5.113753104769962476 ) ) ;
#52252=VECTOR ( 'NONE', #26994, 1000.000000000000227 ) ;
#52253=AXIS2_PLACEMENT_3D ( 'NONE', #45318, #32279, #32548 ) ;
#52254=LINE ( 'NONE', #21301, #17422 ) ;
#52255=CARTESIAN_POINT ( 'NONE',  ( -20.02908140811766913, -1.193365355704625541, 6.079151905931945876 ) ) ;
#52256=DIRECTION ( 'NONE',  ( -0.3313982828793700097, 0.4028455766673915694, -0.8531650599175529814 ) ) ;
#52257=CARTESIAN_POINT ( 'NONE',  ( -10.37421533196711465, -0.1191753592594197858, 10.96012406864405975 ) ) ;
#52258=FACE_OUTER_BOUND ( 'NONE', #41274, .T. ) ;
#52259=CARTESIAN_POINT ( 'NONE',  ( -14.43784130554650424, 0.000000000000000000, 8.601375260372536857 ) ) ;
#52260=DIRECTION ( 'NONE',  ( -0.2426528472758541499, 0.7422098413412800966, -0.6246952433987894571 ) ) ;
#52261=AXIS2_PLACEMENT_3D ( 'NONE', #21890, #34667, #51989 ) ;
#52262=VECTOR ( 'NONE', #53510, 999.9999999999998863 ) ;
#52264=DIRECTION ( 'NONE',  ( -0.6427681459581293666, -0.7660444431189770143, -0.005002170337467561935 ) ) ;
#52265=EDGE_LOOP ( 'NONE', ( #38028, #27796, #22945 ) ) ;
#52266=CARTESIAN_POINT ( 'NONE',  ( -11.67244013076689946, 0.000000000000000000, 11.50401908778467863 ) ) ;
#52267=CARTESIAN_POINT ( 'NONE',  ( -15.87975247367846166, 0.000000000000000000, 2.850166870931599927 ) ) ;
#52268=LINE ( 'NONE', #38136, #36820 ) ;
#52269=EDGE_CURVE ( 'NONE', #36106, #54291, #4029, .T. ) ;
#52270=EDGE_CURVE ( 'NONE', #2049, #35294, #55412, .T. ) ;
#52271=DIRECTION ( 'NONE',  ( -0.9999697198139514409, -0.000000000000000000, -0.007781995580013368816 ) ) ;
#52272=EDGE_CURVE ( 'NONE', #43300, #3456, #37844, .T. ) ;
#52273=DIRECTION ( 'NONE',  ( -0.6427681459581293666, -0.7660444431189770143, -0.005002170337467561935 ) ) ;
#52274=CARTESIAN_POINT ( 'NONE',  ( -13.18201201109693166, 2.714935509636505984, 6.457333944872381437 ) ) ;
#52276=ORIENTED_EDGE ( 'NONE', *, *, #817, .F. ) ;
#52277=ORIENTED_EDGE ( 'NONE', *, *, #31652, .F. ) ;
#52278=DIRECTION ( 'NONE',  ( 0.7660212471507180654, -0.6427876096865404731, 0.005961354470445141482 ) ) ;
#52279=CARTESIAN_POINT ( 'NONE',  ( -20.41930778315827766, 0.3880542636427237180, 5.074537440973727165 ) ) ;
#52281=AXIS2_PLACEMENT_3D ( 'NONE', #44009, #35234, #52264 ) ;
#52282=DIRECTION ( 'NONE',  ( 0.000000000000000000, -1.000000000000000000, 0.000000000000000000 ) ) ;
#52283=VERTEX_POINT ( 'NONE', #54863 ) ;
#52284=DIRECTION ( 'NONE',  ( -0.005002170337468016433, -0.7660444431189770143, 0.6427681459581293666 ) ) ;
#52285=VECTOR ( 'NONE', #8328, 1000.000000000000227 ) ;
#52287=PLANE ( 'NONE',  #3918 ) ;
#52288=EDGE_CURVE ( 'NONE', #1421, #1358, #24757, .T. ) ;
#52289=AXIS2_PLACEMENT_3D ( 'NONE', #8455, #52182, #35708 ) ;
#52290=ORIENTED_EDGE ( 'NONE', *, *, #41163, .F. ) ;
#52291=ORIENTED_EDGE ( 'NONE', *, *, #1491, .F. ) ;
#52292=EDGE_LOOP ( 'NONE', ( #537, #29181, #23137, #45885 ) ) ;
#52293=ADVANCED_FACE ( 'NONE', ( #33843 ), #12273, .F. ) ;
#52294=CARTESIAN_POINT ( 'NONE',  ( 1.086233639165236964, 0.000000000000000000, 2.796443541562362078 ) ) ;
#52295=CARTESIAN_POINT ( 'NONE',  ( -10.74029228357944987, 0.000000000000000000, 11.14194120806293320 ) ) ;
#52296=DIRECTION ( 'NONE',  ( 0.007781995580012663651, 0.000000000000000000, -0.9999697198139515519 ) ) ;
#52297=EDGE_CURVE ( 'NONE', #34418, #8057, #38382, .T. ) ;
#52298=VECTOR ( 'NONE', #14944, 1000.000000000000227 ) ;
#52299=DIRECTION ( 'NONE',  ( -0.005961354470445682716, -0.6427876096865404731, 0.7660212471507180654 ) ) ;
#52300=ORIENTED_EDGE ( 'NONE', *, *, #4209, .T. ) ;
#52301=ORIENTED_EDGE ( 'NONE', *, *, #35122, .F. ) ;
#52302=EDGE_CURVE ( 'NONE', #51780, #41612, #12502, .T. ) ;
#52303=AXIS2_PLACEMENT_3D ( 'NONE', #52491, #31187, #34601 ) ;
#52304=VECTOR ( 'NONE', #25305, 1000.000000000000227 ) ;
#52305=ORIENTED_EDGE ( 'NONE', *, *, #54635, .T. ) ;
#52306=CARTESIAN_POINT ( 'NONE',  ( -14.90368544486988789, -2.784623065533159636, 7.041070140637504693 ) ) ;
#52307=VERTEX_POINT ( 'NONE', #55636 ) ;
#52308=DIRECTION ( 'NONE',  ( -0.9999697198139514409, 0.000000000000000000, -0.007781995580013368816 ) ) ;
#52309=EDGE_CURVE ( 'NONE', #9006, #55190, #12201, .T. ) ;
#52310=ORIENTED_EDGE ( 'NONE', *, *, #3592, .T. ) ;
#52311=CARTESIAN_POINT ( 'NONE',  ( -32.65997012216863737, 0.000000000000000000, 9.567562649885804404 ) ) ;
#52312=FACE_OUTER_BOUND ( 'NONE', #24980, .T. ) ;
#52313=ORIENTED_EDGE ( 'NONE', *, *, #8906, .T. ) ;
#52314=LINE ( 'NONE', #43494, #5966 ) ;
#52315=ORIENTED_EDGE ( 'NONE', *, *, #35218, .F. ) ;
#52316=AXIS2_PLACEMENT_3D ( 'NONE', #7683, #46875, #33520 ) ;
#52317=LINE ( 'NONE', #38393, #13663 ) ;
#52318=ORIENTED_EDGE ( 'NONE', *, *, #47587, .F. ) ;
#52319=LINE ( 'NONE', #49148, #23144 ) ;
#52320=CARTESIAN_POINT ( 'NONE',  ( -13.63673279712320507, -0.1191753592594197858, 12.22739664767016521 ) ) ;
#52321=DIRECTION ( 'NONE',  ( -0.7660212471507179544, -0.6427876096865405842, -0.005961354470445141482 ) ) ;
#52323=DIRECTION ( 'NONE',  ( 0.007781995580012663651, -3.146120232559066537E-19, -0.9999697198139514409 ) ) ;
#52324=PLANE ( 'NONE',  #2851 ) ;
#52325=AXIS2_PLACEMENT_3D ( 'NONE', #19733, #31414, #48730 ) ;
#52326=CARTESIAN_POINT ( 'NONE',  ( -29.86197018149027116, 0.000000000000000000, 8.281335066757780083 ) ) ;
#52327=LINE ( 'NONE', #13140, #42178 ) ;
#52328=PLANE ( 'NONE',  #13091 ) ;
#52329=CARTESIAN_POINT ( 'NONE',  ( -9.512215248562165826, 1.791064371115911102, 2.504789765260621248 ) ) ;
#52330=VECTOR ( 'NONE', #5527, 1000.000000000000114 ) ;
#52331=LINE ( 'NONE', #22511, #11338 ) ;
#52332=VERTEX_POINT ( 'NONE', #29542 ) ;
#52333=DIRECTION ( 'NONE',  ( 0.005002170337468016433, -0.7660444431189770143, -0.6427681459581293666 ) ) ;
#52334=CARTESIAN_POINT ( 'NONE',  ( 2.072287782118878319, 0.000000000000000000, -2.950529333540147015 ) ) ;
#52335=LINE ( 'NONE', #13438, #50451 ) ;
#52336=ORIENTED_EDGE ( 'NONE', *, *, #29887, .F. ) ;
#52337=FACE_OUTER_BOUND ( 'NONE', #45132, .T. ) ;
#52338=LINE ( 'NONE', #48323, #28143 ) ;
#52339=ORIENTED_EDGE ( 'NONE', *, *, #1517, .F. ) ;
#52340=EDGE_CURVE ( 'NONE', #39021, #9132, #42854, .T. ) ;
#52341=CARTESIAN_POINT ( 'NONE',  ( -9.808144436391993182, 0.000000000000000000, 10.77986332834118777 ) ) ;
#52342=AXIS2_PLACEMENT_3D ( 'NONE', #1665, #40592, #18993 ) ;
#52343=CARTESIAN_POINT ( 'NONE',  ( -24.27063949748155380, 0.000000000000000000, 6.308861732390097288 ) ) ;
#52344=ADVANCED_FACE ( 'NONE', ( #7965 ), #4268, .F. ) ;
#52345=EDGE_CURVE ( 'NONE', #32268, #44507, #12760, .T. ) ;
#52346=FACE_OUTER_BOUND ( 'NONE', #50408, .T. ) ;
#52347=DIRECTION ( 'NONE',  ( 0.5364919789714477361, 0.6444004775717706579, 0.5449076811759711036 ) ) ;
#52348=VERTEX_POINT ( 'NONE', #21283 ) ;
#52349=VECTOR ( 'NONE', #52738, 1000.000000000000227 ) ;
#52350=ORIENTED_EDGE ( 'NONE', *, *, #40815, .F. ) ;
#52351=CARTESIAN_POINT ( 'NONE',  ( -10.70769351768068844, 0.000000000000000000, 6.953069797522764439 ) ) ;
#52352=PLANE ( 'NONE',  #13247 ) ;
#52353=CARTESIAN_POINT ( 'NONE',  ( 2.072287782118878319, 0.000000000000000000, -2.950529333540147015 ) ) ;
#52354=CARTESIAN_POINT ( 'NONE',  ( -19.60990026154428278, 0.000000000000000000, 4.498472333781370125 ) ) ;
#52355=CARTESIAN_POINT ( 'NONE',  ( -14.04402961146700335, -5.051250379848162275, 10.42707219621531678 ) ) ;
#52356=CARTESIAN_POINT ( 'NONE',  ( -18.67619601524082285, 0.000000000000000000, 3.936400510096834893 ) ) ;
#52357=EDGE_LOOP ( 'NONE', ( #27157, #39252, #43963, #24837 ) ) ;
#52358=FACE_OUTER_BOUND ( 'NONE', #12460, .T. ) ;
#52359=LINE ( 'NONE', #38746, #41461 ) ;
#52360=ORIENTED_EDGE ( 'NONE', *, *, #5793, .T. ) ;
#52361=CARTESIAN_POINT ( 'NONE',  ( -11.81971693429394854, 0.000000000000000000, 4.728423355324156141 ) ) ;
#52362=LINE ( 'NONE', #40117, #2302 ) ;
#52363=CARTESIAN_POINT ( 'NONE',  ( -23.33771345073609638, -0.1191753592594197858, 5.846786880686956955 ) ) ;
#52364=ORIENTED_EDGE ( 'NONE', *, *, #13424, .T. ) ;
#52365=CARTESIAN_POINT ( 'NONE',  ( -9.285042292104602524, 0.000000000000000000, 3.270820500249148388 ) ) ;
#52366=ORIENTED_EDGE ( 'NONE', *, *, #23993, .F. ) ;
#52367=EDGE_CURVE ( 'NONE', #38901, #53603, #34610, .T. ) ;
#52368=ORIENTED_EDGE ( 'NONE', *, *, #37229, .T. ) ;
#52369=VECTOR ( 'NONE', #40178, 999.9999999999998863 ) ;
#52370=EDGE_LOOP ( 'NONE', ( #20426, #24100, #18269, #33590 ) ) ;
#52371=EDGE_CURVE ( 'NONE', #25320, #46187, #55942, .T. ) ;
#52372=ORIENTED_EDGE ( 'NONE', *, *, #27650, .F. ) ;
#52373=CARTESIAN_POINT ( 'NONE',  ( -20.54204810873173415, 0.000000000000000000, 4.860550213503115558 ) ) ;
#52374=EDGE_CURVE ( 'NONE', #53467, #54772, #20989, .T. ) ;
#52375=ORIENTED_EDGE ( 'NONE', *, *, #35667, .F. ) ;
#52376=LINE ( 'NONE', #35904, #23149 ) ;
#52377=AXIS2_PLACEMENT_3D ( 'NONE', #6708, #15489, #1867 ) ;
#52378=VERTEX_POINT ( 'NONE', #34354 ) ;
#52379=DIRECTION ( 'NONE',  ( 0.7660212471507180654, -0.6427876096865404731, 0.005961354470445141482 ) ) ;
#52381=EDGE_LOOP ( 'NONE', ( #41521, #33549, #23087, #4444 ) ) ;
#52382=DIRECTION ( 'NONE',  ( 0.5449076811759707706, 0.6444004775717708799, -0.5364919789714476250 ) ) ;
#52383=ORIENTED_EDGE ( 'NONE', *, *, #13298, .F. ) ;
#52384=CARTESIAN_POINT ( 'NONE',  ( -14.46888367232926420, 0.000000000000000000, 12.59025272694991315 ) ) ;
#52385=CARTESIAN_POINT ( 'NONE',  ( -13.68976073567942642, 0.000000000000000000, 6.191198521283176603 ) ) ;
#52386=CARTESIAN_POINT ( 'NONE',  ( -12.64114979503688474, -0.1191753592594185784, 3.714037593554236238 ) ) ;
#52387=CARTESIAN_POINT ( 'NONE',  ( -19.57250508090073993, -5.051250379848164940, 4.322785442357456098 ) ) ;
#52388=DIRECTION ( 'NONE',  ( 0.9999697198139515519, 0.000000000000000000, 0.007781995580013368816 ) ) ;
#52389=ORIENTED_EDGE ( 'NONE', *, *, #16425, .T. ) ;
#52390=ORIENTED_EDGE ( 'NONE', *, *, #13867, .T. ) ;
#52391=DIRECTION ( 'NONE',  ( 0.007781995580012663651, 0.000000000000000000, -0.9999697198139515519 ) ) ;
#52392=CARTESIAN_POINT ( 'NONE',  ( -20.29001881650349759, 0.1245042932765033361, 4.966986233812068718 ) ) ;
#52393=EDGE_CURVE ( 'NONE', #15287, #49949, #13048, .T. ) ;
#52395=CARTESIAN_POINT ( 'NONE',  ( -27.99845268667336384, -0.1191753592594197858, 7.657176279295684118 ) ) ;
#52396=LINE ( 'NONE', #4139, #1373 ) ;
#52397=CARTESIAN_POINT ( 'NONE',  ( -20.39447655573265195, -3.756034771668158356, 10.76813197985039139 ) ) ;
#52398=EDGE_LOOP ( 'NONE', ( #7114, #24966, #49021, #47679, #38696 ) ) ;
#52399=CARTESIAN_POINT ( 'NONE',  ( -13.07066190154808361, 0.000000000000000000, 12.04713590736729678 ) ) ;
#52400=EDGE_CURVE ( 'NONE', #53142, #26572, #47964, .T. ) ;
#52401=DIRECTION ( 'NONE',  ( -0.6427681459581293666, -0.7660444431189770143, -0.005002170337467561935 ) ) ;
#52402=EDGE_LOOP ( 'NONE', ( #21131, #2988, #52154, #26236 ) ) ;
#52403=LINE ( 'NONE', #52948, #11633 ) ;
#52404=LINE ( 'NONE', #34506, #46897 ) ;
#52405=EDGE_CURVE ( 'NONE', #40825, #52596, #43428, .T. ) ;
#52406=DIRECTION ( 'NONE',  ( 0.6427681459581294776, -0.7660444431189769032, 0.005002170337467562802 ) ) ;
#52407=EDGE_CURVE ( 'NONE', #54772, #17736, #51658, .T. ) ;
#52408=LINE ( 'NONE', #47280, #16880 ) ;
#52409=PLANE ( 'NONE',  #38318 ) ;
#52410=ORIENTED_EDGE ( 'NONE', *, *, #29248, .F. ) ;
#52411=ORIENTED_EDGE ( 'NONE', *, *, #8027, .F. ) ;
#52412=DIRECTION ( 'NONE',  ( -0.5364919789714478471, 0.6444004775717705469, -0.5449076811759709926 ) ) ;
#52413=DIRECTION ( 'NONE',  ( 0.007781995580012662783, 0.000000000000000000, -0.9999697198139514409 ) ) ;
#52414=CARTESIAN_POINT ( 'NONE',  ( -14.14864952550994559, 0.000000000000000000, 5.448963202999637545 ) ) ;
#52415=EDGE_CURVE ( 'NONE', #32585, #20350, #21832, .T. ) ;
#52416=AXIS2_PLACEMENT_3D ( 'NONE', #7200, #37028, #54895 ) ;
#52417=LINE ( 'NONE', #35368, #48212 ) ;
#52418=LINE ( 'NONE', #1270, #53865 ) ;
#52419=CARTESIAN_POINT ( 'NONE',  ( -10.43023669639197770, 0.000000000000000000, 5.308574737848737790 ) ) ;
#52420=PLANE ( 'NONE',  #2975 ) ;
#52421=ORIENTED_EDGE ( 'NONE', *, *, #40051, .F. ) ;
#52422=EDGE_CURVE ( 'NONE', #55415, #33685, #43682, .T. ) ;
#52423=CARTESIAN_POINT ( 'NONE',  ( -21.47419595591918906, 0.000000000000000000, 5.222628093224860102 ) ) ;
#52424=CARTESIAN_POINT ( 'NONE',  ( -15.86710544311044302, 0.000000000000000000, 13.13336954653252953 ) ) ;
#52425=ORIENTED_EDGE ( 'NONE', *, *, #11286, .F. ) ;
#52426=CARTESIAN_POINT ( 'NONE',  ( -14.94916102560700821, 0.000000000000000000, 2.688082935172642962 ) ) ;
#52427=VERTEX_POINT ( 'NONE', #47695 ) ;
#52428=FACE_OUTER_BOUND ( 'NONE', #33493, .T. ) ;
#52429=PLANE ( 'NONE',  #9394 ) ;
#52430=EDGE_LOOP ( 'NONE', ( #53871, #34605, #19520, #4657, #3638, #3716, #37549, #16775 ) ) ;
#52431=VERTEX_POINT ( 'NONE', #4798 ) ;
#52432=ORIENTED_EDGE ( 'NONE', *, *, #36293, .F. ) ;
#52433=ORIENTED_EDGE ( 'NONE', *, *, #25639, .F. ) ;
#52434=ORIENTED_EDGE ( 'NONE', *, *, #14530, .T. ) ;
#52435=VERTEX_POINT ( 'NONE', #38045 ) ;
#52436=PLANE ( 'NONE',  #30458 ) ;
#52437=CARTESIAN_POINT ( 'NONE',  ( -9.442067484779661513, -0.1191753592594197858, 10.59804618892231254 ) ) ;
#52438=LINE ( 'NONE', #5019, #23104 ) ;
#52439=ORIENTED_EDGE ( 'NONE', *, *, #53734, .F. ) ;
#52440=LINE ( 'NONE', #17814, #36750 ) ;
#52442=ORIENTED_EDGE ( 'NONE', *, *, #42442, .F. ) ;
#52443=ORIENTED_EDGE ( 'NONE', *, *, #20459, .F. ) ;
#52444=LINE ( 'NONE', #4733, #12957 ) ;
#52445=CARTESIAN_POINT ( 'NONE',  ( -20.08971041202067198, -0.1191753592594192862, 5.502731521554907523 ) ) ;
#52446=DIRECTION ( 'NONE',  ( 0.9999697198139515519, 0.000000000000000000, 0.007781995580013368816 ) ) ;
#52447=ORIENTED_EDGE ( 'NONE', *, *, #33931, .F. ) ;
#52448=DIRECTION ( 'NONE',  ( 0.005002170337468016433, -0.7660444431189770143, -0.6427681459581293666 ) ) ;
#52449=ORIENTED_EDGE ( 'NONE', *, *, #41783, .T. ) ;
#52450=EDGE_CURVE ( 'NONE', #52596, #21479, #52235, .T. ) ;
#52451=AXIS2_PLACEMENT_3D ( 'NONE', #18157, #26393, #51952 ) ;
#52452=FACE_OUTER_BOUND ( 'NONE', #33526, .T. ) ;
#52453=PLANE ( 'NONE',  #50185 ) ;
#52454=ADVANCED_FACE ( 'NONE', ( #17885 ), #49073, .F. ) ;
#52455=ADVANCED_FACE ( 'NONE', ( #26961 ), #36052, .F. ) ;
#52456=CARTESIAN_POINT ( 'NONE',  ( -11.22614204225105539, -2.298917212465658277, 4.815461341309315024 ) ) ;
#52457=DIRECTION ( 'NONE',  ( 0.9999697198139515519, 0.000000000000000000, 0.007781995580013368816 ) ) ;
#52458=LINE ( 'NONE', #26911, #53148 ) ;
#52459=DIRECTION ( 'NONE',  ( 0.9999697198139515519, 0.000000000000000000, 0.007781995580013368816 ) ) ;
#52460=PLANE ( 'NONE',  #53850 ) ;
#52461=LINE ( 'NONE', #48472, #55844 ) ;
#52462=ORIENTED_EDGE ( 'NONE', *, *, #53040, .F. ) ;
#52463=DIRECTION ( 'NONE',  ( 0.000000000000000000, -1.000000000000000000, 0.000000000000000000 ) ) ;
#52464=CARTESIAN_POINT ( 'NONE',  ( -18.85347906554464004, 0.000000000000000000, 9.105669829700502760 ) ) ;
#52465=PLANE ( 'NONE',  #40507 ) ;
#52466=EDGE_CURVE ( 'NONE', #41612, #38710, #44523, .T. ) ;
#52467=DIRECTION ( 'NONE',  ( 0.5364919789714477361, 0.6444004775717706579, 0.5449076811759711036 ) ) ;
#52468=DIRECTION ( 'NONE',  ( 0.000000000000000000, -1.000000000000000000, 0.000000000000000000 ) ) ;
#52469=CARTESIAN_POINT ( 'NONE',  ( -23.33849165029409889, 0.000000000000000000, 5.946783852668351855 ) ) ;
#52470=EDGE_CURVE ( 'NONE', #16632, #53347, #32040, .T. ) ;
#52471=CARTESIAN_POINT ( 'NONE',  ( -18.61957337711627858, 0.000000000000000000, 8.568832054460452596 ) ) ;
#52472=CARTESIAN_POINT ( 'NONE',  ( -16.99924723426068951, 0.000000000000000000, 13.49389102713827171 ) ) ;
#52473=ORIENTED_EDGE ( 'NONE', *, *, #46692, .T. ) ;
#52474=CARTESIAN_POINT ( 'NONE',  ( -11.32789590151604209, 0.000000000000000000, 1.238936178477310524 ) ) ;
#52475=DIRECTION ( 'NONE',  ( 0.000000000000000000, -1.000000000000000000, 0.000000000000000000 ) ) ;
#52476=LINE ( 'NONE', #21551, #44509 ) ;
#52477=EDGE_CURVE ( 'NONE', #31034, #40803, #31197, .T. ) ;
#52479=LINE ( 'NONE', #13576, #13989 ) ;
#52480=CARTESIAN_POINT ( 'NONE',  ( -17.83139810946674686, -0.1191753592594197858, 13.85674710641801788 ) ) ;
#52481=DIRECTION ( 'NONE',  ( 0.6427681459581294776, -0.7660444431189769032, 0.005002170337467562802 ) ) ;
#52482=EDGE_CURVE ( 'NONE', #14570, #48938, #27495, .T. ) ;
#52483=CARTESIAN_POINT ( 'NONE',  ( -14.46888367232926420, 0.000000000000000000, 12.59025272694991315 ) ) ;
#52484=CARTESIAN_POINT ( 'NONE',  ( -14.93495759592298988, 0.000000000000000000, 12.77129166681078409 ) ) ;
#52485=VECTOR ( 'NONE', #29906, 1000.000000000000114 ) ;
#52486=ORIENTED_EDGE ( 'NONE', *, *, #8109, .T. ) ;
#52487=EDGE_LOOP ( 'NONE', ( #55266, #30778, #26025, #9772 ) ) ;
#52488=VERTEX_POINT ( 'NONE', #10174 ) ;
#52489=ORIENTED_EDGE ( 'NONE', *, *, #9168, .T. ) ;
#52490=ORIENTED_EDGE ( 'NONE', *, *, #1503, .F. ) ;
#52491=CARTESIAN_POINT ( 'NONE',  ( -19.12962290826653700, 0.000000000000000000, 14.40064212555863854 ) ) ;
#52492=CARTESIAN_POINT ( 'NONE',  ( -27.99923088623136636, 0.000000000000000000, 7.757173251277078130 ) ) ;
#52493=ORIENTED_EDGE ( 'NONE', *, *, #44814, .T. ) ;
#52494=VERTEX_POINT ( 'NONE', #44274 ) ;
#52495=EDGE_CURVE ( 'NONE', #33688, #18589, #18718, .T. ) ;
#52496=EDGE_CURVE ( 'NONE', #44308, #34678, #22678, .T. ) ;
#52497=CARTESIAN_POINT ( 'NONE',  ( -12.13851405436063047, 0.000000000000000000, 11.68505802764555135 ) ) ;
#52498=ORIENTED_EDGE ( 'NONE', *, *, #46826, .F. ) ;
#52499=LINE ( 'NONE', #13594, #42726 ) ;
#52500=LINE ( 'NONE', #23259, #15968 ) ;
#52501=ORIENTED_EDGE ( 'NONE', *, *, #18186, .F. ) ;
#52502=CARTESIAN_POINT ( 'NONE',  ( -17.21548412696117225, 0.000000000000000000, 7.271756736028395451 ) ) ;
#52503=EDGE_CURVE ( 'NONE', #56039, #19075, #53610, .T. ) ;
#52504=EDGE_CURVE ( 'NONE', #308, #37252, #35751, .T. ) ;
#52505=EDGE_CURVE ( 'NONE', #6183, #31672, #52500, .T. ) ;
#52506=ORIENTED_EDGE ( 'NONE', *, *, #10844, .T. ) ;
#52507=FACE_OUTER_BOUND ( 'NONE', #26480, .T. ) ;
#52508=ADVANCED_FACE ( 'NONE', ( #40583 ), #5633, .F. ) ;
#52509=DIRECTION ( 'NONE',  ( 0.007781995580012663651, -3.146120232559066537E-19, -0.9999697198139514409 ) ) ;
#52510=DIRECTION ( 'NONE',  ( 0.005002170337468016433, -0.7660444431189770143, -0.6427681459581293666 ) ) ;
#52511=ORIENTED_EDGE ( 'NONE', *, *, #15279, .F. ) ;
#52512=DIRECTION ( 'NONE',  ( -0.6427681459581293666, -0.7660444431189770143, -0.005002170337467561935 ) ) ;
#52513=LINE ( 'NONE', #22973, #33813 ) ;
#52514=DIRECTION ( 'NONE',  ( -0.005961354470445682716, -0.6427876096865404731, 0.7660212471507180654 ) ) ;
#52515=ORIENTED_EDGE ( 'NONE', *, *, #38449, .F. ) ;
#52516=CARTESIAN_POINT ( 'NONE',  ( -21.24737399725141174, 5.143464774974014553, 4.771029900565397774 ) ) ;
#52517=ORIENTED_EDGE ( 'NONE', *, *, #5629, .T. ) ;
#52519=CARTESIAN_POINT ( 'NONE',  ( -22.40556560354864146, -0.1191753592594197858, 5.484709000965211523 ) ) ;
#52520=PLANE ( 'NONE',  #9683 ) ;
#52521=DIRECTION ( 'NONE',  ( 0.000000000000000000, -1.000000000000000000, 0.000000000000000000 ) ) ;
#52522=ADVANCED_FACE ( 'NONE', ( #27804 ), #14452, .F. ) ;
#52523=CARTESIAN_POINT ( 'NONE',  ( -10.47421230394850866, 0.000000000000000000, 10.95934586908605723 ) ) ;
#52524=DIRECTION ( 'NONE',  ( 0.6427681459581294776, -0.7660444431189769032, 0.005002170337467562802 ) ) ;
#52525=CARTESIAN_POINT ( 'NONE',  ( -7.370172463670563445, -9.191392189769848287, 6.081198852663857402 ) ) ;
#52526=DIRECTION ( 'NONE',  ( 0.000000000000000000, -1.000000000000000000, 0.000000000000000000 ) ) ;
#52527=EDGE_CURVE ( 'NONE', #37525, #18912, #31768, .T. ) ;
#52528=CARTESIAN_POINT ( 'NONE',  ( 2.072287782118878319, 0.000000000000000000, -2.950529333540147015 ) ) ;
#52530=ADVANCED_FACE ( 'NONE', ( #13595 ), #53356, .F. ) ;
#52531=CARTESIAN_POINT ( 'NONE',  ( -9.888614050034579606, -0.1191753592594203132, 7.059447091443916911 ) ) ;
#52532=ORIENTED_EDGE ( 'NONE', *, *, #16253, .F. ) ;
#52533=CARTESIAN_POINT ( 'NONE',  ( -20.54126990917373519, -0.1191753592594197858, 4.760553241521720658 ) ) ;
#52534=CARTESIAN_POINT ( 'NONE',  ( -10.37421533196711465, -0.1191753592594197858, 10.96012406864405975 ) ) ;
#52535=CARTESIAN_POINT ( 'NONE',  ( -14.83712142277997081, 4.172053068839012724, 2.312063226871277077 ) ) ;
#52536=EDGE_CURVE ( 'NONE', #50536, #3468, #48221, .T. ) ;
#52537=DIRECTION ( 'NONE',  ( -0.7660212471507179544, -0.6427876096865405842, -0.005961354470445141482 ) ) ;
#52538=FACE_OUTER_BOUND ( 'NONE', #45017, .T. ) ;
#52539=DIRECTION ( 'NONE',  ( 0.9999697198139515519, 0.000000000000000000, 0.007781995580013368816 ) ) ;
#52541=ORIENTED_EDGE ( 'NONE', *, *, #923, .T. ) ;
#52542=DIRECTION ( 'NONE',  ( 0.5449076811759707706, 0.6444004775717708799, -0.5364919789714476250 ) ) ;
#52543=FACE_OUTER_BOUND ( 'NONE', #18143, .T. ) ;
#52544=ORIENTED_EDGE ( 'NONE', *, *, #2792, .F. ) ;
#52545=PLANE ( 'NONE',  #45794 ) ;
#52546=EDGE_LOOP ( 'NONE', ( #1908, #28484, #24855, #40980 ) ) ;
#52547=LINE ( 'NONE', #35505, #48339 ) ;
#52548=ORIENTED_EDGE ( 'NONE', *, *, #10574, .F. ) ;
#52549=ORIENTED_EDGE ( 'NONE', *, *, #16299, .T. ) ;
#52550=EDGE_LOOP ( 'NONE', ( #40706, #14405, #22105, #799 ) ) ;
#52551=CARTESIAN_POINT ( 'NONE',  ( -17.36532418587302473, -0.1191753592594177458, 13.67570816655714516 ) ) ;
#52552=FACE_OUTER_BOUND ( 'NONE', #10655, .T. ) ;
#52553=CARTESIAN_POINT ( 'NONE',  ( -16.06709938707323460, 0.000000000000000000, 13.13181314741652628 ) ) ;
#52554=EDGE_CURVE ( 'NONE', #24619, #37122, #18131, .T. ) ;
#52556=LINE ( 'NONE', #44325, #31102 ) ;
#52557=EDGE_LOOP ( 'NONE', ( #45486, #36197, #8379 ) ) ;
#52558=EDGE_CURVE ( 'NONE', #34341, #24350, #43976, .T. ) ;
#52559=EDGE_LOOP ( 'NONE', ( #27159, #54, #37776, #45185 ) ) ;
#52560=CARTESIAN_POINT ( 'NONE',  ( -19.60834386242827776, 0.000000000000000000, 4.298478389818581213 ) ) ;
#52561=ORIENTED_EDGE ( 'NONE', *, *, #1849, .F. ) ;
#52562=LINE ( 'NONE', #13658, #38226 ) ;
#52563=ORIENTED_EDGE ( 'NONE', *, *, #34073, .F. ) ;
#52564=FACE_OUTER_BOUND ( 'NONE', #28628, .T. ) ;
#52565=DIRECTION ( 'NONE',  ( -0.9999697198139514409, -0.000000000000000000, -0.007781995580013368816 ) ) ;
#52566=EDGE_CURVE ( 'NONE', #34403, #30589, #37138, .T. ) ;
#52567=ADVANCED_FACE ( 'NONE', ( #23523 ), #32868, .F. ) ;
#52568=EDGE_CURVE ( 'NONE', #52618, #46492, #23786, .T. ) ;
#52569=VERTEX_POINT ( 'NONE', #37710 ) ;
#52570=PLANE ( 'NONE',  #5029 ) ;
#52571=ORIENTED_EDGE ( 'NONE', *, *, #34808, .F. ) ;
#52572=EDGE_CURVE ( 'NONE', #17790, #36664, #24353, .T. ) ;
#52573=CARTESIAN_POINT ( 'NONE',  ( -10.98261119617138526, -1.489407457353158160, 1.099820381026936023 ) ) ;
#52574=VERTEX_POINT ( 'NONE', #36881 ) ;
#52575=CARTESIAN_POINT ( 'NONE',  ( -20.58768131384620403, 5.467268677019013978, 4.504451819298203930 ) ) ;
#52576=CARTESIAN_POINT ( 'NONE',  ( -11.36238454357943084, 0.000000000000000000, 5.670652617570483223 ) ) ;
#52577=DIRECTION ( 'NONE',  ( 0.5449076811759707706, 0.6444004775717708799, -0.5364919789714476250 ) ) ;
#52578=ORIENTED_EDGE ( 'NONE', *, *, #7293, .F. ) ;
#52579=DIRECTION ( 'NONE',  ( 0.000000000000000000, -0.000000000000000000, -1.000000000000000000 ) ) ;
#52580=PLANE ( 'NONE',  #38299 ) ;
#52581=CARTESIAN_POINT ( 'NONE',  ( 2.072287782118878319, 0.000000000000000000, -2.950529333540147015 ) ) ;
#52582=LINE ( 'NONE', #22508, #44996 ) ;
#52583=LINE ( 'NONE', #13681, #5892 ) ;
#52584=DIRECTION ( 'NONE',  ( 0.000000000000000000, -1.000000000000000000, 0.000000000000000000 ) ) ;
#52585=ADVANCED_FACE ( 'NONE', ( #37399 ), #41115, .F. ) ;
#52586=VECTOR ( 'NONE', #30328, 1000.000000000000227 ) ;
#52587=( NAMED_UNIT ( * ) PLANE_ANGLE_UNIT ( ) SI_UNIT ( $, .RADIAN. ) );
#52588=ORIENTED_EDGE ( 'NONE', *, *, #22697, .T. ) ;
#52589=LINE ( 'NONE', #13685, #53387 ) ;
#52590=DIRECTION ( 'NONE',  ( 0.9999697198139515519, 0.000000000000000000, 0.007781995580013368816 ) ) ;
#52591=EDGE_CURVE ( 'NONE', #18181, #52283, #20370, .T. ) ;
#52592=DIRECTION ( 'NONE',  ( -0.005002170337468016433, -0.7660444431189770143, 0.6427681459581293666 ) ) ;
#52593=VERTEX_POINT ( 'NONE', #2203 ) ;
#52594=FACE_OUTER_BOUND ( 'NONE', #50098, .T. ) ;
#52595=CARTESIAN_POINT ( 'NONE',  ( -19.60990026154428278, 0.000000000000000000, 4.498472333781370125 ) ) ;
#52596=VERTEX_POINT ( 'NONE', #29161 ) ;
#52597=PLANE ( 'NONE',  #37974 ) ;
#52598=EDGE_CURVE ( 'NONE', #18918, #17751, #50747, .T. ) ;
#52599=CARTESIAN_POINT ( 'NONE',  ( -17.47449301425473323, -1.975113310420658852, 6.711115685826810839 ) ) ;
#52600=CARTESIAN_POINT ( 'NONE',  ( -11.79859221955444681, 1.095915999411503750, 3.262879877198777034 ) ) ;
#52601=EDGE_CURVE ( 'NONE', #7109, #43104, #10754, .T. ) ;
#52602=DIRECTION ( 'NONE',  ( -0.005002170337468016433, -0.7660444431189770143, 0.6427681459581293666 ) ) ;
#52603=ORIENTED_EDGE ( 'NONE', *, *, #21089, .F. ) ;
#52604=VERTEX_POINT ( 'NONE', #28625 ) ;
#52605=DIRECTION ( 'NONE',  ( 0.000000000000000000, -1.000000000000000000, 0.000000000000000000 ) ) ;
#52606=FACE_OUTER_BOUND ( 'NONE', #6883, .T. ) ;
#52608=CARTESIAN_POINT ( 'NONE',  ( -17.30188903097415576, -0.1191753592594164690, 5.524426992162961625 ) ) ;
#52609=DIRECTION ( 'NONE',  ( 0.9999697198139515519, 0.000000000000000000, 0.007781995580013368816 ) ) ;
#52610=LINE ( 'NONE', #30774, #31254 ) ;
#52611=ORIENTED_EDGE ( 'NONE', *, *, #20974, .T. ) ;
#52612=CARTESIAN_POINT ( 'NONE',  ( -25.20123094555300369, 0.000000000000000000, 6.470945668149052032 ) ) ;
#52614=ORIENTED_EDGE ( 'NONE', *, *, #5545, .T. ) ;
#52615=CARTESIAN_POINT ( 'NONE',  ( -10.74029228357944987, 0.000000000000000000, 11.14194120806293320 ) ) ;
#52616=DIRECTION ( 'NONE',  ( -0.6427681459581293666, -0.7660444431189770143, -0.005002170337467561935 ) ) ;
#52617=LINE ( 'NONE', #9768, #5756 ) ;
#52618=VERTEX_POINT ( 'NONE', #28061 ) ;
#52619=DIRECTION ( 'NONE',  ( 0.7660212471507180654, -0.6427876096865404731, 0.005961354470445141482 ) ) ;
#52621=VECTOR ( 'NONE', #35664, 1000.000000000000227 ) ;
#52622=EDGE_LOOP ( 'NONE', ( #8036, #4876, #23014, #16311 ) ) ;
#52623=ORIENTED_EDGE ( 'NONE', *, *, #15966, .T. ) ;
#52624=ORIENTED_EDGE ( 'NONE', *, *, #33762, .F. ) ;
#52625=DIRECTION ( 'NONE',  ( 0.005961354470445682716, -0.6427876096865404731, -0.7660212471507180654 ) ) ;
#52626=ORIENTED_EDGE ( 'NONE', *, *, #46747, .T. ) ;
#52627=CARTESIAN_POINT ( 'NONE',  ( -17.30476308447943978, -0.1191753592594171213, 5.893736695420727756 ) ) ;
#52628=EDGE_CURVE ( 'NONE', #41034, #36178, #50489, .T. ) ;
#52629=ORIENTED_EDGE ( 'NONE', *, *, #23206, .T. ) ;
#52630=DIRECTION ( 'NONE',  ( -0.5449076811759708816, 0.6444004775717707689, 0.5364919789714475140 ) ) ;
#52631=ORIENTED_EDGE ( 'NONE', *, *, #46164, .T. ) ;
#52632=DIRECTION ( 'NONE',  ( -0.005961354470445682716, -0.6427876096865404731, 0.7660212471507180654 ) ) ;
#52633=ORIENTED_EDGE ( 'NONE', *, *, #6960, .F. ) ;
#52634=EDGE_CURVE ( 'NONE', #10990, #40728, #15286, .T. ) ;
#52635=EDGE_CURVE ( 'NONE', #21963, #32592, #32598, .T. ) ;
#52636=CARTESIAN_POINT ( 'NONE',  ( -21.47341775636118655, -0.1191753592594197858, 5.122631121243466090 ) ) ;
#52637=DIRECTION ( 'NONE',  ( -0.7660212471507179544, -0.6427876096865405842, -0.005961354470445141482 ) ) ;
#52638=DIRECTION ( 'NONE',  ( 0.9999697198139515519, 0.000000000000000000, 0.007781995580013368816 ) ) ;
#52639=LINE ( 'NONE', #27949, #13015 ) ;
#52640=DIRECTION ( 'NONE',  ( -0.2426528472758541499, 0.7422098413412800966, -0.6246952433987894571 ) ) ;
#52641=DIRECTION ( 'NONE',  ( 0.005002170337468016433, -0.7660444431189770143, -0.6427681459581293666 ) ) ;
#52643=ORIENTED_EDGE ( 'NONE', *, *, #40743, .F. ) ;
#52644=DIRECTION ( 'NONE',  ( 0.000000000000000000, -1.000000000000000000, 0.000000000000000000 ) ) ;
#52645=DIRECTION ( 'NONE',  ( 0.000000000000000000, -0.000000000000000000, -1.000000000000000000 ) ) ;
#52646=LINE ( 'NONE', #44689, #7957 ) ;
#52647=LINE ( 'NONE', #43857, #16726 ) ;
#52648=VERTEX_POINT ( 'NONE', #3038 ) ;
#52649=CARTESIAN_POINT ( 'NONE',  ( -12.26710951010334405, 0.000000000000000000, 2.508949224009560108 ) ) ;
#52650=LINE ( 'NONE', #43575, #48635 ) ;
#52651=ORIENTED_EDGE ( 'NONE', *, *, #50465, .F. ) ;
#52652=DIRECTION ( 'NONE',  ( 0.000000000000000000, -0.000000000000000000, -1.000000000000000000 ) ) ;
#52653=CARTESIAN_POINT ( 'NONE',  ( -16.33317936670417225, 0.000000000000000000, 13.31440848639340224 ) ) ;
#52654=EDGE_LOOP ( 'NONE', ( #54336, #9482, #9120, #22549 ) ) ;
#52657=VECTOR ( 'NONE', #41731, 1000.000000000000114 ) ;
#52658=CARTESIAN_POINT ( 'NONE',  ( -10.27421835998572064, 0.000000000000000000, 10.96090226820206048 ) ) ;
#52659=EDGE_CURVE ( 'NONE', #394, #29284, #45643, .T. ) ;
#52660=DIRECTION ( 'NONE',  ( 0.000000000000000000, -0.000000000000000000, -1.000000000000000000 ) ) ;
#52661=VECTOR ( 'NONE', #39183, 999.9999999999998863 ) ;
#52662=CARTESIAN_POINT ( 'NONE',  ( -32.47108885958310509, -1.000000000000000000, 15.83124721154520387 ) ) ;
#52663=ORIENTED_EDGE ( 'NONE', *, *, #1512, .T. ) ;
#52664=ADVANCED_FACE ( 'NONE', ( #7304 ), #6220, .F. ) ;
#52665=VERTEX_POINT ( 'NONE', #33443 ) ;
#52666=FACE_OUTER_BOUND ( 'NONE', #35528, .T. ) ;
#52667=CARTESIAN_POINT ( 'NONE',  ( -16.06709938707323460, 0.000000000000000000, 13.13181314741652628 ) ) ;
#52668=PLANE ( 'NONE',  #14319 ) ;
#52669=FACE_OUTER_BOUND ( 'NONE', #38461, .T. ) ;
#52670=EDGE_CURVE ( 'NONE', #39202, #27276, #1913, .T. ) ;
#52672=ORIENTED_EDGE ( 'NONE', *, *, #38642, .T. ) ;
#52673=CARTESIAN_POINT ( 'NONE',  ( -16.79925329029790149, 0.000000000000000000, 13.49544742625427496 ) ) ;
#52674=CARTESIAN_POINT ( 'NONE',  ( -21.47341775636118655, -0.1191753592594197858, 5.122631121243466090 ) ) ;
#52675=DIRECTION ( 'NONE',  ( -0.005961354470445682716, -0.6427876096865404731, 0.7660212471507180654 ) ) ;
#52676=CARTESIAN_POINT ( 'NONE',  ( -12.15116108492864377, 0.000000000000000000, 1.401855352044617975 ) ) ;
#52677=ORIENTED_EDGE ( 'NONE', *, *, #48812, .F. ) ;
#52678=CARTESIAN_POINT ( 'NONE',  ( -15.50810134761786507, -2.946525016555658905, 7.541554487265736739 ) ) ;
#52679=VERTEX_POINT ( 'NONE', #45367 ) ;
#52680=LINE ( 'NONE', #43604, #52218 ) ;
#52681=CARTESIAN_POINT ( 'NONE',  ( 2.072287782118878319, 0.000000000000000000, -2.950529333540147015 ) ) ;
#52682=ORIENTED_EDGE ( 'NONE', *, *, #28692, .T. ) ;
#52683=VECTOR ( 'NONE', #35788, 1000.000000000000227 ) ;
#52684=VECTOR ( 'NONE', #39216, 999.9999999999998863 ) ;
#52685=LINE ( 'NONE', #13788, #15411 ) ;
#52686=VERTEX_POINT ( 'NONE', #41410 ) ;
#52687=EDGE_LOOP ( 'NONE', ( #3941, #18034, #43552, #23324 ) ) ;
#52688=ORIENTED_EDGE ( 'NONE', *, *, #44745, .F. ) ;
#52689=CARTESIAN_POINT ( 'NONE',  ( -25.20278734466900517, 0.000000000000000000, 6.670939612111840944 ) ) ;
#52690=ORIENTED_EDGE ( 'NONE', *, *, #46363, .F. ) ;
#52691=ORIENTED_EDGE ( 'NONE', *, *, #30894, .F. ) ;
#52692=DIRECTION ( 'NONE',  ( 0.9999697198139515519, 0.000000000000000000, 0.007781995580013368816 ) ) ;
#52693=ADVANCED_FACE ( 'NONE', ( #2497 ), #19817, .F. ) ;
#52694=DIRECTION ( 'NONE',  ( 0.007781995580012662783, 0.000000000000000000, -0.9999697198139514409 ) ) ;
#52695=VERTEX_POINT ( 'NONE', #52163 ) ;
#52696=ADVANCED_FACE ( 'NONE', ( #34550 ), #168, .F. ) ;
#52697=VECTOR ( 'NONE', #9340, 1000.000000000000000 ) ;
#52698=EDGE_LOOP ( 'NONE', ( #6911, #9264, #53068, #35311 ) ) ;
#52699=CARTESIAN_POINT ( 'NONE',  ( -16.85908992509638082, 5.467268677019013090, 3.056140300411222643 ) ) ;
#52700=VERTEX_POINT ( 'NONE', #34008 ) ;
#52701=ORIENTED_EDGE ( 'NONE', *, *, #38472, .F. ) ;
#52702=ADVANCED_FACE ( 'NONE', ( #3614 ), #51332, .F. ) ;
#52703=VECTOR ( 'NONE', #37433, 999.9999999999998863 ) ;
#52704=PLANE ( 'NONE',  #25769 ) ;
#52705=DIRECTION ( 'NONE',  ( -0.5449076811759708816, 0.6444004775717707689, 0.5364919789714475140 ) ) ;
#52706=DIRECTION ( 'NONE',  ( -0.6246952433987894571, 0.7422098413412802076, 0.2426528472758539834 ) ) ;
#52707=VERTEX_POINT ( 'NONE', #21520 ) ;
#52708=LINE ( 'NONE', #22368, #37368 ) ;
#52709=EDGE_LOOP ( 'NONE', ( #18180, #36731, #5320, #55637 ) ) ;
#52710=CARTESIAN_POINT ( 'NONE',  ( -16.79056226515798045, -2.298917212465660054, 3.329998215632909986 ) ) ;
#52712=CARTESIAN_POINT ( 'NONE',  ( -15.07792331919211293, 0.000000000000000000, 5.441731379463618623 ) ) ;
#52713=DIRECTION ( 'NONE',  ( -0.6427681459581293666, -0.7660444431189770143, -0.005002170337467561935 ) ) ;
#52714=CARTESIAN_POINT ( 'NONE',  ( -14.87792937522932668, 0.000000000000000000, 5.443287778579622760 ) ) ;
#52715=CARTESIAN_POINT ( 'NONE',  ( -13.60775715277214637, -0.1191753592594198830, 8.504088575178599285 ) ) ;
#52716=DIRECTION ( 'NONE',  ( -0.7660212471507179544, -0.6427876096865405842, -0.005961354470445141482 ) ) ;
#52717=CARTESIAN_POINT ( 'NONE',  ( -23.33771345073609638, -0.1191753592594197858, 5.846786880686956955 ) ) ;
#52718=ORIENTED_EDGE ( 'NONE', *, *, #25034, .T. ) ;
#52719=CARTESIAN_POINT ( 'NONE',  ( -14.20280369269832832, 0.000000000000000000, 12.40765738797303719 ) ) ;
#52721=VECTOR ( 'NONE', #1888, 1000.000000000000227 ) ;
#52722=AXIS2_PLACEMENT_3D ( 'NONE', #3678, #13349, #56205 ) ;
#52723=CARTESIAN_POINT ( 'NONE',  ( -9.442067484779661513, -0.1191753592594197858, 10.59804618892231254 ) ) ;
#52724=PLANE ( 'NONE',  #12415 ) ;
#52725=CARTESIAN_POINT ( 'NONE',  ( -4.546219555552018399, 7.433331870878916448, -1.452467510021419717 ) ) ;
#52727=DIRECTION ( 'NONE',  ( 0.005002170337468016433, -0.7660444431189770143, -0.6427681459581293666 ) ) ;
#52728=LINE ( 'NONE', #26927, #38643 ) ;
#52729=FACE_OUTER_BOUND ( 'NONE', #14648, .T. ) ;
#52730=VECTOR ( 'NONE', #14079, 999.9999999999998863 ) ;
#52731=VERTEX_POINT ( 'NONE', #16673 ) ;
#52732=CARTESIAN_POINT ( 'NONE',  ( -19.05546973890454154, 0.000000000000000000, 4.872119110114796925 ) ) ;
#52733=FACE_OUTER_BOUND ( 'NONE', #48592, .T. ) ;
#52734=DIRECTION ( 'NONE',  ( 0.000000000000000000, -1.000000000000000000, 0.000000000000000000 ) ) ;
#52735=DIRECTION ( 'NONE',  ( 0.9999697198139515519, 0.000000000000000000, 0.007781995580013368816 ) ) ;
#52736=EDGE_CURVE ( 'NONE', #52707, #32780, #47627, .T. ) ;
#52737=CARTESIAN_POINT ( 'NONE',  ( -11.13784177245837981, 0.000000000000000000, 2.517737446661582723 ) ) ;
#52738=DIRECTION ( 'NONE',  ( 0.007781995580012663651, -3.146120232559066537E-19, -0.9999697198139514409 ) ) ;
#52739=DIRECTION ( 'NONE',  ( -0.5449076811759708816, 0.6444004775717707689, 0.5364919789714475140 ) ) ;
#52741=DIRECTION ( 'NONE',  ( 0.007781995580012663651, 0.000000000000000000, -0.9999697198139515519 ) ) ;
#52742=LINE ( 'NONE', #52484, #3844 ) ;
#52743=EDGE_CURVE ( 'NONE', #27886, #34394, #29763, .T. ) ;
#52744=VERTEX_POINT ( 'NONE', #8164 ) ;
#52745=ADVANCED_FACE ( 'NONE', ( #55874 ), #47326, .F. ) ;
#52746=ADVANCED_FACE ( 'NONE', ( #55567 ), #4470, .F. ) ;
#52747=ORIENTED_EDGE ( 'NONE', *, *, #31239, .F. ) ;
#52749=EDGE_LOOP ( 'NONE', ( #45307, #15480, #2484, #24961 ) ) ;
#52751=DIRECTION ( 'NONE',  ( 0.000000000000000000, -0.000000000000000000, -1.000000000000000000 ) ) ;
#52752=EDGE_CURVE ( 'NONE', #1154, #54036, #8746, .T. ) ;
#52753=DIRECTION ( 'NONE',  ( 0.000000000000000000, -0.000000000000000000, -1.000000000000000000 ) ) ;
#52754=VECTOR ( 'NONE', #26780, 999.9999999999998863 ) ;
#52756=ORIENTED_EDGE ( 'NONE', *, *, #37201, .T. ) ;
#52758=ORIENTED_EDGE ( 'NONE', *, *, #16667, .T. ) ;
#52759=ADVANCED_FACE ( 'NONE', ( #34296 ), #30307, .T. ) ;
#52760=VECTOR ( 'NONE', #25291, 1000.000000000000227 ) ;
#52761=DIRECTION ( 'NONE',  ( 0.9999697198139515519, 0.000000000000000000, 0.007781995580013368816 ) ) ;
#52762=ORIENTED_EDGE ( 'NONE', *, *, #23913, .T. ) ;
#52763=LINE ( 'NONE', #44818, #28261 ) ;
#52764=DIRECTION ( 'NONE',  ( 0.007781995580012663651, -3.146120232559066537E-19, -0.9999697198139514409 ) ) ;
#52765=VERTEX_POINT ( 'NONE', #42245 ) ;
#52766=DIRECTION ( 'NONE',  ( -0.6427681459581293666, -0.7660444431189770143, -0.005002170337467561935 ) ) ;
#52767=EDGE_CURVE ( 'NONE', #53756, #38710, #26063, .T. ) ;
#52768=ORIENTED_EDGE ( 'NONE', *, *, #3204, .F. ) ;
#52769=DIRECTION ( 'NONE',  ( 0.007781995580012663651, 0.000000000000000000, -0.9999697198139515519 ) ) ;
#52770=VECTOR ( 'NONE', #32346, 999.9999999999998863 ) ;
#52771=CARTESIAN_POINT ( 'NONE',  ( -24.27063949748155380, 0.000000000000000000, 6.308861732390097288 ) ) ;
#52772=VECTOR ( 'NONE', #23399, 999.9999999999998863 ) ;
#52774=LINE ( 'NONE', #44533, #28218 ) ;
#52775=DIRECTION ( 'NONE',  ( 0.9999697198139515519, 0.000000000000000000, 0.007781995580013368816 ) ) ;
#52776=ORIENTED_EDGE ( 'NONE', *, *, #9372, .F. ) ;
#52777=DIRECTION ( 'NONE',  ( -0.7660212471507179544, -0.6427876096865405842, -0.005961354470445141482 ) ) ;
#52778=LINE ( 'NONE', #14461, #22022 ) ;
#52779=CARTESIAN_POINT ( 'NONE',  ( -19.78282706061121132, 0.000000000000000000, 6.713118996285826867 ) ) ;
#52780=EDGE_LOOP ( 'NONE', ( #29483, #39511, #28684, #52443 ) ) ;
#52781=CARTESIAN_POINT ( 'NONE',  ( -11.24436505100834260, -0.1191753592594186895, 3.355575625600500711 ) ) ;
#52782=VERTEX_POINT ( 'NONE', #30857 ) ;
#52783=DIRECTION ( 'NONE',  ( -0.6427681459581293666, -0.7660444431189770143, -0.005002170337467561935 ) ) ;
#52784=CARTESIAN_POINT ( 'NONE',  ( -14.00280974873554030, 0.000000000000000000, 12.40921378708904044 ) ) ;
#52785=FACE_OUTER_BOUND ( 'NONE', #30782, .T. ) ;
#52786=CARTESIAN_POINT ( 'NONE',  ( -14.88942558925045745, 0.000000000000000000, 6.920526591610678402 ) ) ;
#52787=VECTOR ( 'NONE', #15193, 1000.000000000000227 ) ;
#52788=DIRECTION ( 'NONE',  ( 0.007781995580012663651, 0.000000000000000000, -0.9999697198139515519 ) ) ;
#52789=CARTESIAN_POINT ( 'NONE',  ( 2.072287782118878319, 0.000000000000000000, -2.950529333540147015 ) ) ;
#52790=DIRECTION ( 'NONE',  ( 0.7660212471507180654, -0.6427876096865404731, 0.005961354470445141482 ) ) ;
#52791=PLANE ( 'NONE',  #29295 ) ;
#52793=ORIENTED_EDGE ( 'NONE', *, *, #23438, .F. ) ;
#52795=DIRECTION ( 'NONE',  ( 0.007781995580012663651, -3.146120232559066537E-19, -0.9999697198139514409 ) ) ;
#52796=FACE_OUTER_BOUND ( 'NONE', #15767, .T. ) ;
#52797=DIRECTION ( 'NONE',  ( 0.005961354470445682716, -0.6427876096865404731, -0.7660212471507180654 ) ) ;
#52798=LINE ( 'NONE', #48562, #52252 ) ;
#52800=VECTOR ( 'NONE', #41678, 1000.000000000000000 ) ;
#52801=CARTESIAN_POINT ( 'NONE',  ( -17.74560456716937296, 0.000000000000000000, 3.774316574337878372 ) ) ;
#52802=EDGE_CURVE ( 'NONE', #3819, #43814, #18079, .T. ) ;
#52803=DIRECTION ( 'NONE',  ( 0.000000000000000000, -1.000000000000000000, 0.000000000000000000 ) ) ;
#52804=DIRECTION ( 'NONE',  ( 0.007781995580012662783, 0.000000000000000000, -0.9999697198139514409 ) ) ;
#52805=ORIENTED_EDGE ( 'NONE', *, *, #3756, .T. ) ;
#52806=VECTOR ( 'NONE', #7878, 999.9999999999998863 ) ;
#52807=VECTOR ( 'NONE', #55367, 999.9999999999998863 ) ;
#52808=VERTEX_POINT ( 'NONE', #53004 ) ;
#52809=DIRECTION ( 'NONE',  ( -0.5364919789714478471, 0.6444004775717705469, -0.5449076811759709926 ) ) ;
#52811=EDGE_CURVE ( 'NONE', #49206, #24901, #22057, .T. ) ;
#52812=ORIENTED_EDGE ( 'NONE', *, *, #45451, .F. ) ;
#52813=CARTESIAN_POINT ( 'NONE',  ( -27.99767448711536133, 0.000000000000000000, 7.557179307314289218 ) ) ;
#52814=VECTOR ( 'NONE', #38470, 1000.000000000000227 ) ;
#52815=ORIENTED_EDGE ( 'NONE', *, *, #12276, .F. ) ;
#52816=LINE ( 'NONE', #18464, #33833 ) ;
#52817=EDGE_CURVE ( 'NONE', #40480, #2840, #14119, .T. ) ;
#52818=ORIENTED_EDGE ( 'NONE', *, *, #43235, .F. ) ;
#52819=ORIENTED_EDGE ( 'NONE', *, *, #26882, .F. ) ;
#52820=ORIENTED_EDGE ( 'NONE', *, *, #38781, .T. ) ;
#52821=LINE ( 'NONE', #40340, #5766 ) ;
#52822=CARTESIAN_POINT ( 'NONE',  ( 2.072287782118878319, 0.000000000000000000, -2.950529333540147015 ) ) ;
#52823=CARTESIAN_POINT ( 'NONE',  ( -13.29462968114988897, -0.3560938001956550081, 2.430427978987968807 ) ) ;
#52824=LINE ( 'NONE', #22738, #6620 ) ;
#52825=ADVANCED_FACE ( 'NONE', ( #31446 ), #5575, .F. ) ;
#52826=ORIENTED_EDGE ( 'NONE', *, *, #44914, .T. ) ;
#52827=ORIENTED_EDGE ( 'NONE', *, *, #19636, .T. ) ;
#52828=VECTOR ( 'NONE', #15436, 999.9999999999998863 ) ;
#52829=EDGE_CURVE ( 'NONE', #10480, #29513, #48761, .T. ) ;
#52830=CARTESIAN_POINT ( 'NONE',  ( -28.93137873341882127, 0.000000000000000000, 8.119251130998824451 ) ) ;
#52831=ORIENTED_EDGE ( 'NONE', *, *, #10544, .F. ) ;
#52832=AXIS2_PLACEMENT_3D ( 'NONE', #34460, #38744, #11757 ) ;
#52833=DIRECTION ( 'NONE',  ( -0.005002170337468016433, -0.7660444431189770143, 0.6427681459581293666 ) ) ;
#52834=VERTEX_POINT ( 'NONE', #53306 ) ;
#52836=FACE_OUTER_BOUND ( 'NONE', #21027, .T. ) ;
#52837=VECTOR ( 'NONE', #55003, 1000.000000000000227 ) ;
#52838=ADVANCED_FACE ( 'NONE', ( #23198 ), #40528, .F. ) ;
#52839=AXIS2_PLACEMENT_3D ( 'NONE', #54983, #15247, #16078 ) ;
#52840=VERTEX_POINT ( 'NONE', #14402 ) ;
#52841=CARTESIAN_POINT ( 'NONE',  ( -13.73672976910459909, 0.000000000000000000, 12.22661844811216270 ) ) ;
#52842=ORIENTED_EDGE ( 'NONE', *, *, #528, .F. ) ;
#52843=EDGE_CURVE ( 'NONE', #15160, #26242, #9269, .T. ) ;
#52844=VECTOR ( 'NONE', #34214, 1000.000000000000227 ) ;
#52845=DIRECTION ( 'NONE',  ( 0.000000000000000000, -0.000000000000000000, -1.000000000000000000 ) ) ;
#52846=VECTOR ( 'NONE', #5334, 999.9999999999998863 ) ;
#52847=VERTEX_POINT ( 'NONE', #44470 ) ;
#52848=CARTESIAN_POINT ( 'NONE',  ( -11.83983530883092961, 0.000000000000000000, 7.313591278128507511 ) ) ;
#52849=LINE ( 'NONE', #44602, #36598 ) ;
#52850=CARTESIAN_POINT ( 'NONE',  ( -11.40636015113596180, 0.000000000000000000, 11.32142374880780089 ) ) ;
#52852=CARTESIAN_POINT ( 'NONE',  ( -12.28016212324047807, 0.000000000000000000, 4.186181981003405994 ) ) ;
#52853=LINE ( 'NONE', #31842, #44616 ) ;
#52854=LINE ( 'NONE', #13962, #43033 ) ;
#52855=VECTOR ( 'NONE', #2508, 1000.000000000000227 ) ;
#52856=DIRECTION ( 'NONE',  ( 0.000000000000000000, -1.000000000000000000, 0.000000000000000000 ) ) ;
#52857=AXIS2_PLACEMENT_3D ( 'NONE', #23714, #9561, #53296 ) ;
#52858=FACE_OUTER_BOUND ( 'NONE', #35901, .T. ) ;
#52859=CARTESIAN_POINT ( 'NONE',  ( -17.20111385943475923, 0.000000000000000000, 5.425208219739572790 ) ) ;
#52860=LINE ( 'NONE', #47797, #39437 ) ;
#52861=ORIENTED_EDGE ( 'NONE', *, *, #7629, .T. ) ;
#52862=FACE_OUTER_BOUND ( 'NONE', #13869, .T. ) ;
#52863=LINE ( 'NONE', #902, #29526 ) ;
#52864=LINE ( 'NONE', #43784, #5150 ) ;
#52865=ORIENTED_EDGE ( 'NONE', *, *, #43402, .F. ) ;
#52866=CARTESIAN_POINT ( 'NONE',  ( -18.78942900545214201, -0.04243879960735808671, 9.270562878879108126 ) ) ;
#52867=LINE ( 'NONE', #21930, #24527 ) ;
#52869=EDGE_CURVE ( 'NONE', #31317, #16382, #39388, .T. ) ;
#52870=VECTOR ( 'NONE', #39870, 999.9999999999998863 ) ;
#52872=LINE ( 'NONE', #35863, #54750 ) ;
#52873=EDGE_CURVE ( 'NONE', #32323, #9930, #13544, .T. ) ;
#52874=VECTOR ( 'NONE', #25306, 1000.000000000000227 ) ;
#52875=DIRECTION ( 'NONE',  ( 0.007781995580012663651, 0.000000000000000000, -0.9999697198139515519 ) ) ;
#52876=CARTESIAN_POINT ( 'NONE',  ( -7.883669827136422725, -9.688797144239941872, 6.280658667077863022 ) ) ;
#52877=ORIENTED_EDGE ( 'NONE', *, *, #42575, .T. ) ;
#52878=ORIENTED_EDGE ( 'NONE', *, *, #48145, .F. ) ;
#52879=ADVANCED_FACE ( 'NONE', ( #17822 ), #43626, .F. ) ;
#52880=DIRECTION ( 'NONE',  ( -0.005961354470445682716, -0.6427876096865404731, 0.7660212471507180654 ) ) ;
#52881=LINE ( 'NONE', #13993, #18678 ) ;
#52882=VECTOR ( 'NONE', #44032, 999.9999999999998863 ) ;
#52884=EDGE_CURVE ( 'NONE', #37965, #32796, #40223, .T. ) ;
#52885=ADVANCED_FACE ( 'NONE', ( #22628 ), #10118, .F. ) ;
#52886=EDGE_CURVE ( 'NONE', #2632, #14570, #30607, .T. ) ;
#52887=VECTOR ( 'NONE', #17959, 1000.000000000000227 ) ;
#52888=FACE_OUTER_BOUND ( 'NONE', #28260, .T. ) ;
#52890=CARTESIAN_POINT ( 'NONE',  ( -17.70012898643225085, -2.784623065533160524, 8.127303779802742767 ) ) ;
#52891=DIRECTION ( 'NONE',  ( 0.000000000000000000, -0.000000000000000000, -1.000000000000000000 ) ) ;
#52892=ORIENTED_EDGE ( 'NONE', *, *, #5092, .T. ) ;
#52893=CARTESIAN_POINT ( 'NONE',  ( -32.65919192261063841, -0.1191753592594197858, 9.467565677904410393 ) ) ;
#52894=AXIS2_PLACEMENT_3D ( 'NONE', #37834, #50603, #41773 ) ;
#52895=CARTESIAN_POINT ( 'NONE',  ( -13.53673582514181106, 0.000000000000000000, 12.22817484722816772 ) ) ;
#52896=AXIS2_PLACEMENT_3D ( 'NONE', #10839, #3439, #15369 ) ;
#52897=ORIENTED_EDGE ( 'NONE', *, *, #5747, .F. ) ;
#52898=FACE_OUTER_BOUND ( 'NONE', #19591, .T. ) ;
#52899=FACE_OUTER_BOUND ( 'NONE', #12899, .T. ) ;
#52900=LINE ( 'NONE', #31337, #22975 ) ;
#52901=ORIENTED_EDGE ( 'NONE', *, *, #47021, .T. ) ;
#52902=DIRECTION ( 'NONE',  ( -0.6427681459581293666, -0.7660444431189770143, -0.005002170337467561935 ) ) ;
#52903=EDGE_CURVE ( 'NONE', #54093, #47959, #43912, .T. ) ;
#52904=ORIENTED_EDGE ( 'NONE', *, *, #53113, .F. ) ;
#52905=EDGE_CURVE ( 'NONE', #48904, #17751, #44219, .T. ) ;
#52906=EDGE_CURVE ( 'NONE', #25423, #52707, #41049, .T. ) ;
#52907=VERTEX_POINT ( 'NONE', #2971 ) ;
#52908=ORIENTED_EDGE ( 'NONE', *, *, #12822, .T. ) ;
#52909=EDGE_CURVE ( 'NONE', #16557, #11724, #2438, .T. ) ;
#52910=VERTEX_POINT ( 'NONE', #6170 ) ;
#52912=ORIENTED_EDGE ( 'NONE', *, *, #25465, .F. ) ;
#52913=VECTOR ( 'NONE', #10420, 1000.000000000000227 ) ;
#52914=CARTESIAN_POINT ( 'NONE',  ( -18.29747203306047609, -0.1191753592594177458, 14.03778604627889059 ) ) ;
#52915=DIRECTION ( 'NONE',  ( 0.7660212471507180654, -0.6427876096865404731, 0.005961354470445141482 ) ) ;
#52916=EDGE_CURVE ( 'NONE', #32990, #2010, #6422, .T. ) ;
#52917=EDGE_LOOP ( 'NONE', ( #27722, #6277, #7674, #44694 ) ) ;
#52918=CARTESIAN_POINT ( 'NONE',  ( -23.33771345073609638, -0.1191753592594197858, 5.846786880686956955 ) ) ;
#52919=ORIENTED_EDGE ( 'NONE', *, *, #16304, .F. ) ;
#52920=DIRECTION ( 'NONE',  ( 0.5364919789714477361, 0.6444004775717706579, 0.5449076811759711036 ) ) ;
#52921=AXIS2_PLACEMENT_3D ( 'NONE', #17333, #39504, #55986 ) ;
#52922=ORIENTED_EDGE ( 'NONE', *, *, #48425, .F. ) ;
#52923=EDGE_CURVE ( 'NONE', #21379, #6407, #37339, .T. ) ;
#52924=DIRECTION ( 'NONE',  ( -0.005002170337468016433, -0.7660444431189770143, 0.6427681459581293666 ) ) ;
#52925=CARTESIAN_POINT ( 'NONE',  ( -17.74404816805336793, 0.000000000000000000, 3.574322630375089460 ) ) ;
#52926=CARTESIAN_POINT ( 'NONE',  ( -14.88337611868230326, -0.03228989815065527041, 2.661499626451061751 ) ) ;
#52927=CARTESIAN_POINT ( 'NONE',  ( -17.40841230952411323, 0.000000000000000000, 6.362265171101888939 ) ) ;
#52928=DIRECTION ( 'NONE',  ( 0.007781995580012663651, -3.146120232559066537E-19, -0.9999697198139514409 ) ) ;
#52929=VECTOR ( 'NONE', #46385, 1000.000000000000227 ) ;
#52930=DIRECTION ( 'NONE',  ( -0.005002170337468016433, -0.7660444431189770143, 0.6427681459581293666 ) ) ;
#52931=ORIENTED_EDGE ( 'NONE', *, *, #31695, .T. ) ;
#52933=VECTOR ( 'NONE', #17847, 1000.000000000000227 ) ;
#52934=ORIENTED_EDGE ( 'NONE', *, *, #54583, .F. ) ;
#52935=CARTESIAN_POINT ( 'NONE',  ( -12.28591023025104079, 0.000000000000000000, 4.924801387518935591 ) ) ;
#52936=CARTESIAN_POINT ( 'NONE',  ( -16.74952957573080425, 0.000000000000000000, 7.106056888501429469 ) ) ;
#52937=LINE ( 'NONE', #18582, #13394 ) ;
#52938=VECTOR ( 'NONE', #8494, 1000.000000000000227 ) ;
#52939=AXIS2_PLACEMENT_3D ( 'NONE', #36913, #54462, #45976 ) ;
#52940=LINE ( 'NONE', #48110, #33068 ) ;
#52941=ORIENTED_EDGE ( 'NONE', *, *, #13384, .T. ) ;
#52942=DIRECTION ( 'NONE',  ( 0.9999697198139515519, 0.000000000000000000, 0.007781995580013368816 ) ) ;
#52943=CARTESIAN_POINT ( 'NONE',  ( -16.25513951096779053, 3.038739411681507185, 8.182458397572339948 ) ) ;
#52944=ORIENTED_EDGE ( 'NONE', *, *, #16034, .T. ) ;
#52945=LINE ( 'NONE', #13758, #11176 ) ;
#52946=LINE ( 'NONE', #48968, #37637 ) ;
#52947=EDGE_LOOP ( 'NONE', ( #6468, #52701, #51978, #117 ) ) ;
#52948=CARTESIAN_POINT ( 'NONE',  ( -21.47419595591918906, 0.000000000000000000, 5.222628093224860102 ) ) ;
#52949=LINE ( 'NONE', #15189, #49621 ) ;
#52951=DIRECTION ( 'NONE',  ( 0.005002170337468016433, -0.7660444431189770143, -0.6427681459581293666 ) ) ;
#52952=FACE_OUTER_BOUND ( 'NONE', #54040, .T. ) ;
#52953=ORIENTED_EDGE ( 'NONE', *, *, #39360, .T. ) ;
#52954=AXIS2_PLACEMENT_3D ( 'NONE', #22272, #47243, #4655 ) ;
#52955=ORIENTED_EDGE ( 'NONE', *, *, #36194, .T. ) ;
#52956=FACE_OUTER_BOUND ( 'NONE', #22359, .T. ) ;
#52957=FACE_OUTER_BOUND ( 'NONE', #46085, .T. ) ;
#52958=LINE ( 'NONE', #18900, #27000 ) ;
#52959=AXIS2_PLACEMENT_3D ( 'NONE', #37026, #41278, #28204 ) ;
#52960=EDGE_CURVE ( 'NONE', #15384, #42326, #37635, .T. ) ;
#52961=ADVANCED_FACE ( 'NONE', ( #19760 ), #41871, .F. ) ;
#52962=CARTESIAN_POINT ( 'NONE',  ( -30.79411802867772607, 0.000000000000000000, 8.643412946479525516 ) ) ;
#52963=CARTESIAN_POINT ( 'NONE',  ( -15.88130887279446490, 0.000000000000000000, 3.050160814894388839 ) ) ;
#52964=VECTOR ( 'NONE', #7115, 999.9999999999998863 ) ;
#52965=ORIENTED_EDGE ( 'NONE', *, *, #11059, .F. ) ;
#52966=EDGE_CURVE ( 'NONE', #34545, #43064, #24016, .T. ) ;
#52967=DIRECTION ( 'NONE',  ( 0.9999697198139515519, 0.000000000000000000, 0.007781995580013368816 ) ) ;
#52968=DIRECTION ( 'NONE',  ( 0.007781995580012663651, -3.146120232559066537E-19, -0.9999697198139514409 ) ) ;
#52969=CARTESIAN_POINT ( 'NONE',  ( -21.47263955680318404, 0.000000000000000000, 5.022634149262071190 ) ) ;
#52970=LINE ( 'NONE', #40494, #29688 ) ;
#52971=VECTOR ( 'NONE', #31261, 1000.000000000000114 ) ;
#52972=ORIENTED_EDGE ( 'NONE', *, *, #7091, .T. ) ;
#52973=LINE ( 'NONE', #10383, #31088 ) ;
#52974=EDGE_LOOP ( 'NONE', ( #21446, #56193, #24077, #41996 ) ) ;
#52975=CARTESIAN_POINT ( 'NONE',  ( -15.95937329197289678, -4.565544526780660917, 10.37393067521759704 ) ) ;
#52976=CARTESIAN_POINT ( 'NONE',  ( -10.57812043228527266, 0.7721120973665049902, 0.7661985235158867980 ) ) ;
#52977=VECTOR ( 'NONE', #25287, 1000.000000000000114 ) ;
#52978=ORIENTED_EDGE ( 'NONE', *, *, #29785, .F. ) ;
#52979=CARTESIAN_POINT ( 'NONE',  ( -27.99923088623136636, 0.000000000000000000, 7.757173251277078130 ) ) ;
#52980=ORIENTED_EDGE ( 'NONE', *, *, #3357, .F. ) ;
#52981=EDGE_CURVE ( 'NONE', #42035, #12550, #10949, .T. ) ;
#52982=VECTOR ( 'NONE', #3926, 999.9999999999998863 ) ;
#52983=ORIENTED_EDGE ( 'NONE', *, *, #23456, .F. ) ;
#52984=ORIENTED_EDGE ( 'NONE', *, *, #11059, .T. ) ;
#52985=CARTESIAN_POINT ( 'NONE',  ( -18.67619601524082285, 0.000000000000000000, 3.936400510096834893 ) ) ;
#52986=VECTOR ( 'NONE', #51569, 999.9999999999998863 ) ;
#52987=EDGE_LOOP ( 'NONE', ( #34952, #31857, #31909, #456 ) ) ;
#52988=ORIENTED_EDGE ( 'NONE', *, *, #42886, .F. ) ;
#52989=DIRECTION ( 'NONE',  ( -0.6246952433987894571, 0.7422098413412802076, 0.2426528472758539834 ) ) ;
#52990=CARTESIAN_POINT ( 'NONE',  ( -10.00813838035478298, 0.000000000000000000, 10.77830692922518452 ) ) ;
#52991=VERTEX_POINT ( 'NONE', #1858 ) ;
#52992=ADVANCED_FACE ( 'NONE', ( #19184 ), #54382, .T. ) ;
#52993=ORIENTED_EDGE ( 'NONE', *, *, #55673, .T. ) ;
#52994=CARTESIAN_POINT ( 'NONE',  ( -15.88130887279446490, 0.000000000000000000, 3.050160814894388839 ) ) ;
#52995=VERTEX_POINT ( 'NONE', #54131 ) ;
#52996=ORIENTED_EDGE ( 'NONE', *, *, #36851, .T. ) ;
#52997=EDGE_CURVE ( 'NONE', #6183, #12574, #15235, .T. ) ;
#52998=VECTOR ( 'NONE', #31712, 1000.000000000000227 ) ;
#52999=DIRECTION ( 'NONE',  ( 0.7660212471507180654, -0.6427876096865404731, 0.005961354470445141482 ) ) ;
#53000=ADVANCED_FACE ( 'NONE', ( #53832 ), #23728, .F. ) ;
#53001=VECTOR ( 'NONE', #10558, 999.9999999999998863 ) ;
#53003=CARTESIAN_POINT ( 'NONE',  ( -21.47419595591918906, 0.000000000000000000, 5.222628093224860102 ) ) ;
#53004=CARTESIAN_POINT ( 'NONE',  ( -15.89360807292448285, -0.1191753592594205352, 3.688726211178170455 ) ) ;
#53005=EDGE_CURVE ( 'NONE', #33548, #20460, #49853, .T. ) ;
#53006=EDGE_LOOP ( 'NONE', ( #33409, #26876, #43796, #15282 ) ) ;
#53007=CARTESIAN_POINT ( 'NONE',  ( -9.768479909093388258, 0.000000000000000000, 5.683056751990515743 ) ) ;
#53008=AXIS2_PLACEMENT_3D ( 'NONE', #21303, #42596, #38062 ) ;
#53009=EDGE_LOOP ( 'NONE', ( #36406, #36350, #10388, #53353 ) ) ;
#53010=EDGE_CURVE ( 'NONE', #25448, #43321, #36513, .T. ) ;
#53011=DIRECTION ( 'NONE',  ( -0.6427681459581293666, -0.7660444431189770143, -0.005002170337467561935 ) ) ;
#53013=VECTOR ( 'NONE', #12387, 999.9999999999998863 ) ;
#53014=LINE ( 'NONE', #9282, #47665 ) ;
#53015=DIRECTION ( 'NONE',  ( 0.5364919789714477361, 0.6444004775717706579, 0.5449076811759711036 ) ) ;
#53016=CARTESIAN_POINT ( 'NONE',  ( -28.93137873341882127, 0.000000000000000000, 8.119251130998824451 ) ) ;
#53017=CARTESIAN_POINT ( 'NONE',  ( -14.96146022573702972, -0.1191753592594187450, 3.326648331456423247 ) ) ;
#53018=AXIS2_PLACEMENT_3D ( 'NONE', #52492, #17281, #35741 ) ;
#53019=CARTESIAN_POINT ( 'NONE',  ( -8.833458008400651096, 0.000000000000000000, 4.951669169011005067 ) ) ;
#53020=ORIENTED_EDGE ( 'NONE', *, *, #15266, .T. ) ;
#53021=CARTESIAN_POINT ( 'NONE',  ( -18.15493648027519669, 0.000000000000000000, 8.572447966228459393 ) ) ;
#53022=VECTOR ( 'NONE', #55579, 999.9999999999998863 ) ;
#53024=CARTESIAN_POINT ( 'NONE',  ( -19.98537980836135119, 5.305366725996514710, 4.275662980210056752 ) ) ;
#53025=FACE_OUTER_BOUND ( 'NONE', #27713, .T. ) ;
#53027=CARTESIAN_POINT ( 'NONE',  ( -13.68401262866885482, 0.000000000000000000, 5.452579114767647894 ) ) ;
#53028=CARTESIAN_POINT ( 'NONE',  ( -20.26176469941677993, 0.000000000000000000, 14.76116360616437895 ) ) ;
#53029=VECTOR ( 'NONE', #49488, 1000.000000000000114 ) ;
#53030=CARTESIAN_POINT ( 'NONE',  ( -12.13851405436063047, 0.000000000000000000, 11.68505802764555135 ) ) ;
#53031=VECTOR ( 'NONE', #7097, 999.9999999999998863 ) ;
#53032=EDGE_LOOP ( 'NONE', ( #44803, #43162, #50183, #19331 ) ) ;
#53033=CARTESIAN_POINT ( 'NONE',  ( -19.18184055174032920, -0.1191753592594164968, 8.260322821228706758 ) ) ;
#53034=DIRECTION ( 'NONE',  ( 0.005961354470445682716, -0.6427876096865404731, -0.7660212471507180654 ) ) ;
#53035=PLANE ( 'NONE',  #21567 ) ;
#53036=ADVANCED_FACE ( 'NONE', ( #19473 ), #54651, .F. ) ;
#53037=CARTESIAN_POINT ( 'NONE',  ( -14.86930721471348171, 0.000000000000000000, 4.335358668806328808 ) ) ;
#53038=CARTESIAN_POINT ( 'NONE',  ( -12.15828988943850675, -2.298917212465657833, 5.177539221031057792 ) ) ;
#53039=CARTESIAN_POINT ( 'NONE',  ( -15.46058576464150569, -0.1191753592594190225, 7.754748858781589149 ) ) ;
#53040=EDGE_CURVE ( 'NONE', #27291, #48737, #31978, .T. ) ;
#53041=EDGE_CURVE ( 'NONE', #14703, #18484, #6997, .T. ) ;
#53042=CARTESIAN_POINT ( 'NONE',  ( -2.276746449950904694, -3.901742918183043418, -2.334007935867973949 ) ) ;
#53043=AXIS2_PLACEMENT_3D ( 'NONE', #43121, #7624, #29790 ) ;
#53044=CARTESIAN_POINT ( 'NONE',  ( -29.86197018149027116, 0.000000000000000000, 8.281335066757780083 ) ) ;
#53045=VECTOR ( 'NONE', #42773, 999.9999999999998863 ) ;
#53046=CARTESIAN_POINT ( 'NONE',  ( -9.502241701925603579, 0.000000000000000000, 2.530466064606057053 ) ) ;
#53047=AXIS2_PLACEMENT_3D ( 'NONE', #49918, #47015, #23279 ) ;
#53048=VERTEX_POINT ( 'NONE', #41609 ) ;
#53049=AXIS2_PLACEMENT_3D ( 'NONE', #30923, #52777, #43437 ) ;
#53050=EDGE_CURVE ( 'NONE', #41210, #48904, #10413, .T. ) ;
#53052=ORIENTED_EDGE ( 'NONE', *, *, #25881, .T. ) ;
#53053=VECTOR ( 'NONE', #3912, 1000.000000000000227 ) ;
#53054=AXIS2_PLACEMENT_3D ( 'NONE', #24499, #39251, #38720 ) ;
#53055=ORIENTED_EDGE ( 'NONE', *, *, #998, .F. ) ;
#53056=AXIS2_PLACEMENT_3D ( 'NONE', #20173, #38073, #47146 ) ;
#53057=VECTOR ( 'NONE', #467, 1000.000000000000227 ) ;
#53058=ORIENTED_EDGE ( 'NONE', *, *, #51796, .F. ) ;
#53059=DIRECTION ( 'NONE',  ( -0.7660212471507179544, -0.6427876096865405842, -0.005961354470445141482 ) ) ;
#53060=LINE ( 'NONE', #52227, #43926 ) ;
#53061=VECTOR ( 'NONE', #21307, 1000.000000000000114 ) ;
#53062=VERTEX_POINT ( 'NONE', #33937 ) ;
#53063=EDGE_LOOP ( 'NONE', ( #28570, #40838, #10110, #18124 ) ) ;
#53064=EDGE_CURVE ( 'NONE', #28751, #5616, #56090, .T. ) ;
#53065=VECTOR ( 'NONE', #55135, 1000.000000000000227 ) ;
#53066=VECTOR ( 'NONE', #21459, 999.9999999999998863 ) ;
#53067=LINE ( 'NONE', #15007, #52069 ) ;
#53068=ORIENTED_EDGE ( 'NONE', *, *, #24887, .T. ) ;
#53069=CARTESIAN_POINT ( 'NONE',  ( 2.072287782118878319, 0.000000000000000000, -2.950529333540147015 ) ) ;
#53070=DIRECTION ( 'NONE',  ( 0.007781995580012662783, 0.000000000000000000, -0.9999697198139514409 ) ) ;
#53071=EDGE_LOOP ( 'NONE', ( #29885, #51699, #5300 ) ) ;
#53072=CARTESIAN_POINT ( 'NONE',  ( -21.47263955680318404, 0.000000000000000000, 5.022634149262071190 ) ) ;
#53073=ORIENTED_EDGE ( 'NONE', *, *, #26069, .F. ) ;
#53074=PLANE ( 'NONE',  #49078 ) ;
#53075=EDGE_CURVE ( 'NONE', #13988, #48977, #17175, .T. ) ;
#53076=DIRECTION ( 'NONE',  ( 0.7660212471507180654, -0.6427876096865404731, 0.005961354470445141482 ) ) ;
#53077=VECTOR ( 'NONE', #30826, 1000.000000000000227 ) ;
#53078=DIRECTION ( 'NONE',  ( -0.6427681459581293666, -0.7660444431189770143, -0.005002170337467561935 ) ) ;
#53079=LINE ( 'NONE', #18729, #48694 ) ;
#53080=VERTEX_POINT ( 'NONE', #25689 ) ;
#53081=FACE_OUTER_BOUND ( 'NONE', #47840, .T. ) ;
#53082=CARTESIAN_POINT ( 'NONE',  ( -19.60990026154428278, 0.000000000000000000, 4.498472333781370125 ) ) ;
#53083=FACE_OUTER_BOUND ( 'NONE', #24017, .T. ) ;
#53084=VECTOR ( 'NONE', #39610, 999.9999999999998863 ) ;
#53085=ORIENTED_EDGE ( 'NONE', *, *, #34188, .T. ) ;
#53086=CARTESIAN_POINT ( 'NONE',  ( -13.22380618444906197, 0.000000000000000000, 6.025498673756209733 ) ) ;
#53087=EDGE_LOOP ( 'NONE', ( #54333, #50852, #53656 ) ) ;
#53088=VECTOR ( 'NONE', #37580, 1000.000000000000227 ) ;
#53089=EDGE_CURVE ( 'NONE', #14783, #38400, #42171, .T. ) ;
#53090=CARTESIAN_POINT ( 'NONE',  ( -15.32532195103871686, 0.000000000000000000, 3.223813647265023619 ) ) ;
#53091=LINE ( 'NONE', #30682, #37805 ) ;
#53092=CARTESIAN_POINT ( 'NONE',  ( -12.53175246298163970, 0.000000000000000000, 2.506889711357553008 ) ) ;
#53093=CARTESIAN_POINT ( 'NONE',  ( -18.67775241435682432, 0.000000000000000000, 4.136394454059623804 ) ) ;
#53094=VECTOR ( 'NONE', #25093, 1000.000000000000114 ) ;
#53095=CARTESIAN_POINT ( 'NONE',  ( -20.24669849012556000, -1.975113310420658852, 4.682809936065343237 ) ) ;
#53096=EDGE_CURVE ( 'NONE', #47218, #3340, #29705, .T. ) ;
#53098=DIRECTION ( 'NONE',  ( -0.7660212471507179544, -0.6427876096865405842, -0.005961354470445141482 ) ) ;
#53099=ADVANCED_FACE ( 'NONE', ( #46713 ), #12910, .F. ) ;
#53100=CARTESIAN_POINT ( 'NONE',  ( -12.54324867700277046, 0.000000000000000000, 3.984128524388611314 ) ) ;
#53102=AXIS2_PLACEMENT_3D ( 'NONE', #15459, #50397, #24830 ) ;
#53103=( NAMED_UNIT ( * ) PLANE_ANGLE_UNIT ( ) SI_UNIT ( $, .RADIAN. ) );
#53104=CARTESIAN_POINT ( 'NONE',  ( -15.60102546347950536, 0.000000000000000000, 12.95077420755565356 ) ) ;
#53105=ORIENTED_EDGE ( 'NONE', *, *, #34777, .T. ) ;
#53106=DIRECTION ( 'NONE',  ( -0.5364919789714478471, 0.6444004775717705469, -0.5449076811759709926 ) ) ;
#53107=PLANE ( 'NONE',  #16050 ) ;
#53108=EDGE_CURVE ( 'NONE', #1004, #45599, #42462, .T. ) ;
#53109=CARTESIAN_POINT ( 'NONE',  ( -14.94916102560700821, 0.000000000000000000, 2.688082935172642962 ) ) ;
#53110=DIRECTION ( 'NONE',  ( 0.007781995580012663651, 0.000000000000000000, -0.9999697198139515519 ) ) ;
#53111=AXIS2_PLACEMENT_3D ( 'NONE', #2519, #15559, #41685 ) ;
#53112=VECTOR ( 'NONE', #19680, 1000.000000000000000 ) ;
#53113=EDGE_CURVE ( 'NONE', #29459, #15659, #21140, .T. ) ;
#53114=DIRECTION ( 'NONE',  ( -0.5364919789714478471, 0.6444004775717705469, -0.5449076811759709926 ) ) ;
#53115=CARTESIAN_POINT ( 'NONE',  ( -14.03700917569638840, -4.565544526780664469, 2.188107406206031502 ) ) ;
#53116=ADVANCED_FACE ( 'NONE', ( #30240 ), #20610, .F. ) ;
#53117=CARTESIAN_POINT ( 'NONE',  ( -22.40478740399063895, 0.000000000000000000, 5.384712028983816623 ) ) ;
#53118=ORIENTED_EDGE ( 'NONE', *, *, #24253, .T. ) ;
#53119=VECTOR ( 'NONE', #22540, 999.9999999999998863 ) ;
#53120=VECTOR ( 'NONE', #37284, 999.9999999999998863 ) ;
#53121=ORIENTED_EDGE ( 'NONE', *, *, #3800, .T. ) ;
#53122=LINE ( 'NONE', #44310, #52231 ) ;
#53123=DIRECTION ( 'NONE',  ( 0.007781995580012663651, 0.000000000000000000, -0.9999697198139515519 ) ) ;
#53125=ORIENTED_EDGE ( 'NONE', *, *, #27912, .F. ) ;
#53126=DIRECTION ( 'NONE',  ( 0.005002170337468016433, -0.7660444431189770143, -0.6427681459581293666 ) ) ;
#53127=EDGE_LOOP ( 'NONE', ( #44621, #48384, #33615, #3990 ) ) ;
#53128=LINE ( 'NONE', #14770, #40159 ) ;
#53129=AXIS2_PLACEMENT_3D ( 'NONE', #40105, #6318, #18239 ) ;
#53130=EDGE_CURVE ( 'NONE', #23668, #42246, #21453, .T. ) ;
#53131=EDGE_LOOP ( 'NONE', ( #45105, #43630, #54311, #1726 ) ) ;
#53132=ORIENTED_EDGE ( 'NONE', *, *, #53580, .F. ) ;
#53133=ORIENTED_EDGE ( 'NONE', *, *, #1487, .T. ) ;
#53134=VECTOR ( 'NONE', #46591, 1000.000000000000114 ) ;
#53135=DIRECTION ( 'NONE',  ( -0.005002170337468016433, -0.7660444431189770143, 0.6427681459581293666 ) ) ;
#53136=CARTESIAN_POINT ( 'NONE',  ( -13.73672976910459909, 0.000000000000000000, 12.22661844811216270 ) ) ;
#53137=VECTOR ( 'NONE', #26835, 1000.000000000000227 ) ;
#53138=DIRECTION ( 'NONE',  ( 0.000000000000000000, -0.000000000000000000, -1.000000000000000000 ) ) ;
#53139=DIRECTION ( 'NONE',  ( 0.5364919789714477361, 0.6444004775717706579, 0.5449076811759711036 ) ) ;
#53140=EDGE_LOOP ( 'NONE', ( #13589, #2130, #23275, #13887 ) ) ;
#53141=VECTOR ( 'NONE', #34631, 1000.000000000000227 ) ;
#53142=VERTEX_POINT ( 'NONE', #37922 ) ;
#53143=AXIS2_PLACEMENT_3D ( 'NONE', #55589, #54455, #2768 ) ;
#53144=VECTOR ( 'NONE', #39871, 1000.000000000000114 ) ;
#53145=CARTESIAN_POINT ( 'NONE',  ( -8.573006763416911369, 0.000000000000000000, 5.492354144215751965 ) ) ;
#53146=EDGE_LOOP ( 'NONE', ( #37248, #9184, #14578, #1502 ) ) ;
#53147=PLANE ( 'NONE',  #20056 ) ;
#53148=VECTOR ( 'NONE', #13555, 999.9999999999998863 ) ;
#53149=ORIENTED_EDGE ( 'NONE', *, *, #39929, .T. ) ;
#53150=DIRECTION ( 'NONE',  ( 0.007781995580012663651, 0.000000000000000000, -0.9999697198139515519 ) ) ;
#53151=DIRECTION ( 'NONE',  ( 0.000000000000000000, -1.000000000000000000, 0.000000000000000000 ) ) ;
#53152=VECTOR ( 'NONE', #43582, 999.9999999999998863 ) ;
#53153=EDGE_LOOP ( 'NONE', ( #34866, #28380, #52993, #17799 ) ) ;
#53154=VECTOR ( 'NONE', #15009, 1000.000000000000227 ) ;
#53155=DIRECTION ( 'NONE',  ( 0.000000000000000000, -0.000000000000000000, -1.000000000000000000 ) ) ;
#53156=EDGE_CURVE ( 'NONE', #42084, #6779, #12640, .T. ) ;
#53157=ORIENTED_EDGE ( 'NONE', *, *, #35532, .F. ) ;
#53158=VECTOR ( 'NONE', #19034, 1000.000000000000227 ) ;
#53159=PLANE ( 'NONE',  #46314 ) ;
#53160=AXIS2_PLACEMENT_3D ( 'NONE', #10836, #28147, #2307 ) ;
#53161=ORIENTED_EDGE ( 'NONE', *, *, #20035, .F. ) ;
#53162=CARTESIAN_POINT ( 'NONE',  ( -20.54204810873173415, 0.000000000000000000, 4.860550213503115558 ) ) ;
#53163=LINE ( 'NONE', #18209, #4008 ) ;
#53164=LINE ( 'NONE', #40657, #17416 ) ;
#53165=EDGE_LOOP ( 'NONE', ( #55442, #24762, #38685, #871, #45288 ) ) ;
#53166=ADVANCED_FACE ( 'NONE', ( #3817 ), #47555, .F. ) ;
#53167=LINE ( 'NONE', #10575, #2004 ) ;
#53168=DIRECTION ( 'NONE',  ( -0.5449076811759708816, 0.6444004775717707689, 0.5364919789714475140 ) ) ;
#53170=CARTESIAN_POINT ( 'NONE',  ( -17.73140113748535285, 0.000000000000000000, 13.85752530597602039 ) ) ;
#53171=DIRECTION ( 'NONE',  ( -0.005002170337468016433, -0.7660444431189770143, 0.6427681459581293666 ) ) ;
#53172=ADVANCED_FACE ( 'NONE', ( #8670 ), #16318, .F. ) ;
#53173=VECTOR ( 'NONE', #47295, 1000.000000000000114 ) ;
#53175=ORIENTED_EDGE ( 'NONE', *, *, #8635, .T. ) ;
#53176=CARTESIAN_POINT ( 'NONE',  ( -15.10247214635037771, 0.000000000000000000, 8.596202949488523259 ) ) ;
#53178=LINE ( 'NONE', #1179, #3313 ) ;
#53179=ORIENTED_EDGE ( 'NONE', *, *, #864, .T. ) ;
#53180=CARTESIAN_POINT ( 'NONE',  ( -13.23374599935418772, 0.000000000000000000, 7.302743542824478240 ) ) ;
#53181=LINE ( 'NONE', #40388, #4594 ) ;
#53182=VECTOR ( 'NONE', #11168, 999.9999999999998863 ) ;
#53184=FACE_OUTER_BOUND ( 'NONE', #11963, .T. ) ;
#53185=ADVANCED_FACE ( 'NONE', ( #3550 ), #4410, .F. ) ;
#53186=VECTOR ( 'NONE', #36403, 1000.000000000000227 ) ;
#53187=PLANE ( 'NONE',  #5808 ) ;
#53188=FACE_OUTER_BOUND ( 'NONE', #22611, .T. ) ;
#53189=ADVANCED_FACE ( 'NONE', ( #16066 ), #7523, .F. ) ;
#53192=AXIS2_PLACEMENT_3D ( 'NONE', #54400, #37356, #12395 ) ;
#53193=ORIENTED_EDGE ( 'NONE', *, *, #27186, .F. ) ;
#53194=LINE ( 'NONE', #359, #26711 ) ;
#53195=CARTESIAN_POINT ( 'NONE',  ( -15.92809671498787694, -0.1191753592594204797, 8.120442650271344931 ) ) ;
#53197=VECTOR ( 'NONE', #48760, 1000.000000000000227 ) ;
#53198=CARTESIAN_POINT ( 'NONE',  ( -23.33771345073609638, -0.1191753592594197858, 5.846786880686956955 ) ) ;
#53199=ADVANCED_FACE ( 'NONE', ( #38181 ), #44677, .F. ) ;
#53200=AXIS2_PLACEMENT_3D ( 'NONE', #19115, #36442, #29893 ) ;
#53201=CARTESIAN_POINT ( 'NONE',  ( -15.99438324446388116, 0.000000000000000000, 3.787944983601566395 ) ) ;
#53202=LINE ( 'NONE', #48922, #2261 ) ;
#53203=ORIENTED_EDGE ( 'NONE', *, *, #13164, .T. ) ;
#53204=PLANE ( 'NONE',  #30149 ) ;
#53205=AXIS2_PLACEMENT_3D ( 'NONE', #3601, #51002, #11828 ) ;
#53206=EDGE_CURVE ( 'NONE', #33376, #9694, #18576, .T. ) ;
#53207=VECTOR ( 'NONE', #14611, 1000.000000000000000 ) ;
#53208=LINE ( 'NONE', #31331, #28770 ) ;
#53209=ORIENTED_EDGE ( 'NONE', *, *, #24998, .T. ) ;
#53210=PLANE ( 'NONE',  #26550 ) ;
#53211=CARTESIAN_POINT ( 'NONE',  ( 2.072287782118878319, 0.000000000000000000, -2.950529333540147015 ) ) ;
#53212=CARTESIAN_POINT ( 'NONE',  ( -10.24305662083960300, 0.000000000000000000, 6.956685709290773900 ) ) ;
#53213=ORIENTED_EDGE ( 'NONE', *, *, #49208, .F. ) ;
#53214=LINE ( 'NONE', #27636, #27458 ) ;
#53215=EDGE_LOOP ( 'NONE', ( #33880, #53125, #7769, #23201 ) ) ;
#53216=VECTOR ( 'NONE', #54932, 1000.000000000000227 ) ;
#53217=ORIENTED_EDGE ( 'NONE', *, *, #8715, .T. ) ;
#53218=ORIENTED_EDGE ( 'NONE', *, *, #43946, .T. ) ;
#53219=ORIENTED_EDGE ( 'NONE', *, *, #1036, .T. ) ;
#53220=CARTESIAN_POINT ( 'NONE',  ( -8.941298941339892892, -0.1191753592594185784, 5.958823107244898942 ) ) ;
#53221=PRODUCT ( 'Integrated Nail File & Cleaner Flip-Out', 'Integrated Nail File & Cleaner Flip-Out', '', ( #8776 ) ) ;
#53222=ORIENTED_EDGE ( 'NONE', *, *, #37441, .T. ) ;
#53224=FACE_OUTER_BOUND ( 'NONE', #16967, .T. ) ;
#53225=PLANE ( 'NONE',  #477 ) ;
#53226=ORIENTED_EDGE ( 'NONE', *, *, #30363, .F. ) ;
#53227=DIRECTION ( 'NONE',  ( 0.9999697198139515519, 0.000000000000000000, 0.007781995580013368816 ) ) ;
#53228=VECTOR ( 'NONE', #1581, 1000.000000000000227 ) ;
#53229=ORIENTED_EDGE ( 'NONE', *, *, #19227, .T. ) ;
#53230=DIRECTION ( 'NONE',  ( -0.005961354470445682716, -0.6427876096865404731, 0.7660212471507180654 ) ) ;
#53231=EDGE_CURVE ( 'NONE', #9862, #15187, #5798, .T. ) ;
#53232=ORIENTED_EDGE ( 'NONE', *, *, #40589, .F. ) ;
#53233=VECTOR ( 'NONE', #37882, 1000.000000000000227 ) ;
#53234=CARTESIAN_POINT ( 'NONE',  ( 2.072287782118878319, 0.000000000000000000, -2.950529333540147015 ) ) ;
#53235=ADVANCED_FACE ( 'NONE', ( #48381 ), #14036, .F. ) ;
#53236=DIRECTION ( 'NONE',  ( 0.007781995580012662783, 0.000000000000000000, -0.9999697198139514409 ) ) ;
#53237=LINE ( 'NONE', #1788, #50416 ) ;
#53238=EDGE_CURVE ( 'NONE', #35268, #35565, #13203, .T. ) ;
#53240=CARTESIAN_POINT ( 'NONE',  ( -14.96640450444030535, 0.4483081953215045656, 2.481088123670064149 ) ) ;
#53241=DIRECTION ( 'NONE',  ( 0.9999697198139515519, 0.000000000000000000, 0.007781995580013368816 ) ) ;
#53243=EDGE_CURVE ( 'NONE', #32666, #47865, #44405, .T. ) ;
#53244=EDGE_CURVE ( 'NONE', #24728, #6162, #39873, .T. ) ;
#53245=ADVANCED_FACE ( 'NONE', ( #9208 ), #18279, .F. ) ;
#53246=ORIENTED_EDGE ( 'NONE', *, *, #31100, .F. ) ;
#53247=VECTOR ( 'NONE', #52775, 999.9999999999998863 ) ;
#53248=LINE ( 'NONE', #957, #55482 ) ;
#53249=LINE ( 'NONE', #53496, #48418 ) ;
#53250=CARTESIAN_POINT ( 'NONE',  ( -17.66575075627584113, 0.000000000000000000, 5.421592307971564217 ) ) ;
#53251=VECTOR ( 'NONE', #24724, 1000.000000000000227 ) ;
#53252=DIRECTION ( 'NONE',  ( 0.5364919789714477361, 0.6444004775717706579, 0.5449076811759711036 ) ) ;
#53253=ORIENTED_EDGE ( 'NONE', *, *, #13491, .T. ) ;
#53254=FACE_OUTER_BOUND ( 'NONE', #142, .T. ) ;
#53256=ORIENTED_EDGE ( 'NONE', *, *, #23735, .T. ) ;
#53258=LINE ( 'NONE', #31664, #23140 ) ;
#53259=ORIENTED_EDGE ( 'NONE', *, *, #7853, .T. ) ;
#53261=PLANE ( 'NONE',  #7911 ) ;
#53262=EDGE_CURVE ( 'NONE', #37795, #9694, #39033, .T. ) ;
#53263=LINE ( 'NONE', #14356, #8736 ) ;
#53264=CARTESIAN_POINT ( 'NONE',  ( -17.90432093095618171, -0.8417996532631553119, 5.018114658037904796 ) ) ;
#53265=EDGE_CURVE ( 'NONE', #6150, #55300, #13484, .T. ) ;
#53266=ORIENTED_EDGE ( 'NONE', *, *, #53615, .F. ) ;
#53267=ORIENTED_EDGE ( 'NONE', *, *, #40969, .F. ) ;
#53268=EDGE_CURVE ( 'NONE', #35388, #21115, #40146, .T. ) ;
#53269=DIRECTION ( 'NONE',  ( -0.5449076811759708816, 0.6444004775717707689, 0.5364919789714475140 ) ) ;
#53270=DIRECTION ( 'NONE',  ( 0.007781995580012663651, -3.146120232559066537E-19, -0.9999697198139514409 ) ) ;
#53271=DIRECTION ( 'NONE',  ( 0.9999697198139515519, 0.000000000000000000, 0.007781995580013368816 ) ) ;
#53272=EDGE_CURVE ( 'NONE', #37046, #35002, #9496, .T. ) ;
#53273=CARTESIAN_POINT ( 'NONE',  ( -10.22263688274503401, -0.03228989815065527735, 0.8511102278423342549 ) ) ;
#53274=VECTOR ( 'NONE', #23378, 999.9999999999998863 ) ;
#53275=FACE_OUTER_BOUND ( 'NONE', #21191, .T. ) ;
#53276=ORIENTED_EDGE ( 'NONE', *, *, #35399, .F. ) ;
#53277=CARTESIAN_POINT ( 'NONE',  ( -21.84802659409251291, 3.038739411681507185, 10.35492567590281254 ) ) ;
#53278=LINE ( 'NONE', #48727, #25649 ) ;
#53279=CARTESIAN_POINT ( 'NONE',  ( -12.26004374870349878, 0.000000000000000000, 1.601014058199056178 ) ) ;
#53280=AXIS2_PLACEMENT_3D ( 'NONE', #14074, #48980, #37300 ) ;
#53281=CARTESIAN_POINT ( 'NONE',  ( -28.92982233430281980, 0.000000000000000000, 7.919257187036034651 ) ) ;
#53282=ORIENTED_EDGE ( 'NONE', *, *, #9583, .T. ) ;
#53283=DIRECTION ( 'NONE',  ( -0.7660212471507179544, -0.6427876096865405842, -0.005961354470445141482 ) ) ;
#53284=VERTEX_POINT ( 'NONE', #4958 ) ;
#53285=LINE ( 'NONE', #992, #5083 ) ;
#53286=LINE ( 'NONE', #17795, #13930 ) ;
#53287=EDGE_LOOP ( 'NONE', ( #45685, #3734, #11376, #4144 ) ) ;
#53288=VECTOR ( 'NONE', #16072, 999.9999999999998863 ) ;
#53289=CARTESIAN_POINT ( 'NONE',  ( -20.54126990917373519, -0.1191753592594197858, 4.760553241521720658 ) ) ;
#53290=VERTEX_POINT ( 'NONE', #952 ) ;
#53291=ORIENTED_EDGE ( 'NONE', *, *, #35947, .T. ) ;
#53292=ORIENTED_EDGE ( 'NONE', *, *, #33372, .T. ) ;
#53293=DIRECTION ( 'NONE',  ( 0.007781995580012662783, 0.000000000000000000, -0.9999697198139514409 ) ) ;
#53294=ORIENTED_EDGE ( 'NONE', *, *, #50780, .F. ) ;
#53295=ORIENTED_EDGE ( 'NONE', *, *, #20859, .T. ) ;
#53296=DIRECTION ( 'NONE',  ( 0.6427681459581294776, -0.7660444431189769032, 0.005002170337467562802 ) ) ;
#53297=CARTESIAN_POINT ( 'NONE',  ( -14.50727508107736519, 4.333955019861511992, 2.178774186237679711 ) ) ;
#53298=VERTEX_POINT ( 'NONE', #10047 ) ;
#53299=ORIENTED_EDGE ( 'NONE', *, *, #50792, .F. ) ;
#53301=ORIENTED_EDGE ( 'NONE', *, *, #17936, .F. ) ;
#53302=ORIENTED_EDGE ( 'NONE', *, *, #34777, .F. ) ;
#53303=ADVANCED_FACE ( 'NONE', ( #1236 ), #103, .F. ) ;
#53304=LINE ( 'NONE', #10409, #27593 ) ;
#53305=DIRECTION ( 'NONE',  ( -0.6427681459581293666, -0.7660444431189770143, -0.005002170337467561935 ) ) ;
#53306=CARTESIAN_POINT ( 'NONE',  ( -8.574563162532918170, 0.000000000000000000, 5.692348088178540877 ) ) ;
#53307=ORIENTED_EDGE ( 'NONE', *, *, #36020, .T. ) ;
#53308=DIRECTION ( 'NONE',  ( -0.9999697198139514409, -0.000000000000000000, -0.007781995580013368816 ) ) ;
#53309=ORIENTED_EDGE ( 'NONE', *, *, #20834, .F. ) ;
#53310=EDGE_CURVE ( 'NONE', #45704, #42498, #4669, .T. ) ;
#53311=EDGE_CURVE ( 'NONE', #15384, #37968, #17747, .T. ) ;
#53312=CARTESIAN_POINT ( 'NONE',  ( -12.60458797795435615, 0.000000000000000000, 11.86609696750642229 ) ) ;
#53313=EDGE_CURVE ( 'NONE', #20000, #23956, #30802, .T. ) ;
#53314=LINE ( 'NONE', #35411, #12421 ) ;
#53315=VECTOR ( 'NONE', #28811, 999.9999999999998863 ) ;
#53317=LINE ( 'NONE', #35697, #4043 ) ;
#53318=CARTESIAN_POINT ( 'NONE',  ( 2.072287782118878319, 0.000000000000000000, -2.950529333540147015 ) ) ;
#53319=PLANE ( 'NONE',  #31368 ) ;
#53320=ORIENTED_EDGE ( 'NONE', *, *, #47573, .F. ) ;
#53321=DIRECTION ( 'NONE',  ( 0.000000000000000000, -0.000000000000000000, -1.000000000000000000 ) ) ;
#53322=ORIENTED_EDGE ( 'NONE', *, *, #55513, .F. ) ;
#53323=AXIS2_PLACEMENT_3D ( 'NONE', #33585, #25935, #24787 ) ;
#53324=DIRECTION ( 'NONE',  ( 0.005961354470445682716, -0.6427876096865404731, -0.7660212471507180654 ) ) ;
#53325=CARTESIAN_POINT ( 'NONE',  ( -25.20123094555300369, 0.000000000000000000, 6.470945668149052032 ) ) ;
#53326=LINE ( 'NONE', #23749, #44442 ) ;
#53327=CARTESIAN_POINT ( 'NONE',  ( -14.56888064431065821, -0.1191753592594197858, 12.58947452739191064 ) ) ;
#53328=PLANE ( 'NONE',  #6906 ) ;
#53330=ORIENTED_EDGE ( 'NONE', *, *, #14297, .T. ) ;
#53331=EDGE_CURVE ( 'NONE', #47842, #20661, #44147, .T. ) ;
#53332=DIRECTION ( 'NONE',  ( 0.007781995580012663651, 0.000000000000000000, -0.9999697198139515519 ) ) ;
#53333=LINE ( 'NONE', #53578, #40395 ) ;
#53334=LINE ( 'NONE', #24048, #48159 ) ;
#53335=EDGE_CURVE ( 'NONE', #7012, #19811, #45800, .T. ) ;
#53336=FACE_OUTER_BOUND ( 'NONE', #2337, .T. ) ;
#53337=LINE ( 'NONE', #53038, #44828 ) ;
#53339=CARTESIAN_POINT ( 'NONE',  ( -10.91749235849797373, 0.6102101463440048335, 2.123504717035824552 ) ) ;
#53340=ADVANCED_FACE ( 'NONE', ( #54575 ), #49790, .F. ) ;
#53341=DIRECTION ( 'NONE',  ( 0.007781995580012663651, -3.146120232559066537E-19, -0.9999697198139514409 ) ) ;
#53343=ORIENTED_EDGE ( 'NONE', *, *, #25096, .T. ) ;
#53344=EDGE_LOOP ( 'NONE', ( #999, #24241, #2883, #52897 ) ) ;
#53345=ORIENTED_EDGE ( 'NONE', *, *, #48981, .F. ) ;
#53347=VERTEX_POINT ( 'NONE', #14872 ) ;
#53348=CARTESIAN_POINT ( 'NONE',  ( -31.72626587586518099, 0.000000000000000000, 9.005490826201270949 ) ) ;
#53349=FACE_OUTER_BOUND ( 'NONE', #47958, .T. ) ;
#53350=AXIS2_PLACEMENT_3D ( 'NONE', #16334, #5660, #36326 ) ;
#53351=ORIENTED_EDGE ( 'NONE', *, *, #35615, .T. ) ;
#53352=VERTEX_POINT ( 'NONE', #6625 ) ;
#53353=ORIENTED_EDGE ( 'NONE', *, *, #471, .F. ) ;
#53354=PLANE ( 'NONE',  #13082 ) ;
#53355=DIRECTION ( 'NONE',  ( 0.000000000000000000, -1.000000000000000000, 0.000000000000000000 ) ) ;
#53356=PLANE ( 'NONE',  #25011 ) ;
#53357=ORIENTED_EDGE ( 'NONE', *, *, #17837, .T. ) ;
#53358=DIRECTION ( 'NONE',  ( -0.005961354470445682716, -0.6427876096865404731, 0.7660212471507180654 ) ) ;
#53359=EDGE_CURVE ( 'NONE', #40111, #12564, #6354, .T. ) ;
#53361=DIRECTION ( 'NONE',  ( 0.9999697198139515519, 0.000000000000000000, 0.007781995580013368816 ) ) ;
#53362=FACE_OUTER_BOUND ( 'NONE', #10526, .T. ) ;
#53363=EDGE_CURVE ( 'NONE', #20696, #34483, #32487, .T. ) ;
#53364=EDGE_CURVE ( 'NONE', #16744, #37607, #10882, .T. ) ;
#53365=CARTESIAN_POINT ( 'NONE',  ( -21.47419595591918906, 0.000000000000000000, 5.222628093224860102 ) ) ;
#53366=DIRECTION ( 'NONE',  ( -0.005961354470445682716, -0.6427876096865404731, 0.7660212471507180654 ) ) ;
#53367=DIRECTION ( 'NONE',  ( -0.9999697198139514409, -0.000000000000000000, -0.007781995580013368816 ) ) ;
#53368=LINE ( 'NONE', #40594, #38348 ) ;
#53369=CARTESIAN_POINT ( 'NONE',  ( -13.08486533123210194, 0.000000000000000000, 1.963927175729152541 ) ) ;
#53370=EDGE_LOOP ( 'NONE', ( #54641, #51785, #30356, #24286 ) ) ;
#53371=LINE ( 'NONE', #40300, #14711 ) ;
#53372=ORIENTED_EDGE ( 'NONE', *, *, #5182, .T. ) ;
#53373=LINE ( 'NONE', #22982, #43765 ) ;
#53374=CARTESIAN_POINT ( 'NONE',  ( -14.04368264607599137, -0.1191753592594188005, 4.811118968023500919 ) ) ;
#53375=DIRECTION ( 'NONE',  ( 0.007781995580012663651, -3.146120232559066537E-19, -0.9999697198139514409 ) ) ;
#53376=CARTESIAN_POINT ( 'NONE',  ( -18.65372086127329609, -5.536956232915662746, 13.01475887526525099 ) ) ;
#53377=LINE ( 'NONE', #40605, #43170 ) ;
#53378=CARTESIAN_POINT ( 'NONE',  ( 2.072287782118878319, 0.000000000000000000, -2.950529333540147015 ) ) ;
#53379=FACE_OUTER_BOUND ( 'NONE', #7308, .T. ) ;
#53380=CARTESIAN_POINT ( 'NONE',  ( -24.27063949748155380, 0.000000000000000000, 6.308861732390097288 ) ) ;
#53381=CARTESIAN_POINT ( 'NONE',  ( -17.09340172029636662, 0.000000000000000000, 9.858031298192779346 ) ) ;
#53382=ORIENTED_EDGE ( 'NONE', *, *, #39212, .T. ) ;
#53383=PLANE ( 'NONE',  #35728 ) ;
#53384=PLANE ( 'NONE',  #8805 ) ;
#53385=CARTESIAN_POINT ( 'NONE',  ( 2.072287782118878319, 0.000000000000000000, -2.950529333540147015 ) ) ;
#53386=DIRECTION ( 'NONE',  ( -0.9999697198139514409, -0.000000000000000000, -0.007781995580013368816 ) ) ;
#53387=VECTOR ( 'NONE', #30999, 1000.000000000000000 ) ;
#53388=CARTESIAN_POINT ( 'NONE',  ( -16.06709938707323460, 0.000000000000000000, 13.13181314741652628 ) ) ;
#53389=ADVANCED_FACE ( 'NONE', ( #19396 ), #41271, .F. ) ;
#53390=CARTESIAN_POINT ( 'NONE',  ( -14.59891615482461802, 0.000000000000000000, 3.598798774942804979 ) ) ;
#53393=ORIENTED_EDGE ( 'NONE', *, *, #48428, .T. ) ;
#53394=ADVANCED_FACE ( 'NONE', ( #24237 ), #27950, .F. ) ;
#53395=LINE ( 'NONE', #9952, #34118 ) ;
#53396=CARTESIAN_POINT ( 'NONE',  ( -12.83519780597105253, -4.727446477803161073, 9.426103502958849134 ) ) ;
#53397=ORIENTED_EDGE ( 'NONE', *, *, #29946, .F. ) ;
#53398=DIRECTION ( 'NONE',  ( 0.5449076811759707706, 0.6444004775717708799, -0.5364919789714476250 ) ) ;
#53399=ADVANCED_FACE ( 'NONE', ( #53754 ), #6103, .F. ) ;
#53400=ORIENTED_EDGE ( 'NONE', *, *, #22834, .F. ) ;
#53401=CARTESIAN_POINT ( 'NONE',  ( -11.83055794499902902, -2.460819163488157546, 5.315945687937546182 ) ) ;
#53402=VERTEX_POINT ( 'NONE', #15170 ) ;
#53403=VERTEX_POINT ( 'NONE', #37272 ) ;
#53404=ORIENTED_EDGE ( 'NONE', *, *, #22595, .T. ) ;
#53405=CARTESIAN_POINT ( 'NONE',  ( -36.91819796696599099, 0.000000000000000000, 21.84982018086542155 ) ) ;
#53406=LINE ( 'NONE', #36644, #55870 ) ;
#53408=CARTESIAN_POINT ( 'NONE',  ( -16.89925026227929195, -0.1191753592594197858, 13.49466922669627422 ) ) ;
#53409=EDGE_LOOP ( 'NONE', ( #22350, #39197, #28859, #5363 ) ) ;
#53410=ORIENTED_EDGE ( 'NONE', *, *, #43473, .F. ) ;
#53411=DIRECTION ( 'NONE',  ( 0.5364919789714477361, 0.6444004775717706579, 0.5449076811759711036 ) ) ;
#53412=ORIENTED_EDGE ( 'NONE', *, *, #27188, .F. ) ;
#53413=FACE_OUTER_BOUND ( 'NONE', #32703, .T. ) ;
#53414=ADVANCED_FACE ( 'NONE', ( #15415 ), #32729, .F. ) ;
#53415=EDGE_LOOP ( 'NONE', ( #18460, #2077, #38893, #18656 ) ) ;
#53416=CARTESIAN_POINT ( 'NONE',  ( -26.13493519185646008, 0.000000000000000000, 7.033017491833586377 ) ) ;
#53417=CARTESIAN_POINT ( 'NONE',  ( -14.89385604187174295, 0.000000000000000000, 7.489830238831231668 ) ) ;
#53419=EDGE_LOOP ( 'NONE', ( #42003, #26512, #43898, #9516 ) ) ;
#53420=ADVANCED_FACE ( 'NONE', ( #40721 ), #28477, .F. ) ;
#53421=CARTESIAN_POINT ( 'NONE',  ( -10.41143597624427919, 0.000000000000000000, 2.892722574339361863 ) ) ;
#53422=ORIENTED_EDGE ( 'NONE', *, *, #16222, .F. ) ;
#53423=EDGE_CURVE ( 'NONE', #44308, #14388, #32200, .T. ) ;
#53424=DIRECTION ( 'NONE',  ( 0.005002170337468016433, -0.7660444431189770143, -0.6427681459581293666 ) ) ;
#53425=VERTEX_POINT ( 'NONE', #23121 ) ;
#53426=FACE_OUTER_BOUND ( 'NONE', #26552, .T. ) ;
#53427=LINE ( 'NONE', #40369, #43893 ) ;
#53428=DIRECTION ( 'NONE',  ( -0.9999697198139514409, -0.000000000000000000, -0.007781995580013368816 ) ) ;
#53429=ORIENTED_EDGE ( 'NONE', *, *, #45563, .T. ) ;
#53430=CARTESIAN_POINT ( 'NONE',  ( -11.20636620717317378, 0.000000000000000000, 11.32298014792380414 ) ) ;
#53431=FACE_OUTER_BOUND ( 'NONE', #26197, .T. ) ;
#53432=CARTESIAN_POINT ( 'NONE',  ( -13.23087194584890369, 0.000000000000000000, 6.933433839566713885 ) ) ;
#53433=FACE_OUTER_BOUND ( 'NONE', #54707, .T. ) ;
#53434=CARTESIAN_POINT ( 'NONE',  ( -14.86224145331363466, 0.000000000000000000, 3.427423502995822879 ) ) ;
#53435=CARTESIAN_POINT ( 'NONE',  ( -14.98732670728457173, -0.1191753592594181482, 6.650435660776302882 ) ) ;
#53436=EDGE_CURVE ( 'NONE', #31087, #13272, #40450, .T. ) ;
#53438=VERTEX_POINT ( 'NONE', #18869 ) ;
#53439=CARTESIAN_POINT ( 'NONE',  ( -20.08396230501010393, -0.1191753592594199662, 4.764112115039379702 ) ) ;
#53440=LINE ( 'NONE', #22514, #33169 ) ;
#53442=ORIENTED_EDGE ( 'NONE', *, *, #3618, .T. ) ;
#53443=DIRECTION ( 'NONE',  ( 0.007781995580012663651, -3.146120232559066537E-19, -0.9999697198139514409 ) ) ;
#53444=LINE ( 'NONE', #10840, #37216 ) ;
#53445=ORIENTED_EDGE ( 'NONE', *, *, #42777, .T. ) ;
#53446=DIRECTION ( 'NONE',  ( 0.000000000000000000, -1.000000000000000000, 0.000000000000000000 ) ) ;
#53447=LINE ( 'NONE', #23616, #14253 ) ;
#53448=FACE_OUTER_BOUND ( 'NONE', #29095, .T. ) ;
#53449=ORIENTED_EDGE ( 'NONE', *, *, #8411, .F. ) ;
#53450=VERTEX_POINT ( 'NONE', #36186 ) ;
#53451=DIRECTION ( 'NONE',  ( 0.005002170337468016433, -0.7660444431189770143, -0.6427681459581293666 ) ) ;
#53452=DIRECTION ( 'NONE',  ( -0.005002170337468016433, -0.7660444431189770143, 0.6427681459581293666 ) ) ;
#53453=CARTESIAN_POINT ( 'NONE',  ( -17.69095614226269930, 3.686347215771511365, 3.436086108215560486 ) ) ;
#53455=PLANE ( 'NONE',  #44607 ) ;
#53456=ORIENTED_EDGE ( 'NONE', *, *, #3280, .T. ) ;
#53457=LINE ( 'NONE', #14556, #34961 ) ;
#53460=CARTESIAN_POINT ( 'NONE',  ( -19.63455492762453858, 0.4483081953215047322, 5.243799167625045499 ) ) ;
#53461=PLANE ( 'NONE',  #8728 ) ;
#53462=ORIENTED_EDGE ( 'NONE', *, *, #36851, .F. ) ;
#53463=CARTESIAN_POINT ( 'NONE',  ( -12.06292385824599123, 0.000000000000000000, 1.971880160572822893 ) ) ;
#53464=DIRECTION ( 'NONE',  ( -0.5364919789714478471, 0.6444004775717705469, -0.5449076811759709926 ) ) ;
#53465=DIRECTION ( 'NONE',  ( -0.005961354470445682716, -0.6427876096865404731, 0.7660212471507180654 ) ) ;
#53466=ADVANCED_FACE ( 'NONE', ( #23403 ), #1790, .F. ) ;
#53467=VERTEX_POINT ( 'NONE', #16531 ) ;
#53469=ORIENTED_EDGE ( 'NONE', *, *, #281, .F. ) ;
#53470=EDGE_CURVE ( 'NONE', #9106, #38880, #50629, .T. ) ;
#53471=EDGE_CURVE ( 'NONE', #33893, #52782, #34169, .T. ) ;
#53472=EDGE_LOOP ( 'NONE', ( #53520, #29614, #13902, #27052 ) ) ;
#53473=ORIENTED_EDGE ( 'NONE', *, *, #7074, .F. ) ;
#53474=LINE ( 'NONE', #49775, #19530 ) ;
#53475=ORIENTED_EDGE ( 'NONE', *, *, #40726, .F. ) ;
#53476=DIRECTION ( 'NONE',  ( 0.007781995580012662783, 0.000000000000000000, -0.9999697198139514409 ) ) ;
#53477=ADVANCED_FACE ( 'NONE', ( #3200 ), #33577, .F. ) ;
#53478=EDGE_LOOP ( 'NONE', ( #16508, #9014, #44120, #36452 ) ) ;
#53479=CARTESIAN_POINT ( 'NONE',  ( -16.92940514515661832, 0.000000000000000000, 4.519332566581076627 ) ) ;
#53480=FACE_OUTER_BOUND ( 'NONE', #24163, .T. ) ;
#53481=EDGE_LOOP ( 'NONE', ( #47306, #13670, #43423, #46378 ) ) ;
#53482=EDGE_CURVE ( 'NONE', #8005, #1853, #50884, .T. ) ;
#53483=DIRECTION ( 'NONE',  ( 0.007781995580012662783, 0.000000000000000000, -0.9999697198139514409 ) ) ;
#53484=ORIENTED_EDGE ( 'NONE', *, *, #22662, .F. ) ;
#53485=EDGE_CURVE ( 'NONE', #32862, #39389, #24489, .T. ) ;
#53486=CARTESIAN_POINT ( 'NONE',  ( -20.54204810873173415, 0.000000000000000000, 4.860550213503115558 ) ) ;
#53487=PLANE ( 'NONE',  #16591 ) ;
#53489=CARTESIAN_POINT ( 'NONE',  ( -9.646137801466288408, 0.000000000000000000, 2.160014162080004851 ) ) ;
#53490=DIRECTION ( 'NONE',  ( 0.9999697198139515519, 0.000000000000000000, 0.007781995580013368816 ) ) ;
#53491=LINE ( 'NONE', #45251, #25565 ) ;
#53492=ORIENTED_EDGE ( 'NONE', *, *, #41769, .F. ) ;
#53493=ADVANCED_FACE ( 'NONE', ( #9072 ), #11987, .F. ) ;
#53494=ORIENTED_EDGE ( 'NONE', *, *, #1156, .F. ) ;
#53495=LINE ( 'NONE', #24493, #11012 ) ;
#53496=CARTESIAN_POINT ( 'NONE',  ( 1.086233639165236964, -1.000000000000000000, 2.796443541562362078 ) ) ;
#53497=DIRECTION ( 'NONE',  ( -0.6427681459581293666, -0.7660444431189770143, -0.005002170337467561935 ) ) ;
#53498=EDGE_CURVE ( 'NONE', #12870, #9978, #7755, .T. ) ;
#53499=CARTESIAN_POINT ( 'NONE',  ( -9.110551994824897193, 0.000000000000000000, 3.538847790438064411 ) ) ;
#53500=ORIENTED_EDGE ( 'NONE', *, *, #52272, .F. ) ;
#53501=PLANE ( 'NONE',  #17729 ) ;
#53502=DIRECTION ( 'NONE',  ( 0.6427681459581294776, -0.7660444431189769032, 0.005002170337467562802 ) ) ;
#53503=EDGE_LOOP ( 'NONE', ( #44484, #21682, #46318, #7680 ) ) ;
#53504=DIRECTION ( 'NONE',  ( 0.000000000000000000, -1.000000000000000000, 0.000000000000000000 ) ) ;
#53506=ORIENTED_EDGE ( 'NONE', *, *, #25043, .T. ) ;
#53508=CARTESIAN_POINT ( 'NONE',  ( 0.000000000000000000, -1.000000000000000000, 0.000000000000000000 ) ) ;
#53509=DIRECTION ( 'NONE',  ( -0.005961354470445682716, -0.6427876096865404731, 0.7660212471507180654 ) ) ;
#53510=DIRECTION ( 'NONE',  ( 0.5364919789714477361, 0.6444004775717706579, 0.5449076811759711036 ) ) ;
#53511=CARTESIAN_POINT ( 'NONE',  ( -19.60912206198628027, -0.1191753592594197858, 4.398475361799976113 ) ) ;
#53512=ORIENTED_EDGE ( 'NONE', *, *, #12944, .F. ) ;
#53513=ORIENTED_EDGE ( 'NONE', *, *, #11932, .F. ) ;
#53514=DIRECTION ( 'NONE',  ( 0.5364919789714477361, 0.6444004775717706579, 0.5449076811759711036 ) ) ;
#53515=DIRECTION ( 'NONE',  ( 0.007781995580012662783, 0.000000000000000000, -0.9999697198139514409 ) ) ;
#53516=PLANE ( 'NONE',  #51474 ) ;
#53518=CARTESIAN_POINT ( 'NONE',  ( -16.92112509763774142, -1.327505506330658003, 5.433334058757370855 ) ) ;
#53519=EDGE_CURVE ( 'NONE', #32268, #14885, #25083, .T. ) ;
#53520=ORIENTED_EDGE ( 'NONE', *, *, #37507, .F. ) ;
#53521=PLANE ( 'NONE',  #12017 ) ;
#53522=DIRECTION ( 'NONE',  ( 0.005961354470445682716, -0.6427876096865404731, -0.7660212471507180654 ) ) ;
#53523=VECTOR ( 'NONE', #779, 1000.000000000000227 ) ;
#53524=CARTESIAN_POINT ( 'NONE',  ( -11.12921961194253306, 0.000000000000000000, 1.409808336888289437 ) ) ;
#53525=LINE ( 'NONE', #45292, #35118 ) ;
#53526=ORIENTED_EDGE ( 'NONE', *, *, #47907, .F. ) ;
#53528=ORIENTED_EDGE ( 'NONE', *, *, #3546, .T. ) ;
#53529=DIRECTION ( 'NONE',  ( 0.005002170337468016433, -0.7660444431189770143, -0.6427681459581293666 ) ) ;
#53530=ADVANCED_FACE ( 'NONE', ( #55430 ), #26377, .F. ) ;
#53531=EDGE_CURVE ( 'NONE', #6183, #2815, #8039, .T. ) ;
#53532=DIRECTION ( 'NONE',  ( 0.007781995580012662783, 0.000000000000000000, -0.9999697198139514409 ) ) ;
#53533=ORIENTED_EDGE ( 'NONE', *, *, #24447, .F. ) ;
#53534=CARTESIAN_POINT ( 'NONE',  ( -18.70240708043708366, 0.4483081953215047322, 4.881721287903300066 ) ) ;
#53535=ORIENTED_EDGE ( 'NONE', *, *, #29406, .F. ) ;
#53537=ORIENTED_EDGE ( 'NONE', *, *, #36755, .F. ) ;
#53538=ORIENTED_EDGE ( 'NONE', *, *, #10886, .T. ) ;
#53540=ORIENTED_EDGE ( 'NONE', *, *, #30342, .T. ) ;
#53541=ORIENTED_EDGE ( 'NONE', *, *, #13260, .T. ) ;
#53542=PLANE ( 'NONE',  #10271 ) ;
#53543=DIRECTION ( 'NONE',  ( 0.005002170337468016433, -0.7660444431189770143, -0.6427681459581293666 ) ) ;
#53544=ORIENTED_EDGE ( 'NONE', *, *, #37865, .F. ) ;
#53545=ORIENTED_EDGE ( 'NONE', *, *, #16301, .T. ) ;
#53546=CARTESIAN_POINT ( 'NONE',  ( -16.96521144160929140, 0.000000000000000000, 9.120364764969224325 ) ) ;
#53547=ADVANCED_FACE ( 'NONE', ( #38398 ), #55723, .F. ) ;
#53548=ORIENTED_EDGE ( 'NONE', *, *, #13506, .F. ) ;
#53549=VERTEX_POINT ( 'NONE', #55168 ) ;
#53551=CARTESIAN_POINT ( 'NONE',  ( -13.14499926216616643, 2.714935509636507316, 1.701275193964931765 ) ) ;
#53553=DIRECTION ( 'NONE',  ( -0.005961354470445682716, -0.6427876096865404731, 0.7660212471507180654 ) ) ;
#53554=CARTESIAN_POINT ( 'NONE',  ( -28.93137873341882127, 0.000000000000000000, 8.119251130998824451 ) ) ;
#53555=ORIENTED_EDGE ( 'NONE', *, *, #47332, .T. ) ;
#53556=CARTESIAN_POINT ( 'NONE',  ( -19.60834386242827776, 0.000000000000000000, 4.298478389818581213 ) ) ;
#53557=EDGE_LOOP ( 'NONE', ( #39950, #16110, #41365, #28363 ) ) ;
#53558=ADVANCED_FACE ( 'NONE', ( #16256 ), #46337, .F. ) ;
#53559=PLANE ( 'NONE',  #2154 ) ;
#53560=VECTOR ( 'NONE', #1483, 999.9999999999998863 ) ;
#53561=LINE ( 'NONE', #23478, #16955 ) ;
#53563=DIRECTION ( 'NONE',  ( -0.9999697198139514409, -0.000000000000000000, -0.007781995580013368816 ) ) ;
#53564=LINE ( 'NONE', #44480, #55675 ) ;
#53565=DIRECTION ( 'NONE',  ( -0.9999697198139514409, -0.000000000000000000, -0.007781995580013368816 ) ) ;
#53566=ORIENTED_EDGE ( 'NONE', *, *, #56086, .T. ) ;
#53567=CARTESIAN_POINT ( 'NONE',  ( -14.12853115097296985, 0.000000000000000000, 2.863795280195287507 ) ) ;
#53568=ORIENTED_EDGE ( 'NONE', *, *, #51679, .T. ) ;
#53569=CARTESIAN_POINT ( 'NONE',  ( -29.86197018149027116, 0.000000000000000000, 8.281335066757780083 ) ) ;
#53570=CARTESIAN_POINT ( 'NONE',  ( -19.79569077582305070, 0.000000000000000000, 14.58012466630350445 ) ) ;
#53571=CARTESIAN_POINT ( 'NONE',  ( 2.072287782118878319, 0.000000000000000000, -2.950529333540147015 ) ) ;
#53572=LINE ( 'NONE', #14678, #24074 ) ;
#53573=DIRECTION ( 'NONE',  ( 0.5364919789714477361, 0.6444004775717706579, 0.5449076811759711036 ) ) ;
#53576=VERTEX_POINT ( 'NONE', #20224 ) ;
#53577=PLANE ( 'NONE',  #3021 ) ;
#53578=CARTESIAN_POINT ( 'NONE',  ( -25.20123094555300369, 0.000000000000000000, 6.470945668149052032 ) ) ;
#53579=CARTESIAN_POINT ( 'NONE',  ( -12.55474489102389946, 0.000000000000000000, 5.461367337419668289 ) ) ;
#53580=EDGE_CURVE ( 'NONE', #8803, #5010, #13604, .T. ) ;
#53581=VECTOR ( 'NONE', #3409, 1000.000000000000114 ) ;
#53582=DIRECTION ( 'NONE',  ( 0.5364919789714477361, 0.6444004775717706579, 0.5449076811759711036 ) ) ;
#53583=CARTESIAN_POINT ( 'NONE',  ( -16.92078298464076624, 0.000000000000000000, 3.411403456807782231 ) ) ;
#53584=EDGE_CURVE ( 'NONE', #27927, #31885, #33324, .T. ) ;
#53585=FACE_OUTER_BOUND ( 'NONE', #25065, .T. ) ;
#53586=LINE ( 'NONE', #6460, #24150 ) ;
#53587=EDGE_CURVE ( 'NONE', #5924, #47914, #44283, .T. ) ;
#53588=CARTESIAN_POINT ( 'NONE',  ( -13.97352483423203573, 0.000000000000000000, 8.646165164180368734 ) ) ;
#53589=EDGE_CURVE ( 'NONE', #33995, #33216, #1384, .T. ) ;
#53590=ADVANCED_FACE ( 'NONE', ( #6229 ), #18423, .F. ) ;
#53591=EDGE_CURVE ( 'NONE', #15384, #37808, #53079, .T. ) ;
#53592=ORIENTED_EDGE ( 'NONE', *, *, #45850, .F. ) ;
#53593=VECTOR ( 'NONE', #22752, 1000.000000000000227 ) ;
#53594=ADVANCED_FACE ( 'NONE', ( #23530 ), #5644, .F. ) ;
#53595=VECTOR ( 'NONE', #45148, 1000.000000000000114 ) ;
#53596=VERTEX_POINT ( 'NONE', #22438 ) ;
#53599=ORIENTED_EDGE ( 'NONE', *, *, #8278, .T. ) ;
#53601=PLANE ( 'NONE',  #7653 ) ;
#53602=EDGE_LOOP ( 'NONE', ( #745, #32298, #14200, #23626 ) ) ;
#53603=VERTEX_POINT ( 'NONE', #40001 ) ;
#53604=EDGE_CURVE ( 'NONE', #22884, #8997, #14727, .T. ) ;
#53605=ORIENTED_EDGE ( 'NONE', *, *, #26141, .T. ) ;
#53606=ADVANCED_FACE ( 'NONE', ( #39746 ), #1087, .F. ) ;
#53608=ADVANCED_FACE ( 'NONE', ( #15019 ), #22687, .F. ) ;
#53609=CARTESIAN_POINT ( 'NONE',  ( -18.67775241435682432, 0.000000000000000000, 4.136394454059623804 ) ) ;
#53610=LINE ( 'NONE', #49360, #45012 ) ;
#53611=EDGE_LOOP ( 'NONE', ( #28386, #10791, #38454, #16162 ) ) ;
#53612=CARTESIAN_POINT ( 'NONE',  ( -15.35495738922491604, -4.403642575758162536, 9.873446328589366772 ) ) ;
#53613=ORIENTED_EDGE ( 'NONE', *, *, #26310, .T. ) ;
#53614=VECTOR ( 'NONE', #47663, 1000.000000000000114 ) ;
#53615=EDGE_CURVE ( 'NONE', #14805, #55847, #32051, .T. ) ;
#53616=VECTOR ( 'NONE', #2207, 1000.000000000000114 ) ;
#53617=DIRECTION ( 'NONE',  ( 0.9999697198139515519, 0.000000000000000000, 0.007781995580013368816 ) ) ;
#53618=CARTESIAN_POINT ( 'NONE',  ( -9.036326005868723144, 0.000000000000000000, 5.319422473152766173 ) ) ;
#53619=ADVANCED_FACE ( 'NONE', ( #27507 ), #48824, .F. ) ;
#53620=CARTESIAN_POINT ( 'NONE',  ( -23.33693525117809386, 0.000000000000000000, 5.746789908705562944 ) ) ;
#53621=CARTESIAN_POINT ( 'NONE',  ( -13.70281334881656043, 0.000000000000000000, 7.868431278277022045 ) ) ;
#53622=DIRECTION ( 'NONE',  ( -0.5449076811759708816, 0.6444004775717707689, 0.5364919789714475140 ) ) ;
#53623=PLANE ( 'NONE',  #19295 ) ;
#53624=PLANE ( 'NONE',  #43930 ) ;
#53625=ORIENTED_EDGE ( 'NONE', *, *, #4556, .T. ) ;
#53626=DIRECTION ( 'NONE',  ( 0.005961354470445682716, -0.6427876096865404731, -0.7660212471507180654 ) ) ;
#53627=ORIENTED_EDGE ( 'NONE', *, *, #53519, .F. ) ;
#53628=DIRECTION ( 'NONE',  ( -0.9999697198139514409, -0.000000000000000000, -0.007781995580013368816 ) ) ;
#53629=FACE_OUTER_BOUND ( 'NONE', #29157, .T. ) ;
#53630=CARTESIAN_POINT ( 'NONE',  ( -24.26986129792355129, -0.1191753592594197858, 6.208864760408702388 ) ) ;
#53631=FACE_OUTER_BOUND ( 'NONE', #287, .T. ) ;
#53632=FACE_OUTER_BOUND ( 'NONE', #19802, .T. ) ;
#53633=LINE ( 'NONE', #49095, #29470 ) ;
#53635=VECTOR ( 'NONE', #24158, 1000.000000000000227 ) ;
#53636=LINE ( 'NONE', #53380, #50964 ) ;
#53637=PRESENTATION_STYLE_ASSIGNMENT (( #48247 ) ) ;
#53638=PLANE ( 'NONE',  #7867 ) ;
#53639=EDGE_LOOP ( 'NONE', ( #24492, #17420, #29575, #49489 ) ) ;
#53640=LINE ( 'NONE', #27532, #7577 ) ;
#53641=DIRECTION ( 'NONE',  ( -0.5449076811759708816, 0.6444004775717707689, 0.5364919789714475140 ) ) ;
#53643=DIRECTION ( 'NONE',  ( -0.9999697198139514409, -0.000000000000000000, -0.007781995580013368816 ) ) ;
#53644=CARTESIAN_POINT ( 'NONE',  ( -11.36082814446342759, 0.000000000000000000, 5.470658673607694311 ) ) ;
#53646=CARTESIAN_POINT ( 'NONE',  ( -13.17065887352947762, -0.1191753592594197858, 12.04635770780929427 ) ) ;
#53647=EDGE_LOOP ( 'NONE', ( #1773, #14706, #39379, #17623 ) ) ;
#53648=VERTEX_POINT ( 'NONE', #53621 ) ;
#53649=LINE ( 'NONE', #27258, #6918 ) ;
#53652=EDGE_CURVE ( 'NONE', #29145, #26892, #48533, .T. ) ;
#53653=ADVANCED_FACE ( 'NONE', ( #36588 ), #23268, .F. ) ;
#53654=VECTOR ( 'NONE', #49258, 999.9999999999998863 ) ;
#53655=AXIS2_PLACEMENT_3D ( 'NONE', #40979, #36443, #35155 ) ;
#53656=ORIENTED_EDGE ( 'NONE', *, *, #35419, .T. ) ;
#53657=DIRECTION ( 'NONE',  ( 0.007781995580012663651, -3.146120232559066537E-19, -0.9999697198139514409 ) ) ;
#53658=ORIENTED_EDGE ( 'NONE', *, *, #32419, .T. ) ;
#53659=LINE ( 'NONE', #11050, #23854 ) ;
#53660=ADVANCED_FACE ( 'NONE', ( #26666 ), #36310, .F. ) ;
#53661=ORIENTED_EDGE ( 'NONE', *, *, #15438, .F. ) ;
#53662=ORIENTED_EDGE ( 'NONE', *, *, #17618, .F. ) ;
#53663=VECTOR ( 'NONE', #21487, 1000.000000000000227 ) ;
#53664=ORIENTED_EDGE ( 'NONE', *, *, #3415, .T. ) ;
#53666=DIRECTION ( 'NONE',  ( 0.2426528472758542054, 0.7422098413412800966, 0.6246952433987894571 ) ) ;
#53667=LINE ( 'NONE', #36939, #27555 ) ;
#53668=ORIENTED_EDGE ( 'NONE', *, *, #17035, .T. ) ;
#53669=VECTOR ( 'NONE', #51021, 1000.000000000000227 ) ;
#53670=ORIENTED_EDGE ( 'NONE', *, *, #14710, .T. ) ;
#53671=VECTOR ( 'NONE', #7053, 1000.000000000000227 ) ;
#53673=ORIENTED_EDGE ( 'NONE', *, *, #38203, .T. ) ;
#53674=PLANE ( 'NONE',  #55456 ) ;
#53676=CARTESIAN_POINT ( 'NONE',  ( -19.60834386242827776, 0.000000000000000000, 4.298478389818581213 ) ) ;
#53677=DIRECTION ( 'NONE',  ( 0.005961354470445682716, -0.6427876096865404731, -0.7660212471507180654 ) ) ;
#53678=EDGE_LOOP ( 'NONE', ( #28792, #7506, #31415, #95 ) ) ;
#53679=CARTESIAN_POINT ( 'NONE',  ( -16.48635313129300783, 3.362543313726510164, 2.978508430039266575 ) ) ;
#53680=EDGE_CURVE ( 'NONE', #23095, #21318, #18142, .T. ) ;
#53681=FACE_OUTER_BOUND ( 'NONE', #18375, .T. ) ;
#53682=ORIENTED_EDGE ( 'NONE', *, *, #48786, .T. ) ;
#53683=EDGE_CURVE ( 'NONE', #8893, #43254, #5109, .T. ) ;
#53684=CARTESIAN_POINT ( 'NONE',  ( -17.21704052607717728, 0.000000000000000000, 7.471750679991184363 ) ) ;
#53685=CARTESIAN_POINT ( 'NONE',  ( -18.33481204970100364, 0.000000000000000000, 5.985723644308105662 ) ) ;
#53686=FACE_OUTER_BOUND ( 'NONE', #41704, .T. ) ;
#53687=EDGE_LOOP ( 'NONE', ( #28817, #2646, #17952, #55935 ) ) ;
#53688=VECTOR ( 'NONE', #46375, 999.9999999999998863 ) ;
#53689=AXIS2_PLACEMENT_3D ( 'NONE', #44911, #6028, #19628 ) ;
#53690=LINE ( 'NONE', #14806, #50037 ) ;
#53691=DIRECTION ( 'NONE',  ( 0.6427681459581294776, -0.7660444431189769032, 0.005002170337467562802 ) ) ;
#53692=EDGE_CURVE ( 'NONE', #23668, #29674, #13880, .T. ) ;
#53693=LINE ( 'NONE', #39815, #45726 ) ;
#53694=PLANE ( 'NONE',  #5071 ) ;
#53695=LINE ( 'NONE', #35847, #34910 ) ;
#53696=DIRECTION ( 'NONE',  ( -0.005961354470445682716, -0.6427876096865404731, 0.7660212471507180654 ) ) ;
#53697=AXIS2_PLACEMENT_3D ( 'NONE', #25196, #46446, #28595 ) ;
#53699=VECTOR ( 'NONE', #32066, 1000.000000000000114 ) ;
#53700=ORIENTED_EDGE ( 'NONE', *, *, #32645, .F. ) ;
#53701=LINE ( 'NONE', #32143, #5357 ) ;
#53702=DIRECTION ( 'NONE',  ( 0.9999697198139515519, 0.000000000000000000, 0.007781995580013368816 ) ) ;
#53704=ORIENTED_EDGE ( 'NONE', *, *, #49108, .F. ) ;
#53705=FACE_OUTER_BOUND ( 'NONE', #4040, .T. ) ;
#53706=DIRECTION ( 'NONE',  ( -0.5364919789714478471, 0.6444004775717705469, -0.5449076811759709926 ) ) ;
#53707=CARTESIAN_POINT ( 'NONE',  ( -14.94838282604900748, -0.1191753592594197858, 2.588085963191248506 ) ) ;
#53708=VECTOR ( 'NONE', #50422, 1000.000000000000114 ) ;
#53710=CARTESIAN_POINT ( 'NONE',  ( 2.072287782118878319, 0.000000000000000000, -2.950529333540147015 ) ) ;
#53711=ORIENTED_EDGE ( 'NONE', *, *, #34376, .T. ) ;
#53712=EDGE_LOOP ( 'NONE', ( #43482, #23839, #4972, #29698 ) ) ;
#53713=CARTESIAN_POINT ( 'NONE',  ( -13.27065584551087163, 0.000000000000000000, 12.04557950825129176 ) ) ;
#53714=FACE_OUTER_BOUND ( 'NONE', #9753, .T. ) ;
#53715=CARTESIAN_POINT ( 'NONE',  ( -14.10280672071693431, -0.1191753592594197858, 12.40843558753103792 ) ) ;
#53716=EDGE_CURVE ( 'NONE', #3230, #1428, #3358, .T. ) ;
#53717=VERTEX_POINT ( 'NONE', #37147 ) ;
#53718=CARTESIAN_POINT ( 'NONE',  ( -15.18036940317838557, -3.108426967578159061, 7.679960954172225129 ) ) ;
#53720=EDGE_LOOP ( 'NONE', ( #30125, #46519, #23994, #28112 ) ) ;
#53722=ADVANCED_FACE ( 'NONE', ( #50194 ), #11302, .F. ) ;
#53723=EDGE_CURVE ( 'NONE', #46605, #12378, #33449, .T. ) ;
#53724=ORIENTED_EDGE ( 'NONE', *, *, #9954, .F. ) ;
#53725=DIRECTION ( 'NONE',  ( 0.5364919789714477361, 0.6444004775717706579, 0.5449076811759711036 ) ) ;
#53726=VECTOR ( 'NONE', #8634, 999.9999999999998863 ) ;
#53727=CARTESIAN_POINT ( 'NONE',  ( -15.13495153988577968, 0.000000000000000000, 12.76973526769478084 ) ) ;
#53728=PLANE ( 'NONE',  #55681 ) ;
#53729=ORIENTED_EDGE ( 'NONE', *, *, #24138, .T. ) ;
#53730=AXIS2_PLACEMENT_3D ( 'NONE', #48796, #19217, #5908 ) ;
#53731=VECTOR ( 'NONE', #55889, 999.9999999999998863 ) ;
#53732=LINE ( 'NONE', #22544, #41942 ) ;
#53733=EDGE_LOOP ( 'NONE', ( #32361, #15055, #38392, #25742 ) ) ;
#53734=EDGE_CURVE ( 'NONE', #21318, #30192, #28911, .T. ) ;
#53735=ORIENTED_EDGE ( 'NONE', *, *, #12638, .F. ) ;
#53736=VECTOR ( 'NONE', #49827, 1000.000000000000000 ) ;
#53737=EDGE_LOOP ( 'NONE', ( #37449, #22554, #7575, #33514 ) ) ;
#53738=DIRECTION ( 'NONE',  ( 0.007781995580012662783, 0.000000000000000000, -0.9999697198139514409 ) ) ;
#53739=VECTOR ( 'NONE', #8454, 999.9999999999998863 ) ;
#53740=VERTEX_POINT ( 'NONE', #15545 ) ;
#53741=FACE_OUTER_BOUND ( 'NONE', #7117, .T. ) ;
#53742=ORIENTED_EDGE ( 'NONE', *, *, #11624, .F. ) ;
#53743=CARTESIAN_POINT ( 'NONE',  ( -12.60458797795435615, 0.000000000000000000, 11.86609696750642229 ) ) ;
#53744=DIRECTION ( 'NONE',  ( -0.005961354470445682716, -0.6427876096865404731, 0.7660212471507180654 ) ) ;
#53745=ORIENTED_EDGE ( 'NONE', *, *, #23595, .T. ) ;
#53746=DIRECTION ( 'NONE',  ( -0.7660212471507179544, -0.6427876096865405842, -0.005961354470445141482 ) ) ;
#53747=VECTOR ( 'NONE', #40849, 999.9999999999998863 ) ;
#53748=VERTEX_POINT ( 'NONE', #24361 ) ;
#53749=AXIS2_PLACEMENT_3D ( 'NONE', #28452, #14849, #10618 ) ;
#53750=FACE_OUTER_BOUND ( 'NONE', #23905, .T. ) ;
#53751=CARTESIAN_POINT ( 'NONE',  ( -10.21299843139749441, 0.000000000000000000, 3.094272917418156243 ) ) ;
#53752=DIRECTION ( 'NONE',  ( -0.005961354470445682716, -0.6427876096865404731, 0.7660212471507180654 ) ) ;
#53753=CARTESIAN_POINT ( 'NONE',  ( -20.14739655590154754, -0.1941918491731548790, 4.826566670133699333 ) ) ;
#53754=FACE_OUTER_BOUND ( 'NONE', #7529, .T. ) ;
#53755=DIRECTION ( 'NONE',  ( 0.000000000000000000, -1.000000000000000000, 0.000000000000000000 ) ) ;
#53756=VERTEX_POINT ( 'NONE', #11011 ) ;
#53757=VECTOR ( 'NONE', #52232, 1000.000000000000227 ) ;
#53758=ORIENTED_EDGE ( 'NONE', *, *, #12443, .F. ) ;
#53759=CARTESIAN_POINT ( 'NONE',  ( -28.92982233430281980, 0.000000000000000000, 7.919257187036034651 ) ) ;
#53760=EDGE_CURVE ( 'NONE', #37629, #16305, #10760, .T. ) ;
#53761=CARTESIAN_POINT ( 'NONE',  ( -12.30984162412481631, 0.000000000000000000, 7.999934106455091509 ) ) ;
#53762=VECTOR ( 'NONE', #36339, 999.9999999999998863 ) ;
#53763=LINE ( 'NONE', #45807, #39698 ) ;
#53764=CARTESIAN_POINT ( 'NONE',  ( -10.41718408325484724, 0.000000000000000000, 3.631341980854890572 ) ) ;
#53765=VERTEX_POINT ( 'NONE', #20677 ) ;
#53766=CARTESIAN_POINT ( 'NONE',  ( -18.67775241435682432, 0.000000000000000000, 4.136394454059623804 ) ) ;
#53767=PLANE ( 'NONE',  #32311 ) ;
#53768=ORIENTED_EDGE ( 'NONE', *, *, #26651, .F. ) ;
#53769=VECTOR ( 'NONE', #12548, 999.9999999999998863 ) ;
#53770=PLANE ( 'NONE',  #38376 ) ;
#53771=PLANE ( 'NONE',  #52150 ) ;
#53772=ORIENTED_EDGE ( 'NONE', *, *, #19211, .T. ) ;
#53773=EDGE_CURVE ( 'NONE', #16343, #12677, #46206, .T. ) ;
#53774=VECTOR ( 'NONE', #33454, 999.9999999999998863 ) ;
#53775=VECTOR ( 'NONE', #25557, 999.9999999999998863 ) ;
#53777=DIRECTION ( 'NONE',  ( 0.6427681459581294776, -0.7660444431189769032, 0.005002170337467562802 ) ) ;
#53778=LINE ( 'NONE', #19420, #54923 ) ;
#53779=EDGE_CURVE ( 'NONE', #25423, #43329, #19826, .T. ) ;
#53780=EDGE_CURVE ( 'NONE', #37968, #40926, #15838, .T. ) ;
#53781=DIRECTION ( 'NONE',  ( 0.005961354470445682716, -0.6427876096865404731, -0.7660212471507180654 ) ) ;
#53782=DIRECTION ( 'NONE',  ( 0.9999697198139515519, 0.000000000000000000, 0.007781995580013368816 ) ) ;
#53783=ORIENTED_EDGE ( 'NONE', *, *, #47852, .F. ) ;
#53784=VECTOR ( 'NONE', #44038, 1000.000000000000000 ) ;
#53785=VECTOR ( 'NONE', #54001, 1000.000000000000227 ) ;
#53786=EDGE_LOOP ( 'NONE', ( #49379, #2190, #24196, #14959 ) ) ;
#53787=DIRECTION ( 'NONE',  ( 0.007781995580012663651, 0.000000000000000000, -0.9999697198139515519 ) ) ;
#53788=DIRECTION ( 'NONE',  ( -0.7660212471507179544, -0.6427876096865405842, -0.005961354470445141482 ) ) ;
#53789=CARTESIAN_POINT ( 'NONE',  ( -17.41260401741867625, 0.000000000000000000, 6.900890633654627848 ) ) ;
#53790=ADVANCED_FACE ( 'NONE', ( #6488 ), #2211, .F. ) ;
#53791=DIRECTION ( 'NONE',  ( 0.9999697198139515519, 0.000000000000000000, 0.007781995580013368816 ) ) ;
#53792=EDGE_CURVE ( 'NONE', #1003, #18912, #45373, .T. ) ;
#53793=VECTOR ( 'NONE', #48818, 1000.000000000000227 ) ;
#53794=DIRECTION ( 'NONE',  ( 0.005002170337468016433, -0.7660444431189770143, -0.6427681459581293666 ) ) ;
#53795=ORIENTED_EDGE ( 'NONE', *, *, #7854, .F. ) ;
#53797=AXIS2_PLACEMENT_3D ( 'NONE', #3873, #21200, #55857 ) ;
#53798=EDGE_CURVE ( 'NONE', #44163, #20837, #23794, .T. ) ;
#53799=CARTESIAN_POINT ( 'NONE',  ( -14.42921914503065750, 0.000000000000000000, 7.493446150599242017 ) ) ;
#53800=LINE ( 'NONE', #22865, #31465 ) ;
#53803=ORIENTED_EDGE ( 'NONE', *, *, #42452, .T. ) ;
#53804=DIRECTION ( 'NONE',  ( -0.6427681459581293666, -0.7660444431189770143, -0.005002170337467561935 ) ) ;
#53805=VECTOR ( 'NONE', #50036, 999.9999999999998863 ) ;
#53806=CARTESIAN_POINT ( 'NONE',  ( -11.67244013076689946, 0.000000000000000000, 11.50401908778467863 ) ) ;
#53807=EDGE_CURVE ( 'NONE', #37343, #8607, #41943, .T. ) ;
#53808=EDGE_LOOP ( 'NONE', ( #48055, #56229, #56208, #6410 ) ) ;
#53809=PLANE ( 'NONE',  #19947 ) ;
#53810=VECTOR ( 'NONE', #918, 999.9999999999998863 ) ;
#53811=ORIENTED_EDGE ( 'NONE', *, *, #26952, .F. ) ;
#53812=EDGE_CURVE ( 'NONE', #20216, #43832, #7313, .T. ) ;
#53813=ORIENTED_EDGE ( 'NONE', *, *, #3453, .F. ) ;
#53815=PLANE ( 'NONE',  #16653 ) ;
#53816=ORIENTED_EDGE ( 'NONE', *, *, #15748, .T. ) ;
#53818=VECTOR ( 'NONE', #50928, 999.9999999999998863 ) ;
#53819=LINE ( 'NONE', #5859, #51027 ) ;
#53820=PLANE ( 'NONE',  #48511 ) ;
#53821=ORIENTED_EDGE ( 'NONE', *, *, #46679, .F. ) ;
#53822=VECTOR ( 'NONE', #8593, 1000.000000000000000 ) ;
#53823=AXIS2_PLACEMENT_3D ( 'NONE', #24644, #11030, #37160 ) ;
#53824=EDGE_LOOP ( 'NONE', ( #50402, #22184, #23181, #22772 ) ) ;
#53825=LINE ( 'NONE', #41863, #35870 ) ;
#53826=VERTEX_POINT ( 'NONE', #29172 ) ;
#53827=ORIENTED_EDGE ( 'NONE', *, *, #52400, .T. ) ;
#53828=VECTOR ( 'NONE', #2775, 1000.000000000000114 ) ;
#53829=LINE ( 'NONE', #53551, #3091 ) ;
#53830=CARTESIAN_POINT ( 'NONE',  ( 2.072287782118878319, 0.000000000000000000, -2.950529333540147015 ) ) ;
#53831=LINE ( 'NONE', #40786, #28701 ) ;
#53832=FACE_OUTER_BOUND ( 'NONE', #17740, .T. ) ;
#53833=ORIENTED_EDGE ( 'NONE', *, *, #23294, .T. ) ;
#53834=PLANE ( 'NONE',  #54633 ) ;
#53835=ORIENTED_EDGE ( 'NONE', *, *, #5487, .F. ) ;
#53836=ADVANCED_FACE ( 'NONE', ( #45954 ), #24092, .F. ) ;
#53837=CARTESIAN_POINT ( 'NONE',  ( -13.47407886980094283, 0.000000000000000000, 4.176890644815381748 ) ) ;
#53839=DIRECTION ( 'NONE',  ( 0.000000000000000000, -0.000000000000000000, -1.000000000000000000 ) ) ;
#53840=VECTOR ( 'NONE', #8655, 1000.000000000000000 ) ;
#53842=LINE ( 'NONE', #14958, #4126 ) ;
#53843=ORIENTED_EDGE ( 'NONE', *, *, #21017, .F. ) ;
#53844=DIRECTION ( 'NONE',  ( -0.7660212471507179544, -0.6427876096865405842, -0.005961354470445141482 ) ) ;
#53845=VECTOR ( 'NONE', #9648, 1000.000000000000000 ) ;
#53846=EDGE_LOOP ( 'NONE', ( #36574, #16408, #41537, #20281 ) ) ;
#53848=CARTESIAN_POINT ( 'NONE',  ( -19.30918475015224800, -5.213152330870663320, 12.73794594145227776 ) ) ;
#53849=DIRECTION ( 'NONE',  ( 0.007781995580012662783, 0.000000000000000000, -0.9999697198139514409 ) ) ;
#53850=AXIS2_PLACEMENT_3D ( 'NONE', #5050, #39693, #51612 ) ;
#53851=DIRECTION ( 'NONE',  ( -0.7660212471507179544, -0.6427876096865405842, -0.005961354470445141482 ) ) ;
#53852=EDGE_CURVE ( 'NONE', #36594, #48082, #45652, .T. ) ;
#53853=DIRECTION ( 'NONE',  ( 0.007781995580012662783, 0.000000000000000000, -0.9999697198139514409 ) ) ;
#53854=VERTEX_POINT ( 'NONE', #37992 ) ;
#53855=VECTOR ( 'NONE', #42372, 999.9999999999998863 ) ;
#53857=DIRECTION ( 'NONE',  ( 0.7660212471507180654, -0.6427876096865404731, 0.005961354470445141482 ) ) ;
#53858=LINE ( 'NONE', #35720, #30937 ) ;
#53859=LINE ( 'NONE', #1052, #5592 ) ;
#53860=EDGE_CURVE ( 'NONE', #25200, #15209, #7063, .T. ) ;
#53861=DIRECTION ( 'NONE',  ( -0.5449076811759708816, 0.6444004775717707689, 0.5364919789714475140 ) ) ;
#53862=DIRECTION ( 'NONE',  ( 0.6427681459581294776, -0.7660444431189769032, 0.005002170337467562802 ) ) ;
#53863=CARTESIAN_POINT ( 'NONE',  ( -12.06867196525655572, 0.000000000000000000, 2.710499567088351824 ) ) ;
#53864=EDGE_CURVE ( 'NONE', #53290, #26301, #55041, .T. ) ;
#53865=VECTOR ( 'NONE', #30830, 999.9999999999998863 ) ;
#53866=AXIS2_PLACEMENT_3D ( 'NONE', #19143, #6128, #36467 ) ;
#53867=DIRECTION ( 'NONE',  ( -0.5449076811759708816, 0.6444004775717707689, 0.5364919789714475140 ) ) ;
#53868=LINE ( 'NONE', #40822, #5679 ) ;
#53869=ORIENTED_EDGE ( 'NONE', *, *, #27602, .T. ) ;
#53870=EDGE_CURVE ( 'NONE', #32666, #15482, #39398, .T. ) ;
#53871=ORIENTED_EDGE ( 'NONE', *, *, #40083, .T. ) ;
#53872=AXIS2_PLACEMENT_3D ( 'NONE', #2969, #54129, #15233 ) ;
#53874=ORIENTED_EDGE ( 'NONE', *, *, #1630, .F. ) ;
#53875=ORIENTED_EDGE ( 'NONE', *, *, #51483, .T. ) ;
#53876=EDGE_LOOP ( 'NONE', ( #41806, #10929, #30892 ) ) ;
#53877=VECTOR ( 'NONE', #41781, 1000.000000000000114 ) ;
#53878=ORIENTED_EDGE ( 'NONE', *, *, #30429, .T. ) ;
#53879=CARTESIAN_POINT ( 'NONE',  ( -14.01701317841955508, 0.000000000000000000, 2.326005055450897085 ) ) ;
#53880=DIRECTION ( 'NONE',  ( 0.9999697198139515519, 0.000000000000000000, 0.007781995580013368816 ) ) ;
#53881=AXIS2_PLACEMENT_3D ( 'NONE', #12649, #25698, #38780 ) ;
#53882=ORIENTED_EDGE ( 'NONE', *, *, #49936, .F. ) ;
#53883=LINE ( 'NONE', #24346, #38571 ) ;
#53884=ORIENTED_EDGE ( 'NONE', *, *, #53335, .F. ) ;
#53885=DIRECTION ( 'NONE',  ( 0.000000000000000000, -1.000000000000000000, 0.000000000000000000 ) ) ;
#53886=VECTOR ( 'NONE', #32590, 1000.000000000000227 ) ;
#53887=CARTESIAN_POINT ( 'NONE',  ( -13.29153558808963531, -0.3560938001956556742, 2.032843665462120697 ) ) ;
#53888=DIRECTION ( 'NONE',  ( -0.7660212471507179544, -0.6427876096865405842, -0.005961354470445141482 ) ) ;
#53890=LINE ( 'NONE', #45121, #40985 ) ;
#53891=EDGE_CURVE ( 'NONE', #22114, #349, #16684, .T. ) ;
#53892=VECTOR ( 'NONE', #16136, 1000.000000000000227 ) ;
#53893=CARTESIAN_POINT ( 'NONE',  ( -11.84139170794692930, 0.000000000000000000, 7.513585222091296423 ) ) ;
#53894=ADVANCED_FACE ( 'NONE', ( #25770 ), #55576, .F. ) ;
#53895=CARTESIAN_POINT ( 'NONE',  ( -27.06630483948590893, -0.1191753592594197858, 7.295098399573937797 ) ) ;
#53896=VECTOR ( 'NONE', #16095, 999.9999999999998863 ) ;
#53897=DIRECTION ( 'NONE',  ( 0.005002170337468016433, -0.7660444431189770143, -0.6427681459581293666 ) ) ;
#53898=CARTESIAN_POINT ( 'NONE',  ( -22.40556560354864146, -0.1191753592594197858, 5.484709000965211523 ) ) ;
#53899=VECTOR ( 'NONE', #16159, 999.9999999999998863 ) ;
#53900=ADVANCED_FACE ( 'NONE', ( #8443 ), #17526, .F. ) ;
#53901=CARTESIAN_POINT ( 'NONE',  ( -21.47341775636118655, -0.1191753592594197858, 5.122631121243466090 ) ) ;
#53902=LINE ( 'NONE', #24363, #52855 ) ;
#53903=FACE_OUTER_BOUND ( 'NONE', #23562, .T. ) ;
#53904=EDGE_CURVE ( 'NONE', #13033, #14383, #33712, .T. ) ;
#53905=DIRECTION ( 'NONE',  ( 0.007781995580012662783, 0.000000000000000000, -0.9999697198139514409 ) ) ;
#53906=ORIENTED_EDGE ( 'NONE', *, *, #28600, .F. ) ;
#53908=EDGE_LOOP ( 'NONE', ( #30909, #26661, #32735, #42444 ) ) ;
#53909=EDGE_CURVE ( 'NONE', #5827, #31801, #34017, .T. ) ;
#53910=ADVANCED_FACE ( 'NONE', ( #51339 ), #56154, .F. ) ;
#53911=EDGE_CURVE ( 'NONE', #24424, #15522, #4211, .T. ) ;
#53912=FACE_OUTER_BOUND ( 'NONE', #49101, .T. ) ;
#53913=CARTESIAN_POINT ( 'NONE',  ( -15.93792926431930645, -1.813211359398158473, 5.848553459476834249 ) ) ;
#53914=DIRECTION ( 'NONE',  ( 0.007781995580012662783, 0.000000000000000000, -0.9999697198139514409 ) ) ;
#53915=CARTESIAN_POINT ( 'NONE',  ( -10.44460696391839427, 0.000000000000000000, 7.155123254137559563 ) ) ;
#53916=CARTESIAN_POINT ( 'NONE',  ( -31.72626587586518099, 0.000000000000000000, 9.005490826201270949 ) ) ;
#53917=LINE ( 'NONE', #16146, #47677 ) ;
#53918=CARTESIAN_POINT ( 'NONE',  ( -16.79925329029790149, 0.000000000000000000, 13.49544742625427496 ) ) ;
#53919=VECTOR ( 'NONE', #36542, 1000.000000000000000 ) ;
#53920=DIRECTION ( 'NONE',  ( 0.5364919789714477361, 0.6444004775717706579, 0.5449076811759711036 ) ) ;
#53921=VECTOR ( 'NONE', #2817, 1000.000000000000227 ) ;
#53922=CARTESIAN_POINT ( 'NONE',  ( -26.13415699229845757, -0.1191753592594197858, 6.933020519852192365 ) ) ;
#53923=DIRECTION ( 'NONE',  ( -0.6427681459581293666, -0.7660444431189770143, -0.005002170337467561935 ) ) ;
#53924=CARTESIAN_POINT ( 'NONE',  ( -31.72782227498118601, 0.000000000000000000, 9.205484770164058972 ) ) ;
#53925=PLANE ( 'NONE',  #4639 ) ;
#53926=VECTOR ( 'NONE', #27889, 1000.000000000000114 ) ;
#53927=FACE_OUTER_BOUND ( 'NONE', #35755, .T. ) ;
#53928=DIRECTION ( 'NONE',  ( -0.6427681459581293666, -0.7660444431189770143, -0.005002170337467561935 ) ) ;
#53929=EDGE_CURVE ( 'NONE', #36681, #5037, #38843, .T. ) ;
#53930=VECTOR ( 'NONE', #37410, 1000.000000000000227 ) ;
#53931=CARTESIAN_POINT ( 'NONE',  ( -10.00813838035478298, 0.000000000000000000, 10.77830692922518452 ) ) ;
#53932=CARTESIAN_POINT ( 'NONE',  ( -12.60458797795435615, 0.000000000000000000, 11.86609696750642229 ) ) ;
#53933=CARTESIAN_POINT ( 'NONE',  ( -19.63737892770141613, -0.1191753592594169270, 7.087566515900918240 ) ) ;
#53935=EDGE_CURVE ( 'NONE', #6267, #53765, #26072, .T. ) ;
#53936=VECTOR ( 'NONE', #54043, 999.9999999999998863 ) ;
#53937=( GEOMETRIC_REPRESENTATION_CONTEXT ( 3 ) GLOBAL_UNCERTAINTY_ASSIGNED_CONTEXT ( ( #28019 ) ) GLOBAL_UNIT_ASSIGNED_CONTEXT ( ( #43780, #52587, #31300 ) ) REPRESENTATION_CONTEXT ( 'NONE', 'WORKASPACE' ) );
#53938=ORIENTED_EDGE ( 'NONE', *, *, #49432, .F. ) ;
#53939=ADVANCED_FACE ( 'NONE', ( #47920 ), #179, .F. ) ;
#53940=LINE ( 'NONE', #23564, #19546 ) ;
#53941=VECTOR ( 'NONE', #18335, 999.9999999999998863 ) ;
#53942=LINE ( 'NONE', #32914, #49391 ) ;
#53943=VECTOR ( 'NONE', #49460, 999.9999999999998863 ) ;
#53944=EDGE_CURVE ( 'NONE', #37711, #7759, #42530, .T. ) ;
#53945=EDGE_LOOP ( 'NONE', ( #44471, #51975, #52922 ) ) ;
#53946=FACE_OUTER_BOUND ( 'NONE', #27363, .T. ) ;
#53947=ORIENTED_EDGE ( 'NONE', *, *, #14977, .F. ) ;
#53949=AXIS2_PLACEMENT_3D ( 'NONE', #26487, #22791, #39278 ) ;
#53950=ORIENTED_EDGE ( 'NONE', *, *, #27450, .T. ) ;
#53953=ORIENTED_EDGE ( 'NONE', *, *, #42840, .F. ) ;
#53955=PLANE ( 'NONE',  #21154 ) ;
#53956=ADVANCED_FACE ( 'NONE', ( #17238 ), #43382, .F. ) ;
#53957=DIRECTION ( 'NONE',  ( 0.5364919789714477361, 0.6444004775717706579, 0.5449076811759711036 ) ) ;
#53958=CARTESIAN_POINT ( 'NONE',  ( -17.65581094137071361, 0.000000000000000000, 4.144347438903294822 ) ) ;
#53959=VERTEX_POINT ( 'NONE', #38251 ) ;
#53960=ORIENTED_EDGE ( 'NONE', *, *, #16904, .F. ) ;
#53961=VECTOR ( 'NONE', #6958, 1000.000000000000227 ) ;
#53962=CARTESIAN_POINT ( 'NONE',  ( -11.67244013076689946, 0.000000000000000000, 11.50401908778467863 ) ) ;
#53963=VECTOR ( 'NONE', #38528, 1000.000000000000227 ) ;
#53964=ORIENTED_EDGE ( 'NONE', *, *, #376, .F. ) ;
#53965=PLANE ( 'NONE',  #36411 ) ;
#53966=ORIENTED_EDGE ( 'NONE', *, *, #14700, .F. ) ;
#53967=VECTOR ( 'NONE', #22448, 1000.000000000000227 ) ;
#53968=FACE_OUTER_BOUND ( 'NONE', #5145, .T. ) ;
#53969=CARTESIAN_POINT ( 'NONE',  ( -14.61328642235102926, 0.000000000000000000, 5.445347291231628084 ) ) ;
#53970=ORIENTED_EDGE ( 'NONE', *, *, #29442, .T. ) ;
#53971=DIRECTION ( 'NONE',  ( 0.000000000000000000, -0.000000000000000000, -1.000000000000000000 ) ) ;
#53972=VECTOR ( 'NONE', #14411, 999.9999999999998863 ) ;
#53973=LINE ( 'NONE', #49970, #49056 ) ;
#53974=AXIS2_PLACEMENT_3D ( 'NONE', #29945, #47245, #21439 ) ;
#53975=AXIS2_PLACEMENT_3D ( 'NONE', #49512, #15674, #23646 ) ;
#53977=CARTESIAN_POINT ( 'NONE',  ( -14.94838282604900748, -0.1191753592594197858, 2.588085963191248506 ) ) ;
#53978=DIRECTION ( 'NONE',  ( -0.5449076811759708816, 0.6444004775717707689, 0.5364919789714475140 ) ) ;
#53979=VECTOR ( 'NONE', #21021, 999.9999999999998863 ) ;
#53980=LINE ( 'NONE', #14270, #1994 ) ;
#53981=ORIENTED_EDGE ( 'NONE', *, *, #20319, .F. ) ;
#53982=AXIS2_PLACEMENT_3D ( 'NONE', #54403, #15253, #28867 ) ;
#53983=ADVANCED_FACE ( 'NONE', ( #52171 ), #43634, .F. ) ;
#53984=EDGE_CURVE ( 'NONE', #27552, #11704, #31455, .T. ) ;
#53985=VECTOR ( 'NONE', #42378, 1000.000000000000227 ) ;
#53986=CARTESIAN_POINT ( 'NONE',  ( -14.49682332889594427, -0.1191753592594190780, 3.330264243224434040 ) ) ;
#53987=DIRECTION ( 'NONE',  ( -0.005961354470445682716, -0.6427876096865404731, 0.7660212471507180654 ) ) ;
#53988=CARTESIAN_POINT ( 'NONE',  ( -17.36532418587302473, -0.1191753592594177458, 13.67570816655714516 ) ) ;
#53989=LINE ( 'NONE', #28138, #11416 ) ;
#53990=EDGE_CURVE ( 'NONE', #47502, #47959, #53314, .T. ) ;
#53991=DIRECTION ( 'NONE',  ( 0.5449076811759707706, 0.6444004775717708799, -0.5364919789714476250 ) ) ;
#53992=FACE_OUTER_BOUND ( 'NONE', #23719, .T. ) ;
#53993=VECTOR ( 'NONE', #37524, 1000.000000000000227 ) ;
#53994=VECTOR ( 'NONE', #22839, 999.9999999999998863 ) ;
#53996=ORIENTED_EDGE ( 'NONE', *, *, #49750, .F. ) ;
#53997=CARTESIAN_POINT ( 'NONE',  ( -16.54234516706728186, -1.975113310420658852, 6.349037806105066295 ) ) ;
#53998=DIRECTION ( 'NONE',  ( -0.9999697198139514409, -0.000000000000000000, -0.007781995580013368816 ) ) ;
#54000=ORIENTED_EDGE ( 'NONE', *, *, #46890, .T. ) ;
#54001=DIRECTION ( 'NONE',  ( -0.5449076811759708816, 0.6444004775717707689, 0.5364919789714475140 ) ) ;
#54002=CARTESIAN_POINT ( 'NONE',  ( -22.40634380310664397, 0.000000000000000000, 5.584705972946605534 ) ) ;
#54003=DIRECTION ( 'NONE',  ( 0.000000000000000000, -0.000000000000000000, -1.000000000000000000 ) ) ;
#54004=DIRECTION ( 'NONE',  ( -0.5449076811759708816, 0.6444004775717707689, 0.5364919789714475140 ) ) ;
#54005=EDGE_CURVE ( 'NONE', #30844, #23916, #53561, .T. ) ;
#54007=VECTOR ( 'NONE', #22165, 1000.000000000000000 ) ;
#54008=EDGE_LOOP ( 'NONE', ( #8394, #31863, #44773, #10191 ) ) ;
#54010=VECTOR ( 'NONE', #50686, 999.9999999999998863 ) ;
#54011=EDGE_CURVE ( 'NONE', #49949, #14352, #49307, .T. ) ;
#54012=CARTESIAN_POINT ( 'NONE',  ( -13.53673582514181106, 0.000000000000000000, 12.22817484722816772 ) ) ;
#54013=VECTOR ( 'NONE', #19970, 1000.000000000000227 ) ;
#54016=ORIENTED_EDGE ( 'NONE', *, *, #26611, .F. ) ;
#54018=AXIS2_PLACEMENT_3D ( 'NONE', #40376, #31846, #49157 ) ;
#54019=VERTEX_POINT ( 'NONE', #39688 ) ;
#54020=FACE_OUTER_BOUND ( 'NONE', #23372, .T. ) ;
#54021=EDGE_CURVE ( 'NONE', #11430, #10050, #13553, .T. ) ;
#54023=EDGE_LOOP ( 'NONE', ( #51069, #55329, #36141, #40440 ) ) ;
#54024=AXIS2_PLACEMENT_3D ( 'NONE', #50932, #15738, #11507 ) ;
#54025=ORIENTED_EDGE ( 'NONE', *, *, #49833, .F. ) ;
#54026=CARTESIAN_POINT ( 'NONE',  ( -10.27421835998572064, 0.000000000000000000, 10.96090226820206048 ) ) ;
#54027=PLANE ( 'NONE',  #27787 ) ;
#54028=LINE ( 'NONE', #19673, #4902 ) ;
#54029=VECTOR ( 'NONE', #50973, 1000.000000000000227 ) ;
#54030=ORIENTED_EDGE ( 'NONE', *, *, #33306, .F. ) ;
#54031=VECTOR ( 'NONE', #33101, 999.9999999999998863 ) ;
#54032=DIRECTION ( 'NONE',  ( 0.005002170337468016433, -0.7660444431189770143, -0.6427681459581293666 ) ) ;
#54033=VECTOR ( 'NONE', #11190, 1000.000000000000227 ) ;
#54034=ORIENTED_EDGE ( 'NONE', *, *, #47928, .T. ) ;
#54035=VECTOR ( 'NONE', #22256, 1000.000000000000227 ) ;
#54036=VERTEX_POINT ( 'NONE', #14664 ) ;
#54037=VECTOR ( 'NONE', #39960, 1000.000000000000227 ) ;
#54038=EDGE_LOOP ( 'NONE', ( #21284, #28544, #55225, #43640 ) ) ;
#54039=LINE ( 'NONE', #14854, #15000 ) ;
#54040=EDGE_LOOP ( 'NONE', ( #36882, #39573, #43900, #30003 ) ) ;
#54041=DIRECTION ( 'NONE',  ( -0.7660212471507179544, -0.6427876096865405842, -0.005961354470445141482 ) ) ;
#54042=ORIENTED_EDGE ( 'NONE', *, *, #39299, .F. ) ;
#54043=DIRECTION ( 'NONE',  ( 0.9999697198139515519, 0.000000000000000000, 0.007781995580013368816 ) ) ;
#54044=DIRECTION ( 'NONE',  ( 0.007781995580012662783, 0.000000000000000000, -0.9999697198139514409 ) ) ;
#54045=ORIENTED_EDGE ( 'NONE', *, *, #8424, .T. ) ;
#54046=FACE_OUTER_BOUND ( 'NONE', #7299, .T. ) ;
#54047=ORIENTED_EDGE ( 'NONE', *, *, #44454, .F. ) ;
#54048=AXIS2_PLACEMENT_3D ( 'NONE', #54356, #40493, #23693 ) ;
#54049=DIRECTION ( 'NONE',  ( 0.007781995580012663651, 0.000000000000000000, -0.9999697198139515519 ) ) ;
#54050=CARTESIAN_POINT ( 'NONE',  ( -9.201257701905497299, -2.398698010759394705, 3.305331372236061327 ) ) ;
#54051=CARTESIAN_POINT ( 'NONE',  ( -10.00813838035478298, 0.000000000000000000, 10.77830692922518452 ) ) ;
#54052=CARTESIAN_POINT ( 'NONE',  ( -19.00053506639916989, 3.524445264749008100, 10.04598931717878507 ) ) ;
#54053=CARTESIAN_POINT ( 'NONE',  ( -18.66354898467281132, 0.000000000000000000, 14.21960318569776582 ) ) ;
#54054=PLANE ( 'NONE',  #41851 ) ;
#54056=VECTOR ( 'NONE', #40465, 1000.000000000000227 ) ;
#54057=ORIENTED_EDGE ( 'NONE', *, *, #6611, .T. ) ;
#54058=EDGE_CURVE ( 'NONE', #15058, #36955, #30865, .T. ) ;
#54059=ORIENTED_EDGE ( 'NONE', *, *, #55848, .F. ) ;
#54060=CARTESIAN_POINT ( 'NONE',  ( -24.26986129792355129, -0.1191753592594197858, 6.208864760408702388 ) ) ;
#54061=CARTESIAN_POINT ( 'NONE',  ( -16.39796932385352335, -0.1117717739994045917, 9.587901738430785414 ) ) ;
#54062=VECTOR ( 'NONE', #23282, 1000.000000000000000 ) ;
#54063=EDGE_CURVE ( 'NONE', #30544, #23505, #18357, .T. ) ;
#54064=EDGE_CURVE ( 'NONE', #32478, #3340, #40536, .T. ) ;
#54066=FACE_OUTER_BOUND ( 'NONE', #47828, .T. ) ;
#54067=VECTOR ( 'NONE', #1678, 999.9999999999998863 ) ;
#54069=LINE ( 'NONE', #36196, #43962 ) ;
#54070=ORIENTED_EDGE ( 'NONE', *, *, #45423, .F. ) ;
#54071=CARTESIAN_POINT ( 'NONE',  ( 2.072287782118878319, 0.000000000000000000, -2.950529333540147015 ) ) ;
#54072=LINE ( 'NONE', #41562, #25946 ) ;
#54073=ORIENTED_EDGE ( 'NONE', *, *, #56174, .F. ) ;
#54074=CARTESIAN_POINT ( 'NONE',  ( -20.54049170961573267, 0.000000000000000000, 4.660556269540326646 ) ) ;
#54077=VECTOR ( 'NONE', #2778, 1000.000000000000227 ) ;
#54078=LINE ( 'NONE', #42119, #12567 ) ;
#54079=CARTESIAN_POINT ( 'NONE',  ( -10.47421230394850866, 0.000000000000000000, 10.95934586908605723 ) ) ;
#54080=VECTOR ( 'NONE', #11781, 1000.000000000000000 ) ;
#54081=LINE ( 'NONE', #45530, #30502 ) ;
#54082=DIRECTION ( 'NONE',  ( 0.5449076811759707706, 0.6444004775717708799, -0.5364919789714476250 ) ) ;
#54083=AXIS2_PLACEMENT_3D ( 'NONE', #27556, #41175, #41469 ) ;
#54084=LINE ( 'NONE', #19140, #31974 ) ;
#54085=ORIENTED_EDGE ( 'NONE', *, *, #39608, .F. ) ;
#54086=AXIS2_PLACEMENT_3D ( 'NONE', #32509, #23146, #1260 ) ;
#54088=LINE ( 'NONE', #32513, #12157 ) ;
#54089=DIRECTION ( 'NONE',  ( 0.005961354470445682716, -0.6427876096865404731, -0.7660212471507180654 ) ) ;
#54090=DIRECTION ( 'NONE',  ( -0.5449076811759708816, 0.6444004775717707689, 0.5364919789714475140 ) ) ;
#54092=CARTESIAN_POINT ( 'NONE',  ( -11.33809474571162568, 2.229229656569007734, 1.014908676700488677 ) ) ;
#54093=VERTEX_POINT ( 'NONE', #52712 ) ;
#54094=DIRECTION ( 'NONE',  ( -0.7660212471507179544, -0.6427876096865405842, -0.005961354470445141482 ) ) ;
#54095=ADVANCED_FACE ( 'NONE', ( #27170 ), #22634, .F. ) ;
#54096=VECTOR ( 'NONE', #28413, 1000.000000000000114 ) ;
#54097=PLANE ( 'NONE',  #37767 ) ;
#54098=DIRECTION ( 'NONE',  ( -0.9999697198139514409, -0.000000000000000000, -0.007781995580013368816 ) ) ;
#54099=ORIENTED_EDGE ( 'NONE', *, *, #54626, .F. ) ;
#54100=EDGE_CURVE ( 'NONE', #3254, #50665, #44477, .T. ) ;
#54101=CARTESIAN_POINT ( 'NONE',  ( -16.25678841961153509, 5.305366725996514710, 2.827351461323074133 ) ) ;
#54102=PLANE ( 'NONE',  #7803 ) ;
#54103=ADVANCED_FACE ( 'NONE', ( #1614 ), #5044, .F. ) ;
#54104=VECTOR ( 'NONE', #50, 1000.000000000000227 ) ;
#54105=CARTESIAN_POINT ( 'NONE',  ( 2.072287782118878319, 0.000000000000000000, -2.950529333540147015 ) ) ;
#54106=ORIENTED_EDGE ( 'NONE', *, *, #20117, .F. ) ;
#54107=CARTESIAN_POINT ( 'NONE',  ( -16.99924723426068951, 0.000000000000000000, 13.49389102713827171 ) ) ;
#54108=VECTOR ( 'NONE', #27620, 999.9999999999998863 ) ;
#54109=ADVANCED_FACE ( 'NONE', ( #22373 ), #13817, .F. ) ;
#54110=ORIENTED_EDGE ( 'NONE', *, *, #23636, .T. ) ;
#54111=ORIENTED_EDGE ( 'NONE', *, *, #33536, .F. ) ;
#54112=VECTOR ( 'NONE', #25493, 999.9999999999998863 ) ;
#54113=VERTEX_POINT ( 'NONE', #43921 ) ;
#54115=ORIENTED_EDGE ( 'NONE', *, *, #3606, .F. ) ;
#54117=CARTESIAN_POINT ( 'NONE',  ( -8.839206115411215592, 0.000000000000000000, 5.690288575526534665 ) ) ;
#54118=VERTEX_POINT ( 'NONE', #36260 ) ;
#54119=AXIS2_PLACEMENT_3D ( 'NONE', #9018, #25225, #30028 ) ;
#54120=ORIENTED_EDGE ( 'NONE', *, *, #21161, .T. ) ;
#54121=DIRECTION ( 'NONE',  ( 0.005961354470445682716, -0.6427876096865404731, -0.7660212471507180654 ) ) ;
#54122=VERTEX_POINT ( 'NONE', #35695 ) ;
#54123=VERTEX_POINT ( 'NONE', #10423 ) ;
#54124=EDGE_CURVE ( 'NONE', #39606, #55191, #27750, .T. ) ;
#54125=VECTOR ( 'NONE', #41998, 999.9999999999998863 ) ;
#54126=ORIENTED_EDGE ( 'NONE', *, *, #13964, .T. ) ;
#54127=VECTOR ( 'NONE', #10843, 1000.000000000000227 ) ;
#54128=DIRECTION ( 'NONE',  ( 0.2426528472758541499, 0.7422098413412800966, 0.6246952433987894571 ) ) ;
#54129=DIRECTION ( 'NONE',  ( -0.7660212471507179544, -0.6427876096865405842, -0.005961354470445141482 ) ) ;
#54130=CARTESIAN_POINT ( 'NONE',  ( -15.88130887279446490, 0.000000000000000000, 3.050160814894388839 ) ) ;
#54131=CARTESIAN_POINT ( 'NONE',  ( -13.21805807743849392, 0.000000000000000000, 5.286879267240680136 ) ) ;
#54132=ADVANCED_FACE ( 'NONE', ( #6176 ), #44225, .F. ) ;
#54133=EDGE_LOOP ( 'NONE', ( #18365, #2533, #21430, #31492 ) ) ;
#54135=EDGE_LOOP ( 'NONE', ( #43664, #31508, #14183, #29600 ) ) ;
#54137=EDGE_CURVE ( 'NONE', #46078, #46605, #49024, .T. ) ;
#54138=LINE ( 'NONE', #45888, #27588 ) ;
#54140=EDGE_CURVE ( 'NONE', #34394, #28247, #23736, .T. ) ;
#54141=AXIS2_PLACEMENT_3D ( 'NONE', #17356, #38388, #46325 ) ;
#54142=DIRECTION ( 'NONE',  ( 0.5449076811759707706, 0.6444004775717708799, -0.5364919789714476250 ) ) ;
#54143=LINE ( 'NONE', #32557, #1317 ) ;
#54144=CARTESIAN_POINT ( 'NONE',  ( -10.20569392527092667, 0.000000000000000000, 2.155659566939837735 ) ) ;
#54145=DIRECTION ( 'NONE',  ( 0.007781995580012663651, 0.000000000000000000, -0.9999697198139515519 ) ) ;
#54146=ORIENTED_EDGE ( 'NONE', *, *, #48311, .F. ) ;
#54147=DIRECTION ( 'NONE',  ( 0.005002170337468016433, -0.7660444431189770143, -0.6427681459581293666 ) ) ;
#54148=ORIENTED_EDGE ( 'NONE', *, *, #36821, .T. ) ;
#54149=DIRECTION ( 'NONE',  ( 0.7660212471507180654, -0.6427876096865404731, 0.005961354470445141482 ) ) ;
#54150=CARTESIAN_POINT ( 'NONE',  ( -14.49293978885484613, 2.067327705546506245, 5.903708077246431429 ) ) ;
#54152=CARTESIAN_POINT ( 'NONE',  ( -11.20636620717317378, 0.000000000000000000, 11.32298014792380414 ) ) ;
#54153=DIRECTION ( 'NONE',  ( 0.9999697198139515519, 0.000000000000000000, 0.007781995580013368816 ) ) ;
#54154=CARTESIAN_POINT ( 'NONE',  ( -9.110551994824897193, -1.000000000000000000, 3.538847790438064411 ) ) ;
#54155=EDGE_CURVE ( 'NONE', #37866, #19153, #28020, .T. ) ;
#54156=VECTOR ( 'NONE', #10663, 999.9999999999998863 ) ;
#54157=ORIENTED_EDGE ( 'NONE', *, *, #43739, .T. ) ;
#54158=CARTESIAN_POINT ( 'NONE',  ( -11.63696731136285756, 0.000000000000000000, 6.945837973986745517 ) ) ;
#54159=CARTESIAN_POINT ( 'NONE',  ( -26.13493519185646008, 0.000000000000000000, 7.033017491833586377 ) ) ;
#54160=DIRECTION ( 'NONE',  ( 0.000000000000000000, -0.000000000000000000, -1.000000000000000000 ) ) ;
#54162=CARTESIAN_POINT ( 'NONE',  ( -9.542064456761055524, 0.000000000000000000, 10.59726798936431180 ) ) ;
#54163=PLANE ( 'NONE',  #30333 ) ;
#54164=FACE_OUTER_BOUND ( 'NONE', #48436, .T. ) ;
#54165=FACE_OUTER_BOUND ( 'NONE', #36224, .T. ) ;
#54167=DIRECTION ( 'NONE',  ( -0.6246952433987893460, -0.7422098413412802076, 0.2426528472758542054 ) ) ;
#54168=ORIENTED_EDGE ( 'NONE', *, *, #40954, .T. ) ;
#54170=EDGE_LOOP ( 'NONE', ( #20317, #10459, #36391, #14931 ) ) ;
#54171=ORIENTED_EDGE ( 'NONE', *, *, #29003, .F. ) ;
#54172=ORIENTED_EDGE ( 'NONE', *, *, #30008, .F. ) ;
#54173=ORIENTED_EDGE ( 'NONE', *, *, #18101, .T. ) ;
#54175=PLANE ( 'NONE',  #32147 ) ;
#54176=EDGE_CURVE ( 'NONE', #42837, #3166, #19771, .T. ) ;
#54177=ORIENTED_EDGE ( 'NONE', *, *, #55833, .F. ) ;
#54178=ORIENTED_EDGE ( 'NONE', *, *, #25472, .T. ) ;
#54180=ADVANCED_FACE ( 'NONE', ( #7005 ), #41618, .F. ) ;
#54181=ORIENTED_EDGE ( 'NONE', *, *, #45857, .F. ) ;
#54182=ADVANCED_FACE ( 'NONE', ( #2699 ), #2147, .F. ) ;
#54183=VECTOR ( 'NONE', #19430, 999.9999999999998863 ) ;
#54185=DIRECTION ( 'NONE',  ( 0.5364919789714477361, 0.6444004775717706579, 0.5449076811759711036 ) ) ;
#54186=DIRECTION ( 'NONE',  ( -0.5364919789714478471, 0.6444004775717705469, -0.5449076811759709926 ) ) ;
#54187=ORIENTED_EDGE ( 'NONE', *, *, #22186, .T. ) ;
#54189=AXIS2_PLACEMENT_3D ( 'NONE', #21080, #47492, #38410 ) ;
#54190=CARTESIAN_POINT ( 'NONE',  ( -17.45025494856319170, -1.975113310420660184, 3.596576296900105163 ) ) ;
#54191=ADVANCED_FACE ( 'NONE', ( #37346 ), #19190, .F. ) ;
#54192=DIRECTION ( 'NONE',  ( -0.005002170337468016433, -0.7660444431189770143, 0.6427681459581293666 ) ) ;
#54193=EDGE_CURVE ( 'NONE', #9210, #40095, #33394, .T. ) ;
#54194=LINE ( 'NONE', #6228, #48084 ) ;
#54195=CARTESIAN_POINT ( 'NONE',  ( -16.81190032086591302, 0.000000000000000000, 3.212244750653343583 ) ) ;
#54196=PLANE ( 'NONE',  #21305 ) ;
#54197=LINE ( 'NONE', #49910, #25669 ) ;
#54198=PLANE ( 'NONE',  #45746 ) ;
#54199=CARTESIAN_POINT ( 'NONE',  ( -17.36532418587302473, -0.1191753592594177458, 13.67570816655714516 ) ) ;
#54200=ORIENTED_EDGE ( 'NONE', *, *, #3393, .T. ) ;
#54201=DIRECTION ( 'NONE',  ( 0.7660212471507180654, -0.6427876096865404731, 0.005961354470445141482 ) ) ;
#54202=ORIENTED_EDGE ( 'NONE', *, *, #20200, .T. ) ;
#54203=ADVANCED_FACE ( 'NONE', ( #29111 ), #49608, .F. ) ;
#54204=CARTESIAN_POINT ( 'NONE',  ( -14.43209319853593975, 0.000000000000000000, 7.862755853857006372 ) ) ;
#54205=LINE ( 'NONE', #6783, #42271 ) ;
#54206=DIRECTION ( 'NONE',  ( -0.6427681459581293666, -0.7660444431189770143, -0.005002170337467561935 ) ) ;
#54207=FACE_OUTER_BOUND ( 'NONE', #25591, .T. ) ;
#54208=FACE_OUTER_BOUND ( 'NONE', #54298, .T. ) ;
#54209=PLANE ( 'NONE',  #53111 ) ;
#54210=EDGE_CURVE ( 'NONE', #24728, #19918, #33112, .T. ) ;
#54211=CARTESIAN_POINT ( 'NONE',  ( -27.99923088623136636, 0.000000000000000000, 7.757173251277078130 ) ) ;
#54212=CARTESIAN_POINT ( 'NONE',  ( -16.43317633868556626, -0.1191753592594197858, 13.31363028683540151 ) ) ;
#54213=DIRECTION ( 'NONE',  ( 0.000000000000000000, -0.000000000000000000, -1.000000000000000000 ) ) ;
#54214=FACE_OUTER_BOUND ( 'NONE', #17823, .T. ) ;
#54215=LINE ( 'NONE', #15568, #26394 ) ;
#54216=LINE ( 'NONE', #37746, #51363 ) ;
#54217=CARTESIAN_POINT ( 'NONE',  ( -19.99425259750860207, -1.651309408375657428, 7.158458511457326701 ) ) ;
#54218=CARTESIAN_POINT ( 'NONE',  ( -7.113423781937636470, -8.942689712534805935, 5.981468945456855479 ) ) ;
#54219=DIRECTION ( 'NONE',  ( 0.9321478471874540261, 0.000000000000000000, -0.3620778797217456546 ) ) ;
#54220=LINE ( 'NONE', #6514, #41957 ) ;
#54221=ORIENTED_EDGE ( 'NONE', *, *, #20598, .F. ) ;
#54222=DIRECTION ( 'NONE',  ( -0.005002170337468016433, -0.7660444431189770143, 0.6427681459581293666 ) ) ;
#54223=ORIENTED_EDGE ( 'NONE', *, *, #21905, .T. ) ;
#54224=CARTESIAN_POINT ( 'NONE',  ( -11.22056963685719211, 0.000000000000000000, 1.239771416285661010 ) ) ;
#54225=FACE_OUTER_BOUND ( 'NONE', #52108, .T. ) ;
#54226=AXIS2_PLACEMENT_3D ( 'NONE', #20546, #25095, #42408 ) ;
#54227=VERTEX_POINT ( 'NONE', #37094 ) ;
#54228=FACE_OUTER_BOUND ( 'NONE', #4652, .T. ) ;
#54229=EDGE_CURVE ( 'NONE', #43270, #27291, #54662, .T. ) ;
#54231=ORIENTED_EDGE ( 'NONE', *, *, #31837, .T. ) ;
#54232=DIRECTION ( 'NONE',  ( -0.9999697198139514409, -0.000000000000000000, -0.007781995580013368816 ) ) ;
#54233=ORIENTED_EDGE ( 'NONE', *, *, #35323, .T. ) ;
#54234=VERTEX_POINT ( 'NONE', #37929 ) ;
#54235=ORIENTED_EDGE ( 'NONE', *, *, #48483, .F. ) ;
#54236=PLANE ( 'NONE',  #37482 ) ;
#54237=CARTESIAN_POINT ( 'NONE',  ( -18.67280312195969216, 3.686347215771509145, 10.18439578408527346 ) ) ;
#54238=CARTESIAN_POINT ( 'NONE',  ( -11.79959855975697103, 0.000000000000000000, 2.143255432519805659 ) ) ;
#54239=EDGE_CURVE ( 'NONE', #27973, #5087, #12650, .T. ) ;
#54240=EDGE_CURVE ( 'NONE', #37866, #30714, #30249, .T. ) ;
#54241=EDGE_CURVE ( 'NONE', #31, #30596, #29711, .T. ) ;
#54242=ORIENTED_EDGE ( 'NONE', *, *, #17153, .F. ) ;
#54243=ORIENTED_EDGE ( 'NONE', *, *, #42139, .F. ) ;
#54244=EDGE_CURVE ( 'NONE', #156, #38273, #4418, .T. ) ;
#54245=CARTESIAN_POINT ( 'NONE',  ( -27.06708303904391144, 0.000000000000000000, 7.395095371555332697 ) ) ;
#54246=EDGE_LOOP ( 'NONE', ( #17785, #43339, #16360, #33505 ) ) ;
#54247=PLANE ( 'NONE',  #16454 ) ;
#54248=ORIENTED_EDGE ( 'NONE', *, *, #54402, .T. ) ;
#54249=DIRECTION ( 'NONE',  ( 0.9999697198139515519, 0.000000000000000000, 0.007781995580013368816 ) ) ;
#54250=CARTESIAN_POINT ( 'NONE',  ( -11.25298721152418935, -0.1191753592594192307, 4.463504735373795995 ) ) ;
#54251=ORIENTED_EDGE ( 'NONE', *, *, #36134, .F. ) ;
#54252=DIRECTION ( 'NONE',  ( 0.6427681459581294776, -0.7660444431189769032, 0.005002170337467562802 ) ) ;
#54253=ADVANCED_FACE ( 'NONE', ( #20868 ), #47858, .F. ) ;
#54254=EDGE_CURVE ( 'NONE', #8862, #21764, #25699, .T. ) ;
#54255=DIRECTION ( 'NONE',  ( -0.005961354470445682716, -0.6427876096865404731, 0.7660212471507180654 ) ) ;
#54256=EDGE_LOOP ( 'NONE', ( #43557, #39922, #55499, #26577 ) ) ;
#54257=DIRECTION ( 'NONE',  ( 0.7660212471507180654, -0.6427876096865404731, 0.005961354470445141482 ) ) ;
#54258=FACE_OUTER_BOUND ( 'NONE', #30653, .T. ) ;
#54259=EDGE_CURVE ( 'NONE', #23248, #24915, #39040, .T. ) ;
#54260=DIRECTION ( 'NONE',  ( 0.007781995580012662783, 0.000000000000000000, -0.9999697198139514409 ) ) ;
#54261=ORIENTED_EDGE ( 'NONE', *, *, #47919, .F. ) ;
#54262=EDGE_CURVE ( 'NONE', #34537, #39978, #16325, .T. ) ;
#54263=AXIS2_PLACEMENT_3D ( 'NONE', #22005, #422, #38792 ) ;
#54264=CARTESIAN_POINT ( 'NONE',  ( -16.00144900586372287, 0.000000000000000000, 4.695880149412071880 ) ) ;
#54265=CARTESIAN_POINT ( 'NONE',  ( -13.66102020062660038, 0.000000000000000000, 2.498101488705531725 ) ) ;
#54266=CARTESIAN_POINT ( 'NONE',  ( -18.66354898467281132, 0.000000000000000000, 14.21960318569776582 ) ) ;
#54267=DIRECTION ( 'NONE',  ( 0.000000000000000000, -0.000000000000000000, -1.000000000000000000 ) ) ;
#54268=CARTESIAN_POINT ( 'NONE',  ( -14.59503576111680800, 1.095915999411503750, 4.349113516364012000 ) ) ;
#54269=PLANE ( 'NONE',  #5245 ) ;
#54271=ORIENTED_EDGE ( 'NONE', *, *, #5060, .F. ) ;
#54272=LINE ( 'NONE', #15366, #3248 ) ;
#54274=ORIENTED_EDGE ( 'NONE', *, *, #4977, .F. ) ;
#54275=FACE_OUTER_BOUND ( 'NONE', #22551, .T. ) ;
#54276=CARTESIAN_POINT ( 'NONE',  ( -9.908141408373387193, -0.1191753592594197858, 10.77908512878318703 ) ) ;
#54277=LINE ( 'NONE', #44932, #34950 ) ;
#54278=LINE ( 'NONE', #32689, #17863 ) ;
#54279=DIRECTION ( 'NONE',  ( 0.000000000000000000, 0.000000000000000000, 1.000000000000000000 ) ) ;
#54280=ORIENTED_EDGE ( 'NONE', *, *, #51883, .F. ) ;
#54281=ORIENTED_EDGE ( 'NONE', *, *, #53683, .T. ) ;
#54282=DIRECTION ( 'NONE',  ( 0.000000000000000000, -1.000000000000000000, 0.000000000000000000 ) ) ;
#54283=EDGE_CURVE ( 'NONE', #53425, #32666, #4135, .T. ) ;
#54284=FACE_OUTER_BOUND ( 'NONE', #24996, .T. ) ;
#54285=EDGE_LOOP ( 'NONE', ( #55926, #24865, #4951, #11067 ) ) ;
#54286=CARTESIAN_POINT ( 'NONE',  ( -19.07558811344151906, 0.000000000000000000, 7.457287032919146519 ) ) ;
#54287=EDGE_CURVE ( 'NONE', #36870, #34792, #16920, .T. ) ;
#54288=EDGE_LOOP ( 'NONE', ( #6404, #55649, #30603, #24543 ) ) ;
#54289=CARTESIAN_POINT ( 'NONE',  ( -17.46532115785441519, 0.000000000000000000, 13.67492996699914265 ) ) ;
#54290=ORIENTED_EDGE ( 'NONE', *, *, #21168, .F. ) ;
#54291=VERTEX_POINT ( 'NONE', #47267 ) ;
#54292=LINE ( 'NONE', #7166, #29301 ) ;
#54293=FACE_OUTER_BOUND ( 'NONE', #40900, .T. ) ;
#54295=EDGE_CURVE ( 'NONE', #6407, #49583, #8113, .T. ) ;
#54296=ADVANCED_FACE ( 'NONE', ( #42180 ), #56096, .F. ) ;
#54297=EDGE_CURVE ( 'NONE', #9050, #35406, #7844, .T. ) ;
#54298=EDGE_LOOP ( 'NONE', ( #55432, #29594, #18711, #21342 ) ) ;
#54299=VECTOR ( 'NONE', #1177, 1000.000000000000227 ) ;
#54300=LINE ( 'NONE', #32710, #53877 ) ;
#54301=ORIENTED_EDGE ( 'NONE', *, *, #44059, .T. ) ;
#54302=ADVANCED_FACE ( 'NONE', ( #33943 ), #38782, .F. ) ;
#54303=ORIENTED_EDGE ( 'NONE', *, *, #23792, .T. ) ;
#54304=VERTEX_POINT ( 'NONE', #16614 ) ;
#54305=LINE ( 'NONE', #40958, #50382 ) ;
#54306=VERTEX_POINT ( 'NONE', #25418 ) ;
#54307=DIRECTION ( 'NONE',  ( 0.000000000000000000, -1.000000000000000000, 0.000000000000000000 ) ) ;
#54308=ORIENTED_EDGE ( 'NONE', *, *, #20159, .T. ) ;
#54309=DIRECTION ( 'NONE',  ( -0.5449076811759708816, 0.6444004775717707689, 0.5364919789714475140 ) ) ;
#54310=DIRECTION ( 'NONE',  ( -0.5364919789714478471, 0.6444004775717705469, -0.5449076811759709926 ) ) ;
#54311=ORIENTED_EDGE ( 'NONE', *, *, #54776, .T. ) ;
#54312=CARTESIAN_POINT ( 'NONE',  ( 2.072287782118878319, 0.000000000000000000, -2.950529333540147015 ) ) ;
#54313=VERTEX_POINT ( 'NONE', #42727 ) ;
#54314=EDGE_CURVE ( 'NONE', #14066, #24768, #3825, .T. ) ;
#54315=EDGE_CURVE ( 'NONE', #22478, #34831, #38478, .T. ) ;
#54316=DIRECTION ( 'NONE',  ( 0.007781995580012663651, 0.000000000000000000, -0.9999697198139515519 ) ) ;
#54317=LINE ( 'NONE', #33322, #10283 ) ;
#54318=DIRECTION ( 'NONE',  ( -0.9999697198139514409, -0.000000000000000000, -0.007781995580013368816 ) ) ;
#54319=LINE ( 'NONE', #54052, #45662 ) ;
#54320=EDGE_CURVE ( 'NONE', #6114, #50554, #27369, .T. ) ;
#54321=DIRECTION ( 'NONE',  ( -0.6427681459581293666, -0.7660444431189770143, -0.005002170337467561935 ) ) ;
#54322=CARTESIAN_POINT ( 'NONE',  ( -18.19747506107908563, 0.000000000000000000, 14.03856424583689311 ) ) ;
#54323=DIRECTION ( 'NONE',  ( -0.5449076811759708816, 0.6444004775717707689, 0.5364919789714475140 ) ) ;
#54324=EDGE_LOOP ( 'NONE', ( #30979, #2899, #42588, #44125, #12963, #32930, #24291, #6391 ) ) ;
#54325=EDGE_CURVE ( 'NONE', #32862, #8418, #48392, .T. ) ;
#54326=EDGE_LOOP ( 'NONE', ( #11398, #7639, #24301, #34110 ) ) ;
#54328=CARTESIAN_POINT ( 'NONE',  ( -14.20280369269832832, 0.000000000000000000, 12.40765738797303719 ) ) ;
#54329=LINE ( 'NONE', #6932, #42097 ) ;
#54330=EDGE_CURVE ( 'NONE', #23038, #52596, #26530, .T. ) ;
#54331=CARTESIAN_POINT ( 'NONE',  ( -8.276713462897552276, 0.000000000000000000, 6.433330163025533288 ) ) ;
#54332=DIRECTION ( 'NONE',  ( 0.000000000000000000, 1.000000000000000000, 0.000000000000000000 ) ) ;
#54333=ORIENTED_EDGE ( 'NONE', *, *, #40083, .F. ) ;
#54334=CARTESIAN_POINT ( 'NONE',  ( -21.47263955680318404, 0.000000000000000000, 5.022634149262071190 ) ) ;
#54335=CARTESIAN_POINT ( 'NONE',  ( -12.33850799832341849, 0.000000000000000000, 11.68350162852954632 ) ) ;
#54336=ORIENTED_EDGE ( 'NONE', *, *, #21970, .F. ) ;
#54337=LINE ( 'NONE', #23419, #18433 ) ;
#54338=CARTESIAN_POINT ( 'NONE',  ( -14.94760462649100496, 0.000000000000000000, 2.488088991209854051 ) ) ;
#54339=ORIENTED_EDGE ( 'NONE', *, *, #44107, .F. ) ;
#54343=LINE ( 'NONE', #45823, #37698 ) ;
#54344=FACE_OUTER_BOUND ( 'NONE', #37191, .T. ) ;
#54346=ORIENTED_EDGE ( 'NONE', *, *, #11911, .F. ) ;
#54347=ORIENTED_EDGE ( 'NONE', *, *, #14530, .F. ) ;
#54348=CARTESIAN_POINT ( 'NONE',  ( -10.87762927220137144, 0.000000000000000000, 3.089100606534142202 ) ) ;
#54349=FACE_OUTER_BOUND ( 'NONE', #38838, .T. ) ;
#54350=LINE ( 'NONE', #29357, #27893 ) ;
#54351=LINE ( 'NONE', #6660, #8697 ) ;
#54352=CARTESIAN_POINT ( 'NONE',  ( -22.76109218059357175, -4.889348428825661230, 13.54736664680453551 ) ) ;
#54353=LINE ( 'NONE', #23158, #44872 ) ;
#54354=ORIENTED_EDGE ( 'NONE', *, *, #41777, .T. ) ;
#54355=CARTESIAN_POINT ( 'NONE',  ( -19.59569683186026268, 0.000000000000000000, 14.58168106541950948 ) ) ;
#54356=CARTESIAN_POINT ( 'NONE',  ( -14.20280369269832832, 0.000000000000000000, 12.40765738797303719 ) ) ;
#54357=DIRECTION ( 'NONE',  ( 0.007781995580012663651, 0.000000000000000000, -0.9999697198139515519 ) ) ;
#54360=DIRECTION ( 'NONE',  ( -0.6427681459581293666, -0.7660444431189770143, -0.005002170337467561935 ) ) ;
#54361=DIRECTION ( 'NONE',  ( -0.6427681459581293666, -0.7660444431189770143, -0.005002170337467561935 ) ) ;
#54362=EDGE_CURVE ( 'NONE', #14416, #33688, #43854, .T. ) ;
#54363=VERTEX_POINT ( 'NONE', #43572 ) ;
#54364=CARTESIAN_POINT ( 'NONE',  ( -18.78795273252095654, 0.000000000000000000, 4.504868919509038783 ) ) ;
#54365=ORIENTED_EDGE ( 'NONE', *, *, #7102, .F. ) ;
#54367=EDGE_CURVE ( 'NONE', #45853, #38452, #52646, .T. ) ;
#54368=ORIENTED_EDGE ( 'NONE', *, *, #41910, .F. ) ;
#54369=ORIENTED_EDGE ( 'NONE', *, *, #54470, .T. ) ;
#54370=ORIENTED_EDGE ( 'NONE', *, *, #12795, .T. ) ;
#54371=VERTEX_POINT ( 'NONE', #14344 ) ;
#54373=VERTEX_POINT ( 'NONE', #53250 ) ;
#54374=ORIENTED_EDGE ( 'NONE', *, *, #19125, .T. ) ;
#54375=PLANE ( 'NONE',  #46757 ) ;
#54376=VERTEX_POINT ( 'NONE', #13752 ) ;
#54377=ORIENTED_EDGE ( 'NONE', *, *, #24391, .T. ) ;
#54378=EDGE_LOOP ( 'NONE', ( #15998, #39486, #15437 ) ) ;
#54379=CARTESIAN_POINT ( 'NONE',  ( -15.89073401941919883, -0.1191753592594213818, 3.319416507920406989 ) ) ;
#54380=LINE ( 'NONE', #15758, #3082 ) ;
#54381=LINE ( 'NONE', #28551, #2384 ) ;
#54382=PLANE ( 'NONE',  #29560 ) ;
#54384=CARTESIAN_POINT ( 'NONE',  ( -11.29627228906843150, -0.03739765774599676518, 1.207800969688126891 ) ) ;
#54385=EDGE_LOOP ( 'NONE', ( #32971, #53412, #53795 ) ) ;
#54386=ORIENTED_EDGE ( 'NONE', *, *, #28161, .T. ) ;
#54387=LINE ( 'NONE', #32807, #14085 ) ;
#54388=DIRECTION ( 'NONE',  ( 0.005961354470445682716, -0.6427876096865404731, -0.7660212471507180654 ) ) ;
#54389=EDGE_CURVE ( 'NONE', #50804, #30507, #22296, .T. ) ;
#54390=CARTESIAN_POINT ( 'NONE',  ( -14.56888064431065821, -0.1191753592594197858, 12.58947452739191064 ) ) ;
#54391=DIRECTION ( 'NONE',  ( 0.5449076811759707706, 0.6444004775717708799, -0.5364919789714476250 ) ) ;
#54392=ADVANCED_FACE ( 'NONE', ( #31656 ), #4677, .F. ) ;
#54393=DIRECTION ( 'NONE',  ( -0.7660212471507179544, -0.6427876096865405842, -0.005961354470445141482 ) ) ;
#54394=CARTESIAN_POINT ( 'NONE',  ( -11.70248683415050550, 9.283552190907606416, 1.327269728845983821 ) ) ;
#54395=EDGE_LOOP ( 'NONE', ( #2195, #22479, #50809, #10132 ) ) ;
#54396=CARTESIAN_POINT ( 'NONE',  ( -18.67619601524082285, 0.000000000000000000, 3.936400510096834893 ) ) ;
#54397=ADVANCED_FACE ( 'NONE', ( #4966 ), #35092, .F. ) ;
#54398=EDGE_LOOP ( 'NONE', ( #28062, #31015, #48439, #1094 ) ) ;
#54399=PLANE ( 'NONE',  #37395 ) ;
#54400=CARTESIAN_POINT ( 'NONE',  ( 2.072287782118878319, 0.000000000000000000, -2.950529333540147015 ) ) ;
#54401=CARTESIAN_POINT ( 'NONE',  ( -16.99924723426068951, 0.000000000000000000, 13.49389102713827171 ) ) ;
#54402=EDGE_CURVE ( 'NONE', #15599, #29943, #23130, .T. ) ;
#54403=CARTESIAN_POINT ( 'NONE',  ( -10.28686539055373395, 0.000000000000000000, 0.6776995926011265547 ) ) ;
#54404=DIRECTION ( 'NONE',  ( -0.3620778797217457656, 0.000000000000000000, -0.9321478471874539151 ) ) ;
#54405=AXIS2_PLACEMENT_3D ( 'NONE', #4225, #21541, #38854 ) ;
#54406=ORIENTED_EDGE ( 'NONE', *, *, #25614, .T. ) ;
#54407=CARTESIAN_POINT ( 'NONE',  ( -11.74614849678306427, -0.1159828484229813300, 7.780976552696367676 ) ) ;
#54408=DIRECTION ( 'NONE',  ( -0.6427681459581293666, -0.7660444431189770143, -0.005002170337467561935 ) ) ;
#54409=CARTESIAN_POINT ( 'NONE',  ( -17.77025923324963230, 0.4483081953215036219, 4.519643408181552857 ) ) ;
#54410=LINE ( 'NONE', #15509, #44571 ) ;
#54411=LINE ( 'NONE', #23759, #28490 ) ;
#54412=FACE_OUTER_BOUND ( 'NONE', #22, .T. ) ;
#54413=DIRECTION ( 'NONE',  ( -0.7660212471507179544, -0.6427876096865405842, -0.005961354470445141482 ) ) ;
#54414=CARTESIAN_POINT ( 'NONE',  ( -25.20123094555300369, 0.000000000000000000, 6.470945668149052032 ) ) ;
#54415=CARTESIAN_POINT ( 'NONE',  ( -18.29747203306047609, -0.1191753592594177458, 14.03778604627889059 ) ) ;
#54416=EDGE_CURVE ( 'NONE', #50902, #4591, #961, .T. ) ;
#54417=ORIENTED_EDGE ( 'NONE', *, *, #6384, .T. ) ;
#54418=EDGE_CURVE ( 'NONE', #428, #11634, #52937, .T. ) ;
#54419=ORIENTED_EDGE ( 'NONE', *, *, #18748, .T. ) ;
#54420=EDGE_CURVE ( 'NONE', #54876, #9595, #21994, .T. ) ;
#54421=ADVANCED_FACE ( 'NONE', ( #48961 ), #18879, .F. ) ;
#54423=VERTEX_POINT ( 'NONE', #14597 ) ;
#54424=EDGE_LOOP ( 'NONE', ( #39916, #15213, #9502, #9818 ) ) ;
#54427=CARTESIAN_POINT ( 'NONE',  ( -9.167413235801063820, -10.93230953041516429, 6.779308203112875297 ) ) ;
#54428=LINE ( 'NONE', #28611, #34006 ) ;
#54429=ORIENTED_EDGE ( 'NONE', *, *, #7430, .F. ) ;
#54430=DIRECTION ( 'NONE',  ( 0.9999697198139515519, 0.000000000000000000, 0.007781995580013368816 ) ) ;
#54431=ORIENTED_EDGE ( 'NONE', *, *, #23120, .F. ) ;
#54432=ORIENTED_EDGE ( 'NONE', *, *, #45423, .T. ) ;
#54433=ADVANCED_FACE ( 'NONE', ( #18026 ), #26262, .F. ) ;
#54434=AXIS2_PLACEMENT_3D ( 'NONE', #54675, #15782, #16083 ) ;
#54436=PLANE ( 'NONE',  #17350 ) ;
#54437=CARTESIAN_POINT ( 'NONE',  ( -18.19747506107908563, 0.000000000000000000, 14.03856424583689311 ) ) ;
#54438=EDGE_LOOP ( 'NONE', ( #52028, #49601, #32848, #11169 ) ) ;
#54439=DIRECTION ( 'NONE',  ( 0.007781995580012663651, 0.000000000000000000, -0.9999697198139515519 ) ) ;
#54440=ORIENTED_EDGE ( 'NONE', *, *, #9721, .F. ) ;
#54441=CARTESIAN_POINT ( 'NONE',  ( -17.66287670277056066, 0.000000000000000000, 5.052282604713799863 ) ) ;
#54442=PLANE ( 'NONE',  #20279 ) ;
#54443=FACE_OUTER_BOUND ( 'NONE', #45659, .T. ) ;
#54444=CARTESIAN_POINT ( 'NONE',  ( -18.22472998780914466, -0.6798977022406571535, 3.938732862525397671 ) ) ;
#54445=CARTESIAN_POINT ( 'NONE',  ( -9.838958146463953724, -0.1191753592594204242, 1.889184547873473452 ) ) ;
#54446=FACE_OUTER_BOUND ( 'NONE', #45840, .T. ) ;
#54447=DIRECTION ( 'NONE',  ( -0.3620778797217457101, 0.000000000000000000, -0.9321478471874540261 ) ) ;
#54448=DIRECTION ( 'NONE',  ( 0.007781995580012663651, -3.146120232559066537E-19, -0.9999697198139514409 ) ) ;
#54449=ORIENTED_EDGE ( 'NONE', *, *, #9774, .F. ) ;
#54450=CARTESIAN_POINT ( 'NONE',  ( -15.93384482199843788, -0.1191753592594196193, 8.859062056786873640 ) ) ;
#54451=EDGE_LOOP ( 'NONE', ( #22193, #39623, #8214, #17733 ) ) ;
#54452=AXIS2_PLACEMENT_3D ( 'NONE', #16181, #33504, #46258 ) ;
#54454=DIRECTION ( 'NONE',  ( -0.5449076811759708816, 0.6444004775717707689, 0.5364919789714475140 ) ) ;
#54455=DIRECTION ( 'NONE',  ( -0.005961354470445682716, -0.6427876096865404731, 0.7660212471507180654 ) ) ;
#54456=ADVANCED_FACE ( 'NONE', ( #410 ), #30808, .F. ) ;
#54457=DIRECTION ( 'NONE',  ( -0.005002170337468016433, -0.7660444431189770143, 0.6427681459581293666 ) ) ;
#54458=CARTESIAN_POINT ( 'NONE',  ( -22.40478740399063895, 0.000000000000000000, 5.384712028983816623 ) ) ;
#54459=FACE_OUTER_BOUND ( 'NONE', #39590, .T. ) ;
#54460=ORIENTED_EDGE ( 'NONE', *, *, #38642, .F. ) ;
#54461=DIRECTION ( 'NONE',  ( 0.5449076811759707706, 0.6444004775717708799, -0.5364919789714476250 ) ) ;
#54462=DIRECTION ( 'NONE',  ( 0.000000000000000000, -1.000000000000000000, 0.000000000000000000 ) ) ;
#54463=DIRECTION ( 'NONE',  ( 0.007781995580012662783, 0.000000000000000000, -0.9999697198139514409 ) ) ;
#54464=DIRECTION ( 'NONE',  ( 0.000000000000000000, -0.000000000000000000, -1.000000000000000000 ) ) ;
#54465=CARTESIAN_POINT ( 'NONE',  ( -26.13493519185646008, 0.000000000000000000, 7.033017491833586377 ) ) ;
#54466=EDGE_CURVE ( 'NONE', #50886, #34260, #10652, .T. ) ;
#54467=VECTOR ( 'NONE', #30737, 1000.000000000000114 ) ;
#54468=CARTESIAN_POINT ( 'NONE',  ( -15.88405162580815855, 3.200641362704010007, 2.749719590951118953 ) ) ;
#54469=DIRECTION ( 'NONE',  ( -0.005961354470445682716, -0.6427876096865404731, 0.7660212471507180654 ) ) ;
#54470=EDGE_CURVE ( 'NONE', #51326, #33913, #50353, .T. ) ;
#54471=CARTESIAN_POINT ( 'NONE',  ( -13.01363368085442040, 0.000000000000000000, 4.719132019136131007 ) ) ;
#54472=ADVANCED_FACE ( 'NONE', ( #11465 ), #27668, .F. ) ;
#54473=DIRECTION ( 'NONE',  ( 0.007781995580012662783, 0.000000000000000000, -0.9999697198139514409 ) ) ;
#54475=VECTOR ( 'NONE', #38014, 999.9999999999998863 ) ;
#54476=DIRECTION ( 'NONE',  ( 0.007781995580012663651, -3.146120232559066537E-19, -0.9999697198139514409 ) ) ;
#54477=ORIENTED_EDGE ( 'NONE', *, *, #45037, .T. ) ;
#54478=LINE ( 'NONE', #20418, #52101 ) ;
#54479=CARTESIAN_POINT ( 'NONE',  ( -11.40636015113596180, 0.000000000000000000, 11.32142374880780089 ) ) ;
#54480=ADVANCED_FACE ( 'NONE', ( #54066 ), #1799, .F. ) ;
#54481=ORIENTED_EDGE ( 'NONE', *, *, #37837, .T. ) ;
#54482=EDGE_CURVE ( 'NONE', #18846, #21097, #45518, .T. ) ;
#54483=VERTEX_POINT ( 'NONE', #40731 ) ;
#54484=CARTESIAN_POINT ( 'NONE',  ( -14.01701317841955508, 0.000000000000000000, 2.326005055450897085 ) ) ;
#54485=EDGE_CURVE ( 'NONE', #18056, #17655, #49533, .T. ) ;
#54486=VERTEX_POINT ( 'NONE', #37281 ) ;
#54487=ORIENTED_EDGE ( 'NONE', *, *, #12708, .T. ) ;
#54489=DIRECTION ( 'NONE',  ( -0.7660212471507179544, -0.6427876096865405842, -0.005961354470445141482 ) ) ;
#54491=DIRECTION ( 'NONE',  ( 0.3313982828793700097, 0.4028455766673915694, 0.8531650599175529814 ) ) ;
#54492=EDGE_CURVE ( 'NONE', #38597, #10075, #24497, .T. ) ;
#54493=AXIS2_PLACEMENT_3D ( 'NONE', #20956, #55603, #37438 ) ;
#54494=VECTOR ( 'NONE', #27502, 1000.000000000000227 ) ;
#54495=VERTEX_POINT ( 'NONE', #14881 ) ;
#54496=ORIENTED_EDGE ( 'NONE', *, *, #45925, .F. ) ;
#54497=EDGE_CURVE ( 'NONE', #48860, #3819, #23949, .T. ) ;
#54498=LINE ( 'NONE', #11901, #52964 ) ;
#54500=VERTEX_POINT ( 'NONE', #10892 ) ;
#54501=DIRECTION ( 'NONE',  ( 0.005002170337468016433, -0.7660444431189770143, -0.6427681459581293666 ) ) ;
#54502=EDGE_LOOP ( 'NONE', ( #49412, #44438, #17933, #6042 ) ) ;
#54503=DIRECTION ( 'NONE',  ( 0.005961354470445682716, -0.6427876096865404731, -0.7660212471507180654 ) ) ;
#54504=DIRECTION ( 'NONE',  ( 0.005961354470445682716, -0.6427876096865404731, -0.7660212471507180654 ) ) ;
#54505=ORIENTED_EDGE ( 'NONE', *, *, #30032, .F. ) ;
#54508=DIRECTION ( 'NONE',  ( 0.6427681459581294776, -0.7660444431189769032, 0.005002170337467562802 ) ) ;
#54509=ORIENTED_EDGE ( 'NONE', *, *, #1849, .T. ) ;
#54510=PLANE ( 'NONE',  #14951 ) ;
#54511=LINE ( 'NONE', #3121, #4906 ) ;
#54512=DIRECTION ( 'NONE',  ( -0.005961354470445682716, -0.6427876096865404731, 0.7660212471507180654 ) ) ;
#54513=EDGE_LOOP ( 'NONE', ( #48885, #53538, #34120, #26510 ) ) ;
#54514=PLANE ( 'NONE',  #45550 ) ;
#54515=CARTESIAN_POINT ( 'NONE',  ( -17.74404816805336793, 0.000000000000000000, 3.574322630375089460 ) ) ;
#54516=DIRECTION ( 'NONE',  ( 0.007781995580012662783, 0.000000000000000000, -0.9999697198139514409 ) ) ;
#54517=EDGE_CURVE ( 'NONE', #3951, #20306, #2072, .T. ) ;
#54518=CARTESIAN_POINT ( 'NONE',  ( -6.264213140240936006, -6.015707657378981388, -0.7851404584205251558 ) ) ;
#54519=FACE_OUTER_BOUND ( 'NONE', #46603, .T. ) ;
#54520=CARTESIAN_POINT ( 'NONE',  ( -25.20123094555300369, 0.000000000000000000, 6.470945668149052032 ) ) ;
#54521=DIRECTION ( 'NONE',  ( 0.000000000000000000, -0.000000000000000000, -1.000000000000000000 ) ) ;
#54522=EDGE_LOOP ( 'NONE', ( #47116, #13794, #7331, #9551 ) ) ;
#54523=CARTESIAN_POINT ( 'NONE',  ( -27.06708303904391144, 0.000000000000000000, 7.395095371555332697 ) ) ;
#54525=ORIENTED_EDGE ( 'NONE', *, *, #21878, .T. ) ;
#54526=DIRECTION ( 'NONE',  ( -0.5364919789714478471, 0.6444004775717705469, -0.5449076811759709926 ) ) ;
#54527=CARTESIAN_POINT ( 'NONE',  ( -28.92982233430281980, 0.000000000000000000, 7.919257187036034651 ) ) ;
#54528=VECTOR ( 'NONE', #18903, 999.9999999999998863 ) ;
#54529=VECTOR ( 'NONE', #556, 1000.000000000000227 ) ;
#54530=CARTESIAN_POINT ( 'NONE',  ( -13.48401868470607035, 0.000000000000000000, 5.454135513883649367 ) ) ;
#54531=DIRECTION ( 'NONE',  ( 0.005002170337468016433, -0.7660444431189770143, -0.6427681459581293666 ) ) ;
#54532=EDGE_CURVE ( 'NONE', #18137, #40042, #20236, .T. ) ;
#54533=CARTESIAN_POINT ( 'NONE',  ( -14.10280672071693431, -0.1191753592594197858, 12.40843558753103792 ) ) ;
#54534=VERTEX_POINT ( 'NONE', #19706 ) ;
#54535=VECTOR ( 'NONE', #439, 1000.000000000000227 ) ;
#54536=EDGE_LOOP ( 'NONE', ( #6181, #757 ) ) ;
#54537=FACE_OUTER_BOUND ( 'NONE', #51752, .T. ) ;
#54538=DIRECTION ( 'NONE',  ( 0.9999697198139515519, 0.000000000000000000, 0.007781995580013368816 ) ) ;
#54539=PLANE ( 'NONE',  #37435 ) ;
#54540=VERTEX_POINT ( 'NONE', #23666 ) ;
#54541=EDGE_CURVE ( 'NONE', #3706, #21619, #53763, .T. ) ;
#54542=DIRECTION ( 'NONE',  ( 0.005961354470445682716, -0.6427876096865404731, -0.7660212471507180654 ) ) ;
#54543=ORIENTED_EDGE ( 'NONE', *, *, #10531, .T. ) ;
#54544=DIRECTION ( 'NONE',  ( 0.9999697198139515519, 0.000000000000000000, 0.007781995580013368816 ) ) ;
#54545=AXIS2_PLACEMENT_3D ( 'NONE', #53486, #31901, #19691 ) ;
#54546=EDGE_CURVE ( 'NONE', #21903, #5703, #24246, .T. ) ;
#54547=ORIENTED_EDGE ( 'NONE', *, *, #10054, .T. ) ;
#54548=ORIENTED_EDGE ( 'NONE', *, *, #32410, .F. ) ;
#54549=DIRECTION ( 'NONE',  ( 0.007781995580012663651, 0.000000000000000000, -0.9999697198139515519 ) ) ;
#54550=DIRECTION ( 'NONE',  ( 0.005961354470445682716, -0.6427876096865404731, -0.7660212471507180654 ) ) ;
#54551=DIRECTION ( 'NONE',  ( -0.9999697198139514409, -0.000000000000000000, -0.007781995580013368816 ) ) ;
#54552=ORIENTED_EDGE ( 'NONE', *, *, #24359, .F. ) ;
#54553=EDGE_CURVE ( 'NONE', #34361, #51735, #28206, .T. ) ;
#54554=PLANE ( 'NONE',  #17477 ) ;
#54556=ORIENTED_EDGE ( 'NONE', *, *, #39039, .T. ) ;
#54557=ADVANCED_FACE ( 'NONE', ( #2906 ), #46091, .F. ) ;
#54558=EDGE_LOOP ( 'NONE', ( #28904, #45106, #40426, #3741 ) ) ;
#54559=FACE_OUTER_BOUND ( 'NONE', #52780, .T. ) ;
#54560=ORIENTED_EDGE ( 'NONE', *, *, #8334, .F. ) ;
#54561=FACE_OUTER_BOUND ( 'NONE', #15716, .T. ) ;
#54562=EDGE_LOOP ( 'NONE', ( #24877, #21633, #20782, #35739 ) ) ;
#54563=FACE_OUTER_BOUND ( 'NONE', #9684, .T. ) ;
#54564=DIRECTION ( 'NONE',  ( -0.7660212471507179544, -0.6427876096865405842, -0.005961354470445141482 ) ) ;
#54565=VECTOR ( 'NONE', #13996, 1000.000000000000227 ) ;
#54566=AXIS2_PLACEMENT_3D ( 'NONE', #22210, #22501, #39237 ) ;
#54567=ORIENTED_EDGE ( 'NONE', *, *, #40485, .F. ) ;
#54569=ORIENTED_EDGE ( 'NONE', *, *, #42886, .T. ) ;
#54570=LINE ( 'NONE', #33019, #31915 ) ;
#54571=CARTESIAN_POINT ( 'NONE',  ( -22.40634380310664397, 0.000000000000000000, 5.584705972946605534 ) ) ;
#54572=AXIS2_PLACEMENT_3D ( 'NONE', #55958, #13065, #21004 ) ;
#54573=CARTESIAN_POINT ( 'NONE',  ( -8.875996589204540044, 0.000000000000000000, 10.41778544861944233 ) ) ;
#54574=CARTESIAN_POINT ( 'NONE',  ( -19.88509817834021476, 3.524445264749009876, 4.293530908292650494 ) ) ;
#54575=FACE_OUTER_BOUND ( 'NONE', #35253, .T. ) ;
#54576=FACE_OUTER_BOUND ( 'NONE', #6820, .T. ) ;
#54577=VERTEX_POINT ( 'NONE', #54331 ) ;
#54578=ADVANCED_FACE ( 'NONE', ( #15423 ), #10347, .F. ) ;
#54579=ORIENTED_EDGE ( 'NONE', *, *, #35191, .T. ) ;
#54580=CARTESIAN_POINT ( 'NONE',  ( -10.89906530112762972, 0.000000000000000000, 5.843584288633468127 ) ) ;
#54581=DIRECTION ( 'NONE',  ( -0.005961354470445682716, -0.6427876096865404731, 0.7660212471507180654 ) ) ;
#54582=AXIS2_PLACEMENT_3D ( 'NONE', #20671, #24618, #8166 ) ;
#54583=EDGE_CURVE ( 'NONE', #44507, #14930, #6111, .T. ) ;
#54584=LINE ( 'NONE', #50636, #29502 ) ;
#54586=DIRECTION ( 'NONE',  ( -0.005002170337468016433, -0.7660444431189770143, 0.6427681459581293666 ) ) ;
#54587=FACE_OUTER_BOUND ( 'NONE', #7718, .T. ) ;
#54588=ORIENTED_EDGE ( 'NONE', *, *, #45461, .T. ) ;
#54589=ADVANCED_FACE ( 'NONE', ( #55440 ), #30174, .F. ) ;
#54590=CARTESIAN_POINT ( 'NONE',  ( -9.121988873521557295, -2.596375463177813536, 3.509404230218840404 ) ) ;
#54591=DIRECTION ( 'NONE',  ( 0.007781995580012663651, 0.000000000000000000, -0.9999697198139515519 ) ) ;
#54592=ORIENTED_EDGE ( 'NONE', *, *, #41247, .F. ) ;
#54593=CARTESIAN_POINT ( 'NONE',  ( -9.905246062020005127, 7.542634850262289525, 0.6291603783969644814 ) ) ;
#54594=DIRECTION ( 'NONE',  ( 0.005002170337468016433, -0.7660444431189770143, -0.6427681459581293666 ) ) ;
#54595=ORIENTED_EDGE ( 'NONE', *, *, #34476, .T. ) ;
#54596=EDGE_CURVE ( 'NONE', #23008, #52604, #4058, .T. ) ;
#54597=EDGE_CURVE ( 'NONE', #44414, #2010, #29903, .T. ) ;
#54600=DIRECTION ( 'NONE',  ( 0.007781995580012663651, 0.000000000000000000, -0.9999697198139515519 ) ) ;
#54601=DIRECTION ( 'NONE',  ( -0.005002170337468016433, -0.7660444431189770143, 0.6427681459581293666 ) ) ;
#54602=AXIS2_PLACEMENT_3D ( 'NONE', #30567, #46502, #55314 ) ;
#54603=DIRECTION ( 'NONE',  ( 0.005961354470445682716, -0.6427876096865404731, -0.7660212471507180654 ) ) ;
#54604=PLANE ( 'NONE',  #28345 ) ;
#54605=EDGE_LOOP ( 'NONE', ( #28642, #8918, #13085, #1078 ) ) ;
#54607=FACE_OUTER_BOUND ( 'NONE', #39897, .T. ) ;
#54608=CARTESIAN_POINT ( 'NONE',  ( -10.74029228357944987, 0.000000000000000000, 11.14194120806293320 ) ) ;
#54609=AXIS2_PLACEMENT_3D ( 'NONE', #39844, #44109, #18246 ) ;
#54611=VECTOR ( 'NONE', #520, 1000.000000000000227 ) ;
#54612=CARTESIAN_POINT ( 'NONE',  ( -17.34579682753419050, -0.1191753592594159833, 9.956070129217877707 ) ) ;
#54613=AXIS2_PLACEMENT_3D ( 'NONE', #5445, #22757, #19053 ) ;
#54614=LINE ( 'NONE', #29069, #53688 ) ;
#54615=ADVANCED_FACE ( 'NONE', ( #38126 ), #51743, .F. ) ;
#54616=CARTESIAN_POINT ( 'NONE',  ( -11.87243407472968926, 0.000000000000000000, 11.50246268866867361 ) ) ;
#54617=ORIENTED_EDGE ( 'NONE', *, *, #16421, .F. ) ;
#54618=LINE ( 'NONE', #50387, #36514 ) ;
#54619=EDGE_CURVE ( 'NONE', #25102, #46963, #29335, .T. ) ;
#54620=LINE ( 'NONE', #3247, #7861 ) ;
#54621=VECTOR ( 'NONE', #50160, 1000.000000000000227 ) ;
#54622=CARTESIAN_POINT ( 'NONE',  ( -20.54762051412559742, -2.298917212465657833, 8.436240138526766685 ) ) ;
#54623=VECTOR ( 'NONE', #40855, 999.9999999999998863 ) ;
#54624=EDGE_LOOP ( 'NONE', ( #8220, #30302, #34977, #5603 ) ) ;
#54626=EDGE_CURVE ( 'NONE', #46096, #50687, #37872, .T. ) ;
#54627=DIRECTION ( 'NONE',  ( 0.000000000000000000, -1.000000000000000000, 0.000000000000000000 ) ) ;
#54628=DIRECTION ( 'NONE',  ( -0.3620778797217456546, 0.000000000000000000, -0.9321478471874540261 ) ) ;
#54629=LINE ( 'NONE', #37611, #50199 ) ;
#54630=ORIENTED_EDGE ( 'NONE', *, *, #38784, .T. ) ;
#54631=ADVANCED_FACE ( 'NONE', ( #16543 ), #51194, .F. ) ;
#54632=CARTESIAN_POINT ( 'NONE',  ( -17.63855930251027360, 4.657758921906509642, 11.37691246524594568 ) ) ;
#54633=AXIS2_PLACEMENT_3D ( 'NONE', #18657, #32282, #49602 ) ;
#54635=EDGE_CURVE ( 'NONE', #52808, #29873, #12305, .T. ) ;
#54636=VERTEX_POINT ( 'NONE', #4359 ) ;
#54637=ORIENTED_EDGE ( 'NONE', *, *, #42598, .F. ) ;
#54638=ORIENTED_EDGE ( 'NONE', *, *, #1674, .T. ) ;
#54639=EDGE_LOOP ( 'NONE', ( #9222, #45725, #11232, #46367 ) ) ;
#54640=DIRECTION ( 'NONE',  ( 0.005961354470445682716, -0.6427876096865404731, -0.7660212471507180654 ) ) ;
#54641=ORIENTED_EDGE ( 'NONE', *, *, #8715, .F. ) ;
#54642=AXIS2_PLACEMENT_3D ( 'NONE', #40280, #45117, #36300 ) ;
#54643=ORIENTED_EDGE ( 'NONE', *, *, #7427, .F. ) ;
#54644=DIRECTION ( 'NONE',  ( 0.005961354470445682716, -0.6427876096865404731, -0.7660212471507180654 ) ) ;
#54645=ORIENTED_EDGE ( 'NONE', *, *, #11076, .F. ) ;
#54646=VECTOR ( 'NONE', #9682, 1000.000000000000000 ) ;
#54647=VERTEX_POINT ( 'NONE', #34178 ) ;
#54648=DIRECTION ( 'NONE',  ( 0.5364919789714477361, 0.6444004775717706579, 0.5449076811759711036 ) ) ;
#54649=LINE ( 'NONE', #24298, #7634 ) ;
#54650=LINE ( 'NONE', #55230, #39577 ) ;
#54651=PLANE ( 'NONE',  #24164 ) ;
#54652=AXIS2_PLACEMENT_3D ( 'NONE', #34824, #150, #11346 ) ;
#54653=ORIENTED_EDGE ( 'NONE', *, *, #555, .F. ) ;
#54654=LINE ( 'NONE', #51256, #41903 ) ;
#54655=ORIENTED_EDGE ( 'NONE', *, *, #4877, .F. ) ;
#54656=VECTOR ( 'NONE', #43771, 999.9999999999998863 ) ;
#54657=VECTOR ( 'NONE', #6780, 1000.000000000000227 ) ;
#54658=ORIENTED_EDGE ( 'NONE', *, *, #39483, .T. ) ;
#54659=LINE ( 'NONE', #25162, #34877 ) ;
#54660=CARTESIAN_POINT ( 'NONE',  ( -10.85057559606751276, 1.095915999411505526, 0.8616983219704370534 ) ) ;
#54662=LINE ( 'NONE', #54390, #9749 ) ;
#54663=VECTOR ( 'NONE', #39591, 1000.000000000000114 ) ;
#54664=VECTOR ( 'NONE', #1747, 1000.000000000000000 ) ;
#54665=LINE ( 'NONE', #45072, #54820 ) ;
#54666=DIRECTION ( 'NONE',  ( 0.6427681459581294776, -0.7660444431189769032, 0.005002170337467562802 ) ) ;
#54667=DIRECTION ( 'NONE',  ( -0.5449076811759708816, 0.6444004775717707689, 0.5364919789714475140 ) ) ;
#54668=ORIENTED_EDGE ( 'NONE', *, *, #41357, .F. ) ;
#54669=CARTESIAN_POINT ( 'NONE',  ( -9.110551994824897193, 0.000000000000000000, 3.538847790438064411 ) ) ;
#54670=ORIENTED_EDGE ( 'NONE', *, *, #10531, .F. ) ;
#54671=ADVANCED_FACE ( 'NONE', ( #33873 ), #42104, .F. ) ;
#54672=EDGE_CURVE ( 'NONE', #21642, #37323, #3210, .T. ) ;
#54673=CARTESIAN_POINT ( 'NONE',  ( -18.42572312212858776, 0.1245042932765033361, 4.242830474368576965 ) ) ;
#54674=PLANE ( 'NONE',  #50459 ) ;
#54675=CARTESIAN_POINT ( 'NONE',  ( 2.072287782118878319, 0.000000000000000000, -2.950529333540147015 ) ) ;
#54676=AXIS2_PLACEMENT_3D ( 'NONE', #20083, #7066, #11014 ) ;
#54677=DIRECTION ( 'NONE',  ( 0.9999697198139515519, 0.000000000000000000, 0.007781995580013368816 ) ) ;
#54678=EDGE_CURVE ( 'NONE', #9132, #11534, #55732, .T. ) ;
#54679=VECTOR ( 'NONE', #30005, 1000.000000000000114 ) ;
#54680=CARTESIAN_POINT ( 'NONE',  ( -20.62011252791016247, -4.565544526780660917, 12.18432007382632598 ) ) ;
#54681=EDGE_LOOP ( 'NONE', ( #38763, #25129, #44891, #2419 ) ) ;
#54682=EDGE_LOOP ( 'NONE', ( #48914, #41512, #8363, #30011 ) ) ;
#54683=CARTESIAN_POINT ( 'NONE',  ( -17.04851670312061884, -5.375054281893165253, 3.332051601646770500 ) ) ;
#54685=PLANE ( 'NONE',  #47833 ) ;
#54686=AXIS2_PLACEMENT_3D ( 'NONE', #18016, #4955, #18865 ) ;
#54687=CARTESIAN_POINT ( 'NONE',  ( -17.83139810946674686, -0.1191753592594197858, 13.85674710641801788 ) ) ;
#54688=CARTESIAN_POINT ( 'NONE',  ( -20.18318107743349898, 0.000000000000000000, 4.663336943499984066 ) ) ;
#54689=AXIS2_PLACEMENT_3D ( 'NONE', #4632, #42977, #4377 ) ;
#54690=DIRECTION ( 'NONE',  ( 0.9999697198139515519, 0.000000000000000000, 0.007781995580013368816 ) ) ;
#54691=DIRECTION ( 'NONE',  ( 0.005002170337468016433, -0.7660444431189770143, -0.6427681459581293666 ) ) ;
#54692=EDGE_CURVE ( 'NONE', #49583, #55978, #8049, .T. ) ;
#54693=LINE ( 'NONE', #50460, #4260 ) ;
#54694=VECTOR ( 'NONE', #677, 999.9999999999998863 ) ;
#54695=CARTESIAN_POINT ( 'NONE',  ( -19.54411535461957783, -0.03228989815065526348, 4.471889025059788914 ) ) ;
#54696=VECTOR ( 'NONE', #23047, 1000.000000000000000 ) ;
#54697=VECTOR ( 'NONE', #39886, 1000.000000000000227 ) ;
#54698=ORIENTED_EDGE ( 'NONE', *, *, #45841, .T. ) ;
#54699=ADVANCED_FACE ( 'NONE', ( #25359 ), #12585, .F. ) ;
#54700=EDGE_CURVE ( 'NONE', #3988, #27645, #8307, .T. ) ;
#54701=VECTOR ( 'NONE', #41712, 1000.000000000000114 ) ;
#54702=EDGE_LOOP ( 'NONE', ( #32422, #44329, #9154, #54168 ) ) ;
#54703=EDGE_LOOP ( 'NONE', ( #24897, #18007, #34971, #30785 ) ) ;
#54704=AXIS2_PLACEMENT_3D ( 'NONE', #18105, #49042, #10144 ) ;
#54705=ORIENTED_EDGE ( 'NONE', *, *, #34840, .F. ) ;
#54706=EDGE_CURVE ( 'NONE', #53425, #37781, #44, .T. ) ;
#54707=EDGE_LOOP ( 'NONE', ( #11885, #21557, #27350, #39977 ) ) ;
#54708=CARTESIAN_POINT ( 'NONE',  ( -12.74767307358684576, 0.000000000000000000, 4.551875772493161776 ) ) ;
#54709=DIRECTION ( 'NONE',  ( 0.9999697198139515519, 0.000000000000000000, 0.007781995580013368816 ) ) ;
#54710=ADVANCED_FACE ( 'NONE', ( #46349 ), #7465, .F. ) ;
#54711=DIRECTION ( 'NONE',  ( 0.5364919789714477361, 0.6444004775717706579, 0.5449076811759711036 ) ) ;
#54712=ORIENTED_EDGE ( 'NONE', *, *, #45197, .F. ) ;
#54713=DIRECTION ( 'NONE',  ( -0.9999697198139514409, -0.000000000000000000, -0.007781995580013368816 ) ) ;
#54714=EDGE_CURVE ( 'NONE', #44660, #21187, #5451, .T. ) ;
#54715=ORIENTED_EDGE ( 'NONE', *, *, #18160, .F. ) ;
#54716=CARTESIAN_POINT ( 'NONE',  ( -26.13493519185646008, 0.000000000000000000, 7.033017491833586377 ) ) ;
#54717=ORIENTED_EDGE ( 'NONE', *, *, #27917, .T. ) ;
#54719=VECTOR ( 'NONE', #53476, 1000.000000000000227 ) ;
#54720=FACE_OUTER_BOUND ( 'NONE', #48542, .T. ) ;
#54721=DIRECTION ( 'NONE',  ( 0.5364919789714477361, 0.6444004775717706579, 0.5449076811759711036 ) ) ;
#54723=PLANE ( 'NONE',  #21034 ) ;
#54724=AXIS2_PLACEMENT_3D ( 'NONE', #32288, #48766, #14408 ) ;
#54726=CARTESIAN_POINT ( 'NONE',  ( -15.90130487007129823, -4.565544526780663581, 2.912263165649522367 ) ) ;
#54727=DIRECTION ( 'NONE',  ( 0.005002170337468016433, -0.7660444431189770143, -0.6427681459581293666 ) ) ;
#54728=VECTOR ( 'NONE', #40539, 1000.000000000000227 ) ;
#54729=CARTESIAN_POINT ( 'NONE',  ( -18.60939481748442859, 0.000000000000000000, 7.260909000724367957 ) ) ;
#54730=DIRECTION ( 'NONE',  ( 0.005002170337468016433, -0.7660444431189770143, -0.6427681459581293666 ) ) ;
#54731=CARTESIAN_POINT ( 'NONE',  ( -10.39574805432858895, 0.000000000000000000, 0.8768582987555647579 ) ) ;
#54732=PLANE ( 'NONE',  #1171 ) ;
#54733=CARTESIAN_POINT ( 'NONE',  ( -18.60077265696858007, 0.000000000000000000, 6.152979890951074893 ) ) ;
#54734=CARTESIAN_POINT ( 'NONE',  ( -14.85781100069234917, 0.000000000000000000, 2.858119855775270945 ) ) ;
#54735=VECTOR ( 'NONE', #26171, 999.9999999999998863 ) ;
#54736=DIRECTION ( 'NONE',  ( -0.6427681459581293666, -0.7660444431189770143, -0.005002170337467561935 ) ) ;
#54738=CARTESIAN_POINT ( 'NONE',  ( -25.20123094555300369, 0.000000000000000000, 6.470945668149052032 ) ) ;
#54739=ORIENTED_EDGE ( 'NONE', *, *, #12644, .F. ) ;
#54740=VECTOR ( 'NONE', #4535, 1000.000000000000000 ) ;
#54741=EDGE_CURVE ( 'NONE', #48042, #5616, #9428, .T. ) ;
#54743=DIRECTION ( 'NONE',  ( -0.6427681459581293666, -0.7660444431189770143, -0.005002170337467561935 ) ) ;
#54744=DIRECTION ( 'NONE',  ( 0.007781995580012663651, -3.146120232559066537E-19, -0.9999697198139514409 ) ) ;
#54745=CARTESIAN_POINT ( 'NONE',  ( -17.73140113748535285, 0.000000000000000000, 13.85752530597602039 ) ) ;
#54746=DIRECTION ( 'NONE',  ( -0.7660212471507179544, -0.6427876096865405842, -0.005961354470445141482 ) ) ;
#54747=CARTESIAN_POINT ( 'NONE',  ( -10.84028925556084388, -0.1191753592594197858, 11.14116300850493246 ) ) ;
#54748=EDGE_CURVE ( 'NONE', #10989, #44493, #43507, .T. ) ;
#54749=ADVANCED_FACE ( 'NONE', ( #52026 ), #26755, .F. ) ;
#54750=VECTOR ( 'NONE', #43519, 999.9999999999998863 ) ;
#54752=VECTOR ( 'NONE', #32763, 999.9999999999998863 ) ;
#54753=EDGE_LOOP ( 'NONE', ( #15148, #11627, #42645, #35384 ) ) ;
#54756=CARTESIAN_POINT ( 'NONE',  ( -15.19945166386478519, 1.257817950434004128, 4.849597862992245823 ) ) ;
#54757=CARTESIAN_POINT ( 'NONE',  ( -12.07527617786294449, 1.419719901456504285, 3.901770690733497915 ) ) ;
#54759=CARTESIAN_POINT ( 'NONE',  ( -13.83747589997588712, 2.391131607591507446, 6.180521011059407321 ) ) ;
#54760=DIRECTION ( 'NONE',  ( -0.6427681459581293666, -0.7660444431189770143, -0.005002170337467561935 ) ) ;
#54761=CARTESIAN_POINT ( 'NONE',  ( -19.60990026154428278, 0.000000000000000000, 4.498472333781370125 ) ) ;
#54762=DIRECTION ( 'NONE',  ( 0.005961354470445682716, -0.6427876096865404731, -0.7660212471507180654 ) ) ;
#54763=EDGE_CURVE ( 'NONE', #13999, #30111, #35548, .T. ) ;
#54764=VERTEX_POINT ( 'NONE', #39818 ) ;
#54765=DIRECTION ( 'NONE',  ( -0.9999697198139514409, -0.000000000000000000, -0.007781995580013368816 ) ) ;
#54766=CARTESIAN_POINT ( 'NONE',  ( -15.62884970628905457, -4.241740624735664156, 2.816763367194973000 ) ) ;
#54767=VERTEX_POINT ( 'NONE', #43778 ) ;
#54768=AXIS2_PLACEMENT_3D ( 'NONE', #48360, #10028, #27337 ) ;
#54769=CARTESIAN_POINT ( 'NONE',  ( -20.87535245856507515, -2.137015261443157232, 8.297833671620280072 ) ) ;
#54770=CARTESIAN_POINT ( 'NONE',  ( -10.27421835998572064, 0.000000000000000000, 10.96090226820206048 ) ) ;
#54771=AXIS2_PLACEMENT_3D ( 'NONE', #15769, #32808, #33393 ) ;
#54772=VERTEX_POINT ( 'NONE', #44614 ) ;
#54773=VECTOR ( 'NONE', #18981, 1000.000000000000114 ) ;
#54774=VERTEX_POINT ( 'NONE', #1175 ) ;
#54775=DIRECTION ( 'NONE',  ( 0.005002170337468016433, -0.7660444431189770143, -0.6427681459581293666 ) ) ;
#54776=EDGE_CURVE ( 'NONE', #31643, #16374, #47795, .T. ) ;
#54777=ORIENTED_EDGE ( 'NONE', *, *, #44200, .T. ) ;
#54778=EDGE_LOOP ( 'NONE', ( #3795, #17792, #37531, #38959, #39782 ) ) ;
#54779=EDGE_LOOP ( 'NONE', ( #23273, #5175, #14111, #9053 ) ) ;
#54780=EDGE_CURVE ( 'NONE', #18328, #14930, #35019, .T. ) ;
#54781=FACE_OUTER_BOUND ( 'NONE', #49671, .T. ) ;
#54782=AXIS2_PLACEMENT_3D ( 'NONE', #14998, #6470, #14176 ) ;
#54784=LINE ( 'NONE', #41999, #52075 ) ;
#54785=VECTOR ( 'NONE', #27819, 1000.000000000000227 ) ;
#54786=ORIENTED_EDGE ( 'NONE', *, *, #38217, .T. ) ;
#54787=EDGE_CURVE ( 'NONE', #8286, #54291, #26204, .T. ) ;
#54788=ORIENTED_EDGE ( 'NONE', *, *, #37925, .F. ) ;
#54789=VECTOR ( 'NONE', #55834, 1000.000000000000227 ) ;
#54791=DIRECTION ( 'NONE',  ( -0.5364919789714478471, 0.6444004775717705469, -0.5449076811759709926 ) ) ;
#54792=EDGE_LOOP ( 'NONE', ( #46411, #31944, #27168, #23241 ) ) ;
#54793=CARTESIAN_POINT ( 'NONE',  ( -17.88167136688104719, 0.000000000000000000, 7.466578369107171653 ) ) ;
#54794=ORIENTED_EDGE ( 'NONE', *, *, #49105, .T. ) ;
#54795=PLANE ( 'NONE',  #27627 ) ;
#54796=CARTESIAN_POINT ( 'NONE',  ( -15.04630770547183971, 2.714935509636507316, 7.181489704315874079 ) ) ;
#54798=VERTEX_POINT ( 'NONE', #52859 ) ;
#54799=PLANE ( 'NONE',  #20980 ) ;
#54800=EDGE_CURVE ( 'NONE', #29572, #14416, #18505, .T. ) ;
#54801=EDGE_CURVE ( 'NONE', #10129, #52847, #21576, .T. ) ;
#54802=VECTOR ( 'NONE', #11654, 1000.000000000000227 ) ;
#54803=CARTESIAN_POINT ( 'NONE',  ( -21.47263955680318404, 0.000000000000000000, 5.022634149262071190 ) ) ;
#54804=ORIENTED_EDGE ( 'NONE', *, *, #29100, .T. ) ;
#54805=CARTESIAN_POINT ( 'NONE',  ( -12.26423545659806003, 0.000000000000000000, 2.139639520751795310 ) ) ;
#54806=VECTOR ( 'NONE', #48881, 1000.000000000000227 ) ;
#54807=PLANE ( 'NONE',  #49153 ) ;
#54808=ADVANCED_FACE ( 'NONE', ( #14280 ), #48315, .F. ) ;
#54809=VERTEX_POINT ( 'NONE', #9992 ) ;
#54810=AXIS2_PLACEMENT_3D ( 'NONE', #47791, #21663, #8897 ) ;
#54811=EDGE_CURVE ( 'NONE', #35804, #1119, #26457, .T. ) ;
#54812=LINE ( 'NONE', #11383, #48264 ) ;
#54813=DIRECTION ( 'NONE',  ( -0.6427681459581293666, -0.7660444431189770143, -0.005002170337467561935 ) ) ;
#54814=LINE ( 'NONE', #23600, #55758 ) ;
#54815=CARTESIAN_POINT ( 'NONE',  ( 2.072287782118878319, 0.000000000000000000, -2.950529333540147015 ) ) ;
#54816=DIRECTION ( 'NONE',  ( -0.3313982828793700097, 0.4028455766673915694, -0.8531650599175529814 ) ) ;
#54817=ADVANCED_FACE ( 'NONE', ( #27300 ), #9735, .F. ) ;
#54818=LINE ( 'NONE', #33267, #32516 ) ;
#54819=CARTESIAN_POINT ( 'NONE',  ( -10.41874342548586085, 8.040039804732380446, 0.8286201928109698800 ) ) ;
#54820=VECTOR ( 'NONE', #49309, 1000.000000000000227 ) ;
#54821=ORIENTED_EDGE ( 'NONE', *, *, #32325, .F. ) ;
#54822=CARTESIAN_POINT ( 'NONE',  ( -18.24553309218274322, -0.1191753592594166911, 7.363743684915764476 ) ) ;
#54823=LINE ( 'NONE', #7395, #30419 ) ;
#54825=ORIENTED_EDGE ( 'NONE', *, *, #16299, .F. ) ;
#54826=VECTOR ( 'NONE', #14106, 1000.000000000000000 ) ;
#54827=DIRECTION ( 'NONE',  ( -0.5364919789714478471, 0.6444004775717705469, -0.5449076811759709926 ) ) ;
#54828=PLANE ( 'NONE',  #45405 ) ;
#54829=AXIS2_PLACEMENT_3D ( 'NONE', #9085, #47725, #25859 ) ;
#54830=EDGE_CURVE ( 'NONE', #44660, #51166, #48898, .T. ) ;
#54831=EDGE_CURVE ( 'NONE', #16476, #18331, #27043, .T. ) ;
#54832=FACE_OUTER_BOUND ( 'NONE', #36340, .T. ) ;
#54833=DIRECTION ( 'NONE',  ( 0.7660212471507180654, -0.6427876096865404731, 0.005961354470445141482 ) ) ;
#54834=CARTESIAN_POINT ( 'NONE',  ( -15.55561282917033594, 0.000000000000000000, 7.115348224689455492 ) ) ;
#54835=EDGE_CURVE ( 'NONE', #33685, #55481, #45200, .T. ) ;
#54836=ORIENTED_EDGE ( 'NONE', *, *, #25324, .T. ) ;
#54837=VECTOR ( 'NONE', #33902, 999.9999999999998863 ) ;
#54839=EDGE_LOOP ( 'NONE', ( #2737, #25522, #7898, #2093 ) ) ;
#54840=CARTESIAN_POINT ( 'NONE',  ( 2.072287782118878319, 0.000000000000000000, -2.950529333540147015 ) ) ;
#54841=CARTESIAN_POINT ( 'NONE',  ( -11.21901323774118708, 0.000000000000000000, 1.039777472322872098 ) ) ;
#54842=VERTEX_POINT ( 'NONE', #31848 ) ;
#54843=FACE_OUTER_BOUND ( 'NONE', #17638, .T. ) ;
#54844=ORIENTED_EDGE ( 'NONE', *, *, #28090, .T. ) ;
#54845=DIRECTION ( 'NONE',  ( 0.7660212471507180654, -0.6427876096865404731, 0.005961354470445141482 ) ) ;
#54846=AXIS2_PLACEMENT_3D ( 'NONE', #51053, #46817, #15860 ) ;
#54848=EDGE_LOOP ( 'NONE', ( #15236, #4333, #40199, #55091 ) ) ;
#54849=ORIENTED_EDGE ( 'NONE', *, *, #11319, .T. ) ;
#54850=VECTOR ( 'NONE', #23466, 999.9999999999998863 ) ;
#54851=CARTESIAN_POINT ( 'NONE',  ( -15.50102849149811135, -0.1191753592594197858, 12.95155240711365430 ) ) ;
#54852=FACE_OUTER_BOUND ( 'NONE', #11531, .T. ) ;
#54854=DIRECTION ( 'NONE',  ( 0.007781995580012663651, 0.000000000000000000, -0.9999697198139515519 ) ) ;
#54855=EDGE_LOOP ( 'NONE', ( #20057, #44309, #18511, #46149, #42454 ) ) ;
#54856=DIRECTION ( 'NONE',  ( -0.7660212471507179544, -0.6427876096865405842, -0.005961354470445141482 ) ) ;
#54857=ADVANCED_FACE ( 'NONE', ( #7139 ), #54269, .F. ) ;
#54858=AXIS2_PLACEMENT_3D ( 'NONE', #34092, #12771, #42022 ) ;
#54859=ORIENTED_EDGE ( 'NONE', *, *, #17724, .T. ) ;
#54861=ORIENTED_EDGE ( 'NONE', *, *, #15121, .T. ) ;
#54862=VECTOR ( 'NONE', #53483, 1000.000000000000227 ) ;
#54863=CARTESIAN_POINT ( 'NONE',  ( -19.08133622045208355, 0.000000000000000000, 8.195906439434676116 ) ) ;
#54864=AXIS2_PLACEMENT_3D ( 'NONE', #46, #340, #5197 ) ;
#54865=CARTESIAN_POINT ( 'NONE',  ( -17.93139508144814442, 0.000000000000000000, 13.85596890686001537 ) ) ;
#54866=ORIENTED_EDGE ( 'NONE', *, *, #54945, .F. ) ;
#54867=VECTOR ( 'NONE', #14545, 999.9999999999998863 ) ;
#54868=CARTESIAN_POINT ( 'NONE',  ( -10.69044919664899318, 0.000000000000000000, 4.737211577976179200 ) ) ;
#54869=ORIENTED_EDGE ( 'NONE', *, *, #42916, .T. ) ;
#54870=FACE_OUTER_BOUND ( 'NONE', #5985, .T. ) ;
#54872=VECTOR ( 'NONE', #28347, 1000.000000000000227 ) ;
#54873=EDGE_CURVE ( 'NONE', #13455, #156, #28141, .T. ) ;
#54874=ORIENTED_EDGE ( 'NONE', *, *, #5368, .T. ) ;
#54875=DIRECTION ( 'NONE',  ( 0.9999697198139515519, 0.000000000000000000, 0.007781995580013368816 ) ) ;
#54876=VERTEX_POINT ( 'NONE', #53435 ) ;
#54877=ADVANCED_FACE ( 'NONE', ( #19899 ), #19060, .F. ) ;
#54878=EDGE_CURVE ( 'NONE', #40214, #50606, #41207, .T. ) ;
#54879=AXIS2_PLACEMENT_3D ( 'NONE', #13921, #8556, #51700 ) ;
#54880=PLANE ( 'NONE',  #28303 ) ;
#54881=VECTOR ( 'NONE', #32682, 1000.000000000000227 ) ;
#54882=LINE ( 'NONE', #49787, #13000 ) ;
#54883=CARTESIAN_POINT ( 'NONE',  ( -11.35376238306358410, 0.000000000000000000, 4.562723507797191047 ) ) ;
#54884=DIRECTION ( 'NONE',  ( 0.5449076811759707706, 0.6444004775717708799, -0.5364919789714476250 ) ) ;
#54885=DIRECTION ( 'NONE',  ( -0.6427681459581293666, -0.7660444431189770143, -0.005002170337467561935 ) ) ;
#54887=ORIENTED_EDGE ( 'NONE', *, *, #12269, .T. ) ;
#54888=ORIENTED_EDGE ( 'NONE', *, *, #44966, .F. ) ;
#54889=EDGE_CURVE ( 'NONE', #19083, #9775, #19638, .T. ) ;
#54890=DIRECTION ( 'NONE',  ( 0.000000000000000000, -1.000000000000000000, 0.000000000000000000 ) ) ;
#54891=FACE_OUTER_BOUND ( 'NONE', #29437, .T. ) ;
#54893=LINE ( 'NONE', #29048, #33027 ) ;
#54894=EDGE_CURVE ( 'NONE', #56189, #54483, #36675, .T. ) ;
#54895=DIRECTION ( 'NONE',  ( 0.005002170337468016433, -0.7660444431189770143, -0.6427681459581293666 ) ) ;
#54896=AXIS2_PLACEMENT_3D ( 'NONE', #50449, #8131, #16345 ) ;
#54897=FACE_OUTER_BOUND ( 'NONE', #42160, .T. ) ;
#54898=ORIENTED_EDGE ( 'NONE', *, *, #3288, .F. ) ;
#54899=VECTOR ( 'NONE', #18565, 1000.000000000000227 ) ;
#54900=CARTESIAN_POINT ( 'NONE',  ( -18.76354595665420177, -0.1191753592594177458, 14.21882498613976331 ) ) ;
#54901=LINE ( 'NONE', #50642, #33191 ) ;
#54902=ORIENTED_EDGE ( 'NONE', *, *, #6294, .F. ) ;
#54903=PLANE ( 'NONE',  #23860 ) ;
#54904=CARTESIAN_POINT ( 'NONE',  ( -18.84739110800622797, 4.981562823951511731, 12.37788115850241333 ) ) ;
#54905=VECTOR ( 'NONE', #26915, 1000.000000000000227 ) ;
#54906=ORIENTED_EDGE ( 'NONE', *, *, #37093, .T. ) ;
#54907=ADVANCED_FACE ( 'NONE', ( #6564 ), #24435, .F. ) ;
#54908=PLANE ( 'NONE',  #34338 ) ;
#54909=LINE ( 'NONE', #55451, #34224 ) ;
#54910=AXIS2_PLACEMENT_3D ( 'NONE', #30316, #48170, #14129 ) ;
#54911=PLANE ( 'NONE',  #32322 ) ;
#54912=DIRECTION ( 'NONE',  ( -0.5449076811759708816, 0.6444004775717707689, 0.5364919789714475140 ) ) ;
#54914=FACE_OUTER_BOUND ( 'NONE', #42465, .T. ) ;
#54915=EDGE_CURVE ( 'NONE', #17921, #41488, #6035, .T. ) ;
#54916=ORIENTED_EDGE ( 'NONE', *, *, #18004, .F. ) ;
#54917=VECTOR ( 'NONE', #31355, 1000.000000000000227 ) ;
#54918=VECTOR ( 'NONE', #37065, 999.9999999999998863 ) ;
#54919=VERTEX_POINT ( 'NONE', #36968 ) ;
#54921=DIRECTION ( 'NONE',  ( 0.5364919789714477361, 0.6444004775717706579, 0.5449076811759711036 ) ) ;
#54922=DIRECTION ( 'NONE',  ( -0.9321478471874540261, 0.000000000000000000, 0.3620778797217457656 ) ) ;
#54923=VECTOR ( 'NONE', #11480, 1000.000000000000114 ) ;
#54925=VECTOR ( 'NONE', #34835, 999.9999999999998863 ) ;
#54926=PLANE ( 'NONE',  #37353 ) ;
#54927=LINE ( 'NONE', #16033, #29473 ) ;
#54928=VECTOR ( 'NONE', #13019, 1000.000000000000227 ) ;
#54929=ORIENTED_EDGE ( 'NONE', *, *, #18025, .F. ) ;
#54930=DIRECTION ( 'NONE',  ( 0.5449076811759707706, 0.6444004775717708799, -0.5364919789714476250 ) ) ;
#54931=VECTOR ( 'NONE', #26569, 999.9999999999998863 ) ;
#54932=DIRECTION ( 'NONE',  ( -0.5449076811759708816, 0.6444004775717707689, 0.5364919789714475140 ) ) ;
#54933=VECTOR ( 'NONE', #29124, 1000.000000000000227 ) ;
#54934=DIRECTION ( 'NONE',  ( 0.5364919789714477361, 0.6444004775717706579, 0.5449076811759711036 ) ) ;
#54935=ORIENTED_EDGE ( 'NONE', *, *, #49772, .F. ) ;
#54936=FACE_OUTER_BOUND ( 'NONE', #51498, .T. ) ;
#54937=DIRECTION ( 'NONE',  ( -0.7660212471507179544, -0.6427876096865405842, -0.005961354470445141482 ) ) ;
#54938=DIRECTION ( 'NONE',  ( 0.6427681459581294776, -0.7660444431189769032, 0.005002170337467562802 ) ) ;
#54939=ORIENTED_EDGE ( 'NONE', *, *, #4620, .F. ) ;
#54940=CARTESIAN_POINT ( 'NONE',  ( -13.46258265577981383, 0.000000000000000000, 2.699651831784322997 ) ) ;
#54941=ADVANCED_FACE ( 'NONE', ( #53992 ), #15108, .F. ) ;
#54943=VECTOR ( 'NONE', #20181, 1000.000000000000000 ) ;
#54944=ORIENTED_EDGE ( 'NONE', *, *, #49755, .T. ) ;
#54945=EDGE_CURVE ( 'NONE', #21963, #12571, #15623, .T. ) ;
#54946=ORIENTED_EDGE ( 'NONE', *, *, #13055, .T. ) ;
#54947=ADVANCED_FACE ( 'NONE', ( #49461 ), #28723, .F. ) ;
#54948=EDGE_LOOP ( 'NONE', ( #33633, #47953, #46665, #21823 ) ) ;
#54949=FACE_OUTER_BOUND ( 'NONE', #50259, .T. ) ;
#54950=VECTOR ( 'NONE', #33652, 1000.000000000000114 ) ;
#54951=ORIENTED_EDGE ( 'NONE', *, *, #8270, .F. ) ;
#54952=EDGE_CURVE ( 'NONE', #18056, #36712, #23604, .T. ) ;
#54953=EDGE_CURVE ( 'NONE', #29572, #22170, #14532, .T. ) ;
#54954=ADVANCED_FACE ( 'NONE', ( #27596 ), #23348, .F. ) ;
#54955=ORIENTED_EDGE ( 'NONE', *, *, #23987, .T. ) ;
#54956=DIRECTION ( 'NONE',  ( 0.000000000000000000, -1.000000000000000000, 0.000000000000000000 ) ) ;
#54957=ORIENTED_EDGE ( 'NONE', *, *, #34476, .F. ) ;
#54959=ORIENTED_EDGE ( 'NONE', *, *, #9842, .F. ) ;
#54961=VECTOR ( 'NONE', #48953, 999.9999999999998863 ) ;
#54962=CARTESIAN_POINT ( 'NONE',  ( -17.80573849810343390, 2.714935509636509536, 3.511664592573657373 ) ) ;
#54963=LINE ( 'NONE', #7521, #46615 ) ;
#54965=CARTESIAN_POINT ( 'NONE',  ( 2.072287782118878319, 0.000000000000000000, -2.950529333540147015 ) ) ;
#54966=DIRECTION ( 'NONE',  ( 0.007781995580012663651, 0.000000000000000000, -0.9999697198139515519 ) ) ;
#54968=AXIS2_PLACEMENT_3D ( 'NONE', #2087, #53509, #10907 ) ;
#54969=VERTEX_POINT ( 'NONE', #1739 ) ;
#54970=VECTOR ( 'NONE', #13871, 1000.000000000000114 ) ;
#54971=EDGE_CURVE ( 'NONE', #23998, #16476, #11670, .T. ) ;
#54972=DIRECTION ( 'NONE',  ( 0.007781995580012663651, -3.146120232559066537E-19, -0.9999697198139514409 ) ) ;
#54973=DIRECTION ( 'NONE',  ( -0.005002170337468016433, -0.7660444431189770143, 0.6427681459581293666 ) ) ;
#54974=AXIS2_PLACEMENT_3D ( 'NONE', #51078, #42843, #16730 ) ;
#54975=EDGE_CURVE ( 'NONE', #12964, #6316, #47419, .T. ) ;
#54977=VECTOR ( 'NONE', #45338, 999.9999999999998863 ) ;
#54978=CARTESIAN_POINT ( 'NONE',  ( -11.74346145839723654, -0.1191753592594190225, 7.779932815735107532 ) ) ;
#54979=ADVANCED_FACE ( 'NONE', ( #34104 ), #29842, .F. ) ;
#54980=CARTESIAN_POINT ( 'NONE',  ( -19.05678739329382054, 0.000000000000000000, 5.041434869409770592 ) ) ;
#54981=CARTESIAN_POINT ( 'NONE',  ( -28.93137873341882127, 0.000000000000000000, 8.119251130998824451 ) ) ;
#54982=ORIENTED_EDGE ( 'NONE', *, *, #20794, .F. ) ;
#54983=CARTESIAN_POINT ( 'NONE',  ( -19.12962290826653700, 0.000000000000000000, 14.40064212555863854 ) ) ;
#54984=EDGE_LOOP ( 'NONE', ( #14440, #51451, #4304, #20935 ) ) ;
#54985=EDGE_CURVE ( 'NONE', #2867, #11647, #17059, .T. ) ;
#54986=CARTESIAN_POINT ( 'NONE',  ( -18.14918837326463219, 0.000000000000000000, 7.833828559712929795 ) ) ;
#54987=DIRECTION ( 'NONE',  ( 0.000000000000000000, -1.000000000000000000, 0.000000000000000000 ) ) ;
#54988=DIRECTION ( 'NONE',  ( 0.9999697198139515519, 0.000000000000000000, 0.007781995580013368816 ) ) ;
#54989=FACE_OUTER_BOUND ( 'NONE', #24461, .T. ) ;
#54991=DIRECTION ( 'NONE',  ( 0.005961354470445682716, -0.6427876096865404731, -0.7660212471507180654 ) ) ;
#54992=VECTOR ( 'NONE', #4445, 999.9999999999998863 ) ;
#54993=EDGE_LOOP ( 'NONE', ( #28744, #14653, #52953, #39507 ) ) ;
#54994=ORIENTED_EDGE ( 'NONE', *, *, #6062, .T. ) ;
#54995=LINE ( 'NONE', #27767, #13024 ) ;
#54996=FACE_OUTER_BOUND ( 'NONE', #17013, .T. ) ;
#54997=LINE ( 'NONE', #29130, #43301 ) ;
#54998=VECTOR ( 'NONE', #35025, 1000.000000000000227 ) ;
#54999=CARTESIAN_POINT ( 'NONE',  ( -9.999901398370125705, 0.000000000000000000, 1.249270938769537542 ) ) ;
#55000=VECTOR ( 'NONE', #38585, 1000.000000000000000 ) ;
#55001=FACE_OUTER_BOUND ( 'NONE', #41896, .T. ) ;
#55003=DIRECTION ( 'NONE',  ( 0.007781995580012662783, 0.000000000000000000, -0.9999697198139514409 ) ) ;
#55004=AXIS2_PLACEMENT_3D ( 'NONE', #4756, #43391, #13301 ) ;
#55005=LINE ( 'NONE', #3011, #33279 ) ;
#55006=CARTESIAN_POINT ( 'NONE',  ( -7.034459185439723150, -6.761815089084117325, -0.4859507367995170024 ) ) ;
#55007=ORIENTED_EDGE ( 'NONE', *, *, #21287, .T. ) ;
#55008=VERTEX_POINT ( 'NONE', #47138 ) ;
#55009=AXIS2_PLACEMENT_3D ( 'NONE', #47258, #29956, #46410 ) ;
#55010=EDGE_CURVE ( 'NONE', #3706, #49287, #20162, .T. ) ;
#55011=VECTOR ( 'NONE', #47614, 1000.000000000000227 ) ;
#55012=ORIENTED_EDGE ( 'NONE', *, *, #28944, .T. ) ;
#55013=VECTOR ( 'NONE', #39338, 999.9999999999998863 ) ;
#55014=EDGE_LOOP ( 'NONE', ( #29007, #42930, #33557, #14447 ) ) ;
#55015=EDGE_CURVE ( 'NONE', #36809, #27553, #50831, .T. ) ;
#55016=ORIENTED_EDGE ( 'NONE', *, *, #45773, .F. ) ;
#55017=ORIENTED_EDGE ( 'NONE', *, *, #28197, .F. ) ;
#55018=DIRECTION ( 'NONE',  ( 0.000000000000000000, -0.000000000000000000, -1.000000000000000000 ) ) ;
#55019=FACE_OUTER_BOUND ( 'NONE', #27115, .T. ) ;
#55020=DIRECTION ( 'NONE',  ( 0.007781995580012662783, 0.000000000000000000, -0.9999697198139514409 ) ) ;
#55021=EDGE_CURVE ( 'NONE', #9595, #26049, #25556, .T. ) ;
#55022=ADVANCED_FACE ( 'NONE', ( #8529 ), #11927, .F. ) ;
#55023=EDGE_CURVE ( 'NONE', #16052, #18488, #21009, .T. ) ;
#55024=EDGE_LOOP ( 'NONE', ( #55291, #3407, #36638, #41460 ) ) ;
#55025=DIRECTION ( 'NONE',  ( 0.007781995580012663651, -3.146120232559066537E-19, -0.9999697198139514409 ) ) ;
#55026=ORIENTED_EDGE ( 'NONE', *, *, #35223, .F. ) ;
#55028=EDGE_CURVE ( 'NONE', #24728, #52574, #38640, .T. ) ;
#55029=ORIENTED_EDGE ( 'NONE', *, *, #47979, .F. ) ;
#55030=AXIS2_PLACEMENT_3D ( 'NONE', #16822, #47469, #25071 ) ;
#55032=CARTESIAN_POINT ( 'NONE',  ( -15.37089526832641617, -1.165603555308157846, 2.814709981181112486 ) ) ;
#55033=CARTESIAN_POINT ( 'NONE',  ( -12.80458192191714595, 0.000000000000000000, 11.86454056839041726 ) ) ;
#55034=ORIENTED_EDGE ( 'NONE', *, *, #45511, .F. ) ;
#55035=LINE ( 'NONE', #3041, #21935 ) ;
#55036=ORIENTED_EDGE ( 'NONE', *, *, #18968, .T. ) ;
#55037=DIRECTION ( 'NONE',  ( -0.7660212471507179544, -0.6427876096865405842, -0.005961354470445141482 ) ) ;
#55039=DIRECTION ( 'NONE',  ( -0.5364919789714478471, 0.6444004775717705469, -0.5449076811759709926 ) ) ;
#55040=EDGE_CURVE ( 'NONE', #54376, #48873, #46571, .T. ) ;
#55041=LINE ( 'NONE', #54195, #17890 ) ;
#55042=VECTOR ( 'NONE', #54988, 999.9999999999998863 ) ;
#55043=DIRECTION ( 'NONE',  ( -0.7660212471507179544, -0.6427876096865405842, -0.005961354470445141482 ) ) ;
#55046=EDGE_CURVE ( 'NONE', #46078, #43561, #16206, .T. ) ;
#55047=CARTESIAN_POINT ( 'NONE',  ( -19.60912206198628027, -0.1191753592594197858, 4.398475361799976113 ) ) ;
#55048=DIRECTION ( 'NONE',  ( 0.005002170337468016433, -0.7660444431189770143, -0.6427681459581293666 ) ) ;
#55049=ORIENTED_EDGE ( 'NONE', *, *, #27520, .F. ) ;
#55051=ORIENTED_EDGE ( 'NONE', *, *, #4342, .F. ) ;
#55052=ADVANCED_FACE ( 'NONE', ( #46880 ), #51423, .F. ) ;
#55053=DIRECTION ( 'NONE',  ( -0.005961354470445682716, -0.6427876096865404731, 0.7660212471507180654 ) ) ;
#55054=PLANE ( 'NONE',  #47756 ) ;
#55055=FACE_OUTER_BOUND ( 'NONE', #42650, .T. ) ;
#55056=DIRECTION ( 'NONE',  ( 0.5449076811759707706, 0.6444004775717708799, -0.5364919789714476250 ) ) ;
#55057=PLANE ( 'NONE',  #14123 ) ;
#55058=EDGE_CURVE ( 'NONE', #34537, #41838, #55964, .T. ) ;
#55059=AXIS2_PLACEMENT_3D ( 'NONE', #2593, #7149, #50587 ) ;
#55060=DIRECTION ( 'NONE',  ( 0.000000000000000000, -0.000000000000000000, -1.000000000000000000 ) ) ;
#55062=ORIENTED_EDGE ( 'NONE', *, *, #52393, .F. ) ;
#55063=LINE ( 'NONE', #50214, #15607 ) ;
#55064=DIRECTION ( 'NONE',  ( 0.9999697198139515519, 0.000000000000000000, 0.007781995580013368816 ) ) ;
#55065=DIRECTION ( 'NONE',  ( -0.5449076811759708816, 0.6444004775717707689, 0.5364919789714475140 ) ) ;
#55069=FACE_OUTER_BOUND ( 'NONE', #4987, .T. ) ;
#55070=FACE_OUTER_BOUND ( 'NONE', #14165, .T. ) ;
#55071=DIRECTION ( 'NONE',  ( 0.5364919789714477361, 0.6444004775717706579, 0.5449076811759711036 ) ) ;
#55072=EDGE_LOOP ( 'NONE', ( #34024, #5306, #1362, #18523 ) ) ;
#55073=CARTESIAN_POINT ( 'NONE',  ( -14.00280974873554030, 0.000000000000000000, 12.40921378708904044 ) ) ;
#55076=ORIENTED_EDGE ( 'NONE', *, *, #15279, .T. ) ;
#55078=ORIENTED_EDGE ( 'NONE', *, *, #34153, .T. ) ;
#55079=EDGE_LOOP ( 'NONE', ( #21495, #21862, #55012, #11916 ) ) ;
#55080=CARTESIAN_POINT ( 'NONE',  ( -12.80458192191714595, 0.000000000000000000, 11.86454056839041726 ) ) ;
#55081=VECTOR ( 'NONE', #38802, 999.9999999999998863 ) ;
#55082=EDGE_LOOP ( 'NONE', ( #16321, #49962, #31570, #24007 ) ) ;
#55083=ORIENTED_EDGE ( 'NONE', *, *, #44725, .T. ) ;
#55084=ORIENTED_EDGE ( 'NONE', *, *, #31330, .F. ) ;
#55085=CARTESIAN_POINT ( 'NONE',  ( -12.28435383113503931, 0.000000000000000000, 4.724807443556146680 ) ) ;
#55087=DIRECTION ( 'NONE',  ( 0.9999697198139515519, 0.000000000000000000, 0.007781995580013368816 ) ) ;
#55088=EDGE_CURVE ( 'NONE', #14403, #7048, #21308, .T. ) ;
#55089=AXIS2_PLACEMENT_3D ( 'NONE', #26909, #31145, #31987 ) ;
#55090=ORIENTED_EDGE ( 'NONE', *, *, #10065, .T. ) ;
#55091=ORIENTED_EDGE ( 'NONE', *, *, #2456, .F. ) ;
#55092=EDGE_CURVE ( 'NONE', #42292, #1604, #46282, .T. ) ;
#55093=EDGE_CURVE ( 'NONE', #16077, #13531, #54818, .T. ) ;
#55094=DIRECTION ( 'NONE',  ( -0.5364919789714478471, 0.6444004775717705469, -0.5449076811759709926 ) ) ;
#55095=FACE_OUTER_BOUND ( 'NONE', #8018, .T. ) ;
#55096=ORIENTED_EDGE ( 'NONE', *, *, #31652, .T. ) ;
#55097=PLANE ( 'NONE',  #13751 ) ;
#55098=ORIENTED_EDGE ( 'NONE', *, *, #24626, .T. ) ;
#55099=CARTESIAN_POINT ( 'NONE',  ( -18.66354898467281132, 0.000000000000000000, 14.21960318569776582 ) ) ;
#55100=FACE_OUTER_BOUND ( 'NONE', #8762, .T. ) ;
#55101=VERTEX_POINT ( 'NONE', #50575 ) ;
#55102=DIRECTION ( 'NONE',  ( 0.9999697198139515519, 0.000000000000000000, 0.007781995580013368816 ) ) ;
#55103=CARTESIAN_POINT ( 'NONE',  ( -21.47419595591918906, 0.000000000000000000, 5.222628093224860102 ) ) ;
#55105=DIRECTION ( 'NONE',  ( -0.7660212471507179544, -0.6427876096865405842, -0.005961354470445141482 ) ) ;
#55106=DIRECTION ( 'NONE',  ( 0.5364919789714477361, 0.6444004775717706579, 0.5449076811759711036 ) ) ;
#55107=CARTESIAN_POINT ( 'NONE',  ( -14.62190858286687956, 0.000000000000000000, 6.553276401004920260 ) ) ;
#55108=ORIENTED_EDGE ( 'NONE', *, *, #13124, .F. ) ;
#55109=CARTESIAN_POINT ( 'NONE',  ( -9.966917453940169480, 0.000000000000000000, 5.481506408911723582 ) ) ;
#55110=LINE ( 'NONE', #11922, #36878 ) ;
#55111=DIRECTION ( 'NONE',  ( 0.5449076811759707706, 0.6444004775717708799, -0.5364919789714476250 ) ) ;
#55112=CARTESIAN_POINT ( 'NONE',  ( -8.574951275837294773, -8.254029952494388311, 0.1124287064424994709 ) ) ;
#55113=EDGE_CURVE ( 'NONE', #51703, #7720, #7391, .T. ) ;
#55114=PLANE ( 'NONE',  #4992 ) ;
#55115=DIRECTION ( 'NONE',  ( 0.000000000000000000, -1.000000000000000000, 0.000000000000000000 ) ) ;
#55116=LINE ( 'NONE', #7690, #38536 ) ;
#55118=DIRECTION ( 'NONE',  ( 0.5449076811759707706, 0.6444004775717708799, -0.5364919789714476250 ) ) ;
#55119=EDGE_CURVE ( 'NONE', #12509, #35868, #42340, .T. ) ;
#55120=DIRECTION ( 'NONE',  ( 0.000000000000000000, -0.000000000000000000, -1.000000000000000000 ) ) ;
#55121=DIRECTION ( 'NONE',  ( -0.7660212471507179544, -0.6427876096865405842, -0.005961354470445141482 ) ) ;
#55122=ORIENTED_EDGE ( 'NONE', *, *, #47171, .T. ) ;
#55123=LINE ( 'NONE', #15633, #13900 ) ;
#55125=VECTOR ( 'NONE', #14813, 1000.000000000000114 ) ;
#55127=LINE ( 'NONE', #2845, #39484 ) ;
#55128=FACE_OUTER_BOUND ( 'NONE', #12812, .T. ) ;
#55129=FACE_OUTER_BOUND ( 'NONE', #54778, .T. ) ;
#55130=EDGE_LOOP ( 'NONE', ( #35970, #33564, #18178, #4254, #30425 ) ) ;
#55131=ORIENTED_EDGE ( 'NONE', *, *, #54780, .F. ) ;
#55132=CARTESIAN_POINT ( 'NONE',  ( -15.34544032557569437, 0.000000000000000000, 5.808981570069377653 ) ) ;
#55133=CARTESIAN_POINT ( 'NONE',  ( -25.20123094555300369, 0.000000000000000000, 6.470945668149052032 ) ) ;
#55134=ORIENTED_EDGE ( 'NONE', *, *, #54470, .F. ) ;
#55135=DIRECTION ( 'NONE',  ( -0.5449076811759708816, 0.6444004775717707689, 0.5364919789714475140 ) ) ;
#55136=VERTEX_POINT ( 'NONE', #18440 ) ;
#55137=CARTESIAN_POINT ( 'NONE',  ( -23.33693525117809386, 0.000000000000000000, 5.746789908705562944 ) ) ;
#55138=ORIENTED_EDGE ( 'NONE', *, *, #16732, .T. ) ;
#55139=ORIENTED_EDGE ( 'NONE', *, *, #53990, .T. ) ;
#55140=ORIENTED_EDGE ( 'NONE', *, *, #12544, .F. ) ;
#55141=CARTESIAN_POINT ( 'NONE',  ( -16.33317936670417225, 0.000000000000000000, 13.31440848639340224 ) ) ;
#55142=ADVANCED_FACE ( 'NONE', ( #30688 ), #48840, .F. ) ;
#55143=DIRECTION ( 'NONE',  ( -0.005961354470445682716, -0.6427876096865404731, 0.7660212471507180654 ) ) ;
#55144=CARTESIAN_POINT ( 'NONE',  ( -26.13493519185646008, 0.000000000000000000, 7.033017491833586377 ) ) ;
#55145=FACE_OUTER_BOUND ( 'NONE', #45905, .T. ) ;
#55146=ORIENTED_EDGE ( 'NONE', *, *, #68, .F. ) ;
#55147=EDGE_CURVE ( 'NONE', #46316, #32796, #48245, .T. ) ;
#55148=ADVANCED_FACE ( 'NONE', ( #44297 ), #4546, .F. ) ;
#55149=ORIENTED_EDGE ( 'NONE', *, *, #43847, .F. ) ;
#55150=ORIENTED_EDGE ( 'NONE', *, *, #28036, .F. ) ;
#55151=LINE ( 'NONE', #46920, #40422 ) ;
#55152=CARTESIAN_POINT ( 'NONE',  ( -14.01545677930355183, 0.000000000000000000, 2.126011111488108174 ) ) ;
#55153=ORIENTED_EDGE ( 'NONE', *, *, #20954, .T. ) ;
#55154=CARTESIAN_POINT ( 'NONE',  ( -16.91060339984674599, 2.714935509636507316, 7.905645463759363167 ) ) ;
#55155=ORIENTED_EDGE ( 'NONE', *, *, #38819, .T. ) ;
#55156=CARTESIAN_POINT ( 'NONE',  ( -11.84964020568542686, 0.6102101463440048335, 2.485582596757569984 ) ) ;
#55157=CARTESIAN_POINT ( 'NONE',  ( -12.80458192191714595, 0.000000000000000000, 11.86454056839041726 ) ) ;
#55158=AXIS2_PLACEMENT_3D ( 'NONE', #2989, #37939, #40607 ) ;
#55159=ORIENTED_EDGE ( 'NONE', *, *, #44902, .F. ) ;
#55161=DIRECTION ( 'NONE',  ( -0.5449076811759708816, 0.6444004775717707689, 0.5364919789714475140 ) ) ;
#55162=ORIENTED_EDGE ( 'NONE', *, *, #24523, .F. ) ;
#55163=EDGE_CURVE ( 'NONE', #14660, #50517, #26140, .T. ) ;
#55164=LINE ( 'NONE', #37268, #10153 ) ;
#55165=LINE ( 'NONE', #25346, #4845 ) ;
#55166=DIRECTION ( 'NONE',  ( 0.5449076811759707706, 0.6444004775717708799, -0.5364919789714476250 ) ) ;
#55167=DIRECTION ( 'NONE',  ( 0.9999697198139515519, 0.000000000000000000, 0.007781995580013368816 ) ) ;
#55168=CARTESIAN_POINT ( 'NONE',  ( -11.61553128243660105, 0.000000000000000000, 4.191354291887420480 ) ) ;
#55169=CARTESIAN_POINT ( 'NONE',  ( -18.67619601524082285, 0.000000000000000000, 3.936400510096834893 ) ) ;
#55170=VERTEX_POINT ( 'NONE', #9086 ) ;
#55173=DIRECTION ( 'NONE',  ( -0.5364919789714478471, 0.6444004775717705469, -0.5449076811759709926 ) ) ;
#55175=DIRECTION ( 'NONE',  ( 0.9999697198139515519, 0.000000000000000000, 0.007781995580013368816 ) ) ;
#55176=DIRECTION ( 'NONE',  ( -0.9999697198139514409, -0.000000000000000000, -0.007781995580013368816 ) ) ;
#55177=CARTESIAN_POINT ( 'NONE',  ( -15.85491555274374065, 0.9340140483890049250, 4.572784929179271707 ) ) ;
#55178=EDGE_LOOP ( 'NONE', ( #32110, #12788, #20053, #13633 ) ) ;
#55179=PLANE ( 'NONE',  #7750 ) ;
#55182=FACE_OUTER_BOUND ( 'NONE', #31354, .T. ) ;
#55183=ORIENTED_EDGE ( 'NONE', *, *, #50432, .T. ) ;
#55184=DIRECTION ( 'NONE',  ( 0.007781995580012662783, 0.000000000000000000, -0.9999697198139514409 ) ) ;
#55185=LINE ( 'NONE', #16552, #14281 ) ;
#55186=EDGE_CURVE ( 'NONE', #40778, #14783, #31530, .T. ) ;
#55187=DIRECTION ( 'NONE',  ( -0.005002170337468016433, -0.7660444431189770143, 0.6427681459581293666 ) ) ;
#55188=FACE_OUTER_BOUND ( 'NONE', #31576, .T. ) ;
#55190=VERTEX_POINT ( 'NONE', #17606 ) ;
#55191=VERTEX_POINT ( 'NONE', #38918 ) ;
#55193=DIRECTION ( 'NONE',  ( 0.000000000000000000, -1.000000000000000000, 0.000000000000000000 ) ) ;
#55194=LINE ( 'NONE', #42427, #8851 ) ;
#55195=EDGE_CURVE ( 'NONE', #27480, #48023, #765, .T. ) ;
#55196=DIRECTION ( 'NONE',  ( 0.000000000000000000, -0.000000000000000000, -1.000000000000000000 ) ) ;
#55197=AXIS2_PLACEMENT_3D ( 'NONE', #40096, #1185, #9156 ) ;
#55198=FACE_OUTER_BOUND ( 'NONE', #15142, .T. ) ;
#55199=CARTESIAN_POINT ( 'NONE',  ( -3.638580343741060652, 5.221061972330257817, -1.805025403446173682 ) ) ;
#55200=ORIENTED_EDGE ( 'NONE', *, *, #39985, .T. ) ;
#55201=ADVANCED_FACE ( 'NONE', ( #21604 ), #4291, .F. ) ;
#55202=DIRECTION ( 'NONE',  ( 0.5364919789714477361, 0.6444004775717706579, 0.5449076811759711036 ) ) ;
#55204=PLANE ( 'NONE',  #15109 ) ;
#55205=LINE ( 'NONE', #8077, #40547 ) ;
#55206=VERTEX_POINT ( 'NONE', #1103 ) ;
#55207=LINE ( 'NONE', #37312, #8432 ) ;
#55208=EDGE_CURVE ( 'NONE', #47873, #45359, #30936, .T. ) ;
#55209=DIRECTION ( 'NONE',  ( 0.007781995580012663651, 0.000000000000000000, -0.9999697198139515519 ) ) ;
#55210=DIRECTION ( 'NONE',  ( 0.9999697198139515519, 0.000000000000000000, 0.007781995580013368816 ) ) ;
#55211=EDGE_LOOP ( 'NONE', ( #16718, #52571, #4947, #8794 ) ) ;
#55212=FACE_OUTER_BOUND ( 'NONE', #38140, .T. ) ;
#55213=ADVANCED_FACE ( 'NONE', ( #578 ), #17908, .F. ) ;
#55214=ORIENTED_EDGE ( 'NONE', *, *, #45068, .T. ) ;
#55215=ADVANCED_FACE ( 'NONE', ( #13371 ), #35232, .F. ) ;
#55216=VERTEX_POINT ( 'NONE', #839 ) ;
#55217=ORIENTED_EDGE ( 'NONE', *, *, #44030, .F. ) ;
#55218=ORIENTED_EDGE ( 'NONE', *, *, #48695, .T. ) ;
#55219=PLANE ( 'NONE',  #31144 ) ;
#55220=EDGE_LOOP ( 'NONE', ( #27022, #20864, #24595, #13191 ) ) ;
#55222=EDGE_CURVE ( 'NONE', #43469, #40926, #35481, .T. ) ;
#55224=DIRECTION ( 'NONE',  ( -0.7660212471507179544, -0.6427876096865405842, -0.005961354470445141482 ) ) ;
#55225=ORIENTED_EDGE ( 'NONE', *, *, #10, .F. ) ;
#55226=ORIENTED_EDGE ( 'NONE', *, *, #19962, .T. ) ;
#55227=ADVANCED_FACE ( 'NONE', ( #31224 ), #26985, .F. ) ;
#55228=LINE ( 'NONE', #15476, #15689 ) ;
#55229=CARTESIAN_POINT ( 'NONE',  ( -11.82989549392580031, 0.000000000000000000, 6.036346409060238116 ) ) ;
#55230=CARTESIAN_POINT ( 'NONE',  ( -18.07890891700271041, -2.137015261443157232, 7.211600032455043774 ) ) ;
#55231=DIRECTION ( 'NONE',  ( -0.7660212471507179544, -0.6427876096865405842, -0.005961354470445141482 ) ) ;
#55232=ORIENTED_EDGE ( 'NONE', *, *, #7163, .T. ) ;
#55233=VECTOR ( 'NONE', #41501, 1000.000000000000227 ) ;
#55234=ORIENTED_EDGE ( 'NONE', *, *, #43473, .T. ) ;
#55235=CARTESIAN_POINT ( 'NONE',  ( -15.90596353887472070, 0.4483081953215036219, 3.795487648738061104 ) ) ;
#55236=CARTESIAN_POINT ( 'NONE',  ( -19.28516736416668920, 0.000000000000000000, 7.994314122122347932 ) ) ;
#55237=DIRECTION ( 'NONE',  ( 0.007781995580012663651, 0.000000000000000000, -0.9999697198139515519 ) ) ;
#55239=FACE_OUTER_BOUND ( 'NONE', #51203, .T. ) ;
#55240=CARTESIAN_POINT ( 'NONE',  ( -9.110551994824897193, -1.000000000000000000, 3.538847790438064411 ) ) ;
#55241=ORIENTED_EDGE ( 'NONE', *, *, #2718, .T. ) ;
#55242=DIRECTION ( 'NONE',  ( 0.5364919789714477361, 0.6444004775717706579, 0.5449076811759711036 ) ) ;
#55243=FACE_OUTER_BOUND ( 'NONE', #31438, .T. ) ;
#55244=ORIENTED_EDGE ( 'NONE', *, *, #7375, .T. ) ;
#55245=PLANE ( 'NONE',  #53350 ) ;
#55246=CARTESIAN_POINT ( 'NONE',  ( -12.17938695170108154, -0.1191753592594188005, 4.086963208580010054 ) ) ;
#55247=DIRECTION ( 'NONE',  ( -0.7660212471507179544, -0.6427876096865405842, -0.005961354470445141482 ) ) ;
#55248=EDGE_CURVE ( 'NONE', #2943, #9219, #43190, .T. ) ;
#55249=CARTESIAN_POINT ( 'NONE',  ( -27.99767448711536133, 0.000000000000000000, 7.557179307314289218 ) ) ;
#55250=CARTESIAN_POINT ( 'NONE',  ( -16.90534462099871860, -1.327505506330658891, 3.405576699991005984 ) ) ;
#55251=ORIENTED_EDGE ( 'NONE', *, *, #28545, .T. ) ;
#55253=CARTESIAN_POINT ( 'NONE',  ( -29.86197018149027116, 0.000000000000000000, 8.281335066757780083 ) ) ;
#55254=CARTESIAN_POINT ( 'NONE',  ( -15.55980453706489541, 0.000000000000000000, 7.653973687242195290 ) ) ;
#55255=FACE_OUTER_BOUND ( 'NONE', #30880, .T. ) ;
#55256=EDGE_CURVE ( 'NONE', #48949, #11834, #10506, .T. ) ;
#55257=ADVANCED_FACE ( 'NONE', ( #16080 ), #23548, .F. ) ;
#55258=DIRECTION ( 'NONE',  ( 0.007781995580012662783, 0.000000000000000000, -0.9999697198139514409 ) ) ;
#55259=CARTESIAN_POINT ( 'NONE',  ( -6.567513199491930465, 4.309502646206702536, -0.6673284152940708314 ) ) ;
#55260=LINE ( 'NONE', #29430, #53663 ) ;
#55261=LINE ( 'NONE', #45916, #38375 ) ;
#55263=LINE ( 'NONE', #16353, #15065 ) ;
#55264=FACE_OUTER_BOUND ( 'NONE', #41335, .T. ) ;
#55265=PLANE ( 'NONE',  #2002 ) ;
#55266=ORIENTED_EDGE ( 'NONE', *, *, #41909, .F. ) ;
#55267=LINE ( 'NONE', #16357, #39540 ) ;
#55269=ORIENTED_EDGE ( 'NONE', *, *, #34675, .F. ) ;
#55270=ADVANCED_FACE ( 'NONE', ( #53379 ), #10775, .F. ) ;
#55271=ORIENTED_EDGE ( 'NONE', *, *, #30236, .F. ) ;
#55272=EDGE_CURVE ( 'NONE', #21762, #39510, #6242, .T. ) ;
#55273=EDGE_LOOP ( 'NONE', ( #43509, #23045, #48504, #7596 ) ) ;
#55275=VERTEX_POINT ( 'NONE', #28083 ) ;
#55276=ORIENTED_EDGE ( 'NONE', *, *, #16957, .F. ) ;
#55277=CARTESIAN_POINT ( 'NONE',  ( -15.86710544311044302, 0.000000000000000000, 13.13336954653252953 ) ) ;
#55278=FACE_OUTER_BOUND ( 'NONE', #12122, .T. ) ;
#55279=CARTESIAN_POINT ( 'NONE',  ( -21.47263955680318404, 0.000000000000000000, 5.022634149262071190 ) ) ;
#55280=EDGE_CURVE ( 'NONE', #23505, #27112, #40861, .T. ) ;
#55282=DIRECTION ( 'NONE',  ( -0.005002170337468016433, -0.7660444431189770143, 0.6427681459581293666 ) ) ;
#55283=ORIENTED_EDGE ( 'NONE', *, *, #13909, .T. ) ;
#55284=CARTESIAN_POINT ( 'NONE',  ( -16.81345671998191449, 0.000000000000000000, 3.412238694616132495 ) ) ;
#55285=ORIENTED_EDGE ( 'NONE', *, *, #53498, .F. ) ;
#55287=DIRECTION ( 'NONE',  ( 0.9999697198139515519, 0.000000000000000000, 0.007781995580013368816 ) ) ;
#55289=VERTEX_POINT ( 'NONE', #36607 ) ;
#55290=DIRECTION ( 'NONE',  ( 0.5449076811759707706, 0.6444004775717708799, -0.5364919789714476250 ) ) ;
#55291=ORIENTED_EDGE ( 'NONE', *, *, #13316, .F. ) ;
#55292=DIRECTION ( 'NONE',  ( 0.9999697198139515519, 0.000000000000000000, 0.007781995580013368816 ) ) ;
#55293=CARTESIAN_POINT ( 'NONE',  ( -17.36532418587302473, -0.1191753592594177458, 13.67570816655714516 ) ) ;
#55294=DIRECTION ( 'NONE',  ( 0.5364919789714477361, 0.6444004775717706579, 0.5449076811759711036 ) ) ;
#55295=CARTESIAN_POINT ( 'NONE',  ( -13.27065584551087163, 0.000000000000000000, 12.04557950825129176 ) ) ;
#55296=CARTESIAN_POINT ( 'NONE',  ( -14.80174839320972779, 0.000000000000000000, 8.967875321077752204 ) ) ;
#55297=LINE ( 'NONE', #16390, #5848 ) ;
#55298=DIRECTION ( 'NONE',  ( -0.6427681459581293666, -0.7660444431189770143, -0.005002170337467561935 ) ) ;
#55299=LINE ( 'NONE', #16392, #26822 ) ;
#55300=VERTEX_POINT ( 'NONE', #54986 ) ;
#55301=DIRECTION ( 'NONE',  ( -0.7660212471507179544, -0.6427876096865405842, -0.005961354470445141482 ) ) ;
#55303=EDGE_CURVE ( 'NONE', #51521, #56197, #37658, .T. ) ;
#55304=PLANE ( 'NONE',  #24712 ) ;
#55305=CARTESIAN_POINT ( 'NONE',  ( -31.72782227498118601, 0.000000000000000000, 9.205484770164058972 ) ) ;
#55306=CARTESIAN_POINT ( 'NONE',  ( -18.19747506107908563, 0.000000000000000000, 14.03856424583689311 ) ) ;
#55307=EDGE_CURVE ( 'NONE', #6779, #28682, #11798, .T. ) ;
#55308=CARTESIAN_POINT ( 'NONE',  ( -18.50873683370415179, -1.003701604285656579, 5.518599004666138619 ) ) ;
#55309=CARTESIAN_POINT ( 'NONE',  ( -8.609916609573598834, 0.000000000000000000, 10.23519010964256637 ) ) ;
#55310=CARTESIAN_POINT ( 'NONE',  ( -22.40634380310664397, 0.000000000000000000, 5.584705972946605534 ) ) ;
#55312=EDGE_LOOP ( 'NONE', ( #46910, #27275, #34553, #40628 ) ) ;
#55313=ADVANCED_FACE ( 'NONE', ( #29119 ), #23284, .F. ) ;
#55314=DIRECTION ( 'NONE',  ( -0.005002170337468016433, -0.7660444431189770143, 0.6427681459581293666 ) ) ;
#55316=PLANE ( 'NONE',  #44888 ) ;
#55317=LINE ( 'NONE', #21245, #39094 ) ;
#55318=ADVANCED_FACE ( 'NONE', ( #1401 ), #46425, .F. ) ;
#55319=EDGE_CURVE ( 'NONE', #34341, #29949, #45390, .T. ) ;
#55320=ADVANCED_FACE ( 'NONE', ( #20628 ), #55245, .F. ) ;
#55321=CARTESIAN_POINT ( 'NONE',  ( -18.61669932361099455, 0.000000000000000000, 8.199522351202686465 ) ) ;
#55323=EDGE_CURVE ( 'NONE', #41560, #12727, #33658, .T. ) ;
#55324=LINE ( 'NONE', #16417, #25918 ) ;
#55325=PLANE ( 'NONE',  #43757 ) ;
#55326=ORIENTED_EDGE ( 'NONE', *, *, #51920, .F. ) ;
#55327=LINE ( 'NONE', #33219, #55735 ) ;
#55328=FACE_OUTER_BOUND ( 'NONE', #6090, .T. ) ;
#55329=ORIENTED_EDGE ( 'NONE', *, *, #24121, .T. ) ;
#55330=ORIENTED_EDGE ( 'NONE', *, *, #8653, .F. ) ;
#55332=ORIENTED_EDGE ( 'NONE', *, *, #5673, .T. ) ;
#55334=ORIENTED_EDGE ( 'NONE', *, *, #48874, .T. ) ;
#55335=LINE ( 'NONE', #7352, #46503 ) ;
#55336=AXIS2_PLACEMENT_3D ( 'NONE', #9599, #18675, #36018 ) ;
#55338=ORIENTED_EDGE ( 'NONE', *, *, #36943, .T. ) ;
#55339=ORIENTED_EDGE ( 'NONE', *, *, #37233, .T. ) ;
#55340=VERTEX_POINT ( 'NONE', #14742 ) ;
#55341=ADVANCED_FACE ( 'NONE', ( #49387 ), #55818, .F. ) ;
#55342=DIRECTION ( 'NONE',  ( 0.005002170337468016433, -0.7660444431189770143, -0.6427681459581293666 ) ) ;
#55344=CARTESIAN_POINT ( 'NONE',  ( -13.27065584551087163, 0.000000000000000000, 12.04557950825129176 ) ) ;
#55345=EDGE_CURVE ( 'NONE', #41612, #5753, #52109, .T. ) ;
#55346=ORIENTED_EDGE ( 'NONE', *, *, #8270, .T. ) ;
#55347=ORIENTED_EDGE ( 'NONE', *, *, #3228, .T. ) ;
#55348=EDGE_CURVE ( 'NONE', #52427, #36412, #50970, .T. ) ;
#55349=CARTESIAN_POINT ( 'NONE',  ( -17.36532418587302473, -0.1191753592594177458, 13.67570816655714516 ) ) ;
#55350=PLANE ( 'NONE',  #56 ) ;
#55352=DIRECTION ( 'NONE',  ( 0.007781995580012662783, 0.000000000000000000, -0.9999697198139514409 ) ) ;
#55353=CARTESIAN_POINT ( 'NONE',  ( -19.61547266693814251, -2.298917212465658277, 8.074162258805023029 ) ) ;
#55354=ORIENTED_EDGE ( 'NONE', *, *, #44899, .F. ) ;
#55355=FACE_OUTER_BOUND ( 'NONE', #45638, .T. ) ;
#55356=PLANE ( 'NONE',  #34892 ) ;
#55357=ORIENTED_EDGE ( 'NONE', *, *, #23093, .F. ) ;
#55358=FACE_OUTER_BOUND ( 'NONE', #18935, .T. ) ;
#55359=DIRECTION ( 'NONE',  ( 0.7660212471507180654, -0.6427876096865404731, 0.005961354470445141482 ) ) ;
#55360=ORIENTED_EDGE ( 'NONE', *, *, #31750, .T. ) ;
#55361=CARTESIAN_POINT ( 'NONE',  ( -17.40685591040811175, 0.000000000000000000, 6.162271227139100027 ) ) ;
#55362=DIRECTION ( 'NONE',  ( -0.3620778797217455991, 0.000000000000000000, -0.9321478471874540261 ) ) ;
#55363=CARTESIAN_POINT ( 'NONE',  ( -11.68519433167736743, -3.432230869623161595, 1.310741292032489236 ) ) ;
#55364=CARTESIAN_POINT ( 'NONE',  ( -15.80875956802750260, 0.000000000000000000, 5.636049899006391861 ) ) ;
#55365=ORIENTED_EDGE ( 'NONE', *, *, #2818, .T. ) ;
#55366=VECTOR ( 'NONE', #42860, 1000.000000000000227 ) ;
#55367=DIRECTION ( 'NONE',  ( 0.9999697198139515519, 0.000000000000000000, 0.007781995580013368816 ) ) ;
#55368=CARTESIAN_POINT ( 'NONE',  ( -17.31082735807079587, 4.819660872929009798, 11.51531893215243230 ) ) ;
#55369=DIRECTION ( 'NONE',  ( 0.007781995580012662783, 0.000000000000000000, -0.9999697198139514409 ) ) ;
#55370=LINE ( 'NONE', #46877, #3225 ) ;
#55371=CARTESIAN_POINT ( 'NONE',  ( -12.13851405436063047, 0.000000000000000000, 11.68505802764555135 ) ) ;
#55372=DIRECTION ( 'NONE',  ( -0.2426528472758542054, 0.7422098413412800966, -0.6246952433987894571 ) ) ;
#55373=AXIS2_PLACEMENT_3D ( 'NONE', #16214, #21016, #8538 ) ;
#55374=CARTESIAN_POINT ( 'NONE',  ( -12.99638935982272514, 0.000000000000000000, 2.503273799589543991 ) ) ;
#55375=VERTEX_POINT ( 'NONE', #47867 ) ;
#55376=DIRECTION ( 'NONE',  ( 0.005961354470445682716, -0.6427876096865404731, -0.7660212471507180654 ) ) ;
#55377=FACE_OUTER_BOUND ( 'NONE', #29373, .T. ) ;
#55378=ORIENTED_EDGE ( 'NONE', *, *, #31181, .T. ) ;
#55379=PLANE ( 'NONE',  #22946 ) ;
#55380=DIRECTION ( 'NONE',  ( 0.000000000000000000, -1.000000000000000000, 0.000000000000000000 ) ) ;
#55381=EDGE_CURVE ( 'NONE', #40111, #21762, #3569, .T. ) ;
#55382=EDGE_CURVE ( 'NONE', #1435, #47262, #4146, .T. ) ;
#55383=CARTESIAN_POINT ( 'NONE',  ( -19.60912206198629804, -0.1191753592594194527, 4.398475361799976113 ) ) ;
#55384=ADVANCED_FACE ( 'NONE', ( #30560 ), #17461, .F. ) ;
#55385=CARTESIAN_POINT ( 'NONE',  ( -16.81345671998191449, 0.000000000000000000, 3.412238694616132495 ) ) ;
#55386=DIRECTION ( 'NONE',  ( 0.005002170337468016433, -0.7660444431189770143, -0.6427681459581293666 ) ) ;
#55387=ORIENTED_EDGE ( 'NONE', *, *, #45827, .T. ) ;
#55388=ORIENTED_EDGE ( 'NONE', *, *, #4134, .T. ) ;
#55390=LINE ( 'NONE', #20764, #11406 ) ;
#55391=DIRECTION ( 'NONE',  ( -0.005002170337468016433, -0.7660444431189770143, 0.6427681459581293666 ) ) ;
#55392=ORIENTED_EDGE ( 'NONE', *, *, #29292, .T. ) ;
#55394=VECTOR ( 'NONE', #49713, 999.9999999999998863 ) ;
#55395=ORIENTED_EDGE ( 'NONE', *, *, #16253, .T. ) ;
#55396=CARTESIAN_POINT ( 'NONE',  ( -16.33317936670417225, 0.000000000000000000, 13.31440848639340224 ) ) ;
#55397=ORIENTED_EDGE ( 'NONE', *, *, #15443, .F. ) ;
#55398=CARTESIAN_POINT ( 'NONE',  ( -16.83150402712250227, -0.1191753592594197719, 4.789423497415446818 ) ) ;
#55399=EDGE_LOOP ( 'NONE', ( #5002, #24846, #43907, #46136 ) ) ;
#55401=EDGE_LOOP ( 'NONE', ( #38957, #39583, #27639, #7432 ) ) ;
#55402=DIRECTION ( 'NONE',  ( 0.000000000000000000, 1.000000000000000000, 0.000000000000000000 ) ) ;
#55403=CARTESIAN_POINT ( 'NONE',  ( -8.840523769800496368, 0.000000000000000000, 5.859604334821510108 ) ) ;
#55404=CARTESIAN_POINT ( 'NONE',  ( -9.280526530289439080, -2.201020558340975430, 3.101258514253283138 ) ) ;
#55405=AXIS2_PLACEMENT_3D ( 'NONE', #48229, #35464, #53078 ) ;
#55406=CARTESIAN_POINT ( 'NONE',  ( -2.276746449950904694, -3.901742918183043418, -2.334007935867973949 ) ) ;
#55407=ORIENTED_EDGE ( 'NONE', *, *, #26353, .T. ) ;
#55408=ADVANCED_FACE ( 'NONE', ( #39335 ), #38489, .F. ) ;
#55410=ORIENTED_EDGE ( 'NONE', *, *, #46940, .F. ) ;
#55411=VERTEX_POINT ( 'NONE', #12658 ) ;
#55412=LINE ( 'NONE', #21355, #53985 ) ;
#55413=ADVANCED_FACE ( 'NONE', ( #42481 ), #26019, .F. ) ;
#55414=CARTESIAN_POINT ( 'NONE',  ( -15.88053067323646417, -0.1191753592594197858, 2.950163842912994383 ) ) ;
#55415=VERTEX_POINT ( 'NONE', #29974 ) ;
#55416=DIRECTION ( 'NONE',  ( -0.005002170337468016433, -0.7660444431189770143, 0.6427681459581293666 ) ) ;
#55417=ADVANCED_FACE ( 'NONE', ( #8968 ), #4688, .F. ) ;
#55418=ORIENTED_EDGE ( 'NONE', *, *, #42389, .T. ) ;
#55419=DIRECTION ( 'NONE',  ( -0.005961354470445682716, -0.6427876096865404731, 0.7660212471507180654 ) ) ;
#55420=PLANE ( 'NONE',  #45723 ) ;
#55421=ORIENTED_EDGE ( 'NONE', *, *, #33192, .F. ) ;
#55422=EDGE_CURVE ( 'NONE', #42447, #48276, #56105, .T. ) ;
#55424=ORIENTED_EDGE ( 'NONE', *, *, #18890, .F. ) ;
#55425=FACE_OUTER_BOUND ( 'NONE', #9555, .T. ) ;
#55427=ORIENTED_EDGE ( 'NONE', *, *, #28059, .F. ) ;
#55428=DIRECTION ( 'NONE',  ( -0.3620778797217456546, 0.000000000000000000, -0.9321478471874540261 ) ) ;
#55429=LINE ( 'NONE', #48039, #24796 ) ;
#55430=FACE_OUTER_BOUND ( 'NONE', #30495, .T. ) ;
#55431=CARTESIAN_POINT ( 'NONE',  ( -20.09291730366250306, -0.1191753592594199662, 5.914810210573124394 ) ) ;
#55432=ORIENTED_EDGE ( 'NONE', *, *, #7298, .T. ) ;
#55434=ORIENTED_EDGE ( 'NONE', *, *, #41735, .F. ) ;
#55435=VECTOR ( 'NONE', #47123, 999.9999999999998863 ) ;
#55436=CARTESIAN_POINT ( 'NONE',  ( -12.80458192191714595, 0.000000000000000000, 11.86454056839041726 ) ) ;
#55437=FACE_OUTER_BOUND ( 'NONE', #19011, .T. ) ;
#55438=DIRECTION ( 'NONE',  ( 0.9999697198139515519, 0.000000000000000000, 0.007781995580013368816 ) ) ;
#55439=CARTESIAN_POINT ( 'NONE',  ( -14.42634509152537348, 0.000000000000000000, 7.124136447341477663 ) ) ;
#55440=FACE_OUTER_BOUND ( 'NONE', #4684, .T. ) ;
#55441=CARTESIAN_POINT ( 'NONE',  ( -17.93139508144814442, 0.000000000000000000, 13.85596890686001537 ) ) ;
#55442=ORIENTED_EDGE ( 'NONE', *, *, #54314, .T. ) ;
#55443=CARTESIAN_POINT ( 'NONE',  ( -18.67619601524082285, 0.000000000000000000, 3.936400510096834893 ) ) ;
#55444=CARTESIAN_POINT ( 'NONE',  ( -17.73140113748535285, 0.000000000000000000, 13.85752530597602039 ) ) ;
#55446=DIRECTION ( 'NONE',  ( 0.2426528472758541499, 0.7422098413412800966, 0.6246952433987894571 ) ) ;
#55447=ORIENTED_EDGE ( 'NONE', *, *, #3039, .T. ) ;
#55448=EDGE_CURVE ( 'NONE', #23248, #5370, #21738, .T. ) ;
#55449=PLANE ( 'NONE',  #24344 ) ;
#55451=CARTESIAN_POINT ( 'NONE',  ( -13.63673279712320507, -0.1191753592594197858, 12.22739664767016521 ) ) ;
#55452=LINE ( 'NONE', #42121, #9623 ) ;
#55453=ADVANCED_FACE ( 'NONE', ( #12077 ), #47574, .F. ) ;
#55455=DIRECTION ( 'NONE',  ( -0.5364919789714478471, 0.6444004775717705469, -0.5449076811759709926 ) ) ;
#55456=AXIS2_PLACEMENT_3D ( 'NONE', #14790, #39529, #620 ) ;
#55458=VERTEX_POINT ( 'NONE', #17191 ) ;
#55459=ORIENTED_EDGE ( 'NONE', *, *, #31929, .T. ) ;
#55460=CARTESIAN_POINT ( 'NONE',  ( -14.94838282604900748, -0.1191753592594197858, 2.588085963191248506 ) ) ;
#55461=CARTESIAN_POINT ( 'NONE',  ( -14.01701317841955508, 0.000000000000000000, 2.326005055450897085 ) ) ;
#55462=LINE ( 'NONE', #20264, #37857 ) ;
#55463=CARTESIAN_POINT ( 'NONE',  ( 4.452747148193316740, -1.000000000000000000, 0.4159841754879232689 ) ) ;
#55464=LINE ( 'NONE', #21417, #4740 ) ;
#55466=ORIENTED_EDGE ( 'NONE', *, *, #28986, .F. ) ;
#55467=CARTESIAN_POINT ( 'NONE',  ( -18.86354292863559579, 0.000000000000000000, 14.21804678658176080 ) ) ;
#55468=EDGE_CURVE ( 'NONE', #49012, #41524, #16624, .T. ) ;
#55469=DIRECTION ( 'NONE',  ( 0.007781995580012662783, 0.000000000000000000, -0.9999697198139514409 ) ) ;
#55470=CARTESIAN_POINT ( 'NONE',  ( -18.67697421479882181, -0.1191753592594197858, 4.036397482078229793 ) ) ;
#55471=ORIENTED_EDGE ( 'NONE', *, *, #38815, .T. ) ;
#55472=DIRECTION ( 'NONE',  ( -0.6427681459581293666, -0.7660444431189770143, -0.005002170337467561935 ) ) ;
#55473=LINE ( 'NONE', #16297, #26798 ) ;
#55474=LINE ( 'NONE', #51231, #44741 ) ;
#55475=ORIENTED_EDGE ( 'NONE', *, *, #29274, .T. ) ;
#55476=VECTOR ( 'NONE', #137, 999.9999999999998863 ) ;
#55477=AXIS2_PLACEMENT_3D ( 'NONE', #15416, #18870, #11153 ) ;
#55478=LINE ( 'NONE', #38754, #12174 ) ;
#55479=VERTEX_POINT ( 'NONE', #30259 ) ;
#55480=EDGE_LOOP ( 'NONE', ( #32490, #49227, #22027, #33423 ) ) ;
#55481=VERTEX_POINT ( 'NONE', #8123 ) ;
#55482=VECTOR ( 'NONE', #27365, 999.9999999999998863 ) ;
#55483=ORIENTED_EDGE ( 'NONE', *, *, #14142, .T. ) ;
#55484=DIRECTION ( 'NONE',  ( 0.007781995580012663651, -3.146120232559066537E-19, -0.9999697198139514409 ) ) ;
#55485=EDGE_LOOP ( 'NONE', ( #49352, #53133, #30735, #39141 ) ) ;
#55486=CARTESIAN_POINT ( 'NONE',  ( -18.29747203306047609, -0.1191753592594177458, 14.03778604627889059 ) ) ;
#55487=ORIENTED_EDGE ( 'NONE', *, *, #3914, .F. ) ;
#55488=CARTESIAN_POINT ( 'NONE',  ( -11.20636620717317378, 0.000000000000000000, 11.32298014792380414 ) ) ;
#55489=EDGE_CURVE ( 'NONE', #54036, #2726, #25427, .T. ) ;
#55490=VERTEX_POINT ( 'NONE', #4429 ) ;
#55491=AXIS2_PLACEMENT_3D ( 'NONE', #10416, #49020, #23474 ) ;
#55492=ORIENTED_EDGE ( 'NONE', *, *, #25017, .F. ) ;
#55493=AXIS2_PLACEMENT_3D ( 'NONE', #40715, #10636, #27656 ) ;
#55494=LINE ( 'NONE', #12907, #39300 ) ;
#55495=LINE ( 'NONE', #13201, #35929 ) ;
#55496=CARTESIAN_POINT ( 'NONE',  ( -17.68874318431810266, 0.000000000000000000, 8.376069934033679942 ) ) ;
#55497=CARTESIAN_POINT ( 'NONE',  ( -20.71696439550653324, 1.743523803501507485, 4.673476716096989669 ) ) ;
#55498=PLANE ( 'NONE',  #35604 ) ;
#55499=ORIENTED_EDGE ( 'NONE', *, *, #6299, .F. ) ;
#55500=ADVANCED_FACE ( 'NONE', ( #39051 ), #27379, .F. ) ;
#55501=VERTEX_POINT ( 'NONE', #35357 ) ;
#55502=LINE ( 'NONE', #41356, #31299 ) ;
#55503=CARTESIAN_POINT ( 'NONE',  ( -24.27063949748155380, 0.000000000000000000, 6.308861732390097288 ) ) ;
#55505=EDGE_CURVE ( 'NONE', #53403, #43303, #9223, .T. ) ;
#55506=DIRECTION ( 'NONE',  ( -0.6427681459581293666, -0.7660444431189770143, -0.005002170337467561935 ) ) ;
#55507=DIRECTION ( 'NONE',  ( 0.6427681459581294776, -0.7660444431189769032, 0.005002170337467562802 ) ) ;
#55508=DIRECTION ( 'NONE',  ( 0.005002170337468016433, -0.7660444431189770143, -0.6427681459581293666 ) ) ;
#55509=DIRECTION ( 'NONE',  ( 0.005002170337468016433, -0.7660444431189770143, -0.6427681459581293666 ) ) ;
#55510=ORIENTED_EDGE ( 'NONE', *, *, #31174, .T. ) ;
#55511=VECTOR ( 'NONE', #20694, 1000.000000000000227 ) ;
#55512=LINE ( 'NONE', #30256, #2037 ) ;
#55513=EDGE_CURVE ( 'NONE', #35388, #21352, #40165, .T. ) ;
#55515=VERTEX_POINT ( 'NONE', #18294 ) ;
#55516=VECTOR ( 'NONE', #25380, 999.9999999999998863 ) ;
#55517=VECTOR ( 'NONE', #36595, 999.9999999999998863 ) ;
#55519=CARTESIAN_POINT ( 'NONE',  ( -17.78377024884693469, -0.1191753592594177180, 7.736669299941538291 ) ) ;
#55520=EDGE_CURVE ( 'NONE', #29513, #27257, #35634, .T. ) ;
#55521=DIRECTION ( 'NONE',  ( 0.6427681459581294776, -0.7660444431189769032, 0.005002170337467562802 ) ) ;
#55522=DIRECTION ( 'NONE',  ( 0.9999697198139515519, 0.000000000000000000, 0.007781995580013368816 ) ) ;
#55523=ADVANCED_FACE ( 'NONE', ( #39637 ), #27680, .F. ) ;
#55524=DIRECTION ( 'NONE',  ( -0.005002170337468016433, -0.7660444431189770143, 0.6427681459581293666 ) ) ;
#55525=EDGE_LOOP ( 'NONE', ( #25264, #10851, #14639, #53232, #23633 ) ) ;
#55526=VECTOR ( 'NONE', #48200, 1000.000000000000227 ) ;
#55527=VECTOR ( 'NONE', #6559, 1000.000000000000227 ) ;
#55528=ORIENTED_EDGE ( 'NONE', *, *, #42920, .F. ) ;
#55529=DIRECTION ( 'NONE',  ( 0.9999697198139515519, 0.000000000000000000, 0.007781995580013368816 ) ) ;
#55531=LINE ( 'NONE', #47030, #31544 ) ;
#55532=EDGE_CURVE ( 'NONE', #16370, #42656, #715, .T. ) ;
#55533=DIRECTION ( 'NONE',  ( 0.000000000000000000, -0.000000000000000000, -1.000000000000000000 ) ) ;
#55534=VECTOR ( 'NONE', #19399, 999.9999999999998863 ) ;
#55536=CARTESIAN_POINT ( 'NONE',  ( -15.78995884787980053, 0.000000000000000000, 3.220197735497015934 ) ) ;
#55537=DIRECTION ( 'NONE',  ( -0.005961354470445682716, -0.6427876096865404731, 0.7660212471507180654 ) ) ;
#55538=EDGE_CURVE ( 'NONE', #8731, #16665, #52403, .T. ) ;
#55539=DIRECTION ( 'NONE',  ( -0.9999697198139514409, -0.000000000000000000, -0.007781995580013368816 ) ) ;
#55541=CARTESIAN_POINT ( 'NONE',  ( -18.75513958955402316, -4.079838673713163111, 4.036286046993806664 ) ) ;
#55542=VERTEX_POINT ( 'NONE', #14059 ) ;
#55543=DIRECTION ( 'NONE',  ( -0.3620778797217457101, 0.000000000000000000, -0.9321478471874540261 ) ) ;
#55544=ORIENTED_EDGE ( 'NONE', *, *, #4885, .T. ) ;
#55545=AXIS2_PLACEMENT_3D ( 'NONE', #44706, #35638, #39896 ) ;
#55546=VERTEX_POINT ( 'NONE', #31390 ) ;
#55547=VERTEX_POINT ( 'NONE', #48710 ) ;
#55548=VERTEX_POINT ( 'NONE', #10066 ) ;
#55549=EDGE_LOOP ( 'NONE', ( #48705, #32788, #3599, #39563 ) ) ;
#55550=ORIENTED_EDGE ( 'NONE', *, *, #33559, .T. ) ;
#55551=VECTOR ( 'NONE', #12612, 999.9999999999998863 ) ;
#55552=LINE ( 'NONE', #24906, #25111 ) ;
#55553=CARTESIAN_POINT ( 'NONE',  ( -16.50213094388420387, 0.000000000000000000, 9.323974620700020921 ) ) ;
#55555=VECTOR ( 'NONE', #20409, 1000.000000000000114 ) ;
#55556=VECTOR ( 'NONE', #55242, 999.9999999999998863 ) ;
#55557=ORIENTED_EDGE ( 'NONE', *, *, #19818, .T. ) ;
#55558=CARTESIAN_POINT ( 'NONE',  ( -14.87171971942530568, 1.419719901456505395, 4.988004329898734213 ) ) ;
#55559=ADVANCED_FACE ( 'NONE', ( #9813 ), #13502, .F. ) ;
#55560=VERTEX_POINT ( 'NONE', #18035 ) ;
#55562=ORIENTED_EDGE ( 'NONE', *, *, #998, .T. ) ;
#55563=AXIS2_PLACEMENT_3D ( 'NONE', #51839, #18057, #35377 ) ;
#55564=AXIS2_PLACEMENT_3D ( 'NONE', #33722, #29780, #47077 ) ;
#55565=CARTESIAN_POINT ( 'NONE',  ( -17.89029352739689926, 0.000000000000000000, 8.574507478880466493 ) ) ;
#55566=DIRECTION ( 'NONE',  ( -0.7660212471507179544, -0.6427876096865405842, -0.005961354470445141482 ) ) ;
#55567=FACE_OUTER_BOUND ( 'NONE', #29018, .T. ) ;
#55568=VERTEX_POINT ( 'NONE', #6375 ) ;
#55569=CARTESIAN_POINT ( 'NONE',  ( -15.09735569160282154, 2.229229656569007290, 6.404192423874666140 ) ) ;
#55570=ORIENTED_EDGE ( 'NONE', *, *, #53041, .F. ) ;
#55571=DIRECTION ( 'NONE',  ( 0.000000000000000000, -1.000000000000000000, 0.000000000000000000 ) ) ;
#55572=AXIS2_PLACEMENT_3D ( 'NONE', #12772, #7975, #32731 ) ;
#55573=CARTESIAN_POINT ( 'NONE',  ( -17.30371862263972815, 4.333955019861511992, 3.265007825402915120 ) ) ;
#55574=AXIS2_PLACEMENT_3D ( 'NONE', #466, #17808, #48152 ) ;
#55575=EDGE_CURVE ( 'NONE', #38023, #26804, #50061, .T. ) ;
#55576=PLANE ( 'NONE',  #28743 ) ;
#55577=LINE ( 'NONE', #16686, #27682 ) ;
#55578=PLANE ( 'NONE',  #28374 ) ;
#55579=DIRECTION ( 'NONE',  ( 0.9999697198139515519, 0.000000000000000000, 0.007781995580013368816 ) ) ;
#55580=DIRECTION ( 'NONE',  ( 0.9999697198139515519, 0.000000000000000000, 0.007781995580013368816 ) ) ;
#55582=VERTEX_POINT ( 'NONE', #2647 ) ;
#55585=VECTOR ( 'NONE', #29319, 1000.000000000000227 ) ;
#55586=CARTESIAN_POINT ( 'NONE',  ( -7.094024697029445825, 2.107956770024262294, 8.730276719704061605 ) ) ;
#55587=CARTESIAN_POINT ( 'NONE',  ( -15.88130887279446490, 0.000000000000000000, 3.050160814894388839 ) ) ;
#55588=ADVANCED_FACE ( 'NONE', ( #19715 ), #15709, .F. ) ;
#55589=CARTESIAN_POINT ( 'NONE',  ( -18.67775241435682432, 0.000000000000000000, 4.136394454059623804 ) ) ;
#55590=VECTOR ( 'NONE', #47148, 1000.000000000000000 ) ;
#55591=LINE ( 'NONE', #55308, #43961 ) ;
#55592=DIRECTION ( 'NONE',  ( -0.5449076811759708816, 0.6444004775717707689, 0.5364919789714475140 ) ) ;
#55593=EDGE_CURVE ( 'NONE', #23151, #47316, #49545, .T. ) ;
#55594=DIRECTION ( 'NONE',  ( 0.000000000000000000, -0.000000000000000000, -1.000000000000000000 ) ) ;
#55595=ORIENTED_EDGE ( 'NONE', *, *, #9959, .F. ) ;
#55596=VECTOR ( 'NONE', #30131, 1000.000000000000227 ) ;
#55597=LINE ( 'NONE', #8778, #5768 ) ;
#55598=PLANE ( 'NONE',  #54846 ) ;
#55599=CARTESIAN_POINT ( 'NONE',  ( -12.94718852056742975, -3.270328918600661883, 1.806108212387832923 ) ) ;
#55600=VECTOR ( 'NONE', #14080, 999.9999999999998863 ) ;
#55601=EDGE_CURVE ( 'NONE', #36400, #33244, #36760, .T. ) ;
#55602=VECTOR ( 'NONE', #2380, 1000.000000000000227 ) ;
#55603=DIRECTION ( 'NONE',  ( 0.7660212471507180654, -0.6427876096865404731, 0.005961354470445141482 ) ) ;
#55604=CARTESIAN_POINT ( 'NONE',  ( -27.06708303904391144, 0.000000000000000000, 7.395095371555332697 ) ) ;
#55605=LINE ( 'NONE', #47667, #3243 ) ;
#55606=DIRECTION ( 'NONE',  ( 0.000000000000000000, -1.000000000000000000, 0.000000000000000000 ) ) ;
#55607=ORIENTED_EDGE ( 'NONE', *, *, #45337, .T. ) ;
#55608=EDGE_CURVE ( 'NONE', #28729, #24227, #54078, .T. ) ;
#55609=VECTOR ( 'NONE', #24402, 1000.000000000000000 ) ;
#55610=CARTESIAN_POINT ( 'NONE',  ( -14.10890107943635385, -1.327505506330656670, 2.319343060825770131 ) ) ;
#55611=AXIS2_PLACEMENT_3D ( 'NONE', #1482, #6043, #905 ) ;
#55612=LINE ( 'NONE', #33745, #30531 ) ;
#55613=ORIENTED_EDGE ( 'NONE', *, *, #28869, .T. ) ;
#55614=ORIENTED_EDGE ( 'NONE', *, *, #48409, .T. ) ;
#55615=DIRECTION ( 'NONE',  ( 0.000000000000000000, 1.000000000000000000, 0.000000000000000000 ) ) ;
#55616=ORIENTED_EDGE ( 'NONE', *, *, #42055, .T. ) ;
#55617=VECTOR ( 'NONE', #55484, 1000.000000000000227 ) ;
#55618=ORIENTED_EDGE ( 'NONE', *, *, #18334, .F. ) ;
#55619=ORIENTED_EDGE ( 'NONE', *, *, #22966, .F. ) ;
#55620=EDGE_LOOP ( 'NONE', ( #3325, #31288, #36788, #26058 ) ) ;
#55623=DIRECTION ( 'NONE',  ( -0.005961354470445682716, -0.6427876096865404731, 0.7660212471507180654 ) ) ;
#55625=VERTEX_POINT ( 'NONE', #15188 ) ;
#55626=ADVANCED_FACE ( 'NONE', ( #37037 ), #28500, .F. ) ;
#55627=ORIENTED_EDGE ( 'NONE', *, *, #8032, .F. ) ;
#55628=VECTOR ( 'NONE', #20493, 1000.000000000000227 ) ;
#55629=ADVANCED_FACE ( 'NONE', ( #37582 ), #54908, .F. ) ;
#55631=DIRECTION ( 'NONE',  ( -0.5449076811759708816, 0.6444004775717707689, 0.5364919789714475140 ) ) ;
#55632=ORIENTED_EDGE ( 'NONE', *, *, #19438, .T. ) ;
#55633=ADVANCED_FACE ( 'NONE', ( #15432 ), #45819, .F. ) ;
#55634=AXIS2_PLACEMENT_3D ( 'NONE', #11505, #50673, #1833 ) ;
#55635=CARTESIAN_POINT ( 'NONE',  ( -23.33693525117809386, 0.000000000000000000, 5.746789908705562944 ) ) ;
#55636=CARTESIAN_POINT ( 'NONE',  ( -12.67276438359499124, -0.1191753592594168437, 7.776444329389642363 ) ) ;
#55637=ORIENTED_EDGE ( 'NONE', *, *, #13639, .T. ) ;
#55638=CARTESIAN_POINT ( 'NONE',  ( -17.58751131637929177, 5.143464774974010112, 12.15420974568715273 ) ) ;
#55640=ADVANCED_FACE ( 'NONE', ( #12006 ), #3222, .F. ) ;
#55641=EDGE_CURVE ( 'NONE', #31613, #40733, #30185, .T. ) ;
#55642=VECTOR ( 'NONE', #14335, 999.9999999999998863 ) ;
#55643=VECTOR ( 'NONE', #41687, 1000.000000000000227 ) ;
#55645=FACE_OUTER_BOUND ( 'NONE', #52550, .T. ) ;
#55646=AXIS2_PLACEMENT_3D ( 'NONE', #44363, #13984, #4624 ) ;
#55647=DIRECTION ( 'NONE',  ( -0.9999697198139514409, -0.000000000000000000, -0.007781995580013368816 ) ) ;
#55648=VECTOR ( 'NONE', #46227, 999.9999999999998863 ) ;
#55649=ORIENTED_EDGE ( 'NONE', *, *, #25010, .T. ) ;
#55650=DIRECTION ( 'NONE',  ( -0.005002170337468016433, -0.7660444431189770143, 0.6427681459581293666 ) ) ;
#55651=LINE ( 'NONE', #38906, #14768 ) ;
#55652=CARTESIAN_POINT ( 'NONE',  ( -14.85936739980835064, 0.000000000000000000, 3.058113799738058969 ) ) ;
#55653=PLANE ( 'NONE',  #25604 ) ;
#55654=EDGE_LOOP ( 'NONE', ( #6716, #38369, #626, #12013 ) ) ;
#55655=CARTESIAN_POINT ( 'NONE',  ( -28.93060053386082231, -0.1191753592594197858, 8.019254159017428663 ) ) ;
#55656=CARTESIAN_POINT ( 'NONE',  ( -9.213964613319133079, 8.977402042007843974, 6.797390339032328477 ) ) ;
#55657=DIRECTION ( 'NONE',  ( 0.005961354470445682716, -0.6427876096865404731, -0.7660212471507180654 ) ) ;
#55660=DIRECTION ( 'NONE',  ( 0.007781995580012663651, 0.000000000000000000, -0.9999697198139515519 ) ) ;
#55661=DIRECTION ( 'NONE',  ( -0.9999697198139514409, -0.000000000000000000, -0.007781995580013368816 ) ) ;
#55663=DIRECTION ( 'NONE',  ( 0.005002170337468016433, -0.7660444431189770143, -0.6427681459581293666 ) ) ;
#55664=AXIS2_PLACEMENT_3D ( 'NONE', #29618, #47177, #42381 ) ;
#55665=ORIENTED_EDGE ( 'NONE', *, *, #20357, .T. ) ;
#55667=ADVANCED_FACE ( 'NONE', ( #52037 ), #21399, .F. ) ;
#55669=ORIENTED_EDGE ( 'NONE', *, *, #45998, .F. ) ;
#55670=DIRECTION ( 'NONE',  ( 0.7660212471507180654, -0.6427876096865404731, 0.005961354470445141482 ) ) ;
#55671=DIRECTION ( 'NONE',  ( 0.9999697198139515519, 0.000000000000000000, 0.007781995580013368816 ) ) ;
#55672=AXIS2_PLACEMENT_3D ( 'NONE', #46414, #3557, #41876 ) ;
#55673=EDGE_CURVE ( 'NONE', #26368, #34449, #26213, .T. ) ;
#55674=DIRECTION ( 'NONE',  ( 0.5364919789714477361, 0.6444004775717706579, 0.5449076811759711036 ) ) ;
#55675=VECTOR ( 'NONE', #45326, 1000.000000000000114 ) ;
#55676=CARTESIAN_POINT ( 'NONE',  ( 2.072287782118878319, 0.000000000000000000, -2.950529333540147015 ) ) ;
#55677=LINE ( 'NONE', #15943, #14785 ) ;
#55678=EDGE_LOOP ( 'NONE', ( #25816, #31803, #13926, #380 ) ) ;
#55679=ORIENTED_EDGE ( 'NONE', *, *, #11972, .T. ) ;
#55680=CARTESIAN_POINT ( 'NONE',  ( -27.99923088623136636, 0.000000000000000000, 7.757173251277078130 ) ) ;
#55681=AXIS2_PLACEMENT_3D ( 'NONE', #46059, #28449, #10861 ) ;
#55683=VERTEX_POINT ( 'NONE', #20816 ) ;
#55685=DIRECTION ( 'NONE',  ( 0.007781995580012663651, -3.146120232559066537E-19, -0.9999697198139514409 ) ) ;
#55686=ORIENTED_EDGE ( 'NONE', *, *, #50118, .T. ) ;
#55688=ORIENTED_EDGE ( 'NONE', *, *, #20893, .F. ) ;
#55689=DIRECTION ( 'NONE',  ( 0.5449076811759707706, 0.6444004775717708799, -0.5364919789714476250 ) ) ;
#55690=VECTOR ( 'NONE', #5285, 999.9999999999998863 ) ;
#55691=EDGE_LOOP ( 'NONE', ( #4642, #33917, #11725, #15217 ) ) ;
#55692=AXIS2_PLACEMENT_3D ( 'NONE', #39899, #5537, #35365 ) ;
#55693=ORIENTED_EDGE ( 'NONE', *, *, #40781, .F. ) ;
#55694=ORIENTED_EDGE ( 'NONE', *, *, #10290, .F. ) ;
#55695=DIRECTION ( 'NONE',  ( -0.005002170337468016433, -0.7660444431189770143, 0.6427681459581293666 ) ) ;
#55696=FACE_OUTER_BOUND ( 'NONE', #33919, .T. ) ;
#55697=CARTESIAN_POINT ( 'NONE',  ( -16.89925026227929195, -0.1191753592594197858, 13.49466922669627422 ) ) ;
#55698=DIRECTION ( 'NONE',  ( 0.005961354470445682716, -0.6427876096865404731, -0.7660212471507180654 ) ) ;
#55699=ORIENTED_EDGE ( 'NONE', *, *, #16651, .F. ) ;
#55700=ORIENTED_EDGE ( 'NONE', *, *, #40424, .F. ) ;
#55701=VECTOR ( 'NONE', #37475, 1000.000000000000000 ) ;
#55702=ORIENTED_EDGE ( 'NONE', *, *, #34231, .T. ) ;
#55703=PLANE ( 'NONE',  #43141 ) ;
#55704=DIRECTION ( 'NONE',  ( 0.9999697198139515519, 0.000000000000000000, 0.007781995580013368816 ) ) ;
#55705=ORIENTED_EDGE ( 'NONE', *, *, #48767, .T. ) ;
#55706=CARTESIAN_POINT ( 'NONE',  ( -25.20278734466900517, 0.000000000000000000, 6.670939612111840944 ) ) ;
#55707=ORIENTED_EDGE ( 'NONE', *, *, #20093, .F. ) ;
#55708=AXIS2_PLACEMENT_3D ( 'NONE', #24431, #14808, #32135 ) ;
#55709=DIRECTION ( 'NONE',  ( -0.7660212471507179544, -0.6427876096865405842, -0.005961354470445141482 ) ) ;
#55710=FACE_OUTER_BOUND ( 'NONE', #41188, .T. ) ;
#55711=ADVANCED_FACE ( 'NONE', ( #43274 ), #8911, .F. ) ;
#55712=EDGE_CURVE ( 'NONE', #36408, #37378, #38421, .T. ) ;
#55713=ORIENTED_EDGE ( 'NONE', *, *, #39732, .F. ) ;
#55714=CARTESIAN_POINT ( 'NONE',  ( -19.60990026154428278, 0.000000000000000000, 4.498472333781370125 ) ) ;
#55715=EDGE_LOOP ( 'NONE', ( #55544, #8937, #47732, #22512 ) ) ;
#55716=EDGE_CURVE ( 'NONE', #55542, #53648, #16274, .T. ) ;
#55717=LINE ( 'NONE', #51475, #33642 ) ;
#55719=VECTOR ( 'NONE', #26531, 1000.000000000000227 ) ;
#55720=ORIENTED_EDGE ( 'NONE', *, *, #19225, .F. ) ;
#55721=DIRECTION ( 'NONE',  ( -0.005961354470445682716, -0.6427876096865404731, 0.7660212471507180654 ) ) ;
#55722=DIRECTION ( 'NONE',  ( 0.6427681459581294776, -0.7660444431189769032, 0.005002170337467562802 ) ) ;
#55723=PLANE ( 'NONE',  #26044 ) ;
#55724=AXIS2_PLACEMENT_3D ( 'NONE', #35447, #8801, #22418 ) ;
#55725=PLANE ( 'NONE',  #50931 ) ;
#55726=VERTEX_POINT ( 'NONE', #50905 ) ;
#55727=VECTOR ( 'NONE', #45806, 1000.000000000000000 ) ;
#55728=CARTESIAN_POINT ( 'NONE',  ( -14.01975593143325050, 3.200641362704010451, 2.025563831507627643 ) ) ;
#55729=FACE_OUTER_BOUND ( 'NONE', #19100, .T. ) ;
#55730=CARTESIAN_POINT ( 'NONE',  ( -17.26532721389163072, 0.000000000000000000, 13.67648636611514590 ) ) ;
#55731=LINE ( 'NONE', #47794, #6766 ) ;
#55732=LINE ( 'NONE', #16848, #17960 ) ;
#55734=AXIS2_PLACEMENT_3D ( 'NONE', #19663, #40409, #27327 ) ;
#55735=VECTOR ( 'NONE', #54765, 1000.000000000000227 ) ;
#55736=PLANE ( 'NONE',  #17665 ) ;
#55737=ORIENTED_EDGE ( 'NONE', *, *, #38058, .T. ) ;
#55738=CARTESIAN_POINT ( 'NONE',  ( -23.33693525117809386, 0.000000000000000000, 5.746789908705562944 ) ) ;
#55739=CARTESIAN_POINT ( 'NONE',  ( -10.37421533196711465, -0.1191753592594197858, 10.96012406864405975 ) ) ;
#55740=ADVANCED_FACE ( 'NONE', ( #30488 ), #38729, .F. ) ;
#55741=FACE_OUTER_BOUND ( 'NONE', #38358, .T. ) ;
#55742=VERTEX_POINT ( 'NONE', #46657 ) ;
#55743=LINE ( 'NONE', #51751, #45865 ) ;
#55744=ORIENTED_EDGE ( 'NONE', *, *, #4568, .T. ) ;
#55746=CARTESIAN_POINT ( 'NONE',  ( -15.13495153988577968, 0.000000000000000000, 12.76973526769478084 ) ) ;
#55747=ADVANCED_FACE ( 'NONE', ( #7781 ), #55449, .F. ) ;
#55748=DIRECTION ( 'NONE',  ( 0.9999697198139515519, 0.000000000000000000, 0.007781995580013368816 ) ) ;
#55749=ADVANCED_FACE ( 'NONE', ( #29657 ), #46956, .F. ) ;
#55751=VECTOR ( 'NONE', #34444, 1000.000000000000227 ) ;
#55752=ORIENTED_EDGE ( 'NONE', *, *, #17742, .F. ) ;
#55753=ORIENTED_EDGE ( 'NONE', *, *, #33495, .F. ) ;
#55754=VECTOR ( 'NONE', #11971, 1000.000000000000227 ) ;
#55756=PLANE ( 'NONE',  #22235 ) ;
#55757=DIRECTION ( 'NONE',  ( 0.9999697198139515519, 0.000000000000000000, 0.007781995580013368816 ) ) ;
#55758=VECTOR ( 'NONE', #20466, 999.9999999999998863 ) ;
#55759=CARTESIAN_POINT ( 'NONE',  ( -9.385817463643999048, -0.1191753592594190225, 3.370039272672538999 ) ) ;
#55760=CARTESIAN_POINT ( 'NONE',  ( -15.02722544478543831, -4.565544526780662693, 10.01185279549585516 ) ) ;
#55761=DIRECTION ( 'NONE',  ( 0.9999697198139515519, 0.000000000000000000, 0.007781995580013368816 ) ) ;
#55762=AXIS2_PLACEMENT_3D ( 'NONE', #46272, #46023, #41485 ) ;
#55763=EDGE_LOOP ( 'NONE', ( #9447, #53500, #15418, #38080 ) ) ;
#55764=CARTESIAN_POINT ( 'NONE',  ( -17.74404816805336793, 0.000000000000000000, 3.574322630375089460 ) ) ;
#55765=CARTESIAN_POINT ( 'NONE',  ( -29.86274838104827367, -0.1191753592594197858, 8.381332038739175871 ) ) ;
#55766=VECTOR ( 'NONE', #23648, 999.9999999999998863 ) ;
#55767=VECTOR ( 'NONE', #47203, 1000.000000000000227 ) ;
#55768=VERTEX_POINT ( 'NONE', #56041 ) ;
#55769=VECTOR ( 'NONE', #1949, 1000.000000000000227 ) ;
#55770=VECTOR ( 'NONE', #21201, 999.9999999999998863 ) ;
#55771=CARTESIAN_POINT ( 'NONE',  ( -11.81265117289410504, 0.000000000000000000, 3.820488189513650656 ) ) ;
#55772=CARTESIAN_POINT ( 'NONE',  ( -13.90996791376045927, 4.657758921906511418, 9.928600946358965729 ) ) ;
#55773=DIRECTION ( 'NONE',  ( 0.5449076811759707706, 0.6444004775717708799, -0.5364919789714476250 ) ) ;
#55774=AXIS2_PLACEMENT_3D ( 'NONE', #48897, #31590, #44351 ) ;
#55775=EDGE_LOOP ( 'NONE', ( #9378, #11732, #13400, #8729 ) ) ;
#55776=FACE_OUTER_BOUND ( 'NONE', #44802, .T. ) ;
#55777=ORIENTED_EDGE ( 'NONE', *, *, #24669, .T. ) ;
#55778=VECTOR ( 'NONE', #42363, 999.9999999999998863 ) ;
#55779=ORIENTED_EDGE ( 'NONE', *, *, #15764, .T. ) ;
#55780=VECTOR ( 'NONE', #703, 1000.000000000000114 ) ;
#55781=ORIENTED_EDGE ( 'NONE', *, *, #41430, .T. ) ;
#55782=ORIENTED_EDGE ( 'NONE', *, *, #22506, .T. ) ;
#55783=CARTESIAN_POINT ( 'NONE',  ( 2.072287782118878319, 0.000000000000000000, -2.950529333540147015 ) ) ;
#55784=ORIENTED_EDGE ( 'NONE', *, *, #4761, .T. ) ;
#55786=ADVANCED_FACE ( 'NONE', ( #17135 ), #51504, .F. ) ;
#55787=ORIENTED_EDGE ( 'NONE', *, *, #48333, .F. ) ;
#55788=DIRECTION ( 'NONE',  ( 0.005002170337468016433, -0.7660444431189770143, -0.6427681459581293666 ) ) ;
#55789=ORIENTED_EDGE ( 'NONE', *, *, #29237, .T. ) ;
#55791=EDGE_CURVE ( 'NONE', #8005, #6902, #48059, .T. ) ;
#55792=EDGE_CURVE ( 'NONE', #33095, #8533, #22520, .T. ) ;
#55793=AXIS2_PLACEMENT_3D ( 'NONE', #14904, #40482, #6129 ) ;
#55795=VECTOR ( 'NONE', #54430, 999.9999999999998863 ) ;
#55796=CARTESIAN_POINT ( 'NONE',  ( -21.06406398147228032, -2.946525016555659793, 4.969309331428991783 ) ) ;
#55797=CARTESIAN_POINT ( 'NONE',  ( -17.11715711133786400, -5.375054281893161701, 12.15219664891527351 ) ) ;
#55798=DIRECTION ( 'NONE',  ( 0.9999697198139515519, 0.000000000000000000, 0.007781995580013368816 ) ) ;
#55799=CARTESIAN_POINT ( 'NONE',  ( -18.67775241435682432, 0.000000000000000000, 4.136394454059623804 ) ) ;
#55800=VECTOR ( 'NONE', #17456, 1000.000000000000227 ) ;
#55801=ORIENTED_EDGE ( 'NONE', *, *, #6827, .T. ) ;
#55802=ORIENTED_EDGE ( 'NONE', *, *, #43525, .T. ) ;
#55803=CARTESIAN_POINT ( 'NONE',  ( -13.21937573182777115, 0.000000000000000000, 5.456195026535657355 ) ) ;
#55804=FACE_OUTER_BOUND ( 'NONE', #23187, .T. ) ;
#55805=AXIS2_PLACEMENT_3D ( 'NONE', #49374, #10490, #45128 ) ;
#55807=CARTESIAN_POINT ( 'NONE',  ( -11.70701794508347682, -0.6798977022406563764, 2.345163033079200599 ) ) ;
#55808=AXIS2_PLACEMENT_3D ( 'NONE', #19320, #882, #53971 ) ;
#55809=VECTOR ( 'NONE', #34000, 1000.000000000000227 ) ;
#55811=LINE ( 'NONE', #35351, #40337 ) ;
#55812=PLANE ( 'NONE',  #2365 ) ;
#55813=ORIENTED_EDGE ( 'NONE', *, *, #16285, .F. ) ;
#55814=LINE ( 'NONE', #16621, #31081 ) ;
#55816=ORIENTED_EDGE ( 'NONE', *, *, #50328, .T. ) ;
#55817=AXIS2_PLACEMENT_3D ( 'NONE', #28082, #28651, #11609 ) ;
#55818=PLANE ( 'NONE',  #20711 ) ;
#55819=LINE ( 'NONE', #4147, #5196 ) ;
#55820=AXIS2_PLACEMENT_3D ( 'NONE', #41534, #32182, #2615 ) ;
#55821=DIRECTION ( 'NONE',  ( 0.007781995580012663651, 0.000000000000000000, -0.9999697198139515519 ) ) ;
#55822=ADVANCED_FACE ( 'NONE', ( #5746 ), #52597, .F. ) ;
#55823=DIRECTION ( 'NONE',  ( 0.007781995580012662783, 0.000000000000000000, -0.9999697198139514409 ) ) ;
#55824=VECTOR ( 'NONE', #13715, 1000.000000000000227 ) ;
#55825=EDGE_LOOP ( 'NONE', ( #29270, #19142, #14257, #43313 ) ) ;
#55826=AXIS2_PLACEMENT_3D ( 'NONE', #54334, #7468, #29338 ) ;
#55827=ADVANCED_FACE ( 'NONE', ( #5463 ), #908, .F. ) ;
#55828=ORIENTED_EDGE ( 'NONE', *, *, #44957, .T. ) ;
#55830=DIRECTION ( 'NONE',  ( 0.6427681459581294776, -0.7660444431189769032, 0.005002170337467562802 ) ) ;
#55831=LINE ( 'NONE', #16941, #5237 ) ;
#55832=PLANE ( 'NONE',  #46387 ) ;
#55833=EDGE_CURVE ( 'NONE', #35388, #37328, #35559, .T. ) ;
#55834=DIRECTION ( 'NONE',  ( 0.007781995580012663651, -3.146120232559066537E-19, -0.9999697198139514409 ) ) ;
#55836=CARTESIAN_POINT ( 'NONE',  ( -1.086233639165236964, 0.000000000000000000, -2.796443541562362078 ) ) ;
#55837=VECTOR ( 'NONE', #360, 1000.000000000000227 ) ;
#55838=LINE ( 'NONE', #8405, #38654 ) ;
#55840=VECTOR ( 'NONE', #39026, 1000.000000000000227 ) ;
#55841=PLANE ( 'NONE',  #35640 ) ;
#55842=EDGE_LOOP ( 'NONE', ( #40782, #3256, #37243, #5362 ) ) ;
#55843=CARTESIAN_POINT ( 'NONE',  ( -13.22799789234362500, 0.000000000000000000, 6.564124136308949531 ) ) ;
#55844=VECTOR ( 'NONE', #13558, 1000.000000000000227 ) ;
#55845=EDGE_LOOP ( 'NONE', ( #16434, #4471, #17167 ) ) ;
#55846=AXIS2_PLACEMENT_3D ( 'NONE', #22450, #18155, #1101 ) ;
#55847=VERTEX_POINT ( 'NONE', #4622 ) ;
#55848=EDGE_CURVE ( 'NONE', #3085, #20285, #22776, .T. ) ;
#55849=VERTEX_POINT ( 'NONE', #9441 ) ;
#55850=VECTOR ( 'NONE', #41683, 1000.000000000000227 ) ;
#55851=ORIENTED_EDGE ( 'NONE', *, *, #29003, .T. ) ;
#55852=AXIS2_PLACEMENT_3D ( 'NONE', #25924, #50882, #3486 ) ;
#55853=ORIENTED_EDGE ( 'NONE', *, *, #16541, .T. ) ;
#55854=ORIENTED_EDGE ( 'NONE', *, *, #12613, .F. ) ;
#55855=PLANE ( 'NONE',  #15922 ) ;
#55856=VECTOR ( 'NONE', #38190, 999.9999999999998863 ) ;
#55857=DIRECTION ( 'NONE',  ( -0.6427681459581293666, -0.7660444431189770143, -0.005002170337467561935 ) ) ;
#55858=EDGE_CURVE ( 'NONE', #866, #42669, #13983, .T. ) ;
#55859=CARTESIAN_POINT ( 'NONE',  ( -19.35468857659533626, 0.1245042932765041271, 4.195977723824240613 ) ) ;
#55860=VECTOR ( 'NONE', #20559, 1000.000000000000227 ) ;
#55861=VECTOR ( 'NONE', #9331, 1000.000000000000000 ) ;
#55862=ORIENTED_EDGE ( 'NONE', *, *, #49306, .F. ) ;
#55864=CARTESIAN_POINT ( 'NONE',  ( -19.53399721238895026, -0.1191753592594167188, 7.353716559204084291 ) ) ;
#55865=ORIENTED_EDGE ( 'NONE', *, *, #31623, .F. ) ;
#55866=DIRECTION ( 'NONE',  ( -0.005002170337468016433, -0.7660444431189770143, 0.6427681459581293666 ) ) ;
#55867=VERTEX_POINT ( 'NONE', #9748 ) ;
#55868=EDGE_CURVE ( 'NONE', #5924, #5706, #31309, .T. ) ;
#55869=ADVANCED_FACE ( 'NONE', ( #53184 ), #4908, .F. ) ;
#55870=VECTOR ( 'NONE', #40891, 1000.000000000000000 ) ;
#55871=VECTOR ( 'NONE', #9602, 1000.000000000000227 ) ;
#55872=CARTESIAN_POINT ( 'NONE',  ( -16.27914457187915431, 0.000000000000000000, 6.371053393753911109 ) ) ;
#55873=PLANE ( 'NONE',  #21937 ) ;
#55874=FACE_OUTER_BOUND ( 'NONE', #47853, .T. ) ;
#55875=VERTEX_POINT ( 'NONE', #48638 ) ;
#55876=DIRECTION ( 'NONE',  ( -0.8531650599175527594, 0.4028455766673922356, 0.3313982828793700652 ) ) ;
#55878=DIRECTION ( 'NONE',  ( 0.7660212471507180654, -0.6427876096865404731, 0.005961354470445141482 ) ) ;
#55879=CARTESIAN_POINT ( 'NONE',  ( -29.86274838104827367, -0.1191753592594197858, 8.381332038739175871 ) ) ;
#55880=VECTOR ( 'NONE', #857, 999.9999999999998863 ) ;
#55881=ADVANCED_FACE ( 'NONE', ( #10003 ), #35031, .F. ) ;
#55882=DIRECTION ( 'NONE',  ( 0.007781995580012663651, -3.146120232559066537E-19, -0.9999697198139514409 ) ) ;
#55883=LINE ( 'NONE', #3360, #31327 ) ;
#55884=LINE ( 'NONE', #42532, #32917 ) ;
#55885=CARTESIAN_POINT ( 'NONE',  ( -15.86710544311044302, 0.000000000000000000, 13.13336954653252953 ) ) ;
#55886=CARTESIAN_POINT ( 'NONE',  ( -21.47341775636118655, -0.1191753592594197858, 5.122631121243466090 ) ) ;
#55888=ORIENTED_EDGE ( 'NONE', *, *, #6967, .T. ) ;
#55889=DIRECTION ( 'NONE',  ( 0.9999697198139515519, 0.000000000000000000, 0.007781995580013368816 ) ) ;
#55890=ORIENTED_EDGE ( 'NONE', *, *, #39078, .F. ) ;
#55891=VECTOR ( 'NONE', #6938, 1000.000000000000114 ) ;
#55892=LINE ( 'NONE', #25492, #38341 ) ;
#55893=DIRECTION ( 'NONE',  ( 0.6427681459581294776, -0.7660444431189769032, 0.005002170337467562802 ) ) ;
#55894=VECTOR ( 'NONE', #29067, 999.9999999999998863 ) ;
#55895=LINE ( 'NONE', #8769, #48988 ) ;
#55896=FACE_OUTER_BOUND ( 'NONE', #25089, .T. ) ;
#55897=LINE ( 'NONE', #43112, #35891 ) ;
#55898=VECTOR ( 'NONE', #1676, 1000.000000000000000 ) ;
#55899=DIRECTION ( 'NONE',  ( 0.7660212471507180654, -0.6427876096865404731, 0.005961354470445141482 ) ) ;
#55901=PLANE ( 'NONE',  #1205 ) ;
#55902=DIRECTION ( 'NONE',  ( 0.9999697198139515519, 0.000000000000000000, 0.007781995580013368816 ) ) ;
#55903=LINE ( 'NONE', #29498, #18205 ) ;
#55904=VECTOR ( 'NONE', #27248, 1000.000000000000227 ) ;
#55905=VECTOR ( 'NONE', #55798, 999.9999999999998863 ) ;
#55906=DIRECTION ( 'NONE',  ( -0.2426528472758542054, 0.7422098413412800966, -0.6246952433987894571 ) ) ;
#55907=EDGE_CURVE ( 'NONE', #34831, #30960, #27311, .T. ) ;
#55908=FACE_OUTER_BOUND ( 'NONE', #44290, .T. ) ;
#55909=PLANE ( 'NONE',  #40425 ) ;
#55910=CARTESIAN_POINT ( 'NONE',  ( -14.04655669958127362, -0.1191753592594190225, 5.180428671281267050 ) ) ;
#55911=ORIENTED_EDGE ( 'NONE', *, *, #37915, .T. ) ;
#55912=VECTOR ( 'NONE', #29148, 1000.000000000000000 ) ;
#55913=VECTOR ( 'NONE', #52875, 999.9999999999998863 ) ;
#55914=CARTESIAN_POINT ( 'NONE',  ( -13.69993929531127641, 0.000000000000000000, 7.499121575019257691 ) ) ;
#55915=DIRECTION ( 'NONE',  ( 0.000000000000000000, -0.000000000000000000, -1.000000000000000000 ) ) ;
#55916=ORIENTED_EDGE ( 'NONE', *, *, #2961, .F. ) ;
#55917=ORIENTED_EDGE ( 'NONE', *, *, #26061, .F. ) ;
#55918=LINE ( 'NONE', #41985, #17415 ) ;
#55919=EDGE_CURVE ( 'NONE', #21299, #48957, #21932, .T. ) ;
#55920=ORIENTED_EDGE ( 'NONE', *, *, #12607, .F. ) ;
#55921=EDGE_CURVE ( 'NONE', #15829, #21263, #26472, .T. ) ;
#55922=ADVANCED_FACE ( 'NONE', ( #34712 ), #43782, .F. ) ;
#55923=VECTOR ( 'NONE', #8076, 999.9999999999998863 ) ;
#55924=ORIENTED_EDGE ( 'NONE', *, *, #43917, .F. ) ;
#55925=ORIENTED_EDGE ( 'NONE', *, *, #46747, .F. ) ;
#55926=ORIENTED_EDGE ( 'NONE', *, *, #3850, .F. ) ;
#55927=PLANE ( 'NONE',  #23030 ) ;
#55928=VERTEX_POINT ( 'NONE', #4361 ) ;
#55929=LINE ( 'NONE', #34908, #8787 ) ;
#55931=LINE ( 'NONE', #29531, #19442 ) ;
#55932=ADVANCED_FACE ( 'NONE', ( #30752 ), #52029, .F. ) ;
#55933=VECTOR ( 'NONE', #2106, 999.9999999999998863 ) ;
#55934=ORIENTED_EDGE ( 'NONE', *, *, #25472, .F. ) ;
#55935=ORIENTED_EDGE ( 'NONE', *, *, #16918, .F. ) ;
#55936=EDGE_CURVE ( 'NONE', #47379, #18119, #22224, .T. ) ;
#55939=PLANE ( 'NONE',  #41763 ) ;
#55940=EDGE_LOOP ( 'NONE', ( #6641, #30359, #10090, #52561 ) ) ;
#55941=CARTESIAN_POINT ( 'NONE',  ( -14.20280369269832832, 0.000000000000000000, 12.40765738797303719 ) ) ;
#55942=LINE ( 'NONE', #3672, #10517 ) ;
#55943=EDGE_LOOP ( 'NONE', ( #17315, #8727, #49506, #19106 ) ) ;
#55944=DIRECTION ( 'NONE',  ( -0.5449076811759708816, 0.6444004775717707689, 0.5364919789714475140 ) ) ;
#55945=EDGE_CURVE ( 'NONE', #27546, #30961, #8052, .T. ) ;
#55946=ORIENTED_EDGE ( 'NONE', *, *, #959, .F. ) ;
#55948=LINE ( 'NONE', #4803, #45463 ) ;
#55949=EDGE_CURVE ( 'NONE', #39505, #34282, #47205, .T. ) ;
#55950=DIRECTION ( 'NONE',  ( -0.9999697198139514409, -0.000000000000000000, -0.007781995580013368816 ) ) ;
#55951=VECTOR ( 'NONE', #31238, 1000.000000000000000 ) ;
#55952=ORIENTED_EDGE ( 'NONE', *, *, #38894, .T. ) ;
#55954=PLANE ( 'NONE',  #55572 ) ;
#55955=DIRECTION ( 'NONE',  ( 0.5364919789714477361, 0.6444004775717706579, 0.5449076811759711036 ) ) ;
#55956=DIRECTION ( 'NONE',  ( 0.9999697198139515519, 0.000000000000000000, 0.007781995580013368816 ) ) ;
#55957=ORIENTED_EDGE ( 'NONE', *, *, #41119, .T. ) ;
#55958=CARTESIAN_POINT ( 'NONE',  ( -10.74029228357944987, 0.000000000000000000, 11.14194120806293320 ) ) ;
#55959=FACE_OUTER_BOUND ( 'NONE', #24470, .T. ) ;
#55960=CARTESIAN_POINT ( 'NONE',  ( -11.16370825400592359, 0.000000000000000000, 5.841524775981462803 ) ) ;
#55961=CARTESIAN_POINT ( 'NONE',  ( 2.072287782118878319, 0.000000000000000000, -2.950529333540147015 ) ) ;
#55962=DIRECTION ( 'NONE',  ( 0.005961354470445682716, -0.6427876096865404731, -0.7660212471507180654 ) ) ;
#55963=FACE_OUTER_BOUND ( 'NONE', #13353, .T. ) ;
#55964=LINE ( 'NONE', #20471, #29802 ) ;
#55965=AXIS2_PLACEMENT_3D ( 'NONE', #9408, #43490, #4589 ) ;
#55966=PLANE ( 'NONE',  #25694 ) ;
#55967=CARTESIAN_POINT ( 'NONE',  ( -16.39560766533424641, -0.1191753592594190225, 8.486136441761102489 ) ) ;
#55968=ORIENTED_EDGE ( 'NONE', *, *, #22720, .F. ) ;
#55969=CARTESIAN_POINT ( 'NONE',  ( -17.74404816805336793, 0.000000000000000000, 3.574322630375089460 ) ) ;
#55970=VERTEX_POINT ( 'NONE', #48 ) ;
#55971=DIRECTION ( 'NONE',  ( 0.005002170337468016433, -0.7660444431189770143, -0.6427681459581293666 ) ) ;
#55972=DIRECTION ( 'NONE',  ( 0.9999697198139515519, 0.000000000000000000, 0.007781995580013368816 ) ) ;
#55973=VECTOR ( 'NONE', #19085, 1000.000000000000000 ) ;
#55975=EDGE_CURVE ( 'NONE', #13455, #48904, #648, .T. ) ;
#55976=CARTESIAN_POINT ( 'NONE',  ( -16.43317633868556626, -0.1191753592594197858, 13.31363028683540151 ) ) ;
#55977=DIRECTION ( 'NONE',  ( 0.005961354470445682716, -0.6427876096865404731, -0.7660212471507180654 ) ) ;
#55978=VERTEX_POINT ( 'NONE', #4063 ) ;
#55980=ORIENTED_EDGE ( 'NONE', *, *, #16669, .F. ) ;
#55981=DIRECTION ( 'NONE',  ( -0.005961354470445682716, -0.6427876096865404731, 0.7660212471507180654 ) ) ;
#55982=LINE ( 'NONE', #25883, #19553 ) ;
#55983=VERTEX_POINT ( 'NONE', #30177 ) ;
#55984=ADVANCED_FACE ( 'NONE', ( #21389 ), #38722, .F. ) ;
#55985=ADVANCED_FACE ( 'NONE', ( #13436 ), #56033, .F. ) ;
#55986=DIRECTION ( 'NONE',  ( -0.6427681459581293666, -0.7660444431189770143, -0.005002170337467561935 ) ) ;
#55987=VECTOR ( 'NONE', #23207, 1000.000000000000227 ) ;
#55988=ORIENTED_EDGE ( 'NONE', *, *, #15275, .F. ) ;
#55989=DIRECTION ( 'NONE',  ( 0.6427681459581294776, -0.7660444431189769032, 0.005002170337467562802 ) ) ;
#55990=ORIENTED_EDGE ( 'NONE', *, *, #33992, .T. ) ;
#55991=DIRECTION ( 'NONE',  ( 0.005961354470445682716, -0.6427876096865404731, -0.7660212471507180654 ) ) ;
#55992=EDGE_CURVE ( 'NONE', #50299, #15763, #52589, .T. ) ;
#55993=VERTEX_POINT ( 'NONE', #17124 ) ;
#55994=VERTEX_POINT ( 'NONE', #48052 ) ;
#55995=ORIENTED_EDGE ( 'NONE', *, *, #42466, .F. ) ;
#55996=LINE ( 'NONE', #21634, #8479 ) ;
#55997=PLANE ( 'NONE',  #17817 ) ;
#55998=DIRECTION ( 'NONE',  ( -0.5449076811759708816, 0.6444004775717707689, 0.5364919789714475140 ) ) ;
#56000=EDGE_CURVE ( 'NONE', #51035, #25453, #21925, .T. ) ;
#56001=ORIENTED_EDGE ( 'NONE', *, *, #55248, .T. ) ;
#56002=ORIENTED_EDGE ( 'NONE', *, *, #13346, .F. ) ;
#56003=ADVANCED_FACE ( 'NONE', ( #16852 ), #34182, .F. ) ;
#56004=ORIENTED_EDGE ( 'NONE', *, *, #438, .F. ) ;
#56005=LINE ( 'NONE', #11706, #16826 ) ;
#56006=CARTESIAN_POINT ( 'NONE',  ( -10.74029228357944987, 0.000000000000000000, 11.14194120806293320 ) ) ;
#56007=EDGE_CURVE ( 'NONE', #26046, #7889, #51494, .T. ) ;
#56008=ORIENTED_EDGE ( 'NONE', *, *, #3302, .T. ) ;
#56009=DIRECTION ( 'NONE',  ( 0.005961354470445682716, -0.6427876096865404731, -0.7660212471507180654 ) ) ;
#56011=PLANE ( 'NONE',  #45943 ) ;
#56012=DIRECTION ( 'NONE',  ( 0.007781995580012663651, -3.146120232559066537E-19, -0.9999697198139514409 ) ) ;
#56013=ADVANCED_FACE ( 'NONE', ( #51746 ), #39253, .F. ) ;
#56014=ORIENTED_EDGE ( 'NONE', *, *, #43556, .T. ) ;
#56015=LINE ( 'NONE', #9411, #48555 ) ;
#56016=ORIENTED_EDGE ( 'NONE', *, *, #10159, .F. ) ;
#56018=DIRECTION ( 'NONE',  ( 0.005002170337468016433, -0.7660444431189770143, -0.6427681459581293666 ) ) ;
#56019=LINE ( 'NONE', #33573, #11201 ) ;
#56020=ORIENTED_EDGE ( 'NONE', *, *, #41719, .F. ) ;
#56021=DIRECTION ( 'NONE',  ( 0.007781995580012663651, -3.146120232559066537E-19, -0.9999697198139514409 ) ) ;
#56022=CARTESIAN_POINT ( 'NONE',  ( -10.37421533196711465, -0.1191753592594197858, 10.96012406864405975 ) ) ;
#56023=DIRECTION ( 'NONE',  ( 0.007781995580012663651, -3.146120232559066537E-19, -0.9999697198139514409 ) ) ;
#56025=VECTOR ( 'NONE', #2301, 999.9999999999998863 ) ;
#56026=CARTESIAN_POINT ( 'NONE',  ( -16.97058086006208555, 0.000000000000000000, 9.810323505063820448 ) ) ;
#56028=PLANE ( 'NONE',  #34942 ) ;
#56029=DIRECTION ( 'NONE',  ( 0.5449076811759707706, 0.6444004775717708799, -0.5364919789714476250 ) ) ;
#56030=DIRECTION ( 'NONE',  ( 0.007781995580012663651, 0.000000000000000000, -0.9999697198139515519 ) ) ;
#56032=ORIENTED_EDGE ( 'NONE', *, *, #19554, .T. ) ;
#56033=PLANE ( 'NONE',  #21651 ) ;
#56035=CARTESIAN_POINT ( 'NONE',  ( -21.47263955680318404, 0.000000000000000000, 5.022634149262071190 ) ) ;
#56036=VERTEX_POINT ( 'NONE', #21669 ) ;
#56037=FACE_OUTER_BOUND ( 'NONE', #9044, .T. ) ;
#56038=DIRECTION ( 'NONE',  ( 0.9999697198139515519, 0.000000000000000000, 0.007781995580013368816 ) ) ;
#56039=VERTEX_POINT ( 'NONE', #17683 ) ;
#56040=ADVANCED_FACE ( 'NONE', ( #15113 ), #31302, .F. ) ;
#56041=CARTESIAN_POINT ( 'NONE',  ( -16.94952351969359583, 0.000000000000000000, 7.104500489385426221 ) ) ;
#56042=CARTESIAN_POINT ( 'NONE',  ( -20.51565478868101167, 0.9340140483890049250, 6.383174327787997981 ) ) ;
#56043=EDGE_CURVE ( 'NONE', #33095, #48860, #36138, .T. ) ;
#56044=CARTESIAN_POINT ( 'NONE',  ( -19.12962290826653700, 0.000000000000000000, 14.40064212555863854 ) ) ;
#56046=ORIENTED_EDGE ( 'NONE', *, *, #54416, .T. ) ;
#56047=ORIENTED_EDGE ( 'NONE', *, *, #17503, .T. ) ;
#56048=DIRECTION ( 'NONE',  ( 0.007781995580012662783, 0.000000000000000000, -0.9999697198139514409 ) ) ;
#56049=DIRECTION ( 'NONE',  ( 0.000000000000000000, -1.000000000000000000, 0.000000000000000000 ) ) ;
#56050=DIRECTION ( 'NONE',  ( -0.6427681459581293666, -0.7660444431189770143, -0.005002170337467561935 ) ) ;
#56051=ADVANCED_FACE ( 'NONE', ( #10276 ), #36387, .F. ) ;
#56052=EDGE_CURVE ( 'NONE', #47466, #51306, #6305, .T. ) ;
#56053=EDGE_CURVE ( 'NONE', #26718, #47865, #18817, .T. ) ;
#56054=FACE_OUTER_BOUND ( 'NONE', #9487, .T. ) ;
#56055=PLANE ( 'NONE',  #1068 ) ;
#56056=LINE ( 'NONE', #47225, #23114 ) ;
#56057=EDGE_LOOP ( 'NONE', ( #13274, #407, #2119, #40942 ) ) ;
#56058=EDGE_CURVE ( 'NONE', #29102, #24902, #53701, .T. ) ;
#56059=FACE_OUTER_BOUND ( 'NONE', #8505, .T. ) ;
#56061=ORIENTED_EDGE ( 'NONE', *, *, #3906, .T. ) ;
#56062=DIRECTION ( 'NONE',  ( -0.005002170337468016433, -0.7660444431189770143, 0.6427681459581293666 ) ) ;
#56063=CARTESIAN_POINT ( 'NONE',  ( -5.316183009807136095, -7.201772371889491708, 5.283359595007837584 ) ) ;
#56064=CARTESIAN_POINT ( 'NONE',  ( -17.83139810946674686, -0.1191753592594197858, 13.85674710641801788 ) ) ;
#56065=ORIENTED_EDGE ( 'NONE', *, *, #38087, .F. ) ;
#56066=AXIS2_PLACEMENT_3D ( 'NONE', #26271, #34793, #34505 ) ;
#56067=DIRECTION ( 'NONE',  ( -0.005961354470445682716, -0.6427876096865404731, 0.7660212471507180654 ) ) ;
#56068=ORIENTED_EDGE ( 'NONE', *, *, #54262, .T. ) ;
#56069=EDGE_CURVE ( 'NONE', #16370, #693, #48901, .T. ) ;
#56070=ADVANCED_FACE ( 'NONE', ( #9996 ), #27046, .F. ) ;
#56071=ORIENTED_EDGE ( 'NONE', *, *, #42633, .F. ) ;
#56072=ORIENTED_EDGE ( 'NONE', *, *, #6930, .T. ) ;
#56074=EDGE_CURVE ( 'NONE', #31761, #40362, #5455, .T. ) ;
#56075=ORIENTED_EDGE ( 'NONE', *, *, #49199, .T. ) ;
#56076=DIRECTION ( 'NONE',  ( 0.5364919789714477361, 0.6444004775717706579, 0.5449076811759711036 ) ) ;
#56078=VERTEX_POINT ( 'NONE', #53439 ) ;
#56081=VERTEX_POINT ( 'NONE', #40383 ) ;
#56082=LINE ( 'NONE', #17168, #22284 ) ;
#56084=PLANE ( 'NONE',  #33885 ) ;
#56085=ORIENTED_EDGE ( 'NONE', *, *, #28799, .T. ) ;
#56086=EDGE_CURVE ( 'NONE', #16370, #3478, #9432, .T. ) ;
#56087=CARTESIAN_POINT ( 'NONE',  ( 1.086233639165236964, 0.000000000000000000, 2.796443541562362078 ) ) ;
#56088=CARTESIAN_POINT ( 'NONE',  ( -19.25833773637261004, 0.000000000000000000, 5.239872414256555366 ) ) ;
#56089=CARTESIAN_POINT ( 'NONE',  ( -11.40636015113596180, 0.000000000000000000, 11.32142374880780089 ) ) ;
#56090=LINE ( 'NONE', #55497, #48652 ) ;
#56091=CARTESIAN_POINT ( 'NONE',  ( -24.27063949748155380, 0.000000000000000000, 6.308861732390097288 ) ) ;
#56092=ORIENTED_EDGE ( 'NONE', *, *, #46138, .F. ) ;
#56093=ORIENTED_EDGE ( 'NONE', *, *, #21708, .T. ) ;
#56094=DIRECTION ( 'NONE',  ( 0.007781995580012662783, 0.000000000000000000, -0.9999697198139514409 ) ) ;
#56095=CARTESIAN_POINT ( 'NONE',  ( -19.81966461146206981, -0.3560938001956550081, 4.964973137040187723 ) ) ;
#56096=PLANE ( 'NONE',  #24242 ) ;
#56097=CARTESIAN_POINT ( 'NONE',  ( -13.59916412377187811, -0.1191753592594181482, 7.399902802595862639 ) ) ;
#56098=CARTESIAN_POINT ( 'NONE',  ( -12.09806905913797515, 3.686347215771511365, 1.263618829885089667 ) ) ;
#56099=CARTESIAN_POINT ( 'NONE',  ( 2.072287782118878319, 0.000000000000000000, -2.950529333540147015 ) ) ;
#56100=VERTEX_POINT ( 'NONE', #53176 ) ;
#56101=CARTESIAN_POINT ( 'NONE',  ( 2.072287782118878319, 0.000000000000000000, -2.950529333540147015 ) ) ;
#56102=CARTESIAN_POINT ( 'NONE',  ( -25.20278734466900517, 0.000000000000000000, 6.670939612111840944 ) ) ;
#56103=ORIENTED_EDGE ( 'NONE', *, *, #10998, .T. ) ;
#56104=VECTOR ( 'NONE', #31007, 1000.000000000000227 ) ;
#56105=LINE ( 'NONE', #47276, #27037 ) ;
#56106=DIRECTION ( 'NONE',  ( -0.7660212471507179544, -0.6427876096865405842, -0.005961354470445141482 ) ) ;
#56107=CARTESIAN_POINT ( 'NONE',  ( -22.40634380310664397, 0.000000000000000000, 5.584705972946605534 ) ) ;
#56108=CARTESIAN_POINT ( 'NONE',  ( -19.53292050415603498, 0.000000000000000000, 6.515057770672818549 ) ) ;
#56109=VERTEX_POINT ( 'NONE', #19342 ) ;
#56110=ORIENTED_EDGE ( 'NONE', *, *, #30823, .T. ) ;
#56111=CARTESIAN_POINT ( 'NONE',  ( -20.54049170961573267, 0.000000000000000000, 4.660556269540326646 ) ) ;
#56112=DIRECTION ( 'NONE',  ( 0.000000000000000000, -0.000000000000000000, -1.000000000000000000 ) ) ;
#56113=CARTESIAN_POINT ( 'NONE',  ( -16.35537091626028428, -0.1191753592594193140, 3.315800596152395308 ) ) ;
#56114=EDGE_CURVE ( 'NONE', #23328, #7205, #9740, .T. ) ;
#56115=LINE ( 'NONE', #51830, #55476 ) ;
#56116=LINE ( 'NONE', #29736, #398 ) ;
#56117=ADVANCED_FACE ( 'NONE', ( #44925 ), #35552, .F. ) ;
#56118=LINE ( 'NONE', #16640, #21923 ) ;
#56119=DIRECTION ( 'NONE',  ( -0.6427681459581293666, -0.7660444431189770143, -0.005002170337467561935 ) ) ;
#56120=EDGE_LOOP ( 'NONE', ( #43432, #10681, #24534, #12947 ) ) ;
#56121=DIRECTION ( 'NONE',  ( 0.000000000000000000, -0.000000000000000000, -1.000000000000000000 ) ) ;
#56122=DIRECTION ( 'NONE',  ( 0.9999697198139515519, 0.000000000000000000, 0.007781995580013368816 ) ) ;
#56123=ORIENTED_EDGE ( 'NONE', *, *, #24359, .T. ) ;
#56124=PLANE ( 'NONE',  #12935 ) ;
#56125=ORIENTED_EDGE ( 'NONE', *, *, #24889, .F. ) ;
#56126=CARTESIAN_POINT ( 'NONE',  ( -11.61684893682587827, 0.000000000000000000, 4.360670051182396811 ) ) ;
#56127=ORIENTED_EDGE ( 'NONE', *, *, #1345, .T. ) ;
#56128=ORIENTED_EDGE ( 'NONE', *, *, #28402, .F. ) ;
#56129=ORIENTED_EDGE ( 'NONE', *, *, #52288, .F. ) ;
#56130=ORIENTED_EDGE ( 'NONE', *, *, #55345, .F. ) ;
#56131=ORIENTED_EDGE ( 'NONE', *, *, #55532, .F. ) ;
#56132=ORIENTED_EDGE ( 'NONE', *, *, #18901, .F. ) ;
#56133=CARTESIAN_POINT ( 'NONE',  ( -10.69775370277556092, 0.000000000000000000, 5.675824928454496821 ) ) ;
#56134=FACE_OUTER_BOUND ( 'NONE', #1022, .T. ) ;
#56135=CARTESIAN_POINT ( 'NONE',  ( -10.42293219026540996, 0.000000000000000000, 4.369961387370421058 ) ) ;
#56136=STYLED_ITEM ( 'NONE', ( #53637 ), #29299 ) ;
#56137=ORIENTED_EDGE ( 'NONE', *, *, #21404, .F. ) ;
#56138=LINE ( 'NONE', #17508, #24948 ) ;
#56139=ORIENTED_EDGE ( 'NONE', *, *, #27128, .T. ) ;
#56140=CARTESIAN_POINT ( 'NONE',  ( -16.51037944162269966, 0.6102101463440037232, 4.295971995366294927 ) ) ;
#56141=EDGE_LOOP ( 'NONE', ( #6985, #15679, #2498, #20960 ) ) ;
#56142=EDGE_CURVE ( 'NONE', #41467, #608, #901, .T. ) ;
#56143=LINE ( 'NONE', #12698, #30314 ) ;
#56144=ADVANCED_FACE ( 'NONE', ( #52862 ), #26759, .F. ) ;
#56145=LINE ( 'NONE', #51017, #8322 ) ;
#56146=DIRECTION ( 'NONE',  ( -0.005961354470445682716, -0.6427876096865404731, 0.7660212471507180654 ) ) ;
#56147=EDGE_CURVE ( 'NONE', #48933, #17177, #13971, .T. ) ;
#56148=ORIENTED_EDGE ( 'NONE', *, *, #26345, .F. ) ;
#56149=PLANE ( 'NONE',  #1973 ) ;
#56150=ORIENTED_EDGE ( 'NONE', *, *, #4786, .T. ) ;
#56151=DIRECTION ( 'NONE',  ( 0.000000000000000000, -0.000000000000000000, -1.000000000000000000 ) ) ;
#56152=ADVANCED_FACE ( 'NONE', ( #3436 ), #15365, .F. ) ;
#56153=CARTESIAN_POINT ( 'NONE',  ( -23.33693525117809386, 0.000000000000000000, 5.746789908705562944 ) ) ;
#56154=PLANE ( 'NONE',  #39624 ) ;
#56155=CARTESIAN_POINT ( 'NONE',  ( -29.86197018149027116, 0.000000000000000000, 8.281335066757780083 ) ) ;
#56156=PLANE ( 'NONE',  #49215 ) ;
#56157=LINE ( 'NONE', #42792, #21271 ) ;
#56158=CARTESIAN_POINT ( 'NONE',  ( -8.473787990993519870, -0.1191753592594177180, 5.593129315755143161 ) ) ;
#56159=CARTESIAN_POINT ( 'NONE',  ( 2.072287782118878319, 0.000000000000000000, -2.950529333540147015 ) ) ;
#56160=ORIENTED_EDGE ( 'NONE', *, *, #54835, .F. ) ;
#56161=LINE ( 'NONE', #12459, #25651 ) ;
#56162=ORIENTED_EDGE ( 'NONE', *, *, #36194, .F. ) ;
#56164=DIRECTION ( 'NONE',  ( -0.5449076811759708816, 0.6444004775717707689, 0.5364919789714475140 ) ) ;
#56165=CARTESIAN_POINT ( 'NONE',  ( -19.60912206198628027, -0.1191753592594197858, 4.398475361799976113 ) ) ;
#56166=LINE ( 'NONE', #17250, #42613 ) ;
#56167=LINE ( 'NONE', #16700, #10461 ) ;
#56168=DIRECTION ( 'NONE',  ( -0.6427681459581293666, -0.7660444431189770143, -0.005002170337467561935 ) ) ;
#56170=CARTESIAN_POINT ( 'NONE',  ( -16.81190032086591302, 0.000000000000000000, 3.212244750653343583 ) ) ;
#56171=EDGE_LOOP ( 'NONE', ( #33831, #42990, #47195, #10667 ) ) ;
#56172=PLANE ( 'NONE',  #41144 ) ;
#56173=CARTESIAN_POINT ( 'NONE',  ( -8.975993561185934055, -0.1191753592594197858, 10.41700724906143982 ) ) ;
#56174=EDGE_CURVE ( 'NONE', #21327, #32882, #20476, .T. ) ;
#56175=FACE_OUTER_BOUND ( 'NONE', #26314, .T. ) ;
#56176=EDGE_CURVE ( 'NONE', #41524, #51537, #33271, .T. ) ;
#56177=DIRECTION ( 'NONE',  ( 0.007781995580012662783, 0.000000000000000000, -0.9999697198139514409 ) ) ;
#56178=PLANE ( 'NONE',  #12109 ) ;
#56179=FACE_OUTER_BOUND ( 'NONE', #48265, .T. ) ;
#56180=EDGE_CURVE ( 'NONE', #32502, #54118, #16209, .T. ) ;
#56181=ADVANCED_FACE ( 'NONE', ( #7693 ), #37809, .F. ) ;
#56182=CARTESIAN_POINT ( 'NONE',  ( -11.63852371047886081, 0.000000000000000000, 7.145831917949534429 ) ) ;
#56183=ORIENTED_EDGE ( 'NONE', *, *, #39376, .T. ) ;
#56185=LINE ( 'NONE', #39134, #42307 ) ;
#56186=ORIENTED_EDGE ( 'NONE', *, *, #39169, .F. ) ;
#56187=EDGE_LOOP ( 'NONE', ( #43018, #12400, #6135, #43970 ) ) ;
#56188=CARTESIAN_POINT ( 'NONE',  ( -18.88751676427461490, -0.3560938001956550081, 4.602895257318442290 ) ) ;
#56189=VERTEX_POINT ( 'NONE', #54822 ) ;
#56190=EDGE_CURVE ( 'NONE', #42734, #9627, #49738, .T. ) ;
#56191=ORIENTED_EDGE ( 'NONE', *, *, #7425, .F. ) ;
#56192=ORIENTED_EDGE ( 'NONE', *, *, #36965, .T. ) ;
#56193=ORIENTED_EDGE ( 'NONE', *, *, #33083, .T. ) ;
#56194=ORIENTED_EDGE ( 'NONE', *, *, #34815, .F. ) ;
#56195=LINE ( 'NONE', #228, #35091 ) ;
#56196=DIRECTION ( 'NONE',  ( -0.5449076811759708816, 0.6444004775717707689, 0.5364919789714475140 ) ) ;
#56197=VERTEX_POINT ( 'NONE', #33527 ) ;
#56199=ORIENTED_EDGE ( 'NONE', *, *, #16105, .F. ) ;
#56200=PLANE ( 'NONE',  #20996 ) ;
#56202=ORIENTED_EDGE ( 'NONE', *, *, #45937, .F. ) ;
#56203=LINE ( 'NONE', #34612, #53793 ) ;
#56204=ORIENTED_EDGE ( 'NONE', *, *, #23773, .T. ) ;
#56205=DIRECTION ( 'NONE',  ( -0.005002170337468016433, -0.7660444431189770143, 0.6427681459581293666 ) ) ;
#56206=EDGE_CURVE ( 'NONE', #43321, #37328, #50835, .T. ) ;
#56207=CARTESIAN_POINT ( 'NONE',  ( -27.06630483948590893, -0.1191753592594197858, 7.295098399573937797 ) ) ;
#56208=ORIENTED_EDGE ( 'NONE', *, *, #34691, .T. ) ;
#56209=CARTESIAN_POINT ( 'NONE',  ( -11.13939817157438306, 0.000000000000000000, 2.717731390624371635 ) ) ;
#56210=CARTESIAN_POINT ( 'NONE',  ( -11.59960461579418300, 0.000000000000000000, 2.144811831635808463 ) ) ;
#56211=DIRECTION ( 'NONE',  ( -0.005002170337468016433, -0.7660444431189770143, 0.6427681459581293666 ) ) ;
#56212=FACE_OUTER_BOUND ( 'NONE', #54753, .T. ) ;
#56213=ORIENTED_EDGE ( 'NONE', *, *, #18140, .T. ) ;
#56214=ADVANCED_FACE ( 'NONE', ( #32681 ), #41748, .F. ) ;
#56215=CARTESIAN_POINT ( 'NONE',  ( -10.58976041405849422, 0.7721120973665051013, 2.261911183942312054 ) ) ;
#56216=LINE ( 'NONE', #52784, #3343 ) ;
#56218=LINE ( 'NONE', #30933, #18694 ) ;
#56219=PLANE ( 'NONE',  #9614 ) ;
#56220=ADVANCED_FACE ( 'NONE', ( #28991 ), #11931, .F. ) ;
#56221=CARTESIAN_POINT ( 'NONE',  ( -14.66752777490137483, 3.362543313726509719, 8.097193451663571295 ) ) ;
#56222=DIRECTION ( 'NONE',  ( 0.007781995580012663651, 0.000000000000000000, -0.9999697198139515519 ) ) ;
#56223=EDGE_CURVE ( 'NONE', #17816, #48176, #29260, .T. ) ;
#56224=LINE ( 'NONE', #840, #45624 ) ;
#56225=DIRECTION ( 'NONE',  ( 0.007781995580012663651, 0.000000000000000000, -0.9999697198139515519 ) ) ;
#56226=VERTEX_POINT ( 'NONE', #46575 ) ;
#56228=CARTESIAN_POINT ( 'NONE',  ( -12.33850799832341849, 0.000000000000000000, 11.68350162852954632 ) ) ;
#56229=ORIENTED_EDGE ( 'NONE', *, *, #6415, .F. ) ;
#56231=ADVANCED_FACE ( 'NONE', ( #24183 ), #19902, .F. ) ;
#56232=DIRECTION ( 'NONE',  ( -0.6427681459581293666, -0.7660444431189770143, -0.005002170337467561935 ) ) ;
#56233=EDGE_CURVE ( 'NONE', #24571, #19740, #42344, .T. ) ;
#56234=DIRECTION ( 'NONE',  ( 0.005961354470445682716, -0.6427876096865404731, -0.7660212471507180654 ) ) ;
#56235=CARTESIAN_POINT ( 'NONE',  ( -19.07977982133608208, 0.000000000000000000, 7.995912495471886317 ) ) ;
ENDSEC;
END-ISO-10303-21;
